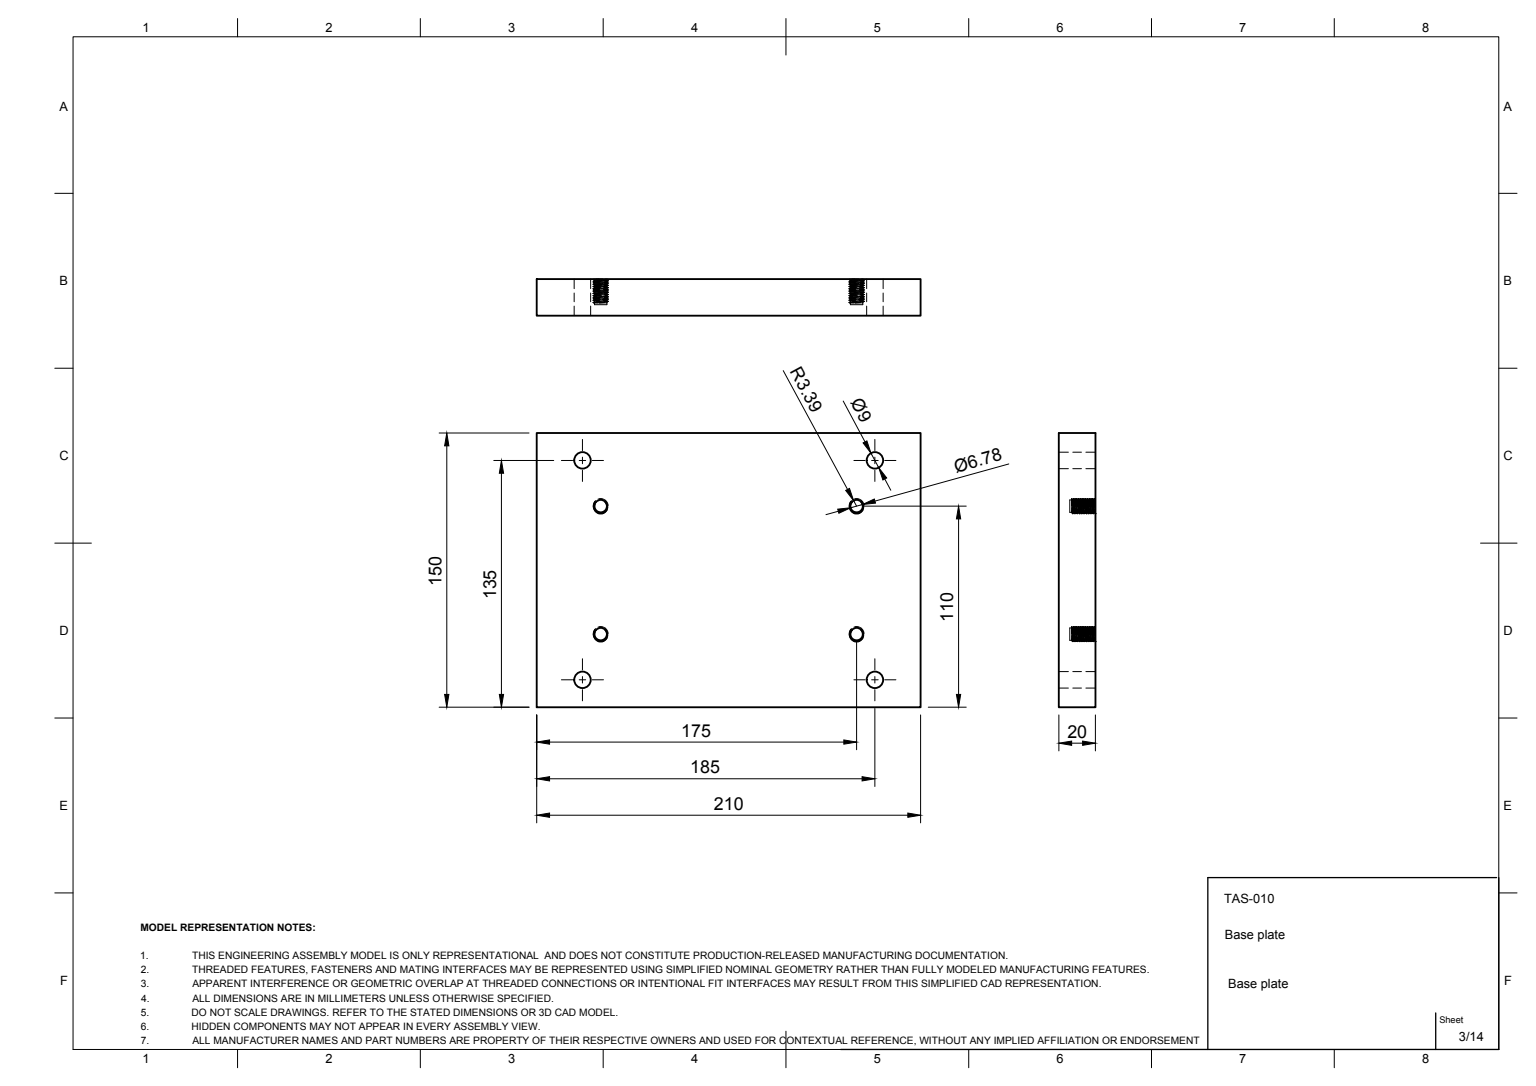
ISO-10303-21;
HEADER;
/* Generated by software containing ST-Developer
 * from STEP Tools, Inc. (www.steptools.com) 
 */

FILE_DESCRIPTION(
/* description */ (
'Independent keyed-quill tailstock, native coupled50mm slider andM16x2
 feed screw, conical dead center, bronze sleeves/thrust washers, cross
-pinned handwheel and bolted guide key. Custom center taper; no standa
rd taper compatibility, machine-bed compatibility or load rating assig
ned.'),
/* implementation_level */ '2;1');

FILE_NAME(
/* name */ 'Base plate.step',
/* time_stamp */ '2026-11-14T07:17:36-08:00',
/* author */ (''),
/* organization */ (''),
/* preprocessor_version */ 'ST-DEVELOPER v20.2',
/* originating_system */ 'Autodesk Translation Framework v15.17.0.0',
/* authorisation */ '');

FILE_SCHEMA (('AUTOMOTIVE_DESIGN { 1 0 10303 214 3 1 1 }'));
ENDSEC;

DATA;
#10=MECHANICAL_DESIGN_GEOMETRIC_PRESENTATION_REPRESENTATION('',(#153),#289387);
#119=SHAPE_REPRESENTATION_RELATIONSHIP('SRR','None',#289454,#136);
#136=ADVANCED_BREP_SHAPE_REPRESENTATION('',(#170),#289370);
#153=STYLED_ITEM('',(#289548),#170);
#170=MANIFOLD_SOLID_BREP('Body1',#16841);
#187=FACE_BOUND('',#1186,.T.);
#188=FACE_BOUND('',#1187,.T.);
#189=FACE_BOUND('',#1188,.T.);
#190=FACE_BOUND('',#1189,.T.);
#191=FACE_BOUND('',#1190,.T.);
#192=FACE_BOUND('',#1191,.T.);
#193=FACE_BOUND('',#1192,.T.);
#194=FACE_BOUND('',#1193,.T.);
#195=FACE_BOUND('',#1195,.T.);
#196=FACE_BOUND('',#1196,.T.);
#197=FACE_BOUND('',#1197,.T.);
#198=FACE_BOUND('',#1198,.T.);
#273=B_SPLINE_SURFACE_WITH_KNOTS('',3,3,((#55782,#55783,#55784,#55785,#55786,
#55787,#55788,#55789,#55790,#55791,#55792,#55793,#55794,#55795,#55796,#55797,
#55798,#55799,#55800,#55801,#55802,#55803,#55804,#55805,#55806,#55807,#55808,
#55809,#55810,#55811,#55812,#55813,#55814,#55815,#55816,#55817,#55818,#55819,
#55820,#55821,#55822,#55823,#55824,#55825,#55826,#55827,#55828,#55829,#55830,
#55831,#55832,#55833,#55834,#55835,#55836,#55837,#55838,#55839,#55840,#55841,
#55842,#55843,#55844,#55845,#55846,#55847,#55848,#55849,#55850,#55851,#55852),
(#55853,#55854,#55855,#55856,#55857,#55858,#55859,#55860,#55861,#55862,
#55863,#55864,#55865,#55866,#55867,#55868,#55869,#55870,#55871,#55872,#55873,
#55874,#55875,#55876,#55877,#55878,#55879,#55880,#55881,#55882,#55883,#55884,
#55885,#55886,#55887,#55888,#55889,#55890,#55891,#55892,#55893,#55894,#55895,
#55896,#55897,#55898,#55899,#55900,#55901,#55902,#55903,#55904,#55905,#55906,
#55907,#55908,#55909,#55910,#55911,#55912,#55913,#55914,#55915,#55916,#55917,
#55918,#55919,#55920,#55921,#55922,#55923),(#55924,#55925,#55926,#55927,
#55928,#55929,#55930,#55931,#55932,#55933,#55934,#55935,#55936,#55937,#55938,
#55939,#55940,#55941,#55942,#55943,#55944,#55945,#55946,#55947,#55948,#55949,
#55950,#55951,#55952,#55953,#55954,#55955,#55956,#55957,#55958,#55959,#55960,
#55961,#55962,#55963,#55964,#55965,#55966,#55967,#55968,#55969,#55970,#55971,
#55972,#55973,#55974,#55975,#55976,#55977,#55978,#55979,#55980,#55981,#55982,
#55983,#55984,#55985,#55986,#55987,#55988,#55989,#55990,#55991,#55992,#55993,
#55994),(#55995,#55996,#55997,#55998,#55999,#56000,#56001,#56002,#56003,
#56004,#56005,#56006,#56007,#56008,#56009,#56010,#56011,#56012,#56013,#56014,
#56015,#56016,#56017,#56018,#56019,#56020,#56021,#56022,#56023,#56024,#56025,
#56026,#56027,#56028,#56029,#56030,#56031,#56032,#56033,#56034,#56035,#56036,
#56037,#56038,#56039,#56040,#56041,#56042,#56043,#56044,#56045,#56046,#56047,
#56048,#56049,#56050,#56051,#56052,#56053,#56054,#56055,#56056,#56057,#56058,
#56059,#56060,#56061,#56062,#56063,#56064,#56065)),.UNSPECIFIED.,.F.,.F.,
 .F.,(4,4),(4,1,1,1,1,1,1,1,1,1,1,1,1,1,1,1,1,1,1,1,1,1,1,1,1,1,1,1,1,1,
1,1,1,1,1,1,1,1,1,1,1,1,1,1,1,1,1,1,1,1,1,1,1,1,1,1,1,1,1,1,1,1,1,1,1,1,
1,1,4),(-0.000703873626500094,0.0807256881124021),(11.8568339491899,12.8481671993964,
13.8387965759765,14.8294259525565,15.8200553291365,16.8106847057165,17.8013140822966,
18.7919434588766,19.7825728354566,20.7732022120367,21.7638315886167,22.7544609651967,
23.7450903417767,24.7357197183568,25.7263490949368,26.7169784715168,27.7076078480968,
28.6982372246769,29.6888666012569,30.6794959778369,31.6701253544169,32.660754730997,
33.651384107577,34.642013484157,35.6326428607371,36.6232722373171,37.6139016138971,
38.6045309904771,39.5951603670572,40.5857897436372,41.5764191202172,42.5670484967972,
43.5576778733773,44.5483072499573,45.5389366265373,46.5295660031174,47.5201953796974,
48.5108247562774,49.5014541328574,50.4920835094375,51.4827128860175,52.4733422625975,
53.4639716391775,54.4546010157576,55.4452303923376,56.4358597689176,57.4264891454977,
58.4171185220777,59.4077478986577,60.3983772752377,61.3890066518178,62.3796360283978,
63.3702654049778,64.3608947815578,65.3515241581379,66.3421535347179,67.3327829112979,
68.3234122878779,69.314041664458,70.304671041038,71.295300417618,72.2859297941981,
73.2765591707781,74.2671885473581,75.2578179239381,76.2484473005182,77.2390766770982,
78.2297060536782,79.2203354302583),.UNSPECIFIED.);
#274=B_SPLINE_SURFACE_WITH_KNOTS('',3,3,((#56163,#56164,#56165,#56166,#56167,
#56168,#56169,#56170,#56171,#56172,#56173,#56174,#56175,#56176,#56177,#56178,
#56179,#56180,#56181,#56182,#56183,#56184,#56185,#56186,#56187,#56188,#56189,
#56190,#56191,#56192,#56193,#56194,#56195,#56196,#56197,#56198,#56199,#56200,
#56201,#56202,#56203,#56204,#56205,#56206,#56207,#56208,#56209,#56210,#56211,
#56212,#56213,#56214,#56215,#56216,#56217,#56218,#56219,#56220,#56221,#56222,
#56223,#56224,#56225,#56226,#56227,#56228,#56229,#56230,#56231,#56232,#56233),
(#56234,#56235,#56236,#56237,#56238,#56239,#56240,#56241,#56242,#56243,
#56244,#56245,#56246,#56247,#56248,#56249,#56250,#56251,#56252,#56253,#56254,
#56255,#56256,#56257,#56258,#56259,#56260,#56261,#56262,#56263,#56264,#56265,
#56266,#56267,#56268,#56269,#56270,#56271,#56272,#56273,#56274,#56275,#56276,
#56277,#56278,#56279,#56280,#56281,#56282,#56283,#56284,#56285,#56286,#56287,
#56288,#56289,#56290,#56291,#56292,#56293,#56294,#56295,#56296,#56297,#56298,
#56299,#56300,#56301,#56302,#56303,#56304),(#56305,#56306,#56307,#56308,
#56309,#56310,#56311,#56312,#56313,#56314,#56315,#56316,#56317,#56318,#56319,
#56320,#56321,#56322,#56323,#56324,#56325,#56326,#56327,#56328,#56329,#56330,
#56331,#56332,#56333,#56334,#56335,#56336,#56337,#56338,#56339,#56340,#56341,
#56342,#56343,#56344,#56345,#56346,#56347,#56348,#56349,#56350,#56351,#56352,
#56353,#56354,#56355,#56356,#56357,#56358,#56359,#56360,#56361,#56362,#56363,
#56364,#56365,#56366,#56367,#56368,#56369,#56370,#56371,#56372,#56373,#56374,
#56375),(#56376,#56377,#56378,#56379,#56380,#56381,#56382,#56383,#56384,
#56385,#56386,#56387,#56388,#56389,#56390,#56391,#56392,#56393,#56394,#56395,
#56396,#56397,#56398,#56399,#56400,#56401,#56402,#56403,#56404,#56405,#56406,
#56407,#56408,#56409,#56410,#56411,#56412,#56413,#56414,#56415,#56416,#56417,
#56418,#56419,#56420,#56421,#56422,#56423,#56424,#56425,#56426,#56427,#56428,
#56429,#56430,#56431,#56432,#56433,#56434,#56435,#56436,#56437,#56438,#56439,
#56440,#56441,#56442,#56443,#56444,#56445,#56446)),.UNSPECIFIED.,.F.,.F.,
 .F.,(4,4),(4,1,1,1,1,1,1,1,1,1,1,1,1,1,1,1,1,1,1,1,1,1,1,1,1,1,1,1,1,1,
1,1,1,1,1,1,1,1,1,1,1,1,1,1,1,1,1,1,1,1,1,1,1,1,1,1,1,1,1,1,1,1,1,1,1,1,
1,1,4),(-0.000445042829947342,0.0809843050226073),(14.3991256467175,15.3897550232976,
16.3803843998776,17.3710137764576,18.3616431530376,19.3522725296177,20.3429019061977,
21.3335312827777,22.3241606593577,23.3147900359378,24.3054194125178,25.2960487890978,
26.2866781656778,27.2773075422579,28.2679369188379,29.2585662954179,30.249195671998,
31.239825048578,32.230454425158,33.221083801738,34.2117131783181,35.2023425548981,
36.1929719314781,37.1836013080582,38.1742306846382,39.1648600612182,40.1554894377982,
41.1461188143783,42.1367481909583,43.1273775675383,44.1180069441183,45.1086363206984,
46.0992656972784,47.0898950738584,48.0805244504384,49.0711538270185,50.0617832035985,
51.0524125801785,52.0430419567586,53.0336713333386,54.0243007099186,55.0149300864986,
56.0055594630787,56.9961888396587,57.9868182162387,58.9774475928187,59.9680769693988,
60.9587063459788,61.9493357225588,62.9399650991389,63.9305944757189,64.9212238522989,
65.9118532288789,66.902482605459,67.893111982039,68.883741358619,69.8743707351991,
70.8650001117791,71.8556294883591,72.8462588649391,73.8368882415191,74.8275176180992,
75.8181469946792,76.8087763712592,77.7994057478393,78.7900351244193,79.7806645009993,
80.7712938775793,81.7626270042512),.UNSPECIFIED.);
#275=B_SPLINE_SURFACE_WITH_KNOTS('',3,3,((#56747,#56748,#56749,#56750,#56751,
#56752,#56753,#56754,#56755,#56756,#56757,#56758,#56759,#56760,#56761,#56762,
#56763,#56764,#56765,#56766,#56767,#56768,#56769,#56770,#56771,#56772,#56773,
#56774,#56775,#56776,#56777,#56778,#56779,#56780,#56781,#56782,#56783,#56784,
#56785,#56786,#56787,#56788,#56789,#56790,#56791,#56792,#56793,#56794,#56795,
#56796,#56797,#56798,#56799,#56800,#56801,#56802,#56803,#56804,#56805,#56806,
#56807,#56808,#56809,#56810,#56811,#56812,#56813,#56814,#56815,#56816,#56817),
(#56818,#56819,#56820,#56821,#56822,#56823,#56824,#56825,#56826,#56827,
#56828,#56829,#56830,#56831,#56832,#56833,#56834,#56835,#56836,#56837,#56838,
#56839,#56840,#56841,#56842,#56843,#56844,#56845,#56846,#56847,#56848,#56849,
#56850,#56851,#56852,#56853,#56854,#56855,#56856,#56857,#56858,#56859,#56860,
#56861,#56862,#56863,#56864,#56865,#56866,#56867,#56868,#56869,#56870,#56871,
#56872,#56873,#56874,#56875,#56876,#56877,#56878,#56879,#56880,#56881,#56882,
#56883,#56884,#56885,#56886,#56887,#56888),(#56889,#56890,#56891,#56892,
#56893,#56894,#56895,#56896,#56897,#56898,#56899,#56900,#56901,#56902,#56903,
#56904,#56905,#56906,#56907,#56908,#56909,#56910,#56911,#56912,#56913,#56914,
#56915,#56916,#56917,#56918,#56919,#56920,#56921,#56922,#56923,#56924,#56925,
#56926,#56927,#56928,#56929,#56930,#56931,#56932,#56933,#56934,#56935,#56936,
#56937,#56938,#56939,#56940,#56941,#56942,#56943,#56944,#56945,#56946,#56947,
#56948,#56949,#56950,#56951,#56952,#56953,#56954,#56955,#56956,#56957,#56958,
#56959),(#56960,#56961,#56962,#56963,#56964,#56965,#56966,#56967,#56968,
#56969,#56970,#56971,#56972,#56973,#56974,#56975,#56976,#56977,#56978,#56979,
#56980,#56981,#56982,#56983,#56984,#56985,#56986,#56987,#56988,#56989,#56990,
#56991,#56992,#56993,#56994,#56995,#56996,#56997,#56998,#56999,#57000,#57001,
#57002,#57003,#57004,#57005,#57006,#57007,#57008,#57009,#57010,#57011,#57012,
#57013,#57014,#57015,#57016,#57017,#57018,#57019,#57020,#57021,#57022,#57023,
#57024,#57025,#57026,#57027,#57028,#57029,#57030)),.UNSPECIFIED.,.F.,.F.,
 .F.,(4,4),(4,1,1,1,1,1,1,1,1,1,1,1,1,1,1,1,1,1,1,1,1,1,1,1,1,1,1,1,1,1,
1,1,1,1,1,1,1,1,1,1,1,1,1,1,1,1,1,1,1,1,1,1,1,1,1,1,1,1,1,1,1,1,1,1,1,1,
1,1,4),(-0.000689732099215623,0.0807182050540442),(11.8568480907172,12.8481671993964,
13.8387965759765,14.8294259525565,15.8200553291365,16.8106847057165,17.8013140822966,
18.7919434588766,19.7825728354566,20.7732022120367,21.7638315886167,22.7544609651967,
23.7450903417767,24.7357197183568,25.7263490949368,26.7169784715168,27.7076078480968,
28.6982372246769,29.6888666012569,30.6794959778369,31.6701253544169,32.660754730997,
33.651384107577,34.642013484157,35.6326428607371,36.6232722373171,37.6139016138971,
38.6045309904771,39.5951603670572,40.5857897436372,41.5764191202172,42.5670484967972,
43.5576778733773,44.5483072499573,45.5389366265373,46.5295660031174,47.5201953796974,
48.5108247562774,49.5014541328574,50.4920835094375,51.4827128860175,52.4733422625975,
53.4639716391775,54.4546010157576,55.4452303923376,56.4358597689176,57.4264891454977,
58.4171185220777,59.4077478986577,60.3983772752377,61.3890066518178,62.3796360283978,
63.3702654049778,64.3608947815578,65.3515241581379,66.3421535347179,67.3327829112979,
68.3234122878779,69.314041664458,70.304671041038,71.295300417618,72.2859297941981,
73.2765591707781,74.2671885473581,75.2578179239381,76.2484473005182,77.2390766770982,
78.2297060536782,79.2203354302583),.UNSPECIFIED.);
#276=B_SPLINE_SURFACE_WITH_KNOTS('',3,3,((#57125,#57126,#57127,#57128,#57129,
#57130,#57131,#57132,#57133,#57134,#57135,#57136,#57137,#57138,#57139,#57140,
#57141,#57142,#57143,#57144,#57145,#57146,#57147,#57148,#57149,#57150,#57151,
#57152,#57153,#57154,#57155,#57156,#57157,#57158,#57159,#57160,#57161,#57162,
#57163,#57164,#57165,#57166,#57167,#57168,#57169,#57170,#57171,#57172,#57173,
#57174,#57175,#57176,#57177,#57178,#57179,#57180,#57181,#57182,#57183,#57184,
#57185,#57186,#57187,#57188,#57189,#57190,#57191,#57192,#57193,#57194,#57195),
(#57196,#57197,#57198,#57199,#57200,#57201,#57202,#57203,#57204,#57205,
#57206,#57207,#57208,#57209,#57210,#57211,#57212,#57213,#57214,#57215,#57216,
#57217,#57218,#57219,#57220,#57221,#57222,#57223,#57224,#57225,#57226,#57227,
#57228,#57229,#57230,#57231,#57232,#57233,#57234,#57235,#57236,#57237,#57238,
#57239,#57240,#57241,#57242,#57243,#57244,#57245,#57246,#57247,#57248,#57249,
#57250,#57251,#57252,#57253,#57254,#57255,#57256,#57257,#57258,#57259,#57260,
#57261,#57262,#57263,#57264,#57265,#57266),(#57267,#57268,#57269,#57270,
#57271,#57272,#57273,#57274,#57275,#57276,#57277,#57278,#57279,#57280,#57281,
#57282,#57283,#57284,#57285,#57286,#57287,#57288,#57289,#57290,#57291,#57292,
#57293,#57294,#57295,#57296,#57297,#57298,#57299,#57300,#57301,#57302,#57303,
#57304,#57305,#57306,#57307,#57308,#57309,#57310,#57311,#57312,#57313,#57314,
#57315,#57316,#57317,#57318,#57319,#57320,#57321,#57322,#57323,#57324,#57325,
#57326,#57327,#57328,#57329,#57330,#57331,#57332,#57333,#57334,#57335,#57336,
#57337),(#57338,#57339,#57340,#57341,#57342,#57343,#57344,#57345,#57346,
#57347,#57348,#57349,#57350,#57351,#57352,#57353,#57354,#57355,#57356,#57357,
#57358,#57359,#57360,#57361,#57362,#57363,#57364,#57365,#57366,#57367,#57368,
#57369,#57370,#57371,#57372,#57373,#57374,#57375,#57376,#57377,#57378,#57379,
#57380,#57381,#57382,#57383,#57384,#57385,#57386,#57387,#57388,#57389,#57390,
#57391,#57392,#57393,#57394,#57395,#57396,#57397,#57398,#57399,#57400,#57401,
#57402,#57403,#57404,#57405,#57406,#57407,#57408)),.UNSPECIFIED.,.F.,.F.,
 .F.,(4,4),(4,1,1,1,1,1,1,1,1,1,1,1,1,1,1,1,1,1,1,1,1,1,1,1,1,1,1,1,1,1,
1,1,1,1,1,1,1,1,1,1,1,1,1,1,1,1,1,1,1,1,1,1,1,1,1,1,1,1,1,1,1,1,1,1,1,1,
1,1,4),(-0.000437656372986427,0.0809703040897196),(14.3991256467175,15.3897550232976,
16.3803843998776,17.3710137764576,18.3616431530376,19.3522725296177,20.3429019061977,
21.3335312827777,22.3241606593577,23.3147900359378,24.3054194125178,25.2960487890978,
26.2866781656779,27.2773075422579,28.2679369188379,29.2585662954179,30.249195671998,
31.239825048578,32.230454425158,33.221083801738,34.2117131783181,35.2023425548981,
36.1929719314781,37.1836013080582,38.1742306846382,39.1648600612182,40.1554894377982,
41.1461188143783,42.1367481909583,43.1273775675383,44.1180069441183,45.1086363206984,
46.0992656972784,47.0898950738584,48.0805244504385,49.0711538270185,50.0617832035985,
51.0524125801785,52.0430419567586,53.0336713333386,54.0243007099186,55.0149300864986,
56.0055594630787,56.9961888396587,57.9868182162387,58.9774475928188,59.9680769693988,
60.9587063459788,61.9493357225588,62.9399650991389,63.9305944757189,64.9212238522989,
65.911853228879,66.902482605459,67.893111982039,68.883741358619,69.8743707351991,
70.8650001117791,71.8556294883591,72.8462588649391,73.8368882415192,74.8275176180992,
75.8181469946792,76.8087763712593,77.7994057478393,78.7900351244193,79.7806645009993,
80.7712938775794,81.7626130033183),.UNSPECIFIED.);
#277=B_SPLINE_SURFACE_WITH_KNOTS('',3,3,((#57712,#57713,#57714,#57715,#57716,
#57717,#57718,#57719,#57720,#57721,#57722,#57723,#57724,#57725,#57726,#57727,
#57728,#57729,#57730,#57731,#57732,#57733,#57734,#57735,#57736,#57737,#57738,
#57739,#57740,#57741,#57742,#57743,#57744,#57745,#57746,#57747,#57748,#57749,
#57750,#57751,#57752,#57753,#57754,#57755,#57756,#57757,#57758,#57759,#57760,
#57761,#57762,#57763,#57764,#57765,#57766,#57767,#57768,#57769,#57770,#57771,
#57772,#57773,#57774,#57775,#57776,#57777,#57778,#57779,#57780,#57781,#57782),
(#57783,#57784,#57785,#57786,#57787,#57788,#57789,#57790,#57791,#57792,
#57793,#57794,#57795,#57796,#57797,#57798,#57799,#57800,#57801,#57802,#57803,
#57804,#57805,#57806,#57807,#57808,#57809,#57810,#57811,#57812,#57813,#57814,
#57815,#57816,#57817,#57818,#57819,#57820,#57821,#57822,#57823,#57824,#57825,
#57826,#57827,#57828,#57829,#57830,#57831,#57832,#57833,#57834,#57835,#57836,
#57837,#57838,#57839,#57840,#57841,#57842,#57843,#57844,#57845,#57846,#57847,
#57848,#57849,#57850,#57851,#57852,#57853),(#57854,#57855,#57856,#57857,
#57858,#57859,#57860,#57861,#57862,#57863,#57864,#57865,#57866,#57867,#57868,
#57869,#57870,#57871,#57872,#57873,#57874,#57875,#57876,#57877,#57878,#57879,
#57880,#57881,#57882,#57883,#57884,#57885,#57886,#57887,#57888,#57889,#57890,
#57891,#57892,#57893,#57894,#57895,#57896,#57897,#57898,#57899,#57900,#57901,
#57902,#57903,#57904,#57905,#57906,#57907,#57908,#57909,#57910,#57911,#57912,
#57913,#57914,#57915,#57916,#57917,#57918,#57919,#57920,#57921,#57922,#57923,
#57924),(#57925,#57926,#57927,#57928,#57929,#57930,#57931,#57932,#57933,
#57934,#57935,#57936,#57937,#57938,#57939,#57940,#57941,#57942,#57943,#57944,
#57945,#57946,#57947,#57948,#57949,#57950,#57951,#57952,#57953,#57954,#57955,
#57956,#57957,#57958,#57959,#57960,#57961,#57962,#57963,#57964,#57965,#57966,
#57967,#57968,#57969,#57970,#57971,#57972,#57973,#57974,#57975,#57976,#57977,
#57978,#57979,#57980,#57981,#57982,#57983,#57984,#57985,#57986,#57987,#57988,
#57989,#57990,#57991,#57992,#57993,#57994,#57995)),.UNSPECIFIED.,.F.,.F.,
 .F.,(4,4),(4,1,1,1,1,1,1,1,1,1,1,1,1,1,1,1,1,1,1,1,1,1,1,1,1,1,1,1,1,1,
1,1,1,1,1,1,1,1,1,1,1,1,1,1,1,1,1,1,1,1,1,1,1,1,1,1,1,1,1,1,1,1,1,1,1,1,
1,1,4),(-0.000703899666689691,0.0807257072263232),(11.8568339231497,12.8481671993964,
13.8387965759764,14.8294259525565,15.8200553291365,16.8106847057165,17.8013140822965,
18.7919434588766,19.7825728354566,20.7732022120366,21.7638315886167,22.7544609651967,
23.7450903417767,24.7357197183567,25.7263490949368,26.7169784715168,27.7076078480968,
28.6982372246768,29.6888666012569,30.6794959778369,31.6701253544169,32.660754730997,
33.651384107577,34.642013484157,35.632642860737,36.6232722373171,37.6139016138971,
38.6045309904771,39.5951603670571,40.5857897436372,41.5764191202172,42.5670484967972,
43.5576778733773,44.5483072499573,45.5389366265373,46.5295660031173,47.5201953796974,
48.5108247562774,49.5014541328574,50.4920835094374,51.4827128860175,52.4733422625975,
53.4639716391775,54.4546010157575,55.4452303923376,56.4358597689176,57.4264891454976,
58.4171185220777,59.4077478986577,60.3983772752377,61.3890066518177,62.3796360283978,
63.3702654049778,64.3608947815578,65.3515241581378,66.3421535347179,67.3327829112979,
68.3234122878779,69.314041664458,70.304671041038,71.295300417618,72.285929794198,
73.2765591707781,74.2671885473581,75.2578179239381,76.2484473005182,77.2390766770982,
78.2297060536782,79.2203354302582),.UNSPECIFIED.);
#278=B_SPLINE_SURFACE_WITH_KNOTS('',3,3,((#58093,#58094,#58095,#58096,#58097,
#58098,#58099,#58100,#58101,#58102,#58103,#58104,#58105,#58106,#58107,#58108,
#58109,#58110,#58111,#58112,#58113,#58114,#58115,#58116,#58117,#58118,#58119,
#58120,#58121,#58122,#58123,#58124,#58125,#58126,#58127,#58128,#58129,#58130,
#58131,#58132,#58133,#58134,#58135,#58136,#58137,#58138,#58139,#58140,#58141,
#58142,#58143,#58144,#58145,#58146,#58147,#58148,#58149,#58150,#58151,#58152,
#58153,#58154,#58155,#58156,#58157,#58158,#58159,#58160,#58161,#58162,#58163),
(#58164,#58165,#58166,#58167,#58168,#58169,#58170,#58171,#58172,#58173,
#58174,#58175,#58176,#58177,#58178,#58179,#58180,#58181,#58182,#58183,#58184,
#58185,#58186,#58187,#58188,#58189,#58190,#58191,#58192,#58193,#58194,#58195,
#58196,#58197,#58198,#58199,#58200,#58201,#58202,#58203,#58204,#58205,#58206,
#58207,#58208,#58209,#58210,#58211,#58212,#58213,#58214,#58215,#58216,#58217,
#58218,#58219,#58220,#58221,#58222,#58223,#58224,#58225,#58226,#58227,#58228,
#58229,#58230,#58231,#58232,#58233,#58234),(#58235,#58236,#58237,#58238,
#58239,#58240,#58241,#58242,#58243,#58244,#58245,#58246,#58247,#58248,#58249,
#58250,#58251,#58252,#58253,#58254,#58255,#58256,#58257,#58258,#58259,#58260,
#58261,#58262,#58263,#58264,#58265,#58266,#58267,#58268,#58269,#58270,#58271,
#58272,#58273,#58274,#58275,#58276,#58277,#58278,#58279,#58280,#58281,#58282,
#58283,#58284,#58285,#58286,#58287,#58288,#58289,#58290,#58291,#58292,#58293,
#58294,#58295,#58296,#58297,#58298,#58299,#58300,#58301,#58302,#58303,#58304,
#58305),(#58306,#58307,#58308,#58309,#58310,#58311,#58312,#58313,#58314,
#58315,#58316,#58317,#58318,#58319,#58320,#58321,#58322,#58323,#58324,#58325,
#58326,#58327,#58328,#58329,#58330,#58331,#58332,#58333,#58334,#58335,#58336,
#58337,#58338,#58339,#58340,#58341,#58342,#58343,#58344,#58345,#58346,#58347,
#58348,#58349,#58350,#58351,#58352,#58353,#58354,#58355,#58356,#58357,#58358,
#58359,#58360,#58361,#58362,#58363,#58364,#58365,#58366,#58367,#58368,#58369,
#58370,#58371,#58372,#58373,#58374,#58375,#58376)),.UNSPECIFIED.,.F.,.F.,
 .F.,(4,4),(4,1,1,1,1,1,1,1,1,1,1,1,1,1,1,1,1,1,1,1,1,1,1,1,1,1,1,1,1,1,
1,1,1,1,1,1,1,1,1,1,1,1,1,1,1,1,1,1,1,1,1,1,1,1,1,1,1,1,1,1,1,1,1,1,1,1,
1,1,4),(-0.000445070994418236,0.080984343609613),(14.3991256467175,15.3897550232975,
16.3803843998776,17.3710137764576,18.3616431530376,19.3522725296176,20.3429019061977,
21.3335312827777,22.3241606593577,23.3147900359377,24.3054194125178,25.2960487890978,
26.2866781656778,27.2773075422579,28.2679369188379,29.2585662954179,30.2491956719979,
31.239825048578,32.230454425158,33.221083801738,34.211713178318,35.2023425548981,
36.1929719314781,37.1836013080581,38.1742306846382,39.1648600612182,40.1554894377982,
41.1461188143782,42.1367481909583,43.1273775675383,44.1180069441183,45.1086363206983,
46.0992656972784,47.0898950738584,48.0805244504384,49.0711538270185,50.0617832035985,
51.0524125801785,52.0430419567585,53.0336713333386,54.0243007099186,55.0149300864986,
56.0055594630786,56.9961888396587,57.9868182162387,58.9774475928187,59.9680769693988,
60.9587063459788,61.9493357225588,62.9399650991388,63.9305944757189,64.9212238522989,
65.9118532288789,66.9024826054589,67.893111982039,68.883741358619,69.874370735199,
70.8650001117791,71.8556294883591,72.8462588649391,73.8368882415191,74.8275176180992,
75.8181469946792,76.8087763712592,77.7994057478392,78.7900351244193,79.7806645009993,
80.7712938775793,81.7626270428382),.UNSPECIFIED.);
#279=B_SPLINE_SURFACE_WITH_KNOTS('',3,3,((#58677,#58678,#58679,#58680,#58681,
#58682,#58683,#58684,#58685,#58686,#58687,#58688,#58689,#58690,#58691,#58692,
#58693,#58694,#58695,#58696,#58697,#58698,#58699,#58700,#58701,#58702,#58703,
#58704,#58705,#58706,#58707,#58708,#58709,#58710,#58711,#58712,#58713,#58714,
#58715,#58716,#58717,#58718,#58719,#58720,#58721,#58722,#58723,#58724,#58725,
#58726,#58727,#58728,#58729,#58730,#58731,#58732,#58733,#58734,#58735,#58736,
#58737,#58738,#58739,#58740,#58741,#58742,#58743,#58744,#58745,#58746,#58747),
(#58748,#58749,#58750,#58751,#58752,#58753,#58754,#58755,#58756,#58757,
#58758,#58759,#58760,#58761,#58762,#58763,#58764,#58765,#58766,#58767,#58768,
#58769,#58770,#58771,#58772,#58773,#58774,#58775,#58776,#58777,#58778,#58779,
#58780,#58781,#58782,#58783,#58784,#58785,#58786,#58787,#58788,#58789,#58790,
#58791,#58792,#58793,#58794,#58795,#58796,#58797,#58798,#58799,#58800,#58801,
#58802,#58803,#58804,#58805,#58806,#58807,#58808,#58809,#58810,#58811,#58812,
#58813,#58814,#58815,#58816,#58817,#58818),(#58819,#58820,#58821,#58822,
#58823,#58824,#58825,#58826,#58827,#58828,#58829,#58830,#58831,#58832,#58833,
#58834,#58835,#58836,#58837,#58838,#58839,#58840,#58841,#58842,#58843,#58844,
#58845,#58846,#58847,#58848,#58849,#58850,#58851,#58852,#58853,#58854,#58855,
#58856,#58857,#58858,#58859,#58860,#58861,#58862,#58863,#58864,#58865,#58866,
#58867,#58868,#58869,#58870,#58871,#58872,#58873,#58874,#58875,#58876,#58877,
#58878,#58879,#58880,#58881,#58882,#58883,#58884,#58885,#58886,#58887,#58888,
#58889),(#58890,#58891,#58892,#58893,#58894,#58895,#58896,#58897,#58898,
#58899,#58900,#58901,#58902,#58903,#58904,#58905,#58906,#58907,#58908,#58909,
#58910,#58911,#58912,#58913,#58914,#58915,#58916,#58917,#58918,#58919,#58920,
#58921,#58922,#58923,#58924,#58925,#58926,#58927,#58928,#58929,#58930,#58931,
#58932,#58933,#58934,#58935,#58936,#58937,#58938,#58939,#58940,#58941,#58942,
#58943,#58944,#58945,#58946,#58947,#58948,#58949,#58950,#58951,#58952,#58953,
#58954,#58955,#58956,#58957,#58958,#58959,#58960)),.UNSPECIFIED.,.F.,.F.,
 .F.,(4,4),(4,1,1,1,1,1,1,1,1,1,1,1,1,1,1,1,1,1,1,1,1,1,1,1,1,1,1,1,1,1,
1,1,1,1,1,1,1,1,1,1,1,1,1,1,1,1,1,1,1,1,1,1,1,1,1,1,1,1,1,1,1,1,1,1,1,1,
1,1,4),(-0.00068967791227708,0.0807181852368366),(11.8568481449041,12.8481671993964,
13.8387965759765,14.8294259525565,15.8200553291365,16.8106847057165,17.8013140822966,
18.7919434588766,19.7825728354566,20.7732022120367,21.7638315886167,22.7544609651967,
23.7450903417767,24.7357197183568,25.7263490949368,26.7169784715168,27.7076078480968,
28.6982372246769,29.6888666012569,30.6794959778369,31.6701253544169,32.660754730997,
33.651384107577,34.642013484157,35.6326428607371,36.6232722373171,37.6139016138971,
38.6045309904771,39.5951603670572,40.5857897436372,41.5764191202172,42.5670484967972,
43.5576778733773,44.5483072499573,45.5389366265373,46.5295660031174,47.5201953796974,
48.5108247562774,49.5014541328574,50.4920835094375,51.4827128860175,52.4733422625975,
53.4639716391775,54.4546010157576,55.4452303923376,56.4358597689176,57.4264891454977,
58.4171185220777,59.4077478986577,60.3983772752377,61.3890066518178,62.3796360283978,
63.3702654049778,64.3608947815578,65.3515241581379,66.3421535347179,67.3327829112979,
68.3234122878779,69.314041664458,70.304671041038,71.295300417618,72.2859297941981,
73.2765591707781,74.2671885473581,75.2578179239381,76.2484473005182,77.2390766770982,
78.2297060536782,79.2203354302583),.UNSPECIFIED.);
#280=B_SPLINE_SURFACE_WITH_KNOTS('',3,3,((#59055,#59056,#59057,#59058,#59059,
#59060,#59061,#59062,#59063,#59064,#59065,#59066,#59067,#59068,#59069,#59070,
#59071,#59072,#59073,#59074,#59075,#59076,#59077,#59078,#59079,#59080,#59081,
#59082,#59083,#59084,#59085,#59086,#59087,#59088,#59089,#59090,#59091,#59092,
#59093,#59094,#59095,#59096,#59097,#59098,#59099,#59100,#59101,#59102,#59103,
#59104,#59105,#59106,#59107,#59108,#59109,#59110,#59111,#59112,#59113,#59114,
#59115,#59116,#59117,#59118,#59119,#59120,#59121,#59122,#59123,#59124,#59125),
(#59126,#59127,#59128,#59129,#59130,#59131,#59132,#59133,#59134,#59135,
#59136,#59137,#59138,#59139,#59140,#59141,#59142,#59143,#59144,#59145,#59146,
#59147,#59148,#59149,#59150,#59151,#59152,#59153,#59154,#59155,#59156,#59157,
#59158,#59159,#59160,#59161,#59162,#59163,#59164,#59165,#59166,#59167,#59168,
#59169,#59170,#59171,#59172,#59173,#59174,#59175,#59176,#59177,#59178,#59179,
#59180,#59181,#59182,#59183,#59184,#59185,#59186,#59187,#59188,#59189,#59190,
#59191,#59192,#59193,#59194,#59195,#59196),(#59197,#59198,#59199,#59200,
#59201,#59202,#59203,#59204,#59205,#59206,#59207,#59208,#59209,#59210,#59211,
#59212,#59213,#59214,#59215,#59216,#59217,#59218,#59219,#59220,#59221,#59222,
#59223,#59224,#59225,#59226,#59227,#59228,#59229,#59230,#59231,#59232,#59233,
#59234,#59235,#59236,#59237,#59238,#59239,#59240,#59241,#59242,#59243,#59244,
#59245,#59246,#59247,#59248,#59249,#59250,#59251,#59252,#59253,#59254,#59255,
#59256,#59257,#59258,#59259,#59260,#59261,#59262,#59263,#59264,#59265,#59266,
#59267),(#59268,#59269,#59270,#59271,#59272,#59273,#59274,#59275,#59276,
#59277,#59278,#59279,#59280,#59281,#59282,#59283,#59284,#59285,#59286,#59287,
#59288,#59289,#59290,#59291,#59292,#59293,#59294,#59295,#59296,#59297,#59298,
#59299,#59300,#59301,#59302,#59303,#59304,#59305,#59306,#59307,#59308,#59309,
#59310,#59311,#59312,#59313,#59314,#59315,#59316,#59317,#59318,#59319,#59320,
#59321,#59322,#59323,#59324,#59325,#59326,#59327,#59328,#59329,#59330,#59331,
#59332,#59333,#59334,#59335,#59336,#59337,#59338)),.UNSPECIFIED.,.F.,.F.,
 .F.,(4,4),(4,1,1,1,1,1,1,1,1,1,1,1,1,1,1,1,1,1,1,1,1,1,1,1,1,1,1,1,1,1,
1,1,1,1,1,1,1,1,1,1,1,1,1,1,1,1,1,1,1,1,1,1,1,1,1,1,1,1,1,1,1,1,1,1,1,1,
1,1,4),(-0.00043763828538554,0.0809702546783821),(14.3991256467175,15.3897550232976,
16.3803843998776,17.3710137764576,18.3616431530376,19.3522725296177,20.3429019061977,
21.3335312827777,22.3241606593577,23.3147900359378,24.3054194125178,25.2960487890978,
26.2866781656779,27.2773075422579,28.2679369188379,29.2585662954179,30.249195671998,
31.239825048578,32.230454425158,33.221083801738,34.2117131783181,35.2023425548981,
36.1929719314781,37.1836013080582,38.1742306846382,39.1648600612182,40.1554894377982,
41.1461188143783,42.1367481909583,43.1273775675383,44.1180069441183,45.1086363206984,
46.0992656972784,47.0898950738584,48.0805244504385,49.0711538270185,50.0617832035985,
51.0524125801785,52.0430419567586,53.0336713333386,54.0243007099186,55.0149300864986,
56.0055594630787,56.9961888396587,57.9868182162387,58.9774475928188,59.9680769693988,
60.9587063459788,61.9493357225588,62.9399650991389,63.9305944757189,64.9212238522989,
65.911853228879,66.902482605459,67.893111982039,68.883741358619,69.8743707351991,
70.8650001117791,71.8556294883591,72.8462588649391,73.8368882415192,74.8275176180992,
75.8181469946792,76.8087763712593,77.7994057478393,78.7900351244193,79.7806645009993,
80.7712938775794,81.7626129539069),.UNSPECIFIED.);
#303=PLANE('',#17160);
#304=PLANE('',#17161);
#305=PLANE('',#17162);
#306=PLANE('',#17163);
#307=PLANE('',#17164);
#308=PLANE('',#17165);
#309=PLANE('',#17166);
#310=PLANE('',#17167);
#311=PLANE('',#17180);
#312=PLANE('',#17181);
#313=PLANE('',#17182);
#314=PLANE('',#17183);
#315=PLANE('',#17184);
#316=PLANE('',#17185);
#423=FACE_OUTER_BOUND('',#1073,.T.);
#424=FACE_OUTER_BOUND('',#1074,.T.);
#425=FACE_OUTER_BOUND('',#1075,.T.);
#426=FACE_OUTER_BOUND('',#1076,.T.);
#427=FACE_OUTER_BOUND('',#1077,.T.);
#428=FACE_OUTER_BOUND('',#1078,.T.);
#429=FACE_OUTER_BOUND('',#1079,.T.);
#430=FACE_OUTER_BOUND('',#1080,.T.);
#431=FACE_OUTER_BOUND('',#1081,.T.);
#432=FACE_OUTER_BOUND('',#1082,.T.);
#433=FACE_OUTER_BOUND('',#1083,.T.);
#434=FACE_OUTER_BOUND('',#1084,.T.);
#435=FACE_OUTER_BOUND('',#1085,.T.);
#436=FACE_OUTER_BOUND('',#1086,.T.);
#437=FACE_OUTER_BOUND('',#1087,.T.);
#438=FACE_OUTER_BOUND('',#1088,.T.);
#439=FACE_OUTER_BOUND('',#1089,.T.);
#440=FACE_OUTER_BOUND('',#1090,.T.);
#441=FACE_OUTER_BOUND('',#1091,.T.);
#442=FACE_OUTER_BOUND('',#1092,.T.);
#443=FACE_OUTER_BOUND('',#1093,.T.);
#444=FACE_OUTER_BOUND('',#1094,.T.);
#445=FACE_OUTER_BOUND('',#1095,.T.);
#446=FACE_OUTER_BOUND('',#1096,.T.);
#447=FACE_OUTER_BOUND('',#1097,.T.);
#448=FACE_OUTER_BOUND('',#1098,.T.);
#449=FACE_OUTER_BOUND('',#1099,.T.);
#450=FACE_OUTER_BOUND('',#1100,.T.);
#451=FACE_OUTER_BOUND('',#1101,.T.);
#452=FACE_OUTER_BOUND('',#1102,.T.);
#453=FACE_OUTER_BOUND('',#1103,.T.);
#454=FACE_OUTER_BOUND('',#1104,.T.);
#455=FACE_OUTER_BOUND('',#1105,.T.);
#456=FACE_OUTER_BOUND('',#1106,.T.);
#457=FACE_OUTER_BOUND('',#1107,.T.);
#458=FACE_OUTER_BOUND('',#1108,.T.);
#459=FACE_OUTER_BOUND('',#1109,.T.);
#460=FACE_OUTER_BOUND('',#1110,.T.);
#461=FACE_OUTER_BOUND('',#1111,.T.);
#462=FACE_OUTER_BOUND('',#1112,.T.);
#463=FACE_OUTER_BOUND('',#1113,.T.);
#464=FACE_OUTER_BOUND('',#1114,.T.);
#465=FACE_OUTER_BOUND('',#1115,.T.);
#466=FACE_OUTER_BOUND('',#1116,.T.);
#467=FACE_OUTER_BOUND('',#1117,.T.);
#468=FACE_OUTER_BOUND('',#1118,.T.);
#469=FACE_OUTER_BOUND('',#1119,.T.);
#470=FACE_OUTER_BOUND('',#1120,.T.);
#471=FACE_OUTER_BOUND('',#1121,.T.);
#472=FACE_OUTER_BOUND('',#1122,.T.);
#473=FACE_OUTER_BOUND('',#1123,.T.);
#474=FACE_OUTER_BOUND('',#1124,.T.);
#475=FACE_OUTER_BOUND('',#1125,.T.);
#476=FACE_OUTER_BOUND('',#1126,.T.);
#477=FACE_OUTER_BOUND('',#1127,.T.);
#478=FACE_OUTER_BOUND('',#1128,.T.);
#479=FACE_OUTER_BOUND('',#1129,.T.);
#480=FACE_OUTER_BOUND('',#1130,.T.);
#481=FACE_OUTER_BOUND('',#1131,.T.);
#482=FACE_OUTER_BOUND('',#1132,.T.);
#483=FACE_OUTER_BOUND('',#1133,.T.);
#484=FACE_OUTER_BOUND('',#1134,.T.);
#485=FACE_OUTER_BOUND('',#1135,.T.);
#486=FACE_OUTER_BOUND('',#1136,.T.);
#487=FACE_OUTER_BOUND('',#1137,.T.);
#488=FACE_OUTER_BOUND('',#1138,.T.);
#489=FACE_OUTER_BOUND('',#1139,.T.);
#490=FACE_OUTER_BOUND('',#1140,.T.);
#491=FACE_OUTER_BOUND('',#1141,.T.);
#492=FACE_OUTER_BOUND('',#1142,.T.);
#493=FACE_OUTER_BOUND('',#1143,.T.);
#494=FACE_OUTER_BOUND('',#1144,.T.);
#495=FACE_OUTER_BOUND('',#1145,.T.);
#496=FACE_OUTER_BOUND('',#1146,.T.);
#497=FACE_OUTER_BOUND('',#1147,.T.);
#498=FACE_OUTER_BOUND('',#1148,.T.);
#499=FACE_OUTER_BOUND('',#1149,.T.);
#500=FACE_OUTER_BOUND('',#1150,.T.);
#501=FACE_OUTER_BOUND('',#1151,.T.);
#502=FACE_OUTER_BOUND('',#1152,.T.);
#503=FACE_OUTER_BOUND('',#1153,.T.);
#504=FACE_OUTER_BOUND('',#1154,.T.);
#505=FACE_OUTER_BOUND('',#1155,.T.);
#506=FACE_OUTER_BOUND('',#1156,.T.);
#507=FACE_OUTER_BOUND('',#1157,.T.);
#508=FACE_OUTER_BOUND('',#1158,.T.);
#509=FACE_OUTER_BOUND('',#1159,.T.);
#510=FACE_OUTER_BOUND('',#1160,.T.);
#511=FACE_OUTER_BOUND('',#1161,.T.);
#512=FACE_OUTER_BOUND('',#1162,.T.);
#513=FACE_OUTER_BOUND('',#1163,.T.);
#514=FACE_OUTER_BOUND('',#1164,.T.);
#515=FACE_OUTER_BOUND('',#1165,.T.);
#516=FACE_OUTER_BOUND('',#1166,.T.);
#517=FACE_OUTER_BOUND('',#1167,.T.);
#518=FACE_OUTER_BOUND('',#1168,.T.);
#519=FACE_OUTER_BOUND('',#1169,.T.);
#520=FACE_OUTER_BOUND('',#1170,.T.);
#521=FACE_OUTER_BOUND('',#1171,.T.);
#522=FACE_OUTER_BOUND('',#1172,.T.);
#523=FACE_OUTER_BOUND('',#1173,.T.);
#524=FACE_OUTER_BOUND('',#1174,.T.);
#525=FACE_OUTER_BOUND('',#1175,.T.);
#526=FACE_OUTER_BOUND('',#1176,.T.);
#527=FACE_OUTER_BOUND('',#1177,.T.);
#528=FACE_OUTER_BOUND('',#1178,.T.);
#529=FACE_OUTER_BOUND('',#1179,.T.);
#530=FACE_OUTER_BOUND('',#1180,.T.);
#531=FACE_OUTER_BOUND('',#1181,.T.);
#532=FACE_OUTER_BOUND('',#1182,.T.);
#533=FACE_OUTER_BOUND('',#1183,.T.);
#534=FACE_OUTER_BOUND('',#1184,.T.);
#535=FACE_OUTER_BOUND('',#1185,.T.);
#536=FACE_OUTER_BOUND('',#1194,.T.);
#1073=EDGE_LOOP('',(#10161,#10162,#10163,#10164,#10165,#10166));
#1074=EDGE_LOOP('',(#10167,#10168,#10169,#10170,#10171,#10172));
#1075=EDGE_LOOP('',(#10173,#10174,#10175,#10176,#10177,#10178));
#1076=EDGE_LOOP('',(#10179,#10180,#10181,#10182,#10183,#10184));
#1077=EDGE_LOOP('',(#10185,#10186,#10187,#10188,#10189,#10190));
#1078=EDGE_LOOP('',(#10191,#10192,#10193,#10194,#10195,#10196));
#1079=EDGE_LOOP('',(#10197,#10198,#10199,#10200,#10201,#10202));
#1080=EDGE_LOOP('',(#10203,#10204,#10205,#10206,#10207,#10208));
#1081=EDGE_LOOP('',(#10209,#10210,#10211,#10212,#10213,#10214));
#1082=EDGE_LOOP('',(#10215,#10216,#10217,#10218,#10219,#10220));
#1083=EDGE_LOOP('',(#10221,#10222,#10223,#10224,#10225,#10226,#10227,#10228));
#1084=EDGE_LOOP('',(#10229,#10230,#10231,#10232,#10233));
#1085=EDGE_LOOP('',(#10234,#10235,#10236,#10237,#10238));
#1086=EDGE_LOOP('',(#10239,#10240,#10241,#10242,#10243));
#1087=EDGE_LOOP('',(#10244,#10245,#10246,#10247,#10248));
#1088=EDGE_LOOP('',(#10249,#10250,#10251,#10252,#10253));
#1089=EDGE_LOOP('',(#10254,#10255,#10256,#10257,#10258));
#1090=EDGE_LOOP('',(#10259,#10260,#10261,#10262,#10263));
#1091=EDGE_LOOP('',(#10264,#10265,#10266,#10267,#10268));
#1092=EDGE_LOOP('',(#10269,#10270,#10271,#10272));
#1093=EDGE_LOOP('',(#10273,#10274,#10275,#10276,#10277,#10278));
#1094=EDGE_LOOP('',(#10279,#10280,#10281,#10282,#10283,#10284));
#1095=EDGE_LOOP('',(#10285,#10286,#10287,#10288,#10289,#10290));
#1096=EDGE_LOOP('',(#10291,#10292,#10293,#10294,#10295,#10296));
#1097=EDGE_LOOP('',(#10297,#10298,#10299,#10300,#10301,#10302));
#1098=EDGE_LOOP('',(#10303,#10304,#10305,#10306,#10307,#10308));
#1099=EDGE_LOOP('',(#10309,#10310,#10311,#10312,#10313,#10314));
#1100=EDGE_LOOP('',(#10315,#10316,#10317,#10318,#10319,#10320));
#1101=EDGE_LOOP('',(#10321,#10322,#10323,#10324,#10325,#10326));
#1102=EDGE_LOOP('',(#10327,#10328,#10329,#10330,#10331,#10332));
#1103=EDGE_LOOP('',(#10333,#10334,#10335,#10336,#10337,#10338,#10339,#10340));
#1104=EDGE_LOOP('',(#10341,#10342,#10343,#10344,#10345));
#1105=EDGE_LOOP('',(#10346,#10347,#10348,#10349,#10350));
#1106=EDGE_LOOP('',(#10351,#10352,#10353,#10354,#10355));
#1107=EDGE_LOOP('',(#10356,#10357,#10358,#10359,#10360));
#1108=EDGE_LOOP('',(#10361,#10362,#10363,#10364,#10365));
#1109=EDGE_LOOP('',(#10366,#10367,#10368,#10369,#10370));
#1110=EDGE_LOOP('',(#10371,#10372,#10373,#10374,#10375));
#1111=EDGE_LOOP('',(#10376,#10377,#10378,#10379,#10380));
#1112=EDGE_LOOP('',(#10381,#10382,#10383,#10384));
#1113=EDGE_LOOP('',(#10385,#10386,#10387,#10388,#10389,#10390));
#1114=EDGE_LOOP('',(#10391,#10392,#10393,#10394,#10395,#10396));
#1115=EDGE_LOOP('',(#10397,#10398,#10399,#10400,#10401,#10402));
#1116=EDGE_LOOP('',(#10403,#10404,#10405,#10406,#10407,#10408));
#1117=EDGE_LOOP('',(#10409,#10410,#10411,#10412,#10413,#10414));
#1118=EDGE_LOOP('',(#10415,#10416,#10417,#10418,#10419,#10420));
#1119=EDGE_LOOP('',(#10421,#10422,#10423,#10424,#10425,#10426));
#1120=EDGE_LOOP('',(#10427,#10428,#10429,#10430,#10431,#10432));
#1121=EDGE_LOOP('',(#10433,#10434,#10435,#10436,#10437,#10438));
#1122=EDGE_LOOP('',(#10439,#10440,#10441,#10442,#10443,#10444));
#1123=EDGE_LOOP('',(#10445,#10446,#10447,#10448,#10449,#10450,#10451,#10452));
#1124=EDGE_LOOP('',(#10453,#10454,#10455,#10456,#10457));
#1125=EDGE_LOOP('',(#10458,#10459,#10460,#10461,#10462));
#1126=EDGE_LOOP('',(#10463,#10464,#10465,#10466,#10467));
#1127=EDGE_LOOP('',(#10468,#10469,#10470,#10471,#10472));
#1128=EDGE_LOOP('',(#10473,#10474,#10475,#10476,#10477));
#1129=EDGE_LOOP('',(#10478,#10479,#10480,#10481,#10482));
#1130=EDGE_LOOP('',(#10483,#10484,#10485,#10486,#10487));
#1131=EDGE_LOOP('',(#10488,#10489,#10490,#10491,#10492));
#1132=EDGE_LOOP('',(#10493,#10494,#10495,#10496));
#1133=EDGE_LOOP('',(#10497,#10498,#10499,#10500,#10501,#10502));
#1134=EDGE_LOOP('',(#10503,#10504,#10505,#10506,#10507,#10508));
#1135=EDGE_LOOP('',(#10509,#10510,#10511,#10512,#10513,#10514));
#1136=EDGE_LOOP('',(#10515,#10516,#10517,#10518,#10519,#10520));
#1137=EDGE_LOOP('',(#10521,#10522,#10523,#10524,#10525,#10526));
#1138=EDGE_LOOP('',(#10527,#10528,#10529,#10530,#10531,#10532));
#1139=EDGE_LOOP('',(#10533,#10534,#10535,#10536,#10537,#10538));
#1140=EDGE_LOOP('',(#10539,#10540,#10541,#10542,#10543,#10544));
#1141=EDGE_LOOP('',(#10545,#10546,#10547,#10548,#10549,#10550));
#1142=EDGE_LOOP('',(#10551,#10552,#10553,#10554,#10555,#10556));
#1143=EDGE_LOOP('',(#10557,#10558,#10559,#10560,#10561,#10562,#10563,#10564));
#1144=EDGE_LOOP('',(#10565,#10566,#10567,#10568,#10569));
#1145=EDGE_LOOP('',(#10570,#10571,#10572,#10573,#10574));
#1146=EDGE_LOOP('',(#10575,#10576,#10577,#10578,#10579));
#1147=EDGE_LOOP('',(#10580,#10581,#10582,#10583,#10584));
#1148=EDGE_LOOP('',(#10585,#10586,#10587,#10588,#10589));
#1149=EDGE_LOOP('',(#10590,#10591,#10592,#10593,#10594));
#1150=EDGE_LOOP('',(#10595,#10596,#10597,#10598,#10599));
#1151=EDGE_LOOP('',(#10600,#10601,#10602,#10603,#10604));
#1152=EDGE_LOOP('',(#10605,#10606,#10607,#10608));
#1153=EDGE_LOOP('',(#10609,#10610,#10611,#10612,#10613,#10614));
#1154=EDGE_LOOP('',(#10615,#10616,#10617,#10618,#10619,#10620));
#1155=EDGE_LOOP('',(#10621,#10622,#10623,#10624,#10625,#10626));
#1156=EDGE_LOOP('',(#10627,#10628,#10629,#10630,#10631,#10632));
#1157=EDGE_LOOP('',(#10633,#10634,#10635,#10636,#10637,#10638));
#1158=EDGE_LOOP('',(#10639,#10640,#10641,#10642,#10643,#10644));
#1159=EDGE_LOOP('',(#10645,#10646,#10647,#10648,#10649,#10650));
#1160=EDGE_LOOP('',(#10651,#10652,#10653,#10654,#10655,#10656));
#1161=EDGE_LOOP('',(#10657,#10658,#10659,#10660,#10661));
#1162=EDGE_LOOP('',(#10662,#10663,#10664,#10665,#10666,#10667,#10668,#10669,
#10670,#10671,#10672,#10673,#10674,#10675,#10676,#10677,#10678,#10679,#10680,
#10681,#10682,#10683,#10684,#10685,#10686,#10687,#10688,#10689,#10690,#10691,
#10692,#10693,#10694,#10695,#10696,#10697,#10698,#10699,#10700,#10701));
#1163=EDGE_LOOP('',(#10702,#10703,#10704,#10705,#10706,#10707,#10708,#10709,
#10710,#10711,#10712,#10713,#10714,#10715,#10716,#10717,#10718,#10719,#10720,
#10721,#10722,#10723,#10724,#10725,#10726,#10727,#10728,#10729,#10730,#10731,
#10732,#10733,#10734,#10735,#10736,#10737,#10738,#10739,#10740,#10741,#10742));
#1164=EDGE_LOOP('',(#10743,#10744,#10745,#10746,#10747));
#1165=EDGE_LOOP('',(#10748,#10749,#10750,#10751,#10752,#10753,#10754,#10755,
#10756,#10757,#10758,#10759,#10760,#10761,#10762,#10763,#10764,#10765,#10766,
#10767,#10768,#10769,#10770,#10771,#10772,#10773,#10774,#10775,#10776,#10777,
#10778,#10779,#10780,#10781,#10782,#10783,#10784,#10785,#10786,#10787));
#1166=EDGE_LOOP('',(#10788,#10789,#10790,#10791,#10792,#10793,#10794,#10795,
#10796,#10797,#10798,#10799,#10800,#10801,#10802,#10803,#10804,#10805,#10806,
#10807,#10808,#10809,#10810,#10811,#10812,#10813,#10814,#10815,#10816,#10817,
#10818,#10819,#10820,#10821,#10822,#10823,#10824,#10825,#10826,#10827,#10828));
#1167=EDGE_LOOP('',(#10829,#10830,#10831,#10832,#10833));
#1168=EDGE_LOOP('',(#10834,#10835,#10836,#10837,#10838,#10839,#10840,#10841,
#10842,#10843,#10844,#10845,#10846,#10847,#10848,#10849,#10850,#10851,#10852,
#10853,#10854,#10855,#10856,#10857,#10858,#10859,#10860,#10861,#10862,#10863,
#10864,#10865,#10866,#10867,#10868,#10869,#10870,#10871,#10872,#10873));
#1169=EDGE_LOOP('',(#10874,#10875,#10876,#10877,#10878,#10879,#10880,#10881,
#10882,#10883,#10884,#10885,#10886,#10887,#10888,#10889,#10890,#10891,#10892,
#10893,#10894,#10895,#10896,#10897,#10898,#10899,#10900,#10901,#10902,#10903,
#10904,#10905,#10906,#10907,#10908,#10909,#10910,#10911,#10912,#10913,#10914));
#1170=EDGE_LOOP('',(#10915,#10916,#10917,#10918,#10919));
#1171=EDGE_LOOP('',(#10920,#10921,#10922,#10923,#10924,#10925,#10926,#10927,
#10928,#10929,#10930,#10931,#10932,#10933,#10934,#10935,#10936,#10937,#10938,
#10939,#10940,#10941,#10942,#10943,#10944,#10945,#10946,#10947,#10948,#10949,
#10950,#10951,#10952,#10953,#10954,#10955,#10956,#10957,#10958,#10959));
#1172=EDGE_LOOP('',(#10960,#10961,#10962,#10963,#10964,#10965,#10966,#10967,
#10968,#10969,#10970,#10971,#10972,#10973,#10974,#10975,#10976,#10977,#10978,
#10979,#10980,#10981,#10982,#10983,#10984,#10985,#10986,#10987,#10988,#10989,
#10990,#10991,#10992,#10993,#10994,#10995,#10996,#10997,#10998,#10999,#11000));
#1173=EDGE_LOOP('',(#11001));
#1174=EDGE_LOOP('',(#11002));
#1175=EDGE_LOOP('',(#11003));
#1176=EDGE_LOOP('',(#11004));
#1177=EDGE_LOOP('',(#11005,#11006,#11007,#11008));
#1178=EDGE_LOOP('',(#11009,#11010,#11011,#11012));
#1179=EDGE_LOOP('',(#11013,#11014,#11015,#11016));
#1180=EDGE_LOOP('',(#11017,#11018,#11019,#11020));
#1181=EDGE_LOOP('',(#11021,#11022,#11023,#11024));
#1182=EDGE_LOOP('',(#11025,#11026,#11027,#11028));
#1183=EDGE_LOOP('',(#11029,#11030,#11031,#11032));
#1184=EDGE_LOOP('',(#11033,#11034,#11035,#11036));
#1185=EDGE_LOOP('',(#11037,#11038,#11039,#11040));
#1186=EDGE_LOOP('',(#11041,#11042,#11043,#11044,#11045));
#1187=EDGE_LOOP('',(#11046,#11047,#11048,#11049,#11050));
#1188=EDGE_LOOP('',(#11051));
#1189=EDGE_LOOP('',(#11052));
#1190=EDGE_LOOP('',(#11053));
#1191=EDGE_LOOP('',(#11054));
#1192=EDGE_LOOP('',(#11055,#11056,#11057,#11058,#11059));
#1193=EDGE_LOOP('',(#11060,#11061,#11062,#11063,#11064));
#1194=EDGE_LOOP('',(#11065,#11066,#11067,#11068));
#1195=EDGE_LOOP('',(#11069));
#1196=EDGE_LOOP('',(#11070));
#1197=EDGE_LOOP('',(#11071));
#1198=EDGE_LOOP('',(#11072));
#1809=CIRCLE('',#17049,4.085);
#1810=CIRCLE('',#17059,4.085);
#1811=CIRCLE('',#17061,3.38975);
#1812=CIRCLE('',#17062,3.38975);
#1813=CIRCLE('',#17063,3.38975);
#1814=CIRCLE('',#17073,3.38975);
#1815=CIRCLE('',#17075,4.085);
#1816=CIRCLE('',#17085,4.085);
#1817=CIRCLE('',#17087,3.38975);
#1818=CIRCLE('',#17088,3.38975);
#1819=CIRCLE('',#17089,3.38975);
#1820=CIRCLE('',#17099,3.38975);
#1821=CIRCLE('',#17101,4.085);
#1822=CIRCLE('',#17111,4.085);
#1823=CIRCLE('',#17113,3.38975);
#1824=CIRCLE('',#17114,3.38975);
#1825=CIRCLE('',#17115,3.38975);
#1826=CIRCLE('',#17125,3.38975);
#1827=CIRCLE('',#17127,4.085);
#1828=CIRCLE('',#17137,4.085);
#1829=CIRCLE('',#17139,3.38975);
#1830=CIRCLE('',#17140,3.38975);
#1831=CIRCLE('',#17141,3.38975);
#1832=CIRCLE('',#17151,3.38975);
#1833=CIRCLE('',#17169,4.5);
#1834=CIRCLE('',#17170,4.5);
#1835=CIRCLE('',#17172,4.5);
#1836=CIRCLE('',#17173,4.5);
#1837=CIRCLE('',#17175,4.5);
#1838=CIRCLE('',#17176,4.5);
#1839=CIRCLE('',#17178,4.5);
#1840=CIRCLE('',#17179,4.5);
#1989=B_SPLINE_CURVE_WITH_KNOTS('',3,(#20219,#20220,#20221,#20222,#20223,
#20224,#20225,#20226,#20227,#20228,#20229,#20230,#20231,#20232,#20233,#20234,
#20235,#20236,#20237,#20238,#20239,#20240,#20241,#20242,#20243,#20244,#20245,
#20246,#20247,#20248,#20249,#20250,#20251,#20252,#20253,#20254,#20255,#20256,
#20257,#20258,#20259,#20260,#20261,#20262,#20263,#20264,#20265,#20266,#20267,
#20268,#20269,#20270,#20271,#20272,#20273,#20274,#20275,#20276,#20277,#20278,
#20279,#20280,#20281,#20282,#20283,#20284,#20285,#20286,#20287,#20288,#20289,
#20290,#20291,#20292,#20293,#20294,#20295,#20296,#20297,#20298,#20299,#20300,
#20301,#20302,#20303,#20304,#20305,#20306,#20307,#20308,#20309,#20310,#20311,
#20312,#20313,#20314,#20315,#20316,#20317,#20318,#20319,#20320,#20321,#20322,
#20323,#20324,#20325,#20326,#20327,#20328,#20329,#20330,#20331,#20332,#20333,
#20334,#20335,#20336,#20337,#20338,#20339,#20340,#20341,#20342,#20343,#20344,
#20345,#20346,#20347,#20348,#20349,#20350,#20351,#20352,#20353,#20354,#20355,
#20356,#20357,#20358,#20359,#20360,#20361,#20362,#20363),.UNSPECIFIED.,
 .F.,.F.,(4,3,3,3,3,3,3,3,3,3,3,3,3,3,3,3,3,3,3,3,3,3,3,3,3,3,3,3,3,3,3,
3,3,3,3,3,3,3,3,3,3,3,3,3,3,3,3,3,4),(74.4826090335725,74.5701170669696,
74.6575762165587,74.7450105784093,74.8324408957047,74.9198879037736,75.0074269134415,
75.0950130962531,75.1827404978775,75.2578179239381,75.3457798849692,75.4336308010057,
75.5213935021216,75.6122752269211,75.6999373474644,75.7875855687495,75.8752403914981,
75.962922316007,76.0506986045304,76.1385311052508,76.2264862371109,76.2484473005182,
76.3362730397008,76.4239894702698,76.5116195619046,76.6025517013038,76.6900866998096,
76.7776100410487,76.8651423567182,76.9527042798826,77.0403648632325,77.1280840300195,
77.2159301399878,77.2390766770982,77.3262112033101,77.4132347402867,77.5001710454324,
77.5913629214631,77.6782061467429,77.7650395395892,77.8518844243916,77.9387621301685,
78.0257467155559,78.1127937623897,78.199978776898,78.2297060536782,78.3409628987117,
78.4504383987289,78.5398161890533),.UNSPECIFIED.);
#1990=B_SPLINE_CURVE_WITH_KNOTS('',3,(#20365,#20366,#20367,#20368),
 .UNSPECIFIED.,.F.,.F.,(4,4),(78.5398163397448,79.2203354302583),
 .UNSPECIFIED.);
#1991=B_SPLINE_CURVE_WITH_KNOTS('',3,(#20372,#20373,#20374,#20375,#20376,
#20377,#20378,#20379,#20380,#20381,#20382,#20383,#20384,#20385,#20386,#20387,
#20388,#20389,#20390,#20391,#20392,#20393,#20394,#20395,#20396,#20397,#20398,
#20399,#20400,#20401,#20402,#20403,#20404,#20405,#20406,#20407,#20408,#20409,
#20410,#20411,#20412,#20413,#20414),.UNSPECIFIED.,.F.,.F.,(4,3,3,3,3,3,
3,3,3,3,3,3,3,3,4),(78.5398163399586,78.6513081866131,78.7649916437635,
78.7900351244193,78.8773287774196,78.9645133671013,79.0516124728846,79.1386521216673,
79.2256605320351,79.3126588903471,79.3996683708265,79.4867645491849,79.5739037704035,
79.6611841726733,79.7442522064414),.UNSPECIFIED.);
#1992=B_SPLINE_CURVE_WITH_KNOTS('',3,(#20415,#20416,#20417,#20418,#20419,
#20420,#20421,#20422,#20423,#20424,#20425,#20426,#20427,#20428,#20429,#20430,
#20431,#20432,#20433,#20434,#20435,#20436,#20437,#20438,#20439,#20440,#20441,
#20442,#20443,#20444,#20445,#20446,#20447,#20448,#20449,#20450,#20451,#20452,
#20453,#20454,#20455,#20456,#20457,#20458,#20459,#20460,#20461,#20462,#20463,
#20464,#20465,#20466,#20467,#20468,#20469,#20470,#20471,#20472,#20473,#20474,
#20475,#20476,#20477,#20478,#20479,#20480,#20481,#20482,#20483,#20484,#20485,
#20486,#20487,#20488,#20489,#20490,#20491,#20492,#20493,#20494,#20495,#20496,
#20497,#20498,#20499,#20500,#20501,#20502,#20503,#20504,#20505,#20506,#20507,
#20508,#20509,#20510,#20511,#20512,#20513,#20514,#20515,#20516,#20517,#20518,
#20519,#20520,#20521,#20522,#20523,#20524,#20525,#20526,#20527,#20528,#20529,
#20530,#20531,#20532,#20533,#20534,#20535,#20536,#20537,#20538,#20539,#20540,
#20541,#20542,#20543,#20544,#20545,#20546,#20547,#20548,#20549,#20550,#20551,
#20552,#20553,#20554,#20555,#20556,#20557,#20558,#20559,#20560,#20561,#20562),
 .UNSPECIFIED.,.F.,.F.,(4,3,3,3,3,3,3,3,3,3,3,3,3,3,3,3,3,3,3,3,3,3,3,3,
3,3,3,3,3,3,3,3,3,3,3,3,3,3,3,3,3,3,3,3,3,3,3,3,3,4),(74.4816274087652,
74.5692304822722,74.6568785799873,74.7446691313286,74.8275176180992,74.9153495028009,
75.0030705517629,75.0907037488907,75.1816341546142,75.2691685016855,75.3566898130181,
75.4442187278137,75.531775885644,75.6194297201104,75.7071409756895,75.7949775432399,
75.8181469946792,75.9059726632625,75.9936877005556,76.0813150947037,76.1722477542731,
76.2597768495321,76.3472931203132,76.4348172103102,76.5223697637486,76.6100193409493,
76.6977265363025,76.785559361159,76.8087763712592,76.8965156836257,76.9841440069646,
77.0716844351596,77.1626495992445,77.2500916523099,77.3375210019096,77.4249583849954,
77.5124245392801,77.5999886071116,77.6876107096917,77.7753597026586,77.7994057478393,
77.8864293135118,77.9733148215533,78.0601212169649,78.1468700360845,78.2335827631578,
78.3203031262511,78.4070268007935,78.4938095091331,78.5398163397448),
 .UNSPECIFIED.);
#1993=B_SPLINE_CURVE_WITH_KNOTS('',3,(#20568,#20569,#20570,#20571,#20572,
#20573,#20574,#20575,#20576,#20577,#20578,#20579,#20580,#20581,#20582,#20583,
#20584,#20585,#20586,#20587,#20588,#20589,#20590,#20591,#20592,#20593,#20594,
#20595,#20596,#20597,#20598,#20599,#20600,#20601,#20602,#20603,#20604,#20605,
#20606,#20607,#20608,#20609,#20610,#20611,#20612,#20613,#20614,#20615,#20616,
#20617,#20618,#20619,#20620,#20621,#20622,#20623,#20624,#20625,#20626,#20627,
#20628,#20629,#20630,#20631,#20632,#20633,#20634,#20635,#20636,#20637,#20638,
#20639,#20640,#20641,#20642,#20643,#20644,#20645,#20646,#20647,#20648,#20649,
#20650,#20651,#20652,#20653,#20654,#20655,#20656,#20657,#20658,#20659,#20660,
#20661,#20662,#20663,#20664,#20665,#20666,#20667,#20668,#20669,#20670,#20671,
#20672,#20673,#20674,#20675,#20676,#20677,#20678,#20679,#20680,#20681,#20682,
#20683,#20684,#20685,#20686,#20687,#20688,#20689,#20690,#20691,#20692,#20693,
#20694,#20695,#20696,#20697,#20698,#20699,#20700,#20701,#20702,#20703,#20704,
#20705,#20706,#20707,#20708,#20709,#20710,#20711,#20712,#20713,#20714,#20715),
 .UNSPECIFIED.,.F.,.F.,(4,3,3,3,3,3,3,3,3,3,3,3,3,3,3,3,3,3,3,3,3,3,3,3,
3,3,3,3,3,3,3,3,3,3,3,3,3,3,3,3,3,3,3,3,3,3,3,3,3,4),(68.1983639736923,
68.2861814027768,68.3234122878779,68.4112289331686,68.4989347821535,68.5865528361021,
68.6774889396466,68.7650083795268,68.8525148961314,68.9400291443268,69.0275717794539,
69.1152113763737,69.2029085438011,69.2907313485085,69.314041664458,69.4018606984001,
69.4895689314358,69.5771893620946,69.6681245719626,69.755646355417,69.8431551993798,
69.9306717562514,70.0182166788918,70.1058585206193,70.19355791062,70.2813828885069,
70.304671041038,70.3924904087626,70.4801989997041,70.5678198116346,70.6587548873826,
70.7462771072879,70.8337864071766,70.9213034388543,71.0088488545995,71.0964912138051,
71.184191136065,71.2720166636101,71.295300417618,71.3826886082915,71.4699662262677,
71.5571567686942,71.6445910516527,71.731686798181,71.8187708746251,71.9058643773058,
71.9935560410698,72.0807764618647,72.1687037471133,72.2566310323619),
 .UNSPECIFIED.);
#1994=B_SPLINE_CURVE_WITH_KNOTS('',3,(#20716,#20717,#20718,#20719,#20720,
#20721,#20722,#20723,#20724,#20725,#20726,#20727,#20728,#20729,#20730,#20731,
#20732,#20733,#20734,#20735,#20736,#20737,#20738,#20739,#20740,#20741,#20742,
#20743,#20744,#20745,#20746,#20747,#20748,#20749,#20750,#20751,#20752,#20753,
#20754,#20755,#20756,#20757,#20758,#20759,#20760,#20761,#20762,#20763,#20764,
#20765,#20766,#20767,#20768,#20769,#20770,#20771,#20772,#20773,#20774,#20775,
#20776,#20777,#20778,#20779,#20780,#20781,#20782,#20783,#20784,#20785,#20786,
#20787,#20788,#20789,#20790,#20791,#20792,#20793,#20794,#20795,#20796,#20797,
#20798,#20799,#20800),.UNSPECIFIED.,.F.,.F.,(4,3,3,3,3,3,3,3,3,3,3,3,3,
3,3,3,3,3,3,3,3,3,3,3,3,3,3,3,4),(72.2566310325652,72.2859297941981,72.3737616647174,
72.4614826996036,72.5491158827769,72.640046293777,72.7275806272787,72.8151019252055,
72.9026308267726,72.9901879715657,73.0778417933396,73.1655530364124,73.2533895918213,
73.2765591707781,73.3643847882656,73.4520997741813,73.5397271167352,73.6306597955631,
73.7181888390195,73.8057050580113,73.8932290962889,73.9807815981339,74.068431124189,
74.1561382685975,74.2439710431921,74.2671885473581,74.3549358239911,74.4425594684545,
74.4826090335725),.UNSPECIFIED.);
#1995=B_SPLINE_CURVE_WITH_KNOTS('',3,(#20802,#20803,#20804,#20805,#20806,
#20807,#20808,#20809,#20810,#20811,#20812,#20813,#20814,#20815,#20816,#20817,
#20818,#20819,#20820,#20821,#20822,#20823,#20824,#20825,#20826,#20827,#20828,
#20829,#20830,#20831,#20832,#20833,#20834,#20835,#20836,#20837,#20838,#20839,
#20840,#20841,#20842,#20843,#20844,#20845,#20846,#20847,#20848,#20849,#20850,
#20851,#20852,#20853,#20854,#20855,#20856,#20857,#20858,#20859,#20860,#20861,
#20862,#20863,#20864,#20865,#20866,#20867,#20868,#20869,#20870,#20871,#20872,
#20873,#20874,#20875,#20876,#20877,#20878,#20879,#20880,#20881,#20882,#20883),
 .UNSPECIFIED.,.F.,.F.,(4,3,3,3,3,3,3,3,3,3,3,3,3,3,3,3,3,3,3,3,3,3,3,3,
3,3,3,4),(72.2566310325652,72.3454126124315,72.4342219267591,72.5230774207564,
72.6120589912192,72.7011092478249,72.7903164501228,72.8462588649391,72.9340782408894,
73.0217868401024,73.1094076603398,73.2003427329872,73.2878649612343,73.3753742694632,
73.4628913094705,73.5504367335256,73.63807910097,73.725779031437,73.8136045670799,
73.8368882415191,73.924681465638,74.0123709321393,74.0999774797657,74.1875218796041,
74.2750311973064,74.362520405566,74.4500269116099,74.4816274087652),
 .UNSPECIFIED.);
#1996=B_SPLINE_CURVE_WITH_KNOTS('',3,(#20884,#20885,#20886,#20887,#20888,
#20889,#20890,#20891,#20892,#20893,#20894,#20895,#20896,#20897,#20898,#20899,
#20900,#20901,#20902,#20903,#20904,#20905,#20906,#20907,#20908,#20909,#20910,
#20911,#20912,#20913,#20914,#20915,#20916,#20917,#20918,#20919,#20920,#20921,
#20922,#20923,#20924,#20925,#20926,#20927,#20928,#20929,#20930,#20931,#20932,
#20933,#20934,#20935,#20936,#20937,#20938,#20939,#20940,#20941,#20942,#20943,
#20944,#20945,#20946,#20947,#20948,#20949,#20950,#20951,#20952,#20953,#20954,
#20955,#20956,#20957,#20958,#20959,#20960,#20961,#20962,#20963,#20964,#20965,
#20966,#20967,#20968,#20969,#20970,#20971,#20972,#20973,#20974,#20975,#20976,
#20977,#20978,#20979,#20980,#20981,#20982,#20983,#20984,#20985,#20986,#20987,
#20988,#20989,#20990,#20991,#20992,#20993,#20994,#20995,#20996,#20997,#20998,
#20999,#21000,#21001,#21002,#21003,#21004,#21005,#21006,#21007,#21008,#21009,
#21010,#21011,#21012,#21013,#21014,#21015,#21016,#21017,#21018,#21019,#21020,
#21021,#21022,#21023,#21024,#21025,#21026,#21027,#21028,#21029,#21030,#21031),
 .UNSPECIFIED.,.F.,.F.,(4,3,3,3,3,3,3,3,3,3,3,3,3,3,3,3,3,3,3,3,3,3,3,3,
3,3,3,3,3,3,3,3,3,3,3,3,3,3,3,3,3,3,3,3,3,3,3,3,3,4),(68.1993401913434,
68.2868763835785,68.3743883543492,68.4618967634435,68.5494222631017,68.6370391881809,
68.7247035247109,68.8125067513156,68.883741358619,68.9715591938061,69.0592662331119,
69.1468854764006,69.2378211337504,69.3253417530268,69.4128494433357,69.5003648582877,
69.5879086519626,69.6755493894878,69.763247688409,69.8510716026728,69.8743707351991,
69.9621887255292,70.0498959227571,70.1375153265216,70.2284509246788,70.3159717097113,
70.4034795674247,70.4909951512383,70.5785391150419,70.6661800236928,70.7538784945183,
70.8417025804987,70.8650001117791,70.9528167537017,71.0405225993166,71.1281406498969,
71.2190767547046,71.3065961912421,71.3941027045195,71.4816169494061,71.569159581247,
71.6567991749293,71.7444963391443,71.8323191406998,71.8556294883591,71.9558798743633,
72.0526975273649,72.1492455770458,72.2453959286712,72.256631032376),
 .UNSPECIFIED.);
#1997=B_SPLINE_CURVE_WITH_KNOTS('',3,(#21037,#21038,#21039,#21040,#21041,
#21042,#21043,#21044,#21045,#21046,#21047,#21048,#21049,#21050,#21051,#21052,
#21053,#21054,#21055,#21056,#21057,#21058,#21059,#21060,#21061,#21062,#21063,
#21064,#21065,#21066,#21067,#21068,#21069,#21070,#21071,#21072,#21073,#21074,
#21075,#21076,#21077,#21078,#21079,#21080,#21081,#21082,#21083,#21084,#21085,
#21086,#21087,#21088,#21089,#21090,#21091,#21092,#21093,#21094,#21095,#21096,
#21097,#21098,#21099,#21100,#21101,#21102,#21103,#21104,#21105,#21106,#21107,
#21108,#21109,#21110,#21111,#21112,#21113,#21114,#21115,#21116,#21117,#21118,
#21119,#21120,#21121,#21122,#21123,#21124,#21125,#21126,#21127,#21128,#21129,
#21130,#21131,#21132,#21133,#21134,#21135,#21136,#21137,#21138,#21139,#21140,
#21141,#21142,#21143,#21144,#21145,#21146,#21147,#21148,#21149,#21150,#21151,
#21152,#21153,#21154,#21155,#21156,#21157,#21158,#21159,#21160,#21161,#21162,
#21163,#21164,#21165,#21166,#21167,#21168,#21169,#21170,#21171,#21172,#21173,
#21174,#21175,#21176,#21177,#21178,#21179,#21180,#21181,#21182,#21183,#21184),
 .UNSPECIFIED.,.F.,.F.,(4,3,3,3,3,3,3,3,3,3,3,3,3,3,3,3,3,3,3,3,3,3,3,3,
3,3,3,3,3,3,3,3,3,3,3,3,3,3,3,3,3,3,3,3,3,3,3,3,3,4),(61.9155759069306,
62.0030907077314,62.0906332894479,62.1782725403716,62.2659688151231,62.3537913799992,
62.3796360283978,62.467453738876,62.5551606542545,62.642779774532,62.7337154783378,
62.8212359776401,62.9087435492969,62.9962588470419,63.0838025250797,63.1714431498601,
63.2591413375884,63.3469651437694,63.3702654049778,63.4580831367133,63.5457900732474,
63.6334092145556,63.7243449104309,63.8118654303222,63.8993730223703,63.986888340288,
64.0744320382573,64.162072682515,64.249770889479,64.337594714396,64.3608947815578,
64.4487125433212,64.5364195101921,64.6240386821059,64.7149743666099,64.8024949175758,
64.8900025408166,64.9775178900099,65.0650616193034,65.1527022947983,65.2404005329847,
65.3282243888632,65.3515241581379,65.4399938083171,65.5283489317369,65.6166094520782,
65.705818520405,65.7939460921638,65.8836959087747,65.9734457253856),
 .UNSPECIFIED.);
#1998=B_SPLINE_CURVE_WITH_KNOTS('',3,(#21185,#21186,#21187,#21188,#21189,
#21190,#21191,#21192,#21193,#21194,#21195,#21196,#21197,#21198,#21199,#21200,
#21201,#21202,#21203,#21204,#21205,#21206,#21207,#21208,#21209,#21210,#21211,
#21212,#21213,#21214,#21215,#21216,#21217,#21218,#21219,#21220,#21221,#21222,
#21223,#21224,#21225,#21226,#21227,#21228,#21229,#21230,#21231,#21232,#21233,
#21234,#21235,#21236,#21237,#21238,#21239,#21240,#21241,#21242,#21243,#21244,
#21245,#21246,#21247,#21248,#21249,#21250,#21251,#21252,#21253,#21254,#21255,
#21256,#21257,#21258,#21259,#21260,#21261,#21262,#21263),.UNSPECIFIED.,
 .F.,.F.,(4,3,3,3,3,3,3,3,3,3,3,3,3,3,3,3,3,3,3,3,3,3,3,3,3,3,4),(65.9734457255974,
66.0719666577025,66.1708766449107,66.2703103694164,66.3421535347179,66.4299713697137,
66.5176784088316,66.6052976519356,66.6962333093559,66.7837539284567,66.8712616185937,
66.9587770333778,67.0463208268888,67.1339615642567,67.2216598630244,67.3094837771413,
67.3327829112979,67.4206084666378,67.5083214326648,67.5959318437032,67.6834846166537,
67.7710004523481,67.8585000197182,67.9460405122724,68.033599715588,68.1212547564394,
68.1983639736923),.UNSPECIFIED.);
#1999=B_SPLINE_CURVE_WITH_KNOTS('',3,(#21265,#21266,#21267,#21268,#21269,
#21270,#21271,#21272,#21273,#21274,#21275,#21276,#21277,#21278,#21279,#21280,
#21281,#21282,#21283,#21284,#21285,#21286,#21287,#21288,#21289,#21290,#21291,
#21292,#21293,#21294,#21295,#21296,#21297,#21298,#21299,#21300,#21301,#21302,
#21303,#21304,#21305,#21306,#21307,#21308,#21309,#21310,#21311,#21312,#21313,
#21314,#21315,#21316,#21317,#21318,#21319,#21320,#21321,#21322,#21323,#21324,
#21325,#21326,#21327,#21328,#21329,#21330,#21331,#21332,#21333,#21334,#21335,
#21336,#21337,#21338,#21339,#21340,#21341,#21342,#21343,#21344,#21345,#21346),
 .UNSPECIFIED.,.F.,.F.,(4,3,3,3,3,3,3,3,3,3,3,3,3,3,3,3,3,3,3,3,3,3,3,3,
3,3,3,4),(65.9734457255662,66.0604573171653,66.1473630253179,66.2341866877522,
66.3209558483152,66.4076973522101,66.4944326209606,66.5811830669334,66.6680217727008,
66.7549076097697,66.8419276275401,66.902482605459,66.9903003674263,67.0780073345023,
67.1656265066219,67.2565621910491,67.3440827422207,67.4315903656668,67.5191057150651,
67.6066494445629,67.6942901202597,67.7819883586472,67.8698122147238,67.893111982039,
67.9809173626158,68.0686254649819,68.1562390275125,68.1993401913434),
 .UNSPECIFIED.);
#2000=B_SPLINE_CURVE_WITH_KNOTS('',3,(#21347,#21348,#21349,#21350,#21351,
#21352,#21353,#21354,#21355,#21356,#21357,#21358,#21359,#21360,#21361,#21362,
#21363,#21364,#21365,#21366,#21367,#21368,#21369,#21370,#21371,#21372,#21373,
#21374,#21375,#21376,#21377,#21378,#21379,#21380,#21381,#21382,#21383,#21384,
#21385,#21386,#21387,#21388,#21389,#21390,#21391,#21392,#21393,#21394,#21395,
#21396,#21397,#21398,#21399,#21400,#21401,#21402,#21403,#21404,#21405,#21406,
#21407,#21408,#21409,#21410,#21411,#21412,#21413,#21414,#21415,#21416,#21417,
#21418,#21419,#21420,#21421,#21422,#21423,#21424,#21425,#21426,#21427,#21428,
#21429,#21430,#21431,#21432,#21433,#21434,#21435,#21436,#21437,#21438,#21439,
#21440,#21441,#21442,#21443,#21444,#21445,#21446,#21447,#21448,#21449,#21450,
#21451,#21452,#21453,#21454,#21455,#21456,#21457,#21458,#21459,#21460,#21461,
#21462,#21463,#21464,#21465,#21466,#21467,#21468,#21469,#21470,#21471,#21472,
#21473,#21474,#21475,#21476,#21477,#21478,#21479,#21480,#21481,#21482,#21483,
#21484,#21485,#21486,#21487,#21488,#21489,#21490,#21491,#21492,#21493,#21494,
#21495,#21496,#21497),.UNSPECIFIED.,.F.,.F.,(4,3,3,3,3,3,3,3,3,3,3,3,3,
3,3,3,3,3,3,3,3,3,3,3,3,3,3,3,3,3,3,3,3,3,3,3,3,3,3,3,3,3,3,3,3,3,3,3,3,
3,4),(61.9154863879853,61.9493357225588,62.0371534448199,62.1248603719797,
62.2124795040232,62.3034152034126,62.3909357143681,62.4784432976163,62.5659586068789,
62.6535022963475,62.741142932374,62.8288411312538,62.9166649483632,62.9399650991389,
63.0277828231756,63.1154897520975,63.2031088858876,63.2940445846165,63.3815650972695,
63.4690726821944,63.5565879931111,63.6441316842093,63.7317723218213,63.8194705222627,
63.9072943408872,63.9305944757189,64.018412204507,64.1061191382139,64.1937382768165,
64.2846739737518,64.3721944912548,64.4597020810347,64.5472173968066,64.6347610927545,
64.7224017351837,64.8100999404289,64.8979237638009,64.9212238522989,65.0090415627175,
65.0967484780368,65.1843675982553,65.2753033020833,65.3628238013271,65.4503313729256,
65.537846670613,65.6253903485929,65.7130309733168,65.800729160989,65.8885529671151,
65.9118532288789,65.9734457253856),.UNSPECIFIED.);
#2001=B_SPLINE_CURVE_WITH_KNOTS('',3,(#21503,#21504,#21505,#21506,#21507,
#21508,#21509,#21510,#21511,#21512,#21513,#21514,#21515,#21516,#21517,#21518,
#21519,#21520,#21521,#21522,#21523,#21524,#21525,#21526,#21527,#21528,#21529,
#21530,#21531,#21532,#21533,#21534,#21535,#21536,#21537,#21538,#21539,#21540,
#21541,#21542,#21543,#21544,#21545,#21546,#21547,#21548,#21549,#21550,#21551,
#21552,#21553,#21554,#21555,#21556,#21557,#21558,#21559,#21560,#21561,#21562,
#21563,#21564,#21565,#21566,#21567,#21568,#21569,#21570,#21571,#21572,#21573,
#21574,#21575,#21576,#21577,#21578,#21579,#21580,#21581,#21582,#21583,#21584,
#21585,#21586,#21587,#21588,#21589,#21590,#21591,#21592,#21593,#21594,#21595,
#21596,#21597,#21598,#21599,#21600,#21601,#21602,#21603,#21604,#21605,#21606,
#21607,#21608,#21609,#21610,#21611,#21612,#21613,#21614,#21615,#21616,#21617,
#21618,#21619,#21620,#21621,#21622,#21623,#21624,#21625,#21626,#21627,#21628,
#21629,#21630,#21631,#21632,#21633,#21634,#21635,#21636,#21637,#21638,#21639,
#21640,#21641,#21642,#21643,#21644,#21645,#21646,#21647,#21648,#21649,#21650),
 .UNSPECIFIED.,.F.,.F.,(4,3,3,3,3,3,3,3,3,3,3,3,3,3,3,3,3,3,3,3,3,3,3,3,
3,3,3,3,3,3,3,3,3,3,3,3,3,3,3,3,3,3,3,3,3,3,3,3,3,4),(55.6330521042359,
55.7206607554735,55.810060632154,55.8975784438563,55.9850858650237,56.0726035486431,
56.1634176037117,56.2510662026952,56.3387753400529,56.4266064512809,56.4358597689176,
56.5236774924357,56.6113844208514,56.6990035541482,56.7899392530668,56.8774597652612,
56.964967349741,57.0524826602265,57.1400263509079,57.2276669881264,57.3153651881873,
57.4031890064531,57.4264891454977,57.5143068691386,57.6020137976755,57.6896329310915,
57.7805686299648,57.8680891422733,57.955596726865,58.0431120374602,58.130655728249,
58.2182963655708,58.305994565733,58.393818384096,58.4171185220777,58.5049362463864,
58.5926431755944,58.6802623096844,58.7711980083061,58.8587185212908,58.9462261065584,
59.0337414178285,59.1212851092902,59.2089257472791,59.2966239481054,59.3844477671235,
59.4077478986577,59.5162980940452,59.6233575451915,59.6902604180837),
 .UNSPECIFIED.);
#2002=B_SPLINE_CURVE_WITH_KNOTS('',3,(#21651,#21652,#21653,#21654,#21655,
#21656,#21657,#21658,#21659,#21660,#21661,#21662,#21663,#21664,#21665,#21666,
#21667,#21668,#21669,#21670,#21671,#21672,#21673,#21674,#21675,#21676,#21677,
#21678,#21679,#21680,#21681,#21682,#21683,#21684,#21685,#21686,#21687,#21688,
#21689,#21690,#21691,#21692,#21693,#21694,#21695,#21696,#21697,#21698,#21699,
#21700,#21701,#21702,#21703,#21704,#21705,#21706,#21707,#21708,#21709,#21710,
#21711,#21712,#21713,#21714,#21715,#21716,#21717,#21718,#21719,#21720,#21721,
#21722,#21723,#21724,#21725,#21726,#21727,#21728,#21729),.UNSPECIFIED.,
 .F.,.F.,(4,3,3,3,3,3,3,3,3,3,3,3,3,3,3,3,3,3,3,3,3,3,3,3,3,3,4),(59.690260418206,
59.778775025335,59.8656202876019,59.9524524305452,60.0392927619904,60.1290638903022,
60.2160327288199,60.3072050020288,60.3983772752377,60.4861949992754,60.5739019281985,
60.6615210619898,60.7524567607183,60.8399772733726,60.9274848582988,61.0150001692168,
61.1025438603164,61.1901844979299,61.2778826983729,61.365706516999,61.3890066518178,
61.4768208703852,61.564528918874,61.6522906658881,61.7398425050512,61.8277092059909,
61.9155759069306),.UNSPECIFIED.);
#2003=B_SPLINE_CURVE_WITH_KNOTS('',3,(#21731,#21732,#21733,#21734,#21735,
#21736,#21737,#21738,#21739,#21740,#21741,#21742,#21743,#21744,#21745,#21746,
#21747,#21748,#21749,#21750,#21751,#21752,#21753,#21754,#21755,#21756,#21757,
#21758,#21759,#21760,#21761,#21762,#21763,#21764,#21765,#21766,#21767,#21768,
#21769,#21770,#21771,#21772,#21773,#21774,#21775,#21776,#21777,#21778,#21779,
#21780,#21781,#21782,#21783,#21784,#21785,#21786,#21787,#21788,#21789,#21790,
#21791,#21792,#21793,#21794,#21795,#21796,#21797,#21798,#21799,#21800,#21801,
#21802,#21803,#21804,#21805,#21806,#21807,#21808,#21809),.UNSPECIFIED.,
 .F.,.F.,(4,3,3,3,3,3,3,3,3,3,3,3,3,3,3,3,3,3,3,3,3,3,3,3,3,3,4),(59.69026041843,
59.7976956857346,59.9067549033635,59.9680769693988,60.0558946930392,60.1436016215755,
60.2312207549911,60.3221564538646,60.4096769661725,60.4971845507636,60.5846998613582,
60.6722435521463,60.7598841894676,60.8475823896291,60.9354062079916,60.9587063459788,
61.0465260468161,61.1342344663959,61.2218546067637,61.3094092403329,61.3969287920588,
61.4844339306926,61.5719453095894,61.6595334389296,61.7471595670043,61.8349150953348,
61.9154863879853),.UNSPECIFIED.);
#2004=B_SPLINE_CURVE_WITH_KNOTS('',3,(#21810,#21811,#21812,#21813,#21814,
#21815,#21816,#21817,#21818,#21819,#21820,#21821,#21822,#21823,#21824,#21825,
#21826,#21827,#21828,#21829,#21830,#21831,#21832,#21833,#21834,#21835,#21836,
#21837,#21838,#21839,#21840,#21841,#21842,#21843,#21844,#21845,#21846,#21847,
#21848,#21849,#21850,#21851,#21852,#21853,#21854,#21855,#21856,#21857,#21858,
#21859,#21860,#21861,#21862,#21863,#21864,#21865,#21866,#21867,#21868,#21869,
#21870,#21871,#21872,#21873,#21874,#21875,#21876,#21877,#21878,#21879,#21880,
#21881,#21882,#21883,#21884,#21885,#21886,#21887,#21888,#21889,#21890,#21891,
#21892,#21893,#21894,#21895,#21896,#21897,#21898,#21899,#21900,#21901,#21902,
#21903,#21904,#21905,#21906,#21907,#21908,#21909,#21910,#21911,#21912,#21913,
#21914,#21915,#21916,#21917,#21918,#21919,#21920,#21921,#21922,#21923,#21924,
#21925,#21926,#21927,#21928,#21929,#21930,#21931,#21932,#21933,#21934,#21935,
#21936,#21937,#21938,#21939,#21940,#21941,#21942,#21943,#21944,#21945,#21946,
#21947,#21948,#21949,#21950,#21951,#21952,#21953,#21954,#21955,#21956,#21957,
#21958,#21959,#21960),.UNSPECIFIED.,.F.,.F.,(4,3,3,3,3,3,3,3,3,3,3,3,3,
3,3,3,3,3,3,3,3,3,3,3,3,3,3,3,3,3,3,3,3,3,3,3,3,3,3,3,3,3,3,3,3,3,3,3,3,
3,4),(55.6321400113866,55.7196839623112,55.8073249236283,55.8950235724135,
55.9828476845365,56.0055594630787,56.0933771867246,56.1810841152679,56.2687032486923,
56.3596389475631,56.4471594598829,56.5346670444873,56.6221823550963,56.7097260459,
56.7973666832387,56.8850648834184,56.9728887018007,56.9961888396587,57.0840065633094,
57.1717134918572,57.2593326252856,57.3502683241548,57.4377888364785,57.5252964210864,
57.6128117316991,57.7003554225064,57.7879960598478,57.8756942600305,57.9635180784152,
57.9868182162387,58.0746359399784,58.1623428686156,58.2499620021338,58.3408977009694,
58.4284182133827,58.51592579808,58.6034411087818,58.6909847996785,58.778625437108,
58.8663236373786,58.9541474558496,58.9774475928187,59.0665491959921,59.1535112710725,
59.2403929922435,59.3272158153754,59.4179769660831,59.5047630081782,59.5915521904114,
59.6783867689599,59.690260418206),.UNSPECIFIED.);
#2005=B_SPLINE_CURVE_WITH_KNOTS('',3,(#21966,#21967,#21968,#21969,#21970,
#21971,#21972,#21973,#21974,#21975,#21976,#21977,#21978,#21979,#21980,#21981,
#21982,#21983,#21984,#21985,#21986,#21987,#21988,#21989,#21990,#21991,#21992,
#21993,#21994,#21995,#21996,#21997,#21998,#21999,#22000,#22001,#22002,#22003,
#22004,#22005,#22006,#22007,#22008,#22009,#22010,#22011,#22012,#22013,#22014,
#22015,#22016,#22017,#22018,#22019,#22020,#22021,#22022,#22023,#22024,#22025,
#22026,#22027,#22028,#22029,#22030,#22031,#22032,#22033,#22034,#22035,#22036,
#22037,#22038,#22039,#22040,#22041,#22042,#22043,#22044,#22045,#22046,#22047,
#22048,#22049,#22050,#22051,#22052,#22053,#22054,#22055,#22056,#22057,#22058,
#22059,#22060,#22061,#22062,#22063,#22064,#22065,#22066,#22067,#22068,#22069,
#22070,#22071,#22072,#22073,#22074,#22075,#22076,#22077,#22078,#22079,#22080,
#22081,#22082,#22083,#22084,#22085,#22086,#22087,#22088,#22089,#22090,#22091,
#22092,#22093,#22094,#22095,#22096,#22097,#22098,#22099,#22100,#22101,#22102,
#22103,#22104,#22105,#22106,#22107,#22108,#22109,#22110,#22111,#22112,#22113),
 .UNSPECIFIED.,.F.,.F.,(4,3,3,3,3,3,3,3,3,3,3,3,3,3,3,3,3,3,3,3,3,3,3,3,
3,3,3,3,3,3,3,3,3,3,3,3,3,3,3,3,3,3,3,3,3,3,3,3,3,4),(49.3487618580268,
49.4365675179812,49.5014541328574,49.5892718565182,49.6769787850765,49.7645979185153,
49.8555336173805,49.943054129715,50.0305617143339,50.1180770249574,50.2056207157755,
50.2932613531282,50.3809595533219,50.4687833717177,50.4920835094375,50.5799012330959,
50.6676081616517,50.7552272950882,50.8461629939543,50.9336835062864,51.0211910909029,
51.1087064015241,51.1962500923399,51.2838907296903,51.3715889298819,51.4594127482754,
51.4827128860175,51.5705306096754,51.6582375382308,51.7458566716667,51.836792370533,
51.9243128828645,52.0118204674805,52.099335778101,52.1868794689162,52.274520106266,
52.3622183064568,52.4500421248497,52.4733422625975,52.5604221705833,52.647391777892,
52.7342748965892,52.8210968701786,52.9078870050405,52.994666687068,53.0814572896196,
53.168330509625,53.2552470964572,53.3422944291726,53.4070751108548),
 .UNSPECIFIED.);
#2006=B_SPLINE_CURVE_WITH_KNOTS('',3,(#22114,#22115,#22116,#22117,#22118,
#22119,#22120,#22121,#22122,#22123,#22124,#22125,#22126,#22127,#22128,#22129,
#22130,#22131,#22132,#22133,#22134,#22135,#22136,#22137,#22138,#22139,#22140,
#22141,#22142,#22143,#22144,#22145,#22146,#22147,#22148,#22149,#22150,#22151,
#22152,#22153,#22154,#22155,#22156,#22157,#22158,#22159,#22160,#22161,#22162,
#22163,#22164,#22165,#22166,#22167,#22168,#22169,#22170,#22171,#22172,#22173,
#22174,#22175,#22176,#22177,#22178,#22179,#22180,#22181,#22182,#22183,#22184,
#22185,#22186,#22187,#22188,#22189,#22190,#22191,#22192,#22193,#22194,#22195,
#22196,#22197,#22198),.UNSPECIFIED.,.F.,.F.,(4,3,3,3,3,3,3,3,3,3,3,3,3,
3,3,3,3,3,3,3,3,3,3,3,3,3,3,3,4),(53.4070751110265,53.4639716391775,53.5517893628235,
53.6394962913669,53.727115424791,53.8180511236619,53.9055716359818,53.9930792205862,
54.0805945311955,54.1681382219994,54.2557788593382,54.3434770595181,54.4313008779004,
54.4546010157576,54.5424187394083,54.6301256679562,54.7177448013845,54.8086805002537,
54.8962010125774,54.9837085971854,55.0712239077979,55.1587675986051,55.2464082359467,
55.3341064361294,55.4219302545142,55.4452303923376,55.5330632331826,55.6207748462577,
55.6330521042359),.UNSPECIFIED.);
#2007=B_SPLINE_CURVE_WITH_KNOTS('',3,(#22200,#22201,#22202,#22203,#22204,
#22205,#22206,#22207,#22208,#22209,#22210,#22211,#22212,#22213,#22214,#22215,
#22216,#22217,#22218,#22219,#22220,#22221,#22222,#22223,#22224,#22225,#22226,
#22227,#22228,#22229,#22230,#22231,#22232,#22233,#22234,#22235,#22236,#22237,
#22238,#22239,#22240,#22241,#22242,#22243,#22244,#22245,#22246,#22247,#22248,
#22249,#22250,#22251,#22252,#22253,#22254,#22255,#22256,#22257,#22258,#22259,
#22260,#22261,#22262,#22263,#22264,#22265,#22266,#22267,#22268,#22269,#22270,
#22271,#22272,#22273,#22274,#22275,#22276,#22277,#22278),.UNSPECIFIED.,
 .F.,.F.,(4,3,3,3,3,3,3,3,3,3,3,3,3,3,3,3,3,3,3,3,3,3,3,3,3,3,4),(53.4070751110265,
53.4952697145472,53.5834738756985,53.6717071431052,53.7600512896597,53.8484511190458,
53.9370104138994,54.0243007099186,54.1121184335766,54.199825362132,54.287444495568,
54.3783801944343,54.465900706766,54.5534082913819,54.6409236020024,54.7284672928175,
54.8161079301673,54.9038061303585,54.9916299487513,55.0149300864986,55.1027351464046,
55.1904358985645,55.2780531741883,55.3665748834878,55.4540907992995,55.543115405343,
55.6321400113866),.UNSPECIFIED.);
#2008=B_SPLINE_CURVE_WITH_KNOTS('',3,(#22279,#22280,#22281,#22282,#22283,
#22284,#22285,#22286,#22287,#22288,#22289,#22290,#22291,#22292,#22293,#22294,
#22295,#22296,#22297,#22298,#22299,#22300,#22301,#22302,#22303,#22304,#22305,
#22306,#22307,#22308,#22309,#22310,#22311,#22312,#22313,#22314,#22315,#22316,
#22317,#22318,#22319,#22320,#22321,#22322,#22323,#22324,#22325,#22326,#22327,
#22328,#22329,#22330,#22331,#22332,#22333,#22334,#22335,#22336,#22337,#22338,
#22339,#22340,#22341,#22342,#22343,#22344,#22345,#22346,#22347,#22348,#22349,
#22350,#22351,#22352,#22353,#22354,#22355,#22356,#22357,#22358,#22359,#22360,
#22361,#22362,#22363,#22364,#22365,#22366,#22367,#22368,#22369,#22370,#22371,
#22372,#22373,#22374,#22375,#22376,#22377,#22378,#22379,#22380,#22381,#22382,
#22383,#22384,#22385,#22386,#22387,#22388,#22389,#22390,#22391,#22392,#22393,
#22394,#22395,#22396,#22397,#22398,#22399,#22400,#22401,#22402,#22403,#22404,
#22405,#22406,#22407,#22408,#22409,#22410,#22411,#22412,#22413,#22414,#22415,
#22416,#22417,#22418,#22419,#22420,#22421,#22422,#22423),.UNSPECIFIED.,
 .F.,.F.,(4,3,3,3,3,3,3,3,3,3,3,3,3,3,3,3,3,3,3,3,3,3,3,3,3,3,3,3,3,3,3,
3,3,3,3,3,3,3,3,3,3,3,3,3,3,3,3,3,4),(49.3498253603234,49.4388200907328,
49.5263372418594,49.6138446717405,49.7013630332064,49.7914680758044,49.8791179240511,
49.9704505638248,50.0617832035985,50.1496009272582,50.2373078558154,50.3249269892531,
50.4158626881187,50.5033832004519,50.5908907850695,50.678406095692,50.7659497865093,
50.853590423861,50.9412886240534,51.029112442448,51.0524125801785,51.1402303038378,
51.2279372323945,51.3155563658318,51.4064920646977,51.4940125770307,51.581520161648,
51.6690354722701,51.7565791630868,51.8442198004381,51.9319180006304,52.0197418190249,
52.0430419567586,52.1308596804195,52.2185666089776,52.3061857424166,52.3971214412818,
52.4846419536162,52.5721495382348,52.6596648488581,52.7472085396768,52.8348491770294,
52.922547377223,53.0103711956187,53.0336713333386,53.1327118219618,53.2314411214165,
53.3295918555088,53.4070751108161),.UNSPECIFIED.);
#2009=B_SPLINE_CURVE_WITH_KNOTS('',3,(#22429,#22430,#22431,#22432,#22433,
#22434,#22435,#22436,#22437,#22438,#22439,#22440,#22441,#22442,#22443,#22444,
#22445,#22446,#22447,#22448,#22449,#22450,#22451,#22452,#22453,#22454,#22455,
#22456,#22457,#22458,#22459,#22460,#22461,#22462,#22463,#22464,#22465,#22466,
#22467,#22468,#22469,#22470,#22471,#22472,#22473,#22474,#22475,#22476,#22477,
#22478,#22479,#22480,#22481,#22482,#22483,#22484,#22485,#22486,#22487,#22488,
#22489,#22490,#22491,#22492,#22493,#22494,#22495,#22496,#22497,#22498,#22499,
#22500,#22501,#22502,#22503,#22504,#22505,#22506,#22507,#22508,#22509,#22510,
#22511,#22512,#22513,#22514,#22515,#22516,#22517,#22518,#22519,#22520,#22521,
#22522,#22523,#22524,#22525,#22526,#22527,#22528,#22529,#22530,#22531,#22532,
#22533,#22534,#22535,#22536,#22537,#22538,#22539,#22540,#22541,#22542,#22543,
#22544,#22545,#22546,#22547,#22548,#22549,#22550,#22551,#22552,#22553,#22554,
#22555,#22556,#22557,#22558,#22559,#22560,#22561,#22562,#22563,#22564,#22565,
#22566,#22567,#22568,#22569,#22570,#22571,#22572,#22573,#22574,#22575,#22576),
 .UNSPECIFIED.,.F.,.F.,(4,3,3,3,3,3,3,3,3,3,3,3,3,3,3,3,3,3,3,3,3,3,3,3,
3,3,3,3,3,3,3,3,3,3,3,3,3,3,3,3,3,3,3,3,3,3,3,3,3,4),(43.0661023012462,
43.1536126300917,43.2411442446049,43.3287694089535,43.4164457561466,43.5042559095106,
43.5576778733773,43.6454955970372,43.7332025255944,43.8208216590323,43.9117573578979,
43.9992778702314,44.0867854548493,44.1743007654716,44.2618444562889,44.3494850936406,
44.4371832938334,44.5250071122282,44.5483072499573,44.6361249736169,44.7238319021739,
44.8114510356116,44.9023867344773,44.9899072468106,45.0774148314283,45.1649301420504,
45.2524738328672,45.3401144702188,45.4278126704111,45.5156364888057,45.5389366265373,
45.6267543501969,45.7144612787542,45.802080412192,45.8930161110577,45.980536623391,
46.0680442080088,46.1555595186313,46.2431032094489,46.3307438468006,46.4184420469933,
46.5062658653882,46.5295660031174,46.6186563250419,46.7076259258587,46.7964937259141,
46.885263700463,46.9739759768097,47.062651294479,47.1238898038469),
 .UNSPECIFIED.);
#2010=B_SPLINE_CURVE_WITH_KNOTS('',3,(#22577,#22578,#22579,#22580,#22581,
#22582,#22583,#22584,#22585,#22586,#22587,#22588,#22589,#22590,#22591,#22592,
#22593,#22594,#22595,#22596,#22597,#22598,#22599,#22600,#22601,#22602,#22603,
#22604,#22605,#22606,#22607,#22608,#22609,#22610,#22611,#22612,#22613,#22614,
#22615,#22616,#22617,#22618,#22619,#22620,#22621,#22622,#22623,#22624,#22625,
#22626,#22627,#22628,#22629,#22630,#22631,#22632,#22633,#22634,#22635,#22636,
#22637,#22638,#22639,#22640,#22641,#22642,#22643,#22644,#22645,#22646,#22647,
#22648,#22649,#22650,#22651,#22652,#22653,#22654,#22655),.UNSPECIFIED.,
 .F.,.F.,(4,3,3,3,3,3,3,3,3,3,3,3,3,3,3,3,3,3,3,3,3,3,3,3,3,3,4),(47.123889804041,
47.2229661979551,47.3199017158507,47.420048547774,47.5201953796974,47.608013103357,
47.695720031914,47.7833391653517,47.8742748642174,47.9617953765507,48.0493029611683,
48.1368182717907,48.2243619626077,48.3120025999592,48.3997008001519,48.4875246185464,
48.5108247562774,48.5986518170988,48.6863658894003,48.773976252068,48.8615284126728,
48.9490430731687,49.0365409030647,49.1240737168936,49.2116250160482,49.2992578782039,
49.3487618580268),.UNSPECIFIED.);
#2011=B_SPLINE_CURVE_WITH_KNOTS('',3,(#22657,#22658,#22659,#22660,#22661,
#22662,#22663,#22664,#22665,#22666,#22667,#22668,#22669,#22670,#22671,#22672,
#22673,#22674,#22675,#22676,#22677,#22678,#22679,#22680,#22681,#22682,#22683,
#22684,#22685,#22686,#22687,#22688,#22689,#22690,#22691,#22692,#22693,#22694,
#22695,#22696,#22697,#22698,#22699,#22700,#22701,#22702,#22703,#22704,#22705,
#22706,#22707,#22708,#22709,#22710,#22711,#22712,#22713,#22714,#22715,#22716,
#22717,#22718,#22719,#22720,#22721,#22722,#22723,#22724,#22725,#22726,#22727,
#22728,#22729,#22730,#22731,#22732,#22733,#22734,#22735,#22736,#22737,#22738),
 .UNSPECIFIED.,.F.,.F.,(4,3,3,3,3,3,3,3,3,3,3,3,3,3,3,3,3,3,3,3,3,3,3,3,
3,3,3,4),(47.1238898040778,47.2112205230625,47.2984421477901,47.3855782233591,
47.4726547355854,47.5596998923632,47.646734849843,47.7337807519318,47.8209134726754,
47.9080890145208,47.9954065966317,48.0805244504384,48.1683421740981,48.2560491026553,
48.3436682360932,48.4346039349589,48.5221244472922,48.60963203191,48.6971473425325,
48.7846910333495,48.8723316707012,48.9600298708938,49.0478536892886,49.0711538270185,
49.1589647615717,49.2466781854582,49.3342970290963,49.3498253603234),
 .UNSPECIFIED.);
#2012=B_SPLINE_CURVE_WITH_KNOTS('',3,(#22739,#22740,#22741,#22742,#22743,
#22744,#22745,#22746,#22747,#22748,#22749,#22750,#22751,#22752,#22753,#22754,
#22755,#22756,#22757,#22758,#22759,#22760,#22761,#22762,#22763,#22764,#22765,
#22766,#22767,#22768,#22769,#22770,#22771,#22772,#22773,#22774,#22775,#22776,
#22777,#22778,#22779,#22780,#22781,#22782,#22783,#22784,#22785,#22786,#22787,
#22788,#22789,#22790,#22791,#22792,#22793,#22794,#22795,#22796,#22797,#22798,
#22799,#22800,#22801,#22802,#22803,#22804,#22805,#22806,#22807,#22808,#22809,
#22810,#22811,#22812,#22813,#22814,#22815,#22816,#22817,#22818,#22819,#22820,
#22821,#22822,#22823,#22824,#22825,#22826,#22827,#22828,#22829,#22830,#22831,
#22832,#22833,#22834,#22835,#22836,#22837,#22838,#22839,#22840,#22841,#22842,
#22843,#22844,#22845,#22846,#22847,#22848,#22849,#22850,#22851,#22852,#22853,
#22854,#22855,#22856,#22857,#22858,#22859,#22860,#22861,#22862,#22863,#22864,
#22865,#22866,#22867,#22868,#22869,#22870,#22871,#22872,#22873,#22874,#22875,
#22876,#22877,#22878,#22879,#22880,#22881,#22882,#22883,#22884,#22885,#22886,
#22887,#22888,#22889),.UNSPECIFIED.,.F.,.F.,(4,3,3,3,3,3,3,3,3,3,3,3,3,
3,3,3,3,3,3,3,3,3,3,3,3,3,3,3,3,3,3,3,3,3,3,3,3,3,3,3,3,3,3,3,3,3,3,3,3,
3,4),(43.0658096208517,43.1273775675383,43.215195291199,43.3029022197572,
43.3905213531959,43.4814570520612,43.5689775643956,43.6564851490144,43.7440004596378,
43.831544150456,43.9191847878087,44.0068829880025,44.0947068063982,44.1180069441183,
44.2058246677777,44.2935315963345,44.381150729772,44.4720864286378,44.5596069409708,
44.6471145255883,44.7346298362104,44.8221735270271,44.9098141643784,44.9975123645708,
45.0853361829653,45.1086363206984,45.1964540443581,45.2841609729151,45.3717801063527,
45.4627158052184,45.5502363175517,45.6377439021694,45.7252592127917,45.8128029036086,
45.9004435409601,45.9881417411528,46.0759655595475,46.0992656972784,46.1870834209382,
46.2747903494953,46.362409482933,46.4533451817987,46.5408656941322,46.62837327875,
46.7158885893725,46.8034322801896,46.8910729175413,46.9787711177341,47.0665949361289,
47.0898950738584,47.1238898038469),.UNSPECIFIED.);
#2013=B_SPLINE_CURVE_WITH_KNOTS('',3,(#22895,#22896,#22897,#22898,#22899,
#22900,#22901,#22902,#22903,#22904,#22905,#22906,#22907,#22908,#22909,#22910,
#22911,#22912,#22913,#22914,#22915,#22916,#22917,#22918,#22919,#22920,#22921,
#22922,#22923,#22924,#22925,#22926,#22927,#22928,#22929,#22930,#22931,#22932,
#22933,#22934,#22935,#22936,#22937,#22938,#22939,#22940,#22941,#22942,#22943,
#22944,#22945,#22946,#22947,#22948,#22949,#22950,#22951,#22952,#22953,#22954,
#22955,#22956,#22957,#22958,#22959,#22960,#22961,#22962,#22963,#22964,#22965,
#22966,#22967,#22968,#22969,#22970,#22971,#22972,#22973,#22974,#22975,#22976,
#22977,#22978,#22979,#22980,#22981,#22982,#22983,#22984,#22985,#22986,#22987,
#22988,#22989,#22990,#22991,#22992,#22993,#22994,#22995,#22996,#22997,#22998,
#22999,#23000,#23001,#23002,#23003,#23004,#23005,#23006,#23007,#23008,#23009,
#23010,#23011,#23012,#23013,#23014,#23015,#23016,#23017,#23018,#23019,#23020,
#23021,#23022,#23023,#23024,#23025,#23026,#23027,#23028,#23029,#23030,#23031,
#23032,#23033,#23034,#23035,#23036,#23037,#23038,#23039,#23040,#23041,#23042),
 .UNSPECIFIED.,.F.,.F.,(4,3,3,3,3,3,3,3,3,3,3,3,3,3,3,3,3,3,3,3,3,3,3,3,
3,3,3,3,3,3,3,3,3,3,3,3,3,3,3,3,3,3,3,3,3,3,3,3,3,4),(36.7834743401322,
36.8711071637446,36.9586711087439,37.0461970549791,37.1337056646341,37.2212175932281,
37.3087534936155,37.3963842592218,37.4840686230105,37.5718836331408,37.6139016138971,
37.7017193375657,37.7894262661317,37.8770453995785,37.9679810984408,38.0555016107834,
38.1430091954105,38.2305245060423,38.3180681968688,38.4057088342298,38.493407034432,
38.5812308528361,38.6045309904771,38.6923487141351,38.7800556426903,38.8676747761262,
38.9586104749926,39.0461309873241,39.13363857194,39.2211538825605,39.3086975733757,
39.3963382107255,39.4840364109164,39.5718602293094,39.5951603670572,39.6829780907158,
39.7706850192718,39.8583041527084,39.9492398515745,40.0367603639067,40.1242679485233,
40.2117832591444,40.2993269499602,40.3869675873106,40.4746657875022,40.5624896058956,
40.5857897436372,40.69875304535,40.809605914276,40.8407044964449),
 .UNSPECIFIED.);
#2014=B_SPLINE_CURVE_WITH_KNOTS('',3,(#23043,#23044,#23045,#23046,#23047,
#23048,#23049,#23050,#23051,#23052,#23053,#23054,#23055,#23056,#23057,#23058,
#23059,#23060,#23061,#23062,#23063,#23064,#23065,#23066,#23067,#23068,#23069,
#23070,#23071,#23072,#23073,#23074,#23075,#23076,#23077,#23078,#23079,#23080,
#23081,#23082,#23083,#23084,#23085,#23086,#23087,#23088,#23089,#23090,#23091,
#23092,#23093,#23094,#23095,#23096,#23097,#23098,#23099,#23100,#23101,#23102,
#23103,#23104,#23105,#23106,#23107,#23108,#23109,#23110,#23111,#23112,#23113,
#23114,#23115,#23116,#23117,#23118,#23119,#23120,#23121,#23122,#23123,#23124),
 .UNSPECIFIED.,.F.,.F.,(4,3,3,3,3,3,3,3,3,3,3,3,3,3,3,3,3,3,3,3,3,3,3,3,
3,3,3,4),(40.8407044966673,40.9273584362594,41.0139637234753,41.1005454082162,
41.1871250286611,41.273724117299,41.360413926364,41.4471549251205,41.5340255171113,
41.5764191202172,41.6642368438767,41.7519437724335,41.8395629058709,41.9304986047367,
42.0180191170698,42.1055267016873,42.1930420123095,42.2805857031267,42.3682263404781,
42.4559245406708,42.5437483590651,42.5670484967972,42.6548657909635,42.7425763493776,
42.8301869080249,42.917739060608,43.005257970339,43.0661023012462),
 .UNSPECIFIED.);
#2015=B_SPLINE_CURVE_WITH_KNOTS('',3,(#23126,#23127,#23128,#23129,#23130,
#23131,#23132,#23133,#23134,#23135,#23136,#23137,#23138,#23139,#23140,#23141,
#23142,#23143,#23144,#23145,#23146,#23147,#23148,#23149,#23150,#23151,#23152,
#23153,#23154,#23155,#23156,#23157,#23158,#23159,#23160,#23161,#23162,#23163,
#23164,#23165,#23166,#23167,#23168,#23169,#23170,#23171,#23172,#23173,#23174,
#23175,#23176,#23177,#23178,#23179,#23180,#23181,#23182,#23183,#23184,#23185,
#23186,#23187,#23188,#23189,#23190,#23191,#23192,#23193,#23194,#23195,#23196,
#23197,#23198,#23199,#23200,#23201,#23202,#23203,#23204),.UNSPECIFIED.,
 .F.,.F.,(4,3,3,3,3,3,3,3,3,3,3,3,3,3,3,3,3,3,3,3,3,3,3,3,3,3,4),(40.8407044968328,
40.9448640922798,41.0502373864949,41.1461188143783,41.2339365380362,41.3216434665914,
41.4092626000271,41.5001982988935,41.5877188112251,41.6752263958409,41.7627417064615,
41.8502853972766,41.9379260346264,42.0256242348173,42.1134480532102,42.1367481909583,
42.224569549295,42.31227922823,42.3999002315181,42.4874540511531,42.574972225742,
42.6624754241101,42.7499842991571,42.8375628974725,42.9251792654583,43.0129084798028,
43.0658096208517),.UNSPECIFIED.);
#2016=B_SPLINE_CURVE_WITH_KNOTS('',3,(#23205,#23206,#23207,#23208,#23209,
#23210,#23211,#23212,#23213,#23214,#23215,#23216,#23217,#23218,#23219,#23220,
#23221,#23222,#23223,#23224,#23225,#23226,#23227,#23228,#23229,#23230,#23231,
#23232,#23233,#23234,#23235,#23236,#23237,#23238,#23239,#23240,#23241,#23242,
#23243,#23244,#23245,#23246,#23247,#23248,#23249,#23250,#23251,#23252,#23253,
#23254,#23255,#23256,#23257,#23258,#23259,#23260,#23261,#23262,#23263,#23264,
#23265,#23266,#23267,#23268,#23269,#23270,#23271,#23272,#23273,#23274,#23275,
#23276,#23277,#23278,#23279,#23280,#23281,#23282,#23283,#23284,#23285,#23286,
#23287,#23288,#23289,#23290,#23291,#23292,#23293,#23294,#23295,#23296,#23297,
#23298,#23299,#23300,#23301,#23302,#23303,#23304,#23305,#23306,#23307,#23308,
#23309,#23310,#23311,#23312,#23313,#23314,#23315,#23316,#23317,#23318,#23319,
#23320,#23321,#23322,#23323,#23324,#23325,#23326,#23327,#23328,#23329,#23330,
#23331,#23332,#23333,#23334,#23335,#23336,#23337,#23338,#23339,#23340,#23341,
#23342,#23343,#23344,#23345,#23346,#23347,#23348,#23349,#23350,#23351,#23352),
 .UNSPECIFIED.,.F.,.F.,(4,3,3,3,3,3,3,3,3,3,3,3,3,3,3,3,3,3,3,3,3,3,3,3,
3,3,3,3,3,3,3,3,3,3,3,3,3,3,3,3,3,3,3,3,3,3,3,3,3,4),(36.7826549237052,
36.8701876778202,36.9578143457823,37.0454928584368,37.1333043041305,37.1836013080582,
37.2714190317939,37.359125960428,37.446745093943,37.5376807927799,37.6252013051928,
37.7127088898905,37.800224200593,37.8877678914908,37.9754085289231,38.0631067291966,
38.1509305476717,38.1742306846382,38.2620484082878,38.349755336835,38.4373744702625,
38.528310169132,38.6158306814555,38.7033382660635,38.7908535766762,38.8783972674837,
38.9660379048259,39.053736105009,39.1415599233944,39.1648600612182,39.2526777848656,
39.3403847134099,39.4280038468351,39.5189395457055,39.6064600580255,39.6939676426297,
39.7814829532385,39.8690266440421,39.9566672813798,40.0443654815587,40.1321892999396,
40.1554894377982,40.242885923383,40.3301773559143,40.4173849585116,40.5045298834924,
40.5916445938404,40.6787389692804,40.7658659689735,40.8407044966673),
 .UNSPECIFIED.);
#2017=B_SPLINE_CURVE_WITH_KNOTS('',3,(#23358,#23359,#23360,#23361,#23362,
#23363,#23364,#23365,#23366,#23367,#23368,#23369,#23370,#23371,#23372,#23373,
#23374,#23375,#23376,#23377,#23378,#23379,#23380,#23381,#23382,#23383,#23384,
#23385,#23386,#23387,#23388,#23389,#23390,#23391,#23392,#23393,#23394,#23395,
#23396,#23397,#23398,#23399,#23400,#23401,#23402,#23403,#23404,#23405,#23406,
#23407,#23408,#23409,#23410,#23411,#23412,#23413,#23414,#23415,#23416,#23417,
#23418,#23419,#23420,#23421,#23422,#23423,#23424,#23425,#23426,#23427,#23428,
#23429,#23430,#23431,#23432,#23433,#23434,#23435,#23436,#23437,#23438,#23439,
#23440,#23441,#23442,#23443,#23444,#23445,#23446,#23447,#23448,#23449,#23450,
#23451,#23452,#23453,#23454,#23455,#23456,#23457,#23458,#23459,#23460,#23461,
#23462,#23463,#23464,#23465,#23466,#23467,#23468,#23469,#23470,#23471,#23472,
#23473,#23474,#23475,#23476,#23477,#23478,#23479,#23480,#23481,#23482,#23483,
#23484,#23485,#23486,#23487,#23488,#23489,#23490,#23491,#23492,#23493,#23494,
#23495,#23496,#23497,#23498,#23499,#23500,#23501,#23502,#23503,#23504,#23505),
 .UNSPECIFIED.,.F.,.F.,(4,3,3,3,3,3,3,3,3,3,3,3,3,3,3,3,3,3,3,3,3,3,3,3,
3,3,3,3,3,3,3,3,3,3,3,3,3,3,3,3,3,3,3,3,3,3,3,3,3,4),(30.499179135538,30.5893375566874,
30.6794959778369,30.7673137002222,30.855020627484,30.9426397596071,31.0335754589583,
31.1210959699375,31.2086035531887,31.2961188624336,31.3836625518638,31.4713031878215,
31.5590013866146,31.6468252036119,31.6701253544169,31.7579430786979,31.8456500078836,
31.9332691419565,32.0242048405866,32.1117253535674,32.1992329388361,32.286748250112,
32.3742919415847,32.4619325795915,32.5496307804401,32.6374545994864,32.660754730997,
32.7485724546252,32.8362793831518,32.9238985165601,33.0148342154372,33.1023547277439,
33.1898623123359,33.2773776229338,33.3649213137274,33.4525619510574,33.5402601512295,
33.6280839696054,33.651384107577,33.738220097311,33.8249459930007,33.9115858335185,
33.9981647381679,34.0847124762968,34.1712506300867,34.2578007697305,34.3444298640546,
34.4311037988402,34.5178962961427,34.557519189277),.UNSPECIFIED.);
#2018=B_SPLINE_CURVE_WITH_KNOTS('',3,(#23506,#23507,#23508,#23509,#23510,
#23511,#23512,#23513,#23514,#23515,#23516,#23517,#23518,#23519,#23520,#23521,
#23522,#23523,#23524,#23525,#23526,#23527,#23528,#23529,#23530,#23531,#23532,
#23533,#23534,#23535,#23536,#23537,#23538,#23539,#23540,#23541,#23542,#23543,
#23544,#23545,#23546,#23547,#23548,#23549,#23550,#23551,#23552,#23553,#23554,
#23555,#23556,#23557,#23558,#23559,#23560,#23561,#23562,#23563,#23564,#23565,
#23566,#23567,#23568,#23569,#23570,#23571,#23572,#23573,#23574,#23575,#23576,
#23577,#23578,#23579,#23580,#23581,#23582,#23583,#23584,#23585,#23586,#23587),
 .UNSPECIFIED.,.F.,.F.,(4,3,3,3,3,3,3,3,3,3,3,3,3,3,3,3,3,3,3,3,3,3,3,3,
3,3,3,4),(34.5575191894877,34.642013484157,34.7298312078922,34.8175381365257,
34.9051572700407,34.9960929688778,35.08361348129,35.1711210659872,35.2586363766893,
35.3461800675866,35.4338207050184,35.5215189052913,35.6093427237659,35.6326428607371,
35.7204605843868,35.8081675129339,35.8957866463615,35.986722345231,36.0742428575545,
36.1617504421624,36.2492657527751,36.3368094435825,36.4244500809247,36.5121482811081,
36.5999720994938,36.6232722373171,36.7110751645277,36.7834743401322),
 .UNSPECIFIED.);
#2019=B_SPLINE_CURVE_WITH_KNOTS('',3,(#23589,#23590,#23591,#23592,#23593,
#23594,#23595,#23596,#23597,#23598,#23599,#23600,#23601,#23602,#23603,#23604,
#23605,#23606,#23607,#23608,#23609,#23610,#23611,#23612,#23613,#23614,#23615,
#23616,#23617,#23618,#23619,#23620,#23621,#23622,#23623,#23624,#23625,#23626,
#23627,#23628,#23629,#23630,#23631,#23632,#23633,#23634,#23635,#23636,#23637,
#23638,#23639,#23640,#23641,#23642,#23643,#23644,#23645,#23646,#23647,#23648,
#23649,#23650,#23651,#23652,#23653,#23654,#23655,#23656,#23657,#23658,#23659,
#23660,#23661,#23662,#23663,#23664,#23665,#23666,#23667,#23668,#23669,#23670),
 .UNSPECIFIED.,.F.,.F.,(4,3,3,3,3,3,3,3,3,3,3,3,3,3,3,3,3,3,3,3,3,3,3,3,
3,3,3,4),(34.5575191894877,34.6452189793789,34.7329127217104,34.8206207339508,
34.9083633387032,34.9962128811143,35.0841246971867,35.1721722031937,35.2023425548981,
35.2901602785259,35.377867207052,35.4654863404597,35.556422039337,35.6439425516432,
35.731450136235,35.8189654468322,35.9065091376253,35.9941497749548,36.0818479751265,
36.1696717935019,36.1929719314781,36.2807796097188,36.3684824147923,36.4561011804982,
36.543654685054,36.6311690814345,36.7186812679009,36.7826549237052),
 .UNSPECIFIED.);
#2020=B_SPLINE_CURVE_WITH_KNOTS('',3,(#23671,#23672,#23673,#23674,#23675,
#23676,#23677,#23678,#23679,#23680,#23681,#23682,#23683,#23684,#23685,#23686,
#23687,#23688,#23689,#23690,#23691,#23692,#23693,#23694,#23695,#23696,#23697,
#23698,#23699,#23700,#23701,#23702,#23703,#23704,#23705,#23706,#23707,#23708,
#23709,#23710,#23711,#23712,#23713,#23714,#23715,#23716,#23717,#23718,#23719,
#23720,#23721,#23722,#23723,#23724,#23725,#23726,#23727,#23728,#23729,#23730,
#23731,#23732,#23733,#23734,#23735,#23736,#23737,#23738,#23739,#23740,#23741,
#23742,#23743,#23744,#23745,#23746,#23747,#23748,#23749,#23750,#23751,#23752,
#23753,#23754,#23755,#23756,#23757,#23758,#23759,#23760,#23761,#23762,#23763,
#23764,#23765,#23766,#23767,#23768,#23769,#23770,#23771,#23772,#23773,#23774,
#23775,#23776,#23777,#23778,#23779,#23780,#23781,#23782,#23783,#23784,#23785,
#23786,#23787,#23788,#23789,#23790,#23791,#23792,#23793,#23794,#23795,#23796,
#23797,#23798,#23799,#23800,#23801,#23802,#23803,#23804,#23805,#23806,#23807,
#23808,#23809,#23810,#23811,#23812,#23813,#23814,#23815,#23816,#23817,#23818),
 .UNSPECIFIED.,.F.,.F.,(4,3,3,3,3,3,3,3,3,3,3,3,3,3,3,3,3,3,3,3,3,3,3,3,
3,3,3,3,3,3,3,3,3,3,3,3,3,3,3,3,3,3,3,3,3,3,3,3,3,4),(30.5002984399058,
30.5878602452616,30.6753851607737,30.7628935103742,30.8504059492333,30.9379431304048,
31.0255755475,31.1132622557034,31.2010787172136,31.239825048578,31.3276427771969,
31.415349710767,31.5029688492647,31.5939045462514,31.6814250637303,31.7689326535164,
31.8564479693238,31.9439916653367,32.0316323078755,32.1193305132559,32.2071543367997,
32.230454425158,32.3182721490473,32.4059790778497,32.4935982115487,32.5845339103224,
32.6720544229544,32.7595620078844,32.8470773188319,32.9346210099875,33.0222616476948,
33.1099598482538,33.1977836670276,33.221083801738,33.3089015241168,33.3966084513723,
33.4842275834887,33.5751632828423,33.6626837938146,33.7501913770588,33.8377066862966,
33.9252503757199,34.0128910116704,34.1005892104557,34.1884130274459,34.2117131783181,
34.313067474497,34.4140179484392,34.5142334839579,34.5575191892806),
 .UNSPECIFIED.);
#2021=B_SPLINE_CURVE_WITH_KNOTS('',3,(#23824,#23825,#23826,#23827,#23828,
#23829,#23830,#23831,#23832,#23833,#23834,#23835,#23836,#23837,#23838,#23839,
#23840,#23841,#23842,#23843,#23844,#23845,#23846,#23847,#23848,#23849,#23850,
#23851,#23852,#23853,#23854,#23855,#23856,#23857,#23858,#23859,#23860,#23861,
#23862,#23863,#23864,#23865,#23866,#23867,#23868,#23869,#23870,#23871,#23872,
#23873,#23874,#23875,#23876,#23877,#23878,#23879,#23880,#23881,#23882,#23883,
#23884,#23885,#23886,#23887,#23888,#23889,#23890,#23891,#23892,#23893,#23894,
#23895,#23896,#23897,#23898,#23899,#23900,#23901,#23902,#23903,#23904,#23905,
#23906,#23907,#23908,#23909,#23910,#23911,#23912,#23913,#23914,#23915,#23916,
#23917,#23918,#23919,#23920,#23921,#23922,#23923,#23924,#23925,#23926,#23927,
#23928,#23929,#23930,#23931,#23932,#23933,#23934,#23935,#23936,#23937,#23938,
#23939,#23940,#23941,#23942,#23943,#23944,#23945,#23946,#23947,#23948,#23949,
#23950,#23951,#23952,#23953,#23954,#23955,#23956,#23957,#23958,#23959,#23960,
#23961,#23962,#23963,#23964,#23965,#23966,#23967,#23968,#23969,#23970,#23971),
 .UNSPECIFIED.,.F.,.F.,(4,3,3,3,3,3,3,3,3,3,3,3,3,3,3,3,3,3,3,3,3,3,3,3,
3,3,3,3,3,3,3,3,3,3,3,3,3,3,3,3,3,3,3,3,3,3,3,3,3,4),(24.2166288571228,
24.3041368674925,24.3916596706009,24.4792726971757,24.566931069276,24.6547311885646,
24.7357197183568,24.8235373294678,24.9112441438101,24.9988631615165,25.0897989031941,
25.1773192967496,25.2648267616694,25.3523419518016,25.4398855214642,25.5275260372822,
25.6152241155778,25.7030478124688,25.7263490949368,25.8141668559407,25.9018738221971,
25.9894929936409,26.0804286783753,26.1679492292338,26.2554568525008,26.3429722018544,
26.4305159314423,26.5181566074283,26.6058548462211,26.6936787028705,26.7169784715168,
26.8047962016822,26.8925031369463,26.9801222772827,27.0710579736345,27.1585784933031,
27.2460860854053,27.3336014036538,27.4211451022311,27.5087857475037,27.5964839557206,
27.6843077822307,27.7076078480968,27.7974230850532,27.8871096166564,27.9766849091007,
28.0661443963394,28.1555357321797,28.2448678041985,28.2743338823081),
 .UNSPECIFIED.);
#2022=B_SPLINE_CURVE_WITH_KNOTS('',3,(#23972,#23973,#23974,#23975,#23976,
#23977,#23978,#23979,#23980,#23981,#23982,#23983,#23984,#23985,#23986,#23987,
#23988,#23989,#23990,#23991,#23992,#23993,#23994,#23995,#23996,#23997,#23998,
#23999,#24000,#24001,#24002,#24003,#24004,#24005,#24006,#24007,#24008,#24009,
#24010,#24011,#24012,#24013,#24014,#24015,#24016,#24017,#24018,#24019,#24020,
#24021,#24022,#24023,#24024,#24025,#24026,#24027,#24028,#24029,#24030,#24031,
#24032,#24033,#24034,#24035,#24036,#24037,#24038,#24039,#24040,#24041,#24042,
#24043,#24044,#24045,#24046,#24047,#24048,#24049,#24050,#24051,#24052,#24053),
 .UNSPECIFIED.,.F.,.F.,(4,3,3,3,3,3,3,3,3,3,3,3,3,3,3,3,3,3,3,3,3,3,3,3,
3,3,3,4),(28.2743338824658,28.3691609854844,28.4643913559285,28.5598306987876,
28.655571310451,28.6982372246769,28.7860549532668,28.8737618868075,28.9613810252757,
29.0523167222734,29.1398372397223,29.227344829478,29.3148601452551,29.4024038412383,
29.4900444837466,29.5777426890967,29.6655665126103,29.6888666012569,29.7766954671533,
29.8670059257014,29.9546146136881,30.0421651506947,30.1296782383663,30.2171745458006,
30.3047008000479,30.392245862666,30.4798596297893,30.499179135538),
 .UNSPECIFIED.);
#2023=B_SPLINE_CURVE_WITH_KNOTS('',3,(#24055,#24056,#24057,#24058,#24059,
#24060,#24061,#24062,#24063,#24064,#24065,#24066,#24067,#24068,#24069,#24070,
#24071,#24072,#24073,#24074,#24075,#24076,#24077,#24078,#24079,#24080,#24081,
#24082,#24083,#24084,#24085,#24086,#24087,#24088,#24089,#24090,#24091,#24092,
#24093,#24094,#24095,#24096,#24097,#24098,#24099,#24100,#24101,#24102,#24103,
#24104,#24105,#24106,#24107,#24108,#24109,#24110,#24111,#24112,#24113,#24114,
#24115,#24116,#24117,#24118,#24119,#24120,#24121,#24122,#24123,#24124,#24125,
#24126,#24127,#24128,#24129,#24130,#24131,#24132,#24133,#24134,#24135,#24136),
 .UNSPECIFIED.,.F.,.F.,(4,3,3,3,3,3,3,3,3,3,3,3,3,3,3,3,3,3,3,3,3,3,3,3,
3,3,3,4),(28.2743338824903,28.3620519963626,28.4496594121888,28.5371792514047,
28.6273526319063,28.7147749201041,28.8021846607065,28.8896026161822,28.9770495498907,
29.0645934767364,29.1521957096281,29.2399222139786,29.2585662954179,29.3463840255884,
29.4340909608579,29.5217101012003,29.61264579755,29.7001663172262,29.7876739093364,
29.8751892275934,29.9627329261795,30.0503735714618,30.1380717796889,30.2258956062094,
30.249195671998,30.3370125939292,30.4247058191897,30.5002984399058),
 .UNSPECIFIED.);
#2024=B_SPLINE_CURVE_WITH_KNOTS('',3,(#24137,#24138,#24139,#24140,#24141,
#24142,#24143,#24144,#24145,#24146,#24147,#24148,#24149,#24150,#24151,#24152,
#24153,#24154,#24155,#24156,#24157,#24158,#24159,#24160,#24161,#24162,#24163,
#24164,#24165,#24166,#24167,#24168,#24169,#24170,#24171,#24172,#24173,#24174,
#24175,#24176,#24177,#24178,#24179,#24180,#24181,#24182,#24183,#24184,#24185,
#24186,#24187,#24188,#24189,#24190,#24191,#24192,#24193,#24194,#24195,#24196,
#24197,#24198,#24199,#24200,#24201,#24202,#24203,#24204,#24205,#24206,#24207,
#24208,#24209,#24210,#24211,#24212,#24213,#24214,#24215,#24216,#24217,#24218,
#24219,#24220,#24221,#24222,#24223,#24224,#24225,#24226,#24227,#24228,#24229,
#24230,#24231,#24232,#24233,#24234,#24235,#24236,#24237,#24238,#24239,#24240,
#24241,#24242,#24243,#24244,#24245,#24246,#24247,#24248,#24249,#24250,#24251,
#24252,#24253,#24254,#24255,#24256,#24257,#24258,#24259,#24260,#24261,#24262,
#24263,#24264,#24265,#24266,#24267,#24268,#24269,#24270,#24271,#24272,#24273,
#24274,#24275,#24276,#24277,#24278,#24279,#24280,#24281,#24282,#24283,#24284,
#24285,#24286,#24287),.UNSPECIFIED.,.F.,.F.,(4,3,3,3,3,3,3,3,3,3,3,3,3,
3,3,3,3,3,3,3,3,3,3,3,3,3,3,3,3,3,3,3,3,3,3,3,3,3,3,3,3,3,3,3,3,3,3,3,3,
3,4),(24.2161577207422,24.3054194125178,24.3932361228833,24.4809420238797,
24.5685601168336,24.6594962008666,24.7470156471117,24.8345221580275,24.9220363884866,
25.0095789938273,25.0972185432613,25.1849156528371,25.272738384953,25.2960487890978,
25.3838667793172,25.4715739764554,25.5591933801517,25.6501289783424,25.7376497633592,
25.8251576210765,25.9126732049139,26.0002171687608,26.0878580774833,26.1755565483974,
26.2633806344902,26.2866781656778,26.374495984922,26.4622030113276,26.5498222447462,
26.6407579069351,26.7282785239503,26.8157862148092,26.9033016331222,26.9908454329701,
27.0784861808025,27.1661844924512,27.2540084228901,27.2773075422579,27.3651251529403,
27.4528319668475,27.540450984113,27.6313867259536,27.7189071190562,27.8064145835193,
27.8939297731919,27.981473342392,28.0691138577458,28.1568119355757,28.2446356320024,
28.2679369188379,28.2743338823081),.UNSPECIFIED.);
#2025=B_SPLINE_CURVE_WITH_KNOTS('',3,(#24293,#24294,#24295,#24296,#24297,
#24298,#24299,#24300,#24301,#24302,#24303,#24304,#24305,#24306,#24307,#24308,
#24309,#24310,#24311,#24312,#24313,#24314,#24315,#24316,#24317,#24318,#24319,
#24320,#24321,#24322,#24323,#24324,#24325,#24326,#24327,#24328,#24329,#24330,
#24331,#24332,#24333,#24334,#24335,#24336,#24337,#24338,#24339,#24340,#24341,
#24342,#24343,#24344,#24345,#24346,#24347,#24348,#24349,#24350,#24351,#24352,
#24353,#24354,#24355,#24356,#24357,#24358,#24359,#24360,#24361,#24362,#24363,
#24364,#24365,#24366,#24367,#24368,#24369,#24370,#24371,#24372,#24373,#24374),
 .UNSPECIFIED.,.F.,.F.,(4,3,3,3,3,3,3,3,3,3,3,3,3,3,3,3,3,3,3,3,3,3,3,3,
3,3,3,4),(15.7079632679489,15.7948129073667,15.8816405851577,15.9684675747776,
16.0553151447895,16.1422596712941,16.2292557094213,16.3163945808846,16.3803843998776,
16.4682246539636,16.5559529120477,16.6435921541955,16.7345198569782,16.8220572814542,
16.9095805630079,16.9971103333933,17.0846672239183,17.1723191161491,17.2600274501478,
17.3478596747392,17.3710137764576,17.4589553852618,17.5467937138014,17.6345494372581,
17.7222397192476,17.8098921203792,17.8975365443745,17.9331346413009),
 .UNSPECIFIED.);
#2026=B_SPLINE_CURVE_WITH_KNOTS('',3,(#24376,#24377,#24378,#24379,#24380),
 .UNSPECIFIED.,.F.,.F.,(4,1,4),(14.3991256467175,15.3897550232976,15.7079551067824),
 .UNSPECIFIED.);
#2027=B_SPLINE_CURVE_WITH_KNOTS('',3,(#24384,#24385,#24386,#24387,#24388,
#24389,#24390,#24391,#24392,#24393,#24394,#24395,#24396,#24397,#24398,#24399,
#24400,#24401,#24402,#24403,#24404,#24405,#24406,#24407,#24408,#24409,#24410,
#24411,#24412,#24413,#24414,#24415,#24416,#24417,#24418,#24419,#24420,#24421,
#24422,#24423,#24424,#24425,#24426,#24427,#24428,#24429,#24430,#24431,#24432,
#24433,#24434,#24435,#24436,#24437,#24438,#24439,#24440,#24441,#24442,#24443,
#24444,#24445,#24446,#24447),.UNSPECIFIED.,.F.,.F.,(4,3,3,3,3,3,3,3,3,3,
3,3,3,3,3,3,3,3,3,3,3,4),(13.8752088702729,13.9625086734267,14.0496981221134,
14.1368008016614,14.2238420656039,14.3108508994986,14.3978484911417,14.4848560152793,
14.5719483730037,14.6590827513909,14.7463566208474,14.8294259525565,14.9162035714637,
15.0028731802399,15.0910094411765,15.1775356372996,15.2640329274542,15.3505229365851,
15.4398830193721,15.5264647163637,15.6172139920484,15.707963267733),
 .UNSPECIFIED.);
#2028=B_SPLINE_CURVE_WITH_KNOTS('',3,(#24448,#24449,#24450,#24451,#24452,
#24453,#24454,#24455,#24456,#24457,#24458,#24459,#24460,#24461,#24462,#24463,
#24464,#24465,#24466,#24467,#24468,#24469,#24470,#24471,#24472,#24473,#24474,
#24475,#24476,#24477,#24478,#24479,#24480,#24481,#24482,#24483,#24484,#24485,
#24486,#24487,#24488,#24489,#24490,#24491,#24492,#24493,#24494,#24495,#24496,
#24497,#24498,#24499,#24500,#24501,#24502,#24503,#24504,#24505,#24506,#24507,
#24508,#24509,#24510,#24511,#24512,#24513,#24514,#24515,#24516,#24517,#24518,
#24519,#24520,#24521,#24522,#24523,#24524,#24525,#24526,#24527,#24528,#24529),
 .UNSPECIFIED.,.F.,.F.,(4,3,3,3,3,3,3,3,3,3,3,3,3,3,3,3,3,3,3,3,3,3,3,3,
3,3,3,4),(15.7079632679489,15.8200553291365,15.9077986255125,15.9954301993008,
16.0829731472548,16.1739370920625,16.2613798278848,16.3488091818115,16.4362458908085,
16.5237106921039,16.6112724073114,16.6988915726886,16.7866367930526,16.8106847057165,
16.8985113458652,16.9862271592627,17.0738551349147,17.1647875033374,17.2523166917918,
17.3398328754298,17.4273566980425,17.5149088038202,17.6025576686082,17.6902639964774,
17.7780957334192,17.8013140822966,17.8891406047116,17.9338701936111),
 .UNSPECIFIED.);
#2029=B_SPLINE_CURVE_WITH_KNOTS('',3,(#24535,#24536,#24537,#24538,#24539,
#24540,#24541,#24542,#24543,#24544,#24545,#24546,#24547,#24548,#24549,#24550,
#24551,#24552,#24553,#24554,#24555,#24556,#24557,#24558,#24559,#24560,#24561,
#24562,#24563,#24564,#24565,#24566,#24567,#24568,#24569,#24570,#24571,#24572,
#24573,#24574,#24575,#24576,#24577,#24578,#24579,#24580,#24581,#24582,#24583,
#24584,#24585,#24586,#24587,#24588,#24589,#24590,#24591,#24592,#24593,#24594,
#24595,#24596,#24597,#24598,#24599,#24600,#24601,#24602,#24603,#24604,#24605,
#24606,#24607,#24608,#24609,#24610,#24611,#24612,#24613,#24614,#24615,#24616,
#24617,#24618,#24619,#24620,#24621,#24622,#24623,#24624,#24625,#24626,#24627,
#24628,#24629,#24630,#24631),.UNSPECIFIED.,.F.,.F.,(4,3,3,3,3,3,3,3,3,3,
3,3,3,3,3,3,3,3,3,3,3,3,3,3,3,3,3,3,3,3,3,3,4),(64.4958550710578,64.5877405518754,
64.6795367572376,64.7712749401722,64.8629839192416,64.9546874336248,65.0464092117959,
65.1382299601248,65.2301041586777,65.3221260934564,65.3815388542818,65.4728325704167,
65.5640050659998,65.655083664424,65.7461008284763,65.837086533478,65.9280653184272,
66.0190617110135,66.1101639042974,66.2013201136695,66.2926413727528,66.3721682308618,
66.4665065443583,66.560706841006,66.6547911225413,66.7487656647496,66.8426763541279,
66.9365429023764,67.0303849773091,67.1242488409515,67.218122240913,67.3120618969904,
67.3627976074418),.UNSPECIFIED.);
#2030=B_SPLINE_CURVE_WITH_KNOTS('',3,(#24639,#24640,#24641,#24642,#24643,
#24644,#24645,#24646,#24647,#24648,#24649,#24650,#24651,#24652,#24653,#24654,
#24655,#24656,#24657,#24658,#24659,#24660,#24661,#24662,#24663,#24664,#24665,
#24666,#24667,#24668,#24669,#24670,#24671,#24672,#24673,#24674,#24675,#24676,
#24677,#24678,#24679,#24680,#24681,#24682,#24683,#24684,#24685,#24686,#24687,
#24688,#24689,#24690,#24691,#24692,#24693,#24694,#24695,#24696,#24697,#24698,
#24699,#24700,#24701,#24702,#24703,#24704,#24705,#24706,#24707,#24708,#24709,
#24710,#24711,#24712,#24713,#24714,#24715,#24716,#24717,#24718,#24719,#24720,
#24721,#24722,#24723,#24724,#24725,#24726,#24727,#24728,#24729,#24730,#24731,
#24732,#24733,#24734,#24735,#24736,#24737,#24738,#24739,#24740,#24741,#24742,
#24743,#24744,#24745,#24746,#24747,#24748,#24749,#24750,#24751,#24752,#24753,
#24754,#24755,#24756,#24757,#24758,#24759,#24760,#24761,#24762,#24763,#24764,
#24765,#24766,#24767,#24768,#24769,#24770,#24771,#24772),.UNSPECIFIED.,
 .F.,.F.,(4,2,2,2,2,2,2,2,2,2,2,2,2,2,2,2,2,2,2,2,2,2,2,2,2,2,2,2,2,2,2,
2,2,2,2,2,2,2,2,2,2,2,2,2,2,2,2,2,2,2,2,2,2,2,2,2,2,2,2,2,2,2,2,2,2,2,4),
(-3.81628572195454,-3.80643866773546,-3.7289890269469,-3.69635642028847,
-3.67358696555601,-3.66320759461619,-3.65514947879411,-3.64613200947775,
-3.63063531030959,-3.55907881352723,-3.50755825416349,-3.49841117462634,
-3.49325168255072,-3.48862143572503,-3.48299898076068,-3.46907587129048,
-3.40635520315938,-3.35744886171428,-3.33831875457717,-3.32860719420934,
-3.32140484128649,-3.31228641200962,-3.29661977844063,-3.21096461869517,
-3.1695503074049,-3.16116346153608,-3.15621127170026,-3.15164116660213,
-3.14477432000345,-3.12611839396488,-3.06726478415051,-3.0201942606498,
-3.0012775305463,-2.99166579553305,-2.98453840907989,-2.97551984633461,
-2.96004985263678,-2.88696905702268,-2.83345567295407,-2.82454988046004,
-2.81951645394583,-2.81494804271254,-2.80940386974122,-2.7983829638169,
-2.73357372147411,-2.67347785362427,-2.65993518965042,-2.65136291329667,
-2.64324935287387,-2.6321021168385,-2.6056649026294,-2.52424439657405,-2.50434946360095,
-2.49082995178553,-2.48488795705161,-2.48038824328513,-2.47493942167255,
-2.46410293089154,-2.41853432457841,-2.37833645217606,-2.33545254736092,
-2.32278435908247,-2.314394627258,-2.30627661646385,-2.29644905848072,-2.27193380836389,
-2.2561223525901),.UNSPECIFIED.);
#2031=B_SPLINE_CURVE_WITH_KNOTS('',3,(#24778,#24779,#24780,#24781,#24782,
#24783,#24784,#24785,#24786,#24787,#24788,#24789,#24790,#24791,#24792,#24793,
#24794,#24795,#24796,#24797,#24798,#24799,#24800,#24801,#24802,#24803,#24804,
#24805,#24806,#24807,#24808,#24809,#24810,#24811,#24812,#24813,#24814,#24815,
#24816,#24817,#24818,#24819,#24820,#24821,#24822,#24823,#24824,#24825,#24826,
#24827,#24828,#24829,#24830,#24831,#24832,#24833,#24834,#24835,#24836,#24837,
#24838,#24839,#24840,#24841,#24842,#24843,#24844,#24845,#24846,#24847,#24848,
#24849,#24850,#24851,#24852,#24853,#24854,#24855,#24856,#24857,#24858,#24859,
#24860,#24861,#24862,#24863,#24864,#24865,#24866,#24867,#24868,#24869,#24870,
#24871,#24872,#24873,#24874,#24875,#24876,#24877,#24878,#24879,#24880,#24881,
#24882,#24883,#24884,#24885,#24886,#24887,#24888,#24889,#24890,#24891,#24892,
#24893,#24894,#24895,#24896,#24897,#24898,#24899,#24900,#24901,#24902,#24903,
#24904,#24905,#24906,#24907,#24908,#24909,#24910,#24911,#24912,#24913,#24914,
#24915,#24916,#24917,#24918,#24919,#24920,#24921,#24922,#24923,#24924,#24925,
#24926,#24927,#24928,#24929,#24930,#24931,#24932,#24933,#24934,#24935,#24936,
#24937,#24938,#24939,#24940,#24941,#24942,#24943,#24944,#24945,#24946,#24947,
#24948,#24949,#24950,#24951,#24952,#24953,#24954,#24955,#24956,#24957),
 .UNSPECIFIED.,.F.,.F.,(4,2,2,2,2,2,2,2,2,2,2,2,2,2,2,2,2,2,2,2,2,2,2,2,
2,2,2,2,2,2,2,2,2,2,2,2,2,2,2,2,2,2,2,2,2,2,2,2,2,2,2,2,2,2,2,2,2,2,2,2,
2,2,2,2,2,2,2,2,2,2,2,2,2,2,2,2,2,2,2,2,2,2,2,2,2,2,2,2,2,4),(-2.01531219133444,
-1.97096131187465,-1.94756113517625,-1.94012698067682,-1.93585896379917,
-1.93117853264063,-1.92401861146501,-1.90127538153087,-1.85608032338612,
-1.7953930822805,-1.77945826407955,-1.77031186389807,-1.76235986603929,
-1.75241944841608,-1.73187216898625,-1.7036030330738,-1.63827855192118,
-1.61166123377425,-1.60392378503505,-1.59912260304415,-1.59439272034915,
-1.58697909918242,-1.56155070245692,-1.50514178477934,-1.45364292800775,
-1.4402684875885,-1.43174241624239,-1.42363150611853,-1.41242250868104,
-1.38366511411774,-1.33624150178711,-1.28002778215006,-1.26961715772864,
-1.26419204985738,-1.25970042936202,-1.25375555082318,-1.24017236639701,
-1.22013779695266,-1.13714097247456,-1.11180009033715,-1.10185986700301,
-1.09371496844786,-1.08536373188661,-1.07288434001335,-1.03233235013473,
-0.990736192507835,-0.940181824435997,-0.931553161911691,-0.926558014688438,
-0.921941243659147,-0.91514398324735,-0.89569732817667,-0.861273493568097,
-0.784285653885893,-0.769118888227675,-0.760212979008701,-0.752212948901535,
-0.741854731159591,-0.718910832501713,-0.685777787176493,-0.621731810715002,
-0.601004644388216,-0.593859184212681,-0.589646692354204,-0.584937044622535,
-0.57754343499821,-0.552081844565888,-0.495521376069438,-0.443741022768495,
-0.430382057575451,-0.421885099929604,-0.413817257681648,-0.402695451495442,
-0.374366526264463,-0.32808343751111,-0.270131437119352,-0.259755235098674,
-0.254347945347254,-0.249852551390498,-0.243889204688283,-0.230266639408721,
-0.210171112010424,-0.130796095410969,-0.10267291099376,-0.0912231649876788,
-0.0831159360069332,-0.0746101682316521,-0.065963232373048,-0.0534862628334782,
-0.00100290464424951),.UNSPECIFIED.);
#2032=B_SPLINE_CURVE_WITH_KNOTS('',3,(#24958,#24959,#24960,#24961,#24962,
#24963,#24964,#24965,#24966,#24967,#24968,#24969,#24970,#24971,#24972,#24973),
 .UNSPECIFIED.,.F.,.F.,(4,3,3,3,3,4),(64.140690693207,64.2575058528083,
64.3766585668236,64.3909094777018,64.4829385165591,64.4958550710578),
 .UNSPECIFIED.);
#2033=B_SPLINE_CURVE_WITH_KNOTS('',3,(#24974,#24975,#24976,#24977,#24978,
#24979,#24980,#24981,#24982,#24983,#24984,#24985,#24986,#24987,#24988,#24989,
#24990,#24991,#24992,#24993,#24994,#24995,#24996,#24997,#24998,#24999,#25000,
#25001,#25002,#25003,#25004,#25005,#25006,#25007,#25008,#25009,#25010,#25011,
#25012,#25013,#25014,#25015,#25016,#25017,#25018,#25019,#25020,#25021,#25022,
#25023,#25024,#25025,#25026,#25027,#25028,#25029,#25030,#25031,#25032,#25033,
#25034,#25035,#25036,#25037,#25038,#25039,#25040,#25041,#25042,#25043,#25044,
#25045,#25046,#25047,#25048,#25049,#25050,#25051,#25052,#25053,#25054,#25055,
#25056,#25057,#25058,#25059,#25060,#25061,#25062,#25063,#25064,#25065,#25066,
#25067,#25068,#25069,#25070,#25071,#25072,#25073,#25074,#25075,#25076,#25077,
#25078,#25079,#25080,#25081,#25082,#25083,#25084,#25085,#25086,#25087,#25088,
#25089,#25090,#25091,#25092,#25093,#25094,#25095,#25096,#25097,#25098,#25099,
#25100,#25101,#25102,#25103,#25104,#25105,#25106,#25107,#25108,#25109,#25110,
#25111,#25112,#25113,#25114,#25115,#25116,#25117,#25118,#25119,#25120,#25121,
#25122,#25123,#25124,#25125,#25126,#25127,#25128,#25129,#25130,#25131,#25132,
#25133,#25134,#25135,#25136,#25137,#25138,#25139,#25140,#25141,#25142,#25143,
#25144,#25145,#25146,#25147,#25148,#25149,#25150,#25151,#25152,#25153,#25154,
#25155,#25156,#25157,#25158,#25159,#25160,#25161,#25162,#25163),
 .UNSPECIFIED.,.F.,.F.,(4,2,2,2,2,2,2,2,2,2,2,2,2,2,2,2,2,2,2,2,2,2,2,2,
2,2,2,2,2,2,2,2,2,2,2,2,2,2,2,2,2,2,2,2,2,2,2,2,2,2,2,2,2,2,2,2,2,2,2,2,
2,2,2,2,2,2,2,2,2,2,2,2,2,2,2,2,2,2,2,2,2,2,2,2,2,2,2,2,2,2,2,2,2,2,4),
(-2.2561223525901,-2.18794493316781,-2.16784145467791,-2.15422362973131,
-2.14827233054965,-2.14377949514829,-2.1383574728123,-2.12763696378004,
-2.07557068505986,-2.02542814297983,-1.99574320518035,-1.98441137185593,
-1.97627866777529,-1.96778863923089,-1.95459516740641,-1.90824864460455,
-1.89817232295126,-1.84077040935874,-1.82031324231676,-1.8132018540541,
-1.80899524807701,-1.80424703975124,-1.79675841565914,-1.77051407282385,
-1.71005738041494,-1.66326870247198,-1.6500470236948,-1.64154701615231,
-1.63341026123651,-1.62208140725898,-1.59245367695536,-1.54248569914341,
-1.49027052229501,-1.47955910320356,-1.47413652359918,-1.46964222528885,
-1.46368601126918,-1.45003657433854,-1.42986341020308,-1.3449342106813,
-1.32115512340047,-1.31144513322938,-1.30335826944968,-1.2949329915766,
-1.28207363598626,-1.23646386735105,-1.22321428986379,-1.16289446283588,
-1.14605691371847,-1.13943804721623,-1.1349042727704,-1.12986844816081,
-1.12103714641948,-1.06611443058207,-0.994986364904734,-0.979376181905608,
-0.970300594820869,-0.96313886242011,-0.953492839907699,-0.93454392951832,
-0.887477121232493,-0.828581870965259,-0.810035182976642,-0.80316990231603,
-0.798593420351695,-0.793649828027475,-0.785249947783325,-0.742837271944505,
-0.671029293352246,-0.647770207755661,-0.637195310418267,-0.629151311747035,
-0.620455931256036,-0.606272863559826,-0.54151183771968,-0.479609055870956,
-0.469567961823065,-0.464219184322762,-0.45971757121563,-0.453661550533784,
-0.439401333543605,-0.41792941366668,-0.369125605709504,-0.317542713439205,
-0.30405674825885,-0.295504788460245,-0.287400283035914,-0.276250164385121,
-0.247956891016996,-0.201846031289555,-0.143710562412784,-0.133296880966846,
-0.127869765806824,-0.123377778264526,-0.121332009443736),.UNSPECIFIED.);
#2034=B_SPLINE_CURVE_WITH_KNOTS('',3,(#25168,#25169,#25170,#25171,#25172,
#25173,#25174,#25175,#25176,#25177,#25178,#25179,#25180,#25181,#25182,#25183,
#25184,#25185,#25186,#25187,#25188,#25189,#25190,#25191,#25192,#25193,#25194,
#25195,#25196,#25197,#25198,#25199,#25200,#25201,#25202,#25203,#25204,#25205,
#25206,#25207,#25208,#25209,#25210,#25211,#25212,#25213,#25214,#25215,#25216,
#25217,#25218,#25219,#25220,#25221,#25222,#25223,#25224,#25225,#25226,#25227,
#25228,#25229,#25230,#25231,#25232,#25233,#25234,#25235,#25236,#25237,#25238,
#25239,#25240,#25241,#25242,#25243,#25244,#25245,#25246,#25247,#25248,#25249,
#25250,#25251,#25252,#25253,#25254,#25255,#25256,#25257,#25258,#25259,#25260,
#25261,#25262,#25263,#25264,#25265,#25266,#25267,#25268,#25269,#25270,#25271,
#25272,#25273,#25274,#25275,#25276,#25277,#25278,#25279,#25280,#25281,#25282,
#25283,#25284,#25285,#25286,#25287,#25288,#25289,#25290,#25291,#25292,#25293,
#25294,#25295,#25296,#25297,#25298,#25299,#25300,#25301,#25302,#25303,#25304,
#25305,#25306,#25307,#25308,#25309,#25310,#25311,#25312,#25313,#25314,#25315,
#25316,#25317,#25318,#25319,#25320,#25321,#25322,#25323,#25324,#25325,#25326,
#25327,#25328,#25329,#25330,#25331,#25332,#25333,#25334,#25335,#25336,#25337,
#25338,#25339,#25340,#25341,#25342,#25343,#25344,#25345,#25346,#25347,#25348,
#25349,#25350,#25351,#25352,#25353,#25354,#25355,#25356,#25357,#25358,#25359),
 .UNSPECIFIED.,.F.,.F.,(4,2,2,2,2,2,2,2,2,2,2,2,2,2,2,2,2,2,2,2,2,2,2,2,
2,2,2,2,2,2,2,2,2,2,2,2,2,2,2,2,2,2,2,2,2,2,2,2,2,2,2,2,2,2,2,2,2,2,2,2,
2,2,2,2,2,2,2,2,2,2,2,2,2,2,2,2,2,2,2,2,2,2,2,2,2,2,2,2,2,2,2,2,2,2,2,4),
(-4.14997297189533,-4.14175280985412,-4.13037581294682,-4.12223295960013,
-4.11375152378661,-4.10061097619511,-4.05524450759479,-3.99356736209229,
-3.96709865418571,-3.95959235541146,-3.95484099186147,-3.95063549212644,
-3.94353654203057,-3.92319554151643,-3.86570010853809,-3.81412382355199,
-3.79835311594367,-3.78933105270749,-3.78136549577479,-3.77124412373233,
-3.74965750732048,-3.67556716598835,-3.63231136666082,-3.62388542106676,
-3.61893613379583,-3.61436226395951,-3.6075125494846,-3.58908242772295,
-3.52272435917552,-3.48920764799781,-3.46609479234241,-3.45571694454457,
-3.44772376651123,-3.43884840681707,-3.42379430597422,-3.34567611473376,
-3.31168948387026,-3.2923933633627,-3.28562337163558,-3.28101831218048,
-3.27602491719038,-3.26739292921559,-3.21666532276177,-3.17490649941335,
-3.13454377999092,-3.12208197223847,-3.11373638625083,-3.10559262176385,
-3.09375529190372,-3.06254761665708,-2.98649192995047,-2.96703260199048,
-2.9537273454854,-2.94783011469683,-2.94338221750868,-2.93793826692684,
-2.92711143942573,-2.88161821217879,-2.84160645049755,-2.79846740250153,
-2.78578352559344,-2.77739365405816,-2.76928310847887,-2.7594740325812,
-2.73505907295769,-2.65099954408003,-2.63089631075354,-2.61727987405498,
-2.61132973271163,-2.60683699047224,-2.60141327344442,-2.59101639031986,
-2.53442580253256,-2.48719093474166,-2.45849676747668,-2.44729230058081,
-2.43917868153043,-2.43064426261403,-2.41724435874358,-2.36459778103599,
-2.31678983370526,-2.29528955557359,-2.28101511737841,-2.27495678142308,
-2.27045484688171,-2.26510755064471,-2.25507378871593,-2.19290431935607,
-2.13594938551761,-2.11923113358561,-2.1090566243364,-2.10108555629539,
-2.09209533465508,-2.07648189546139,-2.02609908967989,-2.01531219133444),
 .UNSPECIFIED.);
#2035=B_SPLINE_CURVE_WITH_KNOTS('',3,(#25361,#25362,#25363,#25364,#25365,
#25366,#25367,#25368,#25369,#25370),.UNSPECIFIED.,.F.,.F.,(4,2,2,2,4),(-0.121332009443736,
-0.117433076213923,-0.103846755183921,-0.0838035258490438,-0.000973468615732111),
 .UNSPECIFIED.);
#2036=B_SPLINE_CURVE_WITH_KNOTS('',3,(#25371,#25372,#25373,#25374,#25375,
#25376,#25377,#25378,#25379,#25380,#25381,#25382,#25383,#25384,#25385,#25386,
#25387,#25388,#25389,#25390,#25391,#25392,#25393,#25394,#25395,#25396,#25397,
#25398,#25399,#25400,#25401,#25402,#25403,#25404,#25405,#25406,#25407,#25408,
#25409,#25410,#25411,#25412,#25413,#25414,#25415,#25416,#25417,#25418,#25419,
#25420,#25421,#25422,#25423,#25424,#25425,#25426,#25427,#25428,#25429,#25430,
#25431,#25432,#25433,#25434,#25435,#25436,#25437,#25438,#25439,#25440,#25441,
#25442,#25443,#25444,#25445,#25446,#25447,#25448,#25449,#25450,#25451,#25452,
#25453,#25454,#25455,#25456,#25457,#25458,#25459,#25460,#25461,#25462,#25463,
#25464,#25465,#25466,#25467,#25468,#25469,#25470,#25471,#25472,#25473,#25474,
#25475,#25476,#25477,#25478,#25479,#25480,#25481,#25482,#25483,#25484,#25485,
#25486,#25487,#25488,#25489,#25490,#25491,#25492,#25493,#25494,#25495,#25496,
#25497,#25498,#25499,#25500,#25501,#25502,#25503,#25504,#25505,#25506,#25507,
#25508,#25509,#25510,#25511,#25512,#25513,#25514,#25515,#25516,#25517,#25518,
#25519,#25520,#25521,#25522,#25523,#25524,#25525,#25526,#25527,#25528,#25529,
#25530,#25531,#25532,#25533,#25534,#25535,#25536,#25537,#25538,#25539,#25540,
#25541,#25542,#25543,#25544,#25545,#25546,#25547,#25548,#25549,#25550),
 .UNSPECIFIED.,.F.,.F.,(4,2,2,2,2,2,2,2,2,2,2,2,2,2,2,2,2,2,2,2,2,2,2,2,
2,2,2,2,2,2,2,2,2,2,2,2,2,2,2,2,2,2,2,2,2,2,2,2,2,2,2,2,2,2,2,2,2,2,2,2,
2,2,2,2,2,2,2,2,2,2,2,2,2,2,2,2,2,2,2,2,2,2,2,2,2,2,2,2,2,4),(-4.27052942922916,
-4.25429608667662,-4.24189246233734,-4.23394077902904,-4.22637806059236,
-4.21788881580779,-4.20471119481784,-4.15669264777507,-4.09273857851959,
-4.07044249891397,-4.06333035151339,-4.05866025259778,-4.05438312449549,
-4.04690037690266,-4.02298512396386,-3.9619226238932,-3.92931818631836,
-3.90663328978521,-3.89632577966203,-3.88834058971791,-3.87942704856534,
-3.86418783388835,-3.78754415413371,-3.75277100860208,-3.73320376740374,
-3.72640049481753,-3.72178935922745,-3.71680797056926,-3.70823233804472,
-3.65874078138611,-3.61839519129027,-3.58981122413048,-3.56910490693356,
-3.55913713158848,-3.55125708078362,-3.54215973658435,-3.52645005771721,
-3.44140062524049,-3.39977130676857,-3.39139790766936,-3.38645964699668,
-3.38187920586303,-3.37499521014691,-3.35631764829852,-3.29020497394183,
-3.25672740134996,-3.23363211907124,-3.22325655728246,-3.21526304321925,
-3.20638518967482,-3.19132148289614,-3.11326159206311,-3.07923831950518,
-3.0599288293698,-3.05315679855113,-3.04855106943138,-3.04355775160095,
-3.03492742643413,-2.98424479437167,-2.94252974762593,-2.90207995312105,
-2.88961004440993,-2.88126237069658,-2.8731190523521,-2.86128689714784,
-2.83012900129916,-2.75400889655473,-2.73454282862846,-2.72123399018241,
-2.71533586833474,-2.7108876553485,-2.70544381965799,-2.69461841189559,
-2.6491539582444,-2.59445299180117,-2.57335947109049,-2.55676425383213,
-2.54757474456073,-2.5396276892574,-2.52974884828246,-2.50954160536983,
-2.41915711567073,-2.39863016650045,-2.38481135655669,-2.37882708512889,
-2.37433114919786,-2.36893101188502,-2.3583292058588,-2.30335561144317,
-2.25592392382822),.UNSPECIFIED.);
#2037=B_SPLINE_CURVE_WITH_KNOTS('',3,(#25556,#25557,#25558,#25559,#25560,
#25561,#25562,#25563,#25564,#25565,#25566,#25567,#25568,#25569,#25570,#25571,
#25572,#25573,#25574,#25575,#25576,#25577,#25578,#25579,#25580,#25581,#25582,
#25583,#25584,#25585,#25586,#25587,#25588,#25589,#25590,#25591,#25592,#25593,
#25594,#25595,#25596,#25597,#25598,#25599,#25600,#25601,#25602,#25603,#25604,
#25605,#25606,#25607,#25608,#25609,#25610,#25611,#25612,#25613,#25614,#25615,
#25616,#25617,#25618,#25619,#25620,#25621,#25622,#25623,#25624,#25625,#25626,
#25627,#25628,#25629,#25630,#25631,#25632,#25633,#25634,#25635,#25636,#25637,
#25638,#25639,#25640,#25641,#25642,#25643,#25644,#25645,#25646,#25647,#25648,
#25649,#25650,#25651,#25652,#25653,#25654,#25655,#25656,#25657,#25658,#25659,
#25660,#25661,#25662,#25663,#25664,#25665,#25666,#25667,#25668,#25669,#25670,
#25671,#25672,#25673,#25674,#25675,#25676,#25677,#25678,#25679,#25680,#25681,
#25682,#25683,#25684,#25685,#25686,#25687,#25688,#25689,#25690,#25691,#25692,
#25693,#25694,#25695,#25696,#25697,#25698,#25699,#25700,#25701,#25702,#25703,
#25704,#25705,#25706,#25707,#25708,#25709,#25710,#25711,#25712,#25713,#25714,
#25715,#25716,#25717,#25718,#25719,#25720,#25721,#25722,#25723,#25724,#25725,
#25726,#25727,#25728,#25729,#25730,#25731,#25732,#25733,#25734,#25735),
 .UNSPECIFIED.,.F.,.F.,(4,2,2,2,2,2,2,2,2,2,2,2,2,2,2,2,2,2,2,2,2,2,2,2,
2,2,2,2,2,2,2,2,2,2,2,2,2,2,2,2,2,2,2,2,2,2,2,2,2,2,2,2,2,2,2,2,2,2,2,2,
2,2,2,2,2,2,2,2,2,2,2,2,2,2,2,2,2,2,2,2,2,2,2,2,2,2,2,2,2,4),(-2.01483558329388,
-1.98146997080009,-1.9013990607951,-1.88509494854619,-1.87587112226953,
-1.86792759796362,-1.85809598862794,-1.83814631598668,-1.81102482899631,
-1.76935892470915,-1.7187272628708,-1.71009908524082,-1.70510649637509,
-1.70050108304905,-1.69372891065386,-1.674416017502,-1.64037990843735,-1.56228782284944,
-1.54722317896616,-1.53834566574842,-1.5303530491234,-1.5199794815247,-1.49689167240493,
-1.46343162693712,-1.39734653935908,-1.3786915508109,-1.37181125363298,
-1.36723185993088,-1.36229324201418,-1.35391632785418,-1.31218521735816,
-1.22725870489533,-1.21151793100958,-1.20241466060299,-1.19453648803323,
-1.18458036031997,-1.16393443449333,-1.13546984099662,-1.09503163767455,
-1.04551525724752,-1.03693915802589,-1.03195810524928,-1.02734787554124,
-1.02054666436825,-1.00099204092101,-0.966251665472124,-0.889497804930624,
-0.874268311749744,-0.865357625128378,-0.857373361616169,-0.84706473601712,
-0.824366315493667,-0.791734014558436,-0.730439506069875,-0.706837621557959,
-0.699385320367477,-0.695114480357264,-0.690439835975098,-0.683302146968559,
-0.660756391237086,-0.616280905357298,-0.554591487400057,-0.538669151672547,
-0.529527229051855,-0.521577711713218,-0.511638641921982,-0.491087788238012,
-0.462808205106245,-0.397376080178613,-0.37088946344326,-0.363163975281902,
-0.358365921414574,-0.353631480009471,-0.346203280632927,-0.320633563231771,
-0.263539306729855,-0.212920748432954,-0.199566083306558,-0.191041640922275,
-0.182924372277182,-0.171693313924057,-0.142789756659854,-0.0949498372545458,
-0.0645510533513762,-0.0348535101730009,-0.026907829164859,-0.0220624118465178,
-0.0178631925402166,-0.0131574371654451,-0.000968299569621017),
 .UNSPECIFIED.);
#2038=B_SPLINE_CURVE_WITH_KNOTS('',3,(#25736,#25737,#25738,#25739,#25740,
#25741),.UNSPECIFIED.,.F.,.F.,(4,2,4),(-4.27074430843839,-4.17177255499699,
-4.14997297189533),.UNSPECIFIED.);
#2039=B_SPLINE_CURVE_WITH_KNOTS('',3,(#25742,#25743,#25744,#25745,#25746,
#25747,#25748,#25749,#25750,#25751,#25752,#25753,#25754,#25755,#25756,#25757,
#25758,#25759,#25760,#25761,#25762,#25763,#25764,#25765,#25766,#25767,#25768,
#25769,#25770,#25771,#25772,#25773,#25774,#25775,#25776,#25777,#25778,#25779,
#25780,#25781,#25782,#25783,#25784,#25785,#25786,#25787,#25788,#25789,#25790,
#25791,#25792,#25793,#25794,#25795,#25796,#25797,#25798,#25799,#25800,#25801,
#25802,#25803,#25804,#25805,#25806,#25807,#25808,#25809,#25810,#25811,#25812,
#25813,#25814,#25815,#25816,#25817,#25818,#25819,#25820,#25821,#25822,#25823,
#25824,#25825,#25826,#25827,#25828,#25829,#25830,#25831,#25832,#25833,#25834,
#25835,#25836,#25837,#25838,#25839,#25840,#25841,#25842,#25843,#25844,#25845,
#25846,#25847,#25848,#25849,#25850,#25851,#25852,#25853,#25854,#25855,#25856,
#25857,#25858,#25859,#25860,#25861,#25862,#25863,#25864,#25865,#25866,#25867,
#25868,#25869,#25870,#25871,#25872,#25873,#25874,#25875,#25876,#25877,#25878,
#25879,#25880,#25881,#25882,#25883,#25884,#25885,#25886,#25887,#25888,#25889,
#25890,#25891,#25892,#25893,#25894,#25895,#25896,#25897,#25898,#25899,#25900,
#25901,#25902,#25903,#25904,#25905,#25906,#25907,#25908,#25909,#25910,#25911,
#25912,#25913,#25914,#25915,#25916,#25917,#25918,#25919,#25920,#25921,#25922,
#25923,#25924,#25925,#25926,#25927,#25928,#25929,#25930,#25931,#25932,#25933,
#25934,#25935),.UNSPECIFIED.,.F.,.F.,(4,2,2,2,2,2,2,2,2,2,2,2,2,2,2,2,2,
2,2,2,2,2,2,2,2,2,2,2,2,2,2,2,2,2,2,2,2,2,2,2,2,2,2,2,2,2,2,2,2,2,2,2,2,
2,2,2,2,2,2,2,2,2,2,2,2,2,2,2,2,2,2,2,2,2,2,2,2,2,2,2,2,2,2,2,2,2,2,2,2,
2,2,2,2,2,2,2,4),(-2.25592392382822,-2.25509772448687,-2.22604616088193,
-2.2147931936834,-2.20667046526772,-2.19814949501622,-2.18481979597181,
-2.13515473211171,-2.06928391620988,-2.05040305233839,-2.04349142525006,
-2.03890564972634,-2.03397616402601,-2.02564434418445,-1.98519838365541,
-1.89804659705601,-1.88275775494733,-1.87375049727423,-1.86578182040898,
-1.85563434551231,-1.83389918493884,-1.80326680949065,-1.78895291866272,
-1.72636402023525,-1.71223008409015,-1.70660547898419,-1.70205886177658,
-1.69705307334562,-1.68836334520215,-1.63267645076848,-1.56213408797115,
-1.54648335400425,-1.53739885166856,-1.52951760645157,-1.51953197034122,
-1.49872281005177,-1.46993969556415,-1.42987384975932,-1.38436881565051,
-1.3735413800765,-1.36809765563457,-1.36365022117063,-1.35775393485197,
-1.34445274399215,-1.3249993145377,-1.24906216761986,-1.21770995572906,
-1.20585609420836,-1.19844969266466,-1.19024380732931,-1.17851142796023,
-1.14552960020076,-1.08405886506413,-1.04375992626897,-1.03531772755092,
-1.03036519774514,-1.02573955510586,-1.0188557138071,-0.998611340913551,
-0.961807728180398,-0.888710974307031,-0.873265031959592,-0.864224769029754,
-0.857058841488895,-0.847365324935507,-0.828162119087105,-0.778739690749397,
-0.715111736795599,-0.701762200208794,-0.695920275116706,-0.691428623404823,
-0.686000538516135,-0.675252405452841,-0.632026708672024,-0.550141623298073,
-0.535601750725324,-0.526833217318771,-0.51881386196569,-0.508222603528512,
-0.483765704786974,-0.447274539175102,-0.392165484605573,-0.368738970813097,
-0.361303430491097,-0.35703583624684,-0.352358179246472,-0.345205180855147,
-0.3225106488646,-0.277490393886692,-0.216546810538548,-0.200615633642746,
-0.19147192401294,-0.183522738882751,-0.173586563679768,-0.153051329620543,
-0.124801908219954,-0.121337432739625),.UNSPECIFIED.);
#2040=B_SPLINE_CURVE_WITH_KNOTS('',3,(#25940,#25941,#25942,#25943,#25944,
#25945,#25946,#25947,#25948,#25949,#25950,#25951,#25952,#25953,#25954,#25955,
#25956,#25957,#25958,#25959,#25960,#25961,#25962,#25963,#25964,#25965,#25966,
#25967,#25968,#25969,#25970,#25971,#25972,#25973,#25974,#25975,#25976,#25977,
#25978,#25979,#25980,#25981,#25982,#25983,#25984,#25985,#25986,#25987,#25988,
#25989,#25990,#25991,#25992,#25993,#25994,#25995,#25996,#25997,#25998,#25999,
#26000,#26001,#26002,#26003,#26004,#26005,#26006,#26007,#26008,#26009,#26010,
#26011,#26012,#26013,#26014,#26015,#26016,#26017,#26018,#26019,#26020,#26021,
#26022,#26023,#26024,#26025,#26026,#26027,#26028,#26029,#26030,#26031,#26032,
#26033,#26034,#26035,#26036,#26037,#26038,#26039,#26040,#26041,#26042,#26043,
#26044,#26045,#26046,#26047,#26048,#26049,#26050,#26051,#26052,#26053,#26054,
#26055,#26056,#26057,#26058,#26059,#26060,#26061,#26062,#26063,#26064,#26065,
#26066,#26067,#26068,#26069,#26070,#26071,#26072,#26073,#26074,#26075,#26076,
#26077,#26078,#26079,#26080,#26081,#26082,#26083,#26084,#26085,#26086,#26087,
#26088,#26089,#26090,#26091,#26092,#26093,#26094,#26095,#26096,#26097,#26098,
#26099,#26100,#26101,#26102,#26103,#26104,#26105,#26106,#26107,#26108,#26109,
#26110,#26111,#26112,#26113,#26114,#26115,#26116,#26117,#26118,#26119,#26120,
#26121,#26122,#26123,#26124,#26125,#26126,#26127,#26128,#26129,#26130,#26131,
#26132,#26133),.UNSPECIFIED.,.F.,.F.,(4,2,2,2,2,2,2,2,2,2,2,2,2,2,2,2,2,
2,2,2,2,2,2,2,2,2,2,2,2,2,2,2,2,2,2,2,2,2,2,2,2,2,2,2,2,2,2,2,2,2,2,2,2,
2,2,2,2,2,2,2,2,2,2,2,2,2,2,2,2,2,2,2,2,2,2,2,2,2,2,2,2,2,2,2,2,2,2,2,2,
2,2,2,2,2,2,2,4),(-4.14962318045641,-4.1028957960099,-4.08275900568692,
-4.06912658694941,-4.06317385603533,-4.0586808858808,-4.0532588951427,-4.04254418367616,
-3.99908569264534,-3.96184529779788,-3.93011045994395,-3.9078403237579,
-3.89760179270109,-3.88962379880533,-3.88067061621028,-3.86523959745287,
-3.79024039014005,-3.75455682673976,-3.73468134476241,-3.72784069100265,
-3.7232225535565,-3.71825409106203,-3.70973957344812,-3.66381801838261,
-3.60658244311081,-3.57472885223454,-3.56312605608663,-3.55494288680084,
-3.54652272604857,-3.53368745502535,-3.49270668607016,-3.42685734092462,
-3.40842353150009,-3.39562367392045,-3.38981395054324,-3.3853295905105,
-3.37979394882608,-3.36849150217141,-3.30279723580273,-3.24230950096875,
-3.22877073103537,-3.22020776403621,-3.21210828654061,-3.20099001525198,
-3.17474106010809,-3.0928213271413,-3.07287792515606,-3.05933836039104,
-3.05340129179138,-3.04890953367263,-3.04347597965416,-3.03270210301197,
-2.98804432518389,-2.94981852831422,-2.91940699686237,-2.89778214898395,
-2.88765353987126,-2.87968669941273,-2.8706678483747,-2.85532494797824,
-2.7812012098716,-2.74502247619566,-2.72498228424258,-2.71812207451106,
-2.71350036536338,-2.70853880595768,-2.70005630817717,-2.65817569796323,
-2.59789249244724,-2.56521190653692,-2.55351264110632,-2.54531207950257,
-2.53789891706674,-2.52791603502456,-2.50204181511961,-2.41971468496225,
-2.39973982716349,-2.38618501249799,-2.38024525794339,-2.37575317598825,
-2.37032132615861,-2.35988651544004,-2.30402094495244,-2.25633609613713,
-2.22748416951023,-2.216258275786,-2.20814066078074,-2.19961225283119,-2.18624359390648,
-2.13506495998405,-2.06320870499089,-2.04961366545058,-2.04373013050453,
-2.03923443671887,-2.0338363107999,-2.02324313951954,-2.01483558329388),
 .UNSPECIFIED.);
#2041=B_SPLINE_CURVE_WITH_KNOTS('',3,(#26135,#26136,#26137,#26138,#26139,
#26140,#26141,#26142,#26143,#26144,#26145,#26146,#26147,#26148,#26149,#26150),
 .UNSPECIFIED.,.F.,.F.,(4,2,2,2,2,2,2,4),(-0.121337432739625,-0.0618078407377174,
-0.0331277321209469,-0.0252541111211411,-0.0204242108037896,-0.0162322866714006,
-0.0115143057840549,-0.000968283308026432),.UNSPECIFIED.);
#2042=B_SPLINE_CURVE_WITH_KNOTS('',3,(#26151,#26152,#26153,#26154,#26155,
#26156,#26157,#26158,#26159,#26160,#26161,#26162,#26163,#26164,#26165,#26166,
#26167,#26168,#26169,#26170,#26171,#26172,#26173,#26174,#26175,#26176,#26177,
#26178,#26179,#26180,#26181,#26182,#26183,#26184,#26185,#26186,#26187,#26188,
#26189,#26190,#26191,#26192,#26193,#26194,#26195,#26196,#26197,#26198,#26199,
#26200,#26201,#26202,#26203,#26204,#26205,#26206,#26207,#26208,#26209,#26210,
#26211,#26212,#26213,#26214,#26215,#26216,#26217,#26218,#26219,#26220,#26221,
#26222,#26223,#26224,#26225,#26226,#26227,#26228,#26229,#26230,#26231,#26232,
#26233,#26234,#26235,#26236,#26237,#26238,#26239,#26240,#26241,#26242,#26243,
#26244,#26245,#26246,#26247,#26248,#26249,#26250,#26251,#26252,#26253,#26254,
#26255,#26256,#26257,#26258,#26259,#26260,#26261,#26262,#26263,#26264,#26265,
#26266,#26267,#26268,#26269,#26270,#26271,#26272,#26273,#26274,#26275,#26276,
#26277,#26278,#26279,#26280,#26281,#26282,#26283,#26284,#26285,#26286,#26287,
#26288,#26289,#26290,#26291,#26292,#26293,#26294,#26295,#26296,#26297,#26298,
#26299,#26300,#26301,#26302,#26303,#26304,#26305,#26306,#26307,#26308,#26309,
#26310,#26311,#26312,#26313,#26314,#26315,#26316,#26317,#26318,#26319,#26320,
#26321,#26322,#26323,#26324,#26325,#26326),.UNSPECIFIED.,.F.,.F.,(4,2,2,
2,2,2,2,2,2,2,2,2,2,2,2,2,2,2,2,2,2,2,2,2,2,2,2,2,2,2,2,2,2,2,2,2,2,2,2,
2,2,2,2,2,2,2,2,2,2,2,2,2,2,2,2,2,2,2,2,2,2,2,2,2,2,2,2,2,2,2,2,2,2,2,2,
2,2,2,2,2,2,2,2,2,2,2,2,4),(-4.27088769108607,-4.20004372531903,-4.14914235892196,
-4.13345932591378,-4.12445452384894,-4.11648529184639,-4.10633337336792,
-4.08457294509138,-3.99632771463989,-3.97593631328513,-3.96218203730146,
-3.95620862655621,-3.95171370854859,-3.94630606005889,-3.93566562522522,
-3.88209760055788,-3.8329164599968,-3.80355051269102,-3.79225658557803,
-3.78412711381278,-3.77561918178471,-3.76235248873147,-3.71447525398381,
-3.65504464061249,-3.62900339592296,-3.62153293064927,-3.6167887482915,
-3.6119989428363,-3.60431519313883,-3.57812380107546,-3.51231833243977,
-3.4839748807748,-3.46339133305325,-3.45344491365451,-3.44549321287851,
-3.436352820761,-3.42044367120488,-3.35783884579242,-3.31405513001084,-3.291699619411,
-3.28458093032357,-3.27990932723283,-3.27563324685243,-3.26815678962916,
-3.24431268032594,-3.18318042327872,-3.15056237791546,-3.12787064523814,
-3.11756164931361,-3.10957592699966,-3.10066242502559,-3.08542491170151,
-3.00875537939623,-2.97399161419925,-2.95442714487183,-2.94762397493205,
-2.9430126787236,-2.93803084840681,-2.92945397631968,-2.87994016749372,
-2.83954993887013,-2.79689367558644,-2.78424620441127,-2.77586347760682,
-2.76774748335614,-2.75791658437811,-2.73336054434251,-2.66292898004654,
-2.62103789304483,-2.61265543376131,-2.60771519135555,-2.60313575224147,
-2.59625740450049,-2.57762166966302,-2.51146558949516,-2.47798053908104,
-2.45488169541337,-2.444505478082,-2.43651181103716,-2.42763414294334,-2.41257164953648,
-2.33450029544884,-2.30048227697617,-2.28117453168675,-2.2744026674282,
-2.26979693117235,-2.2648034725179,-2.2563897994296),.UNSPECIFIED.);
#2043=B_SPLINE_CURVE_WITH_KNOTS('',3,(#26332,#26333,#26334,#26335,#26336,
#26337,#26338,#26339,#26340,#26341,#26342,#26343,#26344,#26345,#26346,#26347,
#26348,#26349,#26350,#26351,#26352,#26353,#26354,#26355,#26356,#26357,#26358,
#26359,#26360,#26361,#26362,#26363,#26364,#26365,#26366,#26367,#26368,#26369,
#26370,#26371,#26372,#26373,#26374,#26375,#26376,#26377,#26378,#26379,#26380,
#26381,#26382,#26383,#26384,#26385,#26386,#26387,#26388,#26389,#26390,#26391,
#26392,#26393,#26394,#26395,#26396,#26397,#26398,#26399,#26400,#26401,#26402,
#26403,#26404,#26405,#26406,#26407,#26408,#26409,#26410,#26411,#26412,#26413,
#26414,#26415,#26416,#26417,#26418,#26419,#26420,#26421,#26422,#26423,#26424,
#26425,#26426,#26427,#26428,#26429,#26430,#26431,#26432,#26433,#26434,#26435,
#26436,#26437,#26438,#26439,#26440,#26441,#26442,#26443,#26444,#26445,#26446,
#26447,#26448,#26449,#26450,#26451,#26452,#26453,#26454,#26455,#26456,#26457,
#26458,#26459,#26460,#26461,#26462,#26463,#26464,#26465,#26466,#26467,#26468,
#26469,#26470,#26471,#26472,#26473,#26474,#26475,#26476,#26477,#26478,#26479,
#26480,#26481,#26482,#26483,#26484,#26485,#26486,#26487,#26488,#26489,#26490,
#26491,#26492,#26493,#26494,#26495,#26496,#26497,#26498,#26499,#26500,#26501,
#26502,#26503,#26504,#26505,#26506,#26507),.UNSPECIFIED.,.F.,.F.,(4,2,2,
2,2,2,2,2,2,2,2,2,2,2,2,2,2,2,2,2,2,2,2,2,2,2,2,2,2,2,2,2,2,2,2,2,2,2,2,
2,2,2,2,2,2,2,2,2,2,2,2,2,2,2,2,2,2,2,2,2,2,2,2,2,2,2,2,2,2,2,2,2,2,2,2,
2,2,2,2,2,2,2,2,2,2,2,2,4),(-2.01518237751153,-2.00712267182729,-1.99118164185661,
-1.98203396219234,-1.97408229311294,-1.96414428584733,-1.94361021744035,
-1.86818283021456,-1.82477456357156,-1.81627202923764,-1.81130564793156,
-1.8066853654038,-1.79983560130326,-1.77989048470612,-1.74400127065025,
-1.66927830353965,-1.65398749885286,-1.64497896036268,-1.63700907656819,
-1.62685996487116,-1.60512088576757,-1.57448259577334,-1.56016142804056,
-1.49755033751929,-1.48342800771361,-1.47780476550589,-1.47325798139218,
-1.46825028170607,-1.45955381381507,-1.40415589212679,-1.33327440080836,
-1.31764360669135,-1.3085625158484,-1.30139983486098,-1.29175690289879,
-1.27283051875749,-1.22620615384422,-1.16811132376968,-1.14856092222509,
-1.14156124308222,-1.13737299838398,-1.13259503869666,-1.12496641779449,
-1.09700639176037,-1.02650397903811,-0.989979396661249,-0.977603521736925,
-0.970106193280953,-0.961980596347843,-0.950708124087972,-0.921502356220064,
-0.872791769537386,-0.818514677423666,-0.80806324464688,-0.80262790350713,
-0.798136169257348,-0.792200997560694,-0.778673625854444,-0.758753957580906,
-0.677230124270598,-0.650589393444395,-0.639425461393946,-0.631318364546774,
-0.622770363894216,-0.609305026236667,-0.551308156133949,-0.490366365208866,
-0.474257389725327,-0.467756145605437,-0.463196460717531,-0.458092893110004,
-0.448941605778493,-0.395505074884607,-0.323317398358109,-0.30778705253575,
-0.29872841746435,-0.291564419957689,-0.281895001676472,-0.262822232408237,
-0.214022824110003,-0.151869558229802,-0.137260569222616,-0.13156168362851,
-0.126997564361412,-0.122030045159923,-0.113518120049323,-0.0671101170439002,
-0.000969905577444465),.UNSPECIFIED.);
#2044=B_SPLINE_CURVE_WITH_KNOTS('',3,(#26508,#26509,#26510,#26511,#26512,
#26513,#26514,#26515,#26516,#26517,#26518,#26519,#26520,#26521,#26522,#26523,
#26524,#26525),.UNSPECIFIED.,.F.,.F.,(4,2,2,2,2,2,2,2,4),(-4.27030726125859,
-4.25516597735123,-4.24333685644313,-4.23537379914972,-4.22781707357167,
-4.21934216175756,-4.20623630186715,-4.15957631638503,-4.14962318045641),
 .UNSPECIFIED.);
#2045=B_SPLINE_CURVE_WITH_KNOTS('',3,(#26526,#26527,#26528,#26529,#26530,
#26531,#26532,#26533,#26534,#26535,#26536,#26537,#26538,#26539,#26540,#26541,
#26542,#26543,#26544,#26545,#26546,#26547,#26548,#26549,#26550,#26551,#26552,
#26553,#26554,#26555,#26556,#26557,#26558,#26559,#26560,#26561,#26562,#26563,
#26564,#26565,#26566,#26567,#26568,#26569,#26570,#26571,#26572,#26573,#26574,
#26575,#26576,#26577,#26578,#26579,#26580,#26581,#26582,#26583,#26584,#26585,
#26586,#26587,#26588,#26589,#26590,#26591,#26592,#26593,#26594,#26595,#26596,
#26597,#26598,#26599,#26600,#26601,#26602,#26603,#26604,#26605,#26606,#26607,
#26608,#26609,#26610,#26611,#26612,#26613,#26614,#26615,#26616,#26617,#26618,
#26619,#26620,#26621,#26622,#26623,#26624,#26625,#26626,#26627,#26628,#26629,
#26630,#26631,#26632,#26633,#26634,#26635,#26636,#26637,#26638,#26639,#26640,
#26641,#26642,#26643,#26644,#26645,#26646,#26647,#26648,#26649,#26650,#26651,
#26652,#26653,#26654,#26655,#26656,#26657,#26658,#26659,#26660,#26661,#26662,
#26663,#26664,#26665,#26666,#26667,#26668,#26669,#26670,#26671,#26672,#26673,
#26674,#26675,#26676,#26677,#26678,#26679,#26680,#26681,#26682,#26683,#26684,
#26685,#26686,#26687,#26688,#26689,#26690,#26691,#26692,#26693,#26694,#26695,
#26696,#26697,#26698,#26699,#26700,#26701,#26702,#26703,#26704,#26705,#26706,
#26707,#26708,#26709,#26710,#26711,#26712,#26713),.UNSPECIFIED.,.F.,.F.,
(4,2,2,2,2,2,2,2,2,2,2,2,2,2,2,2,2,2,2,2,2,2,2,2,2,2,2,2,2,2,2,2,2,2,2,
2,2,2,2,2,2,2,2,2,2,2,2,2,2,2,2,2,2,2,2,2,2,2,2,2,2,2,2,2,2,2,2,2,2,2,2,
2,2,2,2,2,2,2,2,2,2,2,2,2,2,2,2,2,2,2,2,2,2,4),(-2.2563897994296,-2.25617264032142,
-2.20548091493677,-2.16239880479492,-2.13603967360701,-2.11649455008548,
-2.10673645545922,-2.09879612689942,-2.08951252865022,-2.0724450112368,
-2.05054452174938,-1.9913809212883,-1.94809717958013,-1.93959655682586,
-1.93463094162031,-1.93001107380822,-1.92316149683891,-1.90321368826529,
-1.86731364179743,-1.79262592726506,-1.77733406828992,-1.76832595052375,
-1.76035706376507,-1.75021007597095,-1.72847913483958,-1.69785584032169,
-1.6835832988613,-1.62109641911143,-1.60684770186615,-1.60120462159643,
-1.59665354252745,-1.59165708695002,-1.58301162189285,-1.52731288514099,
-1.45668679721837,-1.44104088890487,-1.43195720885795,-1.42407552750146,
-1.41408781097425,-1.39326820372732,-1.36446501805632,-1.32442006286722,
-1.27892357405158,-1.26809647150321,-1.26265268935592,-1.25820507785457,
-1.25230838856538,-1.23900562082609,-1.21954924184611,-1.14358421193059,
-1.11225368255816,-1.1004020157078,-1.09299578363841,-1.08478911903266,
-1.07305370419699,-1.04004773065855,-0.978484287935924,-0.938296895608987,
-0.929857768897369,-0.924905782371132,-0.920279569120465,-0.913393334851917,
-0.89312996778754,-0.856269068150209,-0.783264590511267,-0.767809334516993,
-0.758766858735784,-0.751600905690986,-0.741909614046922,-0.722719555433789,
-0.673279741278467,-0.609661140823291,-0.596298622174021,-0.590454380069076,
-0.585962399243232,-0.580535735965111,-0.569795483902219,-0.526646412262396,
-0.444631843080524,-0.43010976242088,-0.421344692650201,-0.413323926836748,
-0.402724014990961,-0.378213109111515,-0.34159938752182,-0.286177902529273,
-0.263172628756111,-0.255777931681658,-0.251517996100755,-0.246832340785092,
-0.239640249955974,-0.216564334649234,-0.170119922424535,-0.121724239606687),
 .UNSPECIFIED.);
#2046=B_SPLINE_CURVE_WITH_KNOTS('',3,(#26718,#26719,#26720,#26721,#26722,
#26723,#26724,#26725,#26726,#26727,#26728,#26729,#26730,#26731,#26732,#26733,
#26734,#26735,#26736,#26737,#26738,#26739,#26740,#26741,#26742,#26743,#26744,
#26745,#26746,#26747,#26748,#26749,#26750,#26751,#26752,#26753,#26754,#26755,
#26756,#26757,#26758,#26759,#26760,#26761,#26762,#26763,#26764,#26765,#26766,
#26767,#26768,#26769,#26770,#26771,#26772,#26773,#26774,#26775,#26776,#26777,
#26778,#26779,#26780,#26781,#26782,#26783,#26784,#26785,#26786,#26787,#26788,
#26789,#26790,#26791,#26792,#26793,#26794,#26795,#26796,#26797,#26798,#26799,
#26800,#26801,#26802,#26803,#26804,#26805,#26806,#26807,#26808,#26809,#26810,
#26811,#26812,#26813,#26814,#26815,#26816,#26817,#26818,#26819,#26820,#26821,
#26822,#26823,#26824,#26825,#26826,#26827,#26828,#26829,#26830,#26831,#26832,
#26833,#26834,#26835,#26836,#26837,#26838,#26839,#26840,#26841,#26842,#26843,
#26844,#26845,#26846,#26847,#26848,#26849,#26850,#26851,#26852,#26853,#26854,
#26855,#26856,#26857,#26858,#26859,#26860,#26861,#26862,#26863,#26864,#26865,
#26866,#26867,#26868,#26869,#26870,#26871,#26872,#26873,#26874,#26875,#26876,
#26877,#26878,#26879,#26880,#26881,#26882,#26883,#26884,#26885,#26886,#26887,
#26888,#26889,#26890,#26891,#26892,#26893,#26894,#26895,#26896,#26897,#26898,
#26899),.UNSPECIFIED.,.F.,.F.,(4,2,2,2,2,2,2,2,2,2,2,2,2,2,2,2,2,2,2,2,
2,2,2,2,2,2,2,2,2,2,2,2,2,2,2,2,2,2,2,2,2,2,2,2,2,2,2,2,2,2,2,2,2,2,2,2,
2,2,2,2,2,2,2,2,2,2,2,2,2,2,2,2,2,2,2,2,2,2,2,2,2,2,2,2,2,2,2,2,2,2,4),
(-4.150311630865,-4.10299606945067,-4.04866005705388,-4.02763646472151,
-4.01108239179314,-4.00190113589708,-3.9939533593162,-3.98406339802608,
-3.96379447430992,-3.87349631164672,-3.85297464905975,-3.83915834661892,
-3.83317449473006,-3.82867859751466,-3.82327817113619,-3.81267488599199,
-3.75791305318404,-3.70951103085173,-3.68040989731729,-3.66915040706937,
-3.66102658338615,-3.65250766041913,-3.63918796389323,-3.5898475880222,
-3.53168627666754,-3.51420208619552,-3.50188153059365,-3.49615681753122,
-3.49167467013618,-3.48606190448439,-3.47435184063762,-3.40907058508016,
-3.3487781532683,-3.33524332664059,-3.32668061176186,-3.31857983213367,
-3.3074572917442,-3.28117326184155,-3.19928156222836,-3.17933899259548,
-3.16579944878879,-3.15986203239535,-3.1553698585564,-3.14993561436056,
-3.13915984533944,-3.08863721037576,-3.03849098707347,-3.01760520099758,
-3.00113222885726,-2.99196706203714,-2.98401750621197,-2.97410481560841,
-2.95371062609174,-2.87829723089774,-2.83455551857323,-2.82611372437498,
-2.82116050704404,-2.81658746736636,-2.8097455165801,-2.7913770206207,-2.73228693213745,
-2.67531679882263,-2.66188268054417,-2.65334022653678,-2.64522853396833,
-2.63404222977097,-2.60725359781217,-2.52594021823729,-2.50604141679827,
-2.49252268731131,-2.48658854971494,-2.48209635260447,-2.47665900551617,
-2.46619983429442,-2.41081304996555,-2.36281507161715,-2.33385274932512,
-2.32261126610228,-2.31449022374852,-2.30596517243245,-2.29261662411509,
-2.24230405587675,-2.18496900304924,-2.15934795996631,-2.15191388056291,
-2.14717717336084,-2.14295913276517,-2.13579418290333,-2.11299865930798,
-2.06761808012842,-2.01518237751153),.UNSPECIFIED.);
#2047=B_SPLINE_CURVE_WITH_KNOTS('',3,(#26901,#26902,#26903,#26904,#26905,
#26906,#26907,#26908,#26909,#26910,#26911,#26912,#26913,#26914,#26915,#26916),
 .UNSPECIFIED.,.F.,.F.,(4,2,2,2,2,2,2,4),(-0.121724239606687,-0.109689116409445,
-0.0943349200454781,-0.085398485909038,-0.077419071321713,-0.0671558646773077,
-0.0559205022536955,-0.000968878777332341),.UNSPECIFIED.);
#2048=B_SPLINE_CURVE_WITH_KNOTS('',3,(#26917,#26918,#26919,#26920,#26921,
#26922,#26923,#26924,#26925,#26926,#26927,#26928,#26929,#26930,#26931,#26932,
#26933,#26934,#26935,#26936,#26937,#26938,#26939,#26940,#26941,#26942,#26943,
#26944,#26945,#26946,#26947,#26948,#26949,#26950,#26951,#26952,#26953,#26954,
#26955,#26956,#26957,#26958,#26959,#26960,#26961,#26962,#26963,#26964,#26965,
#26966,#26967,#26968,#26969,#26970,#26971,#26972,#26973,#26974,#26975,#26976,
#26977,#26978,#26979,#26980,#26981,#26982,#26983,#26984,#26985,#26986,#26987,
#26988,#26989,#26990,#26991,#26992,#26993,#26994,#26995,#26996,#26997,#26998,
#26999,#27000,#27001,#27002,#27003,#27004,#27005,#27006,#27007,#27008,#27009,
#27010,#27011,#27012,#27013,#27014,#27015,#27016,#27017,#27018,#27019,#27020,
#27021,#27022,#27023,#27024,#27025,#27026,#27027,#27028,#27029,#27030,#27031,
#27032,#27033,#27034,#27035,#27036,#27037,#27038,#27039,#27040,#27041,#27042,
#27043,#27044,#27045,#27046,#27047,#27048,#27049,#27050,#27051,#27052,#27053,
#27054,#27055,#27056,#27057,#27058,#27059,#27060,#27061,#27062,#27063,#27064,
#27065,#27066,#27067,#27068,#27069,#27070,#27071,#27072,#27073,#27074,#27075,
#27076,#27077,#27078,#27079,#27080,#27081,#27082,#27083,#27084,#27085,#27086,
#27087,#27088,#27089,#27090,#27091,#27092,#27093,#27094),.UNSPECIFIED.,
 .F.,.F.,(4,2,2,2,2,2,2,2,2,2,2,2,2,2,2,2,2,2,2,2,2,2,2,2,2,2,2,2,2,2,2,
2,2,2,2,2,2,2,2,2,2,2,2,2,2,2,2,2,2,2,2,2,2,2,2,2,2,2,2,2,2,2,2,2,2,2,2,
2,2,2,2,2,2,2,2,2,2,2,2,2,2,2,2,2,2,2,2,2,4),(-4.27045015464869,-4.20640916810718,
-4.19280331839385,-4.1868548159002,-4.18236190733064,-4.17693615137862,
-4.16620333481853,-4.12235615445556,-4.06637267137441,-4.0450377523509,
-4.02830086392083,-4.01908294880951,-4.01113813674298,-4.00129671497593,
-3.98129639143793,-3.89061914063169,-3.87007413576324,-3.85624671806726,
-3.85026097593406,-3.84576487366844,-3.84036568257061,-3.82976885373702,
-3.77510230313344,-3.7266266749074,-3.69750016649203,-3.68623725311328,
-3.67811277671187,-3.66959477443106,-3.65627992672295,-3.60709454706857,
-3.54879891223297,-3.5229826891724,-3.51553158633684,-3.51079137281393,
-3.50657624053097,-3.49942682828737,-3.47867763530581,-3.41462090646091,
-3.38149031616098,-3.35855667068276,-3.34820724436601,-3.34021640822844,
-3.3313238356518,-3.3161901806783,-3.23866728094364,-3.20435570605279,-3.18494596439479,
-3.17816136321212,-3.17355318203797,-3.16856406508616,-3.15995420526856,
-3.10969996494943,-3.06864322732716,-3.02723231353269,-3.01468240993723,
-3.0063186188984,-2.99818727124355,-2.98829591405804,-2.96334071683561,
-2.87995589929294,-2.85990049593513,-2.84630657219629,-2.84035983369153,
-2.83586679092081,-2.83043907458261,-2.8200257796388,-2.76371298148047,
-2.71629917337403,-2.68754071533038,-2.67632645442353,-2.66821011019436,
-2.65967668629844,-2.64628656644235,-2.59419721711936,-2.54575881315529,
-2.52428005794654,-2.51001496540451,-2.50395752044758,-2.49945507387976,
-2.49410576206915,-2.48406438087974,-2.40806717401893,-2.37295270227563,
-2.34910749997286,-2.3386109027513,-2.33060247116314,-2.32178599736271,
-2.30702015288851,-2.25620565721006),.UNSPECIFIED.);
#2049=B_SPLINE_CURVE_WITH_KNOTS('',3,(#27100,#27101,#27102,#27103,#27104,
#27105,#27106,#27107,#27108,#27109,#27110,#27111,#27112,#27113,#27114,#27115,
#27116,#27117,#27118,#27119,#27120,#27121,#27122,#27123,#27124,#27125,#27126,
#27127,#27128,#27129,#27130,#27131,#27132,#27133,#27134,#27135,#27136,#27137,
#27138,#27139,#27140,#27141,#27142,#27143,#27144,#27145,#27146,#27147,#27148,
#27149,#27150,#27151,#27152,#27153,#27154,#27155,#27156,#27157,#27158,#27159,
#27160,#27161,#27162,#27163,#27164,#27165,#27166,#27167,#27168,#27169,#27170,
#27171,#27172,#27173,#27174,#27175,#27176,#27177,#27178,#27179,#27180,#27181,
#27182,#27183,#27184,#27185,#27186,#27187,#27188,#27189,#27190,#27191,#27192,
#27193,#27194,#27195,#27196,#27197,#27198,#27199,#27200,#27201,#27202,#27203,
#27204,#27205,#27206,#27207,#27208,#27209,#27210,#27211,#27212,#27213,#27214,
#27215,#27216,#27217,#27218,#27219,#27220,#27221,#27222,#27223,#27224,#27225,
#27226,#27227,#27228,#27229,#27230,#27231,#27232,#27233,#27234,#27235,#27236,
#27237,#27238,#27239,#27240,#27241,#27242,#27243,#27244,#27245,#27246,#27247,
#27248,#27249,#27250,#27251,#27252,#27253,#27254,#27255,#27256,#27257,#27258,
#27259,#27260,#27261,#27262,#27263,#27264,#27265,#27266,#27267,#27268,#27269,
#27270,#27271,#27272,#27273,#27274,#27275,#27276,#27277,#27278,#27279),
 .UNSPECIFIED.,.F.,.F.,(4,2,2,2,2,2,2,2,2,2,2,2,2,2,2,2,2,2,2,2,2,2,2,2,
2,2,2,2,2,2,2,2,2,2,2,2,2,2,2,2,2,2,2,2,2,2,2,2,2,2,2,2,2,2,2,2,2,2,2,2,
2,2,2,2,2,2,2,2,2,2,2,2,2,2,2,2,2,2,2,2,2,2,2,2,2,2,2,2,2,4),(-2.01551633957596,
-1.97100294214132,-1.93094368306841,-1.92250712211063,-1.9175550915435,
-1.91292751069057,-1.90603734297219,-1.88574768779601,-1.8488109357755,
-1.77590885108523,-1.76044003913263,-1.75139356733603,-1.74422654750104,
-1.73453655721479,-1.7153596835281,-1.66592165405107,-1.60236003205732,
-1.5889210109553,-1.58306324824702,-1.57856943506887,-1.57315126665527,
-1.562457496166,-1.51975618965176,-1.43698418138697,-1.42256787867547,-1.41382358314604,
-1.40579449200453,-1.39514277907982,-1.37030500794304,-1.33294258801471,
-1.27558170491081,-1.25510795881394,-1.2479925161802,-1.24378379757422,
-1.2390360088733,-1.23154760573345,-1.20529809726063,-1.14480583622687,
-1.09807169318314,-1.08485524782977,-1.07635792298543,-1.06822333168301,
-1.0568969728353,-1.02727497182618,-0.977325459186844,-0.925052903035115,
-0.914344412661386,-0.908923649618214,-0.904430599112063,-0.898476233371473,
-0.884834196318552,-0.864675376124207,-0.779929506593619,-0.75593463786887,
-0.746231063123578,-0.73814638105055,-0.729720122856109,-0.716852606929916,
-0.671103401529981,-0.657071987480944,-0.595146126709241,-0.580266777580344,
-0.574533852783794,-0.569961289634649,-0.565009983052622,-0.556573928640137,
-0.513005122451566,-0.438075136822825,-0.417225725296742,-0.407233269581727,
-0.399279360523891,-0.390173951717792,-0.373990834946602,-0.319159360216256,
-0.254820611503855,-0.242215616854905,-0.23644079240197,-0.231958330174234,
-0.226393722524574,-0.214936164036624,-0.19910293447049,-0.164283060489829,
-0.0964739508057076,-0.0805613449356902,-0.0706123990424877,-0.0626618732903943,
-0.05517979311657,-0.0461811186475704,-0.029023611973482,-0.000968453055024552),
 .UNSPECIFIED.);
#2050=B_SPLINE_CURVE_WITH_KNOTS('',3,(#27280,#27281,#27282,#27283,#27284,
#27285,#27286,#27287,#27288,#27289,#27290,#27291,#27292,#27293,#27294,#27295),
 .UNSPECIFIED.,.F.,.F.,(4,2,2,2,2,2,2,4),(-4.27056840112397,-4.19726488735619,
-4.17775155830065,-4.17095443887722,-4.16634410714741,-4.16135979777357,
-4.15277192253053,-4.150311630865),.UNSPECIFIED.);
#2051=B_SPLINE_CURVE_WITH_KNOTS('',3,(#27296,#27297,#27298,#27299,#27300,
#27301,#27302,#27303,#27304,#27305,#27306,#27307,#27308,#27309,#27310,#27311,
#27312,#27313,#27314,#27315,#27316,#27317,#27318,#27319,#27320,#27321,#27322,
#27323,#27324,#27325,#27326,#27327,#27328,#27329,#27330,#27331,#27332,#27333,
#27334,#27335,#27336,#27337,#27338,#27339,#27340,#27341,#27342,#27343,#27344,
#27345,#27346,#27347,#27348,#27349,#27350,#27351,#27352,#27353,#27354,#27355,
#27356,#27357,#27358,#27359,#27360,#27361,#27362,#27363,#27364,#27365,#27366,
#27367,#27368,#27369,#27370,#27371,#27372,#27373,#27374,#27375,#27376,#27377,
#27378,#27379,#27380,#27381,#27382,#27383,#27384,#27385,#27386,#27387,#27388,
#27389,#27390,#27391,#27392,#27393,#27394,#27395,#27396,#27397,#27398,#27399,
#27400,#27401,#27402,#27403,#27404,#27405,#27406,#27407,#27408,#27409,#27410,
#27411,#27412,#27413,#27414,#27415,#27416,#27417,#27418,#27419,#27420,#27421,
#27422,#27423,#27424,#27425,#27426,#27427,#27428,#27429,#27430,#27431,#27432,
#27433,#27434,#27435,#27436,#27437,#27438,#27439,#27440,#27441,#27442,#27443,
#27444,#27445,#27446,#27447,#27448,#27449,#27450,#27451,#27452,#27453,#27454,
#27455,#27456,#27457,#27458,#27459,#27460,#27461,#27462,#27463,#27464,#27465,
#27466,#27467,#27468,#27469,#27470,#27471,#27472,#27473,#27474,#27475,#27476,
#27477,#27478,#27479,#27480,#27481,#27482,#27483,#27484,#27485,#27486,#27487),
 .UNSPECIFIED.,.F.,.F.,(4,2,2,2,2,2,2,2,2,2,2,2,2,2,2,2,2,2,2,2,2,2,2,2,
2,2,2,2,2,2,2,2,2,2,2,2,2,2,2,2,2,2,2,2,2,2,2,2,2,2,2,2,2,2,2,2,2,2,2,2,
2,2,2,2,2,2,2,2,2,2,2,2,2,2,2,2,2,2,2,2,2,2,2,2,2,2,2,2,2,2,2,2,2,2,2,4),
(-2.25620565721006,-2.22674092288587,-2.17861356694801,-2.17006384376556,
-2.1650876096842,-2.16052647962773,-2.15375021966668,-2.13584867970713,
-2.10485121727545,-2.02455130533443,-2.00841585248802,-1.99922720731249,
-1.99127998732835,-1.98139975680707,-1.96118516900079,-1.886341567801,-1.84187966313487,
-1.83337239223273,-1.82840520954572,-1.82378584202544,-1.81693979999276,
-1.79702333186233,-1.76121833635185,-1.68635600701543,-1.6709014944024,
-1.66194303702644,-1.65396529365384,-1.64373395712913,-1.62150869152567,
-1.5898710638916,-1.55255422062084,-1.50907080851806,-1.49835548384483,
-1.49293315610587,-1.4884399269554,-1.48248678176424,-1.468853485301,-1.44871347772828,
-1.36424333154351,-1.34002873882752,-1.33029090831023,-1.32219763087632,
-1.31378292792677,-1.30097492012888,-1.25610984146421,-1.21740752431863,
-1.17258687220201,-1.16180380234664,-1.15636845560637,-1.15187691404446,
-1.14594225158098,-1.13241706141475,-1.11250160188752,-1.03102495646972,
-1.00434833218206,-0.993179787569088,-0.985072168699662,-0.976526147784555,
-0.963069388925572,-0.905323299020189,-0.844829562827071,-0.828205390863629,
-0.82162099049646,-0.817048046047516,-0.811981325450983,-0.80300411144634,
-0.791565098502637,-0.764730777377551,-0.675964674855657,-0.660849409084116,
-0.651962019042687,-0.643972513331658,-0.633620067058567,-0.610657365934555,
-0.577463843072448,-0.512945867461247,-0.492732449152739,-0.485649855044167,
-0.481447554902438,-0.476692727640427,-0.469168693905066,-0.442487052039814,
-0.379663346979327,-0.335488782814744,-0.322421084625329,-0.313955024257332,
-0.305804270204379,-0.294378107978197,-0.263960037262439,-0.187834051313414,
-0.157993534932162,-0.150022430082447,-0.145171331567268,-0.140480200037555,
-0.133261617963766,-0.121363534210794),.UNSPECIFIED.);
#2052=B_SPLINE_CURVE_WITH_KNOTS('',3,(#27492,#27493,#27494,#27495,#27496,
#27497,#27498,#27499,#27500,#27501,#27502,#27503,#27504,#27505,#27506,#27507,
#27508,#27509,#27510,#27511,#27512,#27513,#27514,#27515,#27516,#27517,#27518,
#27519,#27520,#27521,#27522,#27523,#27524,#27525,#27526,#27527,#27528,#27529,
#27530,#27531,#27532,#27533,#27534,#27535,#27536,#27537,#27538,#27539,#27540,
#27541,#27542,#27543,#27544,#27545,#27546,#27547,#27548,#27549,#27550,#27551,
#27552,#27553,#27554,#27555,#27556,#27557,#27558,#27559,#27560,#27561,#27562,
#27563,#27564,#27565,#27566,#27567,#27568,#27569,#27570,#27571,#27572,#27573,
#27574,#27575,#27576,#27577,#27578,#27579,#27580,#27581,#27582,#27583,#27584,
#27585,#27586,#27587,#27588,#27589,#27590,#27591,#27592,#27593,#27594,#27595,
#27596,#27597,#27598,#27599,#27600,#27601,#27602,#27603,#27604,#27605,#27606,
#27607,#27608,#27609,#27610,#27611,#27612,#27613,#27614,#27615,#27616,#27617,
#27618,#27619,#27620,#27621,#27622,#27623,#27624,#27625,#27626,#27627,#27628,
#27629,#27630,#27631,#27632,#27633,#27634,#27635,#27636,#27637,#27638,#27639,
#27640,#27641,#27642,#27643,#27644,#27645,#27646,#27647,#27648,#27649,#27650,
#27651,#27652,#27653,#27654,#27655,#27656,#27657,#27658,#27659,#27660,#27661,
#27662,#27663,#27664,#27665,#27666,#27667,#27668,#27669,#27670,#27671,#27672,
#27673,#27674,#27675,#27676,#27677,#27678,#27679,#27680,#27681,#27682,#27683,
#27684,#27685),.UNSPECIFIED.,.F.,.F.,(4,2,2,2,2,2,2,2,2,2,2,2,2,2,2,2,2,
2,2,2,2,2,2,2,2,2,2,2,2,2,2,2,2,2,2,2,2,2,2,2,2,2,2,2,2,2,2,2,2,2,2,2,2,
2,2,2,2,2,2,2,2,2,2,2,2,2,2,2,2,2,2,2,2,2,2,2,2,2,2,2,2,2,2,2,2,2,2,2,2,
2,2,2,2,2,2,2,4),(-4.15043685499169,-4.1419927963705,-4.12026298144975,
-4.11011617157691,-4.10214740112473,-4.09313939879801,-4.07784758435589,
-4.00322628867515,-3.967329236326,-3.94738238206905,-3.94053314281837,-3.93591337263554,
-3.93094781458924,-3.92244702024144,-3.87896328723779,-3.80354361600812,
-3.78302437652005,-3.77308986646971,-3.76513953175498,-3.75599179194078,
-3.74004631031488,-3.68203228549128,-3.63484953189147,-3.61158047460792,
-3.60436854905171,-3.59967841803399,-3.5954216481394,-3.58804559255959,
-3.56523623776591,-3.5031541827577,-3.47036983655162,-3.4476000414642,-3.43727858967008,
-3.4292919530732,-3.4203863402354,-3.4051851838402,-3.31684715138366,-3.28986934246889,
-3.27839204643009,-3.26939110276455,-3.26431904240687,-3.25974754922955,
-3.25421199364198,-3.2406204803456,-3.17748921793959,-3.11828981083343,
-3.10478579052343,-3.09622964950842,-3.0881261934985,-3.07698561908038,
-3.05053063620219,-2.96883599039273,-2.94890917238161,-2.93537738443129,
-2.92944143940272,-2.92494955409566,-2.91951464673511,-2.90873472537767,
-2.86397913383808,-2.82548925544464,-2.78030972617508,-2.76747877868622,
-2.75905919739266,-2.7509685826569,-2.74124295120193,-2.71710846127403,
-2.63257753541481,-2.61243936553908,-2.59880592406649,-2.59285268922707,
-2.58835931440768,-2.58293680561772,-2.5722209886904,-2.52875550863412,
-2.49150493957345,-2.45977309719104,-2.43750376856466,-2.42726478468193,
-2.41928611753453,-2.4103318480017,-2.39489808849618,-2.319904261361,-2.28421062147483,
-2.26433104739607,-2.25748949931945,-2.25287089246033,-2.24790207488413,
-2.23938723230488,-2.19354971461565,-2.13624343551609,-2.10493442165203,
-2.09308368434727,-2.08567658415935,-2.07746779196152,-2.06572701939312,
-2.03268716434458,-2.01551633957596),.UNSPECIFIED.);
#2053=B_SPLINE_CURVE_WITH_KNOTS('',3,(#27687,#27688,#27689,#27690,#27691,
#27692,#27693,#27694),.UNSPECIFIED.,.F.,.F.,(4,2,2,4),(-0.121363534210794,
-0.109923186150701,-0.0624718254002537,-0.000969694913198329),
 .UNSPECIFIED.);
#2054=B_SPLINE_CURVE_WITH_KNOTS('',3,(#27695,#27696,#27697,#27698,#27699,
#27700,#27701,#27702,#27703,#27704,#27705,#27706,#27707,#27708,#27709,#27710,
#27711,#27712,#27713,#27714,#27715,#27716,#27717,#27718,#27719,#27720,#27721,
#27722,#27723,#27724,#27725,#27726,#27727,#27728,#27729,#27730,#27731,#27732,
#27733,#27734,#27735,#27736,#27737,#27738,#27739,#27740,#27741,#27742,#27743,
#27744,#27745,#27746,#27747,#27748,#27749,#27750,#27751,#27752,#27753,#27754,
#27755,#27756,#27757,#27758,#27759,#27760,#27761,#27762,#27763,#27764,#27765,
#27766,#27767,#27768,#27769,#27770,#27771,#27772,#27773,#27774,#27775,#27776,
#27777,#27778,#27779,#27780,#27781,#27782,#27783,#27784,#27785,#27786,#27787,
#27788,#27789,#27790,#27791,#27792,#27793,#27794,#27795,#27796,#27797,#27798,
#27799,#27800,#27801,#27802,#27803,#27804,#27805,#27806,#27807,#27808,#27809,
#27810,#27811,#27812,#27813,#27814,#27815,#27816,#27817,#27818,#27819,#27820,
#27821,#27822,#27823,#27824,#27825,#27826,#27827,#27828,#27829,#27830,#27831,
#27832,#27833,#27834,#27835,#27836,#27837,#27838,#27839,#27840,#27841,#27842,
#27843,#27844,#27845,#27846,#27847,#27848,#27849,#27850,#27851,#27852,#27853,
#27854,#27855,#27856,#27857,#27858,#27859,#27860,#27861,#27862,#27863,#27864,
#27865,#27866,#27867,#27868,#27869,#27870,#27871,#27872,#27873,#27874,#27875,
#27876,#27877,#27878,#27879,#27880,#27881,#27882,#27883,#27884,#27885,#27886,
#27887,#27888,#27889,#27890,#27891,#27892,#27893),.UNSPECIFIED.,.F.,.F.,
(4,3,3,3,3,3,3,3,3,3,3,3,3,3,3,3,3,3,3,3,3,3,3,3,3,3,3,3,3,3,3,3,3,3,3,
3,3,3,3,3,3,3,3,3,3,3,3,3,3,3,3,3,3,3,3,3,3,3,3,3,3,3,3,3,3,3,4),(-16.4167960594917,
-16.3231866235492,-16.2295268848231,-16.1346626699374,-16.040780714902,
-15.9454253700912,-15.8500700252804,-15.7580593298271,-15.6661696621755,
-15.574374570756,-15.4826447796787,-15.3909489505858,-15.2992633144944,
-15.207564116827,-15.1157697393145,-15.023926043559,-14.9319324069698,-14.8594406487004,
-14.7674299217847,-14.6755402223328,-14.5837450988209,-14.492015275348,
-14.4003194136853,-14.3086337448901,-14.2169345144247,-14.1251401041729,
-14.0332963756617,-13.9413027066307,-13.8688112721204,-13.7768007118962,
-13.6849111794219,-13.5931162229543,-13.5013865659418,-13.4096908703253,
-13.318005366967,-13.2263063011332,-13.1345120532514,-13.0426684861021,
-12.9506749751077,-12.8781818955404,-12.786171091896,-12.6942813167991,
-12.6024861188083,-12.5107562228943,-12.4190602900613,-12.3273745514424,
-12.2356752525775,-12.1438807765432,-12.0520369835985,-11.9600432530071,
-11.8875525189603,-11.7955415539488,-11.7036516144507,-11.6118562492808,
-11.5201261827394,-11.4284300772306,-11.3367441641075,-11.2450446891281,
-11.1532500355945,-11.0614060641193,-10.969412155172,-10.8969231423803,
-10.8060912020345,-10.7154002356709,-10.6247905981352,-10.5342411095498,
-10.4882942057671),.UNSPECIFIED.);
#2055=B_SPLINE_CURVE_WITH_KNOTS('',3,(#27899,#27900,#27901,#27902,#27903,
#27904,#27905,#27906,#27907,#27908,#27909,#27910,#27911,#27912,#27913,#27914,
#27915,#27916,#27917,#27918,#27919,#27920,#27921,#27922,#27923,#27924,#27925,
#27926,#27927,#27928,#27929,#27930,#27931,#27932,#27933,#27934,#27935,#27936,
#27937,#27938,#27939,#27940,#27941,#27942,#27943,#27944,#27945,#27946,#27947,
#27948,#27949,#27950,#27951,#27952,#27953,#27954,#27955,#27956,#27957,#27958,
#27959,#27960,#27961,#27962,#27963,#27964,#27965,#27966,#27967,#27968,#27969,
#27970,#27971,#27972,#27973,#27974,#27975,#27976,#27977,#27978,#27979,#27980,
#27981,#27982,#27983,#27984,#27985,#27986,#27987,#27988,#27989,#27990,#27991,
#27992,#27993,#27994,#27995,#27996,#27997,#27998,#27999,#28000,#28001,#28002,
#28003,#28004,#28005,#28006,#28007,#28008,#28009,#28010,#28011,#28012,#28013,
#28014,#28015,#28016,#28017,#28018,#28019,#28020,#28021,#28022,#28023,#28024),
 .UNSPECIFIED.,.F.,.F.,(4,2,2,2,2,2,2,2,2,2,2,2,2,2,2,2,2,2,2,2,2,2,2,2,
2,2,2,2,2,2,2,2,2,2,2,2,2,2,2,2,2,2,2,2,2,2,2,2,2,2,2,2,2,2,2,2,2,2,2,2,
2,2,4),(0.000239007866642453,0.00318305016454312,0.00679207464510367,0.0172466284369836,
0.0769673619474505,0.122954072103129,0.140861551821579,0.150881365847671,
0.1596828971895,0.170863291190468,0.194007000851062,0.273005688525858,0.305932246158347,
0.325093786965003,0.331890676084245,0.336513067537287,0.341376727708402,
0.34972879403149,0.393628126390447,0.468758665022071,0.487766655437066,
0.497199828562151,0.5048357524462,0.513704255035803,0.529324403857262,0.619191266485426,
0.658198851426284,0.668293771046563,0.673423197069837,0.677846792969457,
0.683626747950734,0.696674199810325,0.760803263280959,0.8107866841944,0.830135837775079,
0.839912206488528,0.847146427656818,0.856286215974925,0.871959717286507,
0.937838545693914,0.977402766009273,0.998499383907113,1.005550638497,1.0102651641193,
1.01526232509509,1.02379215622777,1.06623872462077,1.12578115720227,1.14775073965833,
1.16486976607114,1.17419354231179,1.1821771218247,1.19200168904993,1.21173750065209,
1.30303662410998,1.32365591982206,1.33752876585011,1.34353448614347,1.34803425906185,
1.35341223548036,1.36396453008937,1.41961717955807,1.42898336541552),
 .UNSPECIFIED.);
#2056=B_SPLINE_CURVE_WITH_KNOTS('',3,(#28027,#28028,#28029,#28030,#28031,
#28032,#28033,#28034,#28035,#28036,#28037,#28038,#28039,#28040,#28041,#28042,
#28043,#28044,#28045,#28046,#28047,#28048,#28049,#28050,#28051,#28052,#28053,
#28054,#28055,#28056,#28057,#28058,#28059,#28060,#28061,#28062,#28063,#28064,
#28065,#28066,#28067,#28068,#28069,#28070,#28071,#28072,#28073,#28074,#28075,
#28076,#28077,#28078,#28079,#28080,#28081,#28082,#28083,#28084,#28085,#28086,
#28087,#28088,#28089,#28090,#28091,#28092,#28093,#28094,#28095,#28096,#28097,
#28098,#28099,#28100,#28101,#28102,#28103,#28104,#28105,#28106,#28107,#28108,
#28109,#28110,#28111,#28112,#28113,#28114,#28115,#28116,#28117,#28118,#28119,
#28120,#28121,#28122,#28123,#28124,#28125,#28126,#28127,#28128,#28129,#28130,
#28131,#28132,#28133,#28134,#28135,#28136,#28137,#28138,#28139,#28140,#28141,
#28142,#28143,#28144,#28145,#28146,#28147,#28148,#28149,#28150,#28151,#28152,
#28153,#28154,#28155,#28156,#28157,#28158,#28159,#28160,#28161,#28162,#28163,
#28164,#28165,#28166,#28167,#28168,#28169,#28170,#28171,#28172,#28173,#28174,
#28175,#28176,#28177,#28178,#28179,#28180,#28181,#28182,#28183,#28184,#28185,
#28186,#28187,#28188,#28189,#28190,#28191,#28192,#28193,#28194,#28195,#28196,
#28197,#28198,#28199,#28200,#28201,#28202,#28203,#28204),.UNSPECIFIED.,
 .F.,.F.,(4,2,2,2,2,2,2,2,2,2,2,2,2,2,2,2,2,2,2,2,2,2,2,2,2,2,2,2,2,2,2,
2,2,2,2,2,2,2,2,2,2,2,2,2,2,2,2,2,2,2,2,2,2,2,2,2,2,2,2,2,2,2,2,2,2,2,2,
2,2,2,2,2,2,2,2,2,2,2,2,2,2,2,2,2,2,2,2,2,4),(-4.02407322506492,-4.01684615812316,
-3.95297570902188,-3.90421498575493,-3.88504620935784,-3.87530282427345,
-3.86807088789497,-3.8589047995826,-3.8431108092334,-3.78310802528751,-3.73942647125242,
-3.71713566051703,-3.70995356631042,-3.70521239123192,-3.70087298610828,
-3.69319560061104,-3.6674783872908,-3.60819888538897,-3.57598547663887,
-3.55347551207692,-3.54316464254709,-3.53514145305865,-3.52614721469809,
-3.51066566198414,-3.43551533470643,-3.39979648673552,-3.37988975750343,
-3.3730303874555,-3.36840094064498,-3.3634498747333,-3.35496208612577,-3.31077821760017,
-3.25221004912553,-3.22001510984916,-3.20840641653873,-3.2002529590541,
-3.19189373426824,-3.1792165221942,-3.14073896558892,-3.07209761455203,
-3.04442119374092,-3.03684141370282,-3.03209247807399,-3.02790838978219,
-3.02091953792342,-3.00145052028715,-2.94323825833587,-2.89127770623233,
-2.87544548946516,-2.86640260894449,-2.85842629218569,-2.84830073736399,
-2.82673707096946,-2.7385292621348,-2.7181541427148,-2.70440489058742,-2.6984244324262,
-2.69392191030839,-2.68850207349082,-2.67813783289135,-2.62020502255187,
-2.57387140102453,-2.5454981561429,-2.53433364362457,-2.52622347853048,
-2.51766973302586,-2.50418970510008,-2.44896022657446,-2.39571829556286,
-2.37097857255921,-2.36362402375918,-2.35890401615598,-2.35467501666104,
-2.34744182311128,-2.32595316564627,-2.26934029012784,-2.21377276203436,
-2.20039586146863,-2.19186910195483,-2.18375812457399,-2.17255001510732,
-2.14562312531643,-2.06445987829934,-2.04457410756517,-2.03106334885449,
-2.02513323148761,-2.02064327949749,-2.01520731591665,-2.01509656764977),
 .UNSPECIFIED.);
#2057=B_SPLINE_CURVE_WITH_KNOTS('',3,(#28210,#28211,#28212,#28213,#28214,
#28215,#28216,#28217,#28218,#28219,#28220,#28221,#28222,#28223,#28224,#28225,
#28226,#28227,#28228,#28229,#28230,#28231,#28232,#28233,#28234,#28235,#28236,
#28237,#28238,#28239,#28240,#28241,#28242,#28243,#28244,#28245,#28246,#28247,
#28248,#28249,#28250,#28251,#28252,#28253,#28254,#28255,#28256,#28257,#28258,
#28259,#28260,#28261,#28262,#28263,#28264,#28265,#28266,#28267,#28268,#28269,
#28270,#28271,#28272,#28273,#28274,#28275,#28276,#28277,#28278,#28279,#28280,
#28281,#28282,#28283,#28284,#28285,#28286,#28287,#28288,#28289,#28290,#28291,
#28292,#28293,#28294,#28295,#28296,#28297,#28298,#28299,#28300,#28301,#28302,
#28303,#28304,#28305,#28306,#28307,#28308,#28309,#28310,#28311,#28312,#28313,
#28314,#28315,#28316,#28317,#28318,#28319,#28320,#28321,#28322,#28323,#28324,
#28325,#28326,#28327,#28328,#28329,#28330,#28331,#28332,#28333,#28334,#28335,
#28336,#28337,#28338,#28339,#28340,#28341,#28342,#28343,#28344,#28345,#28346,
#28347,#28348,#28349,#28350,#28351,#28352,#28353,#28354),.UNSPECIFIED.,
 .F.,.F.,(4,3,3,3,3,3,3,3,3,3,3,3,3,3,3,3,3,3,3,3,3,3,3,3,3,3,3,3,3,3,3,
3,3,3,3,3,3,3,3,3,3,3,3,3,3,3,3,3,4),(74.4826134213612,74.5701017723267,
74.6575413414613,74.7449561905202,74.8323670824359,74.9197947723584,75.0073147299331,
75.0948819850037,75.182590823232,75.2578179239381,75.345788390083,75.4336477306673,
75.5214187672958,75.6122973339486,75.6999675202677,75.787623694431,75.8752863492957,
75.9629759772044,76.0507597426102,76.138599596557,76.2265618479682,76.2484473005182,
76.3363312061505,76.4241058872677,76.5117942396746,76.6027045443526,76.690297437038,
76.7778784327587,76.865468097327,76.9530869976608,77.0408037132434,77.1285785844341,
77.2164793426409,77.2390766770982,77.3260776811172,77.4129675814226,77.4997702486672,
77.5910122242935,77.677722446241,77.7644232260262,77.8511359862967,77.9378821551616,
78.0247366814142,78.1116543275945,78.1987119327436,78.2297060536782,78.3416490186313,
78.4517318766385,78.5398162005936),.UNSPECIFIED.);
#2058=B_SPLINE_CURVE_WITH_KNOTS('',3,(#28356,#28357,#28358,#28359),
 .UNSPECIFIED.,.F.,.F.,(4,4),(78.5398163397448,79.2203354302583),
 .UNSPECIFIED.);
#2059=B_SPLINE_CURVE_WITH_KNOTS('',3,(#28363,#28364,#28365,#28366,#28367,
#28368,#28369,#28370,#28371,#28372,#28373,#28374,#28375,#28376,#28377,#28378,
#28379,#28380,#28381,#28382,#28383,#28384,#28385,#28386,#28387,#28388,#28389,
#28390,#28391,#28392,#28393,#28394,#28395,#28396,#28397,#28398,#28399,#28400,
#28401,#28402,#28403,#28404,#28405),.UNSPECIFIED.,.F.,.F.,(4,3,3,3,3,3,
3,3,3,3,3,3,3,3,4),(78.5398163398758,78.6511929986185,78.7647319104916,
78.7900351244193,78.8773823755869,78.9646206369788,79.0517734317144,79.1388666078676,
79.2259284415399,79.3129800697699,79.4000426173296,79.4871912470598,79.5743826688074,
79.6617143219692,79.7442523237011),.UNSPECIFIED.);
#2060=B_SPLINE_CURVE_WITH_KNOTS('',3,(#28406,#28407,#28408,#28409,#28410,
#28411,#28412,#28413,#28414,#28415,#28416,#28417,#28418,#28419,#28420,#28421,
#28422,#28423,#28424,#28425,#28426,#28427,#28428,#28429,#28430,#28431,#28432,
#28433,#28434,#28435,#28436,#28437,#28438,#28439,#28440,#28441,#28442,#28443,
#28444,#28445,#28446,#28447,#28448,#28449,#28450,#28451,#28452,#28453,#28454,
#28455,#28456,#28457,#28458,#28459,#28460,#28461,#28462,#28463,#28464,#28465,
#28466,#28467,#28468,#28469,#28470,#28471,#28472,#28473,#28474,#28475,#28476,
#28477,#28478,#28479,#28480,#28481,#28482,#28483,#28484,#28485,#28486,#28487,
#28488,#28489,#28490,#28491,#28492,#28493,#28494,#28495,#28496,#28497,#28498,
#28499,#28500,#28501,#28502,#28503,#28504,#28505,#28506,#28507,#28508,#28509,
#28510,#28511,#28512,#28513,#28514,#28515,#28516,#28517,#28518,#28519,#28520,
#28521,#28522,#28523,#28524,#28525,#28526,#28527,#28528,#28529,#28530,#28531,
#28532,#28533,#28534,#28535,#28536,#28537,#28538,#28539,#28540,#28541,#28542,
#28543,#28544,#28545,#28546,#28547,#28548,#28549,#28550,#28551,#28552,#28553),
 .UNSPECIFIED.,.F.,.F.,(4,3,3,3,3,3,3,3,3,3,3,3,3,3,3,3,3,3,3,3,3,3,3,3,
3,3,3,3,3,3,3,3,3,3,3,3,3,3,3,3,3,3,3,3,3,3,3,3,3,4),(74.4816293874842,
74.5692291182483,74.6568738997928,74.7446611966697,74.8275176180992,74.9153514936717,
75.0030745173814,75.0907096711157,75.1816393365611,75.2691755835765,75.356698770865,
75.4442295357681,75.531788515978,75.6194441230468,75.7071571243338,75.7949953852759,
75.8181469946792,75.9059803180108,75.9937030526064,76.0813381770006,76.172267951283,
76.259804809245,76.3473288411951,76.4348606823757,76.522420968548,76.6100782122204,
76.6977930443859,76.7856334044264,76.8087763712593,76.8964962279262,76.9841050707776,
77.0716260157815,77.1625984822888,77.2500211632198,77.3374312133021,77.4248493891094,
77.5122964480626,77.5998416802232,77.6874450752849,77.7751756908071,77.7994057478393,
77.8864521187219,77.9733602235073,78.0601890785893,78.1469602031835,78.2336950644677,
78.3204372261484,78.4071825266451,78.493986476461,78.5398163397448),
 .UNSPECIFIED.);
#2061=B_SPLINE_CURVE_WITH_KNOTS('',3,(#28559,#28560,#28561,#28562,#28563,
#28564,#28565,#28566,#28567,#28568,#28569,#28570,#28571,#28572,#28573,#28574,
#28575,#28576,#28577,#28578,#28579,#28580,#28581,#28582,#28583,#28584,#28585,
#28586,#28587,#28588,#28589,#28590,#28591,#28592,#28593,#28594,#28595,#28596,
#28597,#28598,#28599,#28600,#28601,#28602,#28603,#28604,#28605,#28606,#28607,
#28608,#28609,#28610,#28611,#28612,#28613,#28614,#28615,#28616,#28617,#28618,
#28619,#28620,#28621,#28622,#28623,#28624,#28625,#28626,#28627,#28628,#28629,
#28630,#28631,#28632,#28633,#28634,#28635,#28636,#28637,#28638,#28639,#28640,
#28641,#28642,#28643,#28644,#28645,#28646,#28647,#28648,#28649,#28650,#28651,
#28652,#28653,#28654,#28655,#28656,#28657,#28658,#28659,#28660,#28661,#28662,
#28663,#28664,#28665,#28666,#28667,#28668,#28669,#28670,#28671,#28672,#28673,
#28674,#28675,#28676,#28677,#28678,#28679,#28680,#28681,#28682,#28683,#28684,
#28685,#28686,#28687,#28688,#28689,#28690,#28691,#28692,#28693,#28694,#28695,
#28696,#28697,#28698,#28699,#28700,#28701,#28702,#28703,#28704,#28705,#28706),
 .UNSPECIFIED.,.F.,.F.,(4,3,3,3,3,3,3,3,3,3,3,3,3,3,3,3,3,3,3,3,3,3,3,3,
3,3,3,3,3,3,3,3,3,3,3,3,3,3,3,3,3,3,3,3,3,3,3,3,3,4),(68.1983677761468,
68.2861854312294,68.3234122878779,68.4112283839335,68.4989336833237,68.5865511879601,
68.6774874975223,68.7650063922156,68.8525123660811,68.9400260745581,69.0275681735632,
69.115207242346,69.2029038856652,69.2907261761316,69.314041664458,69.4018609765982,
69.4895694847055,69.5771901870388,69.6681252937887,69.7556473388717,69.8431564403359,
69.9306732503291,70.0182184214548,70.1058605036167,70.1935601296495,70.2813853353724,
70.304671041038,70.392491752492,70.4802016945542,70.5678238633181,70.6587584326056,
70.7462820149109,70.8337926768927,70.9213110688809,71.0088578416761,71.0965015462834,
71.1842028087346,71.2720296586304,71.295300417618,71.3826851492496,71.4699593048868,
71.557146385153,71.6445819660545,71.7316742688595,71.8187549134235,71.9058449991257,
71.9935415074355,72.0807585750809,72.1686948037228,72.2566310323648),
 .UNSPECIFIED.);
#2062=B_SPLINE_CURVE_WITH_KNOTS('',3,(#28707,#28708,#28709,#28710,#28711,
#28712,#28713,#28714,#28715,#28716,#28717,#28718,#28719,#28720,#28721,#28722,
#28723,#28724,#28725,#28726,#28727,#28728,#28729,#28730,#28731,#28732,#28733,
#28734,#28735,#28736,#28737,#28738,#28739,#28740,#28741,#28742,#28743,#28744,
#28745,#28746,#28747,#28748,#28749,#28750,#28751,#28752,#28753,#28754,#28755,
#28756,#28757,#28758,#28759,#28760,#28761,#28762,#28763,#28764,#28765,#28766,
#28767,#28768,#28769,#28770,#28771,#28772,#28773,#28774,#28775,#28776,#28777,
#28778,#28779,#28780,#28781,#28782,#28783,#28784,#28785,#28786,#28787,#28788,
#28789,#28790,#28791),.UNSPECIFIED.,.F.,.F.,(4,3,3,3,3,3,3,3,3,3,3,3,3,
3,3,3,3,3,3,3,3,3,3,3,3,3,3,3,4),(72.2566310325652,72.2859297941981,72.3737636727309,
72.461486699375,72.5491218560152,72.6400515203606,72.7275877701938,72.8151109602629,
72.9026417279069,72.9902007108153,73.0778563205066,73.1655693243747,73.2534075878187,
73.2765591707781,73.3643925061663,73.4521152528864,73.5397503894581,73.6306801591956,
73.7182170293888,73.8057410735688,73.8932729269646,73.9808332253236,74.0684904810804,
74.1562053252846,74.244045697205,74.2671885473581,74.3549162028477,74.4425201963733,
74.4826134213612),.UNSPECIFIED.);
#2063=B_SPLINE_CURVE_WITH_KNOTS('',3,(#28793,#28794,#28795,#28796,#28797,
#28798,#28799,#28800,#28801,#28802,#28803,#28804,#28805,#28806,#28807,#28808,
#28809,#28810,#28811,#28812,#28813,#28814,#28815,#28816,#28817,#28818,#28819,
#28820,#28821,#28822,#28823,#28824,#28825,#28826,#28827,#28828,#28829,#28830,
#28831,#28832,#28833,#28834,#28835,#28836,#28837,#28838,#28839,#28840,#28841,
#28842,#28843,#28844,#28845,#28846,#28847,#28848,#28849,#28850,#28851,#28852,
#28853,#28854,#28855,#28856,#28857,#28858,#28859,#28860,#28861,#28862,#28863,
#28864,#28865,#28866,#28867,#28868,#28869,#28870,#28871,#28872,#28873,#28874),
 .UNSPECIFIED.,.F.,.F.,(4,3,3,3,3,3,3,3,3,3,3,3,3,3,3,3,3,3,3,3,3,3,3,3,
3,3,3,4),(72.2566310325652,72.3454121702325,72.4342210251386,72.5230760434829,
72.6120571169164,72.701106864289,72.7903135426155,72.8462588649391,72.9340795741427,
73.0217895139422,73.1094116804342,73.2003462505698,73.2878698305936,73.3753804902946,
73.462898880005,73.550445650528,73.6380893528825,73.7257906130895,73.8136174607711,
73.8368882415192,73.924678010106,74.0123640175841,74.0999671063111,74.1875080509712,
74.2750139307472,74.3624997101212,74.4500028156712,74.4816293874842),
 .UNSPECIFIED.);
#2064=B_SPLINE_CURVE_WITH_KNOTS('',3,(#28875,#28876,#28877,#28878,#28879,
#28880,#28881,#28882,#28883,#28884,#28885,#28886,#28887,#28888,#28889,#28890,
#28891,#28892,#28893,#28894,#28895,#28896,#28897,#28898,#28899,#28900,#28901,
#28902,#28903,#28904,#28905,#28906,#28907,#28908,#28909,#28910,#28911,#28912,
#28913,#28914,#28915,#28916,#28917,#28918,#28919,#28920,#28921,#28922,#28923,
#28924,#28925,#28926,#28927,#28928,#28929,#28930,#28931,#28932,#28933,#28934,
#28935,#28936,#28937,#28938,#28939,#28940,#28941,#28942,#28943,#28944,#28945,
#28946,#28947,#28948,#28949,#28950,#28951,#28952,#28953,#28954,#28955,#28956,
#28957,#28958,#28959,#28960,#28961,#28962,#28963,#28964,#28965,#28966,#28967,
#28968,#28969,#28970,#28971,#28972,#28973,#28974,#28975,#28976,#28977,#28978,
#28979,#28980,#28981,#28982,#28983,#28984,#28985,#28986,#28987,#28988,#28989,
#28990,#28991,#28992,#28993,#28994,#28995,#28996,#28997,#28998,#28999,#29000,
#29001,#29002,#29003,#29004,#29005,#29006,#29007,#29008,#29009,#29010,#29011,
#29012,#29013,#29014,#29015,#29016,#29017,#29018,#29019,#29020,#29021,#29022),
 .UNSPECIFIED.,.F.,.F.,(4,3,3,3,3,3,3,3,3,3,3,3,3,3,3,3,3,3,3,3,3,3,3,3,
3,3,3,3,3,3,3,3,3,3,3,3,3,3,3,3,3,3,3,3,3,3,3,3,3,4),(68.1993438421936,
68.2868799544457,68.3743918464848,68.4619001781807,68.5494256018561,68.6370424526399,
68.7247067162602,68.8125098704793,68.883741358619,68.9715592198387,69.0592662846378,
69.146885552858,69.2378212006506,69.3253418433216,69.4128495564218,69.5003649935408,
69.5879088087369,69.6755495667265,69.7632478855214,69.8510718186493,69.8743707351991,
69.9621889539972,70.0498963808031,70.1375160149733,70.228451527074,70.3159725431061,
70.403480631639,70.4909964458431,70.5785406393583,70.666181775562,70.75388047295,
70.8417047823176,70.8650001117791,70.9528162087551,71.0405215090665,71.1281390146236,
71.2190753238406,71.306594219448,71.3941001942232,71.4816139036052,71.5691560035092,
71.6567950731775,71.7444917173757,71.8323140087043,71.8556294883591,71.9558798743625,
72.0526994036399,72.149249270526,72.2454013365002,72.2566310323726),
 .UNSPECIFIED.);
#2065=B_SPLINE_CURVE_WITH_KNOTS('',3,(#29028,#29029,#29030,#29031,#29032,
#29033,#29034,#29035,#29036,#29037,#29038,#29039,#29040,#29041,#29042,#29043,
#29044,#29045,#29046,#29047,#29048,#29049,#29050,#29051,#29052,#29053,#29054,
#29055,#29056,#29057,#29058,#29059,#29060,#29061,#29062,#29063,#29064,#29065,
#29066,#29067,#29068,#29069,#29070,#29071,#29072,#29073,#29074,#29075,#29076,
#29077,#29078,#29079,#29080,#29081,#29082,#29083,#29084,#29085,#29086,#29087,
#29088,#29089,#29090,#29091,#29092,#29093,#29094,#29095,#29096,#29097,#29098,
#29099,#29100,#29101,#29102,#29103,#29104,#29105,#29106,#29107,#29108,#29109,
#29110,#29111,#29112,#29113,#29114,#29115,#29116,#29117,#29118,#29119,#29120,
#29121,#29122,#29123,#29124,#29125,#29126,#29127,#29128,#29129,#29130,#29131,
#29132,#29133,#29134,#29135,#29136,#29137,#29138,#29139,#29140,#29141,#29142,
#29143,#29144,#29145,#29146,#29147,#29148,#29149,#29150,#29151,#29152,#29153,
#29154,#29155,#29156,#29157,#29158,#29159,#29160,#29161,#29162,#29163,#29164,
#29165,#29166,#29167,#29168,#29169,#29170,#29171,#29172,#29173,#29174,#29175),
 .UNSPECIFIED.,.F.,.F.,(4,3,3,3,3,3,3,3,3,3,3,3,3,3,3,3,3,3,3,3,3,3,3,3,
3,3,3,3,3,3,3,3,3,3,3,3,3,3,3,3,3,3,3,3,3,3,3,3,3,4),(61.9155795617456,
62.0030943691385,62.0906369582788,62.1782762169576,62.2659725002026,62.3537950725185,
62.3796360283978,62.4674537280612,62.5551606326324,62.6427797421225,62.7337154499794,
62.8212359386107,62.9087434996574,62.9962587868648,63.0838024544475,63.1714430689489,
63.2591412464879,63.3469650426888,63.3702654049778,63.4580831375179,63.5457900747693,
63.6334092167075,63.7243449123138,63.8118654326169,63.8993730249961,63.986888343164,
64.0744320413037,64.1620726856125,64.2497708925579,64.3375947173568,64.3608947815578,
64.4487125810028,64.5364195857099,64.6240387955683,64.7149744658895,64.8024950548288,
64.8900027159882,64.9775181030047,65.0650618699846,65.1527025827746,65.2404008580718,
65.3282247505097,65.3515241581379,65.4399937122585,65.5283487397423,65.6166091643991,
65.7058183046457,65.793945781903,65.8836957536443,65.9734457253856),
 .UNSPECIFIED.);
#2066=B_SPLINE_CURVE_WITH_KNOTS('',3,(#29176,#29177,#29178,#29179,#29180,
#29181,#29182,#29183,#29184,#29185,#29186,#29187,#29188,#29189,#29190,#29191,
#29192,#29193,#29194,#29195,#29196,#29197,#29198,#29199,#29200,#29201,#29202,
#29203,#29204,#29205,#29206,#29207,#29208,#29209,#29210,#29211,#29212,#29213,
#29214,#29215,#29216,#29217,#29218,#29219,#29220,#29221,#29222,#29223,#29224,
#29225,#29226,#29227,#29228,#29229,#29230,#29231,#29232,#29233,#29234,#29235,
#29236,#29237,#29238,#29239,#29240,#29241,#29242,#29243,#29244,#29245,#29246,
#29247,#29248,#29249,#29250,#29251,#29252,#29253,#29254),.UNSPECIFIED.,
 .F.,.F.,(4,3,3,3,3,3,3,3,3,3,3,3,3,3,3,3,3,3,3,3,3,3,3,3,3,3,4),(65.9734457256018,
66.071966587094,66.170876506416,66.2703101698331,66.3421535347179,66.4299713959743,
66.5176784608089,66.6052977290641,66.6962333768433,66.7837540195464,66.8712617326777,
66.9587771698269,67.0463209850518,67.1339617430687,67.2216600618898,67.3094839950423,
67.3327829112979,67.4206086965015,67.508321893594,67.5959325367783,67.6834855424027,
67.7710016110476,67.8585014113932,67.9460421365112,68.0336015719711,68.1212568443822,
68.1983677761468),.UNSPECIFIED.);
#2067=B_SPLINE_CURVE_WITH_KNOTS('',3,(#29256,#29257,#29258,#29259,#29260,
#29261,#29262,#29263,#29264,#29265,#29266,#29267,#29268,#29269,#29270,#29271,
#29272,#29273,#29274,#29275,#29276,#29277,#29278,#29279,#29280,#29281,#29282,
#29283,#29284,#29285,#29286,#29287,#29288,#29289,#29290,#29291,#29292,#29293,
#29294,#29295,#29296,#29297,#29298,#29299,#29300,#29301,#29302,#29303,#29304,
#29305,#29306,#29307,#29308,#29309,#29310,#29311,#29312,#29313,#29314,#29315,
#29316,#29317,#29318,#29319,#29320,#29321,#29322,#29323,#29324,#29325,#29326,
#29327,#29328,#29329,#29330,#29331,#29332,#29333,#29334,#29335,#29336,#29337),
 .UNSPECIFIED.,.F.,.F.,(4,3,3,3,3,3,3,3,3,3,3,3,3,3,3,3,3,3,3,3,3,3,3,3,
3,3,3,4),(65.9734457255634,66.0604573157416,66.1473630223652,66.2341866831643,
66.3209558419399,66.4076973439539,66.4944326107321,66.5811830546428,66.6680217582215,
66.7549075930277,66.8419276084371,66.902482605459,66.9903004048339,67.0780074094708,
67.1656266192589,67.2565622896064,67.3440828784753,67.4315905395642,67.5191059265102,
67.6066496934205,67.6942904061413,67.7819886813696,67.8698125737395,67.893111982039,
67.9809172828592,68.0686253054638,68.1562387884845,68.1993438421936),
 .UNSPECIFIED.);
#2068=B_SPLINE_CURVE_WITH_KNOTS('',3,(#29338,#29339,#29340,#29341,#29342,
#29343,#29344,#29345,#29346,#29347,#29348,#29349,#29350,#29351,#29352,#29353,
#29354,#29355,#29356,#29357,#29358,#29359,#29360,#29361,#29362,#29363,#29364,
#29365,#29366,#29367,#29368,#29369,#29370,#29371,#29372,#29373,#29374,#29375,
#29376,#29377,#29378,#29379,#29380,#29381,#29382,#29383,#29384,#29385,#29386,
#29387,#29388,#29389,#29390,#29391,#29392,#29393,#29394,#29395,#29396,#29397,
#29398,#29399,#29400,#29401,#29402,#29403,#29404,#29405,#29406,#29407,#29408,
#29409,#29410,#29411,#29412,#29413,#29414,#29415,#29416,#29417,#29418,#29419,
#29420,#29421,#29422,#29423,#29424,#29425,#29426,#29427,#29428,#29429,#29430,
#29431,#29432,#29433,#29434,#29435,#29436,#29437,#29438,#29439,#29440,#29441,
#29442,#29443,#29444,#29445,#29446,#29447,#29448,#29449,#29450,#29451,#29452,
#29453,#29454,#29455,#29456,#29457,#29458,#29459,#29460,#29461,#29462,#29463,
#29464,#29465,#29466,#29467,#29468,#29469,#29470,#29471,#29472,#29473,#29474,
#29475,#29476,#29477,#29478,#29479,#29480,#29481,#29482,#29483,#29484,#29485,
#29486,#29487,#29488),.UNSPECIFIED.,.F.,.F.,(4,3,3,3,3,3,3,3,3,3,3,3,3,
3,3,3,3,3,3,3,3,3,3,3,3,3,3,3,3,3,3,3,3,3,3,3,3,3,3,3,3,3,3,3,3,3,3,3,3,
3,4),(61.9154900696683,61.9493357225588,62.0371534434491,62.1248603692403,
62.2124794999189,62.3034151998214,62.3909357094296,62.4784432913393,62.5659585992737,
62.6535022874257,62.7411429221594,62.8288411197586,62.9166649356151,62.9399650991389,
63.0277828228104,63.115489751354,63.2031088847533,63.294044583624,63.3815650958578,
63.4690726803538,63.5565879908324,63.644131681484,63.7317723186389,63.8194705186166,
63.9072943367714,63.9305944757189,64.0184122103381,64.1061191498958,64.1937382943618,
64.2846739891039,64.3721945124643,64.4597021080895,64.5472174296879,64.6347611314377,
64.722401779603,64.8100999905526,64.8979238195393,64.9212238522989,65.0090415519821,
65.0967484565731,65.184367566083,65.2753032739325,65.3628237625834,65.4503313236495,
65.5378466108761,65.6253902784785,65.7130308929987,65.8007290705565,65.8885528667756,
65.911853228879,65.9734457253856),.UNSPECIFIED.);
#2069=B_SPLINE_CURVE_WITH_KNOTS('',3,(#29494,#29495,#29496,#29497,#29498,
#29499,#29500,#29501,#29502,#29503,#29504,#29505,#29506,#29507,#29508,#29509,
#29510,#29511,#29512,#29513,#29514,#29515,#29516,#29517,#29518,#29519,#29520,
#29521,#29522,#29523,#29524,#29525,#29526,#29527,#29528,#29529,#29530,#29531,
#29532,#29533,#29534,#29535,#29536,#29537,#29538,#29539,#29540,#29541,#29542,
#29543,#29544,#29545,#29546,#29547,#29548,#29549,#29550,#29551,#29552,#29553,
#29554,#29555,#29556,#29557,#29558,#29559,#29560,#29561,#29562,#29563,#29564,
#29565,#29566,#29567,#29568,#29569,#29570,#29571,#29572,#29573,#29574,#29575,
#29576,#29577,#29578,#29579,#29580,#29581,#29582,#29583,#29584,#29585,#29586,
#29587,#29588,#29589,#29590,#29591,#29592,#29593,#29594,#29595,#29596,#29597,
#29598,#29599,#29600,#29601,#29602,#29603,#29604,#29605,#29606,#29607,#29608,
#29609,#29610,#29611,#29612,#29613,#29614,#29615,#29616,#29617,#29618,#29619,
#29620,#29621,#29622,#29623,#29624,#29625,#29626,#29627,#29628,#29629,#29630,
#29631,#29632,#29633,#29634,#29635,#29636,#29637,#29638,#29639,#29640,#29641),
 .UNSPECIFIED.,.F.,.F.,(4,3,3,3,3,3,3,3,3,3,3,3,3,3,3,3,3,3,3,3,3,3,3,3,
3,3,3,3,3,3,3,3,3,3,3,3,3,3,3,3,3,3,3,3,3,3,3,3,3,4),(55.6330557694626,
55.7206644177684,55.8100638366621,55.8975816477305,55.9850890690198,56.0726067535167,
56.1634200073669,56.2510686078768,56.3387777472702,56.4266088599168,56.4358597689176,
56.5236774922701,56.6113844205208,56.699003553653,56.7899392526336,56.8774597646661,
56.9649673489852,57.0524826593115,57.1400263498352,57.227666986899,57.315365186807,
57.4031890049234,57.4264891454977,57.5143068690178,57.6020137974319,57.6896329307235,
57.7805686296428,57.8680891418233,57.955596726286,58.0431120367513,58.1306557274094,
58.2182963646001,58.3059945646306,58.3938183828625,58.4171185220777,58.5049362472607,
58.5926431773456,58.6802623123135,58.7711980106065,58.8587185244669,58.9462261106077,
59.0337414227479,59.1212851150754,59.2089257539194,59.2966239555957,59.3844477754498,
59.4077478986577,59.5162980886054,59.6233575348318,59.6902604180773),
 .UNSPECIFIED.);
#2070=B_SPLINE_CURVE_WITH_KNOTS('',3,(#29642,#29643,#29644,#29645,#29646,
#29647,#29648,#29649,#29650,#29651,#29652,#29653,#29654,#29655,#29656,#29657,
#29658,#29659,#29660,#29661,#29662,#29663,#29664,#29665,#29666,#29667,#29668,
#29669,#29670,#29671,#29672,#29673,#29674,#29675,#29676,#29677,#29678,#29679,
#29680,#29681,#29682,#29683,#29684,#29685,#29686,#29687,#29688,#29689,#29690,
#29691,#29692,#29693,#29694,#29695,#29696,#29697,#29698,#29699,#29700,#29701,
#29702,#29703,#29704,#29705,#29706,#29707,#29708,#29709,#29710,#29711,#29712,
#29713,#29714,#29715,#29716,#29717,#29718,#29719,#29720),.UNSPECIFIED.,
 .F.,.F.,(4,3,3,3,3,3,3,3,3,3,3,3,3,3,3,3,3,3,3,3,3,3,3,3,3,3,4),(59.690260418206,
59.778775025335,59.8656202866809,59.9524524287172,60.0392927592702,60.1290638882621,
60.21603272593,60.3072050005838,60.3983772752377,60.4861949989082,60.5739019274507,
60.661521060849,60.7524567597201,60.8399772719529,60.9274848564478,61.0150001669254,
61.1025438575758,61.1901844947297,61.2778826947062,61.3657065128596,61.3890066518178,
61.4768208758585,61.5645289299151,61.6522915878727,61.7398434324448,61.8277114970952,
61.9155795617456),.UNSPECIFIED.);
#2071=B_SPLINE_CURVE_WITH_KNOTS('',3,(#29722,#29723,#29724,#29725,#29726,
#29727,#29728,#29729,#29730,#29731,#29732,#29733,#29734,#29735,#29736,#29737,
#29738,#29739,#29740,#29741,#29742,#29743,#29744,#29745,#29746,#29747,#29748,
#29749,#29750,#29751,#29752,#29753,#29754,#29755,#29756,#29757,#29758,#29759,
#29760,#29761,#29762,#29763,#29764,#29765,#29766,#29767,#29768,#29769,#29770,
#29771,#29772,#29773,#29774,#29775,#29776,#29777,#29778,#29779,#29780,#29781,
#29782,#29783,#29784,#29785,#29786,#29787,#29788,#29789,#29790,#29791,#29792,
#29793,#29794,#29795,#29796,#29797,#29798,#29799,#29800),.UNSPECIFIED.,
 .F.,.F.,(4,3,3,3,3,3,3,3,3,3,3,3,3,3,3,3,3,3,3,3,3,3,3,3,3,3,4),(59.6902604184428,
59.7976956859157,59.9067549038095,59.9680769693988,60.0558946929192,60.1436016213334,
60.2312207546254,60.3221564535446,60.4096769657254,60.4971845501883,60.5846998606539,
60.6722435513123,60.7598841885032,60.8475823885341,60.9354062067663,60.9587063459788,
61.0465260474664,61.1342344677518,61.2218546088791,61.3094092434363,61.3969287962241,
61.4844339359927,61.5719453160961,61.6595334475953,61.7471595778553,61.8349151106683,
61.9154900696683),.UNSPECIFIED.);
#2072=B_SPLINE_CURVE_WITH_KNOTS('',3,(#29801,#29802,#29803,#29804,#29805,
#29806,#29807,#29808,#29809,#29810,#29811,#29812,#29813,#29814,#29815,#29816,
#29817,#29818,#29819,#29820,#29821,#29822,#29823,#29824,#29825,#29826,#29827,
#29828,#29829,#29830,#29831,#29832,#29833,#29834,#29835,#29836,#29837,#29838,
#29839,#29840,#29841,#29842,#29843,#29844,#29845,#29846,#29847,#29848,#29849,
#29850,#29851,#29852,#29853,#29854,#29855,#29856,#29857,#29858,#29859,#29860,
#29861,#29862,#29863,#29864,#29865,#29866,#29867,#29868,#29869,#29870,#29871,
#29872,#29873,#29874,#29875,#29876,#29877,#29878,#29879,#29880,#29881,#29882,
#29883,#29884,#29885,#29886,#29887,#29888,#29889,#29890,#29891,#29892,#29893,
#29894,#29895,#29896,#29897,#29898,#29899,#29900,#29901,#29902,#29903,#29904,
#29905,#29906,#29907,#29908,#29909,#29910,#29911,#29912,#29913,#29914,#29915,
#29916,#29917,#29918,#29919,#29920,#29921,#29922,#29923,#29924,#29925,#29926,
#29927,#29928,#29929,#29930,#29931,#29932,#29933,#29934,#29935,#29936,#29937,
#29938,#29939,#29940,#29941,#29942,#29943,#29944,#29945,#29946,#29947,#29948,
#29949,#29950,#29951),.UNSPECIFIED.,.F.,.F.,(4,3,3,3,3,3,3,3,3,3,3,3,3,
3,3,3,3,3,3,3,3,3,3,3,3,3,3,3,3,3,3,3,3,3,3,3,3,3,3,3,3,3,3,3,3,3,3,3,3,
3,4),(55.6321436659148,55.7196876184786,55.8073285818317,55.8950272334287,
55.9828513473999,56.0055594630787,56.0933771867062,56.1810841152312,56.268703248637,
56.3596389475147,56.4471594598168,56.5346670444033,56.622182354995,56.7097260457814,
56.7973666831032,56.8850648832665,56.9728887016325,56.9961888396587,57.0840065632835,
57.1717134918052,57.259332625207,57.350268324086,57.4377888363829,57.525296420964,
57.6128117315495,57.7003554223297,57.7879960596445,57.8756942598004,57.9635180781585,
57.9868182162387,58.0746359401024,58.1623428688641,58.2499620025063,58.3408977012954,
58.4284182138326,58.5159257986535,58.6034411094777,58.6909848004959,58.7786254380462,
58.8663236384361,58.954147457025,58.9774475928188,59.0665491959922,59.1535112708394,
59.2403929917781,59.3272158146787,59.4179769655605,59.5047630074283,59.5915521894354,
59.6783867677613,59.690260418206),.UNSPECIFIED.);
#2073=B_SPLINE_CURVE_WITH_KNOTS('',3,(#29957,#29958,#29959,#29960,#29961,
#29962,#29963,#29964,#29965,#29966,#29967,#29968,#29969,#29970,#29971,#29972,
#29973,#29974,#29975,#29976,#29977,#29978,#29979,#29980,#29981,#29982,#29983,
#29984,#29985,#29986,#29987,#29988,#29989,#29990,#29991,#29992,#29993,#29994,
#29995,#29996,#29997,#29998,#29999,#30000,#30001,#30002,#30003,#30004,#30005,
#30006,#30007,#30008,#30009,#30010,#30011,#30012,#30013,#30014,#30015,#30016,
#30017,#30018,#30019,#30020,#30021,#30022,#30023,#30024,#30025,#30026,#30027,
#30028,#30029,#30030,#30031,#30032,#30033,#30034,#30035,#30036,#30037,#30038,
#30039,#30040,#30041,#30042,#30043,#30044,#30045,#30046,#30047,#30048,#30049,
#30050,#30051,#30052,#30053,#30054,#30055,#30056,#30057,#30058,#30059,#30060,
#30061,#30062,#30063,#30064,#30065,#30066,#30067,#30068,#30069,#30070,#30071,
#30072,#30073,#30074,#30075,#30076,#30077,#30078,#30079,#30080,#30081,#30082,
#30083,#30084,#30085,#30086,#30087,#30088,#30089,#30090,#30091,#30092,#30093,
#30094,#30095,#30096,#30097,#30098,#30099,#30100,#30101,#30102,#30103,#30104),
 .UNSPECIFIED.,.F.,.F.,(4,3,3,3,3,3,3,3,3,3,3,3,3,3,3,3,3,3,3,3,3,3,3,3,
3,3,3,3,3,3,3,3,3,3,3,3,3,3,3,3,3,3,3,3,3,3,3,3,3,4),(49.3487655263348,
49.4365711876644,49.5014541328574,49.5892718565205,49.676978785081,49.764597918522,
49.8555336173865,49.9430541297232,50.0305617143443,50.11807702497,50.2056207157903,
50.2932613531451,50.3809595533411,50.4687833717389,50.4920835094375,50.5799012330941,
50.6676081616481,50.7552272950827,50.8461629939495,50.9336835062799,51.0211910908946,
51.108706401514,51.1962500923282,51.2838907296769,51.3715889298668,51.4594127482588,
51.4827128860175,51.5705306096707,51.6582375382213,51.7458566716524,51.8367923705205,
51.9243128828472,52.0118204674583,52.0993357780739,52.1868794688843,52.2745201062292,
52.3622183064152,52.4500421248034,52.4733422625975,52.5604221705999,52.6473917779251,
52.7342748966387,52.8210968702446,52.9078870051228,52.9946666871667,53.0814572897348,
53.1683305097564,53.2552470966048,53.3422944293362,53.4070751108575),
 .UNSPECIFIED.);
#2074=B_SPLINE_CURVE_WITH_KNOTS('',3,(#30105,#30106,#30107,#30108,#30109,
#30110,#30111,#30112,#30113,#30114,#30115,#30116,#30117,#30118,#30119,#30120,
#30121,#30122,#30123,#30124,#30125,#30126,#30127,#30128,#30129,#30130,#30131,
#30132,#30133,#30134,#30135,#30136,#30137,#30138,#30139,#30140,#30141,#30142,
#30143,#30144,#30145,#30146,#30147,#30148,#30149,#30150,#30151,#30152,#30153,
#30154,#30155,#30156,#30157,#30158,#30159,#30160,#30161,#30162,#30163,#30164,
#30165,#30166,#30167,#30168,#30169,#30170,#30171,#30172,#30173,#30174,#30175,
#30176,#30177,#30178,#30179,#30180,#30181,#30182,#30183,#30184,#30185,#30186,
#30187,#30188,#30189),.UNSPECIFIED.,.F.,.F.,(4,3,3,3,3,3,3,3,3,3,3,3,3,
3,3,3,3,3,3,3,3,3,3,3,3,3,3,3,4),(53.4070751110265,53.4639716391775,53.551789362805,
53.63949629133,53.7271154247358,53.8180511236135,53.9055716359155,53.9930792205021,
54.0805945310936,54.1681382218801,54.2557788592019,54.3434770593653,54.4313008777312,
54.4546010157576,54.5424187393823,54.6301256679039,54.7177448013059,54.8086805001848,
54.8962010124817,54.9837085970627,55.0712239076482,55.1587675984283,55.2464082357429,
55.3341064358986,55.4219302542566,55.4452303923376,55.5330632323005,55.6207748440915,
55.6330557694626),.UNSPECIFIED.);
#2075=B_SPLINE_CURVE_WITH_KNOTS('',3,(#30191,#30192,#30193,#30194,#30195,
#30196,#30197,#30198,#30199,#30200,#30201,#30202,#30203,#30204,#30205,#30206,
#30207,#30208,#30209,#30210,#30211,#30212,#30213,#30214,#30215,#30216,#30217,
#30218,#30219,#30220,#30221,#30222,#30223,#30224,#30225,#30226,#30227,#30228,
#30229,#30230,#30231,#30232,#30233,#30234,#30235,#30236,#30237,#30238,#30239,
#30240,#30241,#30242,#30243,#30244,#30245,#30246,#30247,#30248,#30249,#30250,
#30251,#30252,#30253,#30254,#30255,#30256,#30257,#30258,#30259,#30260,#30261,
#30262,#30263,#30264,#30265,#30266,#30267,#30268,#30269),.UNSPECIFIED.,
 .F.,.F.,(4,3,3,3,3,3,3,3,3,3,3,3,3,3,3,3,3,3,3,3,3,3,3,3,3,3,4),(53.4070751110265,
53.4952697145479,53.5834738756999,53.6717071431074,53.7600512896627,53.8484511190497,
53.9370104139044,54.0243007099186,54.1121184335719,54.1998253621223,54.2874444955536,
54.3783801944217,54.4659007067484,54.5534082913594,54.6409236019752,54.7284672927857,
54.8161079301308,54.9038061303171,54.9916299487052,55.0149300864986,55.1027351460835,
55.1904358979974,55.2780531734501,55.3665757965662,55.4540917123707,55.5431176891427,
55.6321436659148),.UNSPECIFIED.);
#2076=B_SPLINE_CURVE_WITH_KNOTS('',3,(#30270,#30271,#30272,#30273,#30274,
#30275,#30276,#30277,#30278,#30279,#30280,#30281,#30282,#30283,#30284,#30285,
#30286,#30287,#30288,#30289,#30290,#30291,#30292,#30293,#30294,#30295,#30296,
#30297,#30298,#30299,#30300,#30301,#30302,#30303,#30304,#30305,#30306,#30307,
#30308,#30309,#30310,#30311,#30312,#30313,#30314,#30315,#30316,#30317,#30318,
#30319,#30320,#30321,#30322,#30323,#30324,#30325,#30326,#30327,#30328,#30329,
#30330,#30331,#30332,#30333,#30334,#30335,#30336,#30337,#30338,#30339,#30340,
#30341,#30342,#30343,#30344,#30345,#30346,#30347,#30348,#30349,#30350,#30351,
#30352,#30353,#30354,#30355,#30356,#30357,#30358,#30359,#30360,#30361,#30362,
#30363,#30364,#30365,#30366,#30367,#30368,#30369,#30370,#30371,#30372,#30373,
#30374,#30375,#30376,#30377,#30378,#30379,#30380,#30381,#30382,#30383,#30384,
#30385,#30386,#30387,#30388,#30389,#30390,#30391,#30392,#30393,#30394,#30395,
#30396,#30397,#30398,#30399,#30400,#30401,#30402,#30403,#30404,#30405,#30406,
#30407,#30408,#30409,#30410,#30411,#30412,#30413,#30414),.UNSPECIFIED.,
 .F.,.F.,(4,3,3,3,3,3,3,3,3,3,3,3,3,3,3,3,3,3,3,3,3,3,3,3,3,3,3,3,3,3,3,
3,3,3,3,3,3,3,3,3,3,3,3,3,3,3,3,3,4),(49.3498290191458,49.4388232922024,
49.5263404425959,49.6138478724993,49.7013662347429,49.7914704769568,49.8791203266202,
49.9704517651093,50.0617832035985,50.1496009272579,50.2373078558148,50.3249269892522,
50.4158626881179,50.5033832004509,50.5908907850685,50.6784060956906,50.7659497865075,
50.8535904238588,50.9412886240512,51.0291124424458,51.0524125801785,51.1402303038372,
51.2279372323932,51.3155563658296,51.4064920646957,51.494012577028,51.5815201616446,
51.6690354722663,51.7565791630819,51.8442198004324,51.9319180006241,52.0197418190178,
52.0430419567586,52.1308596804216,52.218566608982,52.3061857424226,52.3971214412871,
52.4846419536238,52.572149538245,52.6596648488705,52.7472085396912,52.834849177046,
52.9225473772421,53.0103711956399,53.0336713333386,53.132711821951,53.2314411213962,
53.3295918554785,53.4070751108119),.UNSPECIFIED.);
#2077=B_SPLINE_CURVE_WITH_KNOTS('',3,(#30420,#30421,#30422,#30423,#30424,
#30425,#30426,#30427,#30428,#30429,#30430,#30431,#30432,#30433,#30434,#30435,
#30436,#30437,#30438,#30439,#30440,#30441,#30442,#30443,#30444,#30445,#30446,
#30447,#30448,#30449,#30450,#30451,#30452,#30453,#30454,#30455,#30456,#30457,
#30458,#30459,#30460,#30461,#30462,#30463,#30464,#30465,#30466,#30467,#30468,
#30469,#30470,#30471,#30472,#30473,#30474,#30475,#30476,#30477,#30478,#30479,
#30480,#30481,#30482,#30483,#30484,#30485,#30486,#30487,#30488,#30489,#30490,
#30491,#30492,#30493,#30494,#30495,#30496,#30497,#30498,#30499,#30500,#30501,
#30502,#30503,#30504,#30505,#30506,#30507,#30508,#30509,#30510,#30511,#30512,
#30513,#30514,#30515,#30516,#30517,#30518,#30519,#30520,#30521,#30522,#30523,
#30524,#30525,#30526,#30527,#30528,#30529,#30530,#30531,#30532,#30533,#30534,
#30535,#30536,#30537,#30538,#30539,#30540,#30541,#30542,#30543,#30544,#30545,
#30546,#30547,#30548,#30549,#30550,#30551,#30552,#30553,#30554,#30555,#30556,
#30557,#30558,#30559,#30560,#30561,#30562,#30563,#30564,#30565,#30566,#30567),
 .UNSPECIFIED.,.F.,.F.,(4,3,3,3,3,3,3,3,3,3,3,3,3,3,3,3,3,3,3,3,3,3,3,3,
3,3,3,3,3,3,3,3,3,3,3,3,3,3,3,3,3,3,3,3,3,3,3,3,3,4),(43.066105953779,43.1536162830819,
43.2411478989153,43.3287730650111,43.4164494147267,43.5042595695875,43.5576778733773,
43.6454955970374,43.733202525595,43.8208216590329,43.9117573578984,43.9992778702323,
44.0867854548505,44.1743007654736,44.2618444562913,44.3494850936434,44.4371832938366,
44.5250071122318,44.5483072499573,44.6361249736168,44.7238319021737,44.8114510356111,
44.9023867344769,44.9899072468099,45.0774148314276,45.1649301420498,45.2524738328665,
45.3401144702178,45.42781267041,45.5156364888046,45.5389366265373,45.6267543501968,
45.7144612787537,45.802080412191,45.8930161110568,45.9805366233901,46.0680442080077,
46.1555595186299,46.2431032094466,46.3307438467981,46.418442046991,46.5062658653857,
46.5295660031174,46.6186563250424,46.7076259258596,46.796493725915,46.8852637004644,
46.9739759768119,47.0626512944817,47.1238898038469),.UNSPECIFIED.);
#2078=B_SPLINE_CURVE_WITH_KNOTS('',3,(#30568,#30569,#30570,#30571,#30572,
#30573,#30574,#30575,#30576,#30577,#30578,#30579,#30580,#30581,#30582,#30583,
#30584,#30585,#30586,#30587,#30588,#30589,#30590,#30591,#30592,#30593,#30594,
#30595,#30596,#30597,#30598,#30599,#30600,#30601,#30602,#30603,#30604,#30605,
#30606,#30607,#30608,#30609,#30610,#30611,#30612,#30613,#30614,#30615,#30616,
#30617,#30618,#30619,#30620,#30621,#30622,#30623,#30624,#30625,#30626,#30627,
#30628,#30629,#30630,#30631,#30632,#30633,#30634,#30635,#30636,#30637,#30638,
#30639,#30640,#30641,#30642,#30643,#30644,#30645,#30646),.UNSPECIFIED.,
 .F.,.F.,(4,3,3,3,3,3,3,3,3,3,3,3,3,3,3,3,3,3,3,3,3,3,3,3,3,3,4),(47.1238898040446,
47.2229661979578,47.3199017158542,47.4200485477758,47.5201953796974,47.6080131033568,
47.6957200319136,47.783339165351,47.8742748642168,47.96179537655,48.0493029611675,
48.1368182717895,48.2243619626063,48.3120025999577,48.3997008001501,48.4875246185446,
48.5108247562774,48.5986518168607,48.6863658889768,48.773976251605,48.8615284122451,
48.9490430728508,49.0365409029311,49.1240737177044,49.2116250178335,49.2992578827453,
49.3487655263348),.UNSPECIFIED.);
#2079=B_SPLINE_CURVE_WITH_KNOTS('',3,(#30648,#30649,#30650,#30651,#30652,
#30653,#30654,#30655,#30656,#30657,#30658,#30659,#30660,#30661,#30662,#30663,
#30664,#30665,#30666,#30667,#30668,#30669,#30670,#30671,#30672,#30673,#30674,
#30675,#30676,#30677,#30678,#30679,#30680,#30681,#30682,#30683,#30684,#30685,
#30686,#30687,#30688,#30689,#30690,#30691,#30692,#30693,#30694,#30695,#30696,
#30697,#30698,#30699,#30700,#30701,#30702,#30703,#30704,#30705,#30706,#30707,
#30708,#30709,#30710,#30711,#30712,#30713,#30714,#30715,#30716,#30717,#30718,
#30719,#30720,#30721,#30722,#30723,#30724,#30725,#30726,#30727,#30728,#30729),
 .UNSPECIFIED.,.F.,.F.,(4,3,3,3,3,3,3,3,3,3,3,3,3,3,3,3,3,3,3,3,3,3,3,3,
3,3,3,4),(47.1238898040745,47.2112205230592,47.2984421477868,47.3855782233556,
47.4726547355819,47.5596998923597,47.6467348498394,47.7337807519277,47.8209134726712,
47.9080890145165,47.9954065966275,48.0805244504385,48.1683421740981,48.2560491026549,
48.3436682360924,48.4346039349582,48.5221244472913,48.609632031909,48.6971473425312,
48.7846910333482,48.8723316706997,48.9600298708923,49.047853689287,49.0711538270185,
49.1589647608137,49.2466781839727,49.3342970267764,49.3498290191458),
 .UNSPECIFIED.);
#2080=B_SPLINE_CURVE_WITH_KNOTS('',3,(#30730,#30731,#30732,#30733,#30734,
#30735,#30736,#30737,#30738,#30739,#30740,#30741,#30742,#30743,#30744,#30745,
#30746,#30747,#30748,#30749,#30750,#30751,#30752,#30753,#30754,#30755,#30756,
#30757,#30758,#30759,#30760,#30761,#30762,#30763,#30764,#30765,#30766,#30767,
#30768,#30769,#30770,#30771,#30772,#30773,#30774,#30775,#30776,#30777,#30778,
#30779,#30780,#30781,#30782,#30783,#30784,#30785,#30786,#30787,#30788,#30789,
#30790,#30791,#30792,#30793,#30794,#30795,#30796,#30797,#30798,#30799,#30800,
#30801,#30802,#30803,#30804,#30805,#30806,#30807,#30808,#30809,#30810,#30811,
#30812,#30813,#30814,#30815,#30816,#30817,#30818,#30819,#30820,#30821,#30822,
#30823,#30824,#30825,#30826,#30827,#30828,#30829,#30830,#30831,#30832,#30833,
#30834,#30835,#30836,#30837,#30838,#30839,#30840,#30841,#30842,#30843,#30844,
#30845,#30846,#30847,#30848,#30849,#30850,#30851,#30852,#30853,#30854,#30855,
#30856,#30857,#30858,#30859,#30860,#30861,#30862,#30863,#30864,#30865,#30866,
#30867,#30868,#30869,#30870,#30871,#30872,#30873,#30874,#30875,#30876,#30877,
#30878,#30879,#30880),.UNSPECIFIED.,.F.,.F.,(4,3,3,3,3,3,3,3,3,3,3,3,3,
3,3,3,3,3,3,3,3,3,3,3,3,3,3,3,3,3,3,3,3,3,3,3,3,3,3,3,3,3,3,3,3,3,3,3,3,
3,4),(43.0658132987337,43.1273775675383,43.2151952912011,43.3029022197614,
43.3905213532023,43.4814570520668,43.5689775644035,43.6564851490246,43.7440004596503,
43.8315441504707,43.9191847878257,44.0068829880218,44.0947068064199,44.1180069441183,
44.205824667777,44.293531596333,44.3811507297697,44.4720864286357,44.559606940968,
44.6471145255847,44.734629836206,44.8221735270219,44.9098141643725,44.9975123645641,
45.0853361829578,45.1086363206984,45.1964540443579,45.2841609729148,45.3717801063522,
45.462715805218,45.5502363175511,45.6377439021686,45.7252592127907,45.8128029036075,
45.9004435409588,45.9881417411512,46.0759655595456,46.0992656972784,46.1870834209385,
46.274790349496,46.3624094829342,46.4533451817997,46.5408656941335,46.6283732787517,
46.7158885893745,46.803432280192,46.8910729175441,46.9787711177372,47.0665949361323,
47.0898950738584,47.1238898038469),.UNSPECIFIED.);
#2081=B_SPLINE_CURVE_WITH_KNOTS('',3,(#30886,#30887,#30888,#30889,#30890,
#30891,#30892,#30893,#30894,#30895,#30896,#30897,#30898,#30899,#30900,#30901,
#30902,#30903,#30904,#30905,#30906,#30907,#30908,#30909,#30910,#30911,#30912,
#30913,#30914,#30915,#30916,#30917,#30918,#30919,#30920,#30921,#30922,#30923,
#30924,#30925,#30926,#30927,#30928,#30929,#30930,#30931,#30932,#30933,#30934,
#30935,#30936,#30937,#30938,#30939,#30940,#30941,#30942,#30943,#30944,#30945,
#30946,#30947,#30948,#30949,#30950,#30951,#30952,#30953,#30954,#30955,#30956,
#30957,#30958,#30959,#30960,#30961,#30962,#30963,#30964,#30965,#30966,#30967,
#30968,#30969,#30970,#30971,#30972,#30973,#30974,#30975,#30976,#30977,#30978,
#30979,#30980,#30981,#30982,#30983,#30984,#30985,#30986,#30987,#30988,#30989,
#30990,#30991,#30992,#30993,#30994,#30995,#30996,#30997,#30998,#30999,#31000,
#31001,#31002,#31003,#31004,#31005,#31006,#31007,#31008,#31009,#31010,#31011,
#31012,#31013,#31014,#31015,#31016,#31017,#31018,#31019,#31020,#31021,#31022,
#31023,#31024,#31025,#31026,#31027,#31028,#31029,#31030,#31031,#31032,#31033),
 .UNSPECIFIED.,.F.,.F.,(4,3,3,3,3,3,3,3,3,3,3,3,3,3,3,3,3,3,3,3,3,3,3,3,
3,3,3,3,3,3,3,3,3,3,3,3,3,3,3,3,3,3,3,3,3,3,3,3,3,4),(36.7834780077634,
36.8711108279984,36.9586747705779,37.0462007156381,37.1337093249822,37.221221254129,
37.308757155933,37.3963879233731,37.4840722897725,37.5718873015088,37.6139016138971,
37.7017193375818,37.7894262661642,37.8770453996276,37.9679810984838,38.0555016108434,
38.1430091954876,38.2305245061365,38.3180681969803,38.4057088343586,38.4934070345781,
38.5812308529995,38.6045309904771,38.6923487141303,38.7800556426808,38.867674776112,
38.9586104749801,39.0461309873068,39.1336385719179,39.2211538825335,39.3086975733438,
39.3963382106888,39.484036410875,39.5718602292632,39.5951603670572,39.6829780907142,
39.7706850192686,39.8583041527034,39.9492398515702,40.0367603639006,40.1242679485154,
40.2117832591348,40.2993269499485,40.386967587297,40.4746657874866,40.5624896058781,
40.5857897436372,40.6987530453557,40.8096059142877,40.8407044965426),
 .UNSPECIFIED.);
#2082=B_SPLINE_CURVE_WITH_KNOTS('',3,(#31034,#31035,#31036,#31037,#31038,
#31039,#31040,#31041,#31042,#31043,#31044,#31045,#31046,#31047,#31048,#31049,
#31050,#31051,#31052,#31053,#31054,#31055,#31056,#31057,#31058,#31059,#31060,
#31061,#31062,#31063,#31064,#31065,#31066,#31067,#31068,#31069,#31070,#31071,
#31072,#31073,#31074,#31075,#31076,#31077,#31078,#31079,#31080,#31081,#31082,
#31083,#31084,#31085,#31086,#31087,#31088,#31089,#31090,#31091,#31092,#31093,
#31094,#31095,#31096,#31097,#31098,#31099,#31100,#31101,#31102,#31103,#31104,
#31105,#31106,#31107,#31108,#31109,#31110,#31111,#31112,#31113,#31114,#31115),
 .UNSPECIFIED.,.F.,.F.,(4,3,3,3,3,3,3,3,3,3,3,3,3,3,3,3,3,3,3,3,3,3,3,3,
3,3,3,4),(40.8407044966673,40.9273584362615,41.0139637234795,41.1005454082225,
41.1871250286696,41.2737241173095,41.3604139263767,41.4471549251354,41.5340255171284,
41.5764191202172,41.6642368438759,41.751943772432,41.8395629058689,41.9304986047349,
42.0180191170672,42.1055267016839,42.1930420123052,42.2805857031212,42.3682263404716,
42.4559245406634,42.543748359057,42.5670484967972,42.6548657905452,42.7425763486162,
42.8301869071651,42.9177390596797,43.0052579701394,43.066105953779),
 .UNSPECIFIED.);
#2083=B_SPLINE_CURVE_WITH_KNOTS('',3,(#31117,#31118,#31119,#31120,#31121,
#31122,#31123,#31124,#31125,#31126,#31127,#31128,#31129,#31130,#31131,#31132,
#31133,#31134,#31135,#31136,#31137,#31138,#31139,#31140,#31141,#31142,#31143,
#31144,#31145,#31146,#31147,#31148,#31149,#31150,#31151,#31152,#31153,#31154,
#31155,#31156,#31157,#31158,#31159,#31160,#31161,#31162,#31163,#31164,#31165,
#31166,#31167,#31168,#31169,#31170,#31171,#31172,#31173,#31174,#31175,#31176,
#31177,#31178,#31179,#31180,#31181,#31182,#31183,#31184,#31185,#31186,#31187,
#31188,#31189,#31190,#31191,#31192,#31193,#31194,#31195),.UNSPECIFIED.,
 .F.,.F.,(4,3,3,3,3,3,3,3,3,3,3,3,3,3,3,3,3,3,3,3,3,3,3,3,3,3,4),(40.8407044968387,
40.9448640923073,41.0502373865448,41.1461188143783,41.2339365380315,41.321643466582,
41.4092626000131,41.5001982988812,41.5877188112079,41.675226395819,41.7627417064346,
41.8502853972449,41.9379260345899,42.0256242347759,42.1134480531641,42.1367481909583,
42.224569549071,42.3122792278348,42.3999002310044,42.487454050736,42.5749722254964,
42.6624754241107,42.7499842994785,42.8375628990187,42.9251792682597,43.0129084859427,
43.0658132987337),.UNSPECIFIED.);
#2084=B_SPLINE_CURVE_WITH_KNOTS('',3,(#31196,#31197,#31198,#31199,#31200,
#31201,#31202,#31203,#31204,#31205,#31206,#31207,#31208,#31209,#31210,#31211,
#31212,#31213,#31214,#31215,#31216,#31217,#31218,#31219,#31220,#31221,#31222,
#31223,#31224,#31225,#31226,#31227,#31228,#31229,#31230,#31231,#31232,#31233,
#31234,#31235,#31236,#31237,#31238,#31239,#31240,#31241,#31242,#31243,#31244,
#31245,#31246,#31247,#31248,#31249,#31250,#31251,#31252,#31253,#31254,#31255,
#31256,#31257,#31258,#31259,#31260,#31261,#31262,#31263,#31264,#31265,#31266,
#31267,#31268,#31269,#31270,#31271,#31272,#31273,#31274,#31275,#31276,#31277,
#31278,#31279,#31280,#31281,#31282,#31283,#31284,#31285,#31286,#31287,#31288,
#31289,#31290,#31291,#31292,#31293,#31294,#31295,#31296,#31297,#31298,#31299,
#31300,#31301,#31302,#31303,#31304,#31305,#31306,#31307,#31308,#31309,#31310,
#31311,#31312,#31313,#31314,#31315,#31316,#31317,#31318,#31319,#31320,#31321,
#31322,#31323,#31324,#31325,#31326,#31327,#31328,#31329,#31330,#31331,#31332,
#31333,#31334,#31335,#31336,#31337,#31338,#31339,#31340,#31341,#31342,#31343),
 .UNSPECIFIED.,.F.,.F.,(4,3,3,3,3,3,3,3,3,3,3,3,3,3,3,3,3,3,3,3,3,3,3,3,
3,3,3,3,3,3,3,3,3,3,3,3,3,3,3,3,3,3,3,3,3,3,3,3,3,4),(36.7826585774627,
36.8701913327661,36.9578180023401,37.0454965173817,37.1333079644416,37.1836013080582,
37.2714190319113,37.3591259606641,37.4467450942998,37.5376807930921,37.6252013056277,
37.7127088904491,37.8002242012759,37.8877678922981,37.9754085298552,38.0631067302538,
38.1509305488533,38.1742306846382,38.2620484082614,38.3497553367818,38.4373744701828,
38.5283101690622,38.6158306813589,38.7033382659399,38.7908535765259,38.8783972673068,
38.9660379046225,39.0537361047798,39.1415599231395,39.1648600612182,39.2526777848493,
39.3403847133773,39.4280038467855,39.5189395456621,39.6064600579645,39.6939676425513,
39.7814829531424,39.8690266439274,39.9566672812469,40.0443654814074,40.1321892997699,
40.1554894377982,40.2428859234006,40.3301773559497,40.417384958565,40.5045298835637,
40.5916445939301,40.6787389693881,40.7658659690996,40.8407044966673),
 .UNSPECIFIED.);
#2085=B_SPLINE_CURVE_WITH_KNOTS('',3,(#31349,#31350,#31351,#31352,#31353,
#31354,#31355,#31356,#31357,#31358,#31359,#31360,#31361,#31362,#31363,#31364,
#31365,#31366,#31367,#31368,#31369,#31370,#31371,#31372,#31373,#31374,#31375,
#31376,#31377,#31378,#31379,#31380,#31381,#31382,#31383,#31384,#31385,#31386,
#31387,#31388,#31389,#31390,#31391,#31392,#31393,#31394,#31395,#31396,#31397,
#31398,#31399,#31400,#31401,#31402,#31403,#31404,#31405,#31406,#31407,#31408,
#31409,#31410,#31411,#31412,#31413,#31414,#31415,#31416,#31417,#31418,#31419,
#31420,#31421,#31422,#31423,#31424,#31425,#31426,#31427,#31428,#31429,#31430,
#31431,#31432,#31433,#31434,#31435,#31436,#31437,#31438,#31439,#31440,#31441,
#31442,#31443,#31444,#31445,#31446,#31447,#31448,#31449,#31450,#31451,#31452,
#31453,#31454,#31455,#31456,#31457,#31458,#31459,#31460,#31461,#31462,#31463,
#31464,#31465,#31466,#31467,#31468,#31469,#31470,#31471,#31472,#31473,#31474,
#31475,#31476,#31477,#31478,#31479,#31480,#31481,#31482,#31483,#31484,#31485,
#31486,#31487,#31488,#31489,#31490,#31491,#31492,#31493,#31494,#31495,#31496),
 .UNSPECIFIED.,.F.,.F.,(4,3,3,3,3,3,3,3,3,3,3,3,3,3,3,3,3,3,3,3,3,3,3,3,
3,3,3,3,3,3,3,3,3,3,3,3,3,3,3,3,3,3,3,3,3,3,3,3,3,4),(30.4991828016751,
30.589339389756,30.6794959778369,30.7673136989645,30.8550206249472,30.9426397557717,
31.0335754556023,31.1210959652419,31.2086035471408,31.2961188550221,31.3836625430786,
31.4713031776546,31.5590013750598,31.6468251906704,31.6701253544169,31.7579430795308,
31.8456500095597,31.9332691444848,32.0242048427988,32.1117253566494,32.1992329427927,
32.2867482549473,32.3742919473016,32.4619325861903,32.5496307879217,32.637454607846,
32.660754730997,32.7485724544946,32.8362793828906,32.9238985161683,33.0148342150944,
33.1023547272717,33.1898623117352,33.2773776222052,33.3649213128719,33.4525619500772,
33.5402601501255,33.6280839683802,33.651384107577,33.738220097186,33.8249459927482,
33.9115858331361,33.9981647376526,34.0847124756467,34.1712506293001,34.2578007688055,
34.3444298629893,34.4311037976332,34.517896294793,34.5575191892807),
 .UNSPECIFIED.);
#2086=B_SPLINE_CURVE_WITH_KNOTS('',3,(#31497,#31498,#31499,#31500,#31501,
#31502,#31503,#31504,#31505,#31506,#31507,#31508,#31509,#31510,#31511,#31512,
#31513,#31514,#31515,#31516,#31517,#31518,#31519,#31520,#31521,#31522,#31523,
#31524,#31525,#31526,#31527,#31528,#31529,#31530,#31531,#31532,#31533,#31534,
#31535,#31536,#31537,#31538,#31539,#31540,#31541,#31542,#31543,#31544,#31545,
#31546,#31547,#31548,#31549,#31550,#31551,#31552,#31553,#31554,#31555,#31556,
#31557,#31558,#31559,#31560,#31561,#31562,#31563,#31564,#31565,#31566,#31567,
#31568,#31569,#31570,#31571,#31572,#31573,#31574,#31575,#31576,#31577,#31578),
 .UNSPECIFIED.,.F.,.F.,(4,3,3,3,3,3,3,3,3,3,3,3,3,3,3,3,3,3,3,3,3,3,3,3,
3,3,3,4),(34.5575191894877,34.642013484157,34.7298312080103,34.8175381367635,
34.9051572703995,34.9960929691917,35.0836134817277,35.1711210665493,35.2586363773767,
35.3461800683992,35.4338207059567,35.5215189063556,35.6093427249555,35.6326428607371,
35.7204605843602,35.8081675128806,35.8957866462814,35.9867223451609,36.0742428574575,
36.1617504420386,36.2492657526244,36.336809443405,36.4244500807206,36.5121482808776,
36.5999720992373,36.6232722373171,36.7110751632177,36.7834780077634),
 .UNSPECIFIED.);
#2087=B_SPLINE_CURVE_WITH_KNOTS('',3,(#31580,#31581,#31582,#31583,#31584,
#31585,#31586,#31587,#31588,#31589,#31590,#31591,#31592,#31593,#31594,#31595,
#31596,#31597,#31598,#31599,#31600,#31601,#31602,#31603,#31604,#31605,#31606,
#31607,#31608,#31609,#31610,#31611,#31612,#31613,#31614,#31615,#31616,#31617,
#31618,#31619,#31620,#31621,#31622,#31623,#31624,#31625,#31626,#31627,#31628,
#31629,#31630,#31631,#31632,#31633,#31634,#31635,#31636,#31637,#31638,#31639,
#31640,#31641,#31642,#31643,#31644,#31645,#31646,#31647,#31648,#31649,#31650,
#31651,#31652,#31653,#31654,#31655,#31656,#31657,#31658,#31659,#31660,#31661),
 .UNSPECIFIED.,.F.,.F.,(4,3,3,3,3,3,3,3,3,3,3,3,3,3,3,3,3,3,3,3,3,3,3,3,
3,3,3,4),(34.5575191894877,34.6452189800033,34.7329127229612,34.820620735829,
34.9083633412095,34.9962128842465,35.0841247009442,35.1721722075712,35.2023425548981,
35.2901602783961,35.3778672067924,35.4654863400703,35.5564220389963,35.643942551174,
35.7314501356379,35.8189654461081,35.9065091367756,35.9941497739812,36.08184797403,
36.1696717922849,36.1929719314781,36.2807796092137,36.3684824138544,36.4561011792004,
36.543654683778,36.6311690802082,36.7186812678126,36.7826585774627),
 .UNSPECIFIED.);
#2088=B_SPLINE_CURVE_WITH_KNOTS('',3,(#31662,#31663,#31664,#31665,#31666,
#31667,#31668,#31669,#31670,#31671,#31672,#31673,#31674,#31675,#31676,#31677,
#31678,#31679,#31680,#31681,#31682,#31683,#31684,#31685,#31686,#31687,#31688,
#31689,#31690,#31691,#31692,#31693,#31694,#31695,#31696,#31697,#31698,#31699,
#31700,#31701,#31702,#31703,#31704,#31705,#31706,#31707,#31708,#31709,#31710,
#31711,#31712,#31713,#31714,#31715,#31716,#31717,#31718,#31719,#31720,#31721,
#31722,#31723,#31724,#31725,#31726,#31727,#31728,#31729,#31730,#31731,#31732,
#31733,#31734,#31735,#31736,#31737,#31738,#31739,#31740,#31741,#31742,#31743,
#31744,#31745,#31746,#31747,#31748,#31749,#31750,#31751,#31752,#31753,#31754,
#31755,#31756,#31757,#31758,#31759,#31760,#31761,#31762,#31763,#31764,#31765,
#31766,#31767,#31768,#31769,#31770,#31771,#31772,#31773,#31774,#31775,#31776,
#31777,#31778,#31779,#31780,#31781,#31782,#31783,#31784,#31785,#31786,#31787,
#31788,#31789,#31790,#31791,#31792,#31793,#31794,#31795,#31796,#31797,#31798,
#31799,#31800,#31801,#31802,#31803,#31804,#31805,#31806,#31807,#31808,#31809),
 .UNSPECIFIED.,.F.,.F.,(4,3,3,3,3,3,3,3,3,3,3,3,3,3,3,3,3,3,3,3,3,3,3,3,
3,3,3,3,3,3,3,3,3,3,3,3,3,3,3,3,3,3,3,3,3,3,3,3,3,4),(30.5003021062259,
30.5878638989066,30.6753888028352,30.7628971416267,30.8504095704628,30.9379467424075,
31.0255791506396,31.1132658507174,31.20108230312,31.239825048578,31.3276427827913,
31.4153497220206,31.5029688662351,31.5939045611004,31.6814250844032,31.7689326800424,
31.8564480017262,31.9439917036335,32.0316323520613,32.1193305633352,32.2071543927338,
32.230454425158,32.31827214858,32.4059790769219,32.4935982101664,32.5845339091129,
32.6720544213114,32.7595620058162,32.8470773163472,32.9346210070955,33.0222616444118,
33.1099598445888,33.1977836629968,33.221083801738,33.308901522868,33.3966084488531,
33.4842275796802,33.5751632795099,33.6626837891521,33.7501913710535,33.8377066789376,
33.9252503669967,34.0128910015754,34.100589198983,34.1884130145959,34.2117131783181,
34.3130674767471,34.4140179529364,34.514233490631,34.5575191892756),
 .UNSPECIFIED.);
#2089=B_SPLINE_CURVE_WITH_KNOTS('',3,(#31815,#31816,#31817,#31818,#31819,
#31820,#31821,#31822,#31823,#31824,#31825,#31826,#31827,#31828,#31829,#31830,
#31831,#31832,#31833,#31834,#31835,#31836,#31837,#31838,#31839,#31840,#31841,
#31842,#31843,#31844,#31845,#31846,#31847,#31848,#31849,#31850,#31851,#31852,
#31853,#31854,#31855,#31856,#31857,#31858,#31859,#31860,#31861,#31862,#31863,
#31864,#31865,#31866,#31867,#31868,#31869,#31870,#31871,#31872,#31873,#31874,
#31875,#31876,#31877,#31878,#31879,#31880,#31881,#31882,#31883,#31884,#31885,
#31886,#31887,#31888,#31889,#31890,#31891,#31892,#31893,#31894,#31895,#31896,
#31897,#31898,#31899,#31900,#31901,#31902,#31903,#31904,#31905,#31906,#31907,
#31908,#31909,#31910,#31911,#31912,#31913,#31914,#31915,#31916,#31917,#31918,
#31919,#31920,#31921,#31922,#31923,#31924,#31925,#31926,#31927,#31928,#31929,
#31930,#31931,#31932,#31933,#31934,#31935,#31936,#31937,#31938,#31939,#31940,
#31941,#31942,#31943,#31944,#31945,#31946,#31947,#31948,#31949,#31950,#31951,
#31952,#31953,#31954,#31955,#31956,#31957,#31958,#31959,#31960,#31961,#31962),
 .UNSPECIFIED.,.F.,.F.,(4,3,3,3,3,3,3,3,3,3,3,3,3,3,3,3,3,3,3,3,3,3,3,3,
3,3,3,3,3,3,3,3,3,3,3,3,3,3,3,3,3,3,3,3,3,3,3,3,3,4),(24.2166325011217,
24.3041405351431,24.3916633633866,24.4792764164281,24.5669348162689,24.6547349628873,
24.7357197183568,24.8235372555985,24.9112439949562,24.9988629366597,25.0897987064443,
25.1773190219343,25.2648264081598,25.3523415190524,25.4398850090128,25.527525444838,
25.615223442877,25.7030470597342,25.7263490949368,25.814166892366,25.9018738954422,
25.9894931040527,26.0804287749857,26.1679493636392,26.2554570248679,26.3429724123092,
26.4305161800693,26.5181568941627,26.6058551710695,26.6936790655524,26.7169784715168,
26.804796201569,26.8925031368074,26.9801222772054,27.0710579735669,27.1585784935172,
27.2460860859821,27.3336014046745,27.4211451037779,27.508785749695,27.5964839586264,
27.6843077859491,27.7076078480968,27.7974230785268,27.8871096033914,27.9766848889006,
28.0661443689486,28.1555356974574,28.2448677619689,28.2743338823081),
 .UNSPECIFIED.);
#2090=B_SPLINE_CURVE_WITH_KNOTS('',3,(#31963,#31964,#31965,#31966,#31967,
#31968,#31969,#31970,#31971,#31972,#31973,#31974,#31975,#31976,#31977,#31978,
#31979,#31980,#31981,#31982,#31983,#31984,#31985,#31986,#31987,#31988,#31989,
#31990,#31991,#31992,#31993,#31994,#31995,#31996,#31997,#31998,#31999,#32000,
#32001,#32002,#32003,#32004,#32005,#32006,#32007,#32008,#32009,#32010,#32011,
#32012,#32013,#32014,#32015,#32016,#32017,#32018,#32019,#32020,#32021,#32022,
#32023,#32024,#32025,#32026,#32027,#32028,#32029,#32030,#32031,#32032,#32033,
#32034,#32035,#32036,#32037,#32038,#32039,#32040,#32041,#32042,#32043,#32044),
 .UNSPECIFIED.,.F.,.F.,(4,3,3,3,3,3,3,3,3,3,3,3,3,3,3,3,3,3,3,3,3,3,3,3,
3,3,3,4),(28.2743338824685,28.3691609663371,28.4643913168018,28.5598306393145,
28.6555712304409,28.6982372246769,28.7860549589011,28.8737618981413,28.9613810423672,
29.0523167372284,29.1398372605426,29.2273448561933,29.3148601778887,29.4024038798072,
29.4900445282464,29.5777427395317,29.6655665689418,29.6888666012569,29.7766954664404,
29.8670063833447,29.9546150704636,30.0421656067926,30.1296786939772,30.2171750011152,
30.3047012558658,30.3922463191219,30.4798600883877,30.4991828016751),
 .UNSPECIFIED.);
#2091=B_SPLINE_CURVE_WITH_KNOTS('',3,(#32046,#32047,#32048,#32049,#32050,
#32051,#32052,#32053,#32054,#32055,#32056,#32057,#32058,#32059,#32060,#32061,
#32062,#32063,#32064,#32065,#32066,#32067,#32068,#32069,#32070,#32071,#32072,
#32073,#32074,#32075,#32076,#32077,#32078,#32079,#32080,#32081,#32082,#32083,
#32084,#32085,#32086,#32087,#32088,#32089,#32090,#32091,#32092,#32093,#32094,
#32095,#32096,#32097,#32098,#32099,#32100,#32101,#32102,#32103,#32104,#32105,
#32106,#32107,#32108,#32109,#32110,#32111,#32112,#32113,#32114,#32115,#32116,
#32117,#32118,#32119,#32120,#32121,#32122,#32123,#32124,#32125,#32126,#32127),
 .UNSPECIFIED.,.F.,.F.,(4,3,3,3,3,3,3,3,3,3,3,3,3,3,3,3,3,3,3,3,3,3,3,3,
3,3,3,4),(28.2743338824878,28.3620520321736,28.4496594841827,28.5371793599059,
28.6273527268449,28.7147750521331,28.8021848299805,28.8896028228172,28.9770497939646,
29.0645937581805,29.1521960284464,29.2399225699005,29.2585662954179,29.3463840254717,
29.4340909607114,29.5217101011108,29.6126457974717,29.7001663174231,29.7876739098888,
29.8751892285822,29.9627329276854,30.0503735736029,30.1380717825348,30.2258956098576,
30.249195671998,30.3370125832184,30.4247057976887,30.5003021062259),
 .UNSPECIFIED.);
#2092=B_SPLINE_CURVE_WITH_KNOTS('',3,(#32128,#32129,#32130,#32131,#32132,
#32133,#32134,#32135,#32136,#32137,#32138,#32139,#32140,#32141,#32142,#32143,
#32144,#32145,#32146,#32147,#32148,#32149,#32150,#32151,#32152,#32153,#32154,
#32155,#32156,#32157,#32158,#32159,#32160,#32161,#32162,#32163,#32164,#32165,
#32166,#32167,#32168,#32169,#32170,#32171,#32172,#32173,#32174,#32175,#32176,
#32177,#32178,#32179,#32180,#32181,#32182,#32183,#32184,#32185,#32186,#32187,
#32188,#32189,#32190,#32191,#32192,#32193,#32194,#32195,#32196,#32197,#32198,
#32199,#32200,#32201,#32202,#32203,#32204,#32205,#32206,#32207,#32208,#32209,
#32210,#32211,#32212,#32213,#32214,#32215,#32216,#32217,#32218,#32219,#32220,
#32221,#32222,#32223,#32224,#32225,#32226,#32227,#32228,#32229,#32230,#32231,
#32232,#32233,#32234,#32235,#32236,#32237,#32238,#32239,#32240,#32241,#32242,
#32243,#32244,#32245,#32246,#32247,#32248,#32249,#32250,#32251,#32252,#32253,
#32254,#32255,#32256,#32257,#32258,#32259,#32260,#32261,#32262,#32263,#32264,
#32265,#32266,#32267,#32268,#32269,#32270,#32271,#32272,#32273,#32274,#32275,
#32276,#32277,#32278),.UNSPECIFIED.,.F.,.F.,(4,3,3,3,3,3,3,3,3,3,3,3,3,
3,3,3,3,3,3,3,3,3,3,3,3,3,3,3,3,3,3,3,3,3,3,3,3,3,3,3,3,3,3,3,3,3,3,3,3,
3,4),(24.2161615786844,24.3054194125178,24.393235614427,24.4809409996466,
24.5685585701688,24.6594948475349,24.7470137580256,24.8345197291811,24.922033416444,
25.0095754757204,25.0972144775499,25.1849110379788,25.2727332228469,25.2960487890978,
25.3838670018774,25.4715744238134,25.5591940542576,25.6501295681851,25.7376505833635,
25.8251586721042,25.9126744875772,26.0002186834226,26.0878598235176,26.1755585257106,
26.2633828411844,26.2866781656779,26.3744960037511,26.4622030498209,26.5498223037114,
26.6407579585298,26.7282785979179,26.8157863118169,26.9033017538155,26.9908455779736,
27.0784863509278,27.1661846882012,27.2540086448129,27.2773075422579,27.3651250796296,
27.4528318191191,27.5404507609564,27.6313865306916,27.7189068463188,27.8064142326825,
27.8939293437142,27.9814728338144,28.0691132697803,28.1568112679608,28.2446348849586,
28.2679369188379,28.2743338823081),.UNSPECIFIED.);
#2093=B_SPLINE_CURVE_WITH_KNOTS('',3,(#32284,#32285,#32286,#32287,#32288,
#32289,#32290,#32291,#32292,#32293,#32294,#32295,#32296,#32297,#32298,#32299,
#32300,#32301,#32302,#32303,#32304,#32305,#32306,#32307,#32308,#32309,#32310,
#32311,#32312,#32313,#32314,#32315,#32316,#32317,#32318,#32319,#32320,#32321,
#32322,#32323,#32324,#32325,#32326,#32327,#32328,#32329,#32330,#32331,#32332,
#32333,#32334,#32335,#32336,#32337,#32338,#32339,#32340,#32341,#32342,#32343,
#32344,#32345,#32346,#32347,#32348,#32349,#32350,#32351,#32352,#32353,#32354,
#32355,#32356,#32357,#32358,#32359,#32360,#32361,#32362,#32363,#32364,#32365),
 .UNSPECIFIED.,.F.,.F.,(4,3,3,3,3,3,3,3,3,3,3,3,3,3,3,3,3,3,3,3,3,3,3,3,
3,3,3,4),(15.7079632679489,15.7946703424306,15.8813545315613,15.9680372193346,
16.0547397844141,16.1415388412398,16.228388975724,16.3153822983035,16.3803843998776,
16.4682786364247,16.5560616599551,16.6437563744183,16.7346635496732,16.8222578350669,
16.9098383863582,16.9974257698594,17.0850405516535,17.1727504498517,17.260516922345,
17.3484070344364,17.3710137764576,17.4589624375309,17.5468079926991,17.6345711086995,
17.7222690062869,17.8099291514913,17.897581481792,17.933138501431),
 .UNSPECIFIED.);
#2094=B_SPLINE_CURVE_WITH_KNOTS('',3,(#32367,#32368,#32369,#32370,#32371),
 .UNSPECIFIED.,.F.,.F.,(4,1,4),(14.3991256467175,15.3897550232976,15.7079550219993),
 .UNSPECIFIED.);
#2095=B_SPLINE_CURVE_WITH_KNOTS('',3,(#32375,#32376,#32377,#32378,#32379,
#32380,#32381,#32382,#32383,#32384,#32385,#32386,#32387,#32388,#32389,#32390,
#32391,#32392,#32393,#32394,#32395,#32396,#32397,#32398,#32399,#32400,#32401,
#32402,#32403,#32404,#32405,#32406,#32407,#32408,#32409,#32410,#32411,#32412,
#32413,#32414,#32415,#32416,#32417,#32418,#32419,#32420,#32421,#32422,#32423,
#32424,#32425,#32426,#32427,#32428,#32429,#32430,#32431,#32432,#32433,#32434,
#32435,#32436,#32437,#32438),.UNSPECIFIED.,.F.,.F.,(4,3,3,3,3,3,3,3,3,3,
3,3,3,3,3,3,3,3,3,3,3,4),(13.8752087529905,13.9625599527458,14.049801399386,
14.1369566191565,14.2240510610285,14.3111134548194,14.3981649381222,14.4852266357263,
14.5723733096138,14.6595621693105,14.7468902564328,14.8294259525565,14.9162044260086,
15.0028750623154,15.091011087993,15.1775387385182,15.2640376415103,15.3505294215583,
15.4398878831029,15.5264717366794,15.617217502208,15.7079632677367),
 .UNSPECIFIED.);
#2096=B_SPLINE_CURVE_WITH_KNOTS('',3,(#32439,#32440,#32441,#32442,#32443,
#32444,#32445,#32446,#32447,#32448,#32449,#32450,#32451,#32452,#32453,#32454,
#32455,#32456,#32457,#32458,#32459,#32460,#32461,#32462,#32463,#32464,#32465,
#32466,#32467,#32468,#32469,#32470,#32471,#32472,#32473,#32474,#32475,#32476,
#32477,#32478,#32479,#32480,#32481,#32482,#32483,#32484,#32485,#32486,#32487,
#32488,#32489,#32490,#32491,#32492,#32493,#32494,#32495,#32496,#32497,#32498,
#32499,#32500,#32501,#32502,#32503,#32504,#32505,#32506,#32507,#32508,#32509,
#32510,#32511,#32512,#32513,#32514,#32515,#32516,#32517,#32518,#32519,#32520),
 .UNSPECIFIED.,.F.,.F.,(4,3,3,3,3,3,3,3,3,3,3,3,3,3,3,3,3,3,3,3,3,3,3,3,
3,3,3,4),(15.7079632679489,15.8200553291365,15.9077801590785,15.9953930214419,
16.0829170361697,16.173887994863,16.2613113585393,16.3487212103233,16.4361383070159,
16.5235834056171,16.6111253805921,16.6987247599939,16.7864502769504,16.8106847057165,
16.8985189148338,16.9862423685142,17.0738780459568,17.1648075504993,17.2523445445389,
17.3398685584644,17.4274002275394,17.5149601874335,17.602616878146,17.6903310246347,
17.7781705099498,17.8013140822966,17.8891423087798,17.9338728552279),
 .UNSPECIFIED.);
#2097=B_SPLINE_CURVE_WITH_KNOTS('',3,(#32526,#32527,#32528,#32529,#32530,
#32531,#32532,#32533,#32534,#32535,#32536,#32537,#32538,#32539,#32540,#32541,
#32542,#32543,#32544,#32545,#32546,#32547,#32548,#32549,#32550,#32551,#32552,
#32553,#32554,#32555,#32556,#32557,#32558,#32559,#32560,#32561,#32562,#32563,
#32564,#32565,#32566,#32567,#32568,#32569,#32570,#32571,#32572,#32573,#32574,
#32575,#32576,#32577,#32578,#32579,#32580,#32581,#32582,#32583,#32584,#32585,
#32586,#32587,#32588,#32589,#32590,#32591,#32592,#32593,#32594,#32595,#32596,
#32597,#32598,#32599,#32600,#32601,#32602,#32603,#32604,#32605,#32606,#32607,
#32608,#32609,#32610,#32611,#32612,#32613,#32614,#32615,#32616,#32617,#32618,
#32619,#32620,#32621,#32622),.UNSPECIFIED.,.F.,.F.,(4,3,3,3,3,3,3,3,3,3,
3,3,3,3,3,3,3,3,3,3,3,3,3,3,3,3,3,3,3,3,3,3,4),(64.4958654271813,64.5878114726323,
64.6796682202886,64.7714666576999,64.8632356888753,64.9549989780416,65.0467801784818,
65.1386594553566,65.2305917565556,65.3226705696143,65.3815388542818,65.4726940042981,
65.5637278110629,65.6546677268432,65.7455466697704,65.8363944318674,65.9272356637036,
66.0180950050278,66.1090616969139,66.200083004819,66.2912717783792,66.3721682308618,
66.4666155697857,66.5609252154487,66.6551188983848,66.7492022645659,66.8432212250325,
66.9371952485092,67.0311437590025,67.1251117412093,67.2190879270455,67.3131274215545,
67.3627976074418),.UNSPECIFIED.);
#2098=B_SPLINE_CURVE_WITH_KNOTS('',3,(#32630,#32631,#32632,#32633,#32634,
#32635,#32636,#32637,#32638,#32639,#32640,#32641,#32642,#32643,#32644,#32645,
#32646,#32647,#32648,#32649,#32650,#32651,#32652,#32653,#32654,#32655,#32656,
#32657,#32658,#32659,#32660,#32661,#32662,#32663,#32664,#32665,#32666,#32667,
#32668,#32669,#32670,#32671,#32672,#32673,#32674,#32675,#32676,#32677,#32678,
#32679,#32680,#32681,#32682,#32683,#32684,#32685,#32686,#32687,#32688,#32689,
#32690,#32691,#32692,#32693,#32694,#32695,#32696,#32697,#32698,#32699,#32700,
#32701,#32702,#32703,#32704,#32705,#32706,#32707,#32708,#32709,#32710,#32711,
#32712,#32713,#32714,#32715,#32716,#32717,#32718,#32719,#32720,#32721,#32722,
#32723,#32724,#32725,#32726,#32727,#32728,#32729,#32730,#32731,#32732,#32733,
#32734,#32735,#32736,#32737,#32738,#32739,#32740,#32741,#32742,#32743,#32744,
#32745,#32746,#32747,#32748,#32749,#32750,#32751,#32752,#32753,#32754,#32755,
#32756,#32757,#32758,#32759,#32760,#32761,#32762,#32763,#32764,#32765,#32766,
#32767),.UNSPECIFIED.,.F.,.F.,(4,2,2,2,2,2,2,2,2,2,2,2,2,2,2,2,2,2,2,2,
2,2,2,2,2,2,2,2,2,2,2,2,2,2,2,2,2,2,2,2,2,2,2,2,2,2,2,2,2,2,2,2,2,2,2,2,
2,2,2,2,2,2,2,2,2,2,2,2,4),(-3.81646514822443,-3.80352815874458,-3.74055056205899,
-3.6908910055397,-3.67160982941172,-3.66182442746867,-3.65456573177332,
-3.64537017487538,-3.62953057477486,-3.57391740471288,-3.52733622427903,
-3.50426956775655,-3.49698761023047,-3.49221053925842,-3.48787708604674,
-3.48025265988004,-3.45518881362056,-3.39537599510592,-3.36309191692142,
-3.34055429809831,-3.33024160712699,-3.32222124734079,-3.31323481495827,
-3.29778023865283,-3.22209772637379,-3.18651335334593,-3.16664977008392,
-3.15980085945556,-3.15517806771929,-3.15023395777695,-3.1417623667696,
-3.09904416338619,-3.03933890749073,-3.00684096618422,-2.99520428269995,
-2.98705224957573,-2.97968775404413,-2.9678900560391,-2.93669357636674,
-2.86010100596757,-2.84058945054392,-2.82727147287481,-2.82139621045025,
-2.81696558366223,-2.81154234728002,-2.80082238375559,-2.74751669952281,
-2.69817545346558,-2.66873737097169,-2.65742225990942,-2.64927841175236,
-2.64075547667854,-2.62746323568623,-2.57899698750133,-2.52042991410282,
-2.49457147695174,-2.48710482355436,-2.48235212473586,-2.47755031232083,
-2.46982254882778,-2.44342430688665,-2.37789105680805,-2.33561274883014,
-2.32299363831771,-2.31461541659801,-2.30649326662958,-2.29664195739933,
-2.27196551483348,-2.25634167253437),.UNSPECIFIED.);
#2099=B_SPLINE_CURVE_WITH_KNOTS('',3,(#32773,#32774,#32775,#32776,#32777,
#32778,#32779,#32780,#32781,#32782,#32783,#32784,#32785,#32786,#32787,#32788,
#32789,#32790,#32791,#32792,#32793,#32794,#32795,#32796,#32797,#32798,#32799,
#32800,#32801,#32802,#32803,#32804,#32805,#32806,#32807,#32808,#32809,#32810,
#32811,#32812,#32813,#32814,#32815,#32816,#32817,#32818,#32819,#32820,#32821,
#32822,#32823,#32824,#32825,#32826,#32827,#32828,#32829,#32830,#32831,#32832,
#32833,#32834,#32835,#32836,#32837,#32838,#32839,#32840,#32841,#32842,#32843,
#32844,#32845,#32846,#32847,#32848,#32849,#32850,#32851,#32852,#32853,#32854,
#32855,#32856,#32857,#32858,#32859,#32860,#32861,#32862,#32863,#32864,#32865,
#32866,#32867,#32868,#32869,#32870,#32871,#32872,#32873,#32874,#32875,#32876,
#32877,#32878,#32879,#32880,#32881,#32882,#32883,#32884,#32885,#32886,#32887,
#32888,#32889,#32890,#32891,#32892,#32893,#32894,#32895,#32896,#32897,#32898,
#32899,#32900,#32901,#32902,#32903,#32904,#32905,#32906,#32907,#32908,#32909,
#32910,#32911,#32912,#32913,#32914,#32915,#32916,#32917,#32918,#32919,#32920,
#32921,#32922,#32923,#32924,#32925,#32926,#32927,#32928,#32929,#32930,#32931,
#32932,#32933,#32934,#32935,#32936,#32937,#32938,#32939,#32940,#32941,#32942,
#32943,#32944,#32945,#32946,#32947,#32948,#32949,#32950,#32951,#32952),
 .UNSPECIFIED.,.F.,.F.,(4,2,2,2,2,2,2,2,2,2,2,2,2,2,2,2,2,2,2,2,2,2,2,2,
2,2,2,2,2,2,2,2,2,2,2,2,2,2,2,2,2,2,2,2,2,2,2,2,2,2,2,2,2,2,2,2,2,2,2,2,
2,2,2,2,2,2,2,2,2,2,2,2,2,2,2,2,2,2,2,2,2,2,2,2,2,2,2,2,2,4),(-2.0152369081143,
-1.97116093935254,-1.94753091842145,-1.94007625758421,-1.93580516021273,
-1.93112989406986,-1.92399263265513,-1.90146055648256,-1.85703316133956,
-1.79531564131364,-1.77939599561947,-1.77025411929421,-1.76230369882244,
-1.75236221422394,-1.73180134000087,-1.70350427661139,-1.63795986816285,
-1.61155643991754,-1.60384784489885,-1.59905375859423,-1.59432123444,-1.58688781614374,
-1.56121123397106,-1.50359636533397,-1.45351941985236,-1.4401843381907,
-1.43166916120953,-1.42355885213667,-1.41233493704493,-1.38344051228533,
-1.33561744850789,-1.2800359484559,-1.2695959769893,-1.26416635707667,-1.25967788516117,
-1.25374660794778,-1.2402335856419,-1.22034290657674,-1.13923059349499,
-1.11220447488099,-1.10097379473918,-1.09285550331387,-1.08432887637475,
-1.07096819851719,-1.01584699984061,-0.959944641081289,-0.937610543838119,
-0.930280989868928,-0.926030573676456,-0.92131532273394,-0.914023034669241,
-0.890052052828789,-0.840042899972904,-0.786122648137173,-0.770164885024668,
-0.761006059984599,-0.753042549073807,-0.74308594691075,-0.722494924734582,
-0.694157093842313,-0.628436109119681,-0.602158900285102,-0.594468386963779,
-0.589677894380495,-0.584971859334526,-0.577579010137999,-0.55206638376495,
-0.495245912786879,-0.443731306813558,-0.430386365139749,-0.421899033029062,
-0.413841244311261,-0.402735400359603,-0.374467917606038,-0.32834286763478,
-0.270175548509306,-0.259654219484075,-0.254286783417145,-0.249794225459742,
-0.243797336648389,-0.229943113817842,-0.209358714925704,-0.130315938037314,
-0.102350790602122,-0.0909273173276217,-0.082827828262194,-0.0743211133442966,
-0.0656697704768997,-0.0531761502260062,-0.00100806979219698),
 .UNSPECIFIED.);
#2100=B_SPLINE_CURVE_WITH_KNOTS('',3,(#32953,#32954,#32955,#32956,#32957,
#32958,#32959,#32960,#32961,#32962,#32963,#32964,#32965,#32966,#32967,#32968),
 .UNSPECIFIED.,.F.,.F.,(4,3,3,3,3,4),(64.1406906932474,64.2573851651463,
64.3763858948088,64.3909094777018,64.482998908666,64.4958654271813),
 .UNSPECIFIED.);
#2101=B_SPLINE_CURVE_WITH_KNOTS('',3,(#32969,#32970,#32971,#32972,#32973,
#32974,#32975,#32976,#32977,#32978,#32979,#32980,#32981,#32982,#32983,#32984,
#32985,#32986,#32987,#32988,#32989,#32990,#32991,#32992,#32993,#32994,#32995,
#32996,#32997,#32998,#32999,#33000,#33001,#33002,#33003,#33004,#33005,#33006,
#33007,#33008,#33009,#33010,#33011,#33012,#33013,#33014,#33015,#33016,#33017,
#33018,#33019,#33020,#33021,#33022,#33023,#33024,#33025,#33026,#33027,#33028,
#33029,#33030,#33031,#33032,#33033,#33034,#33035,#33036,#33037,#33038,#33039,
#33040,#33041,#33042,#33043,#33044,#33045,#33046,#33047,#33048,#33049,#33050,
#33051,#33052,#33053,#33054,#33055,#33056,#33057,#33058,#33059,#33060,#33061,
#33062,#33063,#33064,#33065,#33066,#33067,#33068,#33069,#33070,#33071,#33072,
#33073,#33074,#33075,#33076,#33077,#33078,#33079,#33080,#33081,#33082,#33083,
#33084,#33085,#33086,#33087,#33088,#33089,#33090,#33091,#33092,#33093,#33094,
#33095,#33096,#33097,#33098,#33099,#33100,#33101,#33102,#33103,#33104,#33105,
#33106,#33107,#33108,#33109,#33110,#33111,#33112,#33113,#33114,#33115,#33116,
#33117,#33118,#33119,#33120,#33121,#33122,#33123,#33124,#33125,#33126,#33127,
#33128,#33129,#33130,#33131,#33132,#33133,#33134,#33135,#33136,#33137,#33138,
#33139,#33140,#33141,#33142,#33143,#33144,#33145,#33146,#33147,#33148,#33149,
#33150,#33151,#33152,#33153,#33154,#33155,#33156,#33157,#33158,#33159,#33160),
 .UNSPECIFIED.,.F.,.F.,(4,2,2,2,2,2,2,2,2,2,2,2,2,2,2,2,2,2,2,2,2,2,2,2,
2,2,2,2,2,2,2,2,2,2,2,2,2,2,2,2,2,2,2,2,2,2,2,2,2,2,2,2,2,2,2,2,2,2,2,2,
2,2,2,2,2,2,2,2,2,2,2,2,2,2,2,2,2,2,2,2,2,2,2,2,2,2,2,2,2,2,2,2,2,2,2,4),
(-2.25634167253437,-2.1881420344393,-2.168049575673,-2.15443780714628,-2.14848912535191,
-2.14399843087398,-2.13857965438789,-2.1278681277045,-2.07562952988243,
-2.02559161652123,-1.99594302048512,-1.98461882665343,-1.97649022553089,
-1.96800342456545,-1.95481309853747,-1.90846483912855,-1.89825580196821,
-1.8406412797465,-1.82044982449514,-1.81337296613433,-1.8091737887011,-1.80441908458761,
-1.79689650610624,-1.77023834151946,-1.70756403287971,-1.66318085017836,
-1.65010005426361,-1.64162975442101,-1.63347794624088,-1.62205532028647,
-1.59167987103848,-1.51168740437092,-1.4851849960617,-1.47745602659865,
-1.47265573711118,-1.46792043575924,-1.46049050806918,-1.43491065187996,
-1.37778351626714,-1.32717028643306,-1.31381420923002,-1.30528918918205,
-1.29717168323605,-1.28594095701279,-1.25704474645925,-1.2092365884578,
-1.15360020172603,-1.14315697578276,-1.13772406855693,-1.13323346151996,
-1.12729891705099,-1.11376971895252,-1.09384515720563,-1.01225908311068,
-0.985657119725443,-0.97450007176338,-0.966395847790362,-0.957849093610993,
-0.944382161237028,-0.886282830960741,-0.825168733458591,-0.809251393647724,
-0.802779764037206,-0.798225573719969,-0.793110374492047,-0.78390122175292,
-0.77207225341405,-0.743743823259087,-0.658682421702079,-0.642964108802933,
-0.633866118567348,-0.62598815048635,-0.616026594938854,-0.595347393056453,
-0.5668176888279,-0.526448952506956,-0.476958390382105,-0.468383587220673,
-0.463403023196974,-0.458793320209024,-0.451992976380947,-0.432442005601048,
-0.397712976123245,-0.320904985965978,-0.305683162035318,-0.296774785984468,
-0.288791398065986,-0.278482337522529,-0.255776856562214,-0.223129826757771,
-0.16177743509034,-0.138221073863547,-0.130773566383219,-0.126504039896551,
-0.121829508555764,-0.121375378727905),.UNSPECIFIED.);
#2102=B_SPLINE_CURVE_WITH_KNOTS('',3,(#33165,#33166,#33167,#33168,#33169,
#33170,#33171,#33172,#33173,#33174,#33175,#33176,#33177,#33178,#33179,#33180,
#33181,#33182,#33183,#33184,#33185,#33186,#33187,#33188,#33189,#33190,#33191,
#33192,#33193,#33194,#33195,#33196,#33197,#33198,#33199,#33200,#33201,#33202,
#33203,#33204,#33205,#33206,#33207,#33208,#33209,#33210,#33211,#33212,#33213,
#33214,#33215,#33216,#33217,#33218,#33219,#33220,#33221,#33222,#33223,#33224,
#33225,#33226,#33227,#33228,#33229,#33230,#33231,#33232,#33233,#33234,#33235,
#33236,#33237,#33238,#33239,#33240,#33241,#33242,#33243,#33244,#33245,#33246,
#33247,#33248,#33249,#33250,#33251,#33252,#33253,#33254,#33255,#33256,#33257,
#33258,#33259,#33260,#33261,#33262,#33263,#33264,#33265,#33266,#33267,#33268,
#33269,#33270,#33271,#33272,#33273,#33274,#33275,#33276,#33277,#33278,#33279,
#33280,#33281,#33282,#33283,#33284,#33285,#33286,#33287,#33288,#33289,#33290,
#33291,#33292,#33293,#33294,#33295,#33296,#33297,#33298,#33299,#33300,#33301,
#33302,#33303,#33304,#33305,#33306,#33307,#33308,#33309,#33310,#33311,#33312,
#33313,#33314,#33315,#33316,#33317,#33318,#33319,#33320,#33321,#33322,#33323,
#33324,#33325,#33326,#33327,#33328,#33329,#33330,#33331,#33332,#33333,#33334,
#33335,#33336,#33337,#33338,#33339,#33340,#33341,#33342,#33343,#33344,#33345,
#33346,#33347,#33348,#33349,#33350,#33351,#33352),.UNSPECIFIED.,.F.,.F.,
(4,2,2,2,2,2,2,2,2,2,2,2,2,2,2,2,2,2,2,2,2,2,2,2,2,2,2,2,2,2,2,2,2,2,2,
2,2,2,2,2,2,2,2,2,2,2,2,2,2,2,2,2,2,2,2,2,2,2,2,2,2,2,2,2,2,2,2,2,2,2,2,
2,2,2,2,2,2,2,2,2,2,2,2,2,2,2,2,2,2,2,2,2,2,4),(-4.14975517296478,-4.13455580645905,
-4.12556746444321,-4.11760059569648,-4.10743503864127,-4.08557563722847,
-3.99748878645955,-3.97711222049083,-3.96336669675091,-3.95739663488861,
-3.95290411702709,-3.94749941603641,-3.93686532659078,-3.88059503089609,
-3.83328555535685,-3.80456852375864,-3.79336379782498,-3.7852526376491,
-3.77672322487416,-3.76333652335401,-3.71114023639411,-3.6554136412058,
-3.63013529370559,-3.62273467647168,-3.61800690547128,-3.61378676931684,
-3.6066006522728,-3.58551993804436,-3.52860828680488,-3.47287461898424,
-3.45949144678285,-3.45096297484923,-3.44285184213696,-3.43164571717561,
-3.4047296050034,-3.3256044775181,-3.30454586333963,-3.29047843660382,-3.28445526310384,
-3.27995829565801,-3.27459140202592,-3.26445852073142,-3.18899221391022,
-3.15366979070076,-3.12973423087392,-3.11922683391053,-3.11122072388365,
-3.10241733510474,-3.08769953292715,-3.00713677151403,-2.9592361420963,
-2.95069446403207,-2.94572163867358,-2.94116251510814,-2.93547991723627,
-2.92097098527908,-2.85870140447019,-2.79996955020488,-2.7864838334342,
-2.77793401815398,-2.76983299011081,-2.75869010586304,-2.73218762975779,
-2.65056516586576,-2.63064755019404,-2.61712164255023,-2.61118836144776,
-2.60669880272143,-2.60126746436783,-2.59049618255,-2.54583656858252,-2.50760199607605,
-2.47720377496632,-2.45558779147849,-2.4454639032615,-2.43750120172481,
-2.42848761357944,-2.41315551316623,-2.33897810795571,-2.28628831249504,
-2.27767187816894,-2.27268312163263,-2.26813184656009,-2.26140143449232,
-2.24380539206789,-2.18408900143524,-2.1358713255419,-2.11914928345012,
-2.10897547445082,-2.10100681350048,-2.09202135067769,-2.0764219268981,
-2.02612709481119,-2.0152369081143),.UNSPECIFIED.);
#2103=B_SPLINE_CURVE_WITH_KNOTS('',3,(#33354,#33355,#33356,#33357,#33358,
#33359,#33360,#33361),.UNSPECIFIED.,.F.,.F.,(4,2,2,4),(-0.121375378727905,
-0.114690093556633,-0.0921226174557673,-0.000975323762489068),
 .UNSPECIFIED.);
#2104=B_SPLINE_CURVE_WITH_KNOTS('',3,(#33362,#33363,#33364,#33365,#33366,
#33367,#33368,#33369,#33370,#33371,#33372,#33373,#33374,#33375,#33376,#33377,
#33378,#33379,#33380,#33381,#33382,#33383,#33384,#33385,#33386,#33387,#33388,
#33389,#33390,#33391,#33392,#33393,#33394,#33395,#33396,#33397,#33398,#33399,
#33400,#33401,#33402,#33403,#33404,#33405,#33406,#33407,#33408,#33409,#33410,
#33411,#33412,#33413,#33414,#33415,#33416,#33417,#33418,#33419,#33420,#33421,
#33422,#33423,#33424,#33425,#33426,#33427,#33428,#33429,#33430,#33431,#33432,
#33433,#33434,#33435,#33436,#33437,#33438,#33439,#33440,#33441,#33442,#33443,
#33444,#33445,#33446,#33447,#33448,#33449,#33450,#33451,#33452,#33453,#33454,
#33455,#33456,#33457,#33458,#33459,#33460,#33461,#33462,#33463,#33464,#33465,
#33466,#33467,#33468,#33469,#33470,#33471,#33472,#33473,#33474,#33475,#33476,
#33477,#33478,#33479,#33480,#33481,#33482,#33483,#33484,#33485,#33486,#33487,
#33488,#33489,#33490,#33491,#33492,#33493,#33494,#33495,#33496,#33497,#33498,
#33499,#33500,#33501,#33502,#33503,#33504,#33505,#33506,#33507,#33508,#33509,
#33510,#33511,#33512,#33513,#33514,#33515,#33516,#33517,#33518,#33519,#33520,
#33521,#33522,#33523,#33524,#33525,#33526,#33527,#33528,#33529,#33530,#33531,
#33532,#33533,#33534,#33535,#33536,#33537,#33538,#33539),.UNSPECIFIED.,
 .F.,.F.,(4,2,2,2,2,2,2,2,2,2,2,2,2,2,2,2,2,2,2,2,2,2,2,2,2,2,2,2,2,2,2,
2,2,2,2,2,2,2,2,2,2,2,2,2,2,2,2,2,2,2,2,2,2,2,2,2,2,2,2,2,2,2,2,2,2,2,2,
2,2,2,2,2,2,2,2,2,2,2,2,2,2,2,2,2,2,2,2,2,4),(-4.27125438342981,-4.25501503648509,
-4.24260511705344,-4.23465441741718,-4.22709219941081,-4.21860334803321,
-4.20542534814838,-4.15740314793215,-4.09923643068426,-4.07206829635785,
-4.06450393322421,-4.05974027376557,-4.05497257873807,-4.04738941569824,
-4.02234537977007,-3.96228631289094,-3.91372246976973,-3.90067833068308,
-3.89221664485113,-3.88415466816843,-3.8727770921359,-3.84489478392995,
-3.7649527655659,-3.74516285058777,-3.73169712707356,-3.72577274294145,
-3.72128221104,-3.71584007187348,-3.70502115078077,-3.65964884495702,-3.61991933351525,
-3.57638523703159,-3.56367201746124,-3.55527675665466,-3.54717128623843,
-3.53738109235133,-3.51308591487986,-3.42884257392313,-3.40872384254713,
-3.39509979276722,-3.38914856092271,-3.38465589053771,-3.37923346272373,
-3.36851601051705,-3.32501628043338,-3.28770273394464,-3.25601417416582,
-3.23376567816179,-3.22353092260851,-3.21555361718432,-3.20659896962883,
-3.19115987088382,-3.11619463079249,-3.08046995413687,-3.06057975224822,
-3.05373739595098,-3.04911907461424,-3.04415168149525,-3.03564167781744,
-2.9908661521944,-2.91482699786847,-2.89552106398494,-2.88580792449511,
-2.87863983810974,-2.8696129527188,-2.85423082916165,-2.78046699105375,
-2.7274082730617,-2.71878458698864,-2.71379288662701,-2.7092400356556,-2.70250860873931,
-2.6849169020748,-2.61766719826348,-2.56722834046539,-2.55407975898685,
-2.54559653088004,-2.53754623185693,-2.52623989463462,-2.49882076215399,
-2.41830902274939,-2.39847263128795,-2.38498422640902,-2.37905578439826,
-2.37456471207313,-2.36912503088202,-2.35865213340398,-2.30357121827838,
-2.25622471834554),.UNSPECIFIED.);
#2105=B_SPLINE_CURVE_WITH_KNOTS('',3,(#33545,#33546,#33547,#33548,#33549,
#33550,#33551,#33552,#33553,#33554,#33555,#33556,#33557,#33558,#33559,#33560,
#33561,#33562,#33563,#33564,#33565,#33566,#33567,#33568,#33569,#33570,#33571,
#33572,#33573,#33574,#33575,#33576,#33577,#33578,#33579,#33580,#33581,#33582,
#33583,#33584,#33585,#33586,#33587,#33588,#33589,#33590,#33591,#33592,#33593,
#33594,#33595,#33596,#33597,#33598,#33599,#33600,#33601,#33602,#33603,#33604,
#33605,#33606,#33607,#33608,#33609,#33610,#33611,#33612,#33613,#33614,#33615,
#33616,#33617,#33618,#33619,#33620,#33621,#33622,#33623,#33624,#33625,#33626,
#33627,#33628,#33629,#33630,#33631,#33632,#33633,#33634,#33635,#33636,#33637,
#33638,#33639,#33640,#33641,#33642,#33643,#33644,#33645,#33646,#33647,#33648,
#33649,#33650,#33651,#33652,#33653,#33654,#33655,#33656,#33657,#33658,#33659,
#33660,#33661,#33662,#33663,#33664,#33665,#33666,#33667,#33668,#33669,#33670,
#33671,#33672,#33673,#33674,#33675,#33676,#33677,#33678,#33679,#33680,#33681,
#33682,#33683,#33684,#33685,#33686,#33687,#33688,#33689,#33690,#33691,#33692,
#33693,#33694,#33695,#33696,#33697,#33698,#33699,#33700,#33701,#33702,#33703,
#33704,#33705,#33706,#33707,#33708,#33709,#33710,#33711,#33712,#33713,#33714,
#33715,#33716,#33717,#33718,#33719,#33720,#33721,#33722),.UNSPECIFIED.,
 .F.,.F.,(4,2,2,2,2,2,2,2,2,2,2,2,2,2,2,2,2,2,2,2,2,2,2,2,2,2,2,2,2,2,2,
2,2,2,2,2,2,2,2,2,2,2,2,2,2,2,2,2,2,2,2,2,2,2,2,2,2,2,2,2,2,2,2,2,2,2,2,
2,2,2,2,2,2,2,2,2,2,2,2,2,2,2,2,2,2,2,2,2,4),(-2.01521772153702,-1.98189085311168,
-1.90192497698326,-1.88553068491922,-1.87628868202977,-1.86834789004264,
-1.85854333615922,-1.838736961262,-1.81188688524793,-1.76967090638649,-1.71907053077995,
-1.71044459355391,-1.70545297332107,-1.7008483173261,-1.69407731971124,
-1.67476911418862,-1.64074638077149,-1.56260627468835,-1.54754614456766,
-1.53867045799165,-1.53067908408467,-1.52030667513674,-1.4972202789615,
-1.46376290481328,-1.39771405901254,-1.37901132537832,-1.37212511413708,
-1.36754516291517,-1.36260988022624,-1.35424621040038,-1.31287723514507,
-1.22731770615837,-1.21170187761505,-1.20262624485003,-1.19546625661394,
-1.18582495524724,-1.16689470595396,-1.1201291530442,-1.06178273901728,
-1.04255668617962,-1.03560095446714,-1.0310083758883,-1.02609650594405,
-1.01784021525856,-0.979217569618965,-0.891117769050643,-0.875281537132275,
-0.866159406749446,-0.858285873741104,-0.848363292283576,-0.827896276301347,
-0.752617947548739,-0.709000681849122,-0.700500487252411,-0.69553636561546,
-0.69091907495662,-0.684075273781897,-0.664160007638736,-0.628350626862018,
-0.553520026184348,-0.538248685217414,-0.529247523979435,-0.521281811057072,
-0.511134897410401,-0.489388178113713,-0.458728402328911,-0.444277199347154,
-0.381359106747041,-0.367591630640181,-0.36202819565,-0.357496954051565,
-0.352461575228102,-0.343626805114538,-0.332424032639677,-0.306467348974908,
-0.220414383883096,-0.204698632238166,-0.194807308056524,-0.186863593828534,
-0.177692822509181,-0.16117448170027,-0.14021024908188,-0.0645403267953068,
-0.0348516411336477,-0.0269078611245573,-0.0220637278553226,-0.0178656397223858,
-0.0131614481692901,-0.000969409447366421),.UNSPECIFIED.);
#2106=B_SPLINE_CURVE_WITH_KNOTS('',3,(#33723,#33724,#33725,#33726,#33727,
#33728,#33729,#33730),.UNSPECIFIED.,.F.,.F.,(4,2,2,4),(-4.27041062777532,
-4.20060841514599,-4.15017306640079,-4.14975517296478),.UNSPECIFIED.);
#2107=B_SPLINE_CURVE_WITH_KNOTS('',3,(#33731,#33732,#33733,#33734,#33735,
#33736,#33737,#33738,#33739,#33740,#33741,#33742,#33743,#33744,#33745,#33746,
#33747,#33748,#33749,#33750,#33751,#33752,#33753,#33754,#33755,#33756,#33757,
#33758,#33759,#33760,#33761,#33762,#33763,#33764,#33765,#33766,#33767,#33768,
#33769,#33770,#33771,#33772,#33773,#33774,#33775,#33776,#33777,#33778,#33779,
#33780,#33781,#33782,#33783,#33784,#33785,#33786,#33787,#33788,#33789,#33790,
#33791,#33792,#33793,#33794,#33795,#33796,#33797,#33798,#33799,#33800,#33801,
#33802,#33803,#33804,#33805,#33806,#33807,#33808,#33809,#33810,#33811,#33812,
#33813,#33814,#33815,#33816,#33817,#33818,#33819,#33820,#33821,#33822,#33823,
#33824,#33825,#33826,#33827,#33828,#33829,#33830,#33831,#33832,#33833,#33834,
#33835,#33836,#33837,#33838,#33839,#33840,#33841,#33842,#33843,#33844,#33845,
#33846,#33847,#33848,#33849,#33850,#33851,#33852,#33853,#33854,#33855,#33856,
#33857,#33858,#33859,#33860,#33861,#33862,#33863,#33864,#33865,#33866,#33867,
#33868,#33869,#33870,#33871,#33872,#33873,#33874,#33875,#33876,#33877,#33878,
#33879,#33880,#33881,#33882,#33883,#33884,#33885,#33886,#33887,#33888,#33889,
#33890,#33891,#33892,#33893,#33894,#33895,#33896,#33897,#33898,#33899,#33900,
#33901,#33902,#33903,#33904,#33905,#33906,#33907,#33908,#33909,#33910,#33911,
#33912,#33913,#33914,#33915,#33916,#33917,#33918,#33919,#33920,#33921,#33922),
 .UNSPECIFIED.,.F.,.F.,(4,2,2,2,2,2,2,2,2,2,2,2,2,2,2,2,2,2,2,2,2,2,2,2,
2,2,2,2,2,2,2,2,2,2,2,2,2,2,2,2,2,2,2,2,2,2,2,2,2,2,2,2,2,2,2,2,2,2,2,2,
2,2,2,2,2,2,2,2,2,2,2,2,2,2,2,2,2,2,2,2,2,2,2,2,2,2,2,2,2,2,2,2,2,2,2,4),
(-2.25622471834554,-2.25536552022434,-2.2263312213498,-2.21508125273909,
-2.20695984282477,-2.19843959820622,-2.18510984640676,-2.13543462955219,
-2.06954903287775,-2.0506677105141,-2.04375646235058,-2.03917118349923,
-2.03424269187976,-2.02591367806257,-1.98553135179024,-1.89823898096635,
-1.88279518260011,-1.87384010957296,-1.8658638278209,-1.85563232409652,
-1.83339864969124,-1.8017424399485,-1.76444015904065,-1.72095929769792,
-1.71024466643675,-1.70482314777365,-1.70033095952526,-1.69437991573311,
-1.68075482211882,-1.66063109265217,-1.57638798090588,-1.55206705678386,
-1.5422734746708,-1.53416791689761,-1.52577529122092,-1.51307147037056,
-1.46963808682529,-1.42987874954713,-1.38450816488483,-1.37369021161422,
-1.36824872106627,-1.36380174637027,-1.3579045354989,-1.34459559291259,
-1.32512609984941,-1.24902049537014,-1.21780106291181,-1.20596326157002,
-1.19782065680891,-1.18947759237621,-1.17702226000682,-1.13671198085963,
-1.09495253559571,-1.04786311567467,-1.03708992884157,-1.03165735441404,
-1.0271669086193,-1.02123237517546,-1.00770260449622,-0.987776380251331,
-0.90615254887284,-0.879595278557972,-0.868444245878143,-0.86034116349014,
-0.851792687214371,-0.838316633907228,-0.779904302837737,-0.718216134589707,
-0.703027116179809,-0.696639467277713,-0.692098004501017,-0.686943111476073,
-0.677542229674619,-0.626720905989134,-0.551878241313314,-0.536607702827611,
-0.527606601711726,-0.519640694239043,-0.509493193811317,-0.487743790768027,
-0.45707882617708,-0.442614713573513,-0.379658936821854,-0.365930164001574,
-0.360373089550245,-0.355798193213172,-0.350742414127901,-0.341811809955642,
-0.287605582224593,-0.215870373411604,-0.200310179304,-0.191247303456596,
-0.184087022954339,-0.174431897017359,-0.155423316492378,-0.121316291652191),
 .UNSPECIFIED.);
#2108=B_SPLINE_CURVE_WITH_KNOTS('',3,(#33927,#33928,#33929,#33930,#33931,
#33932,#33933,#33934,#33935,#33936,#33937,#33938,#33939,#33940,#33941,#33942,
#33943,#33944,#33945,#33946,#33947,#33948,#33949,#33950,#33951,#33952,#33953,
#33954,#33955,#33956,#33957,#33958,#33959,#33960,#33961,#33962,#33963,#33964,
#33965,#33966,#33967,#33968,#33969,#33970,#33971,#33972,#33973,#33974,#33975,
#33976,#33977,#33978,#33979,#33980,#33981,#33982,#33983,#33984,#33985,#33986,
#33987,#33988,#33989,#33990,#33991,#33992,#33993,#33994,#33995,#33996,#33997,
#33998,#33999,#34000,#34001,#34002,#34003,#34004,#34005,#34006,#34007,#34008,
#34009,#34010,#34011,#34012,#34013,#34014,#34015,#34016,#34017,#34018,#34019,
#34020,#34021,#34022,#34023,#34024,#34025,#34026,#34027,#34028,#34029,#34030,
#34031,#34032,#34033,#34034,#34035,#34036,#34037,#34038,#34039,#34040,#34041,
#34042,#34043,#34044,#34045,#34046,#34047,#34048,#34049,#34050,#34051,#34052,
#34053,#34054,#34055,#34056,#34057,#34058,#34059,#34060,#34061,#34062,#34063,
#34064,#34065,#34066,#34067,#34068,#34069,#34070,#34071,#34072,#34073,#34074,
#34075,#34076,#34077,#34078,#34079,#34080,#34081,#34082,#34083,#34084,#34085,
#34086,#34087,#34088,#34089,#34090,#34091,#34092,#34093,#34094,#34095,#34096,
#34097,#34098,#34099,#34100,#34101,#34102,#34103,#34104,#34105,#34106,#34107,
#34108,#34109,#34110,#34111,#34112,#34113,#34114,#34115,#34116),
 .UNSPECIFIED.,.F.,.F.,(4,2,2,2,2,2,2,2,2,2,2,2,2,2,2,2,2,2,2,2,2,2,2,2,
2,2,2,2,2,2,2,2,2,2,2,2,2,2,2,2,2,2,2,2,2,2,2,2,2,2,2,2,2,2,2,2,2,2,2,2,
2,2,2,2,2,2,2,2,2,2,2,2,2,2,2,2,2,2,2,2,2,2,2,2,2,2,2,2,2,2,2,2,2,2,4),
(-4.15039881543784,-4.11479463190062,-4.07497675799088,-4.06667127640619,
-4.06174828731719,-4.05716099185009,-4.0502361285809,-4.03124919218212,
-3.94184048425317,-3.92126782833572,-3.90498135058491,-3.89585576632678,
-3.88790537197335,-3.87794541119152,-3.85727461500573,-3.76753823808888,
-3.74705294636872,-3.73325477609339,-3.72727507837133,-3.72278084264605,
-3.71738084643567,-3.70709482045411,-3.63244252110455,-3.59675740841868,
-3.57265758734148,-3.56212247252427,-3.55411104617841,-3.54531736437953,
-3.53065379020532,-3.44965729922197,-3.40203535889951,-3.393497559649,-3.38852479200425,
-3.38396413034893,-3.37827791318012,-3.36375025005964,-3.30147516923983,
-3.25260141180522,-3.23351915224546,-3.22384857891598,-3.21668531871961,
-3.20762973691661,-3.19211032229828,-3.11987835296335,-3.06558246290022,
-3.05694859346522,-3.05195516559223,-3.04740408765511,-3.04068009896399,
-3.0231356547161,-2.96336771938735,-2.95040476509661,-2.91993745716488,
-2.89828531993084,-2.88815294038015,-2.88018689362551,-2.87117299847572,
-2.85584900336914,-2.78152778202518,-2.74544933135652,-2.72544237557882,
-2.71858671558012,-2.71396639039326,-2.70900463200773,-2.70051891299499,
-2.65843322432584,-2.59829384919797,-2.56565012929148,-2.55395607632598,
-2.54575744642759,-2.53834497438165,-2.52836151328386,-2.50246524163413,
-2.42014337336625,-2.40016819903877,-2.3866134437444,-2.38067423788575,
-2.37618287581889,-2.37075248957991,-2.36032231954279,-2.30435307992658,
-2.25671992832685,-2.22788576231526,-2.21666318913448,-2.20854714480596,
-2.20001973962504,-2.18665147938341,-2.13546424758547,-2.06359329968271,
-2.05000033540087,-2.04411768037304,-2.03962273002691,-2.0342258026487,
-2.02363614110582,-2.01521772153702),.UNSPECIFIED.);
#2109=B_SPLINE_CURVE_WITH_KNOTS('',3,(#34118,#34119,#34120,#34121,#34122,
#34123,#34124,#34125,#34126,#34127,#34128,#34129,#34130,#34131,#34132,#34133,
#34134,#34135),.UNSPECIFIED.,.F.,.F.,(4,2,2,2,2,2,2,2,4),(-0.121316291652191,
-0.107361750950517,-0.061796577017454,-0.0331257074193108,-0.0252540591814017,
-0.0204254665052418,-0.0162346899153542,-0.0115182785010899,-0.000969384353663965),
 .UNSPECIFIED.);
#2110=B_SPLINE_CURVE_WITH_KNOTS('',3,(#34136,#34137,#34138,#34139,#34140,
#34141,#34142,#34143,#34144,#34145,#34146,#34147,#34148,#34149,#34150,#34151,
#34152,#34153,#34154,#34155,#34156,#34157,#34158,#34159,#34160,#34161,#34162,
#34163,#34164,#34165,#34166,#34167,#34168,#34169,#34170,#34171,#34172,#34173,
#34174,#34175,#34176,#34177,#34178,#34179,#34180,#34181,#34182,#34183,#34184,
#34185,#34186,#34187,#34188,#34189,#34190,#34191,#34192,#34193,#34194,#34195,
#34196,#34197,#34198,#34199,#34200,#34201,#34202,#34203,#34204,#34205,#34206,
#34207,#34208,#34209,#34210,#34211,#34212,#34213,#34214,#34215,#34216,#34217,
#34218,#34219,#34220,#34221,#34222,#34223,#34224,#34225,#34226,#34227,#34228,
#34229,#34230,#34231,#34232,#34233,#34234,#34235,#34236,#34237,#34238,#34239,
#34240,#34241,#34242,#34243,#34244,#34245,#34246,#34247,#34248,#34249,#34250,
#34251,#34252,#34253,#34254,#34255,#34256,#34257,#34258,#34259,#34260,#34261,
#34262,#34263,#34264,#34265,#34266,#34267,#34268,#34269,#34270,#34271,#34272,
#34273,#34274,#34275,#34276,#34277,#34278,#34279,#34280,#34281,#34282,#34283,
#34284,#34285,#34286,#34287,#34288,#34289,#34290,#34291,#34292,#34293,#34294,
#34295,#34296,#34297,#34298,#34299,#34300,#34301,#34302,#34303,#34304,#34305,
#34306,#34307,#34308,#34309),.UNSPECIFIED.,.F.,.F.,(4,2,2,2,2,2,2,2,2,2,
2,2,2,2,2,2,2,2,2,2,2,2,2,2,2,2,2,2,2,2,2,2,2,2,2,2,2,2,2,2,2,2,2,2,2,2,
2,2,2,2,2,2,2,2,2,2,2,2,2,2,2,2,2,2,2,2,2,2,2,2,2,2,2,2,2,2,2,2,2,2,2,2,
2,2,2,2,4),(-4.27162971850408,-4.21647145483053,-4.16935911810154,-4.14070617443029,
-4.12950679259992,-4.12139380677792,-4.11285740367882,-4.09944885629476,
-4.04646006949341,-3.99134782946366,-3.96619574600893,-3.95880428730962,
-3.95407704652289,-3.94985293354377,-3.94265223304114,-3.92146440205188,
-3.86460330963846,-3.8133320373352,-3.79760013347601,-3.7885857185974,-3.78061867797267,
-3.77048429354131,-3.75391110738484,-3.67617235962659,-3.63512231336485,
-3.62460829613906,-3.619225870845,-3.61472848607077,-3.60882420596542,-3.59510384854512,
-3.53175324938251,-3.47242878199998,-3.45892037960446,-3.45036351153777,
-3.44226087351411,-3.43112399531668,-3.40470154143459,-3.32293733235216,
-3.30300268693756,-3.2894668338292,-3.28353027001578,-3.2790384958121,-3.2736046531874,
-3.26316023679669,-3.20744021218963,-3.15963795216371,-3.13074302890395,
-3.11951128464398,-3.11139276834333,-3.10286645866028,-3.08950780457596,
-3.03879173020421,-2.98880058588685,-2.96737538921008,-2.95313516320461,
-2.94708214192599,-2.94262071031482,-2.93728822221085,-2.92732429090972,
-2.85089527879434,-2.80115910526737,-2.78657615176535,-2.77779812319084,
-2.76978053137152,-2.7593874387562,-2.73644951866057,-2.66407402854572,
-2.6214472071367,-2.61304066857376,-2.60809559919181,-2.60351970426755,
-2.59665861654961,-2.57814627226511,-2.51184798938324,-2.47833472858878,
-2.45522256679618,-2.44484479204605,-2.43685173195352,-2.42797665594156,
-2.41292369964032,-2.33475596651531,-2.30077297787767,-2.28147708800115,
-2.27470707716446,-2.27010206256504,-2.26510897589423,-2.25669555075149),
 .UNSPECIFIED.);
#2111=B_SPLINE_CURVE_WITH_KNOTS('',3,(#34315,#34316,#34317,#34318,#34319,
#34320,#34321,#34322,#34323,#34324,#34325,#34326,#34327,#34328,#34329,#34330,
#34331,#34332,#34333,#34334,#34335,#34336,#34337,#34338,#34339,#34340,#34341,
#34342,#34343,#34344,#34345,#34346,#34347,#34348,#34349,#34350,#34351,#34352,
#34353,#34354,#34355,#34356,#34357,#34358,#34359,#34360,#34361,#34362,#34363,
#34364,#34365,#34366,#34367,#34368,#34369,#34370,#34371,#34372,#34373,#34374,
#34375,#34376,#34377,#34378,#34379,#34380,#34381,#34382,#34383,#34384,#34385,
#34386,#34387,#34388,#34389,#34390,#34391,#34392,#34393,#34394,#34395,#34396,
#34397,#34398,#34399,#34400,#34401,#34402,#34403,#34404,#34405,#34406,#34407,
#34408,#34409,#34410,#34411,#34412,#34413,#34414,#34415,#34416,#34417,#34418,
#34419,#34420,#34421,#34422,#34423,#34424,#34425,#34426,#34427,#34428,#34429,
#34430,#34431,#34432,#34433,#34434,#34435,#34436,#34437,#34438,#34439,#34440,
#34441,#34442,#34443,#34444,#34445,#34446,#34447,#34448,#34449,#34450,#34451,
#34452,#34453,#34454,#34455,#34456,#34457,#34458,#34459,#34460,#34461,#34462,
#34463,#34464,#34465,#34466,#34467,#34468,#34469,#34470,#34471,#34472,#34473,
#34474,#34475,#34476,#34477,#34478,#34479,#34480,#34481,#34482,#34483,#34484,
#34485,#34486,#34487,#34488,#34489,#34490,#34491,#34492,#34493,#34494,#34495,
#34496,#34497,#34498),.UNSPECIFIED.,.F.,.F.,(4,2,2,2,2,2,2,2,2,2,2,2,2,
2,2,2,2,2,2,2,2,2,2,2,2,2,2,2,2,2,2,2,2,2,2,2,2,2,2,2,2,2,2,2,2,2,2,2,2,
2,2,2,2,2,2,2,2,2,2,2,2,2,2,2,2,2,2,2,2,2,2,2,2,2,2,2,2,2,2,2,2,2,2,2,2,
2,2,2,2,2,2,4),(-2.01520948096664,-2.00714966847584,-1.99120964466136,-1.98206359854776,
-1.9741140621053,-1.96417976659391,-1.9436580874181,-1.86826470998595,-1.82479760849636,
-1.81629583250565,-1.811330398371,-1.80671156184379,-1.79986500223167,-1.77993818866968,
-1.74410159940624,-1.66927627089529,-1.65399714801093,-1.64499254446706,
-1.63702447368903,-1.62687550007638,-1.60512834508337,-1.57447188850431,
-1.56005588883022,-1.49722787237706,-1.48333823662209,-1.47775362881404,
-1.47321658496489,-1.46819038909922,-1.45940341807256,-1.44828100046701,
-1.42262517206948,-1.33898213335442,-1.319984716643,-1.31021051423517,-1.30227130083805,
-1.2930051921322,-1.27601870830014,-1.25425667506102,-1.19588572288241,
-1.151537258383,-1.14303198573574,-1.13806614390089,-1.13344830994648,-1.12660520695635,
-1.10670328369768,-1.07093864220888,-0.996000658509977,-0.980556083160654,
-0.971601336953702,-0.963625801812645,-0.953395889306798,-0.931168427582342,
-0.899523888576052,-0.862214307362673,-0.818732447730419,-0.808018510606879,
-0.802597406683794,-0.798105599198714,-0.79215510823377,-0.778531478421417,
-0.758410106682633,-0.674183301024425,-0.649857248695053,-0.640063376602571,
-0.631958227018882,-0.623566683980017,-0.610865829747433,-0.567461727852808,
-0.527686177663002,-0.482310317332872,-0.47149264194447,-0.466051484430089,
-0.461604893462648,-0.455708335641188,-0.442401438811369,-0.422935488793669,
-0.346857777686487,-0.315621487148793,-0.303782398475346,-0.295640057984666,
-0.287298202427402,-0.274846507863389,-0.234570170721794,-0.192797259552049,
-0.145692833123208,-0.134920400312372,-0.129488251705744,-0.124998184520262,
-0.119064185883121,-0.105535772772246,-0.0856116831592208,-0.000971006619263802),
 .UNSPECIFIED.);
#2112=B_SPLINE_CURVE_WITH_KNOTS('',3,(#34499,#34500,#34501,#34502,#34503,
#34504,#34505,#34506,#34507,#34508,#34509,#34510,#34511,#34512,#34513,#34514,
#34515,#34516),.UNSPECIFIED.,.F.,.F.,(4,2,2,2,2,2,2,2,4),(-4.27109517320269,
-4.25595028618041,-4.24411643550503,-4.23615525313697,-4.22859989927471,
-4.22012636940361,-4.20702173602339,-4.16036421318888,-4.15039881543784),
 .UNSPECIFIED.);
#2113=B_SPLINE_CURVE_WITH_KNOTS('',3,(#34517,#34518,#34519,#34520,#34521,
#34522,#34523,#34524,#34525,#34526,#34527,#34528,#34529,#34530,#34531,#34532,
#34533,#34534,#34535,#34536,#34537,#34538,#34539,#34540,#34541,#34542,#34543,
#34544,#34545,#34546,#34547,#34548,#34549,#34550,#34551,#34552,#34553,#34554,
#34555,#34556,#34557,#34558,#34559,#34560,#34561,#34562,#34563,#34564,#34565,
#34566,#34567,#34568,#34569,#34570,#34571,#34572,#34573,#34574,#34575,#34576,
#34577,#34578,#34579,#34580,#34581,#34582,#34583,#34584,#34585,#34586,#34587,
#34588,#34589,#34590,#34591,#34592,#34593,#34594,#34595,#34596,#34597,#34598,
#34599,#34600,#34601,#34602,#34603,#34604,#34605,#34606,#34607,#34608,#34609,
#34610,#34611,#34612,#34613,#34614,#34615,#34616,#34617,#34618,#34619,#34620,
#34621,#34622,#34623,#34624,#34625,#34626,#34627,#34628,#34629,#34630,#34631,
#34632,#34633,#34634,#34635,#34636,#34637,#34638,#34639,#34640,#34641,#34642,
#34643,#34644,#34645,#34646,#34647,#34648,#34649,#34650,#34651,#34652,#34653,
#34654,#34655,#34656,#34657,#34658,#34659,#34660,#34661,#34662,#34663,#34664,
#34665,#34666,#34667,#34668,#34669,#34670,#34671,#34672,#34673,#34674,#34675,
#34676,#34677,#34678,#34679,#34680,#34681,#34682,#34683,#34684,#34685,#34686,
#34687,#34688,#34689,#34690,#34691,#34692,#34693,#34694,#34695,#34696,#34697,
#34698,#34699,#34700,#34701,#34702,#34703,#34704),.UNSPECIFIED.,.F.,.F.,
(4,2,2,2,2,2,2,2,2,2,2,2,2,2,2,2,2,2,2,2,2,2,2,2,2,2,2,2,2,2,2,2,2,2,2,
2,2,2,2,2,2,2,2,2,2,2,2,2,2,2,2,2,2,2,2,2,2,2,2,2,2,2,2,2,2,2,2,2,2,2,2,
2,2,2,2,2,2,2,2,2,2,2,2,2,2,2,2,2,2,2,2,2,2,4),(-2.25669555075149,-2.25647827895454,
-2.20578058586402,-2.16268910067092,-2.13632276437092,-2.11677383023448,
-2.10701565089744,-2.09907620001544,-2.08979480068367,-2.07273525067124,
-2.05084829556189,-1.99176820740479,-1.94834782052542,-1.93984615853667,
-1.9348806641097,-1.9302616643194,-1.92341471009007,-1.90348559916168,-1.86764277222077,
-1.79282472224593,-1.7775441896738,-1.76853912840511,-1.76057087696362,
-1.75042198070147,-1.72867628794975,-1.69802317465763,-1.68362096182469,
-1.62082906624937,-1.60689818337004,-1.60130672704128,-1.59676803218511,
-1.59174535291663,-1.58297530352149,-1.52841708151284,-1.45670808658164,
-1.4411391115441,-1.43207254033551,-1.42491009139806,-1.41525301632689,
-1.39624432081175,-1.34825113184082,-1.28766038015784,-1.27113260619435,
-1.26456398245095,-1.2599939956188,-1.25492155714437,-1.24591584879435,
-1.19490619992112,-1.11940826874441,-1.10402666402093,-1.09508498211598,
-1.0871072916481,-1.07685537733022,-1.05449601422997,-1.02257682305855,
-0.985463330744092,-0.942240468954855,-0.931538012105892,-0.926119254621201,
-0.921627344919087,-0.915674046792797,-0.902033083617493,-0.881875275748018,
-0.797135529117148,-0.773130621423109,-0.763426894080399,-0.755343659332821,
-0.746920618150429,-0.734061707832606,-0.688413450433646,-0.674871928842943,
-0.613983211505506,-0.597814347758796,-0.591304877975362,-0.586745006251162,
-0.581647886094767,-0.572522621328682,-0.519828088916931,-0.446696116133087,
-0.431254578705578,-0.422216765547528,-0.415052805950926,-0.405362078722874,
-0.386165424468412,-0.336727645992747,-0.273083181667143,-0.259746139481906,
-0.253907238003859,-0.249416934433612,-0.24398947565407,-0.233240119710802,
-0.189992222714209,-0.121892388973597,-0.121708560596655),.UNSPECIFIED.);
#2114=B_SPLINE_CURVE_WITH_KNOTS('',3,(#34709,#34710,#34711,#34712,#34713,
#34714,#34715,#34716,#34717,#34718,#34719,#34720,#34721,#34722,#34723,#34724,
#34725,#34726,#34727,#34728,#34729,#34730,#34731,#34732,#34733,#34734,#34735,
#34736,#34737,#34738,#34739,#34740,#34741,#34742,#34743,#34744,#34745,#34746,
#34747,#34748,#34749,#34750,#34751,#34752,#34753,#34754,#34755,#34756,#34757,
#34758,#34759,#34760,#34761,#34762,#34763,#34764,#34765,#34766,#34767,#34768,
#34769,#34770,#34771,#34772,#34773,#34774,#34775,#34776,#34777,#34778,#34779,
#34780,#34781,#34782,#34783,#34784,#34785,#34786,#34787,#34788,#34789,#34790,
#34791,#34792,#34793,#34794,#34795,#34796,#34797,#34798,#34799,#34800,#34801,
#34802,#34803,#34804,#34805,#34806,#34807,#34808,#34809,#34810,#34811,#34812,
#34813,#34814,#34815,#34816,#34817,#34818,#34819,#34820,#34821,#34822,#34823,
#34824,#34825,#34826,#34827,#34828,#34829,#34830,#34831,#34832,#34833,#34834,
#34835,#34836,#34837,#34838,#34839,#34840,#34841,#34842,#34843,#34844,#34845,
#34846,#34847,#34848,#34849,#34850,#34851,#34852,#34853,#34854,#34855,#34856,
#34857,#34858,#34859,#34860,#34861,#34862,#34863,#34864,#34865,#34866,#34867,
#34868,#34869,#34870,#34871,#34872,#34873,#34874,#34875,#34876,#34877,#34878,
#34879,#34880,#34881,#34882,#34883,#34884,#34885,#34886,#34887,#34888,#34889,
#34890,#34891,#34892),.UNSPECIFIED.,.F.,.F.,(4,2,2,2,2,2,2,2,2,2,2,2,2,
2,2,2,2,2,2,2,2,2,2,2,2,2,2,2,2,2,2,2,2,2,2,2,2,2,2,2,2,2,2,2,2,2,2,2,2,
2,2,2,2,2,2,2,2,2,2,2,2,2,2,2,2,2,2,2,2,2,2,2,2,2,2,2,2,2,2,2,2,2,2,2,2,
2,2,2,2,2,2,4),(-4.15027967554863,-4.14937388203919,-4.09344939889395,-4.04579468576531,
-4.01695395733201,-4.00573109430837,-3.99761549210625,-3.98908913029071,
-3.97572374309468,-3.92130918179524,-3.86728344800363,-3.84237233664458,
-3.83500391597726,-3.83028216152486,-3.82605527591796,-3.81883620293387,
-3.79747995843651,-3.73401372265628,-3.68454609972552,-3.67145226361893,
-3.6629814182495,-3.65492686095805,-3.64358731177808,-3.61594467822811,
-3.5357293408631,-3.51591949993915,-3.50244476091155,-3.49651942694312,
-3.49202946323963,-3.48658959364629,-3.47577970153583,-3.43052383209003,
-3.39103653714101,-3.34719942263865,-3.33446540892421,-3.32606687266516,
-3.31796581536067,-3.30819023665638,-3.28398326157704,-3.19964409645301,
-3.17952059517719,-3.16589485981238,-3.15994389013728,-3.15545184075872,
-3.15003067911981,-3.13931715331926,-3.09587695755976,-3.05868726476909,
-3.02690120917323,-3.0046068268778,-2.99436531761095,-2.98638832381839,
-2.97743978961056,-2.96202630565742,-2.88686132114048,-2.83575042883008,
-2.82667852656827,-2.82159194461223,-2.8170269386768,-2.81048989921304,
-2.79415938011912,-2.73335926399411,-2.67542744237923,-2.6619629098778,
-2.65341568467747,-2.64530963875434,-2.63414777431965,-2.6075155577395,
-2.52600660098006,-2.50609318920533,-2.49256800147907,-2.48663365013921,
-2.48214249519008,-2.47670810662228,-2.46625930554312,-2.41066259864094,
-2.36279188127302,-2.33387455273174,-2.3226406742808,-2.31452250201875,
-2.30599822709262,-2.29264633273593,-2.24214136140902,-2.18496208613476,
-2.15937392327269,-2.1519438744113,-2.14720881417966,-2.14299161146603,
-2.13582721378967,-2.11302658787055,-2.06762420495383,-2.01520948096664),
 .UNSPECIFIED.);
#2115=B_SPLINE_CURVE_WITH_KNOTS('',3,(#34894,#34895,#34896,#34897,#34898,
#34899,#34900,#34901,#34902,#34903,#34904,#34905,#34906,#34907,#34908,#34909),
 .UNSPECIFIED.,.F.,.F.,(4,2,2,2,2,2,2,4),(-0.121708560596655,-0.0989053417075304,
-0.0886612869199451,-0.0806657415004705,-0.0718170542222974,-0.0626305895064228,
-0.0422719233860505,-0.000969933537610637),.UNSPECIFIED.);
#2116=B_SPLINE_CURVE_WITH_KNOTS('',3,(#34910,#34911,#34912,#34913,#34914,
#34915,#34916,#34917,#34918,#34919,#34920,#34921,#34922,#34923,#34924,#34925,
#34926,#34927,#34928,#34929,#34930,#34931,#34932,#34933,#34934,#34935,#34936,
#34937,#34938,#34939,#34940,#34941,#34942,#34943,#34944,#34945,#34946,#34947,
#34948,#34949,#34950,#34951,#34952,#34953,#34954,#34955,#34956,#34957,#34958,
#34959,#34960,#34961,#34962,#34963,#34964,#34965,#34966,#34967,#34968,#34969,
#34970,#34971,#34972,#34973,#34974,#34975,#34976,#34977,#34978,#34979,#34980,
#34981,#34982,#34983,#34984,#34985,#34986,#34987,#34988,#34989,#34990,#34991,
#34992,#34993,#34994,#34995,#34996,#34997,#34998,#34999,#35000,#35001,#35002,
#35003,#35004,#35005,#35006,#35007,#35008,#35009,#35010,#35011,#35012,#35013,
#35014,#35015,#35016,#35017,#35018,#35019,#35020,#35021,#35022,#35023,#35024,
#35025,#35026,#35027,#35028,#35029,#35030,#35031,#35032,#35033,#35034,#35035,
#35036,#35037,#35038,#35039,#35040,#35041,#35042,#35043,#35044,#35045,#35046,
#35047,#35048,#35049,#35050,#35051,#35052,#35053,#35054,#35055,#35056,#35057,
#35058,#35059,#35060,#35061,#35062,#35063,#35064,#35065,#35066,#35067,#35068,
#35069,#35070,#35071,#35072,#35073,#35074,#35075,#35076,#35077,#35078,#35079,
#35080,#35081,#35082,#35083,#35084,#35085),.UNSPECIFIED.,.F.,.F.,(4,2,2,
2,2,2,2,2,2,2,2,2,2,2,2,2,2,2,2,2,2,2,2,2,2,2,2,2,2,2,2,2,2,2,2,2,2,2,2,
2,2,2,2,2,2,2,2,2,2,2,2,2,2,2,2,2,2,2,2,2,2,2,2,2,2,2,2,2,2,2,2,2,2,2,2,
2,2,2,2,2,2,2,2,2,2,2,2,4),(-4.27062365544879,-4.2045854016667,-4.19594776882903,
-4.18871320832504,-4.1840190730819,-4.17917307545253,-4.17122421916764,
-4.14176590148942,-4.07982410625505,-4.05144086621091,-4.03083792688231,
-4.02088977072974,-4.01294005531295,-4.00380572398322,-3.98791739849639,
-3.92090316498426,-3.86210949373818,-3.85345171741014,-3.84845329333739,
-3.84390473758457,-3.83719463006745,-3.81975505817798,-3.75990468608033,
-3.7123058962321,-3.69332118613209,-3.68366884260179,-3.67650714934979,
-3.66743785317878,-3.65185473269206,-3.58041310104364,-3.5256247144009,
-3.51689024162895,-3.51187532397132,-3.50733377283615,-3.50172882381573,
-3.48771414779401,-3.42496923263108,-3.36597081471164,-3.35247377611142,
-3.34392014424755,-3.3358178393593,-3.32467700619564,-3.29820919005584,
-3.21651417438742,-3.19658699185784,-3.18305534790896,-3.17712006671082,
-3.17262902203515,-3.167195766215,-3.15642123192552,-3.11175150030842,-3.0735105775042,
-3.02801563126963,-3.0151644298852,-3.00674187060416,-2.99865586845352,
-2.9889449512708,-2.96489947351059,-2.88023905105316,-2.86009124081783,
-2.84645350092496,-2.84050018196501,-2.83600758449604,-2.83058726262261,
-2.82020597141197,-2.76330846481984,-2.71624935782424,-2.68761628669727,
-2.67642022183258,-2.66830834663445,-2.65977196016267,-2.6463609650568,
-2.59320424871988,-2.54532411989866,-2.52417145256917,-2.51005861896083,
-2.50402675351805,-2.49952764668416,-2.49416346978328,-2.48404860475659,
-2.40844300856654,-2.37315847519949,-2.34923736215947,-2.33873005593193,
-2.33072176651715,-2.32191375841392,-2.30718277846463,-2.25630106598102),
 .UNSPECIFIED.);
#2117=B_SPLINE_CURVE_WITH_KNOTS('',3,(#35091,#35092,#35093,#35094,#35095,
#35096,#35097,#35098,#35099,#35100,#35101,#35102,#35103,#35104,#35105,#35106,
#35107,#35108,#35109,#35110,#35111,#35112,#35113,#35114,#35115,#35116,#35117,
#35118,#35119,#35120,#35121,#35122,#35123,#35124,#35125,#35126,#35127,#35128,
#35129,#35130,#35131,#35132,#35133,#35134,#35135,#35136,#35137,#35138,#35139,
#35140,#35141,#35142,#35143,#35144,#35145,#35146,#35147,#35148,#35149,#35150,
#35151,#35152,#35153,#35154,#35155,#35156,#35157,#35158,#35159,#35160,#35161,
#35162,#35163,#35164,#35165,#35166,#35167,#35168,#35169,#35170,#35171,#35172,
#35173,#35174,#35175,#35176,#35177,#35178,#35179,#35180,#35181,#35182,#35183,
#35184,#35185,#35186,#35187,#35188,#35189,#35190,#35191,#35192,#35193,#35194,
#35195,#35196,#35197,#35198,#35199,#35200,#35201,#35202,#35203,#35204,#35205,
#35206,#35207,#35208,#35209,#35210,#35211,#35212,#35213,#35214,#35215,#35216,
#35217,#35218,#35219,#35220,#35221,#35222,#35223,#35224,#35225,#35226,#35227,
#35228,#35229,#35230,#35231,#35232,#35233,#35234,#35235,#35236,#35237,#35238,
#35239,#35240,#35241,#35242,#35243,#35244,#35245,#35246,#35247,#35248,#35249,
#35250,#35251,#35252,#35253,#35254,#35255,#35256,#35257,#35258,#35259,#35260,
#35261,#35262,#35263,#35264,#35265,#35266,#35267,#35268,#35269,#35270,#35271,
#35272),.UNSPECIFIED.,.F.,.F.,(4,2,2,2,2,2,2,2,2,2,2,2,2,2,2,2,2,2,2,2,
2,2,2,2,2,2,2,2,2,2,2,2,2,2,2,2,2,2,2,2,2,2,2,2,2,2,2,2,2,2,2,2,2,2,2,2,
2,2,2,2,2,2,2,2,2,2,2,2,2,2,2,2,2,2,2,2,2,2,2,2,2,2,2,2,2,2,2,2,2,2,4),
(-2.01540403041363,-1.97105087182943,-1.93084919110475,-1.9224104388942,
-1.91745914148358,-1.91283411580665,-1.90595068542143,-1.88570462132828,
-1.84889588021947,-1.77578571549031,-1.76033977362606,-1.75130039884835,
-1.74413574399215,-1.73444478558129,-1.71525041721242,-1.66580267212204,
-1.60216460957617,-1.58881549615542,-1.58297417643701,-1.57848325181503,
-1.57305659400479,-1.56231314834687,-1.51912740404222,-1.43715435929942,
-1.42262529873154,-1.41385990755967,-1.40584139840264,-1.39524837742795,
-1.37077410014621,-1.33424309267047,-1.27904087477932,-1.25572791374213,
-1.24830390298614,-1.24403896045695,-1.23936025072194,-1.23219942426583,
-1.20942266243595,-1.16409962945601,-1.1035462346794,-1.08761075996848,
-1.07846702204661,-1.07051931868482,-1.06058708637759,-1.04006878571749,
-0.964690282576342,-0.92123806632143,-0.912738303588415,-0.907774032884151,
-0.903156268135697,-0.896311282261529,-0.876388936118637,-0.840560173777627,
-0.765753188958409,-0.750477526058375,-0.741474998318385,-0.733508786457134,
-0.723362210779881,-0.701620321460426,-0.670971413661392,-0.656560136610894,
-0.593750419093718,-0.579860058722233,-0.574276101613057,-0.569739966332332,
-0.564715296331333,-0.555932041671417,-0.544814981055154,-0.519175287262509,
-0.435630593574715,-0.416578711984817,-0.406795181440412,-0.398857230770941,
-0.389602566155293,-0.372666787672479,-0.350990251114021,-0.29308907677258,
-0.248139866157751,-0.239633955500326,-0.23466870949306,-0.230052247722714,
-0.223212344624252,-0.203328493638811,-0.165047205734008,-0.0968343148362305,
-0.0807251579815768,-0.0707223802273352,-0.0627697178572486,-0.0552960657740107,
-0.0463378343276242,-0.0291380055809453,-0.000969506735735101),
 .UNSPECIFIED.);
#2118=B_SPLINE_CURVE_WITH_KNOTS('',3,(#35273,#35274,#35275,#35276,#35277,
#35278,#35279,#35280,#35281,#35282,#35283,#35284,#35285,#35286,#35287,#35288),
 .UNSPECIFIED.,.F.,.F.,(4,2,2,2,2,2,2,4),(-4.27050797530105,-4.20918175648102,
-4.18921511742037,-4.17566477666909,-4.16972660284406,-4.16523563613543,
-4.15980525540617,-4.15027967554863),.UNSPECIFIED.);
#2119=B_SPLINE_CURVE_WITH_KNOTS('',3,(#35289,#35290,#35291,#35292,#35293,
#35294,#35295,#35296,#35297,#35298,#35299,#35300,#35301,#35302,#35303,#35304,
#35305,#35306,#35307,#35308,#35309,#35310,#35311,#35312,#35313,#35314,#35315,
#35316,#35317,#35318,#35319,#35320,#35321,#35322,#35323,#35324,#35325,#35326,
#35327,#35328,#35329,#35330,#35331,#35332,#35333,#35334,#35335,#35336,#35337,
#35338,#35339,#35340,#35341,#35342,#35343,#35344,#35345,#35346,#35347,#35348,
#35349,#35350,#35351,#35352,#35353,#35354,#35355,#35356,#35357,#35358,#35359,
#35360,#35361,#35362,#35363,#35364,#35365,#35366,#35367,#35368,#35369,#35370,
#35371,#35372,#35373,#35374,#35375,#35376,#35377,#35378,#35379,#35380,#35381,
#35382,#35383,#35384,#35385,#35386,#35387,#35388,#35389,#35390,#35391,#35392,
#35393,#35394,#35395,#35396,#35397,#35398,#35399,#35400,#35401,#35402,#35403,
#35404,#35405,#35406,#35407,#35408,#35409,#35410,#35411,#35412,#35413,#35414,
#35415,#35416,#35417,#35418,#35419,#35420,#35421,#35422,#35423,#35424,#35425,
#35426,#35427,#35428,#35429,#35430,#35431,#35432,#35433,#35434,#35435,#35436,
#35437,#35438,#35439,#35440,#35441,#35442,#35443,#35444,#35445,#35446,#35447,
#35448,#35449,#35450,#35451,#35452,#35453,#35454,#35455,#35456,#35457,#35458,
#35459,#35460,#35461,#35462,#35463,#35464,#35465,#35466,#35467,#35468,#35469,
#35470,#35471,#35472,#35473,#35474,#35475,#35476,#35477,#35478,#35479,#35480),
 .UNSPECIFIED.,.F.,.F.,(4,2,2,2,2,2,2,2,2,2,2,2,2,2,2,2,2,2,2,2,2,2,2,2,
2,2,2,2,2,2,2,2,2,2,2,2,2,2,2,2,2,2,2,2,2,2,2,2,2,2,2,2,2,2,2,2,2,2,2,2,
2,2,2,2,2,2,2,2,2,2,2,2,2,2,2,2,2,2,2,2,2,2,2,2,2,2,2,2,2,2,2,2,2,2,2,4),
(-2.25630106598102,-2.22665188879084,-2.17869341128798,-2.17014812749761,
-2.16517353502421,-2.16061327301725,-2.15383763824685,-2.13593453700016,
-2.10493148874884,-2.02461880953053,-2.008489005903,-1.99930281207444,-1.99135738846346,
-1.98147908044215,-1.96126788018294,-1.88643911726412,-1.84194590014947,
-1.83343942038279,-1.82847310019824,-1.82385501306422,-1.81701180837149,
-1.79711164667502,-1.7613539425913,-1.68639388790096,-1.67095006657059,
-1.66199507027169,-1.65401890969819,-1.64378763498014,-1.62155477871562,
-1.58990006365558,-1.55259707823166,-1.50911627441789,-1.49840176846068,
-1.49298032102185,-1.48848819578634,-1.48253724097305,-1.46891237560183,
-1.44878900710068,-1.3645481816212,-1.34022673719909,-1.33043315772026,
-1.32232767956074,-1.31393521513241,-1.30123179687271,-1.25780207293039,
-1.21804096198826,-1.17266992891469,-1.16185205132341,-1.1564106215643,
-1.15196371009145,-1.14606660037006,-1.13275795317811,-1.11328895698438,
-1.03718695050705,-1.00596565688298,-0.994127752130195,-0.98598521223695,
-0.97764232529372,-0.965187474978963,-0.924881387000842,-0.883120502128747,
-0.836029481961262,-0.82525642770728,-0.819823926033665,-0.815333544401949,
-0.809399101155309,-0.795869557094396,-0.775943688955905,-0.694322035280049,
-0.667764199661518,-0.656613205219409,-0.648510217404342,-0.639961900885749,
-0.626486229351708,-0.568080916515301,-0.506404869931409,-0.491201225169912,
-0.484812416709915,-0.4802708344267,-0.475116628138645,-0.465718842718387,
-0.418204251226746,-0.339084702663833,-0.324158143105303,-0.315311005813255,
-0.307314811154912,-0.296892298533253,-0.273490499830659,-0.239348203981405,
-0.169039366723416,-0.154450184279452,-0.148755300277396,-0.144193160304904,
-0.139226329550409,-0.1307130459406,-0.12134621462309),.UNSPECIFIED.);
#2120=B_SPLINE_CURVE_WITH_KNOTS('',3,(#35485,#35486,#35487,#35488,#35489,
#35490,#35491,#35492,#35493,#35494,#35495,#35496,#35497,#35498,#35499,#35500,
#35501,#35502,#35503,#35504,#35505,#35506,#35507,#35508,#35509,#35510,#35511,
#35512,#35513,#35514,#35515,#35516,#35517,#35518,#35519,#35520,#35521,#35522,
#35523,#35524,#35525,#35526,#35527,#35528,#35529,#35530,#35531,#35532,#35533,
#35534,#35535,#35536,#35537,#35538,#35539,#35540,#35541,#35542,#35543,#35544,
#35545,#35546,#35547,#35548,#35549,#35550,#35551,#35552,#35553,#35554,#35555,
#35556,#35557,#35558,#35559,#35560,#35561,#35562,#35563,#35564,#35565,#35566,
#35567,#35568,#35569,#35570,#35571,#35572,#35573,#35574,#35575,#35576,#35577,
#35578,#35579,#35580,#35581,#35582,#35583,#35584,#35585,#35586,#35587,#35588,
#35589,#35590,#35591,#35592,#35593,#35594,#35595,#35596,#35597,#35598,#35599,
#35600,#35601,#35602,#35603,#35604,#35605,#35606,#35607,#35608,#35609,#35610,
#35611,#35612,#35613,#35614,#35615,#35616,#35617,#35618,#35619,#35620,#35621,
#35622,#35623,#35624,#35625,#35626,#35627,#35628,#35629,#35630,#35631,#35632,
#35633,#35634,#35635,#35636,#35637,#35638,#35639,#35640,#35641,#35642,#35643,
#35644,#35645,#35646,#35647,#35648,#35649,#35650,#35651,#35652,#35653,#35654,
#35655,#35656,#35657,#35658,#35659,#35660,#35661,#35662,#35663,#35664,#35665,
#35666,#35667,#35668,#35669,#35670,#35671,#35672,#35673,#35674,#35675,#35676,
#35677,#35678),.UNSPECIFIED.,.F.,.F.,(4,2,2,2,2,2,2,2,2,2,2,2,2,2,2,2,2,
2,2,2,2,2,2,2,2,2,2,2,2,2,2,2,2,2,2,2,2,2,2,2,2,2,2,2,2,2,2,2,2,2,2,2,2,
2,2,2,2,2,2,2,2,2,2,2,2,2,2,2,2,2,2,2,2,2,2,2,2,2,2,2,2,2,2,2,2,2,2,2,2,
2,2,2,2,2,2,2,4),(-4.15012784700328,-4.13768479087268,-4.11856038692716,
-4.10888262908483,-4.10171943274022,-4.09267098242306,-4.07718174678539,
-4.00462979355366,-3.95114543254014,-3.94221997146866,-3.93716484225613,
-3.9325888492165,-3.92702866492889,-3.91328394762036,-3.85029839280303,
-3.83580949968707,-3.80513830683069,-3.78338664403422,-3.77323799165445,
-3.76527125700535,-3.75626931161481,-3.74099745979581,-3.66620715221463,
-3.63040419672153,-3.61048991443097,-3.60364585284258,-3.59902809761266,
-3.59406323625909,-3.58556118908269,-3.54203078285546,-3.46664636078207,
-3.44613911912456,-3.43620860411234,-3.42826082946351,-3.41911543440626,
-3.40317277771717,-3.34494399390341,-3.29792230798571,-3.27469641717895,
-3.26749016680202,-3.2628021815342,-3.2585461780006,-3.25116953473084,-3.22834090593342,
-3.16627705022579,-3.11718274732264,-3.10411091757459,-3.09564516189169,
-3.0875890428566,-3.0762363730723,-3.04850387674872,-2.96840978302202,-2.9486111058567,
-2.93514217874399,-2.92921822140438,-2.92472879498221,-2.91928895502453,
-2.90847736434631,-2.8631834416426,-2.82360754468627,-2.7798968508195,-2.76717310780248,
-2.75877726160425,-2.75067583975485,-2.74089619370489,-2.71665888095593,
-2.63237133622941,-2.61225307828568,-2.59863028859254,-2.59268021320517,
-2.5881886725426,-2.58276792116707,-2.5720546432161,-2.52859810689668,-2.49136551580897,
-2.45962357568752,-2.4373511814138,-2.42711407875539,-2.41913830473275,
-2.41018885156645,-2.39476780294479,-2.31969439184951,-2.28405057724413,
-2.26418949417452,-2.25735177354734,-2.252735174401,-2.24776806466829,-2.23925557601856,
-2.19343191938615,-2.1361209766679,-2.10481334371136,-2.09296558141158,
-2.08556108274967,-2.07735584576061,-2.06562164239614,-2.03261516951048,
-2.01540403041363),.UNSPECIFIED.);
#2121=B_SPLINE_CURVE_WITH_KNOTS('',3,(#35680,#35681,#35682,#35683,#35684,
#35685,#35686,#35687),.UNSPECIFIED.,.F.,.F.,(4,2,2,4),(-0.12134621462309,
-0.0841733796356287,-0.0489133595461245,-0.000970789400192507),
 .UNSPECIFIED.);
#2122=B_SPLINE_CURVE_WITH_KNOTS('',3,(#35688,#35689,#35690,#35691,#35692,
#35693,#35694,#35695,#35696,#35697,#35698,#35699,#35700,#35701,#35702,#35703,
#35704,#35705,#35706,#35707,#35708,#35709,#35710,#35711,#35712,#35713,#35714,
#35715,#35716,#35717,#35718,#35719,#35720,#35721,#35722,#35723,#35724,#35725,
#35726,#35727,#35728,#35729,#35730,#35731,#35732,#35733,#35734,#35735,#35736,
#35737,#35738,#35739,#35740,#35741,#35742,#35743,#35744,#35745,#35746,#35747,
#35748,#35749,#35750,#35751,#35752,#35753,#35754,#35755,#35756,#35757,#35758,
#35759,#35760,#35761,#35762,#35763,#35764,#35765,#35766,#35767,#35768,#35769,
#35770,#35771,#35772,#35773,#35774,#35775,#35776,#35777,#35778,#35779,#35780,
#35781,#35782,#35783,#35784,#35785,#35786,#35787,#35788,#35789,#35790,#35791,
#35792,#35793,#35794,#35795,#35796,#35797,#35798,#35799,#35800,#35801,#35802,
#35803,#35804,#35805,#35806,#35807,#35808,#35809,#35810,#35811,#35812,#35813,
#35814,#35815,#35816,#35817,#35818,#35819,#35820,#35821,#35822,#35823,#35824,
#35825,#35826,#35827,#35828,#35829,#35830,#35831,#35832,#35833,#35834,#35835,
#35836,#35837,#35838,#35839,#35840,#35841,#35842,#35843,#35844,#35845,#35846,
#35847,#35848,#35849,#35850,#35851,#35852,#35853,#35854,#35855,#35856,#35857,
#35858,#35859,#35860,#35861,#35862,#35863,#35864,#35865,#35866,#35867,#35868,
#35869,#35870,#35871,#35872,#35873,#35874,#35875,#35876,#35877,#35878,#35879,
#35880,#35881,#35882,#35883,#35884,#35885,#35886),.UNSPECIFIED.,.F.,.F.,
(4,3,3,3,3,3,3,3,3,3,3,3,3,3,3,3,3,3,3,3,3,3,3,3,3,3,3,3,3,3,3,3,3,3,3,
3,3,3,3,3,3,3,3,3,3,3,3,3,3,3,3,3,3,3,3,3,3,3,3,3,3,3,3,3,3,3,4),(-16.4167960594917,
-16.3231866314087,-16.2295269003941,-16.1346626816157,-16.0407807338294,
-15.9454253795549,-15.8500700252804,-15.7580593289838,-15.666169660585,
-15.5743745685141,-15.4826447769296,-15.3909489474181,-15.2992633109964,
-15.207564113087,-15.1157697354696,-15.0239260396849,-14.9319324031901,
-14.8594406487004,-14.7674298823043,-14.6755401432034,-14.5837449799275,
-14.4920151166801,-14.4003192152502,-14.308633506742,-14.2169342366647,
-14.1251397872016,-14.0332960196421,-13.941302312234,-13.8688112721204,
-13.7768007953962,-13.6849113464236,-13.5931164733523,-13.5013868992429,
-13.4096912862,-13.3180058649905,-13.2263068807854,-13.1345127132284,-13.0426692258026,
-12.9506757927242,-12.8781818955404,-12.7861710643817,-12.6942812623679,
-12.6024860380833,-12.510756116906,-12.4190601594478,-12.3273743968664,
-12.2356750747262,-12.1438805766162,-12.0520367622262,-11.9600430114395,
-11.8875525189603,-11.7955413127616,-11.7036511308559,-11.6118555223852,
-11.5201252122009,-11.4284288629229,-11.3367427061933,-11.245042988059,
-11.1532480935682,-11.0614038819903,-10.9694097368279,-10.8969231423803,
-10.8060917931932,-10.7154014179413,-10.624792371434,-10.5342434733015,
-10.4883010731468),.UNSPECIFIED.);
#2123=B_SPLINE_CURVE_WITH_KNOTS('',3,(#35892,#35893,#35894,#35895,#35896,
#35897,#35898,#35899,#35900,#35901,#35902,#35903,#35904,#35905,#35906,#35907,
#35908,#35909,#35910,#35911,#35912,#35913,#35914,#35915,#35916,#35917,#35918,
#35919,#35920,#35921,#35922,#35923,#35924,#35925,#35926,#35927,#35928,#35929,
#35930,#35931,#35932,#35933,#35934,#35935,#35936,#35937,#35938,#35939,#35940,
#35941,#35942,#35943,#35944,#35945,#35946,#35947,#35948,#35949,#35950,#35951,
#35952,#35953,#35954,#35955,#35956,#35957,#35958,#35959,#35960,#35961,#35962,
#35963,#35964,#35965,#35966,#35967,#35968,#35969,#35970,#35971,#35972,#35973,
#35974,#35975,#35976,#35977,#35978,#35979,#35980,#35981,#35982,#35983,#35984,
#35985,#35986,#35987,#35988,#35989,#35990,#35991,#35992,#35993,#35994,#35995,
#35996,#35997,#35998,#35999,#36000,#36001,#36002,#36003,#36004,#36005,#36006,
#36007,#36008,#36009,#36010,#36011,#36012,#36013,#36014,#36015,#36016,#36017,
#36018,#36019),.UNSPECIFIED.,.F.,.F.,(4,2,2,2,2,2,2,2,2,2,2,2,2,2,2,2,2,
2,2,2,2,2,2,2,2,2,2,2,2,2,2,2,2,2,2,2,2,2,2,2,2,2,2,2,2,2,2,2,2,2,2,2,2,
2,2,2,2,2,2,2,2,2,2,4),(0.000234205929175261,0.00314848603653745,0.0067045111635944,
0.0168739000398768,0.0615307527646696,0.107334776582209,0.134796991517308,
0.146454022578125,0.155357023913133,0.1652275816112,0.182046717494131,0.274726979642122,
0.320861047165836,0.329525968901998,0.334551414402502,0.339045553572495,
0.345512518537176,0.362198977451867,0.422255985535926,0.46061653869019,
0.485633015473455,0.496017784180939,0.503706305636458,0.511933002375833,
0.525114218951138,0.577956322639473,0.637361486507521,0.654976985957441,
0.667261308249631,0.672788245216847,0.677173157397879,0.682612824762992,
0.693104287233814,0.735392797844991,0.810846433052819,0.83035092034576,
0.840176814946397,0.847438120612499,0.856601019533708,0.872291963298752,
0.937037200195196,0.977056452679149,0.998292865919186,1.00537849982969,
1.01011462818581,1.01511874622903,1.02366974728301,1.06906727212008,1.126308523086,
1.14786674619417,1.16474307983491,1.17401558827739,1.18199803909754,1.19187567048779,
1.21191633823506,1.30302015212422,1.32363980923898,1.33751136488475,1.3435116830711,
1.34800515020899,1.35337159037266,1.36388540057331,1.42020101528312,1.42896226070502),
 .UNSPECIFIED.);
#2124=B_SPLINE_CURVE_WITH_KNOTS('',3,(#36022,#36023,#36024,#36025,#36026,
#36027,#36028,#36029,#36030,#36031,#36032,#36033,#36034,#36035,#36036,#36037,
#36038,#36039,#36040,#36041,#36042,#36043,#36044,#36045,#36046,#36047,#36048,
#36049,#36050,#36051,#36052,#36053,#36054,#36055,#36056,#36057,#36058,#36059,
#36060,#36061,#36062,#36063,#36064,#36065,#36066,#36067,#36068,#36069,#36070,
#36071,#36072,#36073,#36074,#36075,#36076,#36077,#36078,#36079,#36080,#36081,
#36082,#36083,#36084,#36085,#36086,#36087,#36088,#36089,#36090,#36091,#36092,
#36093,#36094,#36095,#36096,#36097,#36098,#36099,#36100,#36101,#36102,#36103,
#36104,#36105,#36106,#36107,#36108,#36109,#36110,#36111,#36112,#36113,#36114,
#36115,#36116,#36117,#36118,#36119,#36120,#36121,#36122,#36123,#36124,#36125,
#36126,#36127,#36128,#36129,#36130,#36131,#36132,#36133,#36134,#36135,#36136,
#36137,#36138,#36139,#36140,#36141,#36142,#36143,#36144,#36145,#36146,#36147,
#36148,#36149,#36150,#36151,#36152,#36153,#36154,#36155,#36156,#36157,#36158,
#36159,#36160,#36161,#36162,#36163,#36164,#36165,#36166,#36167,#36168,#36169,
#36170,#36171,#36172,#36173,#36174,#36175,#36176,#36177,#36178,#36179,#36180,
#36181,#36182,#36183,#36184,#36185,#36186,#36187,#36188,#36189,#36190,#36191,
#36192,#36193,#36194,#36195,#36196,#36197,#36198,#36199),.UNSPECIFIED.,
 .F.,.F.,(4,2,2,2,2,2,2,2,2,2,2,2,2,2,2,2,2,2,2,2,2,2,2,2,2,2,2,2,2,2,2,
2,2,2,2,2,2,2,2,2,2,2,2,2,2,2,2,2,2,2,2,2,2,2,2,2,2,2,2,2,2,2,2,2,2,2,2,
2,2,2,2,2,2,2,2,2,2,2,2,2,2,2,2,2,2,2,2,2,4),(-4.02494338810148,-4.02193033969876,
-3.93992493724719,-3.90898528817333,-3.88701568625783,-3.87674877851422,
-3.86867619689505,-3.85953432808841,-3.84394574206266,-3.77645666986379,
-3.73831257456779,-3.7176502615311,-3.710629551744,-3.70590583610625,-3.70087859080669,
-3.69222160968196,-3.643742635999,-3.60482700916446,-3.56046904788309,-3.54766406691828,
-3.53922113783566,-3.53107721596669,-3.52124854456094,-3.49689370347662,
-3.41231019774439,-3.39212798293188,-3.37846348207257,-3.37249735705626,
-3.36800653077206,-3.36261445928767,-3.35229640830421,-3.27786616873493,
-3.24206093108382,-3.2179332598802,-3.20742999625514,-3.1994619848219,-3.19073705975483,
-3.17624657194768,-3.09373918090561,-3.0467226990626,-3.03822771032295,
-3.03328531554629,-3.02873160499058,-3.02305902147951,-3.0086003235589,
-2.94621901314478,-2.90693705366131,-2.88931455408222,-2.87482004812651,
-2.86604936768864,-2.85800870802107,-2.84754196753151,-2.8242333757087,
-2.73879282065517,-2.7186051338215,-2.70494404426304,-2.69897577112925,
-2.6944722943758,-2.6890391924984,-2.67861256474836,-2.62251078304219,-2.57499960297815,
-2.54621023157496,-2.53499083918056,-2.52687249649355,-2.51936057425587,
-2.50690999221778,-2.4695974098945,-2.39985326444936,-2.37200580601915,
-2.36438676671624,-2.35961144442308,-2.35542554360662,-2.34842693245584,
-2.32886154200221,-2.27072975957472,-2.21429030497882,-2.20088224133076,
-2.1923506436553,-2.18424566655486,-2.17306335946067,-2.1462659572014,-2.06490482925812,
-2.04500240947859,-2.03148397396127,-2.02555345366618,-2.0210642215966,
-2.01563046295169,-2.01551729291411),.UNSPECIFIED.);
#2125=B_SPLINE_CURVE_WITH_KNOTS('',3,(#36205,#36206,#36207,#36208,#36209,
#36210,#36211,#36212,#36213,#36214,#36215,#36216,#36217,#36218,#36219,#36220,
#36221,#36222,#36223,#36224,#36225,#36226,#36227,#36228,#36229,#36230,#36231,
#36232,#36233,#36234,#36235,#36236,#36237,#36238,#36239,#36240,#36241,#36242,
#36243,#36244,#36245,#36246,#36247,#36248,#36249,#36250,#36251,#36252,#36253,
#36254,#36255,#36256,#36257,#36258,#36259,#36260,#36261,#36262,#36263,#36264,
#36265,#36266,#36267,#36268,#36269,#36270,#36271,#36272,#36273,#36274,#36275,
#36276,#36277,#36278,#36279,#36280,#36281,#36282,#36283,#36284,#36285,#36286,
#36287,#36288,#36289,#36290,#36291,#36292,#36293,#36294,#36295,#36296,#36297,
#36298,#36299,#36300,#36301,#36302,#36303,#36304,#36305,#36306,#36307,#36308,
#36309,#36310,#36311,#36312,#36313,#36314,#36315,#36316,#36317,#36318,#36319,
#36320,#36321,#36322,#36323,#36324,#36325,#36326,#36327,#36328,#36329,#36330,
#36331,#36332,#36333,#36334,#36335,#36336,#36337,#36338,#36339,#36340,#36341,
#36342,#36343,#36344,#36345,#36346,#36347,#36348,#36349),.UNSPECIFIED.,
 .F.,.F.,(4,3,3,3,3,3,3,3,3,3,3,3,3,3,3,3,3,3,3,3,3,3,3,3,3,3,3,3,3,3,3,
3,3,3,3,3,3,3,3,3,3,3,3,3,3,3,3,3,4),(74.4826090388022,74.5701171009061,
74.6575762790477,74.7450106693487,74.8324410149635,74.9198880511916,75.0074270886218,
75.0950132990107,75.182740727668,75.2578179239381,75.345779870584,75.4336307723664,
75.521393459374,75.612275189517,75.6999372963985,75.7875855042096,75.8752403136858,
75.9629222251375,76.0506985009842,76.1385309892356,76.2264861090207,76.2484473005182,
76.3362729479242,76.4239892867612,76.5116192868255,76.6025514606096,76.6900863685774,
76.7776096198249,76.8651418461542,76.9527036807354,77.0403641770883,77.1280832577018,
77.215929283375,77.2390766770982,77.3262114351889,77.413235203979,77.500171740674,
77.5913635297995,77.6782069848409,77.7650406065135,77.8518857190326,77.9387636512412,
78.0257484601057,78.1127957290388,78.199980961869,78.2297060536782,78.3409616690792,
78.450436080729,78.5398161890327),.UNSPECIFIED.);
#2126=B_SPLINE_CURVE_WITH_KNOTS('',3,(#36351,#36352,#36353,#36354),
 .UNSPECIFIED.,.F.,.F.,(4,4),(78.5398163397448,79.2203354302582),
 .UNSPECIFIED.);
#2127=B_SPLINE_CURVE_WITH_KNOTS('',3,(#36358,#36359,#36360,#36361,#36362,
#36363,#36364,#36365,#36366,#36367,#36368,#36369,#36370,#36371,#36372,#36373,
#36374,#36375,#36376,#36377,#36378,#36379,#36380,#36381,#36382,#36383,#36384,
#36385,#36386,#36387,#36388,#36389,#36390,#36391,#36392,#36393,#36394,#36395,
#36396,#36397,#36398,#36399,#36400),.UNSPECIFIED.,.F.,.F.,(4,3,3,3,3,3,
3,3,3,3,3,3,3,3,4),(78.5398163399585,78.6513084307211,78.7649921971891,
78.7900351244193,78.8773286503125,78.9645131129572,79.0516120919081,79.1386516146217,
79.2256598993982,79.3126581327151,79.3996674889143,79.4867635448239,79.573902644392,
79.6611829276023,79.7442522065205),.UNSPECIFIED.);
#2128=B_SPLINE_CURVE_WITH_KNOTS('',3,(#36401,#36402,#36403,#36404,#36405,
#36406,#36407,#36408,#36409,#36410,#36411,#36412,#36413,#36414,#36415,#36416,
#36417,#36418,#36419,#36420,#36421,#36422,#36423,#36424,#36425,#36426,#36427,
#36428,#36429,#36430,#36431,#36432,#36433,#36434,#36435,#36436,#36437,#36438,
#36439,#36440,#36441,#36442,#36443,#36444,#36445,#36446,#36447,#36448,#36449,
#36450,#36451,#36452,#36453,#36454,#36455,#36456,#36457,#36458,#36459,#36460,
#36461,#36462,#36463,#36464,#36465,#36466,#36467,#36468,#36469,#36470,#36471,
#36472,#36473,#36474,#36475,#36476,#36477,#36478,#36479,#36480,#36481,#36482,
#36483,#36484,#36485,#36486,#36487,#36488,#36489,#36490,#36491,#36492,#36493,
#36494,#36495,#36496,#36497,#36498,#36499,#36500,#36501,#36502,#36503,#36504,
#36505,#36506,#36507,#36508,#36509,#36510,#36511,#36512,#36513,#36514,#36515,
#36516,#36517,#36518,#36519,#36520,#36521,#36522,#36523,#36524,#36525,#36526,
#36527,#36528,#36529,#36530,#36531,#36532,#36533,#36534,#36535,#36536,#36537,
#36538,#36539,#36540,#36541,#36542,#36543,#36544,#36545,#36546,#36547,#36548),
 .UNSPECIFIED.,.F.,.F.,(4,3,3,3,3,3,3,3,3,3,3,3,3,3,3,3,3,3,3,3,3,3,3,3,
3,3,3,3,3,3,3,3,3,3,3,3,3,3,3,3,3,3,3,3,3,3,3,3,3,4),(74.4816274181351,
74.5692304984992,74.656878603019,74.7446691610334,74.8275176180992,74.9153494983652,
75.003070542925,75.0907037356887,75.1816341430626,75.2691684858901,75.3566897930302,
75.4442187036887,75.5317758574419,75.6194296879387,75.7071409396066,75.7949775033597,
75.8181469946792,75.9059726472772,75.9936876684966,76.0813150465029,76.1722477120974,
76.2597767911498,76.3472930457285,76.4348171195448,76.5223696568421,76.6100192180418,
76.697726397457,76.7855592065891,76.8087763712592,76.8965157262234,76.9841440922057,
77.0716845630408,77.1626497111406,77.25009180658,77.3375211983859,77.4249586234669,
77.5124248194916,77.5999889284807,77.6876110719292,77.7753601050296,77.7994057478392,
77.8864292608986,77.9733147168126,78.0601210604153,78.1468698280841,78.2335825041045,
78.3203028169223,78.4070264415887,78.4938091009427,78.5398163397448),
 .UNSPECIFIED.);
#2129=B_SPLINE_CURVE_WITH_KNOTS('',3,(#36554,#36555,#36556,#36557,#36558,
#36559,#36560,#36561,#36562,#36563,#36564,#36565,#36566,#36567,#36568,#36569,
#36570,#36571,#36572,#36573,#36574,#36575,#36576,#36577,#36578,#36579,#36580,
#36581,#36582,#36583,#36584,#36585,#36586,#36587,#36588,#36589,#36590,#36591,
#36592,#36593,#36594,#36595,#36596,#36597,#36598,#36599,#36600,#36601,#36602,
#36603,#36604,#36605,#36606,#36607,#36608,#36609,#36610,#36611,#36612,#36613,
#36614,#36615,#36616,#36617,#36618,#36619,#36620,#36621,#36622,#36623,#36624,
#36625,#36626,#36627,#36628,#36629,#36630,#36631,#36632,#36633,#36634,#36635,
#36636,#36637,#36638,#36639,#36640,#36641,#36642,#36643,#36644,#36645,#36646,
#36647,#36648,#36649,#36650,#36651,#36652,#36653,#36654,#36655,#36656,#36657,
#36658,#36659,#36660,#36661,#36662,#36663,#36664,#36665,#36666,#36667,#36668,
#36669,#36670,#36671,#36672,#36673,#36674,#36675,#36676,#36677,#36678,#36679,
#36680,#36681,#36682,#36683,#36684,#36685,#36686,#36687,#36688,#36689,#36690,
#36691,#36692,#36693,#36694,#36695,#36696,#36697,#36698,#36699,#36700,#36701),
 .UNSPECIFIED.,.F.,.F.,(4,3,3,3,3,3,3,3,3,3,3,3,3,3,3,3,3,3,3,3,3,3,3,3,
3,3,3,3,3,3,3,3,3,3,3,3,3,3,3,3,3,3,3,3,3,3,3,3,3,4),(68.1983639794465,
68.2861814082633,68.3234122878779,68.4112289338761,68.498934783569,68.5865528382251,
68.6774889415042,68.7650083820866,68.8525148993902,68.9400291482807,69.0275717840982,
69.1152113816981,69.2029085498004,69.2907313551699,69.314041664458,69.4018606979925,
69.4895689306246,69.5771893608844,69.6681245709036,69.7556463539722,69.8431551975548,
69.9306717540522,70.0182166763247,70.1058585176953,70.1935579073452,70.2813828848927,
70.304671041038,70.3924904070348,70.4801989962389,70.5678198064247,70.6587548828238,
70.7462771009769,70.8337863991138,70.9213034290419,71.0088488430415,71.0964912005166,
71.1841911210527,71.2720166468968,71.295300417618,71.3826886130108,71.4699662357104,
71.5571567828598,71.6445910640475,71.7316868152726,71.8187708963969,71.9058644037372,
71.9935560608934,72.0807764862596,72.1687037593107,72.2566310323619),
 .UNSPECIFIED.);
#2130=B_SPLINE_CURVE_WITH_KNOTS('',3,(#36702,#36703,#36704,#36705,#36706,
#36707,#36708,#36709,#36710,#36711,#36712,#36713,#36714,#36715,#36716,#36717,
#36718,#36719,#36720,#36721,#36722,#36723,#36724,#36725,#36726,#36727,#36728,
#36729,#36730,#36731,#36732,#36733,#36734,#36735,#36736,#36737,#36738,#36739,
#36740,#36741,#36742,#36743,#36744,#36745,#36746,#36747,#36748,#36749,#36750,
#36751,#36752,#36753,#36754,#36755,#36756,#36757,#36758,#36759,#36760,#36761,
#36762,#36763,#36764,#36765,#36766,#36767,#36768,#36769,#36770,#36771,#36772,
#36773,#36774,#36775,#36776,#36777,#36778,#36779,#36780,#36781,#36782,#36783,
#36784,#36785,#36786),.UNSPECIFIED.,.F.,.F.,(4,3,3,3,3,3,3,3,3,3,3,3,3,
3,3,3,3,3,3,3,3,3,3,3,3,3,3,3,4),(72.2566310325652,72.285929794198,72.3737616617343,
72.46148269366,72.5491158738982,72.6400462860082,72.7275806166556,72.8151019117628,
72.9026308105475,72.9901879525983,73.0778417717025,73.1655530121446,73.2533895649997,
73.2765591707781,73.3643847775249,73.4520997526408,73.5397270843495,73.6306597672255,
73.7181887997928,73.8057050078983,73.8932290353041,73.9807815263042,74.0684310416082,
74.1561381753079,74.2439709393373,74.2671885473581,74.3549358526297,74.4425595257674,
74.4826090388022),.UNSPECIFIED.);
#2131=B_SPLINE_CURVE_WITH_KNOTS('',3,(#36788,#36789,#36790,#36791,#36792,
#36793,#36794,#36795,#36796,#36797,#36798,#36799,#36800,#36801,#36802,#36803,
#36804,#36805,#36806,#36807,#36808,#36809,#36810,#36811,#36812,#36813,#36814,
#36815,#36816,#36817,#36818,#36819,#36820,#36821,#36822,#36823,#36824,#36825,
#36826,#36827,#36828,#36829,#36830,#36831,#36832,#36833,#36834,#36835,#36836,
#36837,#36838,#36839,#36840,#36841,#36842,#36843,#36844,#36845,#36846,#36847,
#36848,#36849,#36850,#36851,#36852,#36853,#36854,#36855,#36856,#36857,#36858,
#36859,#36860,#36861,#36862,#36863,#36864,#36865,#36866,#36867,#36868,#36869),
 .UNSPECIFIED.,.F.,.F.,(4,3,3,3,3,3,3,3,3,3,3,3,3,3,3,3,3,3,3,3,3,3,3,3,
3,3,3,4),(72.2566310325652,72.3454126132022,72.434221928334,72.523077423167,
72.6120589945079,72.701109252016,72.7903164552464,72.8462588649391,72.934078238315,
73.0217868349393,73.1094076525767,73.2003427261945,73.2878649518309,73.3753742574496,
73.4628912948501,73.5504367163045,73.6380790811704,73.7257790090688,73.8136045421773,
73.8368882415191,73.9246814727248,74.0123709463197,74.0999775010394,74.1875219079629,
74.2750312327159,74.362520448007,74.4500269610276,74.4816274181351),
 .UNSPECIFIED.);
#2132=B_SPLINE_CURVE_WITH_KNOTS('',3,(#36870,#36871,#36872,#36873,#36874,
#36875,#36876,#36877,#36878,#36879,#36880,#36881,#36882,#36883,#36884,#36885,
#36886,#36887,#36888,#36889,#36890,#36891,#36892,#36893,#36894,#36895,#36896,
#36897,#36898,#36899,#36900,#36901,#36902,#36903,#36904,#36905,#36906,#36907,
#36908,#36909,#36910,#36911,#36912,#36913,#36914,#36915,#36916,#36917,#36918,
#36919,#36920,#36921,#36922,#36923,#36924,#36925,#36926,#36927,#36928,#36929,
#36930,#36931,#36932,#36933,#36934,#36935,#36936,#36937,#36938,#36939,#36940,
#36941,#36942,#36943,#36944,#36945,#36946,#36947,#36948,#36949,#36950,#36951,
#36952,#36953,#36954,#36955,#36956,#36957,#36958,#36959,#36960,#36961,#36962,
#36963,#36964,#36965,#36966,#36967,#36968,#36969,#36970,#36971,#36972,#36973,
#36974,#36975,#36976,#36977,#36978,#36979,#36980,#36981,#36982,#36983,#36984,
#36985,#36986,#36987,#36988,#36989,#36990,#36991,#36992,#36993,#36994,#36995,
#36996,#36997,#36998,#36999,#37000,#37001,#37002,#37003,#37004,#37005,#37006,
#37007,#37008,#37009,#37010,#37011,#37012,#37013,#37014,#37015,#37016,#37017),
 .UNSPECIFIED.,.F.,.F.,(4,3,3,3,3,3,3,3,3,3,3,3,3,3,3,3,3,3,3,3,3,3,3,3,
3,3,3,3,3,3,3,3,3,3,3,3,3,3,3,3,3,3,3,3,3,3,3,3,3,4),(68.1993401972453,
68.2868763896218,68.3743883605345,68.4618967697717,68.549422269573,68.6370391947937,
68.7247035314655,68.8125067582073,68.883741358619,68.9715591937461,69.0592662329932,
69.1468854762243,69.2378211335961,69.3253417528177,69.4128494430728,69.5003648579722,
69.5879086515959,69.675549389072,69.7632476879449,69.851071602163,69.874370735199,
69.9621887251155,70.0498959219278,70.1375153252757,70.2284509235886,70.3159717082027,
70.4034795654982,70.4909951488949,70.5785391122832,70.6661800205218,70.7538784909369,
70.8417025765127,70.8650001117791,70.9528167547558,71.0405226014255,71.1281406530599,
71.2190767574723,71.3065961950559,71.3941027093744,71.4816169552964,71.569159588166,
71.6567991828616,71.7444963480818,71.8323191506235,71.8556294883591,71.9558798743633,
72.0526975236685,72.1492455697667,72.2453959180088,72.2566310323761),
 .UNSPECIFIED.);
#2133=B_SPLINE_CURVE_WITH_KNOTS('',3,(#37023,#37024,#37025,#37026,#37027,
#37028,#37029,#37030,#37031,#37032,#37033,#37034,#37035,#37036,#37037,#37038,
#37039,#37040,#37041,#37042,#37043,#37044,#37045,#37046,#37047,#37048,#37049,
#37050,#37051,#37052,#37053,#37054,#37055,#37056,#37057,#37058,#37059,#37060,
#37061,#37062,#37063,#37064,#37065,#37066,#37067,#37068,#37069,#37070,#37071,
#37072,#37073,#37074,#37075,#37076,#37077,#37078,#37079,#37080,#37081,#37082,
#37083,#37084,#37085,#37086,#37087,#37088,#37089,#37090,#37091,#37092,#37093,
#37094,#37095,#37096,#37097,#37098,#37099,#37100,#37101,#37102,#37103,#37104,
#37105,#37106,#37107,#37108,#37109,#37110,#37111,#37112,#37113,#37114,#37115,
#37116,#37117,#37118,#37119,#37120,#37121,#37122,#37123,#37124,#37125,#37126,
#37127,#37128,#37129,#37130,#37131,#37132,#37133,#37134,#37135,#37136,#37137,
#37138,#37139,#37140,#37141,#37142,#37143,#37144,#37145,#37146,#37147,#37148,
#37149,#37150,#37151,#37152,#37153,#37154,#37155,#37156,#37157,#37158,#37159,
#37160,#37161,#37162,#37163,#37164,#37165,#37166,#37167,#37168,#37169,#37170),
 .UNSPECIFIED.,.F.,.F.,(4,3,3,3,3,3,3,3,3,3,3,3,3,3,3,3,3,3,3,3,3,3,3,3,
3,3,3,3,3,3,3,3,3,3,3,3,3,3,3,3,3,3,3,3,3,3,3,3,3,4),(61.9155759128088,
62.0030907136044,62.0906332953162,62.178272546237,62.2659688209867,62.3537913858594,
62.3796360283978,62.4674537388885,62.5551606542796,62.6427797745698,62.7337154783708,
62.8212359776857,62.9087435493546,62.9962588471121,63.083802525162,63.1714431499544,
63.2591413376945,63.346965143887,63.3702654049778,63.458083136711,63.5457900732432,
63.6334092145493,63.7243449104253,63.8118654303149,63.8993730223614,63.9868883402774,
64.0744320382452,64.1620726825017,64.2497708894643,64.3375947143806,64.3608947815578,
64.4487125432784,64.5364195101062,64.6240386819771,64.7149743664972,64.80249491742,
64.8900025406175,64.9775178897679,65.0650616190193,65.1527022944715,65.2404005326154,
65.3282243884524,65.3515241581378,65.4399938084303,65.528348931963,65.6166094524169,
65.7058185206591,65.7939460925293,65.8836959089575,65.9734457253856),
 .UNSPECIFIED.);
#2134=B_SPLINE_CURVE_WITH_KNOTS('',3,(#37171,#37172,#37173,#37174,#37175,
#37176,#37177,#37178,#37179,#37180,#37181,#37182,#37183,#37184,#37185,#37186,
#37187,#37188,#37189,#37190,#37191,#37192,#37193,#37194,#37195,#37196,#37197,
#37198,#37199,#37200,#37201,#37202,#37203,#37204,#37205,#37206,#37207,#37208,
#37209,#37210,#37211,#37212,#37213,#37214,#37215,#37216,#37217,#37218,#37219,
#37220,#37221,#37222,#37223,#37224,#37225,#37226,#37227,#37228,#37229,#37230,
#37231,#37232,#37233,#37234,#37235,#37236,#37237,#37238,#37239,#37240,#37241,
#37242,#37243,#37244,#37245,#37246,#37247,#37248,#37249),.UNSPECIFIED.,
 .F.,.F.,(4,3,3,3,3,3,3,3,3,3,3,3,3,3,3,3,3,3,3,3,3,3,3,3,3,3,4),(65.9734457255974,
66.0719666577997,66.1708766451026,66.270310369695,66.3421535347179,66.4299713696735,
66.5176784087517,66.6052976518168,66.6962333092519,66.7837539283157,66.8712616184165,
66.9587770331652,67.0463208266417,67.1339615639766,67.2216598627118,67.3094837767978,
67.3327829112979,67.4206084663604,67.5083214321086,67.5959318428673,67.6834846155375,
67.7710004509517,67.8585000180416,67.9460405103184,68.0335997133571,68.1212547539381,
68.1983639794465),.UNSPECIFIED.);
#2135=B_SPLINE_CURVE_WITH_KNOTS('',3,(#37251,#37252,#37253,#37254,#37255,
#37256,#37257,#37258,#37259,#37260,#37261,#37262,#37263,#37264,#37265,#37266,
#37267,#37268,#37269,#37270,#37271,#37272,#37273,#37274,#37275,#37276,#37277,
#37278,#37279,#37280,#37281,#37282,#37283,#37284,#37285,#37286,#37287,#37288,
#37289,#37290,#37291,#37292,#37293,#37294,#37295,#37296,#37297,#37298,#37299,
#37300,#37301,#37302,#37303,#37304,#37305,#37306,#37307,#37308,#37309,#37310,
#37311,#37312,#37313,#37314,#37315,#37316,#37317,#37318,#37319,#37320,#37321,
#37322,#37323,#37324,#37325,#37326,#37327,#37328,#37329,#37330,#37331,#37332),
 .UNSPECIFIED.,.F.,.F.,(4,3,3,3,3,3,3,3,3,3,3,3,3,3,3,3,3,3,3,3,3,3,3,3,
3,3,3,4),(65.9734457255662,66.0604573171659,66.1473630253195,66.2341866877546,
66.3209558483189,66.4076973522153,66.4944326209674,66.581183066942,66.6680217727115,
66.7549076097825,66.8419276275553,66.9024826054589,66.9903003673624,67.0780073343742,
67.1656265064294,67.2565621908806,67.3440827419878,67.4315903653695,67.5191057147038,
67.6066494441382,67.6942901197717,67.781988358096,67.8698122141105,67.893111982039,
67.9809173627593,68.0686254652694,68.1562390279435,68.1993401972453),
 .UNSPECIFIED.);
#2136=B_SPLINE_CURVE_WITH_KNOTS('',3,(#37333,#37334,#37335,#37336,#37337,
#37338,#37339,#37340,#37341,#37342,#37343,#37344,#37345,#37346,#37347,#37348,
#37349,#37350,#37351,#37352,#37353,#37354,#37355,#37356,#37357,#37358,#37359,
#37360,#37361,#37362,#37363,#37364,#37365,#37366,#37367,#37368,#37369,#37370,
#37371,#37372,#37373,#37374,#37375,#37376,#37377,#37378,#37379,#37380,#37381,
#37382,#37383,#37384,#37385,#37386,#37387,#37388,#37389,#37390,#37391,#37392,
#37393,#37394,#37395,#37396,#37397,#37398,#37399,#37400,#37401,#37402,#37403,
#37404,#37405,#37406,#37407,#37408,#37409,#37410,#37411,#37412,#37413,#37414,
#37415,#37416,#37417,#37418,#37419,#37420,#37421,#37422,#37423,#37424,#37425,
#37426,#37427,#37428,#37429,#37430,#37431,#37432,#37433,#37434,#37435,#37436,
#37437,#37438,#37439,#37440,#37441,#37442,#37443,#37444,#37445,#37446,#37447,
#37448,#37449,#37450,#37451,#37452,#37453,#37454,#37455,#37456,#37457,#37458,
#37459,#37460,#37461,#37462,#37463,#37464,#37465,#37466,#37467,#37468,#37469,
#37470,#37471,#37472,#37473,#37474,#37475,#37476,#37477,#37478,#37479,#37480,
#37481,#37482,#37483),.UNSPECIFIED.,.F.,.F.,(4,3,3,3,3,3,3,3,3,3,3,3,3,
3,3,3,3,3,3,3,3,3,3,3,3,3,3,3,3,3,3,3,3,3,3,3,3,3,3,3,3,3,3,3,3,3,3,3,3,
3,4),(61.9154863939113,61.9493357225588,62.0371534448221,62.1248603719843,
62.21247950403,62.3034152034186,62.3909357143763,62.4784432976267,62.5659586068916,
62.6535022963624,62.7411429323911,62.828841131273,62.9166649483845,62.9399650991388,
63.0277828231757,63.115489752098,63.2031088858884,63.2940445846172,63.3815650972706,
63.4690726821958,63.5565879931129,63.6441316842115,63.731772321824,63.8194705222658,
63.9072943408907,63.9305944757189,64.0184122044976,64.1061191381951,64.1937382767883,
64.2846739737272,64.3721944912207,64.4597020809913,64.5472173967536,64.6347610926922,
64.7224017351121,64.8100999403481,64.8979237637111,64.9212238522989,65.0090415627361,
65.096748478074,65.184367598311,65.275303302132,65.3628238013942,65.4503313730109,
65.5378466707163,65.6253903487142,65.7130309734558,65.8007291611456,65.8885529672889,
65.9118532288789,65.9734457253856),.UNSPECIFIED.);
#2137=B_SPLINE_CURVE_WITH_KNOTS('',3,(#37489,#37490,#37491,#37492,#37493,
#37494,#37495,#37496,#37497,#37498,#37499,#37500,#37501,#37502,#37503,#37504,
#37505,#37506,#37507,#37508,#37509,#37510,#37511,#37512,#37513,#37514,#37515,
#37516,#37517,#37518,#37519,#37520,#37521,#37522,#37523,#37524,#37525,#37526,
#37527,#37528,#37529,#37530,#37531,#37532,#37533,#37534,#37535,#37536,#37537,
#37538,#37539,#37540,#37541,#37542,#37543,#37544,#37545,#37546,#37547,#37548,
#37549,#37550,#37551,#37552,#37553,#37554,#37555,#37556,#37557,#37558,#37559,
#37560,#37561,#37562,#37563,#37564,#37565,#37566,#37567,#37568,#37569,#37570,
#37571,#37572,#37573,#37574,#37575,#37576,#37577,#37578,#37579,#37580,#37581,
#37582,#37583,#37584,#37585,#37586,#37587,#37588,#37589,#37590,#37591,#37592,
#37593,#37594,#37595,#37596,#37597,#37598,#37599,#37600,#37601,#37602,#37603,
#37604,#37605,#37606,#37607,#37608,#37609,#37610,#37611,#37612,#37613,#37614,
#37615,#37616,#37617,#37618,#37619,#37620,#37621,#37622,#37623,#37624,#37625,
#37626,#37627,#37628,#37629,#37630,#37631,#37632,#37633,#37634,#37635,#37636),
 .UNSPECIFIED.,.F.,.F.,(4,3,3,3,3,3,3,3,3,3,3,3,3,3,3,3,3,3,3,3,3,3,3,3,
3,3,3,3,3,3,3,3,3,3,3,3,3,3,3,3,3,3,3,3,3,3,3,3,3,4),(55.6330521101367,
55.7206607613694,55.8100606373129,55.8975784490138,55.9850858701811,56.0726035538017,
56.1634176075807,56.2510662065663,56.3387753439269,56.426606455157,56.4358597689176,
56.5236774924359,56.6113844208518,56.6990035541487,56.7899392530673,56.8774597652619,
56.9649673497418,57.0524826602275,57.1400263509091,57.2276669881277,57.3153651881888,
57.4031890064548,57.4264891454976,57.5143068691385,57.6020137976754,57.6896329310915,
57.7805686299647,57.8680891422732,57.9555967268649,58.0431120374601,58.1306557282489,
58.2182963655708,58.3059945657329,58.393818384096,58.4171185220777,58.5049362463856,
58.5926431755931,58.6802623096824,58.7711980083043,58.8587185212883,58.9462261065552,
59.0337414178245,59.1212851092855,59.2089257472737,59.2966239480993,59.3844477671167,
59.4077478986577,59.5162980940516,59.6233575452028,59.6902604180839),
 .UNSPECIFIED.);
#2138=B_SPLINE_CURVE_WITH_KNOTS('',3,(#37637,#37638,#37639,#37640,#37641,
#37642,#37643,#37644,#37645,#37646,#37647,#37648,#37649,#37650,#37651,#37652,
#37653,#37654,#37655,#37656,#37657,#37658,#37659,#37660,#37661,#37662,#37663,
#37664,#37665,#37666,#37667,#37668,#37669,#37670,#37671,#37672,#37673,#37674,
#37675,#37676,#37677,#37678,#37679,#37680,#37681,#37682,#37683,#37684,#37685,
#37686,#37687,#37688,#37689,#37690,#37691,#37692,#37693,#37694,#37695,#37696,
#37697,#37698,#37699,#37700,#37701,#37702,#37703,#37704,#37705,#37706,#37707,
#37708,#37709,#37710,#37711,#37712,#37713,#37714,#37715),.UNSPECIFIED.,
 .F.,.F.,(4,3,3,3,3,3,3,3,3,3,3,3,3,3,3,3,3,3,3,3,3,3,3,3,3,3,4),(59.6902604182061,
59.7787750253351,59.8656202876032,59.9524524305475,60.0392927619938,60.1290638903048,
60.2160327288235,60.3072050020306,60.3983772752377,60.4861949992756,60.5739019281986,
60.6615210619902,60.7524567607187,60.8399772733732,60.9274848582996,61.015000169218,
61.1025438603181,61.190184497932,61.2778826983752,61.3657065170016,61.3890066518177,
61.476820870378,61.5645289188598,61.6522906673471,61.739842506503,61.8277092096559,
61.9155759128088),.UNSPECIFIED.);
#2139=B_SPLINE_CURVE_WITH_KNOTS('',3,(#37717,#37718,#37719,#37720,#37721,
#37722,#37723,#37724,#37725,#37726,#37727,#37728,#37729,#37730,#37731,#37732,
#37733,#37734,#37735,#37736,#37737,#37738,#37739,#37740,#37741,#37742,#37743,
#37744,#37745,#37746,#37747,#37748,#37749,#37750,#37751,#37752,#37753,#37754,
#37755,#37756,#37757,#37758,#37759,#37760,#37761,#37762,#37763,#37764,#37765,
#37766,#37767,#37768,#37769,#37770,#37771,#37772,#37773,#37774,#37775,#37776,
#37777,#37778,#37779,#37780,#37781,#37782,#37783,#37784,#37785,#37786,#37787,
#37788,#37789,#37790,#37791,#37792,#37793,#37794,#37795),.UNSPECIFIED.,
 .F.,.F.,(4,3,3,3,3,3,3,3,3,3,3,3,3,3,3,3,3,3,3,3,3,3,3,3,3,3,4),(59.69026041843,
59.7976956857359,59.9067549033646,59.9680769693988,60.0558946930393,60.1436016215757,
60.2312207549914,60.3221564538648,60.4096769661728,60.4971845507641,60.5846998613588,
60.6722435521473,60.7598841894687,60.8475823896304,60.935406207993,60.9587063459788,
61.0465260468144,61.1342344663927,61.221854606759,61.309409240327,61.3969287920519,
61.4844339306849,61.5719453095809,61.6595334389219,61.7471595669974,61.8349150953326,
61.9154863939113),.UNSPECIFIED.);
#2140=B_SPLINE_CURVE_WITH_KNOTS('',3,(#37796,#37797,#37798,#37799,#37800,
#37801,#37802,#37803,#37804,#37805,#37806,#37807,#37808,#37809,#37810,#37811,
#37812,#37813,#37814,#37815,#37816,#37817,#37818,#37819,#37820,#37821,#37822,
#37823,#37824,#37825,#37826,#37827,#37828,#37829,#37830,#37831,#37832,#37833,
#37834,#37835,#37836,#37837,#37838,#37839,#37840,#37841,#37842,#37843,#37844,
#37845,#37846,#37847,#37848,#37849,#37850,#37851,#37852,#37853,#37854,#37855,
#37856,#37857,#37858,#37859,#37860,#37861,#37862,#37863,#37864,#37865,#37866,
#37867,#37868,#37869,#37870,#37871,#37872,#37873,#37874,#37875,#37876,#37877,
#37878,#37879,#37880,#37881,#37882,#37883,#37884,#37885,#37886,#37887,#37888,
#37889,#37890,#37891,#37892,#37893,#37894,#37895,#37896,#37897,#37898,#37899,
#37900,#37901,#37902,#37903,#37904,#37905,#37906,#37907,#37908,#37909,#37910,
#37911,#37912,#37913,#37914,#37915,#37916,#37917,#37918,#37919,#37920,#37921,
#37922,#37923,#37924,#37925,#37926,#37927,#37928,#37929,#37930,#37931,#37932,
#37933,#37934,#37935,#37936,#37937,#37938,#37939,#37940,#37941,#37942,#37943,
#37944,#37945,#37946),.UNSPECIFIED.,.F.,.F.,(4,3,3,3,3,3,3,3,3,3,3,3,3,
3,3,3,3,3,3,3,3,3,3,3,3,3,3,3,3,3,3,3,3,3,3,3,3,3,3,3,3,3,3,3,3,3,3,3,3,
3,4),(55.6321400172702,55.719683968197,55.8073249295175,55.8950235783074,
55.9828476904339,56.0055594630786,56.0933771867245,56.1810841152678,56.2687032486918,
56.3596389475627,56.4471594598825,56.5346670444869,56.6221823550959,56.7097260458995,
56.7973666832383,56.8850648834183,56.9728887018007,56.9961888396587,57.0840065633094,
57.1717134918572,57.2593326252853,57.3502683241545,57.4377888364782,57.5252964210861,
57.6128117316991,57.7003554225062,57.7879960598478,57.8756942600309,57.9635180784157,
57.9868182162387,58.0746359399782,58.1623428686151,58.2499620021326,58.3408977009683,
58.4284182133814,58.5159257980787,58.6034411087804,58.6909847996761,58.7786254371054,
58.8663236373754,58.954147455846,58.9774475928187,59.0665491959921,59.1535112710729,
59.2403929922443,59.3272158153765,59.4179769660839,59.5047630081795,59.5915521904117,
59.6783867689608,59.6902604182061),.UNSPECIFIED.);
#2141=B_SPLINE_CURVE_WITH_KNOTS('',3,(#37952,#37953,#37954,#37955,#37956,
#37957,#37958,#37959,#37960,#37961,#37962,#37963,#37964,#37965,#37966,#37967,
#37968,#37969,#37970,#37971,#37972,#37973,#37974,#37975,#37976,#37977,#37978,
#37979,#37980,#37981,#37982,#37983,#37984,#37985,#37986,#37987,#37988,#37989,
#37990,#37991,#37992,#37993,#37994,#37995,#37996,#37997,#37998,#37999,#38000,
#38001,#38002,#38003,#38004,#38005,#38006,#38007,#38008,#38009,#38010,#38011,
#38012,#38013,#38014,#38015,#38016,#38017,#38018,#38019,#38020,#38021,#38022,
#38023,#38024,#38025,#38026,#38027,#38028,#38029,#38030,#38031,#38032,#38033,
#38034,#38035,#38036,#38037,#38038,#38039,#38040,#38041,#38042,#38043,#38044,
#38045,#38046,#38047,#38048,#38049,#38050,#38051,#38052,#38053,#38054,#38055,
#38056,#38057,#38058,#38059,#38060,#38061,#38062,#38063,#38064,#38065,#38066,
#38067,#38068,#38069,#38070,#38071,#38072,#38073,#38074,#38075,#38076,#38077,
#38078,#38079,#38080,#38081,#38082,#38083,#38084,#38085,#38086,#38087,#38088,
#38089,#38090,#38091,#38092,#38093,#38094,#38095,#38096,#38097,#38098,#38099),
 .UNSPECIFIED.,.F.,.F.,(4,3,3,3,3,3,3,3,3,3,3,3,3,3,3,3,3,3,3,3,3,3,3,3,
3,3,3,3,3,3,3,3,3,3,3,3,3,3,3,3,3,3,3,3,3,3,3,3,3,4),(49.3487618639327,
49.4365675238893,49.5014541328574,49.5892718565182,49.6769787850764,49.7645979185152,
49.8555336173805,49.943054129715,50.0305617143338,50.1180770249573,50.2056207157754,
50.293261353128,50.3809595533218,50.4687833717175,50.4920835094374,50.5799012330958,
50.6676081616516,50.755227295088,50.8461629939542,50.9336835062863,51.0211910909028,
51.108706401524,51.1962500923399,51.2838907296903,51.3715889298818,51.4594127482754,
51.4827128860175,51.5705306096755,51.6582375382309,51.7458566716667,51.8367923705331,
51.9243128828646,52.0118204674806,52.0993357781011,52.1868794689165,52.2745201062663,
52.3622183064571,52.4500421248501,52.4733422625975,52.5604221705832,52.6473917778918,
52.7342748965889,52.8210968701783,52.90788700504,52.9946666870674,53.0814572896191,
53.1683305096244,53.2552470964566,53.3422944291719,53.4070751108547),
 .UNSPECIFIED.);
#2142=B_SPLINE_CURVE_WITH_KNOTS('',3,(#38100,#38101,#38102,#38103,#38104,
#38105,#38106,#38107,#38108,#38109,#38110,#38111,#38112,#38113,#38114,#38115,
#38116,#38117,#38118,#38119,#38120,#38121,#38122,#38123,#38124,#38125,#38126,
#38127,#38128,#38129,#38130,#38131,#38132,#38133,#38134,#38135,#38136,#38137,
#38138,#38139,#38140,#38141,#38142,#38143,#38144,#38145,#38146,#38147,#38148,
#38149,#38150,#38151,#38152,#38153,#38154,#38155,#38156,#38157,#38158,#38159,
#38160,#38161,#38162,#38163,#38164,#38165,#38166,#38167,#38168,#38169,#38170,
#38171,#38172,#38173,#38174,#38175,#38176,#38177,#38178,#38179,#38180,#38181,
#38182,#38183,#38184),.UNSPECIFIED.,.F.,.F.,(4,3,3,3,3,3,3,3,3,3,3,3,3,
3,3,3,3,3,3,3,3,3,3,3,3,3,3,3,4),(53.4070751110265,53.4639716391775,53.5517893628234,
53.6394962913667,53.7271154247907,53.8180511236615,53.9055716359814,53.9930792205857,
54.0805945311949,54.1681382219988,54.2557788593375,54.3434770595174,54.4313008778997,
54.4546010157575,54.5424187394083,54.6301256679563,54.7177448013847,54.8086805002538,
54.8962010125776,54.9837085971856,55.0712239077982,55.1587675986054,55.2464082359471,
55.3341064361299,55.4219302545147,55.4452303923376,55.5330632331811,55.6207748462539,
55.6330521101367),.UNSPECIFIED.);
#2143=B_SPLINE_CURVE_WITH_KNOTS('',3,(#38186,#38187,#38188,#38189,#38190,
#38191,#38192,#38193,#38194,#38195,#38196,#38197,#38198,#38199,#38200,#38201,
#38202,#38203,#38204,#38205,#38206,#38207,#38208,#38209,#38210,#38211,#38212,
#38213,#38214,#38215,#38216,#38217,#38218,#38219,#38220,#38221,#38222,#38223,
#38224,#38225,#38226,#38227,#38228,#38229,#38230,#38231,#38232,#38233,#38234,
#38235,#38236,#38237,#38238,#38239,#38240,#38241,#38242,#38243,#38244,#38245,
#38246,#38247,#38248,#38249,#38250,#38251,#38252,#38253,#38254,#38255,#38256,
#38257,#38258,#38259,#38260,#38261,#38262,#38263,#38264),.UNSPECIFIED.,
 .F.,.F.,(4,3,3,3,3,3,3,3,3,3,3,3,3,3,3,3,3,3,3,3,3,3,3,3,3,3,4),(53.4070751110265,
53.495269714547,53.5834738756981,53.6717071431048,53.760051289659,53.8484511190451,
53.9370104138986,54.0243007099186,54.1121184335766,54.1998253621318,54.287444495568,
54.3783801944343,54.4659007067658,54.5534082913818,54.6409236020025,54.7284672928177,
54.8161079301674,54.9038061303583,54.991629948751,55.0149300864986,55.1027351464041,
55.1904358985635,55.2780531741872,55.3665748849579,55.4540908007695,55.5431154090198,
55.6321400172702),.UNSPECIFIED.);
#2144=B_SPLINE_CURVE_WITH_KNOTS('',3,(#38265,#38266,#38267,#38268,#38269,
#38270,#38271,#38272,#38273,#38274,#38275,#38276,#38277,#38278,#38279,#38280,
#38281,#38282,#38283,#38284,#38285,#38286,#38287,#38288,#38289,#38290,#38291,
#38292,#38293,#38294,#38295,#38296,#38297,#38298,#38299,#38300,#38301,#38302,
#38303,#38304,#38305,#38306,#38307,#38308,#38309,#38310,#38311,#38312,#38313,
#38314,#38315,#38316,#38317,#38318,#38319,#38320,#38321,#38322,#38323,#38324,
#38325,#38326,#38327,#38328,#38329,#38330,#38331,#38332,#38333,#38334,#38335,
#38336,#38337,#38338,#38339,#38340,#38341,#38342,#38343,#38344,#38345,#38346,
#38347,#38348,#38349,#38350,#38351,#38352,#38353,#38354,#38355,#38356,#38357,
#38358,#38359,#38360,#38361,#38362,#38363,#38364,#38365,#38366,#38367,#38368,
#38369,#38370,#38371,#38372,#38373,#38374,#38375,#38376,#38377,#38378,#38379,
#38380,#38381,#38382,#38383,#38384,#38385,#38386,#38387,#38388,#38389,#38390,
#38391,#38392,#38393,#38394,#38395,#38396,#38397,#38398,#38399,#38400,#38401,
#38402,#38403,#38404,#38405,#38406,#38407,#38408,#38409),.UNSPECIFIED.,
 .F.,.F.,(4,3,3,3,3,3,3,3,3,3,3,3,3,3,3,3,3,3,3,3,3,3,3,3,3,3,3,3,3,3,3,
3,3,3,3,3,3,3,3,3,3,3,3,3,3,3,3,3,4),(49.349825366214,49.438820095887,49.5263372470124,
49.6138446768933,49.7013630383602,49.7914680796698,49.8791179279186,49.9704505657586,
50.0617832035985,50.1496009272581,50.2373078558151,50.3249269892527,50.4158626881185,
50.5033832004516,50.5908907850692,50.6784060956915,50.7659497865088,50.8535904238602,
50.9412886240528,51.0291124424473,51.0524125801785,51.140230303838,51.227937232395,
51.3155563658324,51.4064920646981,51.4940125770313,51.5815201616488,51.669035472271,
51.7565791630885,51.8442198004398,51.931918000632,52.0197418190264,52.0430419567585,
52.1308596804193,52.2185666089775,52.3061857424157,52.3971214412811,52.4846419536155,
52.5721495382344,52.6596648488578,52.7472085396758,52.8348491770283,52.9225473772215,
53.010371195617,53.0336713333386,53.132711821959,53.2314411214127,53.3295918555023,
53.4070751108162),.UNSPECIFIED.);
#2145=B_SPLINE_CURVE_WITH_KNOTS('',3,(#38415,#38416,#38417,#38418,#38419,
#38420,#38421,#38422,#38423,#38424,#38425,#38426,#38427,#38428,#38429,#38430,
#38431,#38432,#38433,#38434,#38435,#38436,#38437,#38438,#38439,#38440,#38441,
#38442,#38443,#38444,#38445,#38446,#38447,#38448,#38449,#38450,#38451,#38452,
#38453,#38454,#38455,#38456,#38457,#38458,#38459,#38460,#38461,#38462,#38463,
#38464,#38465,#38466,#38467,#38468,#38469,#38470,#38471,#38472,#38473,#38474,
#38475,#38476,#38477,#38478,#38479,#38480,#38481,#38482,#38483,#38484,#38485,
#38486,#38487,#38488,#38489,#38490,#38491,#38492,#38493,#38494,#38495,#38496,
#38497,#38498,#38499,#38500,#38501,#38502,#38503,#38504,#38505,#38506,#38507,
#38508,#38509,#38510,#38511,#38512,#38513,#38514,#38515,#38516,#38517,#38518,
#38519,#38520,#38521,#38522,#38523,#38524,#38525,#38526,#38527,#38528,#38529,
#38530,#38531,#38532,#38533,#38534,#38535,#38536,#38537,#38538,#38539,#38540,
#38541,#38542,#38543,#38544,#38545,#38546,#38547,#38548,#38549,#38550,#38551,
#38552,#38553,#38554,#38555,#38556,#38557,#38558,#38559,#38560,#38561,#38562),
 .UNSPECIFIED.,.F.,.F.,(4,3,3,3,3,3,3,3,3,3,3,3,3,3,3,3,3,3,3,3,3,3,3,3,
3,3,3,3,3,3,3,3,3,3,3,3,3,3,3,3,3,3,3,3,3,3,3,3,3,4),(43.0661023071267,
43.1536126359731,43.2411442504889,43.3287694148403,43.4164457620375,43.5042559154041,
43.5576778733773,43.6454955970373,43.7332025255947,43.8208216590325,43.9117573578981,
43.9992778702315,44.0867854548494,44.1743007654717,44.2618444562881,44.3494850936399,
44.4371832938329,44.5250071122277,44.5483072499573,44.6361249736169,44.7238319021739,
44.8114510356114,44.9023867344772,44.9899072468106,45.0774148314281,45.1649301420503,
45.2524738328671,45.3401144702187,45.4278126704115,45.515636488806,45.5389366265373,
45.6267543501971,45.7144612787543,45.8020804121921,45.8930161110578,45.9805366233911,
46.0680442080088,46.155559518631,46.2431032094478,46.3307438467994,46.4184420469919,
46.5062658653866,46.5295660031173,46.6186563250416,46.7076259258581,46.7964937259127,
46.8852637004615,46.9739759768084,47.0626512944777,47.1238898038469),
 .UNSPECIFIED.);
#2146=B_SPLINE_CURVE_WITH_KNOTS('',3,(#38563,#38564,#38565,#38566,#38567,
#38568,#38569,#38570,#38571,#38572,#38573,#38574,#38575,#38576,#38577,#38578,
#38579,#38580,#38581,#38582,#38583,#38584,#38585,#38586,#38587,#38588,#38589,
#38590,#38591,#38592,#38593,#38594,#38595,#38596,#38597,#38598,#38599,#38600,
#38601,#38602,#38603,#38604,#38605,#38606,#38607,#38608,#38609,#38610,#38611,
#38612,#38613,#38614,#38615,#38616,#38617,#38618,#38619,#38620,#38621,#38622,
#38623,#38624,#38625,#38626,#38627,#38628,#38629,#38630,#38631,#38632,#38633,
#38634,#38635,#38636,#38637,#38638,#38639,#38640,#38641),.UNSPECIFIED.,
 .F.,.F.,(4,3,3,3,3,3,3,3,3,3,3,3,3,3,3,3,3,3,3,3,3,3,3,3,3,3,4),(47.123889804041,
47.2229661979551,47.3199017158515,47.4200485477744,47.5201953796974,47.6080131033571,
47.695720031914,47.7833391653516,47.8742748642173,47.9617953765506,48.0493029611683,
48.1368182717905,48.2243619626075,48.312002599959,48.3997008001517,48.4875246185463,
48.5108247562774,48.5986518170984,48.6863658893996,48.7739762520672,48.8615284126721,
48.9490430731682,49.0365409030645,49.1240737168949,49.2116250160511,49.2992578782112,
49.3487618639327),.UNSPECIFIED.);
#2147=B_SPLINE_CURVE_WITH_KNOTS('',3,(#38643,#38644,#38645,#38646,#38647,
#38648,#38649,#38650,#38651,#38652,#38653,#38654,#38655,#38656,#38657,#38658,
#38659,#38660,#38661,#38662,#38663,#38664,#38665,#38666,#38667,#38668,#38669,
#38670,#38671,#38672,#38673,#38674,#38675,#38676,#38677,#38678,#38679,#38680,
#38681,#38682,#38683,#38684,#38685,#38686,#38687,#38688,#38689,#38690,#38691,
#38692,#38693,#38694,#38695,#38696,#38697,#38698,#38699,#38700,#38701,#38702,
#38703,#38704,#38705,#38706,#38707,#38708,#38709,#38710,#38711,#38712,#38713,
#38714,#38715,#38716,#38717,#38718,#38719,#38720,#38721,#38722,#38723,#38724),
 .UNSPECIFIED.,.F.,.F.,(4,3,3,3,3,3,3,3,3,3,3,3,3,3,3,3,3,3,3,3,3,3,3,3,
3,3,3,4),(47.1238898040779,47.2112205230627,47.2984421477902,47.3855782233591,
47.4726547355854,47.5596998923632,47.6467348498431,47.7337807519317,47.8209134726753,
47.9080890145206,47.9954065966316,48.0805244504384,48.1683421740981,48.2560491026551,
48.3436682360925,48.4346039349582,48.5221244472915,48.6096320319093,48.6971473425316,
48.7846910333487,48.8723316707002,48.960029870893,49.0478536892879,49.0711538270185,
49.1589647615704,49.2466781854555,49.3342970290918,49.349825366214),
 .UNSPECIFIED.);
#2148=B_SPLINE_CURVE_WITH_KNOTS('',3,(#38725,#38726,#38727,#38728,#38729,
#38730,#38731,#38732,#38733,#38734,#38735,#38736,#38737,#38738,#38739,#38740,
#38741,#38742,#38743,#38744,#38745,#38746,#38747,#38748,#38749,#38750,#38751,
#38752,#38753,#38754,#38755,#38756,#38757,#38758,#38759,#38760,#38761,#38762,
#38763,#38764,#38765,#38766,#38767,#38768,#38769,#38770,#38771,#38772,#38773,
#38774,#38775,#38776,#38777,#38778,#38779,#38780,#38781,#38782,#38783,#38784,
#38785,#38786,#38787,#38788,#38789,#38790,#38791,#38792,#38793,#38794,#38795,
#38796,#38797,#38798,#38799,#38800,#38801,#38802,#38803,#38804,#38805,#38806,
#38807,#38808,#38809,#38810,#38811,#38812,#38813,#38814,#38815,#38816,#38817,
#38818,#38819,#38820,#38821,#38822,#38823,#38824,#38825,#38826,#38827,#38828,
#38829,#38830,#38831,#38832,#38833,#38834,#38835,#38836,#38837,#38838,#38839,
#38840,#38841,#38842,#38843,#38844,#38845,#38846,#38847,#38848,#38849,#38850,
#38851,#38852,#38853,#38854,#38855,#38856,#38857,#38858,#38859,#38860,#38861,
#38862,#38863,#38864,#38865,#38866,#38867,#38868,#38869,#38870,#38871,#38872,
#38873,#38874,#38875),.UNSPECIFIED.,.F.,.F.,(4,3,3,3,3,3,3,3,3,3,3,3,3,
3,3,3,3,3,3,3,3,3,3,3,3,3,3,3,3,3,3,3,3,3,3,3,3,3,3,3,3,3,3,3,3,3,3,3,3,
3,4),(43.065809626773,43.1273775675383,43.215195291199,43.3029022197571,
43.3905213531958,43.4814570520611,43.5689775643955,43.6564851490144,43.7440004596378,
43.8315441504559,43.9191847878086,44.0068829880024,44.0947068063982,44.1180069441183,
44.2058246677778,44.2935315963346,44.381150729772,44.4720864286378,44.5596069409709,
44.6471145255884,44.7346298362105,44.8221735270273,44.9098141643786,44.9975123645711,
45.0853361829655,45.1086363206983,45.1964540443579,45.2841609729149,45.3717801063525,
45.4627158052182,45.5502363175514,45.637743902169,45.7252592127913,45.8128029036082,
45.9004435409597,45.9881417411522,46.0759655595468,46.0992656972784,46.1870834209383,
46.2747903494955,46.3624094829334,46.453345181799,46.5408656941325,46.6283732787504,
46.715888589373,46.8034322801902,46.8910729175419,46.9787711177347,47.0665949361295,
47.0898950738584,47.1238898038469),.UNSPECIFIED.);
#2149=B_SPLINE_CURVE_WITH_KNOTS('',3,(#38881,#38882,#38883,#38884,#38885,
#38886,#38887,#38888,#38889,#38890,#38891,#38892,#38893,#38894,#38895,#38896,
#38897,#38898,#38899,#38900,#38901,#38902,#38903,#38904,#38905,#38906,#38907,
#38908,#38909,#38910,#38911,#38912,#38913,#38914,#38915,#38916,#38917,#38918,
#38919,#38920,#38921,#38922,#38923,#38924,#38925,#38926,#38927,#38928,#38929,
#38930,#38931,#38932,#38933,#38934,#38935,#38936,#38937,#38938,#38939,#38940,
#38941,#38942,#38943,#38944,#38945,#38946,#38947,#38948,#38949,#38950,#38951,
#38952,#38953,#38954,#38955,#38956,#38957,#38958,#38959,#38960,#38961,#38962,
#38963,#38964,#38965,#38966,#38967,#38968,#38969,#38970,#38971,#38972,#38973,
#38974,#38975,#38976,#38977,#38978,#38979,#38980,#38981,#38982,#38983,#38984,
#38985,#38986,#38987,#38988,#38989,#38990,#38991,#38992,#38993,#38994,#38995,
#38996,#38997,#38998,#38999,#39000,#39001,#39002,#39003,#39004,#39005,#39006,
#39007,#39008,#39009,#39010,#39011,#39012,#39013,#39014,#39015,#39016,#39017,
#39018,#39019,#39020,#39021,#39022,#39023,#39024,#39025,#39026,#39027,#39028),
 .UNSPECIFIED.,.F.,.F.,(4,3,3,3,3,3,3,3,3,3,3,3,3,3,3,3,3,3,3,3,3,3,3,3,
3,3,3,3,3,3,3,3,3,3,3,3,3,3,3,3,3,3,3,3,3,3,3,3,3,4),(36.7834743460371,
36.8711071696441,36.9586711146396,37.0461970608729,37.1337056705273,37.2212175991222,
37.3087534995119,37.3963842651212,37.4840686289141,37.571883639047,37.6139016138971,
37.7017193375656,37.7894262661317,37.8770453995784,37.9679810984408,38.0555016107834,
38.1430091954105,38.2305245060422,38.3180681968687,38.4057088342297,38.4934070344319,
38.581230852836,38.6045309904771,38.6923487141351,38.7800556426905,38.8676747761264,
38.9586104749927,39.0461309873243,39.1336385719403,39.2211538825609,39.3086975733762,
39.396338210726,39.484036410917,39.57186022931,39.5951603670571,39.6829780907157,
39.7706850192716,39.8583041527081,39.9492398515742,40.0367603639064,40.1242679485229,
40.211783259144,40.2993269499597,40.38696758731,40.4746657875014,40.5624896058948,
40.5857897436372,40.6987530453519,40.8096059142798,40.8407044964449),
 .UNSPECIFIED.);
#2150=B_SPLINE_CURVE_WITH_KNOTS('',3,(#39029,#39030,#39031,#39032,#39033,
#39034,#39035,#39036,#39037,#39038,#39039,#39040,#39041,#39042,#39043,#39044,
#39045,#39046,#39047,#39048,#39049,#39050,#39051,#39052,#39053,#39054,#39055,
#39056,#39057,#39058,#39059,#39060,#39061,#39062,#39063,#39064,#39065,#39066,
#39067,#39068,#39069,#39070,#39071,#39072,#39073,#39074,#39075,#39076,#39077,
#39078,#39079,#39080,#39081,#39082,#39083,#39084,#39085,#39086,#39087,#39088,
#39089,#39090,#39091,#39092,#39093,#39094,#39095,#39096,#39097,#39098,#39099,
#39100,#39101,#39102,#39103,#39104,#39105,#39106,#39107,#39108,#39109,#39110),
 .UNSPECIFIED.,.F.,.F.,(4,3,3,3,3,3,3,3,3,3,3,3,3,3,3,3,3,3,3,3,3,3,3,3,
3,3,3,4),(40.8407044966673,40.9273584362595,41.0139637234755,41.1005454082163,
41.1871250286611,41.2737241172989,41.3604139263639,41.4471549251205,41.5340255171112,
41.5764191202172,41.6642368438766,41.7519437724335,41.8395629058709,41.9304986047367,
42.0180191170698,42.1055267016874,42.1930420123095,42.2805857031267,42.368226340478,
42.4559245406704,42.5437483590649,42.5670484967972,42.654865790963,42.7425763493764,
42.8301869080235,42.9177390606068,43.0052579703391,43.0661023071267),
 .UNSPECIFIED.);
#2151=B_SPLINE_CURVE_WITH_KNOTS('',3,(#39112,#39113,#39114,#39115,#39116,
#39117,#39118,#39119,#39120,#39121,#39122,#39123,#39124,#39125,#39126,#39127,
#39128,#39129,#39130,#39131,#39132,#39133,#39134,#39135,#39136,#39137,#39138,
#39139,#39140,#39141,#39142,#39143,#39144,#39145,#39146,#39147,#39148,#39149,
#39150,#39151,#39152,#39153,#39154,#39155,#39156,#39157,#39158,#39159,#39160,
#39161,#39162,#39163,#39164,#39165,#39166,#39167,#39168,#39169,#39170,#39171,
#39172,#39173,#39174,#39175,#39176,#39177,#39178,#39179,#39180,#39181,#39182,
#39183,#39184,#39185,#39186,#39187,#39188,#39189,#39190),.UNSPECIFIED.,
 .F.,.F.,(4,3,3,3,3,3,3,3,3,3,3,3,3,3,3,3,3,3,3,3,3,3,3,3,3,3,4),(40.8407044968327,
40.9448640922813,41.0502373864982,41.1461188143782,41.233936538036,41.3216434665913,
41.409262600027,41.5001982988934,41.5877188112249,41.6752263958407,41.7627417064611,
41.8502853972763,41.9379260346261,42.0256242348169,42.1134480532097,42.1367481909583,
42.2245695492947,42.3122792282294,42.3999002315174,42.4874540511525,42.5749722257416,
42.6624754241103,42.7499842991578,42.8375628974753,42.925179265463,43.012908479813,
43.065809626773),.UNSPECIFIED.);
#2152=B_SPLINE_CURVE_WITH_KNOTS('',3,(#39191,#39192,#39193,#39194,#39195,
#39196,#39197,#39198,#39199,#39200,#39201,#39202,#39203,#39204,#39205,#39206,
#39207,#39208,#39209,#39210,#39211,#39212,#39213,#39214,#39215,#39216,#39217,
#39218,#39219,#39220,#39221,#39222,#39223,#39224,#39225,#39226,#39227,#39228,
#39229,#39230,#39231,#39232,#39233,#39234,#39235,#39236,#39237,#39238,#39239,
#39240,#39241,#39242,#39243,#39244,#39245,#39246,#39247,#39248,#39249,#39250,
#39251,#39252,#39253,#39254,#39255,#39256,#39257,#39258,#39259,#39260,#39261,
#39262,#39263,#39264,#39265,#39266,#39267,#39268,#39269,#39270,#39271,#39272,
#39273,#39274,#39275,#39276,#39277,#39278,#39279,#39280,#39281,#39282,#39283,
#39284,#39285,#39286,#39287,#39288,#39289,#39290,#39291,#39292,#39293,#39294,
#39295,#39296,#39297,#39298,#39299,#39300,#39301,#39302,#39303,#39304,#39305,
#39306,#39307,#39308,#39309,#39310,#39311,#39312,#39313,#39314,#39315,#39316,
#39317,#39318,#39319,#39320,#39321,#39322,#39323,#39324,#39325,#39326,#39327,
#39328,#39329,#39330,#39331,#39332,#39333,#39334,#39335,#39336,#39337,#39338),
 .UNSPECIFIED.,.F.,.F.,(4,3,3,3,3,3,3,3,3,3,3,3,3,3,3,3,3,3,3,3,3,3,3,3,
3,3,3,3,3,3,3,3,3,3,3,3,3,3,3,3,3,3,3,3,3,3,3,3,3,4),(36.7826549295876,
36.8701876837048,36.95781435167,37.0454928643294,37.1333043100256,37.1836013080581,
37.2714190317937,37.3591259604276,37.4467450939429,37.5376807927798,37.6252013051925,
37.71270888989,37.8002242005926,37.8877678914898,37.9754085289219,38.0631067291953,
38.1509305476702,38.1742306846382,38.2620484082879,38.349755336835,38.4373744702629,
38.5283101691323,38.6158306814557,38.7033382660637,38.7908535766762,38.8783972674836,
38.9660379048257,39.0537361050092,39.1415599233948,39.1648600612182,39.2526777848656,
39.3403847134098,39.4280038468348,39.5189395457052,39.6064600580253,39.6939676426298,
39.7814829532385,39.8690266440419,39.9566672813797,40.0443654815585,40.1321892999391,
40.1554894377982,40.242885923383,40.3301773559143,40.4173849585111,40.5045298834919,
40.5916445938398,40.6787389692797,40.7658659689728,40.8407044966673),
 .UNSPECIFIED.);
#2153=B_SPLINE_CURVE_WITH_KNOTS('',3,(#39344,#39345,#39346,#39347,#39348,
#39349,#39350,#39351,#39352,#39353,#39354,#39355,#39356,#39357,#39358,#39359,
#39360,#39361,#39362,#39363,#39364,#39365,#39366,#39367,#39368,#39369,#39370,
#39371,#39372,#39373,#39374,#39375,#39376,#39377,#39378,#39379,#39380,#39381,
#39382,#39383,#39384,#39385,#39386,#39387,#39388,#39389,#39390,#39391,#39392,
#39393,#39394,#39395,#39396,#39397,#39398,#39399,#39400,#39401,#39402,#39403,
#39404,#39405,#39406,#39407,#39408,#39409,#39410,#39411,#39412,#39413,#39414,
#39415,#39416,#39417,#39418,#39419,#39420,#39421,#39422,#39423,#39424,#39425,
#39426,#39427,#39428,#39429,#39430,#39431,#39432,#39433,#39434,#39435,#39436,
#39437,#39438,#39439,#39440,#39441,#39442,#39443,#39444,#39445,#39446,#39447,
#39448,#39449,#39450,#39451,#39452,#39453,#39454,#39455,#39456,#39457,#39458,
#39459,#39460,#39461,#39462,#39463,#39464,#39465,#39466,#39467,#39468,#39469,
#39470,#39471,#39472,#39473,#39474,#39475,#39476,#39477,#39478,#39479,#39480,
#39481,#39482,#39483,#39484,#39485,#39486,#39487,#39488,#39489,#39490,#39491),
 .UNSPECIFIED.,.F.,.F.,(4,3,3,3,3,3,3,3,3,3,3,3,3,3,3,3,3,3,3,3,3,3,3,3,
3,3,3,3,3,3,3,3,3,3,3,3,3,3,3,3,3,3,3,3,3,3,3,3,3,4),(30.4991791414397,
30.5893375596383,30.6794959778369,30.7673137002237,30.8550206274869,30.9426397596114,
31.0335754589621,31.1210959699427,31.2086035531954,31.2961188624419,31.3836625518737,
31.4713031878329,31.5590013866275,31.6468252036264,31.6701253544169,31.7579430786971,
31.845650007882,31.933269141954,32.0242048405844,32.1117253535643,32.1992329388321,
32.2867482501072,32.3742919415789,32.4619325795848,32.5496307804325,32.637454599478,
32.660754730997,32.7485724546253,32.8362793831521,32.9238985165603,33.0148342154374,
33.1023547277442,33.1898623123364,33.2773776229343,33.364921313728,33.4525619510581,
33.5402601512304,33.6280839696064,33.651384107577,33.7382200973112,33.824945993001,
33.9115858335191,33.9981647381688,34.084712476298,34.1712506300881,34.2578007697322,
34.3444298640565,34.4311037988424,34.5178962961451,34.557519189277),
 .UNSPECIFIED.);
#2154=B_SPLINE_CURVE_WITH_KNOTS('',3,(#39492,#39493,#39494,#39495,#39496,
#39497,#39498,#39499,#39500,#39501,#39502,#39503,#39504,#39505,#39506,#39507,
#39508,#39509,#39510,#39511,#39512,#39513,#39514,#39515,#39516,#39517,#39518,
#39519,#39520,#39521,#39522,#39523,#39524,#39525,#39526,#39527,#39528,#39529,
#39530,#39531,#39532,#39533,#39534,#39535,#39536,#39537,#39538,#39539,#39540,
#39541,#39542,#39543,#39544,#39545,#39546,#39547,#39548,#39549,#39550,#39551,
#39552,#39553,#39554,#39555,#39556,#39557,#39558,#39559,#39560,#39561,#39562,
#39563,#39564,#39565,#39566,#39567,#39568,#39569,#39570,#39571,#39572,#39573),
 .UNSPECIFIED.,.F.,.F.,(4,3,3,3,3,3,3,3,3,3,3,3,3,3,3,3,3,3,3,3,3,3,3,3,
3,3,3,4),(34.5575191894877,34.642013484157,34.7298312078921,34.8175381365255,
34.9051572700406,34.9960929688777,35.0836134812899,35.171121065987,35.2586363766889,
35.3461800675859,35.4338207050176,35.5215189052904,35.6093427237649,35.632642860737,
35.7204605843868,35.8081675129339,35.8957866463617,35.9867223452311,36.0742428575547,
36.1617504421628,36.2492657527756,36.3368094435831,36.4244500809253,36.5121482811088,
36.5999720994945,36.6232722373171,36.7110751645256,36.7834743460371),
 .UNSPECIFIED.);
#2155=B_SPLINE_CURVE_WITH_KNOTS('',3,(#39575,#39576,#39577,#39578,#39579,
#39580,#39581,#39582,#39583,#39584,#39585,#39586,#39587,#39588,#39589,#39590,
#39591,#39592,#39593,#39594,#39595,#39596,#39597,#39598,#39599,#39600,#39601,
#39602,#39603,#39604,#39605,#39606,#39607,#39608,#39609,#39610,#39611,#39612,
#39613,#39614,#39615,#39616,#39617,#39618,#39619,#39620,#39621,#39622,#39623,
#39624,#39625,#39626,#39627,#39628,#39629,#39630,#39631,#39632,#39633,#39634,
#39635,#39636,#39637,#39638,#39639,#39640,#39641,#39642,#39643,#39644,#39645,
#39646,#39647,#39648,#39649,#39650,#39651,#39652,#39653,#39654,#39655,#39656),
 .UNSPECIFIED.,.F.,.F.,(4,3,3,3,3,3,3,3,3,3,3,3,3,3,3,3,3,3,3,3,3,3,3,3,
3,3,3,4),(34.5575191894877,34.6452189793779,34.7329127217085,34.8206207339479,
34.908363338699,34.9962128811091,35.0841246971806,35.1721722031867,35.2023425548981,
35.290160278526,35.3778672070522,35.46548634046,35.5564220393372,35.6439425516434,
35.7314501362353,35.8189654468328,35.9065091376259,35.9941497749554,36.0818479751271,
36.1696717935025,36.1929719314781,36.2807796097185,36.368482414792,36.4561011804981,
36.5436546850546,36.6311690814359,36.7186812679047,36.7826549295876),
 .UNSPECIFIED.);
#2156=B_SPLINE_CURVE_WITH_KNOTS('',3,(#39657,#39658,#39659,#39660,#39661,
#39662,#39663,#39664,#39665,#39666,#39667,#39668,#39669,#39670,#39671,#39672,
#39673,#39674,#39675,#39676,#39677,#39678,#39679,#39680,#39681,#39682,#39683,
#39684,#39685,#39686,#39687,#39688,#39689,#39690,#39691,#39692,#39693,#39694,
#39695,#39696,#39697,#39698,#39699,#39700,#39701,#39702,#39703,#39704,#39705,
#39706,#39707,#39708,#39709,#39710,#39711,#39712,#39713,#39714,#39715,#39716,
#39717,#39718,#39719,#39720,#39721,#39722,#39723,#39724,#39725,#39726,#39727,
#39728,#39729,#39730,#39731,#39732,#39733,#39734,#39735,#39736,#39737,#39738,
#39739,#39740,#39741,#39742,#39743,#39744,#39745,#39746,#39747,#39748,#39749,
#39750,#39751,#39752,#39753,#39754,#39755,#39756,#39757,#39758,#39759,#39760,
#39761,#39762,#39763,#39764,#39765,#39766,#39767,#39768,#39769,#39770,#39771,
#39772,#39773,#39774,#39775,#39776,#39777,#39778,#39779,#39780,#39781,#39782,
#39783,#39784,#39785,#39786,#39787,#39788,#39789,#39790,#39791,#39792,#39793,
#39794,#39795,#39796,#39797,#39798,#39799,#39800,#39801,#39802,#39803,#39804),
 .UNSPECIFIED.,.F.,.F.,(4,3,3,3,3,3,3,3,3,3,3,3,3,3,3,3,3,3,3,3,3,3,3,3,
3,3,3,3,3,3,3,3,3,3,3,3,3,3,3,3,3,3,3,3,3,3,3,3,3,4),(30.5002984457891,
30.5878602511594,30.6753851666878,30.7628935163061,30.8504059551847,30.9379431363765,
31.0255755534935,31.11326226172,31.2010787232516,31.239825048578,31.3276427771878,
31.4153497107485,31.5029688492368,31.5939045462269,31.6814250636965,31.7689326534729,
31.8564479692708,31.9439916652747,32.031632307804,32.119330513175,32.2071543367094,
32.230454425158,32.3182721490478,32.405979077851,32.4935982115503,32.5845339103238,
32.6720544229564,32.7595620078866,32.8470773188349,32.9346210099905,33.0222616476981,
33.1099598482573,33.1977836670317,33.221083801738,33.308901524119,33.3966084513758,
33.4842275834946,33.5751632828475,33.6626837938218,33.7501913770681,33.8377066863083,
33.9252503757335,34.0128910116863,34.1005892104745,34.1884130274668,34.211713178318,
34.3130674744917,34.4140179484278,34.5142334839426,34.5575191892806),
 .UNSPECIFIED.);
#2157=B_SPLINE_CURVE_WITH_KNOTS('',3,(#39810,#39811,#39812,#39813,#39814,
#39815,#39816,#39817,#39818,#39819,#39820,#39821,#39822,#39823,#39824,#39825,
#39826,#39827,#39828,#39829,#39830,#39831,#39832,#39833,#39834,#39835,#39836,
#39837,#39838,#39839,#39840,#39841,#39842,#39843,#39844,#39845,#39846,#39847,
#39848,#39849,#39850,#39851,#39852,#39853,#39854,#39855,#39856,#39857,#39858,
#39859,#39860,#39861,#39862,#39863,#39864,#39865,#39866,#39867,#39868,#39869,
#39870,#39871,#39872,#39873,#39874,#39875,#39876,#39877,#39878,#39879,#39880,
#39881,#39882,#39883,#39884,#39885,#39886,#39887,#39888,#39889,#39890,#39891,
#39892,#39893,#39894,#39895,#39896,#39897,#39898,#39899,#39900,#39901,#39902,
#39903,#39904,#39905,#39906,#39907,#39908,#39909,#39910,#39911,#39912,#39913,
#39914,#39915,#39916,#39917,#39918,#39919,#39920,#39921,#39922,#39923,#39924,
#39925,#39926,#39927,#39928,#39929,#39930,#39931,#39932,#39933,#39934,#39935,
#39936,#39937,#39938,#39939,#39940,#39941,#39942,#39943,#39944,#39945,#39946,
#39947,#39948,#39949,#39950,#39951,#39952,#39953,#39954,#39955,#39956,#39957),
 .UNSPECIFIED.,.F.,.F.,(4,3,3,3,3,3,3,3,3,3,3,3,3,3,3,3,3,3,3,3,3,3,3,3,
3,3,3,3,3,3,3,3,3,3,3,3,3,3,3,3,3,3,3,3,3,3,3,3,3,4),(24.2166288630184,
24.3041368733513,24.3916596764232,24.4792727029618,24.5669310750263,24.6547311942768,
24.7357197183567,24.8235373295578,24.9112441439916,24.9988631617908,25.089798903434,
25.1773192970847,25.2648267621001,25.352341952329,25.4398855220887,25.5275260380041,
25.6152241163975,25.7030478133862,25.7263490949368,25.8141668558993,25.9018738221139,
25.9894929935152,26.0804286782654,26.1679492290807,26.2554568523045,26.3429722016151,
26.4305159311601,26.5181566071029,26.6058548458523,26.6936787024586,26.7169784715168,
26.8047962016812,26.8925031369437,26.9801222772785,27.0710579736308,27.158578493298,
27.2460860853985,27.3336014036452,27.4211451022205,27.5087857474913,27.5964839557064,
27.6843077822142,27.7076078480968,27.7974230850615,27.8871096166733,27.9766849091273,
28.0661443963749,28.1555357322244,28.2448678042523,28.2743338823081),
 .UNSPECIFIED.);
#2158=B_SPLINE_CURVE_WITH_KNOTS('',3,(#39958,#39959,#39960,#39961,#39962,
#39963,#39964,#39965,#39966,#39967,#39968,#39969,#39970,#39971,#39972,#39973,
#39974,#39975,#39976,#39977,#39978,#39979,#39980,#39981,#39982,#39983,#39984,
#39985,#39986,#39987,#39988,#39989,#39990,#39991,#39992,#39993,#39994,#39995,
#39996,#39997,#39998,#39999,#40000,#40001,#40002,#40003,#40004,#40005,#40006,
#40007,#40008,#40009,#40010,#40011,#40012,#40013,#40014,#40015,#40016,#40017,
#40018,#40019,#40020,#40021,#40022,#40023,#40024,#40025,#40026,#40027,#40028,
#40029,#40030,#40031,#40032,#40033,#40034,#40035,#40036,#40037,#40038,#40039),
 .UNSPECIFIED.,.F.,.F.,(4,3,3,3,3,3,3,3,3,3,3,3,3,3,3,3,3,3,3,3,3,3,3,3,
3,3,3,4),(28.2743338824658,28.3691609855058,28.4643913559718,28.5598306988534,
28.6555713105395,28.6982372246768,28.7860549532608,28.8737618867956,28.961381025258,
29.0523167222579,29.1398372397006,29.2273448294501,29.314860145221,29.402403841198,
29.4900444837001,29.5777426890439,29.6655665125512,29.6888666012569,29.7766954671531,
29.8670059264389,29.9546146144252,30.0421651514316,30.1296782391034,30.2171745465378,
30.3047008007868,30.3922458634067,30.4798596305342,30.4991791414397),
 .UNSPECIFIED.);
#2159=B_SPLINE_CURVE_WITH_KNOTS('',3,(#40041,#40042,#40043,#40044,#40045,
#40046,#40047,#40048,#40049,#40050,#40051,#40052,#40053,#40054,#40055,#40056,
#40057,#40058,#40059,#40060,#40061,#40062,#40063,#40064,#40065,#40066,#40067,
#40068,#40069,#40070,#40071,#40072,#40073,#40074,#40075,#40076,#40077,#40078,
#40079,#40080,#40081,#40082,#40083,#40084,#40085,#40086,#40087,#40088,#40089,
#40090,#40091,#40092,#40093,#40094,#40095,#40096,#40097,#40098,#40099,#40100,
#40101,#40102,#40103,#40104,#40105,#40106,#40107,#40108,#40109,#40110,#40111,
#40112,#40113,#40114,#40115,#40116,#40117,#40118,#40119,#40120,#40121,#40122),
 .UNSPECIFIED.,.F.,.F.,(4,3,3,3,3,3,3,3,3,3,3,3,3,3,3,3,3,3,3,3,3,3,3,3,
3,3,3,4),(28.2743338824903,28.3620519963015,28.449659412066,28.5371792512195,
28.6273526317443,28.7147749198788,28.8021846604177,28.8896026158296,28.9770495494742,
29.0645934762563,29.1521957090843,29.2399222133715,29.2585662954179,29.3463840255869,
29.4340909608545,29.5217101011948,29.6126457975452,29.7001663172191,29.7876739093267,
29.8751892275808,29.9627329261642,30.0503735714435,30.1380717796675,30.225895606185,
30.2491956719979,30.3370125939443,30.4247058192211,30.5002984457891),
 .UNSPECIFIED.);
#2160=B_SPLINE_CURVE_WITH_KNOTS('',3,(#40123,#40124,#40125,#40126,#40127,
#40128,#40129,#40130,#40131,#40132,#40133,#40134,#40135,#40136,#40137,#40138,
#40139,#40140,#40141,#40142,#40143,#40144,#40145,#40146,#40147,#40148,#40149,
#40150,#40151,#40152,#40153,#40154,#40155,#40156,#40157,#40158,#40159,#40160,
#40161,#40162,#40163,#40164,#40165,#40166,#40167,#40168,#40169,#40170,#40171,
#40172,#40173,#40174,#40175,#40176,#40177,#40178,#40179,#40180,#40181,#40182,
#40183,#40184,#40185,#40186,#40187,#40188,#40189,#40190,#40191,#40192,#40193,
#40194,#40195,#40196,#40197,#40198,#40199,#40200,#40201,#40202,#40203,#40204,
#40205,#40206,#40207,#40208,#40209,#40210,#40211,#40212,#40213,#40214,#40215,
#40216,#40217,#40218,#40219,#40220,#40221,#40222,#40223,#40224,#40225,#40226,
#40227,#40228,#40229,#40230,#40231,#40232,#40233,#40234,#40235,#40236,#40237,
#40238,#40239,#40240,#40241,#40242,#40243,#40244,#40245,#40246,#40247,#40248,
#40249,#40250,#40251,#40252,#40253,#40254,#40255,#40256,#40257,#40258,#40259,
#40260,#40261,#40262,#40263,#40264,#40265,#40266,#40267,#40268,#40269,#40270,
#40271,#40272,#40273),.UNSPECIFIED.,.F.,.F.,(4,3,3,3,3,3,3,3,3,3,3,3,3,
3,3,3,3,3,3,3,3,3,3,3,3,3,3,3,3,3,3,3,3,3,3,3,3,3,3,3,3,3,3,3,3,3,3,3,3,
3,4),(24.2161577263113,24.3054194125178,24.3932361238663,24.4809420258599,
24.5685601198239,24.6594962034832,24.7470156507643,24.8345221627239,24.9220363942335,
25.0095790006303,25.0972185511234,25.1849156617613,25.2727383949358,25.2960487890978,
25.383866778914,25.471573975645,25.5591933789306,25.650128977274,25.737649761874,
25.8251576191729,25.9126732025909,26.0002171660178,26.0878580743214,26.1755565448169,
26.2633806304946,26.2866781656778,26.3744959848762,26.4622030112343,26.5498222446037,
26.6407579068105,26.7282785237727,26.8157862145775,26.9033016328351,26.9908454326265,
27.0784861804008,27.1661844919903,27.2540084223693,27.2773075422579,27.3651251530745,
27.452831967118,27.5404509845215,27.6313867263111,27.7189071195555,27.8064145841616,
27.8939297739781,27.981473343323,28.0691138588222,28.1568119367978,28.2446356333698,
28.2679369188379,28.2743338823081),.UNSPECIFIED.);
#2161=B_SPLINE_CURVE_WITH_KNOTS('',3,(#40279,#40280,#40281,#40282,#40283,
#40284,#40285,#40286,#40287,#40288,#40289,#40290,#40291,#40292,#40293,#40294,
#40295,#40296,#40297,#40298,#40299,#40300,#40301,#40302,#40303,#40304,#40305,
#40306,#40307,#40308,#40309,#40310,#40311,#40312,#40313,#40314,#40315,#40316,
#40317,#40318,#40319,#40320,#40321,#40322,#40323,#40324,#40325,#40326,#40327,
#40328,#40329,#40330,#40331,#40332,#40333,#40334,#40335,#40336,#40337,#40338,
#40339,#40340,#40341,#40342,#40343,#40344,#40345,#40346,#40347,#40348,#40349,
#40350,#40351,#40352,#40353,#40354,#40355,#40356,#40357,#40358,#40359,#40360),
 .UNSPECIFIED.,.F.,.F.,(4,3,3,3,3,3,3,3,3,3,3,3,3,3,3,3,3,3,3,3,3,3,3,3,
3,3,3,4),(15.7079632679489,15.7948132816696,15.88164133663,15.9684687059855,
16.0553166580006,16.142261568354,16.2292579918144,16.3163972482091,16.3803843998776,
16.468224529064,16.5559526601206,16.6435917732961,16.7345195236913,16.8220568152346,
16.9095799626407,16.9971095978197,17.084666352235,17.1723181077271,17.2600263044656,
17.3478583920922,17.3710137764576,17.4589553673584,17.5467936775551,17.6345493822514,
17.7222396449223,17.8098920264127,17.8975364303658,17.9331346486732),
 .UNSPECIFIED.);
#2162=B_SPLINE_CURVE_WITH_KNOTS('',3,(#40362,#40363,#40364,#40365,#40366),
 .UNSPECIFIED.,.F.,.F.,(4,1,4),(14.3991256467175,15.3897550232975,15.707955107058),
 .UNSPECIFIED.);
#2163=B_SPLINE_CURVE_WITH_KNOTS('',3,(#40370,#40371,#40372,#40373,#40374,
#40375,#40376,#40377,#40378,#40379,#40380,#40381,#40382,#40383,#40384,#40385,
#40386,#40387,#40388,#40389,#40390,#40391,#40392,#40393,#40394,#40395,#40396,
#40397,#40398,#40399,#40400,#40401,#40402,#40403,#40404,#40405,#40406,#40407,
#40408,#40409,#40410,#40411,#40412,#40413,#40414,#40415,#40416,#40417,#40418,
#40419,#40420,#40421,#40422,#40423,#40424,#40425,#40426,#40427,#40428,#40429,
#40430,#40431,#40432,#40433),.UNSPECIFIED.,.F.,.F.,(4,3,3,3,3,3,3,3,3,3,
3,3,3,3,3,3,3,3,3,3,3,4),(13.8752088702144,13.9625085938209,14.0496979618328,
14.1368005596739,14.223841740639,14.3108504907928,14.3978479980121,14.4848554371231,
14.571947709351,14.659082001847,14.7463557856079,14.8294259525565,14.9162035685692,
15.002873174162,15.0910094358584,15.1775356280929,15.2640329140993,15.3505229188245,
15.4398830060516,15.5264646980202,15.6172139828766,15.707963267733),
 .UNSPECIFIED.);
#2164=B_SPLINE_CURVE_WITH_KNOTS('',3,(#40434,#40435,#40436,#40437,#40438,
#40439,#40440,#40441,#40442,#40443,#40444,#40445,#40446,#40447,#40448,#40449,
#40450,#40451,#40452,#40453,#40454,#40455,#40456,#40457,#40458,#40459,#40460,
#40461,#40462,#40463,#40464,#40465,#40466,#40467,#40468,#40469,#40470,#40471,
#40472,#40473,#40474,#40475,#40476,#40477,#40478,#40479,#40480,#40481,#40482,
#40483,#40484,#40485,#40486,#40487,#40488,#40489,#40490,#40491,#40492,#40493,
#40494,#40495,#40496,#40497,#40498,#40499,#40500,#40501,#40502,#40503,#40504,
#40505,#40506,#40507,#40508,#40509,#40510,#40511,#40512,#40513,#40514,#40515),
 .UNSPECIFIED.,.F.,.F.,(4,3,3,3,3,3,3,3,3,3,3,3,3,3,3,3,3,3,3,3,3,3,3,3,
3,3,3,4),(15.7079632679489,15.8200553291365,15.9077986523985,15.9954302534377,
16.0829732289737,16.1739371635665,16.2613799276287,16.3488093099911,16.4362460475909,
16.5237108776269,16.6112726216378,16.6988918158899,16.7866370650151,16.8106847057165,
16.8985113353392,16.9862271381107,17.0738551030503,17.1647874754561,17.2523166530516,
17.3398328257959,17.4273566374916,17.5149087323411,17.6025575862392,17.6902639032282,
17.7780956293868,17.8013140822965,17.8891406021589,17.9338702011125),
 .UNSPECIFIED.);
#2165=B_SPLINE_CURVE_WITH_KNOTS('',3,(#40521,#40522,#40523,#40524,#40525,
#40526,#40527,#40528,#40529,#40530,#40531,#40532,#40533,#40534,#40535,#40536,
#40537,#40538,#40539,#40540,#40541,#40542,#40543,#40544,#40545,#40546,#40547,
#40548,#40549,#40550,#40551,#40552,#40553,#40554,#40555,#40556,#40557,#40558,
#40559,#40560,#40561,#40562,#40563,#40564,#40565,#40566,#40567,#40568,#40569,
#40570,#40571,#40572,#40573,#40574,#40575,#40576,#40577,#40578,#40579,#40580,
#40581,#40582,#40583,#40584,#40585,#40586,#40587,#40588,#40589,#40590,#40591,
#40592,#40593,#40594,#40595,#40596,#40597,#40598,#40599,#40600,#40601,#40602,
#40603,#40604,#40605,#40606,#40607,#40608,#40609,#40610,#40611,#40612,#40613,
#40614,#40615,#40616,#40617),.UNSPECIFIED.,.F.,.F.,(4,3,3,3,3,3,3,3,3,3,
3,3,3,3,3,3,3,3,3,3,3,3,3,3,3,3,3,3,3,3,3,3,4),(64.4958550652426,64.5877404030811,
64.6795364658092,64.7712745072369,64.862983345553,64.954686720116,65.0464083595795,
65.1382289717397,65.2301030353743,65.3221248384973,65.3815388542818,65.4728329308018,
65.5640057866637,65.6550847449215,65.7461022669468,65.8370883287862,65.928067469142,
66.0190642154069,66.1101667576848,66.2013233141153,66.292644913399,66.3721682308618,
66.4665062483791,66.5607062484631,66.6547902335657,66.7487644812764,66.842674877868,
66.936541135683,67.0303829231798,67.1242465059106,67.218119628696,67.3120590157693,
67.3627976074418),.UNSPECIFIED.);
#2166=B_SPLINE_CURVE_WITH_KNOTS('',3,(#40625,#40626,#40627,#40628,#40629,
#40630,#40631,#40632,#40633,#40634,#40635,#40636,#40637,#40638,#40639,#40640,
#40641,#40642,#40643,#40644,#40645,#40646,#40647,#40648,#40649,#40650,#40651,
#40652,#40653,#40654,#40655,#40656,#40657,#40658,#40659,#40660,#40661,#40662,
#40663,#40664,#40665,#40666,#40667,#40668,#40669,#40670,#40671,#40672,#40673,
#40674,#40675,#40676,#40677,#40678,#40679,#40680,#40681,#40682,#40683,#40684,
#40685,#40686,#40687,#40688,#40689,#40690,#40691,#40692,#40693,#40694,#40695,
#40696,#40697,#40698,#40699,#40700,#40701,#40702,#40703,#40704,#40705,#40706,
#40707,#40708,#40709,#40710,#40711,#40712,#40713,#40714,#40715,#40716,#40717,
#40718,#40719,#40720,#40721,#40722,#40723,#40724,#40725,#40726,#40727,#40728,
#40729,#40730,#40731,#40732,#40733,#40734,#40735,#40736,#40737,#40738,#40739,
#40740,#40741,#40742,#40743,#40744,#40745,#40746,#40747,#40748,#40749,#40750,
#40751,#40752,#40753,#40754,#40755,#40756,#40757,#40758,#40759,#40760,#40761,
#40762),.UNSPECIFIED.,.F.,.F.,(4,2,2,2,2,2,2,2,2,2,2,2,2,2,2,2,2,2,2,2,
2,2,2,2,2,2,2,2,2,2,2,2,2,2,2,2,2,2,2,2,2,2,2,2,2,2,2,2,2,2,2,2,2,2,2,2,
2,2,2,2,2,2,2,2,2,2,2,2,4),(-3.81690193809338,-3.80414545028679,-3.74006670025191,
-3.69143912438751,-3.67227555739686,-3.66253149013823,-3.65529778374144,
-3.64612779634758,-3.6303228501089,-3.57080907174332,-3.52674181012936,
-3.50434173804963,-3.49714682080329,-3.49240217095334,-3.48806388982645,
-3.48039696001934,-3.45481822290918,-3.39538903941858,-3.36314194761511,
-3.3406137393263,-3.33029784217486,-3.32227202401578,-3.31327616013516,
-3.2977952451329,-3.22257762170979,-3.18687473232911,-3.1669709983955,-3.16011060326152,
-3.15547992791916,-3.15052693251671,-3.1420346445659,-3.09741113398896,
-3.02265432295446,-3.00243450222272,-2.99258160859251,-2.98467194293698,
-2.97554600821613,-2.95958025925697,-2.90534583632465,-2.85485954733824,
-2.83850678214073,-2.82678223374312,-2.82118593506205,-2.81671656323342,
-2.81101396826663,-2.79881933994248,-2.73399278679964,-2.6738834699548,
-2.66033836246495,-2.65176457330894,-2.64364960445811,-2.63250047144603,
-2.60605909251575,-2.52462372080695,-2.5047252556928,-2.49120335488778,
-2.48526031934081,-2.48075981992556,-2.47531004946878,-2.46447168822773,
-2.41889546612772,-2.3786913472785,-2.33579892213381,-2.32312843674949,
-2.31473721833348,-2.30661779422243,-2.2967885560053,-2.27226928694569,
-2.25645475069973),.UNSPECIFIED.);
#2167=B_SPLINE_CURVE_WITH_KNOTS('',3,(#40768,#40769,#40770,#40771,#40772,
#40773,#40774,#40775,#40776,#40777,#40778,#40779,#40780,#40781,#40782,#40783,
#40784,#40785,#40786,#40787,#40788,#40789,#40790,#40791,#40792,#40793,#40794,
#40795,#40796,#40797,#40798,#40799,#40800,#40801,#40802,#40803,#40804,#40805,
#40806,#40807,#40808,#40809,#40810,#40811,#40812,#40813,#40814,#40815,#40816,
#40817,#40818,#40819,#40820,#40821,#40822,#40823,#40824,#40825,#40826,#40827,
#40828,#40829,#40830,#40831,#40832,#40833,#40834,#40835,#40836,#40837,#40838,
#40839,#40840,#40841,#40842,#40843,#40844,#40845,#40846,#40847,#40848,#40849,
#40850,#40851,#40852,#40853,#40854,#40855,#40856,#40857,#40858,#40859,#40860,
#40861,#40862,#40863,#40864,#40865,#40866,#40867,#40868,#40869,#40870,#40871,
#40872,#40873,#40874,#40875,#40876,#40877,#40878,#40879,#40880,#40881,#40882,
#40883,#40884,#40885,#40886,#40887,#40888,#40889,#40890,#40891,#40892,#40893,
#40894,#40895,#40896,#40897,#40898,#40899,#40900,#40901,#40902,#40903,#40904,
#40905,#40906,#40907,#40908,#40909,#40910,#40911,#40912,#40913,#40914,#40915,
#40916,#40917,#40918,#40919,#40920,#40921,#40922,#40923,#40924,#40925,#40926,
#40927,#40928,#40929,#40930,#40931,#40932,#40933,#40934,#40935,#40936,#40937,
#40938,#40939,#40940,#40941,#40942,#40943,#40944,#40945,#40946,#40947),
 .UNSPECIFIED.,.F.,.F.,(4,2,2,2,2,2,2,2,2,2,2,2,2,2,2,2,2,2,2,2,2,2,2,2,
2,2,2,2,2,2,2,2,2,2,2,2,2,2,2,2,2,2,2,2,2,2,2,2,2,2,2,2,2,2,2,2,2,2,2,2,
2,2,2,2,2,2,2,2,2,2,2,2,2,2,2,2,2,2,2,2,2,2,2,2,2,2,2,2,2,4),(-2.01531234407017,
-1.97096071078704,-1.94756117148109,-1.94012707427523,-1.93585906585756,
-1.93117861938418,-1.92401863266923,-1.90127479300297,-1.85607749715525,
-1.79539326600502,-1.77945841106368,-1.77031199891029,-1.76235999565864,
-1.75241957764504,-1.73187232048903,-1.70360323259721,-1.63827914899585,
-1.61166142695045,-1.60392394047654,-1.59912274772414,-1.59439286442838,
-1.58697925931703,-1.56155110645004,-1.50514337105469,-1.45364312936907,
-1.44026864850318,-1.43174256154302,-1.42363164322879,-1.41242264472587,
-1.38366530533075,-1.3362418665076,-1.280027888161,-1.26961727198234,-1.26419216174676,
-1.25970053465287,-1.25375564008212,-1.24017238688386,-1.22013767941578,
-1.13713900350793,-1.11179980248811,-1.10185975090524,-1.0937148900344,
-1.08536358891572,-1.07288389784815,-1.03232843341363,-0.99073421416931,
-0.940181800771379,-0.931553232076937,-0.926558103314133,-0.921941325626722,
-0.915144016305742,-0.895696934292268,-0.86127186389371,-0.784286112040376,
-0.769119060862726,-0.760213094409259,-0.752213079457205,-0.741854976089624,
-0.718911761965742,-0.685780168885447,-0.621742558040532,-0.601006840376462,
-0.593860350086747,-0.589647664390503,-0.584938237636751,-0.577545741920772,
-0.552096825450915,-0.495596634234857,-0.443744339147798,-0.430383760090047,
-0.421886454731182,-0.413818752528643,-0.402697901897264,-0.374376201577517,
-0.328113283163754,-0.270139775620982,-0.259758510931615,-0.254350155192959,
-0.249854865442335,-0.24389290665396,-0.230278661201946,-0.210200479535493,
-0.130807265518076,-0.102676346592433,-0.0912254172311799,-0.0831179788853059,
-0.0746125335939819,-0.0659661057019032,-0.0534904667728278,-0.00100289086636027),
 .UNSPECIFIED.);
#2168=B_SPLINE_CURVE_WITH_KNOTS('',3,(#40948,#40949,#40950,#40951,#40952,
#40953,#40954,#40955,#40956,#40957,#40958,#40959,#40960,#40961,#40962,#40963),
 .UNSPECIFIED.,.F.,.F.,(4,3,3,3,3,4),(64.1406906932069,64.2575061085724,
64.376659147886,64.3909094777018,64.4829383736409,64.4958550652426),
 .UNSPECIFIED.);
#2169=B_SPLINE_CURVE_WITH_KNOTS('',3,(#40964,#40965,#40966,#40967,#40968,
#40969,#40970,#40971,#40972,#40973,#40974,#40975,#40976,#40977,#40978,#40979,
#40980,#40981,#40982,#40983,#40984,#40985,#40986,#40987,#40988,#40989,#40990,
#40991,#40992,#40993,#40994,#40995,#40996,#40997,#40998,#40999,#41000,#41001,
#41002,#41003,#41004,#41005,#41006,#41007,#41008,#41009,#41010,#41011,#41012,
#41013,#41014,#41015,#41016,#41017,#41018,#41019,#41020,#41021,#41022,#41023,
#41024,#41025,#41026,#41027,#41028,#41029,#41030,#41031,#41032,#41033,#41034,
#41035,#41036,#41037,#41038,#41039,#41040,#41041,#41042,#41043,#41044,#41045,
#41046,#41047,#41048,#41049,#41050,#41051,#41052,#41053,#41054,#41055,#41056,
#41057,#41058,#41059,#41060,#41061,#41062,#41063,#41064,#41065,#41066,#41067,
#41068,#41069,#41070,#41071,#41072,#41073,#41074,#41075,#41076,#41077,#41078,
#41079,#41080,#41081,#41082,#41083,#41084,#41085,#41086,#41087,#41088,#41089,
#41090,#41091,#41092,#41093,#41094,#41095,#41096,#41097,#41098,#41099,#41100,
#41101,#41102,#41103,#41104,#41105,#41106,#41107,#41108,#41109,#41110,#41111,
#41112,#41113,#41114,#41115,#41116,#41117,#41118,#41119,#41120,#41121,#41122,
#41123,#41124,#41125,#41126,#41127,#41128,#41129,#41130,#41131,#41132,#41133,
#41134,#41135,#41136,#41137,#41138,#41139,#41140,#41141,#41142,#41143,#41144,
#41145,#41146,#41147,#41148,#41149,#41150,#41151,#41152,#41153,#41154,#41155),
 .UNSPECIFIED.,.F.,.F.,(4,2,2,2,2,2,2,2,2,2,2,2,2,2,2,2,2,2,2,2,2,2,2,2,
2,2,2,2,2,2,2,2,2,2,2,2,2,2,2,2,2,2,2,2,2,2,2,2,2,2,2,2,2,2,2,2,2,2,2,2,
2,2,2,2,2,2,2,2,2,2,2,2,2,2,2,2,2,2,2,2,2,2,2,2,2,2,2,2,2,2,2,2,2,2,2,4),
(-2.25645475069973,-2.188265448513,-2.16815843609405,-2.15453821968529,
-2.14858587548042,-2.14409225088409,-2.13866927501132,-2.12794687637382,
-2.07587180914517,-2.02572030966631,-1.99603011594337,-1.98469628771983,
-1.97656215447964,-1.96807063594224,-1.95487485215768,-1.90852023295647,
-1.89844238129165,-1.84103080710226,-1.82056959567721,-1.81345690373307,
-1.80924954920082,-1.80450052140059,-1.79701064568396,-1.77076241439251,
-1.71029880931953,-1.66349789525828,-1.65027370516261,-1.64177216833422,
-1.63363400967182,-1.62230330094654,-1.59267139016292,-1.54269769962391,
-1.4904687176247,-1.47975562867317,-1.47433213963494,-1.46983704915597,
-1.46387973493251,-1.45022757179672,-1.43005017310064,-1.34509617745399,
-1.3213205756484,-1.31161009754599,-1.303522105511,-1.29509490721011,-1.28223109408553,
-1.23658046206208,-1.22311545002981,-1.16236323575234,-1.14601326662377,
-1.13947205713935,-1.13490538025649,-1.12981840470572,-1.12074815780125,
-1.06918814745251,-0.994513787886353,-0.97921918350772,-0.970210408231548,
-0.962241540986392,-0.95209543013702,-0.930370163976092,-0.899759061955401,
-0.885554438346332,-0.823229219635458,-0.808794455182487,-0.803121969379304,
-0.798563805297194,-0.79358192782134,-0.78500582672239,-0.73552007182797,
-0.657057653698884,-0.642038768689281,-0.633170033097429,-0.625174299932297,
-0.614780909739931,-0.591576030415419,-0.557865252858062,-0.490267689536701,
-0.47307611811594,-0.466400594942164,-0.461857112838476,-0.45684337744927,
-0.448116895776467,-0.392670159420877,-0.321954874120637,-0.306301508353274,
-0.297216285368031,-0.289334882880902,-0.279349669776681,-0.258543889233515,
-0.229767793039436,-0.189691094015558,-0.14418007717786,-0.133351997982961,
-0.127908072083656,-0.123460552149581,-0.121335708249485),.UNSPECIFIED.);
#2170=B_SPLINE_CURVE_WITH_KNOTS('',3,(#41160,#41161,#41162,#41163,#41164,
#41165,#41166,#41167,#41168,#41169,#41170,#41171,#41172,#41173,#41174,#41175,
#41176,#41177,#41178,#41179,#41180,#41181,#41182,#41183,#41184,#41185,#41186,
#41187,#41188,#41189,#41190,#41191,#41192,#41193,#41194,#41195,#41196,#41197,
#41198,#41199,#41200,#41201,#41202,#41203,#41204,#41205,#41206,#41207,#41208,
#41209,#41210,#41211,#41212,#41213,#41214,#41215,#41216,#41217,#41218,#41219,
#41220,#41221,#41222,#41223,#41224,#41225,#41226,#41227,#41228,#41229,#41230,
#41231,#41232,#41233,#41234,#41235,#41236,#41237,#41238,#41239,#41240,#41241,
#41242,#41243,#41244,#41245,#41246,#41247,#41248,#41249,#41250,#41251,#41252,
#41253,#41254,#41255,#41256,#41257,#41258,#41259,#41260,#41261,#41262,#41263,
#41264,#41265,#41266,#41267,#41268,#41269,#41270,#41271,#41272,#41273,#41274,
#41275,#41276,#41277,#41278,#41279,#41280,#41281,#41282,#41283,#41284,#41285,
#41286,#41287,#41288,#41289,#41290,#41291,#41292,#41293,#41294,#41295,#41296,
#41297,#41298,#41299,#41300,#41301,#41302,#41303,#41304,#41305,#41306,#41307,
#41308,#41309,#41310,#41311,#41312,#41313,#41314,#41315,#41316,#41317,#41318,
#41319,#41320,#41321,#41322,#41323,#41324,#41325,#41326,#41327,#41328,#41329,
#41330,#41331,#41332,#41333,#41334,#41335,#41336,#41337,#41338,#41339,#41340,
#41341,#41342,#41343,#41344,#41345,#41346,#41347,#41348,#41349),
 .UNSPECIFIED.,.F.,.F.,(4,2,2,2,2,2,2,2,2,2,2,2,2,2,2,2,2,2,2,2,2,2,2,2,
2,2,2,2,2,2,2,2,2,2,2,2,2,2,2,2,2,2,2,2,2,2,2,2,2,2,2,2,2,2,2,2,2,2,2,2,
2,2,2,2,2,2,2,2,2,2,2,2,2,2,2,2,2,2,2,2,2,2,2,2,2,2,2,2,2,2,2,2,2,2,4),
(-4.15000030030656,-4.13522595040735,-4.12612224403312,-4.1181680101193,
-4.1081727281752,-4.08730727980301,-4.01243572831013,-3.96889446418885,
-3.96046012439918,-3.95550915659461,-3.95093640263236,-3.94409228744308,
-3.92570181317871,-3.86664531623664,-3.81430169542254,-3.79843147169064,
-3.78938914649105,-3.78142655973881,-3.7713372622721,-3.7499361892784,-3.67564526612205,
-3.63231580287583,-3.62388759687953,-3.61893782158866,-3.61436420297819,
-3.60751588561074,-3.58909591392204,-3.52272747619935,-3.48920904052984,
-3.4660953789852,-3.45571739364971,-3.4477241928364,-3.43884889150076,-3.42379510032387,
-3.3456744712235,-3.31168912620144,-3.29239344926946,-3.2856235084116,-3.28101845485011,
-3.27602503329004,-3.2673929348142,-3.21666315206821,-3.1749022291993,-3.13454329118665,
-3.12208179672211,-3.11373626683079,-3.10559244226796,-3.09375481510775,
-3.06254465986431,-2.98649171791725,-2.96703262970778,-2.95372748759616,
-2.94783027314582,-2.94338237337333,-2.93793840032815,-2.92711147250309,
-2.88161688398382,-2.84160215013881,-2.79846697280289,-2.78578337991619,
-2.77739355973636,-2.76928296414223,-2.75947370479395,-2.73505758917039,
-2.65099955049287,-2.6308964216389,-2.61728003269597,-2.61132989618514,
-2.6068371504258,-2.60141341958735,-2.59101648509901,-2.5344267690082,-2.48719136814472,
-2.45849700874451,-2.44729250972131,-2.43917887915967,-2.43064445830223,
-2.41724457248662,-2.36459922493143,-2.3167899239068,-2.29528969457129,
-2.28101527636916,-2.27495694014567,-2.2704550016318,-2.26510769534646,
-2.25507390069574,-2.19290508873731,-2.13594954400614,-2.11923130021793,
-2.10905678828977,-2.10108571336672,-2.09209547865436,-2.07648200164671,
-2.02609895850442,-2.01531234407017),.UNSPECIFIED.);
#2171=B_SPLINE_CURVE_WITH_KNOTS('',3,(#41351,#41352,#41353,#41354,#41355,
#41356,#41357,#41358,#41359,#41360),.UNSPECIFIED.,.F.,.F.,(4,2,2,2,4),(-0.121335708249485,
-0.117564260348161,-0.104263477214096,-0.0848110634910586,-0.000973465629640573),
 .UNSPECIFIED.);
#2172=B_SPLINE_CURVE_WITH_KNOTS('',3,(#41361,#41362,#41363,#41364,#41365,
#41366,#41367,#41368,#41369,#41370,#41371,#41372,#41373,#41374,#41375,#41376,
#41377,#41378,#41379,#41380,#41381,#41382,#41383,#41384,#41385,#41386,#41387,
#41388,#41389,#41390,#41391,#41392,#41393,#41394,#41395,#41396,#41397,#41398,
#41399,#41400,#41401,#41402,#41403,#41404,#41405,#41406,#41407,#41408,#41409,
#41410,#41411,#41412,#41413,#41414,#41415,#41416,#41417,#41418,#41419,#41420,
#41421,#41422,#41423,#41424,#41425,#41426,#41427,#41428,#41429,#41430,#41431,
#41432,#41433,#41434,#41435,#41436,#41437,#41438,#41439,#41440,#41441,#41442,
#41443,#41444,#41445,#41446,#41447,#41448,#41449,#41450,#41451,#41452,#41453,
#41454,#41455,#41456,#41457,#41458,#41459,#41460,#41461,#41462,#41463,#41464,
#41465,#41466,#41467,#41468,#41469,#41470,#41471,#41472,#41473,#41474,#41475,
#41476,#41477,#41478,#41479,#41480,#41481,#41482,#41483,#41484,#41485,#41486,
#41487,#41488,#41489,#41490,#41491,#41492,#41493,#41494,#41495,#41496,#41497,
#41498,#41499,#41500,#41501,#41502,#41503,#41504,#41505,#41506,#41507,#41508,
#41509,#41510,#41511,#41512,#41513,#41514,#41515,#41516,#41517,#41518,#41519,
#41520,#41521,#41522,#41523,#41524,#41525,#41526,#41527,#41528,#41529,#41530,
#41531,#41532,#41533,#41534,#41535,#41536,#41537,#41538,#41539,#41540,#41541,
#41542,#41543,#41544,#41545,#41546),.UNSPECIFIED.,.F.,.F.,(4,2,2,2,2,2,
2,2,2,2,2,2,2,2,2,2,2,2,2,2,2,2,2,2,2,2,2,2,2,2,2,2,2,2,2,2,2,2,2,2,2,2,
2,2,2,2,2,2,2,2,2,2,2,2,2,2,2,2,2,2,2,2,2,2,2,2,2,2,2,2,2,2,2,2,2,2,2,2,
2,2,2,2,2,2,2,2,2,2,2,2,2,2,4),(-4.27050795113119,-4.25427509224251,-4.24187184123641,
-4.23392038678693,-4.22635788692161,-4.21786888783709,-4.2046916503057,
-4.15667450537091,-4.11270201949893,-4.08562384944383,-4.07412039256904,
-4.06510399142198,-4.06002892635896,-4.0554590881063,-4.04889385528842,
-4.03238977752879,-3.97175555728779,-3.9594578584735,-3.91284132260937,
-3.89991610359644,-3.89147808861424,-3.8834006826038,-3.87372829332611,
-3.85018088847584,-3.77871234957384,-3.74995726080526,-3.73801905846285,
-3.72874440550528,-3.72361487282174,-3.71906372566782,-3.71261803819451,
-3.69689454521145,-3.63559155388604,-3.62185217026508,-3.57615591480885,
-3.56329060002804,-3.55486447135609,-3.54677901353323,-3.53707346595768,
-3.51306677924514,-3.42837831455247,-3.40822977720239,-3.39459162077917,
-3.38863782059636,-3.38414465071832,-3.37872316129739,-3.36801149609525,
-3.32462882414156,-3.28740567162125,-3.25561117235718,-3.23331213371091,
-3.22306855011089,-3.21508981602223,-3.20613910625361,-3.19072098630399,
-3.11559915966695,-3.07998223187042,-3.0601288465694,-3.05329070598799,
-3.04867293115153,-3.04370336182409,-3.03518412404142,-2.9885336060331,
-2.95121881375009,-2.91919561683897,-2.89678677364846,-2.88652468954481,
-2.87854389247775,-2.86960359737184,-2.8542365922706,-2.77865856591189,
-2.72776651118525,-2.71876113431754,-2.71368788927925,-2.70911634267098,
-2.70254397524677,-2.68599921173671,-2.61765484911533,-2.56695345195617,
-2.55379060483459,-2.54530373379731,-2.53725374869916,-2.52595409457097,
-2.49858219706786,-2.41803478742769,-2.39819670598228,-2.38470740196583,
-2.37877838414161,-2.37428671496978,-2.36884589115274,-2.35836939704919,
-2.30339600301409,-2.25596412166985),.UNSPECIFIED.);
#2173=B_SPLINE_CURVE_WITH_KNOTS('',3,(#41552,#41553,#41554,#41555,#41556,
#41557,#41558,#41559,#41560,#41561,#41562,#41563,#41564,#41565,#41566,#41567,
#41568,#41569,#41570,#41571,#41572,#41573,#41574,#41575,#41576,#41577,#41578,
#41579,#41580,#41581,#41582,#41583,#41584,#41585,#41586,#41587,#41588,#41589,
#41590,#41591,#41592,#41593,#41594,#41595,#41596,#41597,#41598,#41599,#41600,
#41601,#41602,#41603,#41604,#41605,#41606,#41607,#41608,#41609,#41610,#41611,
#41612,#41613,#41614,#41615,#41616,#41617,#41618,#41619,#41620,#41621,#41622,
#41623,#41624,#41625,#41626,#41627,#41628,#41629,#41630,#41631,#41632,#41633,
#41634,#41635,#41636,#41637,#41638,#41639,#41640,#41641,#41642,#41643,#41644,
#41645,#41646,#41647,#41648,#41649,#41650,#41651,#41652,#41653,#41654,#41655,
#41656,#41657,#41658,#41659,#41660,#41661,#41662,#41663,#41664,#41665,#41666,
#41667,#41668,#41669,#41670,#41671,#41672,#41673,#41674,#41675,#41676,#41677,
#41678,#41679,#41680,#41681,#41682,#41683,#41684,#41685,#41686,#41687,#41688,
#41689,#41690,#41691,#41692,#41693,#41694,#41695,#41696,#41697,#41698,#41699,
#41700,#41701,#41702,#41703,#41704,#41705,#41706,#41707,#41708,#41709,#41710,
#41711,#41712,#41713,#41714,#41715,#41716,#41717,#41718,#41719,#41720,#41721,
#41722,#41723,#41724,#41725,#41726,#41727,#41728,#41729),.UNSPECIFIED.,
 .F.,.F.,(4,2,2,2,2,2,2,2,2,2,2,2,2,2,2,2,2,2,2,2,2,2,2,2,2,2,2,2,2,2,2,
2,2,2,2,2,2,2,2,2,2,2,2,2,2,2,2,2,2,2,2,2,2,2,2,2,2,2,2,2,2,2,2,2,2,2,2,
2,2,2,2,2,2,2,2,2,2,2,2,2,2,2,2,2,2,2,2,2,4),(-2.01478766729567,-1.98142389693945,
-1.90135735049127,-1.88505447692978,-1.87583124846293,-1.8678881810667,
-1.85805706238154,-1.83810810408146,-1.81098734267399,-1.76932464463373,
-1.71869675514139,-1.71006912025876,-1.7050768304324,-1.70047168013875,
-1.69369987558578,-1.6743878931761,-1.64035314228899,-1.56226691515312,
-1.54720299431889,-1.53832596575697,-1.53033382050518,-1.51996091430828,
-1.49687480223465,-1.46341745743288,-1.39734061014468,-1.37868245833986,
-1.3718019831211,-1.36722274917873,-1.36228461190409,-1.35390908580366,
-1.31220651445861,-1.22724137417402,-1.21151030866746,-1.2024094486579,
-1.19453151211719,-1.18457323705081,-1.16391317723629,-1.13542029563517,
-1.09502048355667,-1.04552330017201,-1.03694835231939,-1.03196772929687,
-1.02735769767903,-1.02055649438021,-1.0009998139111,-0.966252100677531,
-0.889520172021265,-0.874289459176133,-0.865378858957684,-0.857395149079794,
-0.847087909724196,-0.824395548004203,-0.791775153128422,-0.730540570037904,
-0.706878780679631,-0.699421142699084,-0.695149448922323,-0.69047613921818,
-0.683344178148795,-0.660850803202293,-0.616563122089116,-0.554623296238921,
-0.53870543267637,-0.529564798957579,-0.521615667916473,-0.51167611442652,
-0.491120496375201,-0.462830958785143,-0.397318212727982,-0.370912933643943,
-0.363200716833005,-0.358405702039758,-0.353669053240905,-0.346229507236389,
-0.320527900062388,-0.262788045056662,-0.212936707808891,-0.199603655886079,
-0.191083975175575,-0.182964918134244,-0.171721015387564,-0.142716955262853,
-0.0645510868593842,-0.0348535160217683,-0.0269078290753282,-0.0220624077458015,
-0.0178631849065608,-0.0131574246501657,-0.000968296068967554),
 .UNSPECIFIED.);
#2174=B_SPLINE_CURVE_WITH_KNOTS('',3,(#41730,#41731,#41732,#41733,#41734,
#41735,#41736,#41737),.UNSPECIFIED.,.F.,.F.,(4,2,2,4),(-4.27065792886625,
-4.20615549532007,-4.15140004945084,-4.15000030030656),.UNSPECIFIED.);
#2175=B_SPLINE_CURVE_WITH_KNOTS('',3,(#41738,#41739,#41740,#41741,#41742,
#41743,#41744,#41745,#41746,#41747,#41748,#41749,#41750,#41751,#41752,#41753,
#41754,#41755,#41756,#41757,#41758,#41759,#41760,#41761,#41762,#41763,#41764,
#41765,#41766,#41767,#41768,#41769,#41770,#41771,#41772,#41773,#41774,#41775,
#41776,#41777,#41778,#41779,#41780,#41781,#41782,#41783,#41784,#41785,#41786,
#41787,#41788,#41789,#41790,#41791,#41792,#41793,#41794,#41795,#41796,#41797,
#41798,#41799,#41800,#41801,#41802,#41803,#41804,#41805,#41806,#41807,#41808,
#41809,#41810,#41811,#41812,#41813,#41814,#41815,#41816,#41817,#41818,#41819,
#41820,#41821,#41822,#41823,#41824,#41825,#41826,#41827,#41828,#41829,#41830,
#41831,#41832,#41833,#41834,#41835,#41836,#41837,#41838,#41839,#41840,#41841,
#41842,#41843,#41844,#41845,#41846,#41847,#41848,#41849,#41850,#41851,#41852,
#41853,#41854,#41855,#41856,#41857,#41858,#41859,#41860,#41861,#41862,#41863,
#41864,#41865,#41866,#41867,#41868,#41869,#41870,#41871,#41872,#41873,#41874,
#41875,#41876,#41877,#41878,#41879,#41880,#41881,#41882,#41883,#41884,#41885,
#41886,#41887,#41888,#41889,#41890,#41891,#41892,#41893,#41894,#41895,#41896,
#41897,#41898,#41899,#41900,#41901,#41902,#41903,#41904,#41905,#41906,#41907,
#41908,#41909,#41910,#41911,#41912,#41913,#41914,#41915,#41916,#41917,#41918,
#41919,#41920,#41921,#41922,#41923,#41924,#41925,#41926,#41927,#41928,#41929,
#41930,#41931),.UNSPECIFIED.,.F.,.F.,(4,2,2,2,2,2,2,2,2,2,2,2,2,2,2,2,2,
2,2,2,2,2,2,2,2,2,2,2,2,2,2,2,2,2,2,2,2,2,2,2,2,2,2,2,2,2,2,2,2,2,2,2,2,
2,2,2,2,2,2,2,2,2,2,2,2,2,2,2,2,2,2,2,2,2,2,2,2,2,2,2,2,2,2,2,2,2,2,2,2,
2,2,2,2,2,2,2,4),(-2.25596412166985,-2.2551379854961,-2.22608637296791,
-2.21483339454486,-2.20671065979714,-2.19818968427851,-2.18485997948021,
-2.13519491500529,-2.06932410101386,-2.05044322982937,-2.0435315989119,
-2.03894582033343,-2.03401633038426,-2.02568450100034,-1.98523838899684,
-1.8980868588721,-1.88279795745333,-1.87379068302208,-1.86582200203709,
-1.85567453631106,-1.83393945445079,-1.80330724510446,-1.78899408232026,
-1.72640696377141,-1.71227107524586,-1.7066461540982,-1.70209946070938,
-1.69709383233158,-1.68840486469955,-1.63237114707048,-1.56221973169301,
-1.54654398055015,-1.53745411601684,-1.52957353028796,-1.5195957794005,
-1.49883118563971,-1.47013551359376,-1.42996647931124,-1.38441460968031,
-1.37358379276728,-1.368139405013,-1.36369202641143,-1.35779658776674,-1.34450037687088,
-1.32505718286995,-1.2492349082855,-1.21777785050964,-1.20591201062179,
-1.19850358834704,-1.19029985459145,-1.17857926328215,-1.14570108425752,
-1.08463669812455,-1.04382719482968,-1.03537074901929,-1.03041516031307,
-1.02579118732442,-1.01891630498404,-0.998748193815775,-0.962177584793591,
-0.888682651366288,-0.873274256426061,-0.864242062250927,-0.857075087309936,
-0.847370404398088,-0.828107243776125,-0.779058623815314,-0.715933260550799,
-0.70238689527521,-0.696859539065917,-0.692290403115334,-0.687214992189357,
-0.678195560823048,-0.66668565535097,-0.639582154705785,-0.551522355782278,
-0.536256091590146,-0.527338087300591,-0.519355704225066,-0.509061387720614,
-0.486447549114657,-0.453993099161195,-0.393692380463093,-0.369003787485475,
-0.361452964589601,-0.357163310527772,-0.352506372867473,-0.345457394138663,
-0.323745255209453,-0.28220043928023,-0.216426521639242,-0.200578912559654,
-0.191453180469336,-0.183578121966971,-0.173655586895282,-0.153195701320748,
-0.121341169407626),.UNSPECIFIED.);
#2176=B_SPLINE_CURVE_WITH_KNOTS('',3,(#41936,#41937,#41938,#41939,#41940,
#41941,#41942,#41943,#41944,#41945,#41946,#41947,#41948,#41949,#41950,#41951,
#41952,#41953,#41954,#41955,#41956,#41957,#41958,#41959,#41960,#41961,#41962,
#41963,#41964,#41965,#41966,#41967,#41968,#41969,#41970,#41971,#41972,#41973,
#41974,#41975,#41976,#41977,#41978,#41979,#41980,#41981,#41982,#41983,#41984,
#41985,#41986,#41987,#41988,#41989,#41990,#41991,#41992,#41993,#41994,#41995,
#41996,#41997,#41998,#41999,#42000,#42001,#42002,#42003,#42004,#42005,#42006,
#42007,#42008,#42009,#42010,#42011,#42012,#42013,#42014,#42015,#42016,#42017,
#42018,#42019,#42020,#42021,#42022,#42023,#42024,#42025,#42026,#42027,#42028,
#42029,#42030,#42031,#42032,#42033,#42034,#42035,#42036,#42037,#42038,#42039,
#42040,#42041,#42042,#42043,#42044,#42045,#42046,#42047,#42048,#42049,#42050,
#42051,#42052,#42053,#42054,#42055,#42056,#42057,#42058,#42059,#42060,#42061,
#42062,#42063,#42064,#42065,#42066,#42067,#42068,#42069,#42070,#42071,#42072,
#42073,#42074,#42075,#42076,#42077,#42078,#42079,#42080,#42081,#42082,#42083,
#42084,#42085,#42086,#42087,#42088,#42089,#42090,#42091,#42092,#42093,#42094,
#42095,#42096,#42097,#42098,#42099,#42100,#42101,#42102,#42103,#42104,#42105,
#42106,#42107,#42108,#42109,#42110,#42111,#42112,#42113,#42114,#42115,#42116,
#42117,#42118,#42119,#42120,#42121,#42122,#42123,#42124,#42125,#42126,#42127,
#42128,#42129),.UNSPECIFIED.,.F.,.F.,(4,2,2,2,2,2,2,2,2,2,2,2,2,2,2,2,2,
2,2,2,2,2,2,2,2,2,2,2,2,2,2,2,2,2,2,2,2,2,2,2,2,2,2,2,2,2,2,2,2,2,2,2,2,
2,2,2,2,2,2,2,2,2,2,2,2,2,2,2,2,2,2,2,2,2,2,2,2,2,2,2,2,2,2,2,2,2,2,2,2,
2,2,2,2,2,2,2,4),(-4.14944962827019,-4.10272140609561,-4.08258792449977,
-4.06895732269192,-4.0630051093006,-4.0585124126523,-4.05309060779653,-4.04237586294686,
-3.99890483705526,-3.96163290205661,-3.92992911186437,-3.90767433471585,
-3.89743876646285,-3.88946148643534,-3.88050745468491,-3.86507065031023,
-3.79013679466601,-3.75442114178497,-3.7345353890308,-3.72769376701249,
-3.72307564625416,-3.71810795052731,-3.70959615865846,-3.66414295848549,
-3.60656472702333,-3.57461604067516,-3.56300244048753,-3.55481768050234,
-3.54640097371988,-3.53358120895505,-3.49276629443858,-3.42675806024391,
-3.40830696029781,-3.39549868426518,-3.38968768882651,-3.38520352012154,
-3.37966957362805,-3.3683749946506,-3.30267708708476,-3.24218935864597,
-3.2286512886369,-3.22008880150768,-3.21198980315496,-3.2008722298171,-3.17462532518238,
-3.09270988792749,-3.07276761846719,-3.05922882914262,-3.05329210381133,
-3.0488006065242,-3.04336736872438,-3.03259412001313,-2.98793890818088,
-2.94971515760834,-2.91930559132735,-2.89768210045214,-2.88755409757852,
-2.87958772172778,-2.8705693834402,-2.85522732124278,-2.78110857098009,
-2.74493162950937,-2.72489250355291,-2.71803268118483,-2.71341123853565,
-2.70844997079813,-2.69996798124049,-2.65809049066428,-2.59781035034129,
-2.56513156021299,-2.55343296377898,-2.545232876767,-2.53782014683422,-2.52783785220864,
-2.50196522337615,-2.41964289722171,-2.39966921094172,-2.3861151904895,
-2.38017578238232,-2.37568396150665,-2.37025242555052,-2.359818212147,-2.3039562408426,
-2.25627402553365,-2.22742373468864,-2.21619848866257,-2.2080813446159,
-2.19955343348292,-2.18618555700907,-2.13500995014627,-2.06315795336684,
-2.04956370438327,-2.04368051160335,-2.03918507904081,-2.03378726581433,
-2.02319470450396,-2.01478766729567),.UNSPECIFIED.);
#2177=B_SPLINE_CURVE_WITH_KNOTS('',3,(#42131,#42132,#42133,#42134,#42135,
#42136,#42137,#42138,#42139,#42140,#42141,#42142,#42143,#42144,#42145,#42146,
#42147,#42148),.UNSPECIFIED.,.F.,.F.,(4,2,2,2,2,2,2,2,4),(-0.121341169407626,
-0.0779221281061221,-0.0618078642818699,-0.0331277363369873,-0.0252541112093821,
-0.0204242081549965,-0.0162322816208417,-0.0115142974486633,-0.000968280968871609),
 .UNSPECIFIED.);
#2178=B_SPLINE_CURVE_WITH_KNOTS('',3,(#42149,#42150,#42151,#42152,#42153,
#42154,#42155,#42156,#42157,#42158,#42159,#42160,#42161,#42162,#42163,#42164,
#42165,#42166,#42167,#42168,#42169,#42170,#42171,#42172,#42173,#42174,#42175,
#42176,#42177,#42178,#42179,#42180,#42181,#42182,#42183,#42184,#42185,#42186,
#42187,#42188,#42189,#42190,#42191,#42192,#42193,#42194,#42195,#42196,#42197,
#42198,#42199,#42200,#42201,#42202,#42203,#42204,#42205,#42206,#42207,#42208,
#42209,#42210,#42211,#42212,#42213,#42214,#42215,#42216,#42217,#42218,#42219,
#42220,#42221,#42222,#42223,#42224,#42225,#42226,#42227,#42228,#42229,#42230,
#42231,#42232,#42233,#42234,#42235,#42236,#42237,#42238,#42239,#42240,#42241,
#42242,#42243,#42244,#42245,#42246,#42247,#42248,#42249,#42250,#42251,#42252,
#42253,#42254,#42255,#42256,#42257,#42258,#42259,#42260,#42261,#42262,#42263,
#42264,#42265,#42266,#42267,#42268,#42269,#42270,#42271,#42272,#42273,#42274,
#42275,#42276,#42277,#42278,#42279,#42280,#42281,#42282,#42283,#42284,#42285,
#42286,#42287,#42288,#42289,#42290,#42291,#42292,#42293,#42294,#42295,#42296,
#42297,#42298,#42299,#42300,#42301,#42302,#42303,#42304,#42305,#42306,#42307,
#42308,#42309,#42310,#42311,#42312,#42313,#42314,#42315,#42316,#42317,#42318,
#42319,#42320,#42321,#42322,#42323,#42324),.UNSPECIFIED.,.F.,.F.,(4,2,2,
2,2,2,2,2,2,2,2,2,2,2,2,2,2,2,2,2,2,2,2,2,2,2,2,2,2,2,2,2,2,2,2,2,2,2,2,
2,2,2,2,2,2,2,2,2,2,2,2,2,2,2,2,2,2,2,2,2,2,2,2,2,2,2,2,2,2,2,2,2,2,2,2,
2,2,2,2,2,2,2,2,2,2,2,2,4),(-4.27077141273018,-4.20105219826454,-4.14924389285938,
-4.13344224297557,-4.12441342514241,-4.11644815710638,-4.10633566142047,
-4.08480338250272,-3.99625327394331,-3.97584256128733,-3.96207920923777,
-3.95610438645374,-3.95160946410396,-3.94620310348259,-3.93556874363832,
-3.88185273707762,-3.83276997960473,-3.80343763128845,-3.79214828949464,
-3.78401976837386,-3.77551076219949,-3.76223801797066,-3.7142017728616,
-3.65491380183328,-3.628900991073,-3.62143313151392,-3.61668958897118,-3.61189936620572,
-3.60421327101246,-3.5779971029985,-3.51221809101799,-3.4838788400994,-3.46329761859604,
-3.45335178833144,-3.4454003311876,-3.43625997065038,-3.42035022059746,
-3.35781378604334,-3.31398312054217,-3.29161478810358,-3.28449488725363,
-3.27982313319493,-3.27554746804555,-3.26807276610443,-3.24424598363636,
-3.18310022914985,-3.15048040740447,-3.12778803788044,-3.1174791186472,
-3.10949359475921,-3.10058045609086,-3.08534392797141,-3.00867199750743,
-2.97391170144308,-2.95434863372959,-2.94754575748717,-2.94293460850252,
-2.93795287863359,-2.92937606689271,-2.8798590595513,-2.83945987944723,
-2.79681775425765,-2.78417163056702,-2.7757893350776,-2.76767342070266,
-2.75784220126321,-2.73328315891535,-2.66285743987781,-2.62096900211229,
-2.61258682758397,-2.60764673373456,-2.6030674157682,-2.59618922529461,
-2.57755375690348,-2.51139982883573,-2.47791577687259,-2.4548176091818,
-2.44444168628536,-2.43644824230045,-2.42757081793226,-2.41250872731763,
-2.33443976584731,-2.30042262870487,-2.28111540045391,-2.27434372236135,
-2.26973811384994,-2.26474479455262,-2.25633136259072),.UNSPECIFIED.);
#2179=B_SPLINE_CURVE_WITH_KNOTS('',3,(#42330,#42331,#42332,#42333,#42334,
#42335,#42336,#42337,#42338,#42339,#42340,#42341,#42342,#42343,#42344,#42345,
#42346,#42347,#42348,#42349,#42350,#42351,#42352,#42353,#42354,#42355,#42356,
#42357,#42358,#42359,#42360,#42361,#42362,#42363,#42364,#42365,#42366,#42367,
#42368,#42369,#42370,#42371,#42372,#42373,#42374,#42375,#42376,#42377,#42378,
#42379,#42380,#42381,#42382,#42383,#42384,#42385,#42386,#42387,#42388,#42389,
#42390,#42391,#42392,#42393,#42394,#42395,#42396,#42397,#42398,#42399,#42400,
#42401,#42402,#42403,#42404,#42405,#42406,#42407,#42408,#42409,#42410,#42411,
#42412,#42413,#42414,#42415,#42416,#42417,#42418,#42419,#42420,#42421,#42422,
#42423,#42424,#42425,#42426,#42427,#42428,#42429,#42430,#42431,#42432,#42433,
#42434,#42435,#42436,#42437,#42438,#42439,#42440,#42441,#42442,#42443,#42444,
#42445,#42446,#42447,#42448,#42449,#42450,#42451,#42452,#42453,#42454,#42455,
#42456,#42457,#42458,#42459,#42460,#42461,#42462,#42463,#42464,#42465,#42466,
#42467,#42468,#42469,#42470,#42471,#42472,#42473,#42474,#42475,#42476,#42477,
#42478,#42479,#42480,#42481,#42482,#42483,#42484,#42485,#42486,#42487,#42488,
#42489,#42490,#42491,#42492,#42493,#42494,#42495,#42496,#42497,#42498,#42499,
#42500,#42501,#42502,#42503,#42504,#42505,#42506,#42507,#42508,#42509),
 .UNSPECIFIED.,.F.,.F.,(4,2,2,2,2,2,2,2,2,2,2,2,2,2,2,2,2,2,2,2,2,2,2,2,
2,2,2,2,2,2,2,2,2,2,2,2,2,2,2,2,2,2,2,2,2,2,2,2,2,2,2,2,2,2,2,2,2,2,2,2,
2,2,2,2,2,2,2,2,2,2,2,2,2,2,2,2,2,2,2,2,2,2,2,2,2,2,2,2,2,4),(-2.01490391173078,
-2.00684535224932,-1.99090656987869,-1.98176017668548,-1.97380962364891,
-1.96387300794123,-1.94334180002067,-1.86792495598627,-1.82452300238471,
-1.81602166620701,-1.81105598315887,-1.80643634844941,-1.79958754143215,
-1.77964518344978,-1.74376087128699,-1.66904877564289,-1.65376009335782,
-1.64475281449409,-1.63678405031052,-1.62663637114586,-1.60490038662731,
-1.57426647920632,-1.5599476420277,-1.49734608835629,-1.48322500072579,
-1.4776024289568,-1.47305625539427,-1.46804932085783,-1.45935436473628,
-1.44838425205299,-1.42328463243156,-1.34383558802149,-1.32129581333781,
-1.31112254981907,-1.30313330385377,-1.29424076639659,-1.27910275296648,
-1.23217962721677,-1.1635671918925,-1.147320065754,-1.14079681607781,-1.13623381255421,
-1.13114051978483,-1.12203734467052,-1.07003987364534,-0.996017413151274,
-0.980660974733026,-0.971639983970414,-0.963674770547508,-0.953553013990797,
-0.931962159377523,-0.901620565065788,-0.863360154938796,-0.81870850428584,
-0.807936563039386,-0.802503883960917,-0.798012824260372,-0.792076555194154,
-0.778538659530865,-0.758595594619598,-0.676735387771622,-0.650406572167471,
-0.63928109732649,-0.631181493311016,-0.622623022395973,-0.609101340019434,
-0.549122463871583,-0.484447291352478,-0.472190648028661,-0.466478497620411,
-0.461997831358171,-0.456376405049407,-0.444614461941354,-0.428205263096451,
-0.377392401210721,-0.323901138220019,-0.308041959160418,-0.298913584026355,
-0.291038545814011,-0.281119056319411,-0.260677242259078,-0.185436394360557,
-0.141752422474655,-0.133250781584499,-0.128285605539653,-0.123667022012404,
-0.116820600046438,-0.0968914194916686,-0.0610422761434274,-0.000969899208267077),
 .UNSPECIFIED.);
#2180=B_SPLINE_CURVE_WITH_KNOTS('',3,(#42510,#42511,#42512,#42513,#42514,
#42515,#42516,#42517,#42518,#42519,#42520,#42521,#42522,#42523,#42524,#42525,
#42526,#42527),.UNSPECIFIED.,.F.,.F.,(4,2,2,2,2,2,2,2,4),(-4.27012660728948,
-4.25498622149472,-4.2431578084548,-4.2351952117576,-4.22763892455177,-4.21916450486579,
-4.20605940887692,-4.15940214927043,-4.14944962827019),.UNSPECIFIED.);
#2181=B_SPLINE_CURVE_WITH_KNOTS('',3,(#42528,#42529,#42530,#42531,#42532,
#42533,#42534,#42535,#42536,#42537,#42538,#42539,#42540,#42541,#42542,#42543,
#42544,#42545,#42546,#42547,#42548,#42549,#42550,#42551,#42552,#42553,#42554,
#42555,#42556,#42557,#42558,#42559,#42560,#42561,#42562,#42563,#42564,#42565,
#42566,#42567,#42568,#42569,#42570,#42571,#42572,#42573,#42574,#42575,#42576,
#42577,#42578,#42579,#42580,#42581,#42582,#42583,#42584,#42585,#42586,#42587,
#42588,#42589,#42590,#42591,#42592,#42593,#42594,#42595,#42596,#42597,#42598,
#42599,#42600,#42601,#42602,#42603,#42604,#42605,#42606,#42607,#42608,#42609,
#42610,#42611,#42612,#42613,#42614,#42615,#42616,#42617,#42618,#42619,#42620,
#42621,#42622,#42623,#42624,#42625,#42626,#42627,#42628,#42629,#42630,#42631,
#42632,#42633,#42634,#42635,#42636,#42637,#42638,#42639,#42640,#42641,#42642,
#42643,#42644,#42645,#42646,#42647,#42648,#42649,#42650,#42651,#42652,#42653,
#42654,#42655,#42656,#42657,#42658,#42659,#42660,#42661,#42662,#42663,#42664,
#42665,#42666,#42667,#42668,#42669,#42670,#42671,#42672,#42673,#42674,#42675,
#42676,#42677,#42678,#42679,#42680,#42681,#42682,#42683,#42684,#42685,#42686,
#42687,#42688,#42689,#42690,#42691,#42692,#42693,#42694,#42695,#42696,#42697,
#42698,#42699,#42700,#42701,#42702,#42703,#42704,#42705,#42706,#42707,#42708,
#42709,#42710,#42711,#42712,#42713,#42714,#42715),.UNSPECIFIED.,.F.,.F.,
(4,2,2,2,2,2,2,2,2,2,2,2,2,2,2,2,2,2,2,2,2,2,2,2,2,2,2,2,2,2,2,2,2,2,2,
2,2,2,2,2,2,2,2,2,2,2,2,2,2,2,2,2,2,2,2,2,2,2,2,2,2,2,2,2,2,2,2,2,2,2,2,
2,2,2,2,2,2,2,2,2,2,2,2,2,2,2,2,2,2,2,2,2,2,4),(-2.25633136259072,-2.25611420428663,
-2.205423913953,-2.16234303250262,-2.13598465614483,-2.11644008911717,-2.10668226851988,
-2.09874216096065,-2.08945881864354,-2.07239176352989,-2.05049186031272,
-1.99132974510706,-1.94804750420133,-1.93954712231086,-1.93458164623434,
-1.92996190624213,-1.92311251593076,-1.90316522735521,-1.86726606648813,
-1.79258072422572,-1.77728927043214,-1.76828139901652,-1.76031273457428,
-1.75016603562434,-1.72843573570909,-1.69781336398404,-1.68354151740539,
-1.62105706991491,-1.60680803792044,-1.60116500163194,-1.59661402246382,
-1.59161776383681,-1.58297281037486,-1.5273236251959,-1.45664432114345,
-1.44100257420494,-1.43191994530131,-1.4247585915353,-1.41512072864443,
-1.39621673224777,-1.34996760181333,-1.29253993250546,-1.27215969970025,
-1.26505610757361,-1.26084977607255,-1.25609962115271,-1.24859881512431,
-1.22219843646328,-1.16090447572383,-1.11506542301896,-1.10189672705302,
-1.09340962723013,-1.08527027217187,-1.07391304283904,-1.04404545349864,
-0.993345872906739,-0.942091550420042,-0.931425399759648,-0.926013246505853,
-0.921519720914318,-0.915554771644664,-0.901847634071452,-0.881551810127337,
-0.794815563417974,-0.771899977648793,-0.761665833410531,-0.753669663013639,
-0.74481159518382,-0.729838700391571,-0.711437220831915,-0.669050121975928,
-0.604364299781365,-0.594522156343336,-0.58921608361287,-0.585161181357674,
-0.579324383659973,-0.56636677947008,-0.547612743951881,-0.478859343724038,
-0.440657941406307,-0.42811978653128,-0.419759862084431,-0.411533850779681,
-0.399691311011088,-0.365718575283084,-0.30013634393097,-0.264835119969563,
-0.256584954392791,-0.251673787837895,-0.247024098672018,-0.24001355455095,
-0.218655483690113,-0.178302679697445,-0.121704891590291),.UNSPECIFIED.);
#2182=B_SPLINE_CURVE_WITH_KNOTS('',3,(#42720,#42721,#42722,#42723,#42724,
#42725,#42726,#42727,#42728,#42729,#42730,#42731,#42732,#42733,#42734,#42735,
#42736,#42737,#42738,#42739,#42740,#42741,#42742,#42743,#42744,#42745,#42746,
#42747,#42748,#42749,#42750,#42751,#42752,#42753,#42754,#42755,#42756,#42757,
#42758,#42759,#42760,#42761,#42762,#42763,#42764,#42765,#42766,#42767,#42768,
#42769,#42770,#42771,#42772,#42773,#42774,#42775,#42776,#42777,#42778,#42779,
#42780,#42781,#42782,#42783,#42784,#42785,#42786,#42787,#42788,#42789,#42790,
#42791,#42792,#42793,#42794,#42795,#42796,#42797,#42798,#42799,#42800,#42801,
#42802,#42803,#42804,#42805,#42806,#42807,#42808,#42809,#42810,#42811,#42812,
#42813,#42814,#42815,#42816,#42817,#42818,#42819,#42820,#42821,#42822,#42823,
#42824,#42825,#42826,#42827,#42828,#42829,#42830,#42831,#42832,#42833,#42834,
#42835,#42836,#42837,#42838,#42839,#42840,#42841,#42842,#42843,#42844,#42845,
#42846,#42847,#42848,#42849,#42850,#42851,#42852,#42853,#42854,#42855,#42856,
#42857,#42858,#42859,#42860,#42861,#42862,#42863,#42864,#42865,#42866,#42867,
#42868,#42869,#42870,#42871,#42872,#42873,#42874,#42875,#42876,#42877,#42878,
#42879,#42880,#42881,#42882,#42883,#42884,#42885,#42886,#42887,#42888,#42889,
#42890,#42891,#42892,#42893,#42894,#42895,#42896,#42897,#42898,#42899,#42900,
#42901,#42902,#42903),.UNSPECIFIED.,.F.,.F.,(4,2,2,2,2,2,2,2,2,2,2,2,2,
2,2,2,2,2,2,2,2,2,2,2,2,2,2,2,2,2,2,2,2,2,2,2,2,2,2,2,2,2,2,2,2,2,2,2,2,
2,2,2,2,2,2,2,2,2,2,2,2,2,2,2,2,2,2,2,2,2,2,2,2,2,2,2,2,2,2,2,2,2,2,2,2,
2,2,2,2,2,2,4),(-4.14974432138309,-4.14846791814416,-4.1036272995958,-4.06490612048757,
-4.02002009343704,-4.00721019973488,-3.99879533019438,-3.99070270227857,
-3.98096668996061,-3.95676135527686,-3.87233139240616,-3.85220164525164,
-3.8385725713699,-3.83262037532498,-3.82812741643513,-3.82270495771739,
-3.81231492892195,-3.75560081303903,-3.70844624827614,-3.67978042381591,
-3.66857943454785,-3.66046607618611,-3.65192989614318,-3.63852280614711,
-3.58554570844267,-3.53810888423012,-3.51659395565881,-3.5023126293188,
-3.49625301678665,-3.49179090280551,-3.48646252704252,-3.47651771098314,
-3.40002224132401,-3.35174657283295,-3.33641956993802,-3.32748836299764,
-3.31950735118771,-3.3092333136485,-3.28674614761279,-3.19948611351233,
-3.17916142907747,-3.16543945796852,-3.15947192283691,-3.15497800549799,
-3.14956737735978,-3.13890959644952,-3.08732629807925,-3.03780055198441,
-3.01704952850813,-3.00065677860689,-2.9915085673212,-2.98355858826363,
-2.97362552027617,-2.95311262981357,-2.87784506758503,-2.83415859324948,
-2.82571944116168,-2.82076723188937,-2.81619466980269,-2.80935277403457,
-2.79098031407557,-2.73190392937765,-2.6749448647585,-2.66151274274947,
-2.65297151067771,-2.64486094521406,-2.63367614088364,-2.60689082964362,
-2.5255895245627,-2.50569357709456,-2.49217677593529,-2.48624347676095,
-2.4817519106473,-2.47631532209191,-2.46585759553819,-2.41047929418916,
-2.36248768990101,-2.33352931465428,-2.32228939467599,-2.31416948994504,
-2.30564563992768,-2.29229898705041,-2.24199412460632,-2.18466667900874,
-2.15904915059887,-2.15161610823454,-2.14688006467059,-2.1426626170076,
-2.13549867704365,-2.11270638785466,-2.06733228386177,-2.01490391173078),
 .UNSPECIFIED.);
#2183=B_SPLINE_CURVE_WITH_KNOTS('',3,(#42905,#42906,#42907,#42908,#42909,
#42910,#42911,#42912,#42913,#42914,#42915,#42916,#42917,#42918,#42919,#42920,
#42921,#42922),.UNSPECIFIED.,.F.,.F.,(4,2,2,2,2,2,2,2,4),(-0.121704891590291,
-0.11342614004661,-0.0976371836018917,-0.0877231932451925,-0.0797752166259034,
-0.0706147557324629,-0.0609728232183739,-0.0409692035001258,-0.000968868351203119),
 .UNSPECIFIED.);
#2184=B_SPLINE_CURVE_WITH_KNOTS('',3,(#42923,#42924,#42925,#42926,#42927,
#42928,#42929,#42930,#42931,#42932,#42933,#42934,#42935,#42936,#42937,#42938,
#42939,#42940,#42941,#42942,#42943,#42944,#42945,#42946,#42947,#42948,#42949,
#42950,#42951,#42952,#42953,#42954,#42955,#42956,#42957,#42958,#42959,#42960,
#42961,#42962,#42963,#42964,#42965,#42966,#42967,#42968,#42969,#42970,#42971,
#42972,#42973,#42974,#42975,#42976,#42977,#42978,#42979,#42980,#42981,#42982,
#42983,#42984,#42985,#42986,#42987,#42988,#42989,#42990,#42991,#42992,#42993,
#42994,#42995,#42996,#42997,#42998,#42999,#43000,#43001,#43002,#43003,#43004,
#43005,#43006,#43007,#43008,#43009,#43010,#43011,#43012,#43013,#43014,#43015,
#43016,#43017,#43018,#43019,#43020,#43021,#43022,#43023,#43024,#43025,#43026,
#43027,#43028,#43029,#43030,#43031,#43032,#43033,#43034,#43035,#43036,#43037,
#43038,#43039,#43040,#43041,#43042,#43043,#43044,#43045,#43046,#43047,#43048,
#43049,#43050,#43051,#43052,#43053,#43054,#43055,#43056,#43057,#43058,#43059,
#43060,#43061,#43062,#43063,#43064,#43065,#43066,#43067,#43068,#43069,#43070,
#43071,#43072,#43073,#43074,#43075,#43076,#43077,#43078,#43079,#43080,#43081,
#43082,#43083,#43084,#43085,#43086,#43087,#43088,#43089,#43090,#43091,#43092,
#43093,#43094,#43095,#43096,#43097,#43098,#43099,#43100),.UNSPECIFIED.,
 .F.,.F.,(4,2,2,2,2,2,2,2,2,2,2,2,2,2,2,2,2,2,2,2,2,2,2,2,2,2,2,2,2,2,2,
2,2,2,2,2,2,2,2,2,2,2,2,2,2,2,2,2,2,2,2,2,2,2,2,2,2,2,2,2,2,2,2,2,2,2,2,
2,2,2,2,2,2,2,2,2,2,2,2,2,2,2,2,2,2,2,2,2,4),(-4.27047542831303,-4.2028023511958,
-4.19484108710681,-4.1880475844779,-4.18343780883772,-4.17845196673257,
-4.16985735720432,-4.11993171814948,-4.06570981841995,-4.04470792430685,
-4.02816651065322,-4.01898762311436,-4.01103937520636,-4.00114554164588,
-3.9808561284274,-3.89058365570733,-3.87006317533269,-3.85624731979524,
-3.85026343488629,-3.84576741756672,-3.84036672789001,-3.82976259748566,
-3.77483604142693,-3.72654571371871,-3.69748263550418,-3.68622794122822,
-3.67810474517564,-3.66958397342759,-3.65625605077966,-3.60666091536594,
-3.54871575368378,-3.52297016480168,-3.51552516790668,-3.51078619120127,
-3.50656998205983,-3.49941491668109,-3.47861923074858,-3.41460643206202,
-3.38148303174929,-3.35855263437229,-3.34820363271455,-3.34021273237256,
-3.33131969027148,-3.31618422149891,-3.23867249433833,-3.20435376611551,
-3.18494143175752,-3.1781564394202,-3.17354813118027,-3.16855903212778,
-3.1599495016037,-3.10970432333238,-3.06868702967458,-3.02723215719761,
-3.01467854240712,-3.00631391868362,-2.99818297232946,-2.98829361080563,
-2.96335366835513,-2.87994817748842,-2.8598910227536,-2.84629619300653,
-2.84034924079151,-2.83585611403274,-2.8304283907749,-2.82001532402029,
-2.76369406971441,-2.71628420232577,-2.68752692754953,-2.67631270100351,
-2.66819625783259,-2.65966261957234,-2.64627192651873,-2.59416504461488,
-2.54574443551906,-2.52426462729073,-2.50999897537829,-2.50394137708579,
-2.49943884997888,-2.49408948254307,-2.48404809314821,-2.40804882580328,
-2.37293413781144,-2.34908870617247,-2.3385919604751,-2.33058339815916,
-2.32176676297337,-2.30700060463983,-2.25618542829049),.UNSPECIFIED.);
#2185=B_SPLINE_CURVE_WITH_KNOTS('',3,(#43106,#43107,#43108,#43109,#43110,
#43111,#43112,#43113,#43114,#43115,#43116,#43117,#43118,#43119,#43120,#43121,
#43122,#43123,#43124,#43125,#43126,#43127,#43128,#43129,#43130,#43131,#43132,
#43133,#43134,#43135,#43136,#43137,#43138,#43139,#43140,#43141,#43142,#43143,
#43144,#43145,#43146,#43147,#43148,#43149,#43150,#43151,#43152,#43153,#43154,
#43155,#43156,#43157,#43158,#43159,#43160,#43161,#43162,#43163,#43164,#43165,
#43166,#43167,#43168,#43169,#43170,#43171,#43172,#43173,#43174,#43175,#43176,
#43177,#43178,#43179,#43180,#43181,#43182,#43183,#43184,#43185,#43186,#43187,
#43188,#43189,#43190,#43191,#43192,#43193,#43194,#43195,#43196,#43197,#43198,
#43199,#43200,#43201,#43202,#43203,#43204,#43205,#43206,#43207,#43208,#43209,
#43210,#43211,#43212,#43213,#43214,#43215,#43216,#43217,#43218,#43219,#43220,
#43221,#43222,#43223,#43224,#43225,#43226,#43227,#43228,#43229,#43230,#43231,
#43232,#43233,#43234,#43235,#43236,#43237,#43238,#43239,#43240,#43241,#43242,
#43243,#43244,#43245,#43246,#43247,#43248,#43249,#43250,#43251,#43252,#43253,
#43254,#43255,#43256,#43257,#43258,#43259,#43260,#43261,#43262,#43263,#43264,
#43265,#43266,#43267,#43268,#43269,#43270,#43271,#43272,#43273,#43274,#43275,
#43276,#43277,#43278,#43279,#43280,#43281,#43282,#43283,#43284,#43285),
 .UNSPECIFIED.,.F.,.F.,(4,2,2,2,2,2,2,2,2,2,2,2,2,2,2,2,2,2,2,2,2,2,2,2,
2,2,2,2,2,2,2,2,2,2,2,2,2,2,2,2,2,2,2,2,2,2,2,2,2,2,2,2,2,2,2,2,2,2,2,2,
2,2,2,2,2,2,2,2,2,2,2,2,2,2,2,2,2,2,2,2,2,2,2,2,2,2,2,2,2,4),(-2.01554578796151,
-1.97103123005403,-1.93097181759248,-1.92253513746472,-1.91758303054684,
-1.9129553724187,-1.90606508035253,-1.88577498368381,-1.84883727333426,
-1.77593475546572,-1.76046564052153,-1.75141901115537,-1.74425187666022,
-1.73456174434985,-1.71538463815053,-1.66594597785084,-1.60238378534787,
-1.58894412989728,-1.58308620274509,-1.57859231117078,-1.57317410730551,
-1.56248042901183,-1.51978089673919,-1.43700366905451,-1.42258772503365,
-1.41384341047713,-1.40581415108061,-1.39516198893724,-1.37032201041875,
-1.33295478886762,-1.27558186874864,-1.25512205871348,-1.24800824509256,
-1.24379977332218,-1.23905147948378,-1.23156093796387,-1.20528740017942,
-1.14467072668409,-1.09807316746509,-1.0848632965148,-1.07636721830375,
-1.06823170834232,-1.05690056197673,-1.02724233745582,-0.977184103456037,
-0.925077313692892,-0.914361436720255,-0.908939171293729,-0.904446196472628,
-0.898493654406605,-0.884862827502424,-0.864727554532776,-0.780313496705148,
-0.756139403078319,-0.746367819413911,-0.738266688958129,-0.729864493060608,
-0.717117419951956,-0.673105607219358,-0.633796923416527,-0.588642416944584,
-0.577838773629542,-0.572399576055189,-0.567908660094148,-0.561979783383725,
-0.548487716707292,-0.528640596521868,-0.448026995938828,-0.420686381152166,
-0.409393112258311,-0.401345376190143,-0.392858894504195,-0.379692361252308,
-0.328859248556321,-0.259893106967106,-0.243977875884682,-0.237505865760107,
-0.232951017645036,-0.22783466941652,-0.218621332049285,-0.206785395676726,
-0.165911353814076,-0.0971919190351272,-0.0808855130853292,-0.0708260347570257,
-0.0628665444576238,-0.0553961706292034,-0.0464698457397591,-0.0292329749492484,
-0.000968449818818451),.UNSPECIFIED.);
#2186=B_SPLINE_CURVE_WITH_KNOTS('',3,(#43286,#43287,#43288,#43289,#43290,
#43291,#43292,#43293,#43294,#43295,#43296,#43297,#43298,#43299,#43300,#43301),
 .UNSPECIFIED.,.F.,.F.,(4,2,2,2,2,2,2,4),(-4.26995744812625,-4.20854418514327,
-4.18863575523228,-4.17511314825444,-4.16917905860353,-4.16468764681411,
-4.15925216914881,-4.14974432138309),.UNSPECIFIED.);
#2187=B_SPLINE_CURVE_WITH_KNOTS('',3,(#43302,#43303,#43304,#43305,#43306,
#43307,#43308,#43309,#43310,#43311,#43312,#43313,#43314,#43315,#43316,#43317,
#43318,#43319,#43320,#43321,#43322,#43323,#43324,#43325,#43326,#43327,#43328,
#43329,#43330,#43331,#43332,#43333,#43334,#43335,#43336,#43337,#43338,#43339,
#43340,#43341,#43342,#43343,#43344,#43345,#43346,#43347,#43348,#43349,#43350,
#43351,#43352,#43353,#43354,#43355,#43356,#43357,#43358,#43359,#43360,#43361,
#43362,#43363,#43364,#43365,#43366,#43367,#43368,#43369,#43370,#43371,#43372,
#43373,#43374,#43375,#43376,#43377,#43378,#43379,#43380,#43381,#43382,#43383,
#43384,#43385,#43386,#43387,#43388,#43389,#43390,#43391,#43392,#43393,#43394,
#43395,#43396,#43397,#43398,#43399,#43400,#43401,#43402,#43403,#43404,#43405,
#43406,#43407,#43408,#43409,#43410,#43411,#43412,#43413,#43414,#43415,#43416,
#43417,#43418,#43419,#43420,#43421,#43422,#43423,#43424,#43425,#43426,#43427,
#43428,#43429,#43430,#43431,#43432,#43433,#43434,#43435,#43436,#43437,#43438,
#43439,#43440,#43441,#43442,#43443,#43444,#43445,#43446,#43447,#43448,#43449,
#43450,#43451,#43452,#43453,#43454,#43455,#43456,#43457,#43458,#43459,#43460,
#43461,#43462,#43463,#43464,#43465,#43466,#43467,#43468,#43469,#43470,#43471,
#43472,#43473,#43474,#43475,#43476,#43477,#43478,#43479,#43480,#43481,#43482,
#43483,#43484,#43485,#43486,#43487,#43488,#43489,#43490,#43491,#43492,#43493,
#43494,#43495),.UNSPECIFIED.,.F.,.F.,(4,2,2,2,2,2,2,2,2,2,2,2,2,2,2,2,2,
2,2,2,2,2,2,2,2,2,2,2,2,2,2,2,2,2,2,2,2,2,2,2,2,2,2,2,2,2,2,2,2,2,2,2,2,
2,2,2,2,2,2,2,2,2,2,2,2,2,2,2,2,2,2,2,2,2,2,2,2,2,2,2,2,2,2,2,2,2,2,2,2,
2,2,2,2,2,2,2,4),(-2.25618542829049,-2.22672059863037,-2.17859210143867,
-2.17004222970896,-2.1650659111468,-2.16050470499341,-2.1537283333742,-2.13582650511268,
-2.10482854960935,-2.02452735676493,-2.00839162929354,-1.99920282934488,
-1.99125547618372,-1.98137508075322,-1.96116015673039,-1.88631530576674,
-1.84185274236897,-1.83334533127237,-1.82837806589094,-1.82375862046547,
-1.81691246100755,-1.79699563439922,-1.76118995674109,-1.68632661276455,
-1.67087182616814,-1.66191321567541,-1.65393533907042,-1.64370383577268,
-1.62147822395032,-1.58984011650555,-1.55252263692881,-1.50903851142576,
-1.49832301054929,-1.49290059266807,-1.48840728803549,-1.48245404131109,
-1.46882050516715,-1.44868013474766,-1.36420813090703,-1.33999353643743,
-1.33025560499249,-1.32216220690252,-1.31374734055386,-1.30093900636659,
-1.25607154766657,-1.21736994013372,-1.17254908536673,-1.16176587002138,
-1.15633043915348,-1.15183882155036,-1.14590404961739,-1.13237857279693,
-1.11246265301048,-1.0309829314971,-1.00430736412699,-0.993138841805342,
-0.985031121717851,-0.976484888847862,-0.963027568594057,-0.905270167198867,
-0.844756859122124,-0.828154058201975,-0.82157301903771,-0.817000569930036,
-0.811932286096004,-0.802947933605645,-0.79149704777724,-0.764618230914736,
-0.675965070528053,-0.660824581060035,-0.651931904544749,-0.643943374134029,
-0.63360032557256,-0.610695460654489,-0.577625649227347,-0.513832000422512,
-0.492876160719128,-0.485703479298056,-0.481484818892183,-0.476751726807192,
-0.469330506797591,-0.443841535130703,-0.387137730974593,-0.33602256950956,
-0.322670478763516,-0.314146339563308,-0.306028421477061,-0.294794925446189,
-0.265875084129225,-0.21798950604371,-0.162533150278821,-0.152084654529271,
-0.146650504880891,-0.142159549066541,-0.136225133701574,-0.122698376414465,
-0.121351841344903),.UNSPECIFIED.);
#2188=B_SPLINE_CURVE_WITH_KNOTS('',3,(#43500,#43501,#43502,#43503,#43504,
#43505,#43506,#43507,#43508,#43509,#43510,#43511,#43512,#43513,#43514,#43515,
#43516,#43517,#43518,#43519,#43520,#43521,#43522,#43523,#43524,#43525,#43526,
#43527,#43528,#43529,#43530,#43531,#43532,#43533,#43534,#43535,#43536,#43537,
#43538,#43539,#43540,#43541,#43542,#43543,#43544,#43545,#43546,#43547,#43548,
#43549,#43550,#43551,#43552,#43553,#43554,#43555,#43556,#43557,#43558,#43559,
#43560,#43561,#43562,#43563,#43564,#43565,#43566,#43567,#43568,#43569,#43570,
#43571,#43572,#43573,#43574,#43575,#43576,#43577,#43578,#43579,#43580,#43581,
#43582,#43583,#43584,#43585,#43586,#43587,#43588,#43589,#43590,#43591,#43592,
#43593,#43594,#43595,#43596,#43597,#43598,#43599,#43600,#43601,#43602,#43603,
#43604,#43605,#43606,#43607,#43608,#43609,#43610,#43611,#43612,#43613,#43614,
#43615,#43616,#43617,#43618,#43619,#43620,#43621,#43622,#43623,#43624,#43625,
#43626,#43627,#43628,#43629,#43630,#43631,#43632,#43633,#43634,#43635,#43636,
#43637,#43638,#43639,#43640,#43641,#43642,#43643,#43644,#43645,#43646,#43647,
#43648,#43649,#43650,#43651,#43652,#43653,#43654,#43655,#43656,#43657,#43658,
#43659,#43660,#43661,#43662,#43663,#43664,#43665,#43666,#43667,#43668,#43669,
#43670,#43671,#43672,#43673,#43674,#43675,#43676,#43677,#43678,#43679,#43680,
#43681,#43682,#43683,#43684,#43685,#43686,#43687,#43688,#43689,#43690,#43691),
 .UNSPECIFIED.,.F.,.F.,(4,2,2,2,2,2,2,2,2,2,2,2,2,2,2,2,2,2,2,2,2,2,2,2,
2,2,2,2,2,2,2,2,2,2,2,2,2,2,2,2,2,2,2,2,2,2,2,2,2,2,2,2,2,2,2,2,2,2,2,2,
2,2,2,2,2,2,2,2,2,2,2,2,2,2,2,2,2,2,2,2,2,2,2,2,2,2,2,2,2,2,2,2,2,2,2,4),
(-4.15046929847984,-4.13270632885826,-4.11676300793453,-4.10770559221249,
-4.09974473951702,-4.08967792181627,-4.06840763326063,-3.99397118374691,
-3.95398662443728,-3.94359230127021,-3.93823371708984,-3.93373316049068,
-3.92779520758228,-3.91442227744894,-3.85092751156094,-3.83634860473377,
-3.79028711258421,-3.77739761162911,-3.76896663538752,-3.76088437034561,
-3.75119214915331,-3.72727135145519,-3.6561071401658,-3.61720744870898,
-3.60693711676568,-3.6016032777906,-3.59709899907138,-3.59112497792671,
-3.57754808483821,-3.51424339085961,-3.46489198826929,-3.44574486133427,
-3.43606094823155,-3.42889512652169,-3.41984579887042,-3.40436097570136,
-3.33172920355803,-3.27846586088945,-3.26945068362377,-3.26437556346478,
-3.25980512841828,-3.25427457441599,-3.24071306075823,-3.17755239429721,
-3.11833702358862,-3.10483235243416,-3.09627598443772,-3.08817244092739,
-3.07703195171029,-3.05057882524173,-2.96888036571166,-2.94895304253389,
-2.93542094903084,-2.92948489351571,-2.92499293441597,-2.91955794913335,
-2.9087779040026,-2.86402239904391,-2.82553399446278,-2.78035124686849,
-2.76751992338799,-2.75910017209899,-2.75100944876956,-2.74128375303232,
-2.71714947473425,-2.63261651967047,-2.61247798609605,-2.5988443072636,
-2.59289097345053,-2.5883975256516,-2.5829749302194,-2.57225894499987,-2.52879278673367,
-2.49154160446548,-2.45980931837968,-2.43753966588343,-2.42730052285845,
-2.41932172725802,-2.41036730867661,-2.39493327852405,-2.31993857812761,
-2.28424424806978,-2.26436431862397,-2.25752265618995,-2.25290397393512,
-2.24793507666022,-2.23942009929252,-2.19358185224284,-2.13627473018799,
-2.10496524348096,-2.09311431952685,-2.08570710035488,-2.07749817419153,
-2.06575720536979,-2.03271675136986,-2.01554578796151),.UNSPECIFIED.);
#2189=B_SPLINE_CURVE_WITH_KNOTS('',3,(#43693,#43694,#43695,#43696,#43697,
#43698,#43699,#43700),.UNSPECIFIED.,.F.,.F.,(4,2,2,4),(-0.121351841344903,
-0.102778514164449,-0.0579874682746311,-0.00096969038325926),
 .UNSPECIFIED.);
#2190=B_SPLINE_CURVE_WITH_KNOTS('',3,(#43701,#43702,#43703,#43704,#43705,
#43706,#43707,#43708,#43709,#43710,#43711,#43712,#43713,#43714,#43715,#43716,
#43717,#43718,#43719,#43720,#43721,#43722,#43723,#43724,#43725,#43726,#43727,
#43728,#43729,#43730,#43731,#43732,#43733,#43734,#43735,#43736,#43737,#43738,
#43739,#43740,#43741,#43742,#43743,#43744,#43745,#43746,#43747,#43748,#43749,
#43750,#43751,#43752,#43753,#43754,#43755,#43756,#43757,#43758,#43759,#43760,
#43761,#43762,#43763,#43764,#43765,#43766,#43767,#43768,#43769,#43770,#43771,
#43772,#43773,#43774,#43775,#43776,#43777,#43778,#43779,#43780,#43781,#43782,
#43783,#43784,#43785,#43786,#43787,#43788,#43789,#43790,#43791,#43792,#43793,
#43794,#43795,#43796,#43797,#43798,#43799,#43800,#43801,#43802,#43803,#43804,
#43805,#43806,#43807,#43808,#43809,#43810,#43811,#43812,#43813,#43814,#43815,
#43816,#43817,#43818,#43819,#43820,#43821,#43822,#43823,#43824,#43825,#43826,
#43827,#43828,#43829,#43830,#43831,#43832,#43833,#43834,#43835,#43836,#43837,
#43838,#43839,#43840,#43841,#43842,#43843,#43844,#43845,#43846,#43847,#43848,
#43849,#43850,#43851,#43852,#43853,#43854,#43855,#43856,#43857,#43858,#43859,
#43860,#43861,#43862,#43863,#43864,#43865,#43866,#43867,#43868,#43869,#43870,
#43871,#43872,#43873,#43874,#43875,#43876,#43877,#43878,#43879,#43880,#43881,
#43882,#43883,#43884,#43885,#43886,#43887,#43888,#43889,#43890,#43891,#43892,
#43893,#43894,#43895,#43896,#43897,#43898,#43899),.UNSPECIFIED.,.F.,.F.,
(4,3,3,3,3,3,3,3,3,3,3,3,3,3,3,3,3,3,3,3,3,3,3,3,3,3,3,3,3,3,3,3,3,3,3,
3,3,3,3,3,3,3,3,3,3,3,3,3,3,3,3,3,3,3,3,3,3,3,3,3,3,3,3,3,3,3,4),(-16.4167960594917,
-16.3231866235391,-16.229526884803,-16.1346626699223,-16.0407807148777,
-15.945425370079,-15.8500700252804,-15.7580593298291,-15.6661696621795,
-15.5743745707618,-15.4826447796861,-15.3909489505947,-15.2992633145047,
-15.2075641168384,-15.1157697393271,-15.0239260435727,-14.9319324069844,
-14.8594406487004,-14.7674299218298,-14.6755402224228,-14.5837450989567,
-14.4920152755291,-14.400319413912,-14.3086337451621,-14.2169345147419,
-14.1251401045348,-14.0332963760681,-13.941302707081,-13.8688112721204,
-13.7768007117943,-13.6849111792182,-13.5931162226491,-13.5013865655354,
-13.4096908698183,-13.3180053663597,-13.2263063004262,-13.1345120524464,
-13.0426684851999,-12.9506749741105,-12.8781818955404,-12.7861710919384,
-12.6942813168831,-12.602486118933,-12.5107562230586,-12.4190602902644,
-12.3273745516834,-12.2356752528554,-12.1438807768566,-12.0520369839466,
-11.9600432533881,-11.8875525189603,-11.7955415542391,-11.7036516150329,
-11.6118562501565,-11.5201261839085,-11.4284300786933,-11.3367441658633,
-11.2450446911762,-11.1532500379329,-11.0614060667469,-10.9694121580842,
-10.8969231423803,-10.8060912012837,-10.715400234171,-10.6247905958859,
-10.5342411065541,-10.4882942077004),.UNSPECIFIED.);
#2191=B_SPLINE_CURVE_WITH_KNOTS('',3,(#43905,#43906,#43907,#43908,#43909,
#43910,#43911,#43912,#43913,#43914,#43915,#43916,#43917,#43918,#43919,#43920,
#43921,#43922,#43923,#43924,#43925,#43926,#43927,#43928,#43929,#43930,#43931,
#43932,#43933,#43934,#43935,#43936,#43937,#43938,#43939,#43940,#43941,#43942,
#43943,#43944,#43945,#43946,#43947,#43948,#43949,#43950,#43951,#43952,#43953,
#43954,#43955,#43956,#43957,#43958,#43959,#43960,#43961,#43962,#43963,#43964,
#43965,#43966,#43967,#43968,#43969,#43970,#43971,#43972,#43973,#43974,#43975,
#43976,#43977,#43978,#43979,#43980,#43981,#43982,#43983,#43984,#43985,#43986,
#43987,#43988,#43989,#43990,#43991,#43992,#43993,#43994,#43995,#43996,#43997,
#43998,#43999,#44000,#44001,#44002,#44003,#44004,#44005,#44006,#44007,#44008,
#44009,#44010,#44011,#44012,#44013,#44014,#44015,#44016,#44017,#44018,#44019,
#44020,#44021,#44022,#44023,#44024,#44025,#44026,#44027,#44028,#44029,#44030,
#44031,#44032),.UNSPECIFIED.,.F.,.F.,(4,2,2,2,2,2,2,2,2,2,2,2,2,2,2,2,2,
2,2,2,2,2,2,2,2,2,2,2,2,2,2,2,2,2,2,2,2,2,2,2,2,2,2,2,2,2,2,2,2,2,2,2,2,
2,2,2,2,2,2,2,2,2,2,4),(0.000239016707890752,0.00315166214361164,0.00671773766773776,
0.0169827679766186,0.0635487110239646,0.112156318829945,0.129455895946306,
0.143873315375382,0.153203387882427,0.162137432678307,0.17287716353032,
0.194033657182551,0.272985524325323,0.305915699365059,0.325078614379287,
0.331875706730879,0.336498161130002,0.341361930413961,0.349714073947605,
0.393602958573611,0.468743405451748,0.487751158624623,0.497184420264035,
0.504820517838277,0.51368934223756,0.52931039522351,0.619175633277945,0.658185238232473,
0.66828046524847,0.673409994408688,0.677833605850783,0.683613544369486,
0.696660790620161,0.760790654083829,0.81077497077889,0.830124034941486,
0.839900410017414,0.84713465343804,0.856274490851527,0.871948121460915,
0.937828225154308,0.977392726828777,0.998489503837954,1.00554079075414,
1.01025533116603,1.01525251794431,1.02378236126374,1.06622533685266,1.12577146809519,
1.14774179735986,1.16486129990916,1.17418522605343,1.18216887676668,1.19199345952817,
1.21172904406483,1.3030291436912,1.32364860922065,1.3375215734021,1.34352735342838,
1.34802717493649,1.35340521592046,1.36395766346144,1.41960965183253,1.42897696838616),
 .UNSPECIFIED.);
#2192=B_SPLINE_CURVE_WITH_KNOTS('',3,(#44035,#44036,#44037,#44038,#44039,
#44040,#44041,#44042,#44043,#44044,#44045,#44046,#44047,#44048,#44049,#44050,
#44051,#44052,#44053,#44054,#44055,#44056,#44057,#44058,#44059,#44060,#44061,
#44062,#44063,#44064,#44065,#44066,#44067,#44068,#44069,#44070,#44071,#44072,
#44073,#44074,#44075,#44076,#44077,#44078,#44079,#44080,#44081,#44082,#44083,
#44084,#44085,#44086,#44087,#44088,#44089,#44090,#44091,#44092,#44093,#44094,
#44095,#44096,#44097,#44098,#44099,#44100,#44101,#44102,#44103,#44104,#44105,
#44106,#44107,#44108,#44109,#44110,#44111,#44112,#44113,#44114,#44115,#44116,
#44117,#44118,#44119,#44120,#44121,#44122,#44123,#44124,#44125,#44126,#44127,
#44128,#44129,#44130,#44131,#44132,#44133,#44134,#44135,#44136,#44137,#44138,
#44139,#44140,#44141,#44142,#44143,#44144,#44145,#44146,#44147,#44148,#44149,
#44150,#44151,#44152,#44153,#44154,#44155,#44156,#44157,#44158,#44159,#44160,
#44161,#44162,#44163,#44164,#44165,#44166,#44167,#44168,#44169,#44170,#44171,
#44172,#44173,#44174,#44175,#44176,#44177,#44178,#44179,#44180,#44181,#44182,
#44183,#44184,#44185,#44186,#44187,#44188,#44189,#44190,#44191,#44192,#44193,
#44194,#44195,#44196,#44197,#44198,#44199,#44200,#44201,#44202,#44203,#44204,
#44205,#44206,#44207,#44208,#44209,#44210),.UNSPECIFIED.,.F.,.F.,(4,2,2,
2,2,2,2,2,2,2,2,2,2,2,2,2,2,2,2,2,2,2,2,2,2,2,2,2,2,2,2,2,2,2,2,2,2,2,2,
2,2,2,2,2,2,2,2,2,2,2,2,2,2,2,2,2,2,2,2,2,2,2,2,2,2,2,2,2,2,2,2,2,2,2,2,
2,2,2,2,2,2,2,2,2,2,2,2,4),(-4.02414899437559,-4.01725069329091,-3.95119121645565,
-3.91323211790503,-3.88805516392213,-3.8772911778161,-3.86918427641931,
-3.86035722164114,-3.84579108688948,-3.76660016120897,-3.72368939308642,
-3.71292566437222,-3.70743568028743,-3.70287775078405,-3.696902579107,-3.68292552867492,
-3.61991469360162,-3.57106522667542,-3.55179493283753,-3.54205679910813,
-3.5348516529627,-3.52575184739845,-3.51017381466984,-3.4378738824274,-3.40050153883197,
-3.38005104542205,-3.3731274348465,-3.36848553490925,-3.36355630707564,
-3.35517047884301,-3.31607714363579,-3.25353266158283,-3.22030437544304,
-3.20857732616469,-3.2004021206995,-3.19207149277192,-3.17953784307398,
-3.14109450170882,-3.07216486309444,-3.04444276755788,-3.03685934018612,
-3.03210961014489,-3.02792601811024,-3.02094000648734,-3.00149302970198,
-2.94326284724269,-2.89129340084666,-2.87545999123913,-2.86641684277024,
-2.85844052559617,-2.84831529139372,-2.82675364675384,-2.73854237802906,
-2.71816695693039,-2.70441754302905,-2.69843704402835,-2.69393450153278,
-2.6885146518464,-2.67815042909065,-2.62021754296784,-2.57388348214683,
-2.54551001820523,-2.53434543589075,-2.52623522438772,-2.51768143347307,
-2.50420134075086,-2.44897165951614,-2.39572951484344,-2.37098968375173,
-2.36363509616993,-2.35891506173386,-2.35468603588276,-2.34745279183694,
-2.32596393102289,-2.26935087648644,-2.21378315056379,-2.2004061807555,
-2.19187937311335,-2.18376834674631,-2.17256016371868,-2.14563307218365,
-2.0644695723789,-2.04458371551823,-2.03107289414446,-2.02514274496808,
-2.02065276747142,-2.01521677086951,-2.01510602195132),.UNSPECIFIED.);
#2193=B_SPLINE_CURVE_WITH_KNOTS('',3,(#44216,#44217,#44218,#44219,#44220,
#44221,#44222,#44223,#44224,#44225,#44226,#44227,#44228,#44229,#44230,#44231,
#44232,#44233,#44234,#44235,#44236,#44237,#44238,#44239,#44240,#44241,#44242,
#44243,#44244,#44245,#44246,#44247,#44248,#44249,#44250,#44251,#44252,#44253,
#44254,#44255,#44256,#44257,#44258,#44259,#44260,#44261,#44262,#44263,#44264,
#44265,#44266,#44267,#44268,#44269,#44270,#44271,#44272,#44273,#44274,#44275,
#44276,#44277,#44278,#44279,#44280,#44281,#44282,#44283,#44284,#44285,#44286,
#44287,#44288,#44289,#44290,#44291,#44292,#44293,#44294,#44295,#44296,#44297,
#44298,#44299,#44300,#44301,#44302,#44303,#44304,#44305,#44306,#44307,#44308,
#44309,#44310,#44311,#44312,#44313,#44314,#44315,#44316,#44317,#44318,#44319,
#44320,#44321,#44322,#44323,#44324,#44325,#44326,#44327,#44328,#44329,#44330,
#44331,#44332,#44333,#44334,#44335,#44336,#44337,#44338,#44339,#44340,#44341,
#44342,#44343,#44344,#44345,#44346,#44347,#44348,#44349,#44350,#44351,#44352,
#44353,#44354,#44355,#44356,#44357,#44358,#44359,#44360),.UNSPECIFIED.,
 .F.,.F.,(4,3,3,3,3,3,3,3,3,3,3,3,3,3,3,3,3,3,3,3,3,3,3,3,3,3,3,3,3,3,3,
3,3,3,3,3,3,3,3,3,3,3,3,3,3,3,3,3,4),(74.4826134639429,74.5701017210815,
74.6575411968586,74.7449559528723,74.8323667521485,74.9197943499317,75.0073142166116,
75.0948813813697,75.1825901309915,75.2578179239381,75.3457884273519,75.4336478048373,
75.5214188779625,75.612297430782,75.6999676523823,75.78762386132,75.8752865504186,
75.9629762119858,76.0507600100425,76.1385998960894,76.2265621785653,76.2484473005182,
76.3363314594677,76.4241063946703,76.5117950016086,76.6027052110448,76.6902983576817,
76.7778796066848,76.8654695235803,76.9530886749992,77.0408056385432,77.1285807561576,
77.2164817566519,77.2390766770982,77.3260771415733,77.412966501338,77.4997686274976,
77.5910108057702,77.6777204878012,77.7644207287209,77.8511329515665,77.9378785848385,
78.0247325806727,78.1116496986136,78.1987067829138,78.2297060536782,78.3416517190473,
78.4517369676243,78.5398162006367),.UNSPECIFIED.);
#2194=B_SPLINE_CURVE_WITH_KNOTS('',3,(#44362,#44363,#44364,#44365),
 .UNSPECIFIED.,.F.,.F.,(4,4),(78.5398163397448,79.2203354302583),
 .UNSPECIFIED.);
#2195=B_SPLINE_CURVE_WITH_KNOTS('',3,(#44369,#44370,#44371,#44372,#44373,
#44374,#44375,#44376,#44377,#44378,#44379,#44380,#44381,#44382,#44383,#44384,
#44385,#44386,#44387,#44388,#44389,#44390,#44391,#44392,#44393,#44394,#44395,
#44396,#44397,#44398,#44399,#44400,#44401,#44402,#44403,#44404,#44405,#44406,
#44407,#44408,#44409,#44410,#44411),.UNSPECIFIED.,.F.,.F.,(4,3,3,3,3,3,
3,3,3,3,3,3,3,3,4),(78.5398163398759,78.6511924917076,78.7647307704921,
78.7900351244193,78.8773825896874,78.9646210658141,79.0517740756938,79.1388674668699,
79.2259295154673,79.3129813583285,79.4000441200288,79.4871929619449,79.5743845951527,
79.6617164564392,79.7442523245248),.UNSPECIFIED.);
#2196=B_SPLINE_CURVE_WITH_KNOTS('',3,(#44412,#44413,#44414,#44415,#44416,
#44417,#44418,#44419,#44420,#44421,#44422,#44423,#44424,#44425,#44426,#44427,
#44428,#44429,#44430,#44431,#44432,#44433,#44434,#44435,#44436,#44437,#44438,
#44439,#44440,#44441,#44442,#44443,#44444,#44445,#44446,#44447,#44448,#44449,
#44450,#44451,#44452,#44453,#44454,#44455,#44456,#44457,#44458,#44459,#44460,
#44461,#44462,#44463,#44464,#44465,#44466,#44467,#44468,#44469,#44470,#44471,
#44472,#44473,#44474,#44475,#44476,#44477,#44478,#44479,#44480,#44481,#44482,
#44483,#44484,#44485,#44486,#44487,#44488,#44489,#44490,#44491,#44492,#44493,
#44494,#44495,#44496,#44497,#44498,#44499,#44500,#44501,#44502,#44503,#44504,
#44505,#44506,#44507,#44508,#44509,#44510,#44511,#44512,#44513,#44514,#44515,
#44516,#44517,#44518,#44519,#44520,#44521,#44522,#44523,#44524,#44525,#44526,
#44527,#44528,#44529,#44530,#44531,#44532,#44533,#44534,#44535,#44536,#44537,
#44538,#44539,#44540,#44541,#44542,#44543,#44544,#44545,#44546,#44547,#44548,
#44549,#44550,#44551,#44552,#44553,#44554,#44555,#44556,#44557,#44558,#44559),
 .UNSPECIFIED.,.F.,.F.,(4,3,3,3,3,3,3,3,3,3,3,3,3,3,3,3,3,3,3,3,3,3,3,3,
3,3,3,3,3,3,3,3,3,3,3,3,3,3,3,3,3,3,3,3,3,3,3,3,3,4),(74.4816294174661,
74.5692291326888,74.6568738988186,74.7446611805597,74.8275176180992,74.9153515022495,
75.0030745344625,75.0907096966175,75.1816393588752,75.2691756140558,75.3566988094021,
75.4442295822475,75.5317885702762,75.6194441849438,75.7071571937103,75.7949954619019,
75.8181469946792,75.9059803529528,75.9937031226878,76.0813382823747,76.1722680434853,
76.2598049368958,76.3473290042904,76.4348608808726,76.5224212023653,76.6100784810607,
76.6977933481166,76.7856337425876,76.8087763712593,76.8964961427356,76.9841049002744,
77.0716257599405,77.1625982584278,77.2500208544713,77.3374308199701,77.4248489115836,
77.512295886818,77.5998410363746,77.6874443493797,77.7751748842725,77.7994057478393,
77.8864522154222,77.9733604160186,78.0601893663266,78.1469605854896,78.2336955406122,
78.3204377947017,78.4071831868706,78.4939872267225,78.5398163397448),
 .UNSPECIFIED.);
#2197=B_SPLINE_CURVE_WITH_KNOTS('',3,(#44565,#44566,#44567,#44568,#44569,
#44570,#44571,#44572,#44573,#44574,#44575,#44576,#44577,#44578,#44579,#44580,
#44581,#44582,#44583,#44584,#44585,#44586,#44587,#44588,#44589,#44590,#44591,
#44592,#44593,#44594,#44595,#44596,#44597,#44598,#44599,#44600,#44601,#44602,
#44603,#44604,#44605,#44606,#44607,#44608,#44609,#44610,#44611,#44612,#44613,
#44614,#44615,#44616,#44617,#44618,#44619,#44620,#44621,#44622,#44623,#44624,
#44625,#44626,#44627,#44628,#44629,#44630,#44631,#44632,#44633,#44634,#44635,
#44636,#44637,#44638,#44639,#44640,#44641,#44642,#44643,#44644,#44645,#44646,
#44647,#44648,#44649,#44650,#44651,#44652,#44653,#44654,#44655,#44656,#44657,
#44658,#44659,#44660,#44661,#44662,#44663,#44664,#44665,#44666,#44667,#44668,
#44669,#44670,#44671,#44672,#44673,#44674,#44675,#44676,#44677,#44678,#44679,
#44680,#44681,#44682,#44683,#44684,#44685,#44686,#44687,#44688,#44689,#44690,
#44691,#44692,#44693,#44694,#44695,#44696,#44697,#44698,#44699,#44700,#44701,
#44702,#44703,#44704,#44705,#44706,#44707,#44708,#44709,#44710,#44711,#44712),
 .UNSPECIFIED.,.F.,.F.,(4,3,3,3,3,3,3,3,3,3,3,3,3,3,3,3,3,3,3,3,3,3,3,3,
3,3,3,3,3,3,3,3,3,3,3,3,3,3,3,3,3,3,3,3,3,3,3,3,3,4),(68.1983678147316,
68.2861854710949,68.3234122878779,68.4112283810042,68.4989336774631,68.5865511791694,
68.6774874898305,68.7650063816156,68.8525123525859,68.9400260581836,69.0275681543285,
69.1152072202934,69.2029038608162,69.2907261485386,69.314041664458,69.4018609779144,
69.4895694873212,69.5771901909359,69.6681252971987,69.755647343511,69.8431564461835,
69.9306732573624,70.0182184296503,70.1058605129341,70.1935601400665,70.2813853468485,
70.304671041038,70.3924917596528,70.4802017089149,70.5678238849091,70.6587584514977,
70.7462820410624,70.8337927103019,70.9213111095382,71.0088578895641,71.09650160134,
71.1842028709319,71.2720297278734,71.295300417618,71.3826851317177,71.469959269805,
71.5571463325211,71.6445819200016,71.7316742053465,71.8187548325092,71.9058449008842,
71.9935414337543,72.0807584843929,72.1686947583788,72.2566310323648),
 .UNSPECIFIED.);
#2198=B_SPLINE_CURVE_WITH_KNOTS('',3,(#44713,#44714,#44715,#44716,#44717,
#44718,#44719,#44720,#44721,#44722,#44723,#44724,#44725,#44726,#44727,#44728,
#44729,#44730,#44731,#44732,#44733,#44734,#44735,#44736,#44737,#44738,#44739,
#44740,#44741,#44742,#44743,#44744,#44745,#44746,#44747,#44748,#44749,#44750,
#44751,#44752,#44753,#44754,#44755,#44756,#44757,#44758,#44759,#44760,#44761,
#44762,#44763,#44764,#44765,#44766,#44767,#44768,#44769,#44770,#44771,#44772,
#44773,#44774,#44775,#44776,#44777,#44778,#44779,#44780,#44781,#44782,#44783,
#44784,#44785,#44786,#44787,#44788,#44789,#44790,#44791,#44792,#44793,#44794,
#44795,#44796,#44797),.UNSPECIFIED.,.F.,.F.,(4,3,3,3,3,3,3,3,3,3,3,3,3,
3,3,3,3,3,3,3,3,3,3,3,3,3,3,3,4),(72.2566310325652,72.2859297941981,72.3737636821433,
72.4614867181185,72.5491218839988,72.6400515448462,72.7275878036391,72.8151110025499,
72.9026417789087,72.9902007703964,73.0778563884256,73.1655694005009,73.2534076718996,
73.2765591707781,73.3643925445142,73.4521153297987,73.5397505051032,73.6306802603851,
73.7182171694824,73.8057412525619,73.8932731448105,73.9808334819333,74.068490776127,
74.1562056586224,74.2440460683294,74.2671885473581,74.3549161093617,74.4425200092409,
74.4826134639429),.UNSPECIFIED.);
#2199=B_SPLINE_CURVE_WITH_KNOTS('',3,(#44799,#44800,#44801,#44802,#44803,
#44804,#44805,#44806,#44807,#44808,#44809,#44810,#44811,#44812,#44813,#44814,
#44815,#44816,#44817,#44818,#44819,#44820,#44821,#44822,#44823,#44824,#44825,
#44826,#44827,#44828,#44829,#44830,#44831,#44832,#44833,#44834,#44835,#44836,
#44837,#44838,#44839,#44840,#44841,#44842,#44843,#44844,#44845,#44846,#44847,
#44848,#44849,#44850,#44851,#44852,#44853,#44854,#44855,#44856,#44857,#44858,
#44859,#44860,#44861,#44862,#44863,#44864,#44865,#44866,#44867,#44868,#44869,
#44870,#44871,#44872,#44873,#44874,#44875,#44876,#44877,#44878,#44879,#44880),
 .UNSPECIFIED.,.F.,.F.,(4,3,3,3,3,3,3,3,3,3,3,3,3,3,3,3,3,3,3,3,3,3,3,3,
3,3,3,4),(72.2566310325652,72.3454121678946,72.4342210203789,72.5230760362226,
72.6120571070531,72.7011068517644,72.7903135273602,72.8462588649391,72.934079580666,
73.0217895270243,73.1094117001026,73.2003462677797,73.2878698544167,73.3753805207293,
73.4628989170425,73.5504456941521,73.638089403037,73.7257906697492,73.8136175238493,
73.8368882415192,73.924677994041,74.0123639854369,74.0999670580816,74.1875079866763,
74.2750138504675,74.3624996138977,74.4500027036407,74.4816294174661),
 .UNSPECIFIED.);
#2200=B_SPLINE_CURVE_WITH_KNOTS('',3,(#44881,#44882,#44883,#44884,#44885,
#44886,#44887,#44888,#44889,#44890,#44891,#44892,#44893,#44894,#44895,#44896,
#44897,#44898,#44899,#44900,#44901,#44902,#44903,#44904,#44905,#44906,#44907,
#44908,#44909,#44910,#44911,#44912,#44913,#44914,#44915,#44916,#44917,#44918,
#44919,#44920,#44921,#44922,#44923,#44924,#44925,#44926,#44927,#44928,#44929,
#44930,#44931,#44932,#44933,#44934,#44935,#44936,#44937,#44938,#44939,#44940,
#44941,#44942,#44943,#44944,#44945,#44946,#44947,#44948,#44949,#44950,#44951,
#44952,#44953,#44954,#44955,#44956,#44957,#44958,#44959,#44960,#44961,#44962,
#44963,#44964,#44965,#44966,#44967,#44968,#44969,#44970,#44971,#44972,#44973,
#44974,#44975,#44976,#44977,#44978,#44979,#44980,#44981,#44982,#44983,#44984,
#44985,#44986,#44987,#44988,#44989,#44990,#44991,#44992,#44993,#44994,#44995,
#44996,#44997,#44998,#44999,#45000,#45001,#45002,#45003,#45004,#45005,#45006,
#45007,#45008,#45009,#45010,#45011,#45012,#45013,#45014,#45015,#45016,#45017,
#45018,#45019,#45020,#45021,#45022,#45023,#45024,#45025,#45026,#45027,#45028),
 .UNSPECIFIED.,.F.,.F.,(4,3,3,3,3,3,3,3,3,3,3,3,3,3,3,3,3,3,3,3,3,3,3,3,
3,3,3,3,3,3,3,3,3,3,3,3,3,3,3,3,3,3,3,3,3,3,3,3,3,4),(68.1993438798599,
68.2868799916938,68.3743918833257,68.4619002146255,68.5494256379166,68.637042488327,
68.7247067515849,68.8125099054391,68.883741358619,68.971559219945,69.0592662848475,
69.1468855531686,69.2378212009224,69.3253418436864,69.4128495568768,69.500364994083,
69.5879088093621,69.6755495674304,69.7632478863016,69.8510718195009,69.8743707351991,
69.9621889551786,70.0498963831715,70.137516018533,70.2284515301888,70.3159725474149,
70.4034806371411,70.4909964525364,70.5785406472388,70.6661817846189,70.7538804831779,
70.8417047937,70.8650001117791,70.9528162060867,71.0405215037276,71.1281390066153,
71.2190753168333,71.3065942097912,71.394100181929,71.4816138886882,71.5691559859863,
71.6567950530876,71.7444916947385,71.8323139835676,71.8556294883591,71.9558798743625,
72.0526994126788,72.1492492883176,72.2454013625398,72.2566310323726),
 .UNSPECIFIED.);
#2201=B_SPLINE_CURVE_WITH_KNOTS('',3,(#45034,#45035,#45036,#45037,#45038,
#45039,#45040,#45041,#45042,#45043,#45044,#45045,#45046,#45047,#45048,#45049,
#45050,#45051,#45052,#45053,#45054,#45055,#45056,#45057,#45058,#45059,#45060,
#45061,#45062,#45063,#45064,#45065,#45066,#45067,#45068,#45069,#45070,#45071,
#45072,#45073,#45074,#45075,#45076,#45077,#45078,#45079,#45080,#45081,#45082,
#45083,#45084,#45085,#45086,#45087,#45088,#45089,#45090,#45091,#45092,#45093,
#45094,#45095,#45096,#45097,#45098,#45099,#45100,#45101,#45102,#45103,#45104,
#45105,#45106,#45107,#45108,#45109,#45110,#45111,#45112,#45113,#45114,#45115,
#45116,#45117,#45118,#45119,#45120,#45121,#45122,#45123,#45124,#45125,#45126,
#45127,#45128,#45129,#45130,#45131,#45132,#45133,#45134,#45135,#45136,#45137,
#45138,#45139,#45140,#45141,#45142,#45143,#45144,#45145,#45146,#45147,#45148,
#45149,#45150,#45151,#45152,#45153,#45154,#45155,#45156,#45157,#45158,#45159,
#45160,#45161,#45162,#45163,#45164,#45165,#45166,#45167,#45168,#45169,#45170,
#45171,#45172,#45173,#45174,#45175,#45176,#45177,#45178,#45179,#45180,#45181),
 .UNSPECIFIED.,.F.,.F.,(4,3,3,3,3,3,3,3,3,3,3,3,3,3,3,3,3,3,3,3,3,3,3,3,
3,3,3,3,3,3,3,3,3,3,3,3,3,3,3,3,3,3,3,3,3,3,3,3,3,4),(61.9155795994057,
62.0030944068429,62.0906369960354,62.1782762547704,62.2659725380791,62.3537951104487,
62.3796360283978,62.4674537279978,62.5551606325058,62.6427797419325,62.7337154498132,
62.8212359383819,62.9087434993666,62.9962587865121,63.0838024540337,63.1714430684749,
63.2591412459543,63.3469650420966,63.3702654049778,63.4580831375175,63.545790074768,
63.633409216705,63.7243449123116,63.8118654326121,63.8993730249881,63.9868883431528,
64.0744320412883,64.1620726855925,64.2497708925329,64.3375947173261,64.3608947815578,
64.4487125812256,64.5364195861566,64.6240387962398,64.7149744664771,64.8024950556412,
64.8900027170247,64.977518104265,65.0650618714678,65.1527025844783,65.240400859995,
65.3282247526493,65.3515241581379,65.4399937117072,65.5283487386399,65.6166091627478,
65.7058183034073,65.7939457801226,65.8836957527541,65.9734457253856),
 .UNSPECIFIED.);
#2202=B_SPLINE_CURVE_WITH_KNOTS('',3,(#45182,#45183,#45184,#45185,#45186,
#45187,#45188,#45189,#45190,#45191,#45192,#45193,#45194,#45195,#45196,#45197,
#45198,#45199,#45200,#45201,#45202,#45203,#45204,#45205,#45206,#45207,#45208,
#45209,#45210,#45211,#45212,#45213,#45214,#45215,#45216,#45217,#45218,#45219,
#45220,#45221,#45222,#45223,#45224,#45225,#45226,#45227,#45228,#45229,#45230,
#45231,#45232,#45233,#45234,#45235,#45236,#45237,#45238,#45239,#45240,#45241,
#45242,#45243,#45244,#45245,#45246,#45247,#45248,#45249,#45250,#45251,#45252,
#45253,#45254,#45255,#45256,#45257,#45258,#45259,#45260),.UNSPECIFIED.,
 .F.,.F.,(4,3,3,3,3,3,3,3,3,3,3,3,3,3,3,3,3,3,3,3,3,3,3,3,3,3,4),(65.9734457256019,
66.0719665867376,66.1708765057206,66.2703101688383,66.3421535347179,66.4299713960909,
66.5176784610392,66.6052977294049,66.6962333771415,66.7837540199466,66.8712617331766,
66.958777170421,67.0463209857378,67.133961743841,67.2216600627455,67.3094839959762,
67.3327829112979,67.4206086977955,67.5083218961891,67.5959325406812,67.6834855476166,
67.7710016175743,67.8585014192332,67.9460421456659,68.0336015824382,68.1212568561678,
68.1983678147316),.UNSPECIFIED.);
#2203=B_SPLINE_CURVE_WITH_KNOTS('',3,(#45262,#45263,#45264,#45265,#45266,
#45267,#45268,#45269,#45270,#45271,#45272,#45273,#45274,#45275,#45276,#45277,
#45278,#45279,#45280,#45281,#45282,#45283,#45284,#45285,#45286,#45287,#45288,
#45289,#45290,#45291,#45292,#45293,#45294,#45295,#45296,#45297,#45298,#45299,
#45300,#45301,#45302,#45303,#45304,#45305,#45306,#45307,#45308,#45309,#45310,
#45311,#45312,#45313,#45314,#45315,#45316,#45317,#45318,#45319,#45320,#45321,
#45322,#45323,#45324,#45325,#45326,#45327,#45328,#45329,#45330,#45331,#45332,
#45333,#45334,#45335,#45336,#45337,#45338,#45339,#45340,#45341,#45342,#45343),
 .UNSPECIFIED.,.F.,.F.,(4,3,3,3,3,3,3,3,3,3,3,3,3,3,3,3,3,3,3,3,3,3,3,3,
3,3,3,4),(65.9734457255633,66.0604573157294,66.14736302234,66.2341866831258,
66.3209558418872,66.4076973438865,66.4944326106493,66.5811830545443,66.6680217581067,
66.7549075928963,66.8419276082886,66.902482605459,66.990300405037,67.0780074098778,
67.16562661987,67.2565622901411,67.3440828792145,67.4315905405076,67.5191059276573,
67.6066496947706,67.6942904076922,67.7819886831202,67.869812575687,67.893111982039,
67.9809172824462,68.0686253046379,68.1562387872474,68.1993438798599),
 .UNSPECIFIED.);
#2204=B_SPLINE_CURVE_WITH_KNOTS('',3,(#45344,#45345,#45346,#45347,#45348,
#45349,#45350,#45351,#45352,#45353,#45354,#45355,#45356,#45357,#45358,#45359,
#45360,#45361,#45362,#45363,#45364,#45365,#45366,#45367,#45368,#45369,#45370,
#45371,#45372,#45373,#45374,#45375,#45376,#45377,#45378,#45379,#45380,#45381,
#45382,#45383,#45384,#45385,#45386,#45387,#45388,#45389,#45390,#45391,#45392,
#45393,#45394,#45395,#45396,#45397,#45398,#45399,#45400,#45401,#45402,#45403,
#45404,#45405,#45406,#45407,#45408,#45409,#45410,#45411,#45412,#45413,#45414,
#45415,#45416,#45417,#45418,#45419,#45420,#45421,#45422,#45423,#45424,#45425,
#45426,#45427,#45428,#45429,#45430,#45431,#45432,#45433,#45434,#45435,#45436,
#45437,#45438,#45439,#45440,#45441,#45442,#45443,#45444,#45445,#45446,#45447,
#45448,#45449,#45450,#45451,#45452,#45453,#45454,#45455,#45456,#45457,#45458,
#45459,#45460,#45461,#45462,#45463,#45464,#45465,#45466,#45467,#45468,#45469,
#45470,#45471,#45472,#45473,#45474,#45475,#45476,#45477,#45478,#45479,#45480,
#45481,#45482,#45483,#45484,#45485,#45486,#45487,#45488,#45489,#45490,#45491,
#45492,#45493,#45494),.UNSPECIFIED.,.F.,.F.,(4,3,3,3,3,3,3,3,3,3,3,3,3,
3,3,3,3,3,3,3,3,3,3,3,3,3,3,3,3,3,3,3,3,3,3,3,3,3,3,3,3,3,3,3,3,3,3,3,3,
3,4),(61.9154901076124,61.9493357225588,62.0371534434414,62.124860369225,
62.2124794998959,62.3034151998013,62.3909357094019,62.4784432913042,62.5659585992311,
62.6535022873757,62.7411429221022,62.8288411196942,62.9166649355437,62.9399650991389,
63.0277828228076,63.1154897513483,63.2031088847447,63.2940445836165,63.3815650958472,
63.4690726803401,63.5565879908155,63.6441316814639,63.7317723186155,63.8194705185899,
63.9072943367414,63.9305944757189,64.0184122103713,64.1061191499622,64.1937382944615,
64.2846739891911,64.3721945125848,64.4597021082432,64.5472174298747,64.6347611316574,
64.7224017798552,64.8100999908372,64.8979238198559,64.9212238522989,65.0090415519244,
65.0967484564579,65.1843675659104,65.2753032737815,65.3628237623755,65.4503313233851,
65.5378466105556,65.6253902781022,65.7130308925677,65.8007290700712,65.8885528662372,
65.911853228879,65.9734457253856),.UNSPECIFIED.);
#2205=B_SPLINE_CURVE_WITH_KNOTS('',3,(#45500,#45501,#45502,#45503,#45504,
#45505,#45506,#45507,#45508,#45509,#45510,#45511,#45512,#45513,#45514,#45515,
#45516,#45517,#45518,#45519,#45520,#45521,#45522,#45523,#45524,#45525,#45526,
#45527,#45528,#45529,#45530,#45531,#45532,#45533,#45534,#45535,#45536,#45537,
#45538,#45539,#45540,#45541,#45542,#45543,#45544,#45545,#45546,#45547,#45548,
#45549,#45550,#45551,#45552,#45553,#45554,#45555,#45556,#45557,#45558,#45559,
#45560,#45561,#45562,#45563,#45564,#45565,#45566,#45567,#45568,#45569,#45570,
#45571,#45572,#45573,#45574,#45575,#45576,#45577,#45578,#45579,#45580,#45581,
#45582,#45583,#45584,#45585,#45586,#45587,#45588,#45589,#45590,#45591,#45592,
#45593,#45594,#45595,#45596,#45597,#45598,#45599,#45600,#45601,#45602,#45603,
#45604,#45605,#45606,#45607,#45608,#45609,#45610,#45611,#45612,#45613,#45614,
#45615,#45616,#45617,#45618,#45619,#45620,#45621,#45622,#45623,#45624,#45625,
#45626,#45627,#45628,#45629,#45630,#45631,#45632,#45633,#45634,#45635,#45636,
#45637,#45638,#45639,#45640,#45641,#45642,#45643,#45644,#45645,#45646,#45647),
 .UNSPECIFIED.,.F.,.F.,(4,3,3,3,3,3,3,3,3,3,3,3,3,3,3,3,3,3,3,3,3,3,3,3,
3,3,3,3,3,3,3,3,3,3,3,3,3,3,3,3,3,3,3,3,3,3,3,3,3,4),(55.633055807239,55.7206644555141,
55.8100638696896,55.897581680751,55.9850891020412,56.0726067865466,56.1634200321393,
56.2510686326646,56.3387777720785,56.4266088847394,56.4358597689176,56.5236774922691,
56.6113844205186,56.6990035536499,56.7899392526309,56.8774597646623,56.9649673489804,
57.0524826593056,57.1400263498282,57.2276669868911,57.3153651867981,57.4031890049135,
57.4264891454977,57.5143068690169,57.6020137974301,57.6896329307208,57.7805686296404,
57.86808914182,57.9555967262817,58.043112036746,58.1306557274031,58.2182963645929,
58.3059945646225,58.3938183828535,58.4171185220777,58.5049362472664,58.5926431773569,
58.6802623123306,58.7711980106215,58.8587185244875,58.9462261106341,59.0337414227797,
59.1212851151128,59.2089257539622,59.296623955644,59.3844477755035,59.4077478986577,
59.5162980885706,59.6233575347649,59.6902604180773),.UNSPECIFIED.);
#2206=B_SPLINE_CURVE_WITH_KNOTS('',3,(#45648,#45649,#45650,#45651,#45652,
#45653,#45654,#45655,#45656,#45657,#45658,#45659,#45660,#45661,#45662,#45663,
#45664,#45665,#45666,#45667,#45668,#45669,#45670,#45671,#45672,#45673,#45674,
#45675,#45676,#45677,#45678,#45679,#45680,#45681,#45682,#45683,#45684,#45685,
#45686,#45687,#45688,#45689,#45690,#45691,#45692,#45693,#45694,#45695,#45696,
#45697,#45698,#45699,#45700,#45701,#45702,#45703,#45704,#45705,#45706,#45707,
#45708,#45709,#45710,#45711,#45712,#45713,#45714,#45715,#45716,#45717,#45718,
#45719,#45720,#45721,#45722,#45723,#45724,#45725,#45726),.UNSPECIFIED.,
 .F.,.F.,(4,3,3,3,3,3,3,3,3,3,3,3,3,3,3,3,3,3,3,3,3,3,3,3,3,3,4),(59.690260418206,
59.778775025335,59.8656202866756,59.9524524287065,60.0392927592542,60.1290638882501,
60.2160327259131,60.3072050005754,60.3983772752377,60.4861949989052,60.5739019274446,
60.6615210608397,60.7524567597119,60.8399772719413,60.9274848564327,61.0150001669067,
61.1025438575537,61.1901844947038,61.2778826946767,61.3657065128266,61.3890066518178,
61.4768208758908,61.5645289299805,61.6522915973368,61.7398434419403,61.827711520673,
61.9155795994057),.UNSPECIFIED.);
#2207=B_SPLINE_CURVE_WITH_KNOTS('',3,(#45728,#45729,#45730,#45731,#45732,
#45733,#45734,#45735,#45736,#45737,#45738,#45739,#45740,#45741,#45742,#45743,
#45744,#45745,#45746,#45747,#45748,#45749,#45750,#45751,#45752,#45753,#45754,
#45755,#45756,#45757,#45758,#45759,#45760,#45761,#45762,#45763,#45764,#45765,
#45766,#45767,#45768,#45769,#45770,#45771,#45772,#45773,#45774,#45775,#45776,
#45777,#45778,#45779,#45780,#45781,#45782,#45783,#45784,#45785,#45786,#45787,
#45788,#45789,#45790,#45791,#45792,#45793,#45794,#45795,#45796,#45797,#45798,
#45799,#45800,#45801,#45802,#45803,#45804,#45805,#45806),.UNSPECIFIED.,
 .F.,.F.,(4,3,3,3,3,3,3,3,3,3,3,3,3,3,3,3,3,3,3,3,3,3,3,3,3,3,4),(59.6902604184428,
59.7976956859163,59.9067549038113,59.9680769693988,60.0558946929184,60.1436016213319,
60.231220754623,60.3221564535424,60.4096769657224,60.4971845501845,60.5846998606492,
60.6722435513067,60.7598841884968,60.8475823885268,60.9354062067581,60.9587063459788,
61.0465260474693,61.1342344677582,61.2218546088897,61.3094092434533,61.3969287962482,
61.4844339360247,61.5719453161366,61.6595334476544,61.7471595779332,61.8349151107887,
61.9154901076124),.UNSPECIFIED.);
#2208=B_SPLINE_CURVE_WITH_KNOTS('',3,(#45807,#45808,#45809,#45810,#45811,
#45812,#45813,#45814,#45815,#45816,#45817,#45818,#45819,#45820,#45821,#45822,
#45823,#45824,#45825,#45826,#45827,#45828,#45829,#45830,#45831,#45832,#45833,
#45834,#45835,#45836,#45837,#45838,#45839,#45840,#45841,#45842,#45843,#45844,
#45845,#45846,#45847,#45848,#45849,#45850,#45851,#45852,#45853,#45854,#45855,
#45856,#45857,#45858,#45859,#45860,#45861,#45862,#45863,#45864,#45865,#45866,
#45867,#45868,#45869,#45870,#45871,#45872,#45873,#45874,#45875,#45876,#45877,
#45878,#45879,#45880,#45881,#45882,#45883,#45884,#45885,#45886,#45887,#45888,
#45889,#45890,#45891,#45892,#45893,#45894,#45895,#45896,#45897,#45898,#45899,
#45900,#45901,#45902,#45903,#45904,#45905,#45906,#45907,#45908,#45909,#45910,
#45911,#45912,#45913,#45914,#45915,#45916,#45917,#45918,#45919,#45920,#45921,
#45922,#45923,#45924,#45925,#45926,#45927,#45928,#45929,#45930,#45931,#45932,
#45933,#45934,#45935,#45936,#45937,#45938,#45939,#45940,#45941,#45942,#45943,
#45944,#45945,#45946,#45947,#45948,#45949,#45950,#45951,#45952,#45953,#45954,
#45955,#45956,#45957),.UNSPECIFIED.,.F.,.F.,(4,3,3,3,3,3,3,3,3,3,3,3,3,
3,3,3,3,3,3,3,3,3,3,3,3,3,3,3,3,3,3,3,3,3,3,3,3,3,3,3,3,3,3,3,3,3,3,3,3,
3,4),(55.6321437035808,55.719687656161,55.807328619535,55.8950272711616,
55.9828513851517,56.0055594630787,56.0933771867062,56.181084115231,56.2687032486367,
56.3596389475144,56.4471594598163,56.5346670444028,56.6221823549943,56.7097260457809,
56.7973666831025,56.8850648832657,56.9728887016316,56.9961888396587,57.0840065632834,
57.1717134918049,57.2593326252068,57.3502683240858,57.4377888363825,57.5252964209634,
57.6128117315488,57.7003554223288,57.7879960596434,57.875694259799,57.9635180781567,
57.9868182162387,58.0746359401032,58.1623428688656,58.2499620025095,58.3408977012982,
58.4284182138362,58.5159257986579,58.6034411094834,58.6909848005021,58.778625438053,
58.8663236384434,58.954147457033,58.9774475928188,59.0665491959922,59.153511270838,
59.2403929917755,59.3272158146748,59.4179769655576,59.5047630074242,59.5915521894301,
59.6783867677546,59.690260418206),.UNSPECIFIED.);
#2209=B_SPLINE_CURVE_WITH_KNOTS('',3,(#45963,#45964,#45965,#45966,#45967,
#45968,#45969,#45970,#45971,#45972,#45973,#45974,#45975,#45976,#45977,#45978,
#45979,#45980,#45981,#45982,#45983,#45984,#45985,#45986,#45987,#45988,#45989,
#45990,#45991,#45992,#45993,#45994,#45995,#45996,#45997,#45998,#45999,#46000,
#46001,#46002,#46003,#46004,#46005,#46006,#46007,#46008,#46009,#46010,#46011,
#46012,#46013,#46014,#46015,#46016,#46017,#46018,#46019,#46020,#46021,#46022,
#46023,#46024,#46025,#46026,#46027,#46028,#46029,#46030,#46031,#46032,#46033,
#46034,#46035,#46036,#46037,#46038,#46039,#46040,#46041,#46042,#46043,#46044,
#46045,#46046,#46047,#46048,#46049,#46050,#46051,#46052,#46053,#46054,#46055,
#46056,#46057,#46058,#46059,#46060,#46061,#46062,#46063,#46064,#46065,#46066,
#46067,#46068,#46069,#46070,#46071,#46072,#46073,#46074,#46075,#46076,#46077,
#46078,#46079,#46080,#46081,#46082,#46083,#46084,#46085,#46086,#46087,#46088,
#46089,#46090,#46091,#46092,#46093,#46094,#46095,#46096,#46097,#46098,#46099,
#46100,#46101,#46102,#46103,#46104,#46105,#46106,#46107,#46108,#46109,#46110),
 .UNSPECIFIED.,.F.,.F.,(4,3,3,3,3,3,3,3,3,3,3,3,3,3,3,3,3,3,3,3,3,3,3,3,
3,3,3,3,3,3,3,3,3,3,3,3,3,3,3,3,3,3,3,3,3,3,3,3,3,4),(49.3487655641429,
49.4365712254866,49.5014541328574,49.5892718565205,49.676978785081,49.764597918522,
49.8555336173865,49.9430541297232,50.0305617143443,50.11807702497,50.2056207157904,
50.2932613531452,50.3809595533411,50.468783371739,50.4920835094375,50.5799012330941,
50.6676081616481,50.7552272950827,50.8461629939495,50.9336835062799,51.0211910908947,
51.1087064015141,51.1962500923283,51.2838907296771,51.371588929867,51.4594127482591,
51.4827128860175,51.5705306096707,51.6582375382212,51.7458566716522,51.8367923705204,
51.9243128828471,52.0118204674581,52.0993357780737,52.186879468884,52.2745201062289,
52.3622183064147,52.4500421248028,52.4733422625975,52.5604221705999,52.6473917779252,
52.7342748966389,52.8210968702449,52.9078870051233,52.9946666871673,53.0814572897356,
53.1683305097573,53.2552470966057,53.3422944293372,53.4070751108575),
 .UNSPECIFIED.);
#2210=B_SPLINE_CURVE_WITH_KNOTS('',3,(#46111,#46112,#46113,#46114,#46115,
#46116,#46117,#46118,#46119,#46120,#46121,#46122,#46123,#46124,#46125,#46126,
#46127,#46128,#46129,#46130,#46131,#46132,#46133,#46134,#46135,#46136,#46137,
#46138,#46139,#46140,#46141,#46142,#46143,#46144,#46145,#46146,#46147,#46148,
#46149,#46150,#46151,#46152,#46153,#46154,#46155,#46156,#46157,#46158,#46159,
#46160,#46161,#46162,#46163,#46164,#46165,#46166,#46167,#46168,#46169,#46170,
#46171,#46172,#46173,#46174,#46175,#46176,#46177,#46178,#46179,#46180,#46181,
#46182,#46183,#46184,#46185,#46186,#46187,#46188,#46189,#46190,#46191,#46192,
#46193,#46194,#46195),.UNSPECIFIED.,.F.,.F.,(4,3,3,3,3,3,3,3,3,3,3,3,3,
3,3,3,3,3,3,3,3,3,3,3,3,3,3,3,4),(53.4070751110265,53.4639716391775,53.5517893628049,
53.6394962913298,53.7271154247354,53.8180511236132,53.9055716359151,53.9930792205016,
54.080594531093,54.1681382218795,54.2557788592012,54.3434770593642,54.43130087773,
54.4546010157576,54.5424187393821,54.6301256679035,54.7177448013052,54.8086805001843,
54.8962010124809,54.9837085970618,55.0712239076471,55.158767598427,55.2464082357414,
55.3341064358969,55.4219302542547,55.4452303923376,55.533063232291,55.6207748440684,
55.633055807239),.UNSPECIFIED.);
#2211=B_SPLINE_CURVE_WITH_KNOTS('',3,(#46197,#46198,#46199,#46200,#46201,
#46202,#46203,#46204,#46205,#46206,#46207,#46208,#46209,#46210,#46211,#46212,
#46213,#46214,#46215,#46216,#46217,#46218,#46219,#46220,#46221,#46222,#46223,
#46224,#46225,#46226,#46227,#46228,#46229,#46230,#46231,#46232,#46233,#46234,
#46235,#46236,#46237,#46238,#46239,#46240,#46241,#46242,#46243,#46244,#46245,
#46246,#46247,#46248,#46249,#46250,#46251,#46252,#46253,#46254,#46255,#46256,
#46257,#46258,#46259,#46260,#46261,#46262,#46263,#46264,#46265,#46266,#46267,
#46268,#46269,#46270,#46271,#46272,#46273,#46274,#46275),.UNSPECIFIED.,
 .F.,.F.,(4,3,3,3,3,3,3,3,3,3,3,3,3,3,3,3,3,3,3,3,3,3,3,3,3,3,4),(53.4070751110265,
53.4952697145479,53.5834738757,53.6717071431077,53.760051289663,53.8484511190502,
53.937010413905,54.0243007099186,54.1121184335718,54.1998253621224,54.2874444955536,
54.3783801944217,54.4659007067484,54.5534082913595,54.6409236019751,54.7284672927852,
54.8161079301302,54.9038061303163,54.9916299487045,55.0149300864986,55.1027351460802,
55.1904358979913,55.2780531734419,55.3665758059767,55.4540917217808,55.5431177126808,
55.6321437035808),.UNSPECIFIED.);
#2212=B_SPLINE_CURVE_WITH_KNOTS('',3,(#46276,#46277,#46278,#46279,#46280,
#46281,#46282,#46283,#46284,#46285,#46286,#46287,#46288,#46289,#46290,#46291,
#46292,#46293,#46294,#46295,#46296,#46297,#46298,#46299,#46300,#46301,#46302,
#46303,#46304,#46305,#46306,#46307,#46308,#46309,#46310,#46311,#46312,#46313,
#46314,#46315,#46316,#46317,#46318,#46319,#46320,#46321,#46322,#46323,#46324,
#46325,#46326,#46327,#46328,#46329,#46330,#46331,#46332,#46333,#46334,#46335,
#46336,#46337,#46338,#46339,#46340,#46341,#46342,#46343,#46344,#46345,#46346,
#46347,#46348,#46349,#46350,#46351,#46352,#46353,#46354,#46355,#46356,#46357,
#46358,#46359,#46360,#46361,#46362,#46363,#46364,#46365,#46366,#46367,#46368,
#46369,#46370,#46371,#46372,#46373,#46374,#46375,#46376,#46377,#46378,#46379,
#46380,#46381,#46382,#46383,#46384,#46385,#46386,#46387,#46388,#46389,#46390,
#46391,#46392,#46393,#46394,#46395,#46396,#46397,#46398,#46399,#46400,#46401,
#46402,#46403,#46404,#46405,#46406,#46407,#46408,#46409,#46410,#46411,#46412,
#46413,#46414,#46415,#46416,#46417,#46418,#46419,#46420),.UNSPECIFIED.,
 .F.,.F.,(4,3,3,3,3,3,3,3,3,3,3,3,3,3,3,3,3,3,3,3,3,3,3,3,3,3,3,3,3,3,3,
3,3,3,3,3,3,3,3,3,3,3,3,3,3,3,3,3,4),(49.3498290568562,49.4388233251989,
49.5263404755851,49.6138479054887,49.7013662677403,49.7914705017049,49.8791203513828,
49.9704517774906,50.0617832035985,50.149600927258,50.2373078558148,50.324926989252,
50.4158626881178,50.5033832004509,50.5908907850683,50.6784060956903,50.7659497865072,
50.8535904238585,50.9412886240507,51.0291124424452,51.0524125801785,51.1402303038371,
51.227937232393,51.3155563658297,51.4064920646958,51.4940125770281,51.5815201616448,
51.6690354722663,51.7565791630822,51.8442198004329,51.9319180006247,52.0197418190183,
52.0430419567586,52.1308596804217,52.2185666089819,52.3061857424226,52.3971214412871,
52.4846419536239,52.5721495382451,52.6596648488706,52.7472085396905,52.8348491770453,
52.9225473772411,53.0103711956392,53.0336713333386,53.1327118219515,53.2314411213958,
53.3295918554781,53.4070751108119),.UNSPECIFIED.);
#2213=B_SPLINE_CURVE_WITH_KNOTS('',3,(#46426,#46427,#46428,#46429,#46430,
#46431,#46432,#46433,#46434,#46435,#46436,#46437,#46438,#46439,#46440,#46441,
#46442,#46443,#46444,#46445,#46446,#46447,#46448,#46449,#46450,#46451,#46452,
#46453,#46454,#46455,#46456,#46457,#46458,#46459,#46460,#46461,#46462,#46463,
#46464,#46465,#46466,#46467,#46468,#46469,#46470,#46471,#46472,#46473,#46474,
#46475,#46476,#46477,#46478,#46479,#46480,#46481,#46482,#46483,#46484,#46485,
#46486,#46487,#46488,#46489,#46490,#46491,#46492,#46493,#46494,#46495,#46496,
#46497,#46498,#46499,#46500,#46501,#46502,#46503,#46504,#46505,#46506,#46507,
#46508,#46509,#46510,#46511,#46512,#46513,#46514,#46515,#46516,#46517,#46518,
#46519,#46520,#46521,#46522,#46523,#46524,#46525,#46526,#46527,#46528,#46529,
#46530,#46531,#46532,#46533,#46534,#46535,#46536,#46537,#46538,#46539,#46540,
#46541,#46542,#46543,#46544,#46545,#46546,#46547,#46548,#46549,#46550,#46551,
#46552,#46553,#46554,#46555,#46556,#46557,#46558,#46559,#46560,#46561,#46562,
#46563,#46564,#46565,#46566,#46567,#46568,#46569,#46570,#46571,#46572,#46573),
 .UNSPECIFIED.,.F.,.F.,(4,3,3,3,3,3,3,3,3,3,3,3,3,3,3,3,3,3,3,3,3,3,3,3,
3,3,3,3,3,3,3,3,3,3,3,3,3,3,3,3,3,3,3,3,3,3,3,3,3,4),(43.0661059914245,
43.1536163207319,43.2411479365787,43.3287731026926,43.4164494524346,43.5042596073108,
43.5576778733773,43.6454955970374,43.7332025255949,43.8208216590328,43.9117573578984,
43.9992778702322,44.0867854548504,44.1743007654729,44.2618444562906,44.3494850936427,
44.4371832938357,44.5250071122309,44.5483072499573,44.6361249736169,44.7238319021739,
44.8114510356115,44.9023867344772,44.9899072468104,45.077414831428,45.1649301420504,
45.2524738328672,45.3401144702188,45.4278126704114,45.5156364888059,45.5389366265373,
45.6267543501969,45.7144612787539,45.8020804121914,45.8930161110571,45.9805366233903,
46.0680442080077,46.1555595186297,46.2431032094465,46.3307438467979,46.4184420469911,
46.5062658653855,46.5295660031174,46.6186563250424,46.7076259258596,46.7964937259149,
46.8852637004643,46.9739759768119,47.0626512944818,47.1238898038469),
 .UNSPECIFIED.);
#2214=B_SPLINE_CURVE_WITH_KNOTS('',3,(#46574,#46575,#46576,#46577,#46578,
#46579,#46580,#46581,#46582,#46583,#46584,#46585,#46586,#46587,#46588,#46589,
#46590,#46591,#46592,#46593,#46594,#46595,#46596,#46597,#46598,#46599,#46600,
#46601,#46602,#46603,#46604,#46605,#46606,#46607,#46608,#46609,#46610,#46611,
#46612,#46613,#46614,#46615,#46616,#46617,#46618,#46619,#46620,#46621,#46622,
#46623,#46624,#46625,#46626,#46627,#46628,#46629,#46630,#46631,#46632,#46633,
#46634,#46635,#46636,#46637,#46638,#46639,#46640,#46641,#46642,#46643,#46644,
#46645,#46646,#46647,#46648,#46649,#46650,#46651,#46652),.UNSPECIFIED.,
 .F.,.F.,(4,3,3,3,3,3,3,3,3,3,3,3,3,3,3,3,3,3,3,3,3,3,3,3,3,3,4),(47.1238898040446,
47.2229661979578,47.3199017158545,47.420048547776,47.5201953796974,47.6080131033568,
47.6957200319137,47.7833391653511,47.8742748642169,47.96179537655,48.0493029611674,
48.1368182717896,48.2243619626063,48.3120025999576,48.39970080015,48.4875246185445,
48.5108247562774,48.5986518168583,48.6863658889724,48.7739762516002,48.8615284122406,
48.9490430728474,49.0365409029296,49.1240737177127,49.2116250178518,49.2992578827919,
49.3487655641429),.UNSPECIFIED.);
#2215=B_SPLINE_CURVE_WITH_KNOTS('',3,(#46654,#46655,#46656,#46657,#46658,
#46659,#46660,#46661,#46662,#46663,#46664,#46665,#46666,#46667,#46668,#46669,
#46670,#46671,#46672,#46673,#46674,#46675,#46676,#46677,#46678,#46679,#46680,
#46681,#46682,#46683,#46684,#46685,#46686,#46687,#46688,#46689,#46690,#46691,
#46692,#46693,#46694,#46695,#46696,#46697,#46698,#46699,#46700,#46701,#46702,
#46703,#46704,#46705,#46706,#46707,#46708,#46709,#46710,#46711,#46712,#46713,
#46714,#46715,#46716,#46717,#46718,#46719,#46720,#46721,#46722,#46723,#46724,
#46725,#46726,#46727,#46728,#46729,#46730,#46731,#46732,#46733,#46734,#46735),
 .UNSPECIFIED.,.F.,.F.,(4,3,3,3,3,3,3,3,3,3,3,3,3,3,3,3,3,3,3,3,3,3,3,3,
3,3,3,4),(47.1238898040744,47.2112205230592,47.2984421477866,47.3855782233556,
47.4726547355818,47.5596998923596,47.6467348498393,47.7337807519279,47.8209134726714,
47.9080890145168,47.9954065966277,48.0805244504385,48.1683421740981,48.256049102655,
48.3436682360926,48.4346039349583,48.5221244472915,48.6096320319092,48.6971473425314,
48.7846910333482,48.8723316706997,48.9600298708923,49.047853689287,49.0711538270185,
49.1589647608053,49.2466781839562,49.3342970267507,49.3498290568562),
 .UNSPECIFIED.);
#2216=B_SPLINE_CURVE_WITH_KNOTS('',3,(#46736,#46737,#46738,#46739,#46740,
#46741,#46742,#46743,#46744,#46745,#46746,#46747,#46748,#46749,#46750,#46751,
#46752,#46753,#46754,#46755,#46756,#46757,#46758,#46759,#46760,#46761,#46762,
#46763,#46764,#46765,#46766,#46767,#46768,#46769,#46770,#46771,#46772,#46773,
#46774,#46775,#46776,#46777,#46778,#46779,#46780,#46781,#46782,#46783,#46784,
#46785,#46786,#46787,#46788,#46789,#46790,#46791,#46792,#46793,#46794,#46795,
#46796,#46797,#46798,#46799,#46800,#46801,#46802,#46803,#46804,#46805,#46806,
#46807,#46808,#46809,#46810,#46811,#46812,#46813,#46814,#46815,#46816,#46817,
#46818,#46819,#46820,#46821,#46822,#46823,#46824,#46825,#46826,#46827,#46828,
#46829,#46830,#46831,#46832,#46833,#46834,#46835,#46836,#46837,#46838,#46839,
#46840,#46841,#46842,#46843,#46844,#46845,#46846,#46847,#46848,#46849,#46850,
#46851,#46852,#46853,#46854,#46855,#46856,#46857,#46858,#46859,#46860,#46861,
#46862,#46863,#46864,#46865,#46866,#46867,#46868,#46869,#46870,#46871,#46872,
#46873,#46874,#46875,#46876,#46877,#46878,#46879,#46880,#46881,#46882,#46883,
#46884,#46885,#46886),.UNSPECIFIED.,.F.,.F.,(4,3,3,3,3,3,3,3,3,3,3,3,3,
3,3,3,3,3,3,3,3,3,3,3,3,3,3,3,3,3,3,3,3,3,3,3,3,3,3,3,3,3,3,3,3,3,3,3,3,
3,4),(43.0658133366405,43.1273775675383,43.2151952912012,43.3029022197615,
43.3905213532024,43.4814570520669,43.5689775644036,43.6564851490247,43.7440004596504,
43.8315441504708,43.9191847878258,44.0068829880219,44.09470680642,44.1180069441183,
44.205824667777,44.293531596333,44.3811507297696,44.4720864286357,44.559606940968,
44.6471145255847,44.734629836206,44.8221735270219,44.9098141643725,44.9975123645641,
45.0853361829577,45.1086363206984,45.1964540443579,45.2841609729147,45.3717801063521,
45.4627158052179,45.550236317551,45.6377439021685,45.7252592127906,45.8128029036074,
45.9004435409588,45.9881417411512,46.0759655595457,46.0992656972784,46.1870834209386,
46.2747903494961,46.3624094829342,46.4533451817998,46.5408656941336,46.6283732787517,
46.7158885893746,46.8034322801918,46.8910729175439,46.978771117737,47.0665949361321,
47.0898950738584,47.1238898038469),.UNSPECIFIED.);
#2217=B_SPLINE_CURVE_WITH_KNOTS('',3,(#46892,#46893,#46894,#46895,#46896,
#46897,#46898,#46899,#46900,#46901,#46902,#46903,#46904,#46905,#46906,#46907,
#46908,#46909,#46910,#46911,#46912,#46913,#46914,#46915,#46916,#46917,#46918,
#46919,#46920,#46921,#46922,#46923,#46924,#46925,#46926,#46927,#46928,#46929,
#46930,#46931,#46932,#46933,#46934,#46935,#46936,#46937,#46938,#46939,#46940,
#46941,#46942,#46943,#46944,#46945,#46946,#46947,#46948,#46949,#46950,#46951,
#46952,#46953,#46954,#46955,#46956,#46957,#46958,#46959,#46960,#46961,#46962,
#46963,#46964,#46965,#46966,#46967,#46968,#46969,#46970,#46971,#46972,#46973,
#46974,#46975,#46976,#46977,#46978,#46979,#46980,#46981,#46982,#46983,#46984,
#46985,#46986,#46987,#46988,#46989,#46990,#46991,#46992,#46993,#46994,#46995,
#46996,#46997,#46998,#46999,#47000,#47001,#47002,#47003,#47004,#47005,#47006,
#47007,#47008,#47009,#47010,#47011,#47012,#47013,#47014,#47015,#47016,#47017,
#47018,#47019,#47020,#47021,#47022,#47023,#47024,#47025,#47026,#47027,#47028,
#47029,#47030,#47031,#47032,#47033,#47034,#47035,#47036,#47037,#47038,#47039),
 .UNSPECIFIED.,.F.,.F.,(4,3,3,3,3,3,3,3,3,3,3,3,3,3,3,3,3,3,3,3,3,3,3,3,
3,3,3,3,3,3,3,3,3,3,3,3,3,3,3,3,3,3,3,3,3,3,3,3,3,4),(36.7834780455645,
36.8711108657648,36.9586748083193,37.0462007533675,37.1337093627084,37.2212212918609,
37.3087571936796,37.3963879611388,37.4840723275651,37.571887339318,37.6139016138971,
37.7017193375819,37.7894262661645,37.877045399628,37.9679810984841,38.0555016108438,
38.1430091954881,38.2305245061372,38.318068196981,38.4057088343595,38.4934070345791,
38.5812308530006,38.6045309904771,38.6923487141302,38.7800556426807,38.8676747761118,
38.95861047498,39.0461309873066,39.1336385719176,39.2211538825333,39.3086975733436,
39.3963382106886,39.4840364108747,39.5718602292628,39.5951603670572,39.6829780907142,
39.7706850192685,39.8583041527033,39.9492398515701,40.0367603639005,40.1242679485152,
40.2117832591345,40.2993269499484,40.3869675872969,40.4746657874865,40.5624896058781,
40.5857897436372,40.6987530453545,40.809605914287,40.8407044965425),
 .UNSPECIFIED.);
#2218=B_SPLINE_CURVE_WITH_KNOTS('',3,(#47040,#47041,#47042,#47043,#47044,
#47045,#47046,#47047,#47048,#47049,#47050,#47051,#47052,#47053,#47054,#47055,
#47056,#47057,#47058,#47059,#47060,#47061,#47062,#47063,#47064,#47065,#47066,
#47067,#47068,#47069,#47070,#47071,#47072,#47073,#47074,#47075,#47076,#47077,
#47078,#47079,#47080,#47081,#47082,#47083,#47084,#47085,#47086,#47087,#47088,
#47089,#47090,#47091,#47092,#47093,#47094,#47095,#47096,#47097,#47098,#47099,
#47100,#47101,#47102,#47103,#47104,#47105,#47106,#47107,#47108,#47109,#47110,
#47111,#47112,#47113,#47114,#47115,#47116,#47117,#47118,#47119,#47120,#47121),
 .UNSPECIFIED.,.F.,.F.,(4,3,3,3,3,3,3,3,3,3,3,3,3,3,3,3,3,3,3,3,3,3,3,3,
3,3,3,4),(40.8407044966673,40.9273584362615,41.0139637234795,41.1005454082225,
41.1871250286695,41.2737241173095,41.3604139263767,41.4471549251353,41.5340255171282,
41.5764191202172,41.6642368438759,41.7519437724319,41.8395629058685,41.9304986047346,
42.0180191170668,42.1055267016834,42.1930420123047,42.2805857031209,42.3682263404714,
42.4559245406633,42.543748359057,42.5670484967972,42.6548657905408,42.7425763486081,
42.830186907156,42.9177390596702,43.0052579701374,43.0661059914245),
 .UNSPECIFIED.);
#2219=B_SPLINE_CURVE_WITH_KNOTS('',3,(#47123,#47124,#47125,#47126,#47127,
#47128,#47129,#47130,#47131,#47132,#47133,#47134,#47135,#47136,#47137,#47138,
#47139,#47140,#47141,#47142,#47143,#47144,#47145,#47146,#47147,#47148,#47149,
#47150,#47151,#47152,#47153,#47154,#47155,#47156,#47157,#47158,#47159,#47160,
#47161,#47162,#47163,#47164,#47165,#47166,#47167,#47168,#47169,#47170,#47171,
#47172,#47173,#47174,#47175,#47176,#47177,#47178,#47179,#47180,#47181,#47182,
#47183,#47184,#47185,#47186,#47187,#47188,#47189,#47190,#47191,#47192,#47193,
#47194,#47195,#47196,#47197,#47198,#47199,#47200,#47201),.UNSPECIFIED.,
 .F.,.F.,(4,3,3,3,3,3,3,3,3,3,3,3,3,3,3,3,3,3,3,3,3,3,3,3,3,3,4),(40.8407044968387,
40.9448640923073,41.0502373865446,41.1461188143783,41.2339365380315,41.3216434665819,
41.4092626000131,41.5001982988812,41.5877188112079,41.6752263958189,41.7627417064345,
41.8502853972449,41.9379260345899,42.0256242347759,42.1134480531641,42.1367481909583,
42.2245695490687,42.3122792278308,42.3999002309991,42.4874540507318,42.5749722254939,
42.6624754241108,42.7499842994818,42.8375628990347,42.9251792682886,43.012908486006,
43.0658133366405),.UNSPECIFIED.);
#2220=B_SPLINE_CURVE_WITH_KNOTS('',3,(#47202,#47203,#47204,#47205,#47206,
#47207,#47208,#47209,#47210,#47211,#47212,#47213,#47214,#47215,#47216,#47217,
#47218,#47219,#47220,#47221,#47222,#47223,#47224,#47225,#47226,#47227,#47228,
#47229,#47230,#47231,#47232,#47233,#47234,#47235,#47236,#47237,#47238,#47239,
#47240,#47241,#47242,#47243,#47244,#47245,#47246,#47247,#47248,#47249,#47250,
#47251,#47252,#47253,#47254,#47255,#47256,#47257,#47258,#47259,#47260,#47261,
#47262,#47263,#47264,#47265,#47266,#47267,#47268,#47269,#47270,#47271,#47272,
#47273,#47274,#47275,#47276,#47277,#47278,#47279,#47280,#47281,#47282,#47283,
#47284,#47285,#47286,#47287,#47288,#47289,#47290,#47291,#47292,#47293,#47294,
#47295,#47296,#47297,#47298,#47299,#47300,#47301,#47302,#47303,#47304,#47305,
#47306,#47307,#47308,#47309,#47310,#47311,#47312,#47313,#47314,#47315,#47316,
#47317,#47318,#47319,#47320,#47321,#47322,#47323,#47324,#47325,#47326,#47327,
#47328,#47329,#47330,#47331,#47332,#47333,#47334,#47335,#47336,#47337,#47338,
#47339,#47340,#47341,#47342,#47343,#47344,#47345,#47346,#47347,#47348,#47349),
 .UNSPECIFIED.,.F.,.F.,(4,3,3,3,3,3,3,3,3,3,3,3,3,3,3,3,3,3,3,3,3,3,3,3,
3,3,3,3,3,3,3,3,3,3,3,3,3,3,3,3,3,3,3,3,3,3,3,3,3,4),(36.7826586151206,
36.870191370437,36.9578180400284,37.0454965550951,37.1333080021703,37.1836013080582,
37.271419031912,37.3591259606657,37.4467450943021,37.5376807930941,37.6252013056306,
37.7127088904528,37.8002242012807,37.887767892304,37.9754085298621,38.0631067302617,
38.1509305488621,38.1742306846382,38.2620484082612,38.3497553367814,38.4373744701818,
38.5283101690614,38.6158306813579,38.7033382659388,38.7908535765245,38.8783972673053,
38.9660379046209,39.0537361047776,39.1415599231371,39.1648600612182,39.2526777848493,
39.3403847133773,39.4280038467852,39.5189395456618,39.6064600579642,39.6939676425507,
39.7814829531414,39.8690266439265,39.9566672812459,40.0443654814061,40.1321892997682,
40.1554894377982,40.2428859234006,40.3301773559497,40.417384958565,40.5045298835639,
40.5916445939303,40.6787389693886,40.7658659691,40.8407044966673),
 .UNSPECIFIED.);
#2221=B_SPLINE_CURVE_WITH_KNOTS('',3,(#47355,#47356,#47357,#47358,#47359,
#47360,#47361,#47362,#47363,#47364,#47365,#47366,#47367,#47368,#47369,#47370,
#47371,#47372,#47373,#47374,#47375,#47376,#47377,#47378,#47379,#47380,#47381,
#47382,#47383,#47384,#47385,#47386,#47387,#47388,#47389,#47390,#47391,#47392,
#47393,#47394,#47395,#47396,#47397,#47398,#47399,#47400,#47401,#47402,#47403,
#47404,#47405,#47406,#47407,#47408,#47409,#47410,#47411,#47412,#47413,#47414,
#47415,#47416,#47417,#47418,#47419,#47420,#47421,#47422,#47423,#47424,#47425,
#47426,#47427,#47428,#47429,#47430,#47431,#47432,#47433,#47434,#47435,#47436,
#47437,#47438,#47439,#47440,#47441,#47442,#47443,#47444,#47445,#47446,#47447,
#47448,#47449,#47450,#47451,#47452,#47453,#47454,#47455,#47456,#47457,#47458,
#47459,#47460,#47461,#47462,#47463,#47464,#47465,#47466,#47467,#47468,#47469,
#47470,#47471,#47472,#47473,#47474,#47475,#47476,#47477,#47478,#47479,#47480,
#47481,#47482,#47483,#47484,#47485,#47486,#47487,#47488,#47489,#47490,#47491,
#47492,#47493,#47494,#47495,#47496,#47497,#47498,#47499,#47500,#47501,#47502),
 .UNSPECIFIED.,.F.,.F.,(4,3,3,3,3,3,3,3,3,3,3,3,3,3,3,3,3,3,3,3,3,3,3,3,
3,3,3,3,3,3,3,3,3,3,3,3,3,3,3,3,3,3,3,3,3,3,3,3,3,4),(30.4991828394597,
30.5893394086483,30.6794959778369,30.7673136989568,30.8550206249318,30.9426397557483,
31.0335754555819,31.1210959652133,31.208603547104,31.2961188549769,31.383662543025,
31.4713031775926,31.5590013749893,31.6468251905915,31.6701253544169,31.7579430795362,
31.8456500095705,31.9332691445012,32.0242048428132,32.1117253566694,32.1992329428183,
32.2867482549787,32.3742919473387,32.4619325862332,32.5496307879704,32.6374546079003,
32.660754730997,32.7485724544937,32.8362793828887,32.9238985161654,33.0148342150918,
33.1023547272682,33.1898623117308,33.2773776221998,33.3649213128656,33.4525619500699,
33.5402601501174,33.6280839683712,33.651384107577,33.7382200971852,33.8249459927466,
33.9115858331337,33.9981647376494,34.0847124756428,34.1712506292952,34.2578007687998,
34.3444298629828,34.431103797626,34.517896294785,34.5575191892807),
 .UNSPECIFIED.);
#2222=B_SPLINE_CURVE_WITH_KNOTS('',3,(#47503,#47504,#47505,#47506,#47507,
#47508,#47509,#47510,#47511,#47512,#47513,#47514,#47515,#47516,#47517,#47518,
#47519,#47520,#47521,#47522,#47523,#47524,#47525,#47526,#47527,#47528,#47529,
#47530,#47531,#47532,#47533,#47534,#47535,#47536,#47537,#47538,#47539,#47540,
#47541,#47542,#47543,#47544,#47545,#47546,#47547,#47548,#47549,#47550,#47551,
#47552,#47553,#47554,#47555,#47556,#47557,#47558,#47559,#47560,#47561,#47562,
#47563,#47564,#47565,#47566,#47567,#47568,#47569,#47570,#47571,#47572,#47573,
#47574,#47575,#47576,#47577,#47578,#47579,#47580,#47581,#47582,#47583,#47584),
 .UNSPECIFIED.,.F.,.F.,(4,3,3,3,3,3,3,3,3,3,3,3,3,3,3,3,3,3,3,3,3,3,3,3,
3,3,3,4),(34.5575191894877,34.642013484157,34.7298312080111,34.8175381367651,
34.905157270402,34.9960929691939,35.0836134817308,35.1711210665532,35.2586363773814,
35.3461800684051,35.4338207059635,35.5215189063633,35.6093427249641,35.6326428607371,
35.72046058436,35.8081675128802,35.8957866462808,35.9867223451604,36.0742428574568,
36.1617504420376,36.2492657526232,36.3368094434037,36.4244500807191,36.5121482808759,
36.5999720992353,36.6232722373171,36.7110751632043,36.7834780455645),
 .UNSPECIFIED.);
#2223=B_SPLINE_CURVE_WITH_KNOTS('',3,(#47586,#47587,#47588,#47589,#47590,
#47591,#47592,#47593,#47594,#47595,#47596,#47597,#47598,#47599,#47600,#47601,
#47602,#47603,#47604,#47605,#47606,#47607,#47608,#47609,#47610,#47611,#47612,
#47613,#47614,#47615,#47616,#47617,#47618,#47619,#47620,#47621,#47622,#47623,
#47624,#47625,#47626,#47627,#47628,#47629,#47630,#47631,#47632,#47633,#47634,
#47635,#47636,#47637,#47638,#47639,#47640,#47641,#47642,#47643,#47644,#47645,
#47646,#47647,#47648,#47649,#47650,#47651,#47652,#47653,#47654,#47655,#47656,
#47657,#47658,#47659,#47660,#47661,#47662,#47663,#47664,#47665,#47666,#47667),
 .UNSPECIFIED.,.F.,.F.,(4,3,3,3,3,3,3,3,3,3,3,3,3,3,3,3,3,3,3,3,3,3,3,3,
3,3,3,4),(34.5575191894877,34.6452189800071,34.7329127229688,34.8206207358406,
34.9083633412251,34.9962128842659,35.0841247009675,35.1721722075983,35.2023425548981,
35.2901602783952,35.3778672067906,35.4654863400676,35.5564220389939,35.6439425511707,
35.7314501356336,35.818965446103,35.9065091367695,35.9941497739741,36.081847974022,
36.1696717922762,36.1929719314781,36.2807796092091,36.3684824138462,36.4561011791891,
36.5436546837677,36.6311690801989,36.7186812678158,36.7826586151206),
 .UNSPECIFIED.);
#2224=B_SPLINE_CURVE_WITH_KNOTS('',3,(#47668,#47669,#47670,#47671,#47672,
#47673,#47674,#47675,#47676,#47677,#47678,#47679,#47680,#47681,#47682,#47683,
#47684,#47685,#47686,#47687,#47688,#47689,#47690,#47691,#47692,#47693,#47694,
#47695,#47696,#47697,#47698,#47699,#47700,#47701,#47702,#47703,#47704,#47705,
#47706,#47707,#47708,#47709,#47710,#47711,#47712,#47713,#47714,#47715,#47716,
#47717,#47718,#47719,#47720,#47721,#47722,#47723,#47724,#47725,#47726,#47727,
#47728,#47729,#47730,#47731,#47732,#47733,#47734,#47735,#47736,#47737,#47738,
#47739,#47740,#47741,#47742,#47743,#47744,#47745,#47746,#47747,#47748,#47749,
#47750,#47751,#47752,#47753,#47754,#47755,#47756,#47757,#47758,#47759,#47760,
#47761,#47762,#47763,#47764,#47765,#47766,#47767,#47768,#47769,#47770,#47771,
#47772,#47773,#47774,#47775,#47776,#47777,#47778,#47779,#47780,#47781,#47782,
#47783,#47784,#47785,#47786,#47787,#47788,#47789,#47790,#47791,#47792,#47793,
#47794,#47795,#47796,#47797,#47798,#47799,#47800,#47801,#47802,#47803,#47804,
#47805,#47806,#47807,#47808,#47809,#47810,#47811,#47812,#47813,#47814,#47815),
 .UNSPECIFIED.,.F.,.F.,(4,3,3,3,3,3,3,3,3,3,3,3,3,3,3,3,3,3,3,3,3,3,3,3,
3,3,3,3,3,3,3,3,3,3,3,3,3,3,3,3,3,3,3,3,3,3,3,3,3,4),(30.5003021439847,
30.5878639365854,30.6753888404462,30.7628971791787,30.8504096079639,30.9379467798666,
31.0255791880603,31.1132658881075,31.2010823404694,31.239825048578,31.3276427828231,
31.4153497220844,31.5029688663314,31.5939045611847,31.6814250845207,31.7689326801932,
31.8564480019105,31.9439917038511,32.0316323523121,32.1193305636194,32.2071543930516,
32.230454425158,32.3182721485766,32.405979076915,32.4935982101567,32.5845339091044,
32.6720544212997,32.7595620058012,32.8470773163295,32.9346210070747,33.022261644388,
33.1099598445619,33.1977836629669,33.221083801738,33.3089015228609,33.3966084488389,
33.4842275796583,33.5751632794908,33.6626837891255,33.7501913710195,33.8377066788955,
33.9252503669469,34.0128910015178,34.1005891989182,34.1884130145237,34.2117131783181,
34.3130674767607,34.4140179529609,34.5142334906665,34.5575191892756),
 .UNSPECIFIED.);
#2225=B_SPLINE_CURVE_WITH_KNOTS('',3,(#47821,#47822,#47823,#47824,#47825,
#47826,#47827,#47828,#47829,#47830,#47831,#47832,#47833,#47834,#47835,#47836,
#47837,#47838,#47839,#47840,#47841,#47842,#47843,#47844,#47845,#47846,#47847,
#47848,#47849,#47850,#47851,#47852,#47853,#47854,#47855,#47856,#47857,#47858,
#47859,#47860,#47861,#47862,#47863,#47864,#47865,#47866,#47867,#47868,#47869,
#47870,#47871,#47872,#47873,#47874,#47875,#47876,#47877,#47878,#47879,#47880,
#47881,#47882,#47883,#47884,#47885,#47886,#47887,#47888,#47889,#47890,#47891,
#47892,#47893,#47894,#47895,#47896,#47897,#47898,#47899,#47900,#47901,#47902,
#47903,#47904,#47905,#47906,#47907,#47908,#47909,#47910,#47911,#47912,#47913,
#47914,#47915,#47916,#47917,#47918,#47919,#47920,#47921,#47922,#47923,#47924,
#47925,#47926,#47927,#47928,#47929,#47930,#47931,#47932,#47933,#47934,#47935,
#47936,#47937,#47938,#47939,#47940,#47941,#47942,#47943,#47944,#47945,#47946,
#47947,#47948,#47949,#47950,#47951,#47952,#47953,#47954,#47955,#47956,#47957,
#47958,#47959,#47960,#47961,#47962,#47963,#47964,#47965,#47966,#47967,#47968),
 .UNSPECIFIED.,.F.,.F.,(4,3,3,3,3,3,3,3,3,3,3,3,3,3,3,3,3,3,3,3,3,3,3,3,
3,3,3,3,3,3,3,3,3,3,3,3,3,3,3,3,3,3,3,3,3,3,3,3,3,4),(24.2166325387365,
24.3041405728609,24.3916634012199,24.4792764543864,24.5669348543629,24.6547350011096,
24.7357197183568,24.8235372551853,24.9112439941232,24.9988629354017,25.0897987053436,
25.1773190203967,25.2648264061816,25.3523415166308,25.4398850061448,25.5275254415223,
25.6152234391129,25.7030470555221,25.7263490949368,25.8141668925815,25.9018738958755,
25.9894931047059,26.0804287755572,26.1679493644343,26.2554570258878,26.3429724135546,
26.4305161815409,26.5181568958598,26.6058551729917,26.6936790676986,26.7169784715168,
26.8047962015636,26.8925031367968,26.9801222771902,27.0710579735536,27.1585784935006,
27.2460860859628,27.333601404653,27.4211451037538,27.5087857496696,27.5964839586007,
27.6843077859232,27.7076078480968,27.7974230784913,27.8871096033198,27.9766848887918,
28.0661443688007,28.1555356972699,28.2448677617403,28.2743338823081),
 .UNSPECIFIED.);
#2226=B_SPLINE_CURVE_WITH_KNOTS('',3,(#47969,#47970,#47971,#47972,#47973,
#47974,#47975,#47976,#47977,#47978,#47979,#47980,#47981,#47982,#47983,#47984,
#47985,#47986,#47987,#47988,#47989,#47990,#47991,#47992,#47993,#47994,#47995,
#47996,#47997,#47998,#47999,#48000,#48001,#48002,#48003,#48004,#48005,#48006,
#48007,#48008,#48009,#48010,#48011,#48012,#48013,#48014,#48015,#48016,#48017,
#48018,#48019,#48020,#48021,#48022,#48023,#48024,#48025,#48026,#48027,#48028,
#48029,#48030,#48031,#48032,#48033,#48034,#48035,#48036,#48037,#48038,#48039,
#48040,#48041,#48042,#48043,#48044,#48045,#48046,#48047,#48048,#48049,#48050),
 .UNSPECIFIED.,.F.,.F.,(4,3,3,3,3,3,3,3,3,3,3,3,3,3,3,3,3,3,3,3,3,3,3,3,
3,3,3,4),(28.2743338824685,28.3691609662208,28.464391316564,28.5598306389529,
28.6555712299543,28.6982372246769,28.786054958936,28.8737618982115,28.9613810424729,
29.0523167373209,29.1398372606714,29.2273448563586,29.3148601780908,29.4024038800461,
29.4900445285221,29.5777427398441,29.6655665692908,29.6888666012569,29.7766954664342,
29.8670063880624,29.9546150751734,30.0421656114966,30.1296786986772,30.2171750058131,
30.3047012605698,30.3922463238332,30.479860093122,30.4991828394597),
 .UNSPECIFIED.);
#2227=B_SPLINE_CURVE_WITH_KNOTS('',3,(#48052,#48053,#48054,#48055,#48056,
#48057,#48058,#48059,#48060,#48061,#48062,#48063,#48064,#48065,#48066,#48067,
#48068,#48069,#48070,#48071,#48072,#48073,#48074,#48075,#48076,#48077,#48078,
#48079,#48080,#48081,#48082,#48083,#48084,#48085,#48086,#48087,#48088,#48089,
#48090,#48091,#48092,#48093,#48094,#48095,#48096,#48097,#48098,#48099,#48100,
#48101,#48102,#48103,#48104,#48105,#48106,#48107,#48108,#48109,#48110,#48111,
#48112,#48113,#48114,#48115,#48116,#48117,#48118,#48119,#48120,#48121,#48122,
#48123,#48124,#48125,#48126,#48127,#48128,#48129,#48130,#48131,#48132,#48133),
 .UNSPECIFIED.,.F.,.F.,(4,3,3,3,3,3,3,3,3,3,3,3,3,3,3,3,3,3,3,3,3,3,3,3,
3,3,3,4),(28.2743338824878,28.3620520323679,28.4496594845734,28.5371793604949,
28.6273527273603,28.7147750528498,28.8021848308995,28.8896028239389,28.9770497952893,
29.0645937597082,29.1521960301773,29.2399225718329,29.2585662954179,29.3463840254668,
29.434090960702,29.5217101010972,29.6126457974598,29.7001663174082,29.7876739098713,
29.8751892285622,29.9627329276637,30.0503735735801,30.1380717825111,30.2258956098337,
30.249195671998,30.3370125831573,30.4247057975662,30.5003021439847),
 .UNSPECIFIED.);
#2228=B_SPLINE_CURVE_WITH_KNOTS('',3,(#48134,#48135,#48136,#48137,#48138,
#48139,#48140,#48141,#48142,#48143,#48144,#48145,#48146,#48147,#48148,#48149,
#48150,#48151,#48152,#48153,#48154,#48155,#48156,#48157,#48158,#48159,#48160,
#48161,#48162,#48163,#48164,#48165,#48166,#48167,#48168,#48169,#48170,#48171,
#48172,#48173,#48174,#48175,#48176,#48177,#48178,#48179,#48180,#48181,#48182,
#48183,#48184,#48185,#48186,#48187,#48188,#48189,#48190,#48191,#48192,#48193,
#48194,#48195,#48196,#48197,#48198,#48199,#48200,#48201,#48202,#48203,#48204,
#48205,#48206,#48207,#48208,#48209,#48210,#48211,#48212,#48213,#48214,#48215,
#48216,#48217,#48218,#48219,#48220,#48221,#48222,#48223,#48224,#48225,#48226,
#48227,#48228,#48229,#48230,#48231,#48232,#48233,#48234,#48235,#48236,#48237,
#48238,#48239,#48240,#48241,#48242,#48243,#48244,#48245,#48246,#48247,#48248,
#48249,#48250,#48251,#48252,#48253,#48254,#48255,#48256,#48257,#48258,#48259,
#48260,#48261,#48262,#48263,#48264,#48265,#48266,#48267,#48268,#48269,#48270,
#48271,#48272,#48273,#48274,#48275,#48276,#48277,#48278,#48279,#48280,#48281,
#48282,#48283,#48284),.UNSPECIFIED.,.F.,.F.,(4,3,3,3,3,3,3,3,3,3,3,3,3,
3,3,3,3,3,3,3,3,3,3,3,3,3,3,3,3,3,3,3,3,3,3,3,3,3,3,3,3,3,3,3,3,3,3,3,3,
3,4),(24.21616161747,24.3054194125178,24.393235611936,24.4809409946289,
24.5685585625919,24.6594948409052,24.7470137487717,24.8345197172836,24.9220334018862,
25.0095754584884,25.0972144576362,25.1849110153759,25.2727331975642,25.2960487890978,
25.3838670030276,25.4715744261254,25.5591940577416,25.6501295712336,25.7376505876018,
25.8251586775367,25.9126744942071,26.000218691252,26.0878598325432,26.1755585359319,
26.2633828525917,26.2866781656779,26.3744960038223,26.4622030499671,26.5498223039364,
26.6407579587266,26.7282785982027,26.8157863121929,26.9033017542858,26.9908455785413,
27.0784863515969,27.1661846889744,27.254008645693,27.2773075422579,27.3651250792531,
27.4528318183603,27.5404507598101,27.6313865296886,27.7189068449178,27.8064142308805,
27.8939293415086,27.9814728312022,28.0691132667604,28.1568112645317,28.2446348811215,
28.2679369188379,28.2743338823081),.UNSPECIFIED.);
#2229=B_SPLINE_CURVE_WITH_KNOTS('',3,(#48290,#48291,#48292,#48293,#48294,
#48295,#48296,#48297,#48298,#48299,#48300,#48301,#48302,#48303,#48304,#48305,
#48306,#48307,#48308,#48309,#48310,#48311,#48312,#48313,#48314,#48315,#48316,
#48317,#48318,#48319,#48320,#48321,#48322,#48323,#48324,#48325,#48326,#48327,
#48328,#48329,#48330,#48331,#48332,#48333,#48334,#48335,#48336,#48337,#48338,
#48339,#48340,#48341,#48342,#48343,#48344,#48345,#48346,#48347,#48348,#48349,
#48350,#48351,#48352,#48353,#48354,#48355,#48356,#48357,#48358,#48359,#48360,
#48361,#48362,#48363,#48364,#48365,#48366,#48367,#48368,#48369,#48370,#48371),
 .UNSPECIFIED.,.F.,.F.,(4,3,3,3,3,3,3,3,3,3,3,3,3,3,3,3,3,3,3,3,3,3,3,3,
3,3,3,4),(15.7079632679489,15.7946698168415,15.8813534775319,15.9680356344082,
16.0547376665272,16.1415361894612,16.2283857888847,16.3153785783739,16.3803843998776,
16.4682788564933,16.5560621028591,16.6437570426224,16.7346641343518,16.8222586496917,
16.9098394322283,16.9974270480132,17.0850420628687,17.1727521940932,17.2605188998545,
17.3484092437941,17.3710137764576,17.4589624658426,17.5468080500348,17.6345711957375,
17.7222691239434,17.8099293002927,17.8975816624113,17.9331385422654),
 .UNSPECIFIED.);
#2230=B_SPLINE_CURVE_WITH_KNOTS('',3,(#48373,#48374,#48375,#48376,#48377),
 .UNSPECIFIED.,.F.,.F.,(4,1,4),(14.3991256467175,15.3897550232976,15.7079550217499),
 .UNSPECIFIED.);
#2231=B_SPLINE_CURVE_WITH_KNOTS('',3,(#48381,#48382,#48383,#48384,#48385,
#48386,#48387,#48388,#48389,#48390,#48391,#48392,#48393,#48394,#48395,#48396,
#48397,#48398,#48399,#48400,#48401,#48402,#48403,#48404,#48405,#48406,#48407,
#48408,#48409,#48410,#48411,#48412,#48413,#48414,#48415,#48416,#48417,#48418,
#48419,#48420,#48421,#48422,#48423,#48424,#48425,#48426,#48427,#48428,#48429,
#48430,#48431,#48432,#48433,#48434,#48435,#48436,#48437,#48438,#48439,#48440,
#48441,#48442,#48443,#48444),.UNSPECIFIED.,.F.,.F.,(4,3,3,3,3,3,3,3,3,3,
3,3,3,3,3,3,3,3,3,3,3,4),(13.8752087520864,13.9625601789458,14.0498018549144,
14.1369573059842,14.2240519813441,14.3111146099278,14.3981663291118,14.4852282634698,
14.5723751741815,14.6595642711191,14.7468925938367,14.8294259525565,14.9162044274587,
15.0028750659864,15.0910110912051,15.1775387458644,15.2640376537039,15.3505294393131,
15.439887896419,15.5264717573148,15.6172175125258,15.7079632677367),
 .UNSPECIFIED.);
#2232=B_SPLINE_CURVE_WITH_KNOTS('',3,(#48445,#48446,#48447,#48448,#48449,
#48450,#48451,#48452,#48453,#48454,#48455,#48456,#48457,#48458,#48459,#48460,
#48461,#48462,#48463,#48464,#48465,#48466,#48467,#48468,#48469,#48470,#48471,
#48472,#48473,#48474,#48475,#48476,#48477,#48478,#48479,#48480,#48481,#48482,
#48483,#48484,#48485,#48486,#48487,#48488,#48489,#48490,#48491,#48492,#48493,
#48494,#48495,#48496,#48497,#48498,#48499,#48500,#48501,#48502,#48503,#48504,
#48505,#48506,#48507,#48508,#48509,#48510,#48511,#48512,#48513,#48514,#48515,
#48516,#48517,#48518,#48519,#48520,#48521,#48522,#48523,#48524,#48525,#48526),
 .UNSPECIFIED.,.F.,.F.,(4,3,3,3,3,3,3,3,3,3,3,3,3,3,3,3,3,3,3,3,3,3,3,3,
3,3,3,4),(15.7079632679489,15.8200553291365,15.9077800709228,15.9953928439823,
16.082916768368,16.1738877605365,16.2613110318231,16.3487207906136,16.436137793803,
16.523582798485,16.6111246793828,16.6987239645013,16.7864493875845,16.8106847057165,
16.8985189524792,16.9862424441556,17.0738781598958,17.1648076501959,17.2523446830397,
17.3398687358889,17.4274004439648,17.5149604428944,17.6026171724979,17.6903313578386,
17.7781708816529,17.8013140822966,17.8891423167076,17.9338728886362),
 .UNSPECIFIED.);
#2233=B_SPLINE_CURVE_WITH_KNOTS('',3,(#48532,#48533,#48534,#48535,#48536,
#48537,#48538,#48539,#48540,#48541,#48542,#48543,#48544,#48545,#48546,#48547,
#48548,#48549,#48550,#48551,#48552,#48553,#48554,#48555,#48556,#48557,#48558,
#48559,#48560,#48561,#48562,#48563,#48564,#48565,#48566,#48567,#48568,#48569,
#48570,#48571,#48572,#48573,#48574,#48575,#48576,#48577,#48578,#48579,#48580,
#48581,#48582,#48583,#48584,#48585,#48586,#48587,#48588,#48589,#48590,#48591,
#48592,#48593,#48594,#48595,#48596,#48597,#48598,#48599,#48600,#48601,#48602,
#48603,#48604,#48605,#48606,#48607,#48608,#48609,#48610,#48611,#48612,#48613,
#48614,#48615,#48616,#48617,#48618,#48619,#48620,#48621,#48622,#48623,#48624,
#48625,#48626,#48627,#48628),.UNSPECIFIED.,.F.,.F.,(4,3,3,3,3,3,3,3,3,3,
3,3,3,3,3,3,3,3,3,3,3,3,3,3,3,3,3,3,3,3,3,3,4),(64.4958654892591,64.5878117777329,
64.6796687687264,64.7714674489333,64.8632367224699,64.9550002532635,65.0467816942969,
65.1386612087587,65.230593746165,65.32267279102,65.3815388542818,65.4726934888845,
65.5637267792503,65.65466617812,65.7455446050282,65.8363918516251,65.9272325688873,
66.0180913969724,66.1090575805604,66.2000783819247,66.2912666572051,66.3721682308618,
66.4666159606274,66.5609259986622,66.655120074501,66.7492038319741,66.8432231820123,
66.9371975924462,67.0311464863855,67.1251148440193,67.2190914006473,67.3131312555883,
67.3627976074418),.UNSPECIFIED.);
#2234=B_SPLINE_CURVE_WITH_KNOTS('',3,(#48636,#48637,#48638,#48639,#48640,
#48641,#48642,#48643,#48644,#48645,#48646,#48647,#48648,#48649,#48650,#48651,
#48652,#48653,#48654,#48655,#48656,#48657,#48658,#48659,#48660,#48661,#48662,
#48663,#48664,#48665,#48666,#48667,#48668,#48669,#48670,#48671,#48672,#48673,
#48674,#48675,#48676,#48677,#48678,#48679,#48680,#48681,#48682,#48683,#48684,
#48685,#48686,#48687,#48688,#48689,#48690,#48691,#48692,#48693,#48694,#48695,
#48696,#48697,#48698,#48699,#48700,#48701,#48702,#48703,#48704,#48705,#48706,
#48707,#48708,#48709,#48710,#48711,#48712,#48713,#48714,#48715,#48716,#48717,
#48718,#48719,#48720,#48721,#48722,#48723,#48724,#48725,#48726,#48727,#48728,
#48729,#48730,#48731,#48732,#48733,#48734,#48735,#48736,#48737,#48738,#48739,
#48740,#48741,#48742,#48743,#48744,#48745,#48746,#48747,#48748,#48749,#48750,
#48751,#48752,#48753,#48754,#48755,#48756,#48757,#48758,#48759,#48760,#48761,
#48762,#48763,#48764,#48765,#48766,#48767,#48768,#48769,#48770,#48771,#48772,
#48773),.UNSPECIFIED.,.F.,.F.,(4,2,2,2,2,2,2,2,2,2,2,2,2,2,2,2,2,2,2,2,
2,2,2,2,2,2,2,2,2,2,2,2,2,2,2,2,2,2,2,2,2,2,2,2,2,2,2,2,2,2,2,2,2,2,2,2,
2,2,2,2,2,2,2,2,2,2,2,2,4),(-3.8159802817818,-3.80236928524017,-3.75530370914742,
-3.70539731607039,-3.67564854302536,-3.6642164672265,-3.65598257013116,
-3.64735517776101,-3.63386237542377,-3.5789052995534,-3.53734500310367,
-3.51562868770045,-3.50122878070881,-3.49507048308581,-3.49052592416303,
-3.48509252990008,-3.47446797917823,-3.41948587521002,-3.37154346450627,
-3.34261109281059,-3.33134419424982,-3.32318920456458,-3.31461302861812,
-3.30114856638697,-3.24798780205897,-3.19268324308138,-3.17557277292305,
-3.16343646290805,-3.15773838047819,-3.15369957451371,-3.14830620227463,
-3.13797979421403,-3.08043879953883,-3.03375250468406,-3.00528314402067,
-2.99414913468061,-2.98608602511283,-2.97760658199937,-2.96430289364066,
-2.9143495461893,-2.84003610723327,-2.82685565896935,-2.82100429808657,
-2.81657562389555,-2.81113520453627,-2.80065823852271,-2.74667311239221,
-2.69768131291251,-2.66836269863596,-2.65706395587901,-2.64892354714072,
-2.64039685966665,-2.62708318745669,-2.57794967788699,-2.51997090039894,
-2.49423218958418,-2.48677658100827,-2.48202656404952,-2.47722287235016,
-2.46948479101221,-2.44309613626079,-2.37758240781103,-2.33531134436267,
-2.32269382308117,-2.31431656263378,-2.30619527608143,-2.29634492992303,
-2.27167043501862,-2.25604913488483),.UNSPECIFIED.);
#2235=B_SPLINE_CURVE_WITH_KNOTS('',3,(#48779,#48780,#48781,#48782,#48783,
#48784,#48785,#48786,#48787,#48788,#48789,#48790,#48791,#48792,#48793,#48794,
#48795,#48796,#48797,#48798,#48799,#48800,#48801,#48802,#48803,#48804,#48805,
#48806,#48807,#48808,#48809,#48810,#48811,#48812,#48813,#48814,#48815,#48816,
#48817,#48818,#48819,#48820,#48821,#48822,#48823,#48824,#48825,#48826,#48827,
#48828,#48829,#48830,#48831,#48832,#48833,#48834,#48835,#48836,#48837,#48838,
#48839,#48840,#48841,#48842,#48843,#48844,#48845,#48846,#48847,#48848,#48849,
#48850,#48851,#48852,#48853,#48854,#48855,#48856,#48857,#48858,#48859,#48860,
#48861,#48862,#48863,#48864,#48865,#48866,#48867,#48868,#48869,#48870,#48871,
#48872,#48873,#48874,#48875,#48876,#48877,#48878,#48879,#48880,#48881,#48882,
#48883,#48884,#48885,#48886,#48887,#48888,#48889,#48890,#48891,#48892,#48893,
#48894,#48895,#48896,#48897,#48898,#48899,#48900,#48901,#48902,#48903,#48904,
#48905,#48906,#48907,#48908,#48909,#48910,#48911,#48912,#48913,#48914,#48915,
#48916,#48917,#48918,#48919,#48920,#48921,#48922,#48923,#48924,#48925,#48926,
#48927,#48928,#48929,#48930,#48931,#48932,#48933,#48934,#48935,#48936,#48937,
#48938,#48939,#48940,#48941,#48942,#48943,#48944,#48945,#48946,#48947,#48948,
#48949,#48950,#48951,#48952,#48953,#48954,#48955,#48956),.UNSPECIFIED.,
 .F.,.F.,(4,2,2,2,2,2,2,2,2,2,2,2,2,2,2,2,2,2,2,2,2,2,2,2,2,2,2,2,2,2,2,
2,2,2,2,2,2,2,2,2,2,2,2,2,2,2,2,2,2,2,2,2,2,2,2,2,2,2,2,2,2,2,2,2,2,2,2,
2,2,2,2,2,2,2,2,2,2,2,2,2,2,2,2,2,2,2,2,2,4),(-2.01524637946625,-1.97117235359194,
-1.94754198410681,-1.94008740470034,-1.93581638535977,-1.9311412347247,
-1.9240042022512,-1.90147334034537,-1.85704954887112,-1.79532974948722,
-1.7794104985436,-1.77026883070907,-1.76231858115783,-1.75237729671238,
-1.7318167846165,-1.70352017593473,-1.6379760780529,-1.61157416540518,-1.60386591515836,
-1.599071971706,-1.59433952209767,-1.58690611473692,-1.56122832853527,-1.50360611181347,
-1.45354024952445,-1.44020574428231,-1.43169081758819,-1.42358066511926,
-1.41235683362176,-1.38346177215334,-1.33563610667739,-1.28006147076001,
-1.26962145811798,-1.26419190422336,-1.25970354180774,-1.25377248259357,
-1.24026025600279,-1.2203710498627,-1.13927393268819,-1.11223801117913,
-1.10100549967706,-1.09296737951648,-1.08446141052123,-1.07120127978754,
-1.0184293339982,-0.942861807503496,-0.932758346196491,-0.927394150303743,
-0.922883724142963,-0.916822306019369,-0.902590749912535,-0.881187682739607,
-0.831583136723827,-0.780875674958192,-0.767517114608159,-0.758981876333513,
-0.750847493623583,-0.739580408237012,-0.710495026366432,-0.66218164615411,
-0.607297393457773,-0.596820714586557,-0.591380744981763,-0.58695263940325,
-0.58110226227966,-0.567925162310321,-0.493673847496277,-0.443617250335225,
-0.430310419772939,-0.421831183565596,-0.41376984617743,-0.40264082068429,
-0.374198582348755,-0.327584026627377,-0.270017981651149,-0.259699110258334,
-0.25430785025771,-0.250269655836963,-0.244571093057724,-0.232428975475039,
-0.215304479889232,-0.159910383024156,-0.106818477230286,-0.0933557651507457,
-0.0847809752165488,-0.0766275291918341,-0.0685599868093,-0.0576300795599785,
-0.00100809160743357),.UNSPECIFIED.);
#2236=B_SPLINE_CURVE_WITH_KNOTS('',3,(#48957,#48958,#48959,#48960,#48961,
#48962,#48963,#48964,#48965,#48966,#48967,#48968,#48969,#48970,#48971,#48972),
 .UNSPECIFIED.,.F.,.F.,(4,3,3,3,3,4),(64.1406906932476,64.2573846340332,
64.3763846980835,64.3909094777018,64.4829991505123,64.4958654892591),
 .UNSPECIFIED.);
#2237=B_SPLINE_CURVE_WITH_KNOTS('',3,(#48973,#48974,#48975,#48976,#48977,
#48978,#48979,#48980,#48981,#48982,#48983,#48984,#48985,#48986,#48987,#48988,
#48989,#48990,#48991,#48992,#48993,#48994,#48995,#48996,#48997,#48998,#48999,
#49000,#49001,#49002,#49003,#49004,#49005,#49006,#49007,#49008,#49009,#49010,
#49011,#49012,#49013,#49014,#49015,#49016,#49017,#49018,#49019,#49020,#49021,
#49022,#49023,#49024,#49025,#49026,#49027,#49028,#49029,#49030,#49031,#49032,
#49033,#49034,#49035,#49036,#49037,#49038,#49039,#49040,#49041,#49042,#49043,
#49044,#49045,#49046,#49047,#49048,#49049,#49050,#49051,#49052,#49053,#49054,
#49055,#49056,#49057,#49058,#49059,#49060,#49061,#49062,#49063,#49064,#49065,
#49066,#49067,#49068,#49069,#49070,#49071,#49072,#49073,#49074,#49075,#49076,
#49077,#49078,#49079,#49080,#49081,#49082,#49083,#49084,#49085,#49086,#49087,
#49088,#49089,#49090,#49091,#49092,#49093,#49094,#49095,#49096,#49097,#49098,
#49099,#49100,#49101,#49102,#49103,#49104,#49105,#49106,#49107,#49108,#49109,
#49110,#49111,#49112,#49113,#49114,#49115,#49116,#49117,#49118,#49119,#49120,
#49121,#49122,#49123,#49124,#49125,#49126,#49127,#49128,#49129,#49130,#49131,
#49132,#49133,#49134,#49135,#49136,#49137,#49138,#49139,#49140,#49141,#49142,
#49143,#49144,#49145,#49146,#49147,#49148,#49149,#49150,#49151,#49152,#49153,
#49154,#49155,#49156,#49157,#49158,#49159,#49160,#49161,#49162),
 .UNSPECIFIED.,.F.,.F.,(4,2,2,2,2,2,2,2,2,2,2,2,2,2,2,2,2,2,2,2,2,2,2,2,
2,2,2,2,2,2,2,2,2,2,2,2,2,2,2,2,2,2,2,2,2,2,2,2,2,2,2,2,2,2,2,2,2,2,2,2,
2,2,2,2,2,2,2,2,2,2,2,2,2,2,2,2,2,2,2,2,2,2,2,2,2,2,2,2,2,2,2,2,2,2,4),
(-2.25604913488483,-2.18785682196863,-2.1677665984532,-2.15415633770891,
-2.14820831459379,-2.14371811797818,-2.13829994497247,-2.12758962218332,
-2.07535601862155,-2.02532397048771,-1.99567874743702,-1.9843558171834,
-1.9762281176329,-1.96774225382847,-1.95455337705862,-1.90821016361135,
-1.89800167760216,-1.84039253906393,-1.82020439264348,-1.81312844983984,
-1.8089297603779,-1.80417554470848,-1.79665363768787,-1.76999657250674,
-1.70731917786023,-1.66295132923247,-1.64987267443735,-1.6414034449495,
-1.63325244010934,-1.62183055829978,-1.59145440354981,-1.51186515502239,
-1.4850327587046,-1.47727675810207,-1.47247099490959,-1.46774153435521,
-1.46033774641746,-1.43504432541337,-1.37927263921278,-1.32705473382731,
-1.31366328842835,-1.30513166470767,-1.29701900053342,-1.28581315536973,
-1.2570980580444,-1.20980433332651,-1.15335997391034,-1.14295942718709,
-1.1375357734097,-1.13304479263005,-1.12709928463253,-1.11350267226373,
-1.09343690594463,-1.00996122365891,-0.985048121694844,-0.97516537845347,
-0.96703905858256,-0.958678447450702,-0.946129553874666,-0.904674580323758,
-0.863705539291906,-0.813492846415116,-0.80488680199612,-0.79990010068119,
-0.795294144258878,-0.788513475771654,-0.769122775692711,-0.734859512674769,
-0.657191088238776,-0.642073170891989,-0.633186072483549,-0.625198026828659,
-0.614849270916213,-0.591903637284072,-0.558745703553591,-0.494445285291431,
-0.474004190800517,-0.466894047003265,-0.462687188973309,-0.457940424847267,
-0.450451651684341,-0.42417839347516,-0.363549730670916,-0.316901444116721,
-0.303730372528516,-0.295244402092222,-0.287108117489695,-0.275758635725873,
-0.245937237329409,-0.195376087353446,-0.143900431522099,-0.133244640209012,
-0.127835451999951,-0.123343133097485,-0.121334274483195),.UNSPECIFIED.);
#2238=B_SPLINE_CURVE_WITH_KNOTS('',3,(#49167,#49168,#49169,#49170,#49171,
#49172,#49173,#49174,#49175,#49176,#49177,#49178,#49179,#49180,#49181,#49182,
#49183,#49184,#49185,#49186,#49187,#49188,#49189,#49190,#49191,#49192,#49193,
#49194,#49195,#49196,#49197,#49198,#49199,#49200,#49201,#49202,#49203,#49204,
#49205,#49206,#49207,#49208,#49209,#49210,#49211,#49212,#49213,#49214,#49215,
#49216,#49217,#49218,#49219,#49220,#49221,#49222,#49223,#49224,#49225,#49226,
#49227,#49228,#49229,#49230,#49231,#49232,#49233,#49234,#49235,#49236,#49237,
#49238,#49239,#49240,#49241,#49242,#49243,#49244,#49245,#49246,#49247,#49248,
#49249,#49250,#49251,#49252,#49253,#49254,#49255,#49256,#49257,#49258,#49259,
#49260,#49261,#49262,#49263,#49264,#49265,#49266,#49267,#49268,#49269,#49270,
#49271,#49272,#49273,#49274,#49275,#49276,#49277,#49278,#49279,#49280,#49281,
#49282,#49283,#49284,#49285,#49286,#49287,#49288,#49289,#49290,#49291,#49292,
#49293,#49294,#49295,#49296,#49297,#49298,#49299,#49300,#49301,#49302,#49303,
#49304,#49305,#49306,#49307,#49308,#49309,#49310,#49311,#49312,#49313,#49314,
#49315,#49316,#49317,#49318,#49319,#49320,#49321,#49322,#49323,#49324,#49325,
#49326,#49327,#49328,#49329,#49330,#49331,#49332,#49333,#49334,#49335,#49336,
#49337,#49338,#49339,#49340,#49341,#49342,#49343,#49344,#49345,#49346,#49347,
#49348,#49349,#49350,#49351,#49352,#49353,#49354,#49355,#49356,#49357,#49358,
#49359,#49360),.UNSPECIFIED.,.F.,.F.,(4,2,2,2,2,2,2,2,2,2,2,2,2,2,2,2,2,
2,2,2,2,2,2,2,2,2,2,2,2,2,2,2,2,2,2,2,2,2,2,2,2,2,2,2,2,2,2,2,2,2,2,2,2,
2,2,2,2,2,2,2,2,2,2,2,2,2,2,2,2,2,2,2,2,2,2,2,2,2,2,2,2,2,2,2,2,2,2,2,2,
2,2,2,2,2,2,2,4),(-4.14968971221015,-4.14613951770191,-4.13262163571353,
-4.12406566573447,-4.11596862875263,-4.10484711285268,-4.07852895524875,
-3.99670216147919,-3.97676939988255,-3.96323638410418,-3.95730208629117,
-3.95281245028536,-3.94738170196693,-3.93661443909146,-3.89098960514216,
-3.85089696882983,-3.82210862915545,-3.80129997335259,-3.7913166767727,
-3.78343838033831,-3.7743585808226,-3.75871950313345,-3.68813361491474,
-3.63256265076525,-3.62386903190368,-3.61886365513924,-3.61431976026846,
-3.60870090187122,-3.59459458900767,-3.53195385063498,-3.51759732217433,
-3.48696491482241,-3.46523327149188,-3.45508900339031,-3.4471237372455,
-3.43812138120597,-3.42284367255486,-3.34813929946971,-3.31229871400597,
-3.29237302873156,-3.28552826973011,-3.28091088650699,-3.27594737989848,
-3.26744946343817,-3.22429086396982,-3.16499709098304,-3.13258183956557,
-3.12091628752857,-3.11272446056812,-3.10530952507597,-3.09530962117868,
-3.06916829712429,-2.98922582993614,-2.96803754036205,-2.95390921989029,
-2.94787581874199,-2.94337753239159,-2.9380166087374,-2.92791376940292,
-2.86711668424234,-2.8224084221447,-2.79463084720547,-2.78355320158664,
-2.77546252641307,-2.76689014345078,-2.75329564111982,-2.69304424079818,
-2.64395541033935,-2.62020570696751,-2.61294807566401,-2.6082498829655,
-2.60400461130362,-2.59668223221427,-2.57437218158575,-2.51182753723812,
-2.47896322475052,-2.45615794159679,-2.44583366787227,-2.43785007869641,
-2.4289533173454,-2.41378162372494,-2.33662853949002,-2.28623673404108,
-2.27765066894587,-2.27266847580768,-2.26811427010957,-2.26136667566018,
-2.24365075162703,-2.18403519633135,-2.13587825420236,-2.11915654499046,
-2.10898295059721,-2.10101446510982,-2.09202920817599,-2.07643016420023,
-2.02613671851317,-2.01524637946625),.UNSPECIFIED.);
#2239=B_SPLINE_CURVE_WITH_KNOTS('',3,(#49362,#49363,#49364,#49365,#49366,
#49367,#49368,#49369,#49370,#49371),.UNSPECIFIED.,.F.,.F.,(4,2,2,2,4),(-0.121334274483195,
-0.117378401436383,-0.103666538849867,-0.0833593375923389,-0.000975325102178241),
 .UNSPECIFIED.);
#2240=B_SPLINE_CURVE_WITH_KNOTS('',3,(#49372,#49373,#49374,#49375,#49376,
#49377,#49378,#49379,#49380,#49381,#49382,#49383,#49384,#49385,#49386,#49387,
#49388,#49389,#49390,#49391,#49392,#49393,#49394,#49395,#49396,#49397,#49398,
#49399,#49400,#49401,#49402,#49403,#49404,#49405,#49406,#49407,#49408,#49409,
#49410,#49411,#49412,#49413,#49414,#49415,#49416,#49417,#49418,#49419,#49420,
#49421,#49422,#49423,#49424,#49425,#49426,#49427,#49428,#49429,#49430,#49431,
#49432,#49433,#49434,#49435,#49436,#49437,#49438,#49439,#49440,#49441,#49442,
#49443,#49444,#49445,#49446,#49447,#49448,#49449,#49450,#49451,#49452,#49453,
#49454,#49455,#49456,#49457,#49458,#49459,#49460,#49461,#49462,#49463,#49464,
#49465,#49466,#49467,#49468,#49469,#49470,#49471,#49472,#49473,#49474,#49475,
#49476,#49477,#49478,#49479,#49480,#49481,#49482,#49483,#49484,#49485,#49486,
#49487,#49488,#49489,#49490,#49491,#49492,#49493,#49494,#49495,#49496,#49497,
#49498,#49499,#49500,#49501,#49502,#49503,#49504,#49505,#49506,#49507,#49508,
#49509,#49510,#49511,#49512,#49513,#49514,#49515,#49516,#49517,#49518,#49519,
#49520,#49521,#49522,#49523,#49524,#49525,#49526,#49527,#49528,#49529,#49530,
#49531,#49532,#49533,#49534,#49535,#49536,#49537,#49538,#49539,#49540,#49541,
#49542,#49543,#49544,#49545,#49546,#49547,#49548,#49549),.UNSPECIFIED.,
 .F.,.F.,(4,2,2,2,2,2,2,2,2,2,2,2,2,2,2,2,2,2,2,2,2,2,2,2,2,2,2,2,2,2,2,
2,2,2,2,2,2,2,2,2,2,2,2,2,2,2,2,2,2,2,2,2,2,2,2,2,2,2,2,2,2,2,2,2,2,2,2,
2,2,2,2,2,2,2,2,2,2,2,2,2,2,2,2,2,2,2,2,2,4),(-4.27069253146465,-4.25382227564401,
-4.2410426801416,-4.23324808460416,-4.22556529108036,-4.21681634818942,
-4.20237008358997,-4.1342605407797,-4.0923109481809,-4.07047931789365,-4.06341753057571,
-4.05875809547891,-4.05447147190329,-4.04693624734976,-4.0224311118733,
-3.96189731402034,-3.91320956523195,-3.90015976209251,-3.89169779047831,
-3.88363791998101,-3.87226738797422,-3.84442414769242,-3.76445167164648,
-3.74466127208302,-3.73119589173919,-3.72527210468108,-3.72078221765012,
-3.71534109709162,-3.70452486961746,-3.6591753402215,-3.61948628985693,
-3.57591319779884,-3.56319850511883,-3.55480381666027,-3.5467000203529,
-3.53691322525324,-3.51263421085097,-3.42838703269747,-3.40827009117478,
-3.39464748699942,-3.38869703966519,-3.38420502666613,-3.37878347287155,
-3.36806797283986,-3.32458313858687,-3.2872941225708,-3.2555937538825,-3.23334059738502,
-3.22310601583075,-3.21512974845548,-3.20617720020493,-3.19074416813872,
-3.11575537148139,-3.08005534121769,-3.06017455323844,-3.05333398191888,
-3.04871648592878,-3.04374955702078,-3.0352395509004,-2.99017113554231,
-2.91447268163651,-2.89515239069106,-2.8854374846631,-2.87827014713962,
-2.86924687178384,-2.85387762247084,-2.78001722702751,-2.72705236436821,
-2.71843083651246,-2.71344005991677,-2.70888778972161,-2.70215684585707,
-2.68456422902658,-2.61732795283435,-2.5668973474104,-2.55375073916023,
-2.54526876573048,-2.53721964486301,-2.52591494163477,-2.49849966893336,
-2.41799983763994,-2.39816635687508,-2.38467993045638,-2.37875235869401,
-2.37426194619358,-2.36882306565325,-2.35835171448144,-2.30327850121938,
-2.25593923477587),.UNSPECIFIED.);
#2241=B_SPLINE_CURVE_WITH_KNOTS('',3,(#49555,#49556,#49557,#49558,#49559,
#49560,#49561,#49562,#49563,#49564,#49565,#49566,#49567,#49568,#49569,#49570,
#49571,#49572,#49573,#49574,#49575,#49576,#49577,#49578,#49579,#49580,#49581,
#49582,#49583,#49584,#49585,#49586,#49587,#49588,#49589,#49590,#49591,#49592,
#49593,#49594,#49595,#49596,#49597,#49598,#49599,#49600,#49601,#49602,#49603,
#49604,#49605,#49606,#49607,#49608,#49609,#49610,#49611,#49612,#49613,#49614,
#49615,#49616,#49617,#49618,#49619,#49620,#49621,#49622,#49623,#49624,#49625,
#49626,#49627,#49628,#49629,#49630,#49631,#49632,#49633,#49634,#49635,#49636,
#49637,#49638,#49639,#49640,#49641,#49642,#49643,#49644,#49645,#49646,#49647,
#49648,#49649,#49650,#49651,#49652,#49653,#49654,#49655,#49656,#49657,#49658,
#49659,#49660,#49661,#49662,#49663,#49664,#49665,#49666,#49667,#49668,#49669,
#49670,#49671,#49672,#49673,#49674,#49675,#49676,#49677,#49678,#49679,#49680,
#49681,#49682,#49683,#49684,#49685,#49686,#49687,#49688,#49689,#49690,#49691,
#49692,#49693,#49694,#49695,#49696,#49697,#49698,#49699,#49700,#49701,#49702,
#49703,#49704,#49705,#49706,#49707,#49708,#49709,#49710,#49711,#49712,#49713,
#49714,#49715,#49716,#49717,#49718,#49719,#49720,#49721,#49722,#49723,#49724,
#49725,#49726,#49727,#49728,#49729,#49730,#49731,#49732),.UNSPECIFIED.,
 .F.,.F.,(4,2,2,2,2,2,2,2,2,2,2,2,2,2,2,2,2,2,2,2,2,2,2,2,2,2,2,2,2,2,2,
2,2,2,2,2,2,2,2,2,2,2,2,2,2,2,2,2,2,2,2,2,2,2,2,2,2,2,2,2,2,2,2,2,2,2,2,
2,2,2,2,2,2,2,2,2,2,2,2,2,2,2,2,2,2,2,2,2,4),(-2.01502246037067,-1.98169731450777,
-1.90173558673302,-1.88534179650667,-1.87610017858487,-1.86815977443268,
-1.8583557727864,-1.83855078644552,-1.81170282860945,-1.76948827394314,
-1.71888939864403,-1.71026383110115,-1.70527244185678,-1.70066801345141,
-1.69389737184125,-1.67459033691109,-1.64056994241434,-1.56243214447281,
-1.54737291312349,-1.53849769038798,-1.53050669467853,-1.52013472071676,
-1.49704903882493,-1.46359242696767,-1.39754179029721,-1.37884478289928,
-1.37195955880564,-1.36737994953238,-1.36244468686577,-1.35408040494002,
-1.31268467923658,-1.22717780313807,-1.21155281906764,-1.20247550035619,
-1.19531609855523,-1.18567806575067,-1.16676364345449,-1.12027345163667,
-1.06242059062369,-1.04258023954654,-1.03554531205344,-1.0313521582367,
-1.02658668181786,-1.01900971328711,-0.991672189360913,-0.925070766363241,
-0.88479634268939,-0.872029014353895,-0.863624830605795,-0.85543617843434,
-0.843789291295884,-0.811533743398526,-0.752825065341529,-0.708952106137622,
-0.700450621704578,-0.695486224320385,-0.690869081385854,-0.684026076462995,
-0.66411747655555,-0.628328069107437,-0.553461921603732,-0.538014259570234,
-0.529060042405756,-0.521086336756685,-0.510860659524785,-0.488650609722859,
-0.457039276156101,-0.419706029191237,-0.376226435046764,-0.365509402071225,
-0.360088356969347,-0.355597561360689,-0.349649667012437,-0.336037089967,
-0.315937113439235,-0.231966595891586,-0.207458658425235,-0.197637940992484,
-0.189527377553755,-0.181147286875157,-0.168497956766223,-0.125752974196045,
-0.0645402929535018,-0.034851635230439,-0.026907861210298,-0.0220637319845611,
-0.0178656474137155,-0.0131614607899771,-0.000969412843418152),
 .UNSPECIFIED.);
#2242=B_SPLINE_CURVE_WITH_KNOTS('',3,(#49733,#49734,#49735,#49736,#49737,
#49738),.UNSPECIFIED.,.F.,.F.,(4,2,4),(-4.27034593055923,-4.20600833774116,
-4.14968971221015),.UNSPECIFIED.);
#2243=B_SPLINE_CURVE_WITH_KNOTS('',3,(#49739,#49740,#49741,#49742,#49743,
#49744,#49745,#49746,#49747,#49748,#49749,#49750,#49751,#49752,#49753,#49754,
#49755,#49756,#49757,#49758,#49759,#49760,#49761,#49762,#49763,#49764,#49765,
#49766,#49767,#49768,#49769,#49770,#49771,#49772,#49773,#49774,#49775,#49776,
#49777,#49778,#49779,#49780,#49781,#49782,#49783,#49784,#49785,#49786,#49787,
#49788,#49789,#49790,#49791,#49792,#49793,#49794,#49795,#49796,#49797,#49798,
#49799,#49800,#49801,#49802,#49803,#49804,#49805,#49806,#49807,#49808,#49809,
#49810,#49811,#49812,#49813,#49814,#49815,#49816,#49817,#49818,#49819,#49820,
#49821,#49822,#49823,#49824,#49825,#49826,#49827,#49828,#49829,#49830,#49831,
#49832,#49833,#49834,#49835,#49836,#49837,#49838,#49839,#49840,#49841,#49842,
#49843,#49844,#49845,#49846,#49847,#49848,#49849,#49850,#49851,#49852,#49853,
#49854,#49855,#49856,#49857,#49858,#49859,#49860,#49861,#49862,#49863,#49864,
#49865,#49866,#49867,#49868,#49869,#49870,#49871,#49872,#49873,#49874,#49875,
#49876,#49877,#49878,#49879,#49880,#49881,#49882,#49883,#49884,#49885,#49886,
#49887,#49888,#49889,#49890,#49891,#49892,#49893,#49894,#49895,#49896,#49897,
#49898,#49899,#49900,#49901,#49902,#49903,#49904,#49905,#49906,#49907,#49908,
#49909,#49910,#49911,#49912,#49913,#49914,#49915,#49916,#49917,#49918,#49919,
#49920,#49921,#49922,#49923,#49924,#49925,#49926,#49927,#49928,#49929,#49930),
 .UNSPECIFIED.,.F.,.F.,(4,2,2,2,2,2,2,2,2,2,2,2,2,2,2,2,2,2,2,2,2,2,2,2,
2,2,2,2,2,2,2,2,2,2,2,2,2,2,2,2,2,2,2,2,2,2,2,2,2,2,2,2,2,2,2,2,2,2,2,2,
2,2,2,2,2,2,2,2,2,2,2,2,2,2,2,2,2,2,2,2,2,2,2,2,2,2,2,2,2,2,2,2,2,2,2,4),
(-2.25593923477587,-2.2550800414557,-2.22605005401396,-2.21480174339244,
-2.20668152750578,-2.19816253331147,-2.18483473372666,-2.13516675811743,
-2.06929076115446,-2.05041220285426,-2.04350196827854,-2.03891736272286,
-2.03398959635608,-2.02566181201838,-1.98528561620682,-1.89800555339563,
-1.88256410357354,-1.87361036234211,-1.86563524958772,-1.85540522181267,
-1.83317465503591,-1.80152277322564,-1.76422626907087,-1.72075189506879,
-1.71003883794084,-1.70461811566501,-1.70012658756494,-1.69417641947781,
-1.68055333710693,-1.66043258711796,-1.57620231475946,-1.55188450553228,
-1.54209229075394,-1.53398790637176,-1.52559653843235,-1.51289470815902,
-1.46946940876894,-1.42971453814165,-1.38434994422378,-1.37353353023355,
-1.36809282923244,-1.36360363996874,-1.35768114283175,-1.34422045505091,
-1.32443675254983,-1.2445998529737,-1.21661712545391,-1.20522620707125,
-1.19716382796879,-1.18870956817852,-1.1756931807367,-1.12753268451687,
-1.06887401673824,-1.0423783162708,-1.03465305628698,-1.02985577760556,
-1.0251228962551,-1.01769861701944,-0.992161626551961,-0.935222833816181,
-0.884409072451034,-0.871050988798573,-0.862527190624263,-0.854412603354564,
-0.843188781145115,-0.814328499114182,-0.766611290749401,-0.71088080989809,
-0.700446240037341,-0.695015849579098,-0.690525947368874,-0.684590488731045,
-0.671051976519683,-0.651106350960472,-0.569203907306135,-0.542906860628762,
-0.531786573129396,-0.523689487113011,-0.515132634773628,-0.501611462487577,
-0.441578622240588,-0.376801212678062,-0.364645841538989,-0.358952947263029,
-0.354473714820259,-0.348837072030278,-0.336988373591138,-0.32041252621164,
-0.26853063150797,-0.211863930273245,-0.19824643768441,-0.189669715927705,
-0.181581929282899,-0.170519406312706,-0.142846285350935,-0.121312221259422),
 .UNSPECIFIED.);
#2244=B_SPLINE_CURVE_WITH_KNOTS('',3,(#49935,#49936,#49937,#49938,#49939,
#49940,#49941,#49942,#49943,#49944,#49945,#49946,#49947,#49948,#49949,#49950,
#49951,#49952,#49953,#49954,#49955,#49956,#49957,#49958,#49959,#49960,#49961,
#49962,#49963,#49964,#49965,#49966,#49967,#49968,#49969,#49970,#49971,#49972,
#49973,#49974,#49975,#49976,#49977,#49978,#49979,#49980,#49981,#49982,#49983,
#49984,#49985,#49986,#49987,#49988,#49989,#49990,#49991,#49992,#49993,#49994,
#49995,#49996,#49997,#49998,#49999,#50000,#50001,#50002,#50003,#50004,#50005,
#50006,#50007,#50008,#50009,#50010,#50011,#50012,#50013,#50014,#50015,#50016,
#50017,#50018,#50019,#50020,#50021,#50022,#50023,#50024,#50025,#50026,#50027,
#50028,#50029,#50030,#50031,#50032,#50033,#50034,#50035,#50036,#50037,#50038,
#50039,#50040,#50041,#50042,#50043,#50044,#50045,#50046,#50047,#50048,#50049,
#50050,#50051,#50052,#50053,#50054,#50055,#50056,#50057,#50058,#50059,#50060,
#50061,#50062,#50063,#50064,#50065,#50066,#50067,#50068,#50069,#50070,#50071,
#50072,#50073,#50074,#50075,#50076,#50077,#50078,#50079,#50080,#50081,#50082,
#50083,#50084,#50085,#50086,#50087,#50088,#50089,#50090,#50091,#50092,#50093,
#50094,#50095,#50096,#50097,#50098,#50099,#50100,#50101,#50102,#50103,#50104,
#50105,#50106,#50107,#50108,#50109,#50110,#50111,#50112,#50113,#50114,#50115,
#50116,#50117,#50118,#50119,#50120,#50121,#50122,#50123,#50124,#50125,#50126,
#50127,#50128,#50129,#50130),.UNSPECIFIED.,.F.,.F.,(4,2,2,2,2,2,2,2,2,2,
2,2,2,2,2,2,2,2,2,2,2,2,2,2,2,2,2,2,2,2,2,2,2,2,2,2,2,2,2,2,2,2,2,2,2,2,
2,2,2,2,2,2,2,2,2,2,2,2,2,2,2,2,2,2,2,2,2,2,2,2,2,2,2,2,2,2,2,2,2,2,2,2,
2,2,2,2,2,2,2,2,2,2,2,2,2,2,2,4),(-4.14991050821145,-4.10258403056536,-4.08280372408018,
-4.06934364215264,-4.06342116292215,-4.05893181733817,-4.05349079841364,
-4.04267327848696,-3.99729287255898,-3.95753145847438,-3.91406325561467,
-3.90135730538617,-3.89296497549934,-3.88486097738506,-3.87507089466387,
-3.85076662092273,-3.7665644894935,-3.74645229828964,-3.73283238898894,
-3.72688277390483,-3.72239124293459,-3.71697008987701,-3.70625487088741,
-3.6553904889722,-3.60542183439986,-3.5845761651439,-3.56812811842537,-3.55897012962597,
-3.55102326351955,-3.54110940847704,-3.52069606524622,-3.44531330018553,
-3.41554115104302,-3.40334758723133,-3.39392310798449,-3.38876305627559,
-3.38422271837605,-3.3778441766149,-3.36276784594267,-3.3009533336059,-3.25231306484021,
-3.23325322223389,-3.22358713789573,-3.2164245835296,-3.20736645766327,
-3.19183390654462,-3.11977135048715,-3.06533941999265,-3.05670486852015,
-3.05171144694938,-3.04716069726048,-3.04043765779841,-3.02289843783961,
-2.96312970168028,-2.95016545104569,-2.91969943144597,-2.89804824697386,
-2.88791634043941,-2.87995067691451,-2.87093722765783,-2.85561402224077,
-2.78129575563538,-2.74521932994297,-2.72521343008392,-2.71835811146044,
-2.713738011316,-2.70877648959731,-2.70029116682257,-2.65820686740767,-2.59807079980261,
-2.56542875111248,-2.55373527283697,-2.54553704070586,-2.53812492514167,
-2.52814193969286,-2.50224684150195,-2.41992891809295,-2.39995469690588,
-2.38640058933983,-2.38046166899047,-2.37597052381414,-2.37054040170487,
-2.36011074480476,-2.30414385396667,-2.25651314094471,-2.22768040864393,
-2.21645838219754,-2.20834273065099,-2.19981573612492,-2.18644811597091,
-2.13526330321036,-2.06339574347577,-2.0498034354368,-2.04392106431644,
-2.03942633111184,-2.034029665389,-2.02344052083963,-2.01502246037067),
 .UNSPECIFIED.);
#2245=B_SPLINE_CURVE_WITH_KNOTS('',3,(#50132,#50133,#50134,#50135,#50136,
#50137,#50138,#50139,#50140,#50141,#50142,#50143,#50144,#50145,#50146,#50147,
#50148,#50149),.UNSPECIFIED.,.F.,.F.,(4,2,2,2,2,2,2,2,4),(-0.121312221259422,
-0.0984195014592903,-0.0617965384739233,-0.0331257004132508,-0.0252540589033955,
-0.0204254706852453,-0.016234698007148,-0.0115182919411119,-0.000969387966873082),
 .UNSPECIFIED.);
#2246=B_SPLINE_CURVE_WITH_KNOTS('',3,(#50150,#50151,#50152,#50153,#50154,
#50155,#50156,#50157,#50158,#50159,#50160,#50161,#50162,#50163,#50164,#50165,
#50166,#50167,#50168,#50169,#50170,#50171,#50172,#50173,#50174,#50175,#50176,
#50177,#50178,#50179,#50180,#50181,#50182,#50183,#50184,#50185,#50186,#50187,
#50188,#50189,#50190,#50191,#50192,#50193,#50194,#50195,#50196,#50197,#50198,
#50199,#50200,#50201,#50202,#50203,#50204,#50205,#50206,#50207,#50208,#50209,
#50210,#50211,#50212,#50213,#50214,#50215,#50216,#50217,#50218,#50219,#50220,
#50221,#50222,#50223,#50224,#50225,#50226,#50227,#50228,#50229,#50230,#50231,
#50232,#50233,#50234,#50235,#50236,#50237,#50238,#50239,#50240,#50241,#50242,
#50243,#50244,#50245,#50246,#50247,#50248,#50249,#50250,#50251,#50252,#50253,
#50254,#50255,#50256,#50257,#50258,#50259,#50260,#50261,#50262,#50263,#50264,
#50265,#50266,#50267,#50268,#50269,#50270,#50271,#50272,#50273,#50274,#50275,
#50276,#50277,#50278,#50279,#50280,#50281,#50282,#50283,#50284,#50285,#50286,
#50287,#50288,#50289,#50290,#50291,#50292,#50293,#50294,#50295,#50296,#50297,
#50298,#50299,#50300,#50301,#50302,#50303,#50304,#50305,#50306,#50307,#50308,
#50309,#50310,#50311,#50312,#50313,#50314,#50315,#50316,#50317,#50318,#50319,
#50320,#50321,#50322,#50323),.UNSPECIFIED.,.F.,.F.,(4,2,2,2,2,2,2,2,2,2,
2,2,2,2,2,2,2,2,2,2,2,2,2,2,2,2,2,2,2,2,2,2,2,2,2,2,2,2,2,2,2,2,2,2,2,2,
2,2,2,2,2,2,2,2,2,2,2,2,2,2,2,2,2,2,2,2,2,2,2,2,2,2,2,2,2,2,2,2,2,2,2,2,
2,2,2,2,4),(-4.27179890156562,-4.23186784878015,-4.15611311581933,-4.13679228513219,
-4.12707638101779,-4.1199080341674,-4.11088313381104,-4.09551022507233,
-4.02165293833365,-3.98530180834149,-3.96520398302602,-3.95833718332906,
-3.95371451219657,-3.94875599018934,-3.94028658401118,-3.89907062209992,
-3.83824534133803,-3.80542158098759,-3.79370621401721,-3.7855031905106,
-3.77809361624191,-3.76622196597541,-3.73471554955944,-3.65895662485527,
-3.63952164967748,-3.6262280356811,-3.62033293713632,-3.61588548764024,
-3.61044090738187,-3.59960963313656,-3.55406154891125,-3.51395291467636,
-3.48515232452518,-3.46433494081551,-3.4543475771836,-3.4464661252529,-3.43738275109183,
-3.42173768346061,-3.35111860148115,-3.29562793963435,-3.28687623499795,
-3.28185720778926,-3.27731648857647,-3.27065589280916,-3.25355938436952,
-3.18579393001903,-3.13522756519233,-3.12207225016118,-3.1135876300787,
-3.10553806195894,-3.0942362276997,-3.06684610115723,-2.98629851768257,
-2.96645922108836,-2.9529693977907,-2.94704070025515,-2.94254959277758,
-2.9371100642068,-2.92663796449747,-2.87196021014954,-2.80132245417822,
-2.78673624097538,-2.77795728893227,-2.76993950532062,-2.75954708739381,
-2.73661473129622,-2.66422909172293,-2.62159778033585,-2.61319078998254,
-2.60824548722877,-2.60366940403785,-2.5968080752331,-2.57829534358584,
-2.51199366845522,-2.47847884305241,-2.45536562328426,-2.44498738862789,
-2.43699398049138,-2.42811852458821,-2.41306494152108,-2.33489345590886,
-2.30090909812101,-2.28161240347054,-2.27484210241728,-2.27023688857187,
-2.26524358446378,-2.25682980023252),.UNSPECIFIED.);
#2247=B_SPLINE_CURVE_WITH_KNOTS('',3,(#50329,#50330,#50331,#50332,#50333,
#50334,#50335,#50336,#50337,#50338,#50339,#50340,#50341,#50342,#50343,#50344,
#50345,#50346,#50347,#50348,#50349,#50350,#50351,#50352,#50353,#50354,#50355,
#50356,#50357,#50358,#50359,#50360,#50361,#50362,#50363,#50364,#50365,#50366,
#50367,#50368,#50369,#50370,#50371,#50372,#50373,#50374,#50375,#50376,#50377,
#50378,#50379,#50380,#50381,#50382,#50383,#50384,#50385,#50386,#50387,#50388,
#50389,#50390,#50391,#50392,#50393,#50394,#50395,#50396,#50397,#50398,#50399,
#50400,#50401,#50402,#50403,#50404,#50405,#50406,#50407,#50408,#50409,#50410,
#50411,#50412,#50413,#50414,#50415,#50416,#50417,#50418,#50419,#50420,#50421,
#50422,#50423,#50424,#50425,#50426,#50427,#50428,#50429,#50430,#50431,#50432,
#50433,#50434,#50435,#50436,#50437,#50438,#50439,#50440,#50441,#50442,#50443,
#50444,#50445,#50446,#50447,#50448,#50449,#50450,#50451,#50452,#50453,#50454,
#50455,#50456,#50457,#50458,#50459,#50460,#50461,#50462,#50463,#50464,#50465,
#50466,#50467,#50468,#50469,#50470,#50471,#50472,#50473,#50474,#50475,#50476,
#50477,#50478,#50479,#50480,#50481,#50482,#50483,#50484,#50485,#50486,#50487,
#50488,#50489,#50490,#50491,#50492,#50493,#50494,#50495,#50496,#50497,#50498,
#50499,#50500,#50501,#50502,#50503,#50504,#50505,#50506,#50507,#50508,#50509,
#50510,#50511,#50512),.UNSPECIFIED.,.F.,.F.,(4,2,2,2,2,2,2,2,2,2,2,2,2,
2,2,2,2,2,2,2,2,2,2,2,2,2,2,2,2,2,2,2,2,2,2,2,2,2,2,2,2,2,2,2,2,2,2,2,2,
2,2,2,2,2,2,2,2,2,2,2,2,2,2,2,2,2,2,2,2,2,2,2,2,2,2,2,2,2,2,2,2,2,2,2,2,
2,2,2,2,2,2,4),(-2.01495508295737,-2.00689615841809,-1.99095787635076,-1.98181283293574,
-1.97386417025694,-1.96393096995103,-1.94341156801903,-1.86802652050232,
-1.82456397519696,-1.81606312892168,-1.81109823935513,-1.8064799111471,
-1.79963410833907,-1.77970952549718,-1.74387700955012,-1.66905952164474,
-1.65378210197524,-1.64477849293584,-1.63681129693617,-1.62666343070455,
-1.60491862225422,-1.57426545218282,-1.55985073881598,-1.49702891170059,
-1.4831414982134,-1.4775576181753,-1.47302109882991,-1.46799539337194,-1.45920909748763,
-1.44808742164175,-1.42243265291249,-1.33878525297366,-1.31979995593782,
-1.31002880612164,-1.30209056293848,-1.29282388104751,-1.27583124811816,
-1.25405780599962,-1.19561454389183,-1.15137606520766,-1.14287218231421,
-1.13790698348621,-1.13328960556872,-1.12644697680209,-1.10654491983909,
-1.07077727665911,-0.995859699638924,-0.980415474630749,-0.971461436046849,
-0.963486827109749,-0.953258514592142,-0.931036323348952,-0.899401132689867,
-0.862088773811877,-0.818608594539454,-0.807895692988189,-0.802475156607295,
-0.797983845401291,-0.792034046590277,-0.778412144371624,-0.758293468483079,
-0.674082771065319,-0.649753962210217,-0.639960324206288,-0.631855859419937,
-0.623465525661463,-0.610767508812456,-0.567387632567234,-0.527601526817668,
-0.482223677970243,-0.47140670302522,-0.465966047675366,-0.46151995392572,
-0.455624168672415,-0.442319466311555,-0.422857163337568,-0.346804907095297,
-0.315556429021794,-0.303716815498926,-0.296314528806867,-0.288109423296191,
-0.276370796192306,-0.243314325268445,-0.181541391456794,-0.141617731666903,
-0.133188731148189,-0.128240014992132,-0.123614708489622,-0.116727004986083,
-0.0964384694353698,-0.0594955002376233,-0.000970997524927105),
 .UNSPECIFIED.);
#2248=B_SPLINE_CURVE_WITH_KNOTS('',3,(#50513,#50514,#50515,#50516,#50517,
#50518,#50519,#50520,#50521,#50522,#50523,#50524,#50525,#50526,#50527,#50528,
#50529,#50530),.UNSPECIFIED.,.F.,.F.,(4,2,2,2,2,2,2,2,4),(-4.27059030084637,
-4.25544757169058,-4.24361540156102,-4.23565536546824,-4.22810109817617,
-4.21962878643441,-4.20652603409915,-4.15987520303184,-4.14991050821145),
 .UNSPECIFIED.);
#2249=B_SPLINE_CURVE_WITH_KNOTS('',3,(#50531,#50532,#50533,#50534,#50535,
#50536,#50537,#50538,#50539,#50540,#50541,#50542,#50543,#50544,#50545,#50546,
#50547,#50548,#50549,#50550,#50551,#50552,#50553,#50554,#50555,#50556,#50557,
#50558,#50559,#50560,#50561,#50562,#50563,#50564,#50565,#50566,#50567,#50568,
#50569,#50570,#50571,#50572,#50573,#50574,#50575,#50576,#50577,#50578,#50579,
#50580,#50581,#50582,#50583,#50584,#50585,#50586,#50587,#50588,#50589,#50590,
#50591,#50592,#50593,#50594,#50595,#50596,#50597,#50598,#50599,#50600,#50601,
#50602,#50603,#50604,#50605,#50606,#50607,#50608,#50609,#50610,#50611,#50612,
#50613,#50614,#50615,#50616,#50617,#50618,#50619,#50620,#50621,#50622,#50623,
#50624,#50625,#50626,#50627,#50628,#50629,#50630,#50631,#50632,#50633,#50634,
#50635,#50636,#50637,#50638,#50639,#50640,#50641,#50642,#50643,#50644,#50645,
#50646,#50647,#50648,#50649,#50650,#50651,#50652,#50653,#50654,#50655,#50656,
#50657,#50658,#50659,#50660,#50661,#50662,#50663,#50664,#50665,#50666,#50667,
#50668,#50669,#50670,#50671,#50672,#50673,#50674,#50675,#50676,#50677,#50678,
#50679,#50680,#50681,#50682,#50683,#50684,#50685,#50686,#50687,#50688,#50689,
#50690,#50691,#50692,#50693,#50694,#50695,#50696,#50697,#50698,#50699,#50700,
#50701,#50702,#50703,#50704,#50705,#50706,#50707,#50708,#50709,#50710,#50711,
#50712,#50713,#50714,#50715,#50716,#50717,#50718),.UNSPECIFIED.,.F.,.F.,
(4,2,2,2,2,2,2,2,2,2,2,2,2,2,2,2,2,2,2,2,2,2,2,2,2,2,2,2,2,2,2,2,2,2,2,
2,2,2,2,2,2,2,2,2,2,2,2,2,2,2,2,2,2,2,2,2,2,2,2,2,2,2,2,2,2,2,2,2,2,2,2,
2,2,2,2,2,2,2,2,2,2,2,2,2,2,2,2,2,2,2,2,2,2,4),(-2.25682980023252,-2.25661250994356,
-2.20591257576506,-2.16281917118168,-2.13645165548217,-2.1169018521095,
-2.10714324506673,-2.09920344941743,-2.08992165103755,-2.07286138092067,
-2.05097351320595,-1.99189112121632,-1.94846836710502,-1.93996632939605,
-1.93500061792971,-1.93038141875548,-1.92353417342988,-1.90360425218822,
-1.86776004680764,-1.79293828114798,-1.7776571174334,-1.76865167205481,
-1.76068307377045,-1.75053372660918,-1.7287870318966,-1.69813247594623,
-1.6837292262318,-1.62093360426141,-1.60700311727575,-1.60141158179645,
-1.59687272734449,-1.5918497418494,-1.58307889778798,-1.52849127241406,
-1.4568114331574,-1.44123923617918,-1.43217172506076,-1.42500902950786,
-1.41535226570942,-1.39634664209088,-1.34840773421741,-1.28791964058421,
-1.27126858243578,-1.26468001100106,-1.26010659180953,-1.25504232594926,
-1.24607590567697,-1.23465494675142,-1.2078893145758,-1.11890400261765,
-1.10382968798458,-1.09495104026401,-1.08696025643398,-1.07659325769416,
-1.05354021592884,-1.0201545541671,-0.954535073066022,-0.935406972779673,
-0.928463685195102,-0.92387308407564,-0.918956447793143,-0.910679620498813,
-0.871583711698889,-0.78201784921328,-0.767075074254779,-0.758224156700196,
-0.750228098639219,-0.739810878433548,-0.716444905435652,-0.682381818962293,
-0.612588687674437,-0.597492388887194,-0.591112830477054,-0.586572586060987,
-0.581413763313979,-0.571993817454269,-0.517287834361057,-0.447099468186158,
-0.431428251344811,-0.422341143590254,-0.414463128361396,-0.404488982464491,
-0.383733974638334,-0.355054707383274,-0.314847093571687,-0.269304023175076,
-0.258475328608771,-0.253032386465008,-0.248586505264217,-0.242693697072303,
-0.229406404558046,-0.209979860025607,-0.134328372818447,-0.121726265633444),
 .UNSPECIFIED.);
#2250=B_SPLINE_CURVE_WITH_KNOTS('',3,(#50723,#50724,#50725,#50726,#50727,
#50728,#50729,#50730,#50731,#50732,#50733,#50734,#50735,#50736,#50737,#50738,
#50739,#50740,#50741,#50742,#50743,#50744,#50745,#50746,#50747,#50748,#50749,
#50750,#50751,#50752,#50753,#50754,#50755,#50756,#50757,#50758,#50759,#50760,
#50761,#50762,#50763,#50764,#50765,#50766,#50767,#50768,#50769,#50770,#50771,
#50772,#50773,#50774,#50775,#50776,#50777,#50778,#50779,#50780,#50781,#50782,
#50783,#50784,#50785,#50786,#50787,#50788,#50789,#50790,#50791,#50792,#50793,
#50794,#50795,#50796,#50797,#50798,#50799,#50800,#50801,#50802,#50803,#50804,
#50805,#50806,#50807,#50808,#50809,#50810,#50811,#50812,#50813,#50814,#50815,
#50816,#50817,#50818,#50819,#50820,#50821,#50822,#50823,#50824,#50825,#50826,
#50827,#50828,#50829,#50830,#50831,#50832,#50833,#50834,#50835,#50836,#50837,
#50838,#50839,#50840,#50841,#50842,#50843,#50844,#50845,#50846,#50847,#50848,
#50849,#50850,#50851,#50852,#50853,#50854,#50855,#50856,#50857,#50858,#50859,
#50860,#50861,#50862,#50863,#50864,#50865,#50866,#50867,#50868,#50869,#50870,
#50871,#50872,#50873,#50874,#50875,#50876,#50877,#50878,#50879,#50880,#50881,
#50882,#50883,#50884,#50885,#50886,#50887,#50888,#50889,#50890,#50891,#50892,
#50893,#50894,#50895,#50896,#50897,#50898,#50899,#50900,#50901,#50902,#50903,
#50904),.UNSPECIFIED.,.F.,.F.,(4,2,2,2,2,2,2,2,2,2,2,2,2,2,2,2,2,2,2,2,
2,2,2,2,2,2,2,2,2,2,2,2,2,2,2,2,2,2,2,2,2,2,2,2,2,2,2,2,2,2,2,2,2,2,2,2,
2,2,2,2,2,2,2,2,2,2,2,2,2,2,2,2,2,2,2,2,2,2,2,2,2,2,2,2,2,2,2,2,2,2,4),
(-4.14982650109305,-4.1082873562313,-4.03324515804132,-4.01292358148232,
-4.00302634855727,-3.99508089494166,-3.98591142787804,-3.96985567421038,
-3.91185516252669,-3.8648129285416,-3.84158169981968,-3.83437491440773,
-3.82968682075502,-3.82543092738862,-3.81805484803389,-3.7952317618859,
-3.73316273078659,-3.6840670492864,-3.67099515387706,-3.66252939411821,
-3.65447329869181,-3.64312071007598,-3.61538867767319,-3.53529391966009,
-3.51549518972057,-3.50202624071291,-3.49610228589735,-3.4916128655996,
-3.48617303864717,-3.47536149953984,-3.43006828533371,-3.39049394461776,
-3.34678119115582,-3.33405730208145,-3.32566143067199,-3.31756003629561,
-3.30778048711826,-3.28354377230916,-3.19925548416821,-3.1791371768581,
-3.16551436513755,-3.159564287869,-3.15507274944567,-3.14965200580156,-3.13893875631023,
-3.09548280903759,-3.05825154495698,-3.0265084516441,-3.00423550502694,
-2.99399831377212,-2.98602253535218,-2.9770731443316,-2.96165237912129,
-2.88657642140549,-2.83541038289319,-2.82633734706489,-2.82125087459975,
-2.81668653397386,-2.81015123254805,-2.7938288120438,-2.73302986116154,
-2.67510130030553,-2.6616381434093,-2.65309183599168,-2.64498669158846,
-2.63382611939545,-2.60719732470529,-2.52569662487933,-2.50578533783049,
-2.49226160437534,-2.48632789952198,-2.48183723769271,-2.4764034512305,
-2.46595582275543,-2.41036452589907,-2.36249942517703,-2.33358539067036,
-2.32235276123421,-2.31423548341687,-2.30571214072808,-2.29236169239625,
-2.24186162469394,-2.18468907522819,-2.15910380673045,-2.15167458095321,
-2.1469400423572,-2.1427233022465,-2.13555968771329,-2.11276153245501,-2.06736403238497,
-2.01495508295737),.UNSPECIFIED.);
#2251=B_SPLINE_CURVE_WITH_KNOTS('',3,(#50906,#50907,#50908,#50909,#50910,
#50911,#50912,#50913,#50914,#50915,#50916,#50917,#50918,#50919,#50920,#50921),
 .UNSPECIFIED.,.F.,.F.,(4,2,2,2,2,2,2,4),(-0.121726265633444,-0.102713804360095,
-0.0908325869755382,-0.0834232988331032,-0.0752256878954314,-0.0670488432893421,
-0.0557586804094333,-0.000969944449356401),.UNSPECIFIED.);
#2252=B_SPLINE_CURVE_WITH_KNOTS('',3,(#50922,#50923,#50924,#50925,#50926,
#50927,#50928,#50929,#50930,#50931,#50932,#50933,#50934,#50935,#50936,#50937,
#50938,#50939,#50940,#50941,#50942,#50943,#50944,#50945,#50946,#50947,#50948,
#50949,#50950,#50951,#50952,#50953,#50954,#50955,#50956,#50957,#50958,#50959,
#50960,#50961,#50962,#50963,#50964,#50965,#50966,#50967,#50968,#50969,#50970,
#50971,#50972,#50973,#50974,#50975,#50976,#50977,#50978,#50979,#50980,#50981,
#50982,#50983,#50984,#50985,#50986,#50987,#50988,#50989,#50990,#50991,#50992,
#50993,#50994,#50995,#50996,#50997,#50998,#50999,#51000,#51001,#51002,#51003,
#51004,#51005,#51006,#51007,#51008,#51009,#51010,#51011,#51012,#51013,#51014,
#51015,#51016,#51017,#51018,#51019,#51020,#51021,#51022,#51023,#51024,#51025,
#51026,#51027,#51028,#51029,#51030,#51031,#51032,#51033,#51034,#51035,#51036,
#51037,#51038,#51039,#51040,#51041,#51042,#51043,#51044,#51045,#51046,#51047,
#51048,#51049,#51050,#51051,#51052,#51053,#51054,#51055,#51056,#51057,#51058,
#51059,#51060,#51061,#51062,#51063,#51064,#51065,#51066,#51067,#51068,#51069,
#51070,#51071,#51072,#51073,#51074,#51075,#51076,#51077,#51078,#51079,#51080,
#51081,#51082,#51083,#51084,#51085,#51086,#51087,#51088,#51089,#51090,#51091,
#51092,#51093,#51094,#51095,#51096,#51097,#51098,#51099,#51100,#51101),
 .UNSPECIFIED.,.F.,.F.,(4,2,2,2,2,2,2,2,2,2,2,2,2,2,2,2,2,2,2,2,2,2,2,2,
2,2,2,2,2,2,2,2,2,2,2,2,2,2,2,2,2,2,2,2,2,2,2,2,2,2,2,2,2,2,2,2,2,2,2,2,
2,2,2,2,2,2,2,2,2,2,2,2,2,2,2,2,2,2,2,2,2,2,2,2,2,2,2,2,2,4),(-4.27066642005769,
-4.20450669432558,-4.19591865740787,-4.18871611366403,-4.18402833466105,
-4.17917337930773,-4.17118368822046,-4.14103271644137,-4.07807885739943,
-4.03719297500419,-4.02468825619013,-4.01633511798358,-4.00819979996669,
-3.99828582349113,-3.97314189738097,-3.88998252595607,-3.86994487373079,
-3.85636020284215,-3.85041604760643,-3.84592441665616,-3.84049796566513,
-3.82975788290823,-3.76345750597047,-3.72287200729123,-3.70492262509248,
-3.69023113630502,-3.68143124171302,-3.67342075096437,-3.66307499420352,
-3.63946209474127,-3.56748834589091,-3.53859744257702,-3.52662489882081,
-3.51733016194855,-3.51219688443914,-3.50764792098268,-3.50121313539205,
-3.48556689753791,-3.42418867343737,-3.36593649721675,-3.35246218155466,
-3.34391317329678,-3.33580849643624,-3.32465347500487,-3.29807095676384,
-3.21650779525402,-3.19659069829215,-3.18306388503558,-3.17712939848285,
-3.17263838888996,-3.1672044812344,-3.1564267122281,-3.11170137393137,-3.07330764627421,
-3.02799881035847,-3.01516017231304,-3.00674010509332,-2.99865238218313,
-2.9889344048032,-2.9648433797927,-2.88024096795973,-2.86009721401144,-2.8464613928347,
-2.84050837578946,-2.83601577966916,-2.8305951826985,-2.82021266003633,
-2.76333596297476,-2.7162634462516,-2.68762556427817,-2.67642881459227,
-2.66831679128014,-2.65978055953677,-2.64637047528827,-2.59326002313963,
-2.54532916737113,-2.52417745267427,-2.5100650394432,-2.50403322216664,
-2.4995340983232,-2.49416983757404,-2.48405465993704,-2.40844992956381,
-2.37316459242375,-2.3492430700218,-2.33873566156012,-2.33072732260278,
-2.32191928835796,-2.30718833518643,-2.25630608464035),.UNSPECIFIED.);
#2253=B_SPLINE_CURVE_WITH_KNOTS('',3,(#51107,#51108,#51109,#51110,#51111,
#51112,#51113,#51114,#51115,#51116,#51117,#51118,#51119,#51120,#51121,#51122,
#51123,#51124,#51125,#51126,#51127,#51128,#51129,#51130,#51131,#51132,#51133,
#51134,#51135,#51136,#51137,#51138,#51139,#51140,#51141,#51142,#51143,#51144,
#51145,#51146,#51147,#51148,#51149,#51150,#51151,#51152,#51153,#51154,#51155,
#51156,#51157,#51158,#51159,#51160,#51161,#51162,#51163,#51164,#51165,#51166,
#51167,#51168,#51169,#51170,#51171,#51172,#51173,#51174,#51175,#51176,#51177,
#51178,#51179,#51180,#51181,#51182,#51183,#51184,#51185,#51186,#51187,#51188,
#51189,#51190,#51191,#51192,#51193,#51194,#51195,#51196,#51197,#51198,#51199,
#51200,#51201,#51202,#51203,#51204,#51205,#51206,#51207,#51208,#51209,#51210,
#51211,#51212,#51213,#51214,#51215,#51216,#51217,#51218,#51219,#51220,#51221,
#51222,#51223,#51224,#51225,#51226,#51227,#51228,#51229,#51230,#51231,#51232,
#51233,#51234,#51235,#51236,#51237,#51238,#51239,#51240,#51241,#51242,#51243,
#51244,#51245,#51246,#51247,#51248,#51249,#51250,#51251,#51252,#51253,#51254,
#51255,#51256,#51257,#51258,#51259,#51260,#51261,#51262,#51263,#51264,#51265,
#51266,#51267,#51268,#51269,#51270,#51271,#51272,#51273,#51274,#51275,#51276,
#51277,#51278,#51279,#51280,#51281,#51282,#51283,#51284,#51285,#51286,#51287,
#51288),.UNSPECIFIED.,.F.,.F.,(4,2,2,2,2,2,2,2,2,2,2,2,2,2,2,2,2,2,2,2,
2,2,2,2,2,2,2,2,2,2,2,2,2,2,2,2,2,2,2,2,2,2,2,2,2,2,2,2,2,2,2,2,2,2,2,2,
2,2,2,2,2,2,2,2,2,2,2,2,2,2,2,2,2,2,2,2,2,2,2,2,2,2,2,2,2,2,2,2,2,2,4),
(-2.01540403112139,-1.97105136948028,-1.93084922841608,-1.92241046674066,
-1.91745917003503,-1.9128341508167,-1.90595073915008,-1.88570480379444,
-1.84889644755654,-1.77578561155131,-1.76033973643343,-1.75130038095629,
-1.74413573114024,-1.73444476642549,-1.71525033646811,-1.66580262697228,
-1.60216445243628,-1.58881545732867,-1.58297416056085,-1.57848324138124,
-1.5730565755451,-1.56231307435975,-1.51912676950302,-1.43715461635382,
-1.42262543062796,-1.41386001862441,-1.40584152515428,-1.39524857680718,
-1.37077473063976,-1.33424469865971,-1.27904499091919,-1.25572860599391,
-1.24830426835741,-1.2440392661089,-1.23936062382481,-1.23220011854312,
-1.20942644959956,-1.1641148584887,-1.10354597476904,-1.08761064848205,
-1.07846694715354,-1.07051924808615,-1.06058698533554,-1.04006848479775,
-0.964689634107515,-0.921238054893156,-0.91273830108402,-0.907774035032211,
-0.903156274572745,-0.896311295802245,-0.876388979019519,-0.84056029548628,
-0.765753154174027,-0.750477512485586,-0.741474994270852,-0.733508789374499,
-0.72336222092219,-0.701620342579102,-0.670971450466201,-0.656560122439426,
-0.593750375264972,-0.57986004552223,-0.574276096265196,-0.569739965685457,
-0.564715299207513,-0.555932048192157,-0.54481499123808,-0.519175302046611,
-0.435630653447615,-0.416578735157652,-0.406795202486274,-0.398857258392173,
-0.389602611106648,-0.37266689432786,-0.350990459195165,-0.293089836872497,
-0.248139868711028,-0.239633959232288,-0.234668716220123,-0.230052259616926,
-0.223212368372139,-0.203328586427172,-0.165047175600778,-0.0968343570779647,
-0.0807251782686702,-0.0707223989749149,-0.0627697428924434,-0.0552960986842517,
-0.0463378825376443,-0.0291380428848708,-0.000969509926115122),
 .UNSPECIFIED.);
#2254=B_SPLINE_CURVE_WITH_KNOTS('',3,(#51289,#51290,#51291,#51292,#51293,
#51294,#51295,#51296,#51297,#51298,#51299,#51300,#51301,#51302,#51303,#51304),
 .UNSPECIFIED.,.F.,.F.,(4,2,2,2,2,2,2,4),(-4.2700769044163,-4.19726735642565,
-4.17736906543256,-4.17052691070852,-4.16590950518612,-4.16094397358122,
-4.152438800623,-4.14982650109305),.UNSPECIFIED.);
#2255=B_SPLINE_CURVE_WITH_KNOTS('',3,(#51305,#51306,#51307,#51308,#51309,
#51310,#51311,#51312,#51313,#51314,#51315,#51316,#51317,#51318,#51319,#51320,
#51321,#51322,#51323,#51324,#51325,#51326,#51327,#51328,#51329,#51330,#51331,
#51332,#51333,#51334,#51335,#51336,#51337,#51338,#51339,#51340,#51341,#51342,
#51343,#51344,#51345,#51346,#51347,#51348,#51349,#51350,#51351,#51352,#51353,
#51354,#51355,#51356,#51357,#51358,#51359,#51360,#51361,#51362,#51363,#51364,
#51365,#51366,#51367,#51368,#51369,#51370,#51371,#51372,#51373,#51374,#51375,
#51376,#51377,#51378,#51379,#51380,#51381,#51382,#51383,#51384,#51385,#51386,
#51387,#51388,#51389,#51390,#51391,#51392,#51393,#51394,#51395,#51396,#51397,
#51398,#51399,#51400,#51401,#51402,#51403,#51404,#51405,#51406,#51407,#51408,
#51409,#51410,#51411,#51412,#51413,#51414,#51415,#51416,#51417,#51418,#51419,
#51420,#51421,#51422,#51423,#51424,#51425,#51426,#51427,#51428,#51429,#51430,
#51431,#51432,#51433,#51434,#51435,#51436,#51437,#51438,#51439,#51440,#51441,
#51442,#51443,#51444,#51445,#51446,#51447,#51448,#51449,#51450,#51451,#51452,
#51453,#51454,#51455,#51456,#51457,#51458,#51459,#51460,#51461,#51462,#51463,
#51464,#51465,#51466,#51467,#51468,#51469,#51470,#51471,#51472,#51473,#51474,
#51475,#51476,#51477,#51478,#51479,#51480,#51481,#51482,#51483,#51484,#51485,
#51486,#51487,#51488,#51489,#51490,#51491,#51492,#51493,#51494,#51495,#51496,
#51497,#51498),.UNSPECIFIED.,.F.,.F.,(4,2,2,2,2,2,2,2,2,2,2,2,2,2,2,2,2,
2,2,2,2,2,2,2,2,2,2,2,2,2,2,2,2,2,2,2,2,2,2,2,2,2,2,2,2,2,2,2,2,2,2,2,2,
2,2,2,2,2,2,2,2,2,2,2,2,2,2,2,2,2,2,2,2,2,2,2,2,2,2,2,2,2,2,2,2,2,2,2,2,
2,2,2,2,2,2,2,4),(-2.25630608464035,-2.22665608863465,-2.17869788383292,
-2.17015256186819,-2.16517794394682,-2.16061765643055,-2.15384198147782,
-2.13593876315631,-2.10493550210421,-2.02462227724864,-2.00849239269026,
-1.99930614997329,-1.99136068286754,-1.9814823195733,-1.96127100384044,
-1.88644182286149,-1.84194822390737,-1.83344169373867,-1.82847534548915,
-1.82385723388452,-1.81701399612784,-1.79711376566932,-1.76135599915273,
-1.68639514367998,-1.67095126243185,-1.66199622203288,-1.65402001705065,
-1.64378867863304,-1.62155565749395,-1.58990068614956,-1.55259751550503,
-1.5091164493172,-1.49840187926288,-1.49298040097717,-1.48848825145647,
-1.48253726694896,-1.4689123452172,-1.44878890771564,-1.36454833446142,
-1.34022610404596,-1.33043236932,-1.32232682201949,-1.3139343467314,-1.30123103488885,
-1.25780347391481,-1.21804023857895,-1.17266803485197,-1.16185003086918,
-1.15640855809648,-1.15196162368115,-1.14606450014982,-1.13275588923714,
-1.11328701361728,-1.03718725397823,-1.00596326367933,-0.994124996952157,
-0.985982358008743,-0.977639492242221,-0.965184913902923,-0.924882635268002,
-0.883119213883946,-0.836025355105792,-0.825252215367661,-0.819819678630679,
-0.815329273066339,-0.809394805584559,-0.795865237590222,-0.775939367664903,
-0.69431878705586,-0.667759389674627,-0.656608154368171,-0.648505092507639,
-0.639956788739636,-0.626481334627401,-0.568085212898543,-0.506426166795781,
-0.491199464899958,-0.484808698147212,-0.480266811200401,-0.475113532638111,
-0.465720282655782,-0.453578513085589,-0.424013595510056,-0.349463049411302,
-0.328263161010679,-0.318210567271455,-0.310253382564873,-0.301192145033339,
-0.285220312656599,-0.2320659815783,-0.171333807383222,-0.154989143431792,
-0.148450884418965,-0.143886597679154,-0.138802702872771,-0.129739418416578,
-0.121361672833077),.UNSPECIFIED.);
#2256=B_SPLINE_CURVE_WITH_KNOTS('',3,(#51503,#51504,#51505,#51506,#51507,
#51508,#51509,#51510,#51511,#51512,#51513,#51514,#51515,#51516,#51517,#51518,
#51519,#51520,#51521,#51522,#51523,#51524,#51525,#51526,#51527,#51528,#51529,
#51530,#51531,#51532,#51533,#51534,#51535,#51536,#51537,#51538,#51539,#51540,
#51541,#51542,#51543,#51544,#51545,#51546,#51547,#51548,#51549,#51550,#51551,
#51552,#51553,#51554,#51555,#51556,#51557,#51558,#51559,#51560,#51561,#51562,
#51563,#51564,#51565,#51566,#51567,#51568,#51569,#51570,#51571,#51572,#51573,
#51574,#51575,#51576,#51577,#51578,#51579,#51580,#51581,#51582,#51583,#51584,
#51585,#51586,#51587,#51588,#51589,#51590,#51591,#51592,#51593,#51594,#51595,
#51596,#51597,#51598,#51599,#51600,#51601,#51602,#51603,#51604,#51605,#51606,
#51607,#51608,#51609,#51610,#51611,#51612,#51613,#51614,#51615,#51616,#51617,
#51618,#51619,#51620,#51621,#51622,#51623,#51624,#51625,#51626,#51627,#51628,
#51629,#51630,#51631,#51632,#51633,#51634,#51635,#51636,#51637,#51638,#51639,
#51640,#51641,#51642,#51643,#51644,#51645,#51646,#51647,#51648,#51649,#51650,
#51651,#51652,#51653,#51654,#51655,#51656,#51657,#51658,#51659,#51660,#51661,
#51662,#51663,#51664,#51665,#51666,#51667,#51668,#51669,#51670,#51671,#51672,
#51673,#51674,#51675,#51676,#51677,#51678,#51679,#51680,#51681,#51682,#51683,
#51684,#51685,#51686,#51687,#51688,#51689,#51690,#51691,#51692,#51693,#51694,
#51695,#51696),.UNSPECIFIED.,.F.,.F.,(4,2,2,2,2,2,2,2,2,2,2,2,2,2,2,2,2,
2,2,2,2,2,2,2,2,2,2,2,2,2,2,2,2,2,2,2,2,2,2,2,2,2,2,2,2,2,2,2,2,2,2,2,2,
2,2,2,2,2,2,2,2,2,2,2,2,2,2,2,2,2,2,2,2,2,2,2,2,2,2,2,2,2,2,2,2,2,2,2,2,
2,2,2,2,2,2,2,4),(-4.15012799910223,-4.13770291279851,-4.11856720368116,
-4.10888734005964,-4.10172395829129,-4.09267707088321,-4.07719508535689,
-4.00456088298881,-3.95114469027171,-3.94221968518544,-3.93716465558241,
-3.93258862930004,-3.92702828456003,-3.91328258296434,-3.85029795249565,
-3.83580935355281,-3.80513828910692,-3.78338669329017,-3.77323805832315,
-3.76527133227511,-3.75626939157692,-3.74099753609209,-3.66620732335969,
-3.63040431130387,-3.61049001390752,-3.60364595454235,-3.5990282030219,
-3.59406334872494,-3.58556132032129,-3.54203293479802,-3.46664739859655,
-3.44613955153438,-3.43620893417147,-3.42826115932338,-3.41911585377816,
-3.40317359139517,-3.34475719783788,-3.29787751298955,-3.27468857687821,
-3.26748603690984,-3.26279880766999,-3.25854208311828,-3.25116161400311,
-3.22829489262859,-3.16626651847937,-3.11718164650289,-3.10411035642869,
-3.09564471523164,-3.08758854087377,-3.07623551312685,-3.04850065947577,
-2.96840940456376,-2.94861095795744,-2.93514214427853,-2.92921820920294,
-2.92472878803074,-2.91928894084348,-2.90847729856123,-2.86318255149109,
-2.8236048949081,-2.77989650195236,-2.76717293403115,-2.75877712798345,
-2.75067569051386,-2.74089595926649,-2.71665806699367,-2.6323712564819,
-2.61225305439068,-2.5986302936305,-2.59268022619285,-2.58818868980108,
-2.58276794214718,-2.57205466861945,-2.52859814615984,-2.49136559965593,
-2.45962361679968,-2.43735120527208,-2.42711410508525,-2.41913833749668,
-2.41018889650569,-2.39476788277872,-2.31969419661528,-2.28405052658235,
-2.26418949498752,-2.25735178411163,-2.25273518973789,-2.24776808371841,
-2.23925559963183,-2.19343197119745,-2.13612099482066,-2.10481335580357,
-2.09296559891226,-2.0855611059612,-2.07735587741152,-2.06562169077769,
-2.03261531170587,-2.01540403112139),.UNSPECIFIED.);
#2257=B_SPLINE_CURVE_WITH_KNOTS('',3,(#51698,#51699,#51700,#51701,#51702,
#51703,#51704,#51705),.UNSPECIFIED.,.F.,.F.,(4,2,2,4),(-0.121361672833077,
-0.0788430327264066,-0.0196534734691905,-0.000970778274795699),
 .UNSPECIFIED.);
#2258=B_SPLINE_CURVE_WITH_KNOTS('',3,(#51706,#51707,#51708,#51709,#51710,
#51711,#51712,#51713,#51714,#51715,#51716,#51717,#51718,#51719,#51720,#51721,
#51722,#51723,#51724,#51725,#51726,#51727,#51728,#51729,#51730,#51731,#51732,
#51733,#51734,#51735,#51736,#51737,#51738,#51739,#51740,#51741,#51742,#51743,
#51744,#51745,#51746,#51747,#51748,#51749,#51750,#51751,#51752,#51753,#51754,
#51755,#51756,#51757,#51758,#51759,#51760,#51761,#51762,#51763,#51764,#51765,
#51766,#51767,#51768,#51769,#51770,#51771,#51772,#51773,#51774,#51775,#51776,
#51777,#51778,#51779,#51780,#51781,#51782,#51783,#51784,#51785,#51786,#51787,
#51788,#51789,#51790,#51791,#51792,#51793,#51794,#51795,#51796,#51797,#51798,
#51799,#51800,#51801,#51802,#51803,#51804,#51805,#51806,#51807,#51808,#51809,
#51810,#51811,#51812,#51813,#51814,#51815,#51816,#51817,#51818,#51819,#51820,
#51821,#51822,#51823,#51824,#51825,#51826,#51827,#51828,#51829,#51830,#51831,
#51832,#51833,#51834,#51835,#51836,#51837,#51838,#51839,#51840,#51841,#51842,
#51843,#51844,#51845,#51846,#51847,#51848,#51849,#51850,#51851,#51852,#51853,
#51854,#51855,#51856,#51857,#51858,#51859,#51860,#51861,#51862,#51863,#51864,
#51865,#51866,#51867,#51868,#51869,#51870,#51871,#51872,#51873,#51874,#51875,
#51876,#51877,#51878,#51879,#51880,#51881,#51882,#51883,#51884,#51885,#51886,
#51887,#51888,#51889,#51890,#51891,#51892,#51893,#51894,#51895,#51896,#51897,
#51898,#51899,#51900,#51901,#51902,#51903,#51904),.UNSPECIFIED.,.F.,.F.,
(4,3,3,3,3,3,3,3,3,3,3,3,3,3,3,3,3,3,3,3,3,3,3,3,3,3,3,3,3,3,3,3,3,3,3,
3,3,3,3,3,3,3,3,3,3,3,3,3,3,3,3,3,3,3,3,3,3,3,3,3,3,3,3,3,3,3,4),(-16.4167960594917,
-16.3231866314518,-16.2295269004793,-16.1346626816796,-16.0407807339324,
-15.9454253796064,-15.8500700252804,-15.7580593289842,-15.6661696605864,
-15.5743745685169,-15.4826447769347,-15.3909489474259,-15.2992633110076,
-15.2075641131019,-15.1157697354889,-15.0239260397092,-14.93193240322,-14.8594406487004,
-14.7674298820707,-14.675540142735,-14.5837449792239,-14.4920151157411,
-14.4003192140759,-14.3086335053328,-14.2169342350209,-14.1251397853258,
-14.0332960175352,-13.9413023098999,-13.8688112721204,-13.7768007958635,
-13.684911347358,-13.5931164747535,-13.5013869011079,-13.4096912885271,
-13.3180058677772,-13.2263068840292,-13.1345127169216,-13.0426692299422,
-12.9506757972999,-12.8781818955404,-12.7861710642596,-12.6942812621272,
-12.6024860377262,-12.5107561164391,-12.4190601588747,-12.3273743961905,
-12.2356750739514,-12.1438805757485,-12.0520367612691,-11.9600430103993,
-11.8875525189603,-11.7955413114026,-11.7036511281309,-11.6118555182898,
-11.5201252067329,-11.4284288560818,-11.3367426979798,-11.2450429784762,
-11.1532480826281,-11.0614038696983,-10.9694097232057,-10.8969231423803,
-10.8060917963888,-10.7154014243328,-10.6247923810207,-10.5342434860829,
-10.4883011219526),.UNSPECIFIED.);
#2259=B_SPLINE_CURVE_WITH_KNOTS('',3,(#51910,#51911,#51912,#51913,#51914,
#51915,#51916,#51917,#51918,#51919,#51920,#51921,#51922,#51923,#51924,#51925,
#51926,#51927,#51928,#51929,#51930,#51931,#51932,#51933,#51934,#51935,#51936,
#51937,#51938,#51939,#51940,#51941,#51942,#51943,#51944,#51945,#51946,#51947,
#51948,#51949,#51950,#51951,#51952,#51953,#51954,#51955,#51956,#51957,#51958,
#51959,#51960,#51961,#51962,#51963,#51964,#51965,#51966,#51967,#51968,#51969,
#51970,#51971,#51972,#51973,#51974,#51975,#51976,#51977,#51978,#51979,#51980,
#51981,#51982,#51983,#51984,#51985,#51986,#51987,#51988,#51989,#51990,#51991,
#51992,#51993,#51994,#51995,#51996,#51997,#51998,#51999,#52000,#52001,#52002,
#52003,#52004,#52005,#52006,#52007,#52008,#52009,#52010,#52011,#52012,#52013,
#52014,#52015,#52016,#52017,#52018,#52019,#52020,#52021,#52022,#52023,#52024,
#52025,#52026,#52027,#52028,#52029,#52030,#52031,#52032,#52033,#52034,#52035,
#52036,#52037),.UNSPECIFIED.,.F.,.F.,(4,2,2,2,2,2,2,2,2,2,2,2,2,2,2,2,2,
2,2,2,2,2,2,2,2,2,2,2,2,2,2,2,2,2,2,2,2,2,2,2,2,2,2,2,2,2,2,2,2,2,2,2,2,
2,2,2,2,2,2,2,2,2,2,4),(0.00023418752938069,0.00315081488393006,0.00670998306291529,
0.0168928125761018,0.0617594987574512,0.107919044930031,0.13495437600853,
0.146551589240641,0.155447730774231,0.165349469766094,0.182321728836201,
0.274969220724888,0.320871474826383,0.329529544441537,0.334553533174522,
0.339048055301246,0.345518406077316,0.362224844207103,0.422266001158218,
0.460621487816279,0.485635852341467,0.496020108702134,0.503708340411375,
0.511934797877298,0.525115762712998,0.577959271430399,0.637362858857812,
0.654978060519609,0.667262186287639,0.672789027783616,0.677173957550166,
0.682613655152971,0.693105144563507,0.735404306501783,0.810846805884277,
0.830352008521856,0.840178129618988,0.847439558359909,0.856602561112202,
0.872293580606378,0.937032602343338,0.977054528538225,0.998291751472804,
1.0053775651737,1.01011380108815,1.01511794681386,1.02366902545801,1.06908163979997,
1.12631128277454,1.14786738106989,1.1647424587352,1.17401470273502,1.1819971517978,
1.19187506987937,1.21191738201843,1.30301994754333,1.32363958307489,1.33751112151411,
1.34351141290234,1.34800485063959,1.35337123845478,1.36388487750363,1.4202032623988,
1.42896198809384),.UNSPECIFIED.);
#2260=B_SPLINE_CURVE_WITH_KNOTS('',3,(#52040,#52041,#52042,#52043,#52044,
#52045,#52046,#52047,#52048,#52049,#52050,#52051,#52052,#52053,#52054,#52055,
#52056,#52057,#52058,#52059,#52060,#52061,#52062,#52063,#52064,#52065,#52066,
#52067,#52068,#52069,#52070,#52071,#52072,#52073,#52074,#52075,#52076,#52077,
#52078,#52079,#52080,#52081,#52082,#52083,#52084,#52085,#52086,#52087,#52088,
#52089,#52090,#52091,#52092,#52093,#52094,#52095,#52096,#52097,#52098,#52099,
#52100,#52101,#52102,#52103,#52104,#52105,#52106,#52107,#52108,#52109,#52110,
#52111,#52112,#52113,#52114,#52115,#52116,#52117,#52118,#52119,#52120,#52121,
#52122,#52123,#52124,#52125,#52126,#52127,#52128,#52129,#52130,#52131,#52132,
#52133,#52134,#52135,#52136,#52137,#52138,#52139,#52140,#52141,#52142,#52143,
#52144,#52145,#52146,#52147,#52148,#52149,#52150,#52151,#52152,#52153,#52154,
#52155,#52156,#52157,#52158,#52159,#52160,#52161,#52162,#52163,#52164,#52165,
#52166,#52167,#52168,#52169,#52170,#52171,#52172,#52173,#52174,#52175,#52176,
#52177,#52178,#52179,#52180,#52181,#52182,#52183,#52184,#52185,#52186,#52187,
#52188,#52189,#52190,#52191,#52192,#52193,#52194,#52195,#52196,#52197,#52198,
#52199,#52200,#52201,#52202,#52203,#52204,#52205,#52206,#52207,#52208,#52209,
#52210,#52211,#52212,#52213,#52214,#52215,#52216,#52217,#52218,#52219),
 .UNSPECIFIED.,.F.,.F.,(4,2,2,2,2,2,2,2,2,2,2,2,2,2,2,2,2,2,2,2,2,2,2,2,
2,2,2,2,2,2,2,2,2,2,2,2,2,2,2,2,2,2,2,2,2,2,2,2,2,2,2,2,2,2,2,2,2,2,2,2,
2,2,2,2,2,2,2,2,2,2,2,2,2,2,2,2,2,2,2,2,2,2,2,2,2,2,2,2,2,4),(-4.02402267163659,
-4.01660595258704,-3.95364176009931,-3.90430146731395,-3.88483392599072,
-3.87501536411647,-3.86775531655484,-3.85858850312061,-3.84287671102708,
-3.77920201461287,-3.73848912010533,-3.7170474773943,-3.70993954359626,
-3.705199173783,-3.7002031284654,-3.69168818039025,-3.65041139171089,-3.59001474375477,
-3.56790954289913,-3.55071788283664,-3.54138346606413,-3.5334060536903,
-3.52360876674235,-3.50832050943198,-3.41269493655136,-3.39182620271596,
-3.37783653980434,-3.3718171792667,-3.36736237564828,-3.36202916308435,
-3.35198712933449,-3.29045477172602,-3.24614198279102,-3.2185400092547,
-3.20752498482568,-3.19948208104683,-3.19096441943396,-3.17747171542151,
-3.11821642741899,-3.06778904700215,-3.05145196237189,-3.03973923673363,
-3.03415037267497,-3.02968538196736,-3.02398781229025,-3.0118123363106,
-2.94698203397978,-2.93186411164734,-2.88560078676851,-2.87268493316162,
-2.86423951203056,-2.85614471713959,-2.84643799289944,-2.82247190522749,
-2.73812598012657,-2.71801934401764,-2.70439812184665,-2.6984375285932,
-2.69393573458594,-2.68849957327305,-2.67805405001853,-2.62240817981378,
-2.5746329162323,-2.54575474923565,-2.53452556263767,-2.52640726863891,
-2.51890030133127,-2.50646958836968,-2.46934448982591,-2.39943761366767,
-2.37156973861686,-2.36395056390614,-2.35917606270683,-2.35499160524717,
-2.34799665369331,-2.3284502377363,-2.27032315783059,-2.21389269381728,
-2.20048802607827,-2.19195869010734,-2.18385593227559,-2.17267680296184,
-2.14588753507544,-2.06454709742011,-2.04464994359441,-2.03113510631806,
-2.02520618075471,-2.02071816153257,-2.01528587790108,-2.01517272200403),
 .UNSPECIFIED.);
#2261=B_SPLINE_CURVE_WITH_KNOTS('',3,(#52222,#52223,#52224,#52225,#52226,
#52227,#52228,#52229,#52230,#52231,#52232,#52233,#52234,#52235,#52236,#52237,
#52238,#52239,#52240,#52241,#52242,#52243,#52244,#52245,#52246,#52247,#52248,
#52249,#52250,#52251,#52252,#52253,#52254,#52255,#52256,#52257,#52258,#52259,
#52260,#52261,#52262,#52263,#52264,#52265,#52266,#52267,#52268,#52269,#52270,
#52271,#52272,#52273,#52274,#52275,#52276,#52277,#52278,#52279,#52280,#52281,
#52282,#52283,#52284,#52285,#52286,#52287,#52288,#52289,#52290,#52291,#52292,
#52293,#52294,#52295,#52296,#52297,#52298,#52299,#52300,#52301,#52302,#52303,
#52304,#52305,#52306,#52307,#52308,#52309,#52310,#52311,#52312,#52313,#52314,
#52315,#52316,#52317,#52318,#52319,#52320,#52321,#52322,#52323,#52324,#52325,
#52326,#52327,#52328,#52329,#52330,#52331,#52332,#52333,#52334,#52335,#52336,
#52337,#52338,#52339,#52340,#52341,#52342,#52343,#52344,#52345,#52346,#52347,
#52348,#52349,#52350,#52351,#52352,#52353,#52354,#52355,#52356,#52357,#52358,
#52359,#52360,#52361,#52362,#52363,#52364,#52365,#52366,#52367,#52368,#52369,
#52370,#52371,#52372,#52373,#52374,#52375,#52376,#52377,#52378,#52379,#52380,
#52381,#52382,#52383,#52384,#52385,#52386,#52387,#52388,#52389,#52390,#52391,
#52392,#52393,#52394,#52395,#52396,#52397),.UNSPECIFIED.,.F.,.F.,(4,2,2,
2,2,2,2,2,2,2,2,2,2,2,2,2,2,2,2,2,2,2,2,2,2,2,2,2,2,2,2,2,2,2,2,2,2,2,2,
2,2,2,2,2,2,2,2,2,2,2,2,2,2,2,2,2,2,2,2,2,2,2,2,2,2,2,2,2,2,2,2,2,2,2,2,
2,2,2,2,2,2,2,2,2,2,2,2,4),(-2.01517272200403,-2.00451421475811,-1.96106213155183,
-1.87951619754589,-1.86492309862471,-1.85614311422181,-1.84812622090925,
-1.83755726436441,-1.81324564606162,-1.77708203346033,-1.70369549294232,
-1.69307996863779,-1.68767734350376,-1.68318290544184,-1.67720460568732,
-1.66341335324765,-1.64293966426981,-1.55346008976567,-1.53259330238081,
-1.52259968181013,-1.5146479566336,-1.50554850677165,-1.48938602999012,
-1.4347071153928,-1.37072646907013,-1.35774588054285,-1.35196797134065,
-1.34748247238081,-1.34200777300546,-1.3310132088857,-1.31603793420628,
-1.27348537786853,-1.20912347912388,-1.19324792318433,-1.18411814316633,
-1.17617086320738,-1.16622377577733,-1.1456150627671,-1.11722019791397,
-1.05093302106982,-1.02531256885602,-1.01768284795244,-1.01290659752773,
-1.0081551939923,-1.00064276234197,-0.974082766992665,-0.911915808755105,
-0.86703122091171,-0.853922549591104,-0.845449779320622,-0.837306845451479,
-0.825915741171162,-0.79576116729459,-0.695354578463866,-0.683865194435322,
-0.678295195949978,-0.673813967315783,-0.668047991095213,-0.655488413935762,
-0.63752948906932,-0.575701553691541,-0.530441315366723,-0.51730861014069,
-0.508830588232313,-0.500689966397516,-0.489314451871821,-0.4592873642273,
-0.408092241917568,-0.357558247253426,-0.346880926698242,-0.341467588406309,
-0.336975847578333,-0.331017140459763,-0.317340732788108,-0.297107608098964,
-0.211268921629903,-0.187660629047367,-0.17731726515844,-0.169308914596127,
-0.160511666378622,-0.145825197766476,-0.127884076061152,-0.0873207091797893,
-0.0200345644038687,-0.0101360220370331,-0.00509855288362194,-0.00252798223428485,
-0.000974350499079791),.UNSPECIFIED.);
#2262=B_SPLINE_CURVE_WITH_KNOTS('',3,(#52398,#52399,#52400,#52401,#52402,
#52403,#52404,#52405,#52406,#52407,#52408,#52409),.UNSPECIFIED.,.F.,.F.,
(4,2,2,2,2,4),(-4.27068267614152,-4.26906071683224,-4.26567284309363,-4.25534850711771,
-4.18701167929227,-4.15012799910223),.UNSPECIFIED.);
#2263=B_SPLINE_CURVE_WITH_KNOTS('',3,(#52411,#52412,#52413,#52414,#52415,
#52416,#52417,#52418,#52419,#52420,#52421,#52422,#52423),.UNSPECIFIED.,
 .F.,.F.,(4,3,3,3,4),(-10.4883011219526,-10.3977630967638,-10.3072244319694,
-10.2166042167435,-10.133610752539),.UNSPECIFIED.);
#2264=B_SPLINE_CURVE_WITH_KNOTS('',3,(#52424,#52425,#52426,#52427,#52428,
#52429,#52430,#52431,#52432,#52433,#52434,#52435,#52436,#52437,#52438,#52439,
#52440,#52441,#52442,#52443,#52444,#52445,#52446,#52447,#52448,#52449,#52450,
#52451,#52452,#52453,#52454,#52455,#52456,#52457,#52458,#52459,#52460,#52461,
#52462,#52463,#52464,#52465,#52466,#52467,#52468,#52469,#52470,#52471,#52472,
#52473,#52474,#52475,#52476,#52477,#52478,#52479,#52480,#52481,#52482,#52483,
#52484,#52485,#52486,#52487,#52488,#52489,#52490,#52491,#52492,#52493,#52494,
#52495,#52496,#52497,#52498,#52499,#52500,#52501,#52502,#52503,#52504,#52505,
#52506,#52507,#52508,#52509,#52510,#52511,#52512,#52513,#52514,#52515,#52516,
#52517,#52518,#52519,#52520,#52521,#52522,#52523,#52524,#52525,#52526,#52527,
#52528,#52529,#52530,#52531,#52532,#52533,#52534,#52535,#52536,#52537,#52538,
#52539,#52540,#52541,#52542,#52543,#52544,#52545,#52546,#52547,#52548,#52549,
#52550,#52551,#52552,#52553,#52554,#52555,#52556,#52557,#52558,#52559,#52560,
#52561,#52562,#52563,#52564,#52565,#52566,#52567,#52568,#52569,#52570,#52571,
#52572,#52573,#52574,#52575,#52576,#52577,#52578,#52579,#52580,#52581,#52582,
#52583,#52584,#52585,#52586,#52587,#52588,#52589,#52590,#52591,#52592,#52593,
#52594,#52595,#52596,#52597,#52598,#52599,#52600,#52601),.UNSPECIFIED.,
 .F.,.F.,(4,2,2,2,2,2,2,2,2,2,2,2,2,2,2,2,2,2,2,2,2,2,2,2,2,2,2,2,2,2,2,
2,2,2,2,2,2,2,2,2,2,2,2,2,2,2,2,2,2,2,2,2,2,2,2,2,2,2,2,2,2,2,2,2,2,2,2,
2,2,2,2,2,2,2,2,2,2,2,2,2,2,2,2,2,2,2,2,2,4),(1.42896198809384,1.4676069046044,
1.49633027241518,1.50749827636214,1.5155673490849,1.5240365280871,1.53728877174833,
1.5856502766483,1.64518673674128,1.6712521509008,1.6786940485876,1.68341067942742,
1.68819090857537,1.69583141257155,1.72154466244348,1.78102387516357,1.82893164231001,
1.84221479084182,1.85073553946781,1.85887953677657,1.87019885072875,1.89969164795299,
1.94930827429658,2.00173039829016,2.0124269241899,2.01785490779613,2.02235727248275,
2.02833362993651,2.04209051972532,2.06248418843395,2.15077369753267,2.1724548842877,
2.18259358848788,2.19056211931748,2.19957632750544,2.21530288889363,2.26651687946367,
2.32322707232744,2.34464354272712,2.35186934148753,2.35609705492575,2.36081358114991,
2.36816706397028,2.39294998783131,2.44641636492676,2.50135512008876,2.51480899963436,
2.52334897391691,2.53144756370541,2.54259774884853,2.57093333455923,2.61716552701576,
2.67527627765604,2.68567969679657,2.69110154802672,2.69559135910075,2.70153415836735,
2.71511130517783,2.73513362263386,2.8180962147721,2.843405383942,2.85333937569815,
2.86148077414723,2.86982992057021,2.88230887593711,2.9228780881293,2.96449929249285,
3.01508129559219,3.02370613434759,3.02869859883741,3.03330426787174,3.04007886361942,
3.05941690492843,3.09352562777417,3.17153224569895,3.18654898104897,3.19541532466561,
3.20340816947816,3.21379660117432,3.23698277850097,3.27065804936337,3.32737136699031,
3.35346761275655,3.36114044099337,3.36592658200327,3.37066988522707,3.37814303984516,
3.38715189303689,3.44292570109838),.UNSPECIFIED.);
#2265=B_SPLINE_CURVE_WITH_KNOTS('',3,(#52604,#52605,#52606,#52607,#52608,
#52609,#52610,#52611,#52612,#52613,#52614,#52615,#52616,#52617,#52618,#52619,
#52620,#52621,#52622,#52623,#52624,#52625,#52626,#52627,#52628,#52629,#52630,
#52631,#52632,#52633,#52634,#52635,#52636,#52637,#52638,#52639,#52640,#52641,
#52642,#52643,#52644,#52645,#52646,#52647,#52648,#52649,#52650,#52651,#52652,
#52653,#52654,#52655,#52656,#52657,#52658,#52659,#52660,#52661,#52662,#52663,
#52664,#52665,#52666,#52667,#52668,#52669,#52670,#52671,#52672,#52673,#52674,
#52675,#52676,#52677,#52678,#52679,#52680,#52681,#52682,#52683,#52684,#52685,
#52686,#52687,#52688,#52689,#52690,#52691,#52692,#52693,#52694,#52695,#52696,
#52697,#52698,#52699,#52700,#52701,#52702,#52703,#52704,#52705,#52706,#52707,
#52708,#52709,#52710,#52711,#52712,#52713,#52714,#52715,#52716,#52717,#52718,
#52719,#52720,#52721,#52722,#52723,#52724,#52725,#52726,#52727,#52728,#52729,
#52730,#52731,#52732,#52733,#52734,#52735,#52736,#52737,#52738,#52739,#52740,
#52741,#52742,#52743,#52744,#52745,#52746,#52747,#52748),.UNSPECIFIED.,
 .F.,.F.,(4,3,3,3,3,3,3,3,3,3,3,3,3,3,3,3,3,3,3,3,3,3,3,3,3,3,3,3,3,3,3,
3,3,3,3,3,3,3,3,3,3,3,3,3,3,3,3,3,4),(17.9338728886362,18.0215470171645,
18.109145290346,18.1966963826855,18.2842238107557,18.3717482174281,18.4592902384062,
18.5469240273282,18.6346056657183,18.7224257637154,18.7919434588766,18.8797490912985,
18.9674437658401,19.0550504983712,19.1459907905069,19.233498614164,19.3209934256709,
19.4084958923916,19.4960266821179,19.5836543980516,19.6713396497812,19.7591505784758,
19.7825728354566,19.8703935858385,19.9581035608051,20.045725756466,20.1366603134123,
20.2241839074821,20.3116945756246,20.3992129681634,20.4867597358884,20.5744034271253,
20.6621046713552,20.7499314960658,20.7732022120367,20.8610213198291,20.9487296628209,
21.0363502391096,21.127285407798,21.2148074249428,21.3023165347146,21.3898333892518,
21.4773786411749,21.5650208574271,21.6527206487517,21.740546064198,21.7638315886167,
21.8810147460357,21.9911485751285),.UNSPECIFIED.);
#2266=B_SPLINE_CURVE_WITH_KNOTS('',3,(#52749,#52750,#52751,#52752,#52753,
#52754,#52755,#52756,#52757,#52758,#52759,#52760,#52761,#52762,#52763,#52764,
#52765,#52766,#52767,#52768,#52769,#52770,#52771,#52772,#52773,#52774,#52775,
#52776,#52777,#52778,#52779,#52780,#52781,#52782,#52783,#52784,#52785,#52786,
#52787,#52788,#52789,#52790,#52791,#52792,#52793,#52794,#52795,#52796,#52797,
#52798,#52799,#52800,#52801,#52802,#52803,#52804,#52805,#52806,#52807,#52808,
#52809,#52810,#52811,#52812,#52813,#52814,#52815,#52816,#52817,#52818,#52819,
#52820,#52821,#52822,#52823,#52824,#52825,#52826,#52827,#52828,#52829,#52830),
 .UNSPECIFIED.,.F.,.F.,(4,3,3,3,3,3,3,3,3,3,3,3,3,3,3,3,3,3,3,3,3,3,3,3,
3,3,3,4),(21.9911485753198,22.0776479350916,22.1640847934423,22.2504889236019,
22.3368820188365,22.4232857594527,22.5097743554891,22.5963065092834,22.6829750966663,
22.7544609651967,22.842279179636,22.9299866032483,23.0176062353834,23.1085417486826,
23.1960627655776,23.2835708560414,23.3710866732419,23.4586308708177,23.5462720126386,
23.6339707165569,23.7217950337417,23.7450903417767,23.8329109711975,23.9206243020769,
24.0082360027158,24.0957890755062,24.1833037493284,24.2166325387365),
 .UNSPECIFIED.);
#2267=B_SPLINE_CURVE_WITH_KNOTS('',3,(#52832,#52833,#52834,#52835,#52836,
#52837,#52838,#52839,#52840,#52841,#52842,#52843,#52844,#52845,#52846,#52847,
#52848,#52849,#52850,#52851,#52852,#52853,#52854,#52855,#52856,#52857,#52858,
#52859,#52860,#52861,#52862,#52863,#52864,#52865,#52866,#52867,#52868,#52869,
#52870,#52871,#52872,#52873,#52874,#52875,#52876,#52877,#52878,#52879,#52880,
#52881,#52882,#52883,#52884,#52885,#52886,#52887,#52888,#52889,#52890,#52891,
#52892,#52893,#52894,#52895,#52896,#52897,#52898,#52899,#52900,#52901,#52902,
#52903,#52904,#52905,#52906,#52907,#52908,#52909,#52910,#52911,#52912,#52913),
 .UNSPECIFIED.,.F.,.F.,(4,3,3,3,3,3,3,3,3,3,3,3,3,3,3,3,3,3,3,3,3,3,3,3,
3,3,3,4),(21.9911485753334,22.0925692444526,22.1945700829516,22.2972271432548,
22.3241606593577,22.4119814069087,22.4996913790177,22.5873135717981,22.6782481298156,
22.7657717209657,22.8532823861793,22.9408007757831,23.0283475405699,23.1159912288789,
23.2036924701836,23.2915192919947,23.3147900359378,23.4026144680511,23.4903268534229,
23.5810561989288,23.6686091896034,23.75612672866,23.8436294826255,23.9311381021069,
24.0187103272813,24.1063207651217,24.1940286371691,24.21616161747),
 .UNSPECIFIED.);
#2268=B_SPLINE_CURVE_WITH_KNOTS('',3,(#52914,#52915,#52916,#52917,#52918,
#52919,#52920,#52921,#52922,#52923,#52924,#52925,#52926,#52927,#52928,#52929,
#52930,#52931,#52932,#52933,#52934,#52935,#52936,#52937,#52938,#52939,#52940,
#52941,#52942,#52943,#52944,#52945,#52946,#52947,#52948,#52949,#52950,#52951,
#52952,#52953,#52954,#52955,#52956,#52957,#52958,#52959,#52960,#52961,#52962,
#52963,#52964,#52965,#52966,#52967,#52968,#52969,#52970,#52971,#52972,#52973,
#52974,#52975,#52976,#52977,#52978,#52979,#52980,#52981,#52982,#52983,#52984,
#52985,#52986,#52987,#52988,#52989,#52990,#52991,#52992,#52993,#52994,#52995,
#52996,#52997,#52998,#52999,#53000,#53001,#53002,#53003,#53004,#53005,#53006,
#53007,#53008,#53009,#53010,#53011,#53012,#53013,#53014,#53015,#53016,#53017,
#53018,#53019,#53020,#53021,#53022,#53023,#53024,#53025,#53026,#53027,#53028,
#53029,#53030,#53031,#53032,#53033,#53034,#53035,#53036,#53037,#53038,#53039,
#53040,#53041,#53042,#53043,#53044,#53045,#53046,#53047,#53048,#53049,#53050,
#53051,#53052,#53053,#53054,#53055,#53056,#53057,#53058,#53059,#53060,#53061),
 .UNSPECIFIED.,.F.,.F.,(4,3,3,3,3,3,3,3,3,3,3,3,3,3,3,3,3,3,3,3,3,3,3,3,
3,3,3,3,3,3,3,3,3,3,3,3,3,3,3,3,3,3,3,3,3,3,3,3,3,4),(17.9331385422654,
18.0208128771327,18.1085789253771,18.1963916734127,18.2843454815269,18.3616431530376,
18.449367930366,18.5369807394303,18.6245047002394,18.7154756789117,18.8028989874472,
18.8903087837302,18.9777258246176,19.0651708671648,19.152712785992,19.2403121091229,
19.3280375700532,19.3522725296177,19.4401067612013,19.5278302375573,19.6154659378553,
19.7063954338981,19.7939324510954,19.8814564882501,19.9689881806001,20.0565481637901,
20.1442048777122,20.2319190473871,20.3197585556779,20.3429019061977,20.4307340335604,
20.5184556443017,20.6060897189339,20.6970199144144,20.784555920573,20.8720791767411,
20.9596103201831,21.047169988739,21.1348267395123,21.2225411511409,21.3103812019963,
21.3335312827777,21.421325086341,21.5090102364101,21.5966075330255,21.6841377047948,
21.7716264493274,21.8590906176265,21.9465691639125,21.9911485751285),
 .UNSPECIFIED.);
#2269=B_SPLINE_CURVE_WITH_KNOTS('',3,(#53064,#53065,#53066,#53067,#53068,
#53069,#53070,#53071,#53072,#53073,#53074,#53075,#53076,#53077,#53078,#53079,
#53080,#53081,#53082,#53083,#53084,#53085,#53086,#53087,#53088,#53089,#53090,
#53091,#53092,#53093,#53094,#53095,#53096,#53097,#53098,#53099,#53100,#53101,
#53102,#53103,#53104,#53105,#53106,#53107,#53108,#53109,#53110,#53111,#53112,
#53113,#53114,#53115,#53116,#53117,#53118,#53119,#53120,#53121,#53122,#53123,
#53124,#53125,#53126,#53127,#53128,#53129,#53130,#53131,#53132,#53133,#53134,
#53135,#53136,#53137,#53138,#53139,#53140,#53141,#53142,#53143,#53144,#53145,
#53146,#53147,#53148,#53149,#53150,#53151,#53152,#53153,#53154,#53155,#53156,
#53157,#53158,#53159,#53160,#53161,#53162,#53163,#53164,#53165,#53166,#53167,
#53168,#53169,#53170,#53171,#53172,#53173,#53174,#53175,#53176,#53177,#53178,
#53179,#53180,#53181,#53182,#53183,#53184,#53185,#53186,#53187,#53188,#53189,
#53190,#53191,#53192,#53193,#53194,#53195,#53196,#53197,#53198,#53199,#53200,
#53201,#53202,#53203,#53204,#53205,#53206,#53207,#53208,#53209,#53210,#53211,
#53212,#53213,#53214,#53215,#53216,#53217,#53218,#53219,#53220,#53221,#53222,
#53223,#53224,#53225,#53226,#53227,#53228,#53229,#53230,#53231,#53232,#53233,
#53234,#53235,#53236,#53237,#53238,#53239,#53240,#53241),.UNSPECIFIED.,
 .F.,.F.,(4,2,2,2,2,2,2,2,2,2,2,2,2,2,2,2,2,2,2,2,2,2,2,2,2,2,2,2,2,2,2,
2,2,2,2,2,2,2,2,2,2,2,2,2,2,2,2,2,2,2,2,2,2,2,2,2,2,2,2,2,2,2,2,2,2,2,2,
2,2,2,2,2,2,2,2,2,2,2,2,2,2,2,2,2,2,2,2,2,4),(-2.01510602195132,-2.0044317114712,
-1.96086731396523,-1.87949599766812,-1.86487540474218,-1.85608815869749,
-1.84807038027914,-1.83750866339353,-1.81325484667234,-1.77722657183864,
-1.70350257554885,-1.69306672196303,-1.68763383237778,-1.68314108510995,
-1.6772000959313,-1.6636390055709,-1.64364926666656,-1.56120372012365,-1.53540663865066,
-1.52542898772208,-1.51801717690807,-1.50981563675015,-1.49810995219668,
-1.46536847004356,-1.40484166951035,-1.36333421682153,-1.3548606689335,
-1.34990125877571,-1.34527920866447,-1.33841487704988,-1.31833650282153,
-1.28203942000067,-1.20806208840535,-1.1926999558903,-1.18367771130796,
-1.17571266540575,-1.16559288782027,-1.14401382787951,-1.11369663955315,
-1.07539876741578,-1.03073039487558,-1.01995710283299,-1.01452415556432,
-1.01003293556814,-1.00409665429345,-0.99056026333586,-0.970620902600873,
-0.888820995130883,-0.862431544129402,-0.851298906545881,-0.843197568132834,
-0.834640384824886,-0.821127484121622,-0.761499315502669,-0.697519577552796,
-0.684544058961901,-0.67876561523136,-0.67427829789425,-0.668799256910654,
-0.65778942132117,-0.64278773401885,-0.600103559402819,-0.535928015486579,
-0.52004600642507,-0.510912491352526,-0.502961801435924,-0.493010086867018,
-0.472389476168545,-0.443974486443278,-0.37757160740112,-0.352080491709411,
-0.344459917436211,-0.339684332581721,-0.334928725731316,-0.327401144965952,
-0.300677559471162,-0.237623252380554,-0.193682918097719,-0.180635753336664,
-0.17217381440158,-0.164020425050653,-0.152579434675949,-0.122043130566837,
-0.0710903605481419,-0.021239433825702,-0.0106102094200809,-0.00529049879569223,
-0.00261560889277293,-0.000972523347507427),.UNSPECIFIED.);
#2270=B_SPLINE_CURVE_WITH_KNOTS('',3,(#53242,#53243,#53244,#53245,#53246,
#53247,#53248,#53249,#53250,#53251,#53252,#53253),.UNSPECIFIED.,.F.,.F.,
(4,2,2,2,2,4),(-4.2710288732429,-4.26942616966666,-4.26606147541147,-4.25584756501187,
-4.18561723202379,-4.15046929847984),.UNSPECIFIED.);
#2271=B_SPLINE_CURVE_WITH_KNOTS('',3,(#53255,#53256,#53257,#53258,#53259,
#53260,#53261,#53262,#53263,#53264,#53265,#53266,#53267),.UNSPECIFIED.,
 .F.,.F.,(4,3,3,3,4),(-10.4882942077004,-10.3977555936811,-10.3072163406073,
-10.2165955445259,-10.1336107524811),.UNSPECIFIED.);
#2272=B_SPLINE_CURVE_WITH_KNOTS('',3,(#53268,#53269,#53270,#53271,#53272,
#53273,#53274,#53275,#53276,#53277,#53278,#53279,#53280,#53281,#53282,#53283,
#53284,#53285,#53286,#53287,#53288,#53289,#53290,#53291,#53292,#53293,#53294,
#53295,#53296,#53297,#53298,#53299,#53300,#53301,#53302,#53303,#53304,#53305,
#53306,#53307,#53308,#53309,#53310,#53311,#53312,#53313,#53314,#53315,#53316,
#53317,#53318,#53319,#53320,#53321,#53322,#53323,#53324,#53325,#53326,#53327,
#53328,#53329,#53330,#53331,#53332,#53333,#53334,#53335,#53336,#53337,#53338,
#53339,#53340,#53341,#53342,#53343,#53344,#53345,#53346,#53347,#53348,#53349,
#53350,#53351,#53352,#53353,#53354,#53355,#53356,#53357,#53358,#53359,#53360,
#53361,#53362,#53363,#53364,#53365,#53366,#53367,#53368,#53369,#53370,#53371,
#53372,#53373,#53374,#53375,#53376,#53377,#53378,#53379,#53380,#53381,#53382,
#53383,#53384,#53385,#53386,#53387,#53388,#53389,#53390,#53391,#53392,#53393,
#53394,#53395,#53396,#53397,#53398,#53399,#53400,#53401,#53402,#53403,#53404,
#53405,#53406,#53407,#53408,#53409,#53410,#53411,#53412,#53413,#53414,#53415,
#53416,#53417,#53418,#53419,#53420,#53421,#53422,#53423,#53424,#53425,#53426,
#53427,#53428,#53429,#53430,#53431,#53432,#53433,#53434,#53435,#53436,#53437,
#53438,#53439,#53440,#53441,#53442,#53443),.UNSPECIFIED.,.F.,.F.,(4,2,2,
2,2,2,2,2,2,2,2,2,2,2,2,2,2,2,2,2,2,2,2,2,2,2,2,2,2,2,2,2,2,2,2,2,2,2,2,
2,2,2,2,2,2,2,2,2,2,2,2,2,2,2,2,2,2,2,2,2,2,2,2,2,2,2,2,2,2,2,2,2,2,2,2,
2,2,2,2,2,2,2,2,2,2,2,2,4),(1.42897696838616,1.46741399900062,1.4962817479625,
1.50747664149338,1.51555765934761,1.52403315896472,1.53728303602105,1.58537646119945,
1.64510865215483,1.67121576218021,1.67866660797506,1.68338860514827,1.68816973070354,
1.69581320288804,1.72155830573022,1.78120631517213,1.82889207245565,1.84216294039551,
1.85067949012597,1.85882195563953,1.87014297564165,1.89966061686505,1.94933774210726,
2.00176272089881,2.01246140564018,2.01788787305856,2.02238900944671,2.02836248149229,
2.04210041037211,2.06245363617006,2.15010509400306,2.17227445881266,2.18249818450072,
2.19047736960002,2.19944523199193,2.21493670413336,2.26438130308697,2.33884697895409,
2.34917345804516,2.35458322536127,2.35907669657421,2.365044492506,2.37877582324682,
2.39912186739911,2.48670846944777,2.50678412169201,2.51674076021563,2.52414497203279,
2.53234581491239,2.54406530112091,2.57695399226888,2.63803562873668,2.67894607028684,
2.68740441471095,2.69235881500317,2.69698225534397,2.70385339807908,2.72398463101445,
2.76043868950381,2.83408916429931,2.84948139257655,2.85851191435645,2.86568181947272,
2.87539621406065,2.89470112244532,2.97069396812108,3.01544306822901,3.02395342326548,
3.02892203382812,3.0335418016751,3.04038829051741,3.06030844694979,3.09612412908314,
3.17102746566376,3.18640753138475,3.19535063730725,3.20333113420022,3.21358891054149,
3.23597107785262,3.26793788023563,3.32626235462994,3.35340566644226,3.36119484109002,
3.36600727683016,3.37073089151171,3.37810455280796,3.3869574035366,3.44309910570526),
 .UNSPECIFIED.);
#2273=B_SPLINE_CURVE_WITH_KNOTS('',3,(#53446,#53447,#53448,#53449,#53450,
#53451,#53452,#53453,#53454,#53455,#53456,#53457,#53458,#53459,#53460,#53461,
#53462,#53463,#53464,#53465,#53466,#53467,#53468,#53469,#53470,#53471,#53472,
#53473,#53474,#53475,#53476,#53477,#53478,#53479,#53480,#53481,#53482,#53483,
#53484,#53485,#53486,#53487,#53488,#53489,#53490,#53491,#53492,#53493,#53494,
#53495,#53496,#53497,#53498,#53499,#53500,#53501,#53502,#53503,#53504,#53505,
#53506,#53507,#53508,#53509,#53510,#53511,#53512,#53513,#53514,#53515,#53516,
#53517,#53518,#53519,#53520,#53521,#53522,#53523,#53524,#53525,#53526,#53527,
#53528,#53529,#53530,#53531,#53532,#53533,#53534,#53535,#53536,#53537,#53538,
#53539,#53540,#53541,#53542,#53543,#53544,#53545,#53546,#53547,#53548,#53549,
#53550,#53551,#53552,#53553,#53554,#53555,#53556,#53557,#53558,#53559,#53560,
#53561,#53562,#53563,#53564,#53565,#53566,#53567,#53568,#53569,#53570,#53571,
#53572,#53573,#53574,#53575,#53576,#53577,#53578,#53579,#53580,#53581,#53582,
#53583,#53584,#53585,#53586,#53587,#53588,#53589,#53590),.UNSPECIFIED.,
 .F.,.F.,(4,3,3,3,3,3,3,3,3,3,3,3,3,3,3,3,3,3,3,3,3,3,3,3,3,3,3,3,3,3,3,
3,3,3,3,3,3,3,3,3,3,3,3,3,3,3,3,3,4),(17.9338702011125,18.0215425533029,
18.1091390113459,18.1966882365676,18.2842137661014,18.37173624473,18.4592763100473,
18.5469081112597,18.6345877412305,18.7224058161635,18.7919434588766,18.8797523806305,
18.9674503898695,19.0550604981952,19.1459995403529,19.2335108212493,19.3210091141967,
19.4085150829,19.4960493915041,19.5836806339246,19.6713694207407,19.7591838703614,
19.7825728354566,19.8703922597118,19.9581008960562,20.0457217423095,20.1366568010254,
20.2241790274407,20.3116883235665,20.3992053412126,20.4867507326539,20.574393052463,
20.6620929264883,20.749918393224,20.7732022120366,20.8610210912083,20.948729198936,
21.0363495336298,21.1272847905032,21.2148065516797,21.3023154005905,21.3898319896304,
21.4773769716732,21.565018912844,21.6527184257294,21.7405435598915,21.7638315886167,
21.8810158240277,21.9911485751285),.UNSPECIFIED.);
#2274=B_SPLINE_CURVE_WITH_KNOTS('',3,(#53591,#53592,#53593,#53594,#53595,
#53596,#53597,#53598,#53599,#53600,#53601,#53602,#53603,#53604,#53605,#53606,
#53607,#53608,#53609,#53610,#53611,#53612,#53613,#53614,#53615,#53616,#53617,
#53618,#53619,#53620,#53621,#53622,#53623,#53624,#53625,#53626,#53627,#53628,
#53629,#53630,#53631,#53632,#53633,#53634,#53635,#53636,#53637,#53638,#53639,
#53640,#53641,#53642,#53643,#53644,#53645,#53646,#53647,#53648,#53649,#53650,
#53651,#53652,#53653,#53654,#53655,#53656,#53657,#53658,#53659,#53660,#53661,
#53662,#53663,#53664,#53665,#53666,#53667,#53668,#53669,#53670,#53671,#53672),
 .UNSPECIFIED.,.F.,.F.,(4,3,3,3,3,3,3,3,3,3,3,3,3,3,3,3,3,3,3,3,3,3,3,3,
3,3,3,4),(21.991148575271,22.0776484880045,22.1640859049774,22.2504905972469,
22.3368842576987,22.4232885662622,22.5097777320238,22.5963104573412,22.6829796147006,
22.7544609651967,22.8422789538582,22.9299861494228,23.0176055515318,23.1085411503124,
23.1960619337185,23.2835697898192,23.3710853720355,23.4586293342593,23.5462702413632,
23.6339687106596,23.7217927951481,23.7450903417767,23.8329109525581,23.9206242639271,
24.0082359437503,24.0957889950546,24.183303645942,24.2166288630184),
 .UNSPECIFIED.);
#2275=B_SPLINE_CURVE_WITH_KNOTS('',3,(#53674,#53675,#53676,#53677,#53678,
#53679,#53680,#53681,#53682,#53683,#53684,#53685,#53686,#53687,#53688,#53689,
#53690,#53691,#53692,#53693,#53694,#53695,#53696,#53697,#53698,#53699,#53700,
#53701,#53702,#53703,#53704,#53705,#53706,#53707,#53708,#53709,#53710,#53711,
#53712,#53713,#53714,#53715,#53716,#53717,#53718,#53719,#53720,#53721,#53722,
#53723,#53724,#53725,#53726,#53727,#53728,#53729,#53730,#53731,#53732,#53733,
#53734,#53735,#53736,#53737,#53738,#53739,#53740,#53741,#53742,#53743,#53744,
#53745,#53746,#53747,#53748,#53749,#53750,#53751,#53752,#53753,#53754,#53755),
 .UNSPECIFIED.,.F.,.F.,(4,3,3,3,3,3,3,3,3,3,3,3,3,3,3,3,3,3,3,3,3,3,3,3,
3,3,3,4),(21.991148575328,22.0925750235656,22.1945818624572,22.297244987739,
22.3241606593577,22.4119800908502,22.4996887345,22.5873095881174,22.6782446440949,
22.7657668779734,22.8532761815859,22.940793206734,23.0283386056848,23.1159809329764,
23.2036808144772,23.2915062886212,23.3147900359377,23.4026142419743,23.4903263946006,
23.5810553110645,23.6686080538086,23.756125339587,23.8436278351851,23.931136191465,
24.0187081467531,24.1063183109976,24.1940259041244,24.2161577263113),
 .UNSPECIFIED.);
#2276=B_SPLINE_CURVE_WITH_KNOTS('',3,(#53756,#53757,#53758,#53759,#53760,
#53761,#53762,#53763,#53764,#53765,#53766,#53767,#53768,#53769,#53770,#53771,
#53772,#53773,#53774,#53775,#53776,#53777,#53778,#53779,#53780,#53781,#53782,
#53783,#53784,#53785,#53786,#53787,#53788,#53789,#53790,#53791,#53792,#53793,
#53794,#53795,#53796,#53797,#53798,#53799,#53800,#53801,#53802,#53803,#53804,
#53805,#53806,#53807,#53808,#53809,#53810,#53811,#53812,#53813,#53814,#53815,
#53816,#53817,#53818,#53819,#53820,#53821,#53822,#53823,#53824,#53825,#53826,
#53827,#53828,#53829,#53830,#53831,#53832,#53833,#53834,#53835,#53836,#53837,
#53838,#53839,#53840,#53841,#53842,#53843,#53844,#53845,#53846,#53847,#53848,
#53849,#53850,#53851,#53852,#53853,#53854,#53855,#53856,#53857,#53858,#53859,
#53860,#53861,#53862,#53863,#53864,#53865,#53866,#53867,#53868,#53869,#53870,
#53871,#53872,#53873,#53874,#53875,#53876,#53877,#53878,#53879,#53880,#53881,
#53882,#53883,#53884,#53885,#53886,#53887,#53888,#53889,#53890,#53891,#53892,
#53893,#53894,#53895,#53896,#53897,#53898,#53899,#53900,#53901,#53902,#53903),
 .UNSPECIFIED.,.F.,.F.,(4,3,3,3,3,3,3,3,3,3,3,3,3,3,3,3,3,3,3,3,3,3,3,3,
3,3,3,3,3,3,3,3,3,3,3,3,3,3,3,3,3,3,3,3,3,3,3,3,3,4),(17.9331346486732,
18.0208008418309,18.1085586009925,18.1963629732292,18.2843083139475,18.3616431530376,
18.449386361552,18.5370178462857,18.6245607041036,18.7155246822929,18.8029673258297,
18.8903965868309,18.9778332023575,19.0652979097325,19.1528595308134,19.2404786018306,
19.3282237282067,19.3522725296176,19.4400992041747,19.5278150523077,19.6154430629779,
19.7063754183804,19.7939046423309,19.8814208615799,19.9689447198792,20.0564968613797,
20.1441457617657,20.2318521252015,20.3196838973925,20.3429019061977,20.4307323340458,
20.5184522034034,20.6060844970501,20.6970153452661,20.7845494822013,20.8720708396058,
20.9596000566279,21.0471577729739,21.1348125427106,21.2225249541539,21.3103629916908,
21.3335312827777,21.4213282095817,21.5090165240303,21.5966170225215,21.6841504300686,
21.771642449676,21.8591099162917,21.9465917807573,21.9911485751285),
 .UNSPECIFIED.);
#2277=B_SPLINE_CURVE_WITH_KNOTS('',3,(#53906,#53907,#53908,#53909,#53910,
#53911,#53912,#53913,#53914,#53915,#53916,#53917,#53918,#53919,#53920,#53921,
#53922,#53923,#53924,#53925,#53926,#53927,#53928,#53929,#53930,#53931,#53932,
#53933,#53934,#53935,#53936,#53937,#53938,#53939,#53940,#53941,#53942,#53943,
#53944,#53945,#53946,#53947,#53948,#53949,#53950,#53951,#53952,#53953,#53954,
#53955,#53956,#53957,#53958,#53959,#53960,#53961,#53962,#53963,#53964,#53965,
#53966,#53967,#53968,#53969,#53970,#53971,#53972,#53973,#53974,#53975,#53976,
#53977,#53978,#53979,#53980,#53981,#53982,#53983,#53984,#53985,#53986,#53987,
#53988,#53989,#53990,#53991,#53992,#53993,#53994,#53995,#53996,#53997,#53998,
#53999,#54000,#54001,#54002,#54003,#54004,#54005,#54006,#54007,#54008,#54009,
#54010,#54011,#54012,#54013,#54014,#54015,#54016,#54017,#54018,#54019,#54020,
#54021,#54022,#54023,#54024,#54025,#54026,#54027,#54028,#54029,#54030,#54031,
#54032,#54033,#54034,#54035,#54036,#54037,#54038,#54039,#54040,#54041,#54042,
#54043,#54044,#54045,#54046,#54047,#54048,#54049,#54050,#54051,#54052,#54053,
#54054,#54055,#54056,#54057,#54058,#54059,#54060,#54061,#54062,#54063,#54064,
#54065,#54066,#54067,#54068,#54069,#54070,#54071,#54072,#54073,#54074,#54075,
#54076,#54077),.UNSPECIFIED.,.F.,.F.,(4,2,2,2,2,2,2,2,2,2,2,2,2,2,2,2,2,
2,2,2,2,2,2,2,2,2,2,2,2,2,2,2,2,2,2,2,2,2,2,2,2,2,2,2,2,2,2,2,2,2,2,2,2,
2,2,2,2,2,2,2,2,2,2,2,2,2,2,2,2,2,2,2,2,2,2,2,2,2,2,2,2,2,2,2,2,4),(-2.01551729291411,
-2.00485584560195,-1.9613915699149,-1.87982452303997,-1.86522737907853,
-1.85644500508538,-1.84842595738612,-1.83785420115296,-1.81353634332151,
-1.77736369470597,-1.70395574528014,-1.69333764465119,-1.68793362022894,
-1.68343796383025,-1.67745797292388,-1.6636625306281,-1.64318232872964,
-1.55366278916108,-1.53280190555801,-1.52280762463715,-1.51485391558332,
-1.50575061817829,-1.48957690053267,-1.43482754925375,-1.3707039488082,
-1.35908927001258,-1.35340586146658,-1.34884603156413,-1.34387258184106,
-1.33533020945826,-1.28751745267307,-1.20672559278948,-1.19202597681336,
-1.18322540000485,-1.17521692252114,-1.16469923606476,-1.14070480745836,
-1.10525773627288,-1.03012385305295,-1.01993357496737,-1.01455413556473,
-1.01005787674292,-1.00405044403608,-0.990084278654935,-0.969241387422245,
-0.873420503508213,-0.857034650446284,-0.847795136008765,-0.839855203327756,
-0.830050051574538,-0.810236190278846,-0.783370261830456,-0.741177824036141,
-0.69061076330626,-0.681987282930691,-0.676996515365108,-0.672392333456984,
-0.665621325643081,-0.646307595833169,-0.612265525127834,-0.534186499210383,
-0.51912275174109,-0.510247270411892,-0.502257491914246,-0.491889169034531,
-0.468821161619825,-0.435400792448215,-0.369554225159334,-0.350664203474423,
-0.343753450025736,-0.339169526250929,-0.334243640603721,-0.325921163238598,
-0.285642987253449,-0.198226315501195,-0.182821766418207,-0.173876946954676,
-0.165902457938223,-0.155663032031858,-0.133367585790185,-0.101577600200077,
-0.0380060262036244,-0.0150834299228487,-0.00785356191111222,-0.00370416980883594,
-0.000974342611802808),.UNSPECIFIED.);
#2278=B_SPLINE_CURVE_WITH_KNOTS('',3,(#54078,#54079,#54080,#54081,#54082,
#54083,#54084,#54085,#54086,#54087,#54088,#54089),.UNSPECIFIED.,.F.,.F.,
(4,2,2,2,2,4),(-4.27068267975062,-4.26906145758045,-4.26567463808812,-4.25535529738831,
-4.18692414937688,-4.15012784700328),.UNSPECIFIED.);
#2279=B_SPLINE_CURVE_WITH_KNOTS('',3,(#54091,#54092,#54093,#54094,#54095,
#54096,#54097,#54098,#54099,#54100,#54101,#54102,#54103),.UNSPECIFIED.,
 .F.,.F.,(4,3,3,3,4),(-10.4883010731468,-10.397763044796,-10.3072243768395,
-10.216604158493,-10.1336107525393),.UNSPECIFIED.);
#2280=B_SPLINE_CURVE_WITH_KNOTS('',3,(#54104,#54105,#54106,#54107,#54108,
#54109,#54110,#54111,#54112,#54113,#54114,#54115,#54116,#54117,#54118,#54119,
#54120,#54121,#54122,#54123,#54124,#54125,#54126,#54127,#54128,#54129,#54130,
#54131,#54132,#54133,#54134,#54135,#54136,#54137,#54138,#54139,#54140,#54141,
#54142,#54143,#54144,#54145,#54146,#54147,#54148,#54149,#54150,#54151,#54152,
#54153,#54154,#54155,#54156,#54157,#54158,#54159,#54160,#54161,#54162,#54163,
#54164,#54165,#54166,#54167,#54168,#54169,#54170,#54171,#54172,#54173,#54174,
#54175,#54176,#54177,#54178,#54179,#54180,#54181,#54182,#54183,#54184,#54185,
#54186,#54187,#54188,#54189,#54190,#54191,#54192,#54193,#54194,#54195,#54196,
#54197,#54198,#54199,#54200,#54201,#54202,#54203,#54204,#54205,#54206,#54207,
#54208,#54209,#54210,#54211,#54212,#54213,#54214,#54215,#54216,#54217,#54218,
#54219,#54220,#54221,#54222,#54223,#54224,#54225,#54226,#54227,#54228,#54229,
#54230,#54231,#54232,#54233,#54234,#54235,#54236,#54237,#54238,#54239,#54240,
#54241,#54242,#54243,#54244,#54245,#54246,#54247,#54248,#54249,#54250,#54251,
#54252,#54253,#54254,#54255,#54256,#54257,#54258,#54259,#54260,#54261,#54262,
#54263,#54264,#54265,#54266,#54267,#54268,#54269,#54270,#54271,#54272,#54273,
#54274,#54275,#54276,#54277,#54278,#54279,#54280,#54281),.UNSPECIFIED.,
 .F.,.F.,(4,2,2,2,2,2,2,2,2,2,2,2,2,2,2,2,2,2,2,2,2,2,2,2,2,2,2,2,2,2,2,
2,2,2,2,2,2,2,2,2,2,2,2,2,2,2,2,2,2,2,2,2,2,2,2,2,2,2,2,2,2,2,2,2,2,2,2,
2,2,2,2,2,2,2,2,2,2,2,2,2,2,2,2,2,2,2,2,2,4),(1.42896226070502,1.46760630807409,
1.49633027514612,1.50749839411284,1.51556752003582,1.52403673018617,1.53728897428289,
1.5856494956979,1.64518666713393,1.67125223828278,1.67869417368618,1.68341082794888,
1.68819106050374,1.69583157802488,1.72154498345669,1.78102501648932,1.82893172626393,
1.84221481544433,1.85073554231687,1.85887952965337,1.87019884611771,1.89969173097079,
1.94930855097605,2.00173087151417,2.01242740034867,2.01785537427144,2.02235773171005,
2.02833407399051,2.04209087049889,2.0624843409397,2.15077067139438,2.17245429937023,
2.18259343056372,2.19056201115673,2.19957597506071,2.21530130486682,2.26650589711478,
2.32319739803509,2.34463814477,2.3518667079049,2.35609493908851,2.36081086712881,
2.36816144281155,2.39291279821649,2.44623889947685,2.50134065548667,2.51480195401738,
2.52334346069836,2.53144130861827,2.54258691783137,2.57088859138895,2.61702655972888,
2.67526013133429,2.68567373581047,2.69109771876124,2.69558732092313,2.70152728280376,
2.71508756196999,2.73507475771854,2.81756899567094,2.84329917656217,2.85327126333096,
2.86068193557275,2.86888518304589,2.8805991291241,2.91341048992409,2.97421532664369,
3.01538147111956,3.023848666603,3.02880742911736,3.03343054553154,3.0403003236911,
3.06042763051094,3.09687264547184,3.17066339032726,3.18597708686976,3.19498813737077,
3.20295360792355,3.21308789873877,3.23475506836586,3.26525360577859,3.32507674682859,
3.35312000980341,3.36097522902233,3.36580074958091,3.37051004368903,3.37782039401938,
3.38657571455232,3.44294074553524),.UNSPECIFIED.);
#2281=B_SPLINE_CURVE_WITH_KNOTS('',3,(#54284,#54285,#54286,#54287,#54288,
#54289,#54290,#54291,#54292,#54293,#54294,#54295,#54296,#54297,#54298,#54299,
#54300,#54301,#54302,#54303,#54304,#54305,#54306,#54307,#54308,#54309,#54310,
#54311,#54312,#54313,#54314,#54315,#54316,#54317,#54318,#54319,#54320,#54321,
#54322,#54323,#54324,#54325,#54326,#54327,#54328,#54329,#54330,#54331,#54332,
#54333,#54334,#54335,#54336,#54337,#54338,#54339,#54340,#54341,#54342,#54343,
#54344,#54345,#54346,#54347,#54348,#54349,#54350,#54351,#54352,#54353,#54354,
#54355,#54356,#54357,#54358,#54359,#54360,#54361,#54362,#54363,#54364,#54365,
#54366,#54367,#54368,#54369,#54370,#54371,#54372,#54373,#54374,#54375,#54376,
#54377,#54378,#54379,#54380,#54381,#54382,#54383,#54384,#54385,#54386,#54387,
#54388,#54389,#54390,#54391,#54392,#54393,#54394,#54395,#54396,#54397,#54398,
#54399,#54400,#54401,#54402,#54403,#54404,#54405,#54406,#54407,#54408,#54409,
#54410,#54411,#54412,#54413,#54414,#54415,#54416,#54417,#54418,#54419,#54420,
#54421,#54422,#54423,#54424,#54425,#54426,#54427,#54428),.UNSPECIFIED.,
 .F.,.F.,(4,3,3,3,3,3,3,3,3,3,3,3,3,3,3,3,3,3,3,3,3,3,3,3,3,3,3,3,3,3,3,
3,3,3,3,3,3,3,3,3,3,3,3,3,3,3,3,3,4),(17.9338728552279,18.0215469755457,
18.1091452403261,18.1966963240079,18.2842237432648,18.3717481409769,18.4592901528567,
18.5469239325214,18.6346055615492,18.7224256501151,18.7919434588766,18.8797491078548,
18.9674437991789,19.0550505486975,19.1459908345424,19.2334986755925,19.3209935046125,
19.4084959889484,19.4960267963733,19.583654530042,19.6713397995486,19.7591507459476,
19.7825728354566,19.870393578819,19.9581035467,20.0457257352183,20.1366602948206,
20.2241838816509,20.3116945425309,20.3992129277918,20.4867596882313,20.5744033722082,
20.6621046091846,20.749931426706,20.7732022120367,20.8610213187728,20.9487296606754,
21.0363502358434,21.1272854049401,21.2148074208924,21.302316529447,21.3898333827436,
21.4773786334039,21.5650208483663,21.6527206383839,21.7405460525077,21.7638315886167,
21.8810147511443,21.9911485751285),.UNSPECIFIED.);
#2282=B_SPLINE_CURVE_WITH_KNOTS('',3,(#54429,#54430,#54431,#54432,#54433,
#54434,#54435,#54436,#54437,#54438,#54439,#54440,#54441,#54442,#54443,#54444,
#54445,#54446,#54447,#54448,#54449,#54450,#54451,#54452,#54453,#54454,#54455,
#54456,#54457,#54458,#54459,#54460,#54461,#54462,#54463,#54464,#54465,#54466,
#54467,#54468,#54469,#54470,#54471,#54472,#54473,#54474,#54475,#54476,#54477,
#54478,#54479,#54480,#54481,#54482,#54483,#54484,#54485,#54486,#54487,#54488,
#54489,#54490,#54491,#54492,#54493,#54494,#54495,#54496,#54497,#54498,#54499,
#54500,#54501,#54502,#54503,#54504,#54505,#54506,#54507,#54508,#54509,#54510),
 .UNSPECIFIED.,.F.,.F.,(4,3,3,3,3,3,3,3,3,3,3,3,3,3,3,3,3,3,3,3,3,3,3,3,
3,3,3,4),(21.9911485753201,22.0776479380628,22.1640847994147,22.2504889325943,
22.3368820308656,22.4232857745334,22.5097743736308,22.5963065304959,22.6829751209414,
22.7544609651967,22.842279178373,22.9299866007098,23.0176062315584,23.1085417453356,
23.1960627609244,23.283570850077,23.3710866659631,23.4586308622222,23.5462720027297,
23.6339707053352,23.721795021218,23.7450903417767,23.8329109711241,23.9206243019256,
24.0082360024787,24.0957890751796,24.1833037489021,24.2166325011217),
 .UNSPECIFIED.);
#2283=B_SPLINE_CURVE_WITH_KNOTS('',3,(#54512,#54513,#54514,#54515,#54516,
#54517,#54518,#54519,#54520,#54521,#54522,#54523,#54524,#54525,#54526,#54527,
#54528,#54529,#54530,#54531,#54532,#54533,#54534,#54535,#54536,#54537,#54538,
#54539,#54540,#54541,#54542,#54543,#54544,#54545,#54546,#54547,#54548,#54549,
#54550,#54551,#54552,#54553,#54554,#54555,#54556,#54557,#54558,#54559,#54560,
#54561,#54562,#54563,#54564,#54565,#54566,#54567,#54568,#54569,#54570,#54571,
#54572,#54573,#54574,#54575,#54576,#54577,#54578,#54579,#54580,#54581,#54582,
#54583,#54584,#54585,#54586,#54587,#54588,#54589,#54590,#54591,#54592,#54593),
 .UNSPECIFIED.,.F.,.F.,(4,3,3,3,3,3,3,3,3,3,3,3,3,3,3,3,3,3,3,3,3,3,3,3,
3,3,3,4),(21.9911485753333,22.0925692721343,22.1945701393998,22.2972272288129,
22.3241606593577,22.4119814005141,22.4996913661684,22.587313552442,22.678248112879,
22.7657716974341,22.8532823560317,22.9408007390053,23.0283474971554,23.1159911788507,
23.2036924135476,23.2915192288096,23.3147900359378,23.4026144670927,23.4903268514756,
23.5810561923767,23.6686091819928,23.7561267199653,23.8436294728221,23.9311380911715,
24.0187103151771,24.1063207518307,24.1940286226559,24.2161615786844),
 .UNSPECIFIED.);
#2284=B_SPLINE_CURVE_WITH_KNOTS('',3,(#54594,#54595,#54596,#54597,#54598,
#54599,#54600,#54601,#54602,#54603,#54604,#54605,#54606,#54607,#54608,#54609,
#54610,#54611,#54612,#54613,#54614,#54615,#54616,#54617,#54618,#54619,#54620,
#54621,#54622,#54623,#54624,#54625,#54626,#54627,#54628,#54629,#54630,#54631,
#54632,#54633,#54634,#54635,#54636,#54637,#54638,#54639,#54640,#54641,#54642,
#54643,#54644,#54645,#54646,#54647,#54648,#54649,#54650,#54651,#54652,#54653,
#54654,#54655,#54656,#54657,#54658,#54659,#54660,#54661,#54662,#54663,#54664,
#54665,#54666,#54667,#54668,#54669,#54670,#54671,#54672,#54673,#54674,#54675,
#54676,#54677,#54678,#54679,#54680,#54681,#54682,#54683,#54684,#54685,#54686,
#54687,#54688,#54689,#54690,#54691,#54692,#54693,#54694,#54695,#54696,#54697,
#54698,#54699,#54700,#54701,#54702,#54703,#54704,#54705,#54706,#54707,#54708,
#54709,#54710,#54711,#54712,#54713,#54714,#54715,#54716,#54717,#54718,#54719,
#54720,#54721,#54722,#54723,#54724,#54725,#54726,#54727,#54728,#54729,#54730,
#54731,#54732,#54733,#54734,#54735,#54736,#54737,#54738,#54739,#54740,#54741),
 .UNSPECIFIED.,.F.,.F.,(4,3,3,3,3,3,3,3,3,3,3,3,3,3,3,3,3,3,3,3,3,3,3,3,
3,3,3,3,3,3,3,3,3,3,3,3,3,3,3,3,3,3,3,3,3,3,3,3,3,4),(17.933138501431,18.0208128037283,
18.1085788187915,18.1963915332837,18.2843453074777,18.3616431530376,18.4493680107016,
18.5369809011481,18.6245049442856,18.7154758924521,18.8028992851819,18.8903091662094,
18.9777262923058,19.0651714204417,19.1527134250011,19.2403128340521,19.328038380529,
19.3522725296177,19.4401067268995,19.5278301686341,19.6154658340362,19.7063953430564,
19.7939323248959,19.881456326584,19.9689879833974,20.0565479310192,20.1442046095046,
20.2319187437788,20.31975821699,20.3429019061977,20.4307340263315,20.5184556296605,
20.6060896967071,20.697019894966,20.7845558931506,20.8720791412141,20.959610276429,
21.0471699366439,21.1348266789459,21.2225410820182,21.3103811242552,21.3335312827777,
21.4213251004975,21.509010264913,21.596607576048,21.6841377624944,21.7716265218872,
21.8590907051537,21.946569266503,21.9911485751285),.UNSPECIFIED.);
#2285=B_SPLINE_CURVE_WITH_KNOTS('',3,(#54744,#54745,#54746,#54747,#54748,
#54749,#54750,#54751,#54752,#54753,#54754,#54755,#54756,#54757,#54758,#54759,
#54760,#54761,#54762,#54763,#54764,#54765,#54766,#54767,#54768,#54769,#54770,
#54771,#54772,#54773,#54774,#54775,#54776,#54777,#54778,#54779,#54780,#54781,
#54782,#54783,#54784,#54785,#54786,#54787,#54788,#54789,#54790,#54791,#54792,
#54793,#54794,#54795,#54796,#54797,#54798,#54799,#54800,#54801,#54802,#54803,
#54804,#54805,#54806,#54807,#54808,#54809,#54810,#54811,#54812,#54813,#54814,
#54815,#54816,#54817,#54818,#54819,#54820,#54821,#54822,#54823,#54824,#54825,
#54826,#54827,#54828,#54829,#54830,#54831,#54832,#54833,#54834,#54835,#54836,
#54837,#54838,#54839,#54840,#54841,#54842,#54843,#54844,#54845,#54846,#54847,
#54848,#54849,#54850,#54851,#54852,#54853,#54854,#54855,#54856,#54857,#54858,
#54859,#54860,#54861,#54862,#54863,#54864,#54865,#54866,#54867,#54868,#54869,
#54870,#54871,#54872,#54873,#54874,#54875,#54876,#54877,#54878,#54879,#54880,
#54881,#54882,#54883,#54884,#54885,#54886,#54887,#54888,#54889,#54890,#54891,
#54892,#54893,#54894,#54895,#54896,#54897,#54898,#54899,#54900,#54901,#54902,
#54903,#54904,#54905,#54906,#54907,#54908,#54909,#54910,#54911,#54912,#54913,
#54914,#54915,#54916,#54917,#54918,#54919,#54920,#54921),.UNSPECIFIED.,
 .F.,.F.,(4,2,2,2,2,2,2,2,2,2,2,2,2,2,2,2,2,2,2,2,2,2,2,2,2,2,2,2,2,2,2,
2,2,2,2,2,2,2,2,2,2,2,2,2,2,2,2,2,2,2,2,2,2,2,2,2,2,2,2,2,2,2,2,2,2,2,2,
2,2,2,2,2,2,2,2,2,2,2,2,2,2,2,2,2,2,2,2,2,4),(-2.01509656764977,-2.00442233309338,
-1.9608583577495,-1.87948704543101,-1.86486657550063,-1.85607938554859,
-1.84806164739386,-1.83749996772665,-1.81324616040176,-1.77721781116714,
-1.70349473386971,-1.69305883332441,-1.68762595096638,-1.68313323006403,
-1.67719230258546,-1.66363146043247,-1.64364219553089,-1.56120202888727,
-1.53540039744752,-1.52542244956876,-1.51801059822966,-1.50980918998896,
-1.49810404406586,-1.46536688483646,-1.4048564047723,-1.36332861833298,
-1.35485467935966,-1.34989520288803,-1.34527322972197,-1.33840921159076,
-1.31833327766372,-1.2820434608007,-1.20805411918878,-1.19269330151755,
-1.18367137174265,-1.17570633079864,-1.16558618798958,-1.14400480293205,
-1.11368284458367,-1.07539126960149,-1.03072531611218,-1.01995220604332,
-1.01451931294949,-1.01002811585744,-1.00409183718097,-0.990555342435218,
-0.970615723187036,-0.888811585450084,-0.862426344445932,-0.85129421014968,
-0.843192989048181,-0.834635706030987,-0.821122162907508,-0.761468710728449,
-0.697439338488143,-0.684516130021924,-0.678746703584717,-0.674259955026725,
-0.668773483690929,-0.657725090667497,-0.642652460849895,-0.599590832733255,
-0.535943149624645,-0.520051552054786,-0.510916016790236,-0.502965578788175,
-0.493016829977024,-0.47241272073589,-0.444029850769972,-0.37785629362894,
-0.352121194415033,-0.344479781412078,-0.339699733192449,-0.334948449595917,
-0.327441082075921,-0.300958007167124,-0.239215749908723,-0.193873240375049,
-0.180734101219078,-0.172253508725591,-0.164111456249471,-0.152735532858041,
-0.122716224619186,-0.0713397715117924,-0.0212389669004389,-0.0106100332438987,
-0.00529042794641405,-0.00261557680526768,-0.000972528424130169),
 .UNSPECIFIED.);
#2286=B_SPLINE_CURVE_WITH_KNOTS('',3,(#54922,#54923,#54924,#54925,#54926,
#54927,#54928,#54929,#54930,#54931,#54932,#54933),.UNSPECIFIED.,.F.,.F.,
(4,2,2,2,2,4),(-4.27097705097338,-4.26723027831455,-4.26003241710359,-4.23690981860426,
-4.17261700115569,-4.15043685499169),.UNSPECIFIED.);
#2287=B_SPLINE_CURVE_WITH_KNOTS('',3,(#54935,#54936,#54937,#54938,#54939,
#54940,#54941,#54942,#54943,#54944,#54945,#54946,#54947),.UNSPECIFIED.,
 .F.,.F.,(4,3,3,3,4),(-10.4882942057671,-10.3977555924899,-10.3072163401549,
-10.2165955448043,-10.1336107524809),.UNSPECIFIED.);
#2288=B_SPLINE_CURVE_WITH_KNOTS('',3,(#54948,#54949,#54950,#54951,#54952,
#54953,#54954,#54955,#54956,#54957,#54958,#54959,#54960,#54961,#54962,#54963,
#54964,#54965,#54966,#54967,#54968,#54969,#54970,#54971,#54972,#54973,#54974,
#54975,#54976,#54977,#54978,#54979,#54980,#54981,#54982,#54983,#54984,#54985,
#54986,#54987,#54988,#54989,#54990,#54991,#54992,#54993,#54994,#54995,#54996,
#54997,#54998,#54999,#55000,#55001,#55002,#55003,#55004,#55005,#55006,#55007,
#55008,#55009,#55010,#55011,#55012,#55013,#55014,#55015,#55016,#55017,#55018,
#55019,#55020,#55021,#55022,#55023,#55024,#55025,#55026,#55027,#55028,#55029,
#55030,#55031,#55032,#55033,#55034,#55035,#55036,#55037,#55038,#55039,#55040,
#55041,#55042,#55043,#55044,#55045,#55046,#55047,#55048,#55049,#55050,#55051,
#55052,#55053,#55054,#55055,#55056,#55057,#55058,#55059,#55060,#55061,#55062,
#55063,#55064,#55065,#55066,#55067,#55068,#55069,#55070,#55071,#55072,#55073,
#55074,#55075,#55076,#55077,#55078,#55079,#55080,#55081,#55082,#55083,#55084,
#55085,#55086,#55087,#55088,#55089,#55090,#55091,#55092,#55093,#55094,#55095,
#55096,#55097,#55098,#55099,#55100,#55101,#55102,#55103,#55104,#55105,#55106,
#55107,#55108,#55109,#55110,#55111,#55112,#55113,#55114,#55115,#55116,#55117,
#55118,#55119,#55120,#55121,#55122,#55123),.UNSPECIFIED.,.F.,.F.,(4,2,2,
2,2,2,2,2,2,2,2,2,2,2,2,2,2,2,2,2,2,2,2,2,2,2,2,2,2,2,2,2,2,2,2,2,2,2,2,
2,2,2,2,2,2,2,2,2,2,2,2,2,2,2,2,2,2,2,2,2,2,2,2,2,2,2,2,2,2,2,2,2,2,2,2,
2,2,2,2,2,2,2,2,2,2,2,2,4),(1.42898336541552,1.46742042112348,1.49628767324879,
1.50748242560879,1.51556335490523,1.52403877281142,1.53728854434148,1.58538207353613,
1.64511336640643,1.67122017213511,1.67867093854414,1.68339288630674,1.68817396892759,
1.69581737063309,1.7215622074559,1.78120946774099,1.82889513342733,1.84216590412159,
1.85068238563881,1.8588247819375,1.87014569937684,1.89966303694102,1.94933960584668,
2.00176420693129,2.0124627931025,2.01788921483925,2.02239031356692,2.02836373761618,
2.04210157404567,2.0624546801884,2.15010624733382,2.17227476486632,2.18249828827888,
2.19047738888946,2.19944523224858,2.21493687033016,2.26438326886928,2.33884446341765,
2.34917154282268,2.35458140550876,2.35907481829952,2.36504235539273,2.37877234152408,
2.39911564013077,2.48666264161458,2.50894350254305,2.51918007663318,2.52715367372913,
2.53609874002411,2.55150650100293,2.60038497279164,2.67585417911298,2.68599672903178,
2.69136531045916,2.69586331645455,2.70188621777872,2.71593968890811,2.73696465367393,
2.82131097911041,2.84470522745123,2.85517774105293,2.86320851512811,2.87195340468667,
2.88636803507151,2.94862908948105,3.0128998568419,3.02278794986426,3.02810540927959,
3.03257077225844,3.03865180033539,3.05306208137573,3.07485511640371,3.12305130328204,
3.17486450111713,3.18824825716846,3.19678029661692,3.20489719519077,3.21611528228411,
3.24467251611403,3.29167571826644,3.34865407437406,3.35903110763528,3.36445108845531,
3.36894453296996,3.37490069007886,3.38161060650366,3.3934525021966,3.44312968008527),
 .UNSPECIFIED.);
#2289=B_SPLINE_CURVE_WITH_KNOTS('',3,(#55126,#55127,#55128,#55129,#55130,
#55131,#55132,#55133,#55134,#55135,#55136,#55137,#55138,#55139,#55140,#55141,
#55142,#55143,#55144,#55145,#55146,#55147,#55148,#55149,#55150,#55151,#55152,
#55153,#55154,#55155,#55156,#55157,#55158,#55159,#55160,#55161,#55162,#55163,
#55164,#55165,#55166,#55167,#55168,#55169,#55170,#55171,#55172,#55173,#55174,
#55175,#55176,#55177,#55178,#55179,#55180,#55181,#55182,#55183,#55184,#55185,
#55186,#55187,#55188,#55189,#55190,#55191,#55192,#55193,#55194,#55195,#55196,
#55197,#55198,#55199,#55200,#55201,#55202,#55203,#55204,#55205,#55206,#55207,
#55208,#55209,#55210,#55211,#55212,#55213,#55214,#55215,#55216,#55217,#55218,
#55219,#55220,#55221,#55222,#55223,#55224,#55225,#55226,#55227,#55228,#55229,
#55230,#55231,#55232,#55233,#55234,#55235,#55236,#55237,#55238,#55239,#55240,
#55241,#55242,#55243,#55244,#55245,#55246,#55247,#55248,#55249,#55250,#55251,
#55252,#55253,#55254,#55255,#55256,#55257,#55258,#55259,#55260,#55261,#55262,
#55263,#55264,#55265,#55266,#55267,#55268,#55269,#55270),.UNSPECIFIED.,
 .F.,.F.,(4,3,3,3,3,3,3,3,3,3,3,3,3,3,3,3,3,3,3,3,3,3,3,3,3,3,3,3,3,3,3,
3,3,3,3,3,3,3,3,3,3,3,3,3,3,3,3,3,4),(17.9338701936111,18.0215425484498,
18.1091390091939,18.1966882371871,18.2842137695347,18.3717362510166,18.4592763192238,
18.5469081233696,18.6345877563007,18.7224058342168,18.7919434588766,18.8797523761682,
18.9674503808827,19.0550604846278,19.1459995284814,19.2335108046853,19.3210090929069,
19.4085150568561,19.4960493606828,19.583680598315,19.6713693803307,19.7591838251699,
19.7825728354566,19.8703922614065,19.9581008994616,20.0457217474393,20.136656805514,
20.2241790336769,20.3116883315558,20.3992053509585,20.4867507441582,20.5743930657194,
20.6620929414952,20.7499184099657,20.7732022120367,20.8610210915467,20.948729199622,
21.0363495346721,21.1272847914152,21.2148065529677,21.302315402261,21.3898319916896,
21.4773769741273,21.5650189156996,21.652718428991,21.7405435635626,21.7638315886167,
21.8810158224684,21.9911485751285),.UNSPECIFIED.);
#2290=B_SPLINE_CURVE_WITH_KNOTS('',3,(#55271,#55272,#55273,#55274,#55275,
#55276,#55277,#55278,#55279,#55280,#55281,#55282,#55283,#55284,#55285,#55286,
#55287,#55288,#55289,#55290,#55291,#55292,#55293,#55294,#55295,#55296,#55297,
#55298,#55299,#55300,#55301,#55302,#55303,#55304,#55305,#55306,#55307,#55308,
#55309,#55310,#55311,#55312,#55313,#55314,#55315,#55316,#55317,#55318,#55319,
#55320,#55321,#55322,#55323,#55324,#55325,#55326,#55327,#55328,#55329,#55330,
#55331,#55332,#55333,#55334,#55335,#55336,#55337,#55338,#55339,#55340,#55341,
#55342,#55343,#55344,#55345,#55346,#55347,#55348,#55349,#55350,#55351,#55352),
 .UNSPECIFIED.,.F.,.F.,(4,3,3,3,3,3,3,3,3,3,3,3,3,3,3,3,3,3,3,3,3,3,3,3,
3,3,3,4),(21.9911485752709,22.0776484873086,22.1640859035787,22.2504905951409,
22.3368842548815,22.4232885627304,22.5097777277752,22.5963104523736,22.682979609016,
22.7544609651967,22.8422789541284,22.9299861499661,23.0176055523507,23.108541151029,
23.1960619347146,23.2835697910957,23.3710853735935,23.4586293360987,23.5462702434834,
23.6339687130605,23.7217927978273,23.7450903417767,23.8329109525895,23.9206242639913,
24.0082359438482,24.0957889951867,24.1833036461088,24.2166288571228),
 .UNSPECIFIED.);
#2291=B_SPLINE_CURVE_WITH_KNOTS('',3,(#55354,#55355,#55356,#55357,#55358,
#55359,#55360,#55361,#55362,#55363,#55364,#55365,#55366,#55367,#55368,#55369,
#55370,#55371,#55372,#55373,#55374,#55375,#55376,#55377,#55378,#55379,#55380,
#55381,#55382,#55383,#55384,#55385,#55386,#55387,#55388,#55389,#55390,#55391,
#55392,#55393,#55394,#55395,#55396,#55397,#55398,#55399,#55400,#55401,#55402,
#55403,#55404,#55405,#55406,#55407,#55408,#55409,#55410,#55411,#55412,#55413,
#55414,#55415,#55416,#55417,#55418,#55419,#55420,#55421,#55422,#55423,#55424,
#55425,#55426,#55427,#55428,#55429,#55430,#55431,#55432,#55433,#55434,#55435),
 .UNSPECIFIED.,.F.,.F.,(4,3,3,3,3,3,3,3,3,3,3,3,3,3,3,3,3,3,3,3,3,3,3,3,
3,3,3,4),(21.991148575328,22.0925750122967,22.1945818395017,22.2972449529874,
22.3241606593577,22.4119800933751,22.4996887395737,22.5873095957602,22.6782446507824,
22.7657668872646,22.853276193489,22.9407932212544,23.0283386228251,23.1159809527272,
23.203680836836,23.2915063135646,23.3147900359378,23.4026142424768,23.4903263956193,
23.5810553112597,23.6686080545512,23.7561253408872,23.8436278370528,23.9311361939092,
24.0187081497838,24.106318314622,24.1940259083462,24.2161577207422),
 .UNSPECIFIED.);
#2292=B_SPLINE_CURVE_WITH_KNOTS('',3,(#55436,#55437,#55438,#55439,#55440,
#55441,#55442,#55443,#55444,#55445,#55446,#55447,#55448,#55449,#55450,#55451,
#55452,#55453,#55454,#55455,#55456,#55457,#55458,#55459,#55460,#55461,#55462,
#55463,#55464,#55465,#55466,#55467,#55468,#55469,#55470,#55471,#55472,#55473,
#55474,#55475,#55476,#55477,#55478,#55479,#55480,#55481,#55482,#55483,#55484,
#55485,#55486,#55487,#55488,#55489,#55490,#55491,#55492,#55493,#55494,#55495,
#55496,#55497,#55498,#55499,#55500,#55501,#55502,#55503,#55504,#55505,#55506,
#55507,#55508,#55509,#55510,#55511,#55512,#55513,#55514,#55515,#55516,#55517,
#55518,#55519,#55520,#55521,#55522,#55523,#55524,#55525,#55526,#55527,#55528,
#55529,#55530,#55531,#55532,#55533,#55534,#55535,#55536,#55537,#55538,#55539,
#55540,#55541,#55542,#55543,#55544,#55545,#55546,#55547,#55548,#55549,#55550,
#55551,#55552,#55553,#55554,#55555,#55556,#55557,#55558,#55559,#55560,#55561,
#55562,#55563,#55564,#55565,#55566,#55567,#55568,#55569,#55570,#55571,#55572,
#55573,#55574,#55575,#55576,#55577,#55578,#55579,#55580,#55581,#55582,#55583),
 .UNSPECIFIED.,.F.,.F.,(4,3,3,3,3,3,3,3,3,3,3,3,3,3,3,3,3,3,3,3,3,3,3,3,
3,3,3,3,3,3,3,3,3,3,3,3,3,3,3,3,3,3,3,3,3,3,3,3,3,4),(17.9331346413009,
18.0208008549548,18.1085586349722,18.1963630282738,18.2843083902826,18.3616431530376,
18.4493863215626,18.5370177657643,18.6245605825582,18.7155245759407,18.8029671774752,
18.8903963961828,18.9778329691677,19.0652976337961,19.1528592120373,19.2404782401086,
19.328223323708,19.3522725296177,19.4400992198406,19.5278150837884,19.6154431104019,
19.7063754598764,19.7939046999881,19.8814209354505,19.9689448099973,20.0564969677625,
20.144145884356,20.2318522639848,20.3196840522245,20.3429019061977,20.4307323378319,
20.5184522110659,20.6060845086748,20.6970153554376,20.7845494965245,20.8720708581442,
20.9596000794408,21.047157800116,21.1348125742423,21.222524990115,21.3103630321082,
21.3335312827777,21.421328203082,21.5090165109469,21.5966170027785,21.6841504035972,
21.7716424163973,21.8591098761587,21.9465917337312,21.9911485751285),
 .UNSPECIFIED.);
#2293=B_SPLINE_CURVE_WITH_KNOTS('',3,(#55585,#55586,#55587,#55588,#55589,
#55590,#55591,#55592,#55593,#55594,#55595,#55596,#55597,#55598,#55599,#55600,
#55601,#55602,#55603,#55604,#55605,#55606,#55607,#55608,#55609,#55610,#55611,
#55612,#55613,#55614,#55615,#55616,#55617,#55618,#55619,#55620,#55621,#55622,
#55623,#55624,#55625,#55626,#55627,#55628,#55629,#55630,#55631,#55632,#55633,
#55634,#55635,#55636,#55637,#55638,#55639,#55640,#55641,#55642,#55643,#55644,
#55645,#55646,#55647,#55648,#55649,#55650,#55651,#55652,#55653,#55654,#55655,
#55656,#55657,#55658,#55659,#55660,#55661,#55662,#55663,#55664,#55665,#55666,
#55667,#55668,#55669,#55670,#55671,#55672,#55673,#55674,#55675,#55676,#55677,
#55678,#55679,#55680,#55681),.UNSPECIFIED.,.F.,.F.,(4,3,3,3,3,3,3,3,3,3,
3,3,3,3,3,3,3,3,3,3,3,3,3,3,3,3,3,3,3,3,3,3,4),(-0.760759816994444,-0.728264991811328,
-0.695770166628212,-0.679277258312604,-0.673133552693547,-0.639296875083126,
-0.609964780509387,-0.599335840102474,-0.591522810183719,-0.556929583326479,
-0.521819327675206,-0.48700557018393,-0.46641420726125,-0.455506208456746,
-0.450683812595539,-0.414689753833517,-0.404640118493211,-0.369640440894481,
-0.33464076329575,-0.314658074377986,-0.309087722362195,-0.304655337289647,
-0.268706903554133,-0.232146738196951,-0.195137918029292,-0.172257529468521,
-0.161271461718819,-0.155984382027272,-0.118128117568438,-0.0801985115663637,
-0.0429532259117857,-0.0149177406115184,-7.75271862796333E-5),
 .UNSPECIFIED.);
#2294=B_SPLINE_CURVE_WITH_KNOTS('',3,(#55682,#55683,#55684,#55685,#55686,
#55687,#55688,#55689,#55690,#55691,#55692,#55693,#55694,#55695,#55696,#55697,
#55698,#55699,#55700,#55701,#55702,#55703,#55704,#55705,#55706,#55707,#55708,
#55709,#55710,#55711,#55712,#55713,#55714,#55715,#55716,#55717,#55718,#55719,
#55720,#55721,#55722,#55723,#55724,#55725,#55726,#55727,#55728,#55729,#55730,
#55731,#55732,#55733,#55734,#55735,#55736,#55737,#55738,#55739,#55740,#55741,
#55742,#55743,#55744,#55745,#55746,#55747,#55748,#55749,#55750,#55751,#55752,
#55753,#55754,#55755,#55756,#55757,#55758,#55759,#55760,#55761,#55762,#55763,
#55764,#55765,#55766,#55767,#55768,#55769,#55770,#55771,#55772,#55773,#55774,
#55775,#55776,#55777,#55778,#55779,#55780,#55781),.UNSPECIFIED.,.F.,.F.,
(4,3,3,3,3,3,3,3,3,3,3,3,3,3,3,3,3,3,3,3,3,3,3,3,3,3,3,3,3,3,3,3,3,4),(-0.757763664684544,
-0.720381973657696,-0.682469288080949,-0.665926778923518,-0.657236479192177,
-0.619823586647078,-0.58844849796256,-0.574621441004157,-0.568708672760664,
-0.563214615962493,-0.526686992270663,-0.490320816525781,-0.45498363839703,
-0.433443448090507,-0.420354083330733,-0.414509335427944,-0.379623925576214,
-0.368822877170939,-0.33339680623558,-0.297701811576582,-0.279872858492725,
-0.274338169979935,-0.269571988414296,-0.234853323947987,-0.200243129273121,
-0.165977491882068,-0.146785125676167,-0.136607374511969,-0.130842930290342,
-0.0974426608405007,-0.0645413522423534,-0.0326213770037655,-0.0124385622348649,
0.),.UNSPECIFIED.);
#2295=B_SPLINE_CURVE_WITH_KNOTS('',3,(#56066,#56067,#56068,#56069,#56070,
#56071,#56072,#56073,#56074,#56075,#56076,#56077,#56078,#56079,#56080,#56081,
#56082,#56083,#56084,#56085,#56086,#56087,#56088,#56089,#56090,#56091,#56092,
#56093,#56094,#56095,#56096,#56097,#56098,#56099,#56100,#56101,#56102,#56103,
#56104,#56105,#56106,#56107,#56108,#56109,#56110,#56111,#56112,#56113,#56114,
#56115,#56116,#56117,#56118,#56119,#56120,#56121,#56122,#56123,#56124,#56125,
#56126,#56127,#56128,#56129,#56130,#56131,#56132,#56133,#56134,#56135,#56136,
#56137,#56138,#56139,#56140,#56141,#56142,#56143,#56144,#56145,#56146,#56147,
#56148,#56149,#56150,#56151,#56152,#56153,#56154,#56155,#56156,#56157,#56158,
#56159,#56160,#56161,#56162),.UNSPECIFIED.,.F.,.F.,(4,3,3,3,3,3,3,3,3,3,
3,3,3,3,3,3,3,3,3,3,3,3,3,3,3,3,3,3,3,3,3,3,4),(0.,0.0317312806353046,0.0642559409710066,
0.0977155979249547,0.129677601589085,0.134721269266439,0.168713657830876,
0.203412250787311,0.238085926099261,0.267345190569703,0.27293511481588,
0.277770698819479,0.313396265799393,0.348890032601819,0.355122983981029,
0.389870418620742,0.41193498250944,0.417350288416101,0.422249312177161,
0.457204205816802,0.493397395543351,0.529989879387874,0.55660407456938,
0.565580838002556,0.571298452925119,0.608611867141919,0.64218476056642,
0.656270742946784,0.66268483640152,0.700540820507026,0.7381751635799,0.742903440839923,
0.757686396975181),.UNSPECIFIED.);
#2296=B_SPLINE_CURVE_WITH_KNOTS('',3,(#56448,#56449,#56450,#56451),
 .UNSPECIFIED.,.F.,.F.,(4,4),(-0.0163901208212989,0.),.UNSPECIFIED.);
#2297=B_SPLINE_CURVE_WITH_KNOTS('',3,(#56452,#56453,#56454,#56455,#56456,
#56457,#56458,#56459,#56460,#56461,#56462,#56463,#56464,#56465,#56466,#56467,
#56468,#56469,#56470,#56471,#56472,#56473,#56474,#56475,#56476,#56477,#56478,
#56479,#56480,#56481,#56482,#56483,#56484,#56485,#56486,#56487,#56488,#56489,
#56490,#56491,#56492,#56493,#56494,#56495,#56496,#56497,#56498,#56499,#56500,
#56501,#56502,#56503,#56504,#56505,#56506,#56507,#56508,#56509,#56510,#56511,
#56512,#56513,#56514,#56515,#56516,#56517,#56518,#56519,#56520,#56521,#56522,
#56523,#56524,#56525,#56526,#56527,#56528,#56529,#56530,#56531,#56532,#56533,
#56534,#56535,#56536,#56537,#56538,#56539,#56540,#56541,#56542,#56543,#56544,
#56545,#56546,#56547,#56548),.UNSPECIFIED.,.F.,.F.,(4,3,3,3,3,3,3,3,3,3,
3,3,3,3,3,3,3,3,3,3,3,3,3,3,3,3,3,3,3,3,3,3,4),(0.,0.0369273503214421,0.075453949697969,
0.113980549074496,0.148593722241587,0.155414829285566,0.15991268003852,
0.196868730101154,0.233511857819008,0.269948573766588,0.300182913927748,
0.30668030757842,0.311558445745243,0.346837776429413,0.381907055493282,
0.390885934411227,0.426888021696901,0.446975199311113,0.453110029126761,
0.457477086043627,0.492330531618533,0.527975345133486,0.56362015864844,
0.586702996757923,0.593773585511785,0.59917438939843,0.633033686297888,
0.662014224183436,0.675195718914722,0.683250103205775,0.715766483365038,
0.7482828635243,0.760759816994426),.UNSPECIFIED.);
#2298=B_SPLINE_CURVE_WITH_KNOTS('',3,(#56550,#56551,#56552,#56553,#56554,
#56555,#56556,#56557,#56558,#56559,#56560,#56561,#56562,#56563,#56564,#56565,
#56566,#56567,#56568,#56569,#56570,#56571,#56572,#56573,#56574,#56575,#56576,
#56577,#56578,#56579,#56580,#56581,#56582,#56583,#56584,#56585,#56586,#56587,
#56588,#56589,#56590,#56591,#56592,#56593,#56594,#56595,#56596,#56597,#56598,
#56599,#56600,#56601,#56602,#56603,#56604,#56605,#56606,#56607,#56608,#56609,
#56610,#56611,#56612,#56613,#56614,#56615,#56616,#56617,#56618,#56619,#56620,
#56621,#56622,#56623,#56624,#56625,#56626,#56627,#56628,#56629,#56630,#56631,
#56632,#56633,#56634,#56635,#56636,#56637,#56638,#56639,#56640,#56641,#56642,
#56643,#56644,#56645,#56646),.UNSPECIFIED.,.F.,.F.,(4,3,3,3,3,3,3,3,3,3,
3,3,3,3,3,3,3,3,3,3,3,3,3,3,3,3,3,3,3,3,3,3,4),(-0.760759816994476,-0.72867719727751,
-0.695709509772144,-0.679296483390001,-0.67313674552237,-0.639623085494667,
-0.605457437465359,-0.599329771118666,-0.591523612514049,-0.556772239761969,
-0.521698252355195,-0.486799294770719,-0.466411345045984,-0.455503194092392,
-0.450680887225085,-0.414687271005122,-0.404640118493233,-0.369644644590622,
-0.334649170688011,-0.31466595630823,-0.309139237774412,-0.304706649237392,
-0.26876366107657,-0.23220698919768,-0.195198522951163,-0.172299540947597,
-0.161302847522944,-0.15637940503376,-0.118526813930542,-0.0805957826481643,
-0.0433462769323225,-0.0149177406115232,-7.70745645911542E-5),
 .UNSPECIFIED.);
#2299=B_SPLINE_CURVE_WITH_KNOTS('',3,(#56647,#56648,#56649,#56650,#56651,
#56652,#56653,#56654,#56655,#56656,#56657,#56658,#56659,#56660,#56661,#56662,
#56663,#56664,#56665,#56666,#56667,#56668,#56669,#56670,#56671,#56672,#56673,
#56674,#56675,#56676,#56677,#56678,#56679,#56680,#56681,#56682,#56683,#56684,
#56685,#56686,#56687,#56688,#56689,#56690,#56691,#56692,#56693,#56694,#56695,
#56696,#56697,#56698,#56699,#56700,#56701,#56702,#56703,#56704,#56705,#56706,
#56707,#56708,#56709,#56710,#56711,#56712,#56713,#56714,#56715,#56716,#56717,
#56718,#56719,#56720,#56721,#56722,#56723,#56724,#56725,#56726,#56727,#56728,
#56729,#56730,#56731,#56732,#56733,#56734,#56735,#56736,#56737,#56738,#56739,
#56740,#56741,#56742,#56743,#56744,#56745,#56746),.UNSPECIFIED.,.F.,.F.,
(4,3,3,3,3,3,3,3,3,3,3,3,3,3,3,3,3,3,3,3,3,3,3,3,3,3,3,3,3,3,3,3,3,4),(-0.757763664684541,
-0.720112840922623,-0.682462017160704,-0.665890632802888,-0.657236256652766,
-0.619823116120217,-0.588448296754926,-0.57462061065214,-0.568701943316166,
-0.563203084666934,-0.526652622723307,-0.490393340155699,-0.455008271985665,
-0.433438531484178,-0.420355266574036,-0.414509519578869,-0.379626370547332,
-0.368822877170946,-0.333397756276839,-0.297724697737825,-0.279872859743228,
-0.274339772740684,-0.269574604924806,-0.234866697539682,-0.200136844250274,
-0.166019399733717,-0.146788550715945,-0.136613171362025,-0.130388812283381,
-0.0969950806536839,-0.0641041103661313,-0.0321947839414556,-0.0124385622348649,
0.),.UNSPECIFIED.);
#2300=B_SPLINE_CURVE_WITH_KNOTS('',3,(#57031,#57032,#57033,#57034,#57035,
#57036,#57037,#57038,#57039,#57040,#57041,#57042,#57043,#57044,#57045,#57046,
#57047,#57048,#57049,#57050,#57051,#57052,#57053,#57054,#57055,#57056,#57057,
#57058,#57059,#57060,#57061,#57062,#57063,#57064,#57065,#57066,#57067,#57068,
#57069,#57070,#57071,#57072,#57073,#57074,#57075,#57076,#57077,#57078,#57079,
#57080,#57081,#57082,#57083,#57084,#57085,#57086,#57087,#57088,#57089,#57090,
#57091,#57092,#57093,#57094,#57095,#57096,#57097,#57098,#57099,#57100,#57101,
#57102,#57103,#57104,#57105,#57106,#57107,#57108,#57109,#57110,#57111,#57112,
#57113,#57114,#57115,#57116,#57117,#57118,#57119,#57120,#57121,#57122,#57123,
#57124),.UNSPECIFIED.,.F.,.F.,(4,3,3,3,3,3,3,3,3,3,3,3,3,3,3,3,3,3,3,3,
3,3,3,3,3,3,3,3,3,3,3,4),(7.37877496047656E-15,0.0324242548762023,0.0650764812389879,
0.0985463434422195,0.129697019504787,0.134733032820196,0.169300198334513,
0.203925126369526,0.238560097109361,0.273001694877465,0.278364300420405,
0.314020733983785,0.349481131532155,0.355122983981017,0.389954438528394,
0.411931265454395,0.417329657811387,0.422220055612132,0.457543827286333,
0.493520000679641,0.53011436736757,0.556569343667961,0.565759141712967,
0.571513495091189,0.608852677501213,0.637578888089422,0.651941993383527,
0.660700630375842,0.666305098677632,0.704604269758768,0.742903440839903,
0.757686857130631),.UNSPECIFIED.);
#2301=B_SPLINE_CURVE_WITH_KNOTS('',3,(#57410,#57411,#57412,#57413),
 .UNSPECIFIED.,.F.,.F.,(4,4),(-0.0162873320748038,0.),.UNSPECIFIED.);
#2302=B_SPLINE_CURVE_WITH_KNOTS('',3,(#57414,#57415,#57416,#57417,#57418,
#57419,#57420,#57421,#57422,#57423,#57424,#57425,#57426,#57427,#57428,#57429,
#57430,#57431,#57432,#57433,#57434,#57435,#57436,#57437,#57438,#57439,#57440,
#57441,#57442,#57443,#57444,#57445,#57446,#57447,#57448,#57449,#57450,#57451,
#57452,#57453,#57454,#57455,#57456,#57457,#57458,#57459,#57460,#57461,#57462,
#57463,#57464,#57465,#57466,#57467,#57468,#57469,#57470,#57471,#57472,#57473,
#57474,#57475,#57476,#57477,#57478,#57479,#57480,#57481,#57482,#57483,#57484,
#57485,#57486,#57487,#57488,#57489,#57490,#57491,#57492,#57493,#57494,#57495,
#57496,#57497,#57498,#57499,#57500,#57501,#57502,#57503,#57504,#57505,#57506,
#57507,#57508,#57509,#57510,#57511,#57512,#57513),.UNSPECIFIED.,.F.,.F.,
(4,3,3,3,3,3,3,3,3,3,3,3,3,3,3,3,3,3,3,3,3,3,3,3,3,3,3,3,3,3,3,3,3,4),(8.40311229217861E-15,
0.037154906704243,0.0748575402003926,0.112713526298086,0.148602209914868,
0.155563216342729,0.160137581649395,0.197101195136362,0.233889668479667,
0.269838109891337,0.300344302506693,0.307574466956952,0.312824195400226,
0.348077394899254,0.383139909542925,0.390885934411227,0.426911554808929,
0.446975445769724,0.453109734545746,0.457476473349302,0.492419953500651,
0.527549736956349,0.562225774259029,0.586701706612183,0.593769976980005,
0.599171096269385,0.633029003473375,0.662011207283425,0.673224422339548,
0.681404190977219,0.683249578743692,0.715766221134031,0.74828286352437,
0.7607598169945),.UNSPECIFIED.);
#2303=B_SPLINE_CURVE_WITH_KNOTS('',3,(#57515,#57516,#57517,#57518,#57519,
#57520,#57521,#57522,#57523,#57524,#57525,#57526,#57527,#57528,#57529,#57530,
#57531,#57532,#57533,#57534,#57535,#57536,#57537,#57538,#57539,#57540,#57541,
#57542,#57543,#57544,#57545,#57546,#57547,#57548,#57549,#57550,#57551,#57552,
#57553,#57554,#57555,#57556,#57557,#57558,#57559,#57560,#57561,#57562,#57563,
#57564,#57565,#57566,#57567,#57568,#57569,#57570,#57571,#57572,#57573,#57574,
#57575,#57576,#57577,#57578,#57579,#57580,#57581,#57582,#57583,#57584,#57585,
#57586,#57587,#57588,#57589,#57590,#57591,#57592,#57593,#57594,#57595,#57596,
#57597,#57598,#57599,#57600,#57601,#57602,#57603,#57604,#57605,#57606,#57607,
#57608,#57609,#57610,#57611),.UNSPECIFIED.,.F.,.F.,(4,3,3,3,3,3,3,3,3,3,
3,3,3,3,3,3,3,3,3,3,3,3,3,3,3,3,3,3,3,3,3,3,4),(-0.760759816994569,-0.728265012223969,
-0.695770207453369,-0.679277205036654,-0.673133543750063,-0.639296880860471,
-0.60996478556457,-0.599335856776469,-0.591522808027896,-0.556929595372945,
-0.521884160161627,-0.486981466865639,-0.466414215846013,-0.455506217424483,
-0.450683821468725,-0.414689761897011,-0.404640118493263,-0.369640429831607,
-0.334640741169951,-0.314658053635049,-0.309087585707408,-0.304655192905571,
-0.268706744459819,-0.232146569596101,-0.19513774849793,-0.17225741155648,
-0.161271373612937,-0.155984378195552,-0.118128111533916,-0.080198505595755,
-0.0429532188256224,-0.0149177406115174,-7.75300628616282E-5),
 .UNSPECIFIED.);
#2304=B_SPLINE_CURVE_WITH_KNOTS('',3,(#57612,#57613,#57614,#57615,#57616,
#57617,#57618,#57619,#57620,#57621,#57622,#57623,#57624,#57625,#57626,#57627,
#57628,#57629,#57630,#57631,#57632,#57633,#57634,#57635,#57636,#57637,#57638,
#57639,#57640,#57641,#57642,#57643,#57644,#57645,#57646,#57647,#57648,#57649,
#57650,#57651,#57652,#57653,#57654,#57655,#57656,#57657,#57658,#57659,#57660,
#57661,#57662,#57663,#57664,#57665,#57666,#57667,#57668,#57669,#57670,#57671,
#57672,#57673,#57674,#57675,#57676,#57677,#57678,#57679,#57680,#57681,#57682,
#57683,#57684,#57685,#57686,#57687,#57688,#57689,#57690,#57691,#57692,#57693,
#57694,#57695,#57696,#57697,#57698,#57699,#57700,#57701,#57702,#57703,#57704,
#57705,#57706,#57707,#57708,#57709,#57710,#57711),.UNSPECIFIED.,.F.,.F.,
(4,3,3,3,3,3,3,3,3,3,3,3,3,3,3,3,3,3,3,3,3,3,3,3,3,3,3,3,3,3,3,3,3,4),(-0.757763664684454,
-0.720381983678288,-0.682469301582833,-0.665926845916897,-0.657236479144063,
-0.619823586771666,-0.588448498071578,-0.574621442191374,-0.568708683306026,
-0.563214634116051,-0.526663060420545,-0.490401464824994,-0.455014148149494,
-0.433443455337693,-0.420354081977822,-0.414509335454218,-0.379623921634209,
-0.36882287717096,-0.333396805704032,-0.29770181177085,-0.279872858674851,
-0.274338167969609,-0.269571984980098,-0.234909244560119,-0.200298697723679,
-0.165977486809442,-0.14678512123762,-0.136607366744964,-0.130842926885658,
-0.0973672231254303,-0.0647374859486738,-0.0326213606334859,-0.0124385622348654,
0.),.UNSPECIFIED.);
#2305=B_SPLINE_CURVE_WITH_KNOTS('',3,(#57996,#57997,#57998,#57999,#58000,
#58001,#58002,#58003,#58004,#58005,#58006,#58007,#58008,#58009,#58010,#58011,
#58012,#58013,#58014,#58015,#58016,#58017,#58018,#58019,#58020,#58021,#58022,
#58023,#58024,#58025,#58026,#58027,#58028,#58029,#58030,#58031,#58032,#58033,
#58034,#58035,#58036,#58037,#58038,#58039,#58040,#58041,#58042,#58043,#58044,
#58045,#58046,#58047,#58048,#58049,#58050,#58051,#58052,#58053,#58054,#58055,
#58056,#58057,#58058,#58059,#58060,#58061,#58062,#58063,#58064,#58065,#58066,
#58067,#58068,#58069,#58070,#58071,#58072,#58073,#58074,#58075,#58076,#58077,
#58078,#58079,#58080,#58081,#58082,#58083,#58084,#58085,#58086,#58087,#58088,
#58089,#58090,#58091,#58092),.UNSPECIFIED.,.F.,.F.,(4,3,3,3,3,3,3,3,3,3,
3,3,3,3,3,3,3,3,3,3,3,3,3,3,3,3,3,3,3,3,3,3,4),(0.,0.0317312649685969,0.0642559110632862,
0.0974710776091265,0.12967756590561,0.134721247960768,0.168753867071307,
0.20335447753473,0.238023614120417,0.267345161024578,0.27293499338489,0.277770512668279,
0.3133960762696,0.348889848578609,0.355122983980998,0.389870425600039,0.411934989052527,
0.417350324507801,0.422249364155745,0.457397349687017,0.493693649725071,
0.529989949763124,0.556604136147715,0.56558068166977,0.571298424882708,
0.608725571359697,0.642184740832426,0.65627071778627,0.66268481658205,0.700540800689733,
0.738175144334356,0.74290344083985,0.757686395020893),.UNSPECIFIED.);
#2306=B_SPLINE_CURVE_WITH_KNOTS('',3,(#58378,#58379,#58380,#58381),
 .UNSPECIFIED.,.F.,.F.,(4,4),(-0.0163907070131913,0.),.UNSPECIFIED.);
#2307=B_SPLINE_CURVE_WITH_KNOTS('',3,(#58382,#58383,#58384,#58385,#58386,
#58387,#58388,#58389,#58390,#58391,#58392,#58393,#58394,#58395,#58396,#58397,
#58398,#58399,#58400,#58401,#58402,#58403,#58404,#58405,#58406,#58407,#58408,
#58409,#58410,#58411,#58412,#58413,#58414,#58415,#58416,#58417,#58418,#58419,
#58420,#58421,#58422,#58423,#58424,#58425,#58426,#58427,#58428,#58429,#58430,
#58431,#58432,#58433,#58434,#58435,#58436,#58437,#58438,#58439,#58440,#58441,
#58442,#58443,#58444,#58445,#58446,#58447,#58448,#58449,#58450,#58451,#58452,
#58453,#58454,#58455,#58456,#58457,#58458,#58459,#58460,#58461,#58462,#58463,
#58464,#58465,#58466,#58467,#58468,#58469,#58470,#58471,#58472,#58473,#58474,
#58475,#58476,#58477,#58478),.UNSPECIFIED.,.F.,.F.,(4,3,3,3,3,3,3,3,3,3,
3,3,3,3,3,3,3,3,3,3,3,3,3,3,3,3,3,3,3,3,3,3,4),(0.,0.0371488255941907,0.0748481542789714,
0.112705168174495,0.148593698835094,0.15541443824774,0.159912176538531,
0.196868224356431,0.233511365402667,0.269948093072399,0.300182553407106,
0.306678475117778,0.311556542095174,0.347097110787367,0.381905205719197,
0.39088593441123,0.426888020859033,0.446975198525616,0.453110029188261,
0.457477086646452,0.492330532691639,0.527975346805991,0.563620160920343,
0.586702998745845,0.593773594183896,0.599174397431784,0.633258020605501,
0.662014231335216,0.675195728621906,0.683250104575177,0.715766484049769,
0.74828286352436,0.760759816994485),.UNSPECIFIED.);
#2308=B_SPLINE_CURVE_WITH_KNOTS('',3,(#58480,#58481,#58482,#58483,#58484,
#58485,#58486,#58487,#58488,#58489,#58490,#58491,#58492,#58493,#58494,#58495,
#58496,#58497,#58498,#58499,#58500,#58501,#58502,#58503,#58504,#58505,#58506,
#58507,#58508,#58509,#58510,#58511,#58512,#58513,#58514,#58515,#58516,#58517,
#58518,#58519,#58520,#58521,#58522,#58523,#58524,#58525,#58526,#58527,#58528,
#58529,#58530,#58531,#58532,#58533,#58534,#58535,#58536,#58537,#58538,#58539,
#58540,#58541,#58542,#58543,#58544,#58545,#58546,#58547,#58548,#58549,#58550,
#58551,#58552,#58553,#58554,#58555,#58556,#58557,#58558,#58559,#58560,#58561,
#58562,#58563,#58564,#58565,#58566,#58567,#58568,#58569,#58570,#58571,#58572,
#58573,#58574,#58575,#58576),.UNSPECIFIED.,.F.,.F.,(4,3,3,3,3,3,3,3,3,3,
3,3,3,3,3,3,3,3,3,3,3,3,3,3,3,3,3,3,3,3,3,3,4),(-0.760759816994486,-0.728677168897516,
-0.695709459409064,-0.679296550858681,-0.673136756605015,-0.639623073529853,
-0.605457412994165,-0.599329749581528,-0.591523615338422,-0.5567722273375,
-0.52169823453926,-0.486799286134059,-0.466411335710125,-0.455503184191866,
-0.450680877744631,-0.414687263581558,-0.404640118493239,-0.370062588212486,
-0.334594449163023,-0.314665985300723,-0.309139425335693,-0.304706824750879,
-0.268763856298477,-0.232207196979931,-0.195198731916467,-0.17229968507175,
-0.161302955218476,-0.156379428357842,-0.118526840186713,-0.0805958087489636,
-0.0433463054005835,-0.0149177406115234,-7.70748816987286E-5),
 .UNSPECIFIED.);
#2309=B_SPLINE_CURVE_WITH_KNOTS('',3,(#58577,#58578,#58579,#58580,#58581,
#58582,#58583,#58584,#58585,#58586,#58587,#58588,#58589,#58590,#58591,#58592,
#58593,#58594,#58595,#58596,#58597,#58598,#58599,#58600,#58601,#58602,#58603,
#58604,#58605,#58606,#58607,#58608,#58609,#58610,#58611,#58612,#58613,#58614,
#58615,#58616,#58617,#58618,#58619,#58620,#58621,#58622,#58623,#58624,#58625,
#58626,#58627,#58628,#58629,#58630,#58631,#58632,#58633,#58634,#58635,#58636,
#58637,#58638,#58639,#58640,#58641,#58642,#58643,#58644,#58645,#58646,#58647,
#58648,#58649,#58650,#58651,#58652,#58653,#58654,#58655,#58656,#58657,#58658,
#58659,#58660,#58661,#58662,#58663,#58664,#58665,#58666,#58667,#58668,#58669,
#58670,#58671,#58672,#58673,#58674,#58675,#58676),.UNSPECIFIED.,.F.,.F.,
(4,3,3,3,3,3,3,3,3,3,3,3,3,3,3,3,3,3,3,3,3,3,3,3,3,3,3,3,3,3,3,3,3,4),(-0.75776366468452,
-0.72011282712767,-0.68246198957082,-0.665890495352086,-0.657236255224794,
-0.61982311437852,-0.588448295761168,-0.574620607209714,-0.568701916322679,
-0.563203038262648,-0.5266525809423,-0.490393307629812,-0.455008248392471,
-0.433438511839063,-0.420355271578355,-0.414509520573623,-0.379626380580655,
-0.368822877170925,-0.333217025002694,-0.297701813310625,-0.27987286011839,
-0.274339780902846,-0.26957461784756,-0.234866709644299,-0.200136856371557,
-0.166019419234261,-0.146788567732903,-0.136613199619544,-0.130845342725424,
-0.0974461208295118,-0.0645472684616144,-0.0326317837335634,-0.0124385622348647,
0.),.UNSPECIFIED.);
#2310=B_SPLINE_CURVE_WITH_KNOTS('',3,(#58961,#58962,#58963,#58964,#58965,
#58966,#58967,#58968,#58969,#58970,#58971,#58972,#58973,#58974,#58975,#58976,
#58977,#58978,#58979,#58980,#58981,#58982,#58983,#58984,#58985,#58986,#58987,
#58988,#58989,#58990,#58991,#58992,#58993,#58994,#58995,#58996,#58997,#58998,
#58999,#59000,#59001,#59002,#59003,#59004,#59005,#59006,#59007,#59008,#59009,
#59010,#59011,#59012,#59013,#59014,#59015,#59016,#59017,#59018,#59019,#59020,
#59021,#59022,#59023,#59024,#59025,#59026,#59027,#59028,#59029,#59030,#59031,
#59032,#59033,#59034,#59035,#59036,#59037,#59038,#59039,#59040,#59041,#59042,
#59043,#59044,#59045,#59046,#59047,#59048,#59049,#59050,#59051,#59052,#59053,
#59054),.UNSPECIFIED.,.F.,.F.,(4,3,3,3,3,3,3,3,3,3,3,3,3,3,3,3,3,3,3,3,
3,3,3,3,3,3,3,3,3,3,3,4),(7.37877496047521E-15,0.0324242735236978,0.0650765288202324,
0.0985464079585014,0.129697094094769,0.134733078671135,0.168898023091528,
0.203503086561803,0.238170057614052,0.267361263736785,0.273576206797938,
0.27836433821044,0.314020768760248,0.349481163000816,0.355122983981023,
0.3899544235958,0.411931250623808,0.417329575041924,0.42221994011044,0.457543689126243,
0.493519846720045,0.530114209763389,0.556569206240022,0.564438243045673,
0.572420851034514,0.609740985058124,0.647119750965754,0.656486576561947,
0.666305087445587,0.704604264142757,0.742903440839926,0.757686856778839),
 .UNSPECIFIED.);
#2311=B_SPLINE_CURVE_WITH_KNOTS('',3,(#59340,#59341,#59342,#59343),
 .UNSPECIFIED.,.F.,.F.,(4,4),(-0.0162873178926763,0.),.UNSPECIFIED.);
#2312=B_SPLINE_CURVE_WITH_KNOTS('',3,(#59344,#59345,#59346,#59347,#59348,
#59349,#59350,#59351,#59352,#59353,#59354,#59355,#59356,#59357,#59358,#59359,
#59360,#59361,#59362,#59363,#59364,#59365,#59366,#59367,#59368,#59369,#59370,
#59371,#59372,#59373,#59374,#59375,#59376,#59377,#59378,#59379,#59380,#59381,
#59382,#59383,#59384,#59385,#59386,#59387,#59388,#59389,#59390,#59391,#59392,
#59393,#59394,#59395,#59396,#59397,#59398,#59399,#59400,#59401,#59402,#59403,
#59404,#59405,#59406,#59407,#59408,#59409,#59410,#59411,#59412,#59413,#59414,
#59415,#59416,#59417,#59418,#59419,#59420,#59421,#59422,#59423,#59424,#59425,
#59426,#59427,#59428,#59429,#59430,#59431,#59432,#59433,#59434,#59435,#59436,
#59437,#59438,#59439,#59440),.UNSPECIFIED.,.F.,.F.,(4,3,3,3,3,3,3,3,3,3,
3,3,3,3,3,3,3,3,3,3,3,3,3,3,3,3,3,3,3,3,3,3,4),(8.4031122921758E-15,0.0371549281743425,
0.0748575730861908,0.11271355525129,0.148602239855083,0.155563764461372,
0.1601385507907,0.197102163001497,0.233890618711408,0.269839031867023,0.300344999315642,
0.307576069988628,0.312824559625132,0.34807774400219,0.383140250103658,
0.39088593441124,0.426911555703311,0.446975446515054,0.453109732596831,
0.457476469900029,0.492419949903742,0.527549734179228,0.562225766766138,
0.586701700129649,0.593769962691508,0.599171083400769,0.633028984861318,
0.662011195208229,0.675191763445889,0.683249576797649,0.715766220161021,
0.748282863524393,0.760759816994521),.UNSPECIFIED.);
#3941=LINE('',#20217,#4578);
#3942=LINE('',#20566,#4579);
#3943=LINE('',#21035,#4580);
#3944=LINE('',#21501,#4581);
#3945=LINE('',#21964,#4582);
#3946=LINE('',#22427,#4583);
#3947=LINE('',#22893,#4584);
#3948=LINE('',#23356,#4585);
#3949=LINE('',#23822,#4586);
#3950=LINE('',#24291,#4587);
#3951=LINE('',#24533,#4588);
#3952=LINE('',#24635,#4589);
#3953=LINE('',#24776,#4590);
#3954=LINE('',#25167,#4591);
#3955=LINE('',#25554,#4592);
#3956=LINE('',#25939,#4593);
#3957=LINE('',#26330,#4594);
#3958=LINE('',#26717,#4595);
#3959=LINE('',#27098,#4596);
#3960=LINE('',#27491,#4597);
#3961=LINE('',#27897,#4598);
#3962=LINE('',#28208,#4599);
#3963=LINE('',#28557,#4600);
#3964=LINE('',#29026,#4601);
#3965=LINE('',#29492,#4602);
#3966=LINE('',#29955,#4603);
#3967=LINE('',#30418,#4604);
#3968=LINE('',#30884,#4605);
#3969=LINE('',#31347,#4606);
#3970=LINE('',#31813,#4607);
#3971=LINE('',#32282,#4608);
#3972=LINE('',#32524,#4609);
#3973=LINE('',#32626,#4610);
#3974=LINE('',#32771,#4611);
#3975=LINE('',#33164,#4612);
#3976=LINE('',#33543,#4613);
#3977=LINE('',#33926,#4614);
#3978=LINE('',#34313,#4615);
#3979=LINE('',#34708,#4616);
#3980=LINE('',#35089,#4617);
#3981=LINE('',#35484,#4618);
#3982=LINE('',#35890,#4619);
#3983=LINE('',#36203,#4620);
#3984=LINE('',#36552,#4621);
#3985=LINE('',#37021,#4622);
#3986=LINE('',#37487,#4623);
#3987=LINE('',#37950,#4624);
#3988=LINE('',#38413,#4625);
#3989=LINE('',#38879,#4626);
#3990=LINE('',#39342,#4627);
#3991=LINE('',#39808,#4628);
#3992=LINE('',#40277,#4629);
#3993=LINE('',#40519,#4630);
#3994=LINE('',#40621,#4631);
#3995=LINE('',#40766,#4632);
#3996=LINE('',#41159,#4633);
#3997=LINE('',#41550,#4634);
#3998=LINE('',#41935,#4635);
#3999=LINE('',#42328,#4636);
#4000=LINE('',#42719,#4637);
#4001=LINE('',#43104,#4638);
#4002=LINE('',#43499,#4639);
#4003=LINE('',#43903,#4640);
#4004=LINE('',#44214,#4641);
#4005=LINE('',#44563,#4642);
#4006=LINE('',#45032,#4643);
#4007=LINE('',#45498,#4644);
#4008=LINE('',#45961,#4645);
#4009=LINE('',#46424,#4646);
#4010=LINE('',#46890,#4647);
#4011=LINE('',#47353,#4648);
#4012=LINE('',#47819,#4649);
#4013=LINE('',#48288,#4650);
#4014=LINE('',#48530,#4651);
#4015=LINE('',#48632,#4652);
#4016=LINE('',#48777,#4653);
#4017=LINE('',#49166,#4654);
#4018=LINE('',#49553,#4655);
#4019=LINE('',#49934,#4656);
#4020=LINE('',#50327,#4657);
#4021=LINE('',#50722,#4658);
#4022=LINE('',#51105,#4659);
#4023=LINE('',#51502,#4660);
#4024=LINE('',#51908,#4661);
#4025=LINE('',#59449,#4662);
#4026=LINE('',#59455,#4663);
#4027=LINE('',#59461,#4664);
#4028=LINE('',#59467,#4665);
#4029=LINE('',#59472,#4666);
#4030=LINE('',#59474,#4667);
#4031=LINE('',#59476,#4668);
#4032=LINE('',#59477,#4669);
#4033=LINE('',#59480,#4670);
#4034=LINE('',#59482,#4671);
#4035=LINE('',#59483,#4672);
#4036=LINE('',#59486,#4673);
#4037=LINE('',#59488,#4674);
#4038=LINE('',#59489,#4675);
#4039=LINE('',#59491,#4676);
#4040=LINE('',#59492,#4677);
#4578=VECTOR('',#17895,4.085);
#4579=VECTOR('',#17900,4.085);
#4580=VECTOR('',#17903,4.085);
#4581=VECTOR('',#17906,4.085);
#4582=VECTOR('',#17909,4.085);
#4583=VECTOR('',#17912,4.085);
#4584=VECTOR('',#17915,4.085);
#4585=VECTOR('',#17918,4.085);
#4586=VECTOR('',#17921,4.085);
#4587=VECTOR('',#17924,4.085);
#4588=VECTOR('',#17929,3.38975);
#4589=VECTOR('',#17932,3.38975);
#4590=VECTOR('',#17939,3.38975);
#4591=VECTOR('',#17942,3.38975);
#4592=VECTOR('',#17945,3.38975);
#4593=VECTOR('',#17948,3.38975);
#4594=VECTOR('',#17951,3.38975);
#4595=VECTOR('',#17954,3.38975);
#4596=VECTOR('',#17957,3.38975);
#4597=VECTOR('',#17960,3.38975);
#4598=VECTOR('',#17963,3.38975);
#4599=VECTOR('',#17968,4.085);
#4600=VECTOR('',#17973,4.085);
#4601=VECTOR('',#17976,4.085);
#4602=VECTOR('',#17979,4.085);
#4603=VECTOR('',#17982,4.085);
#4604=VECTOR('',#17985,4.085);
#4605=VECTOR('',#17988,4.085);
#4606=VECTOR('',#17991,4.085);
#4607=VECTOR('',#17994,4.085);
#4608=VECTOR('',#17997,4.085);
#4609=VECTOR('',#18002,3.38975);
#4610=VECTOR('',#18005,3.38975);
#4611=VECTOR('',#18012,3.38975);
#4612=VECTOR('',#18015,3.38975);
#4613=VECTOR('',#18018,3.38975);
#4614=VECTOR('',#18021,3.38975);
#4615=VECTOR('',#18024,3.38975);
#4616=VECTOR('',#18027,3.38975);
#4617=VECTOR('',#18030,3.38975);
#4618=VECTOR('',#18033,3.38975);
#4619=VECTOR('',#18036,3.38975);
#4620=VECTOR('',#18041,4.085);
#4621=VECTOR('',#18046,4.085);
#4622=VECTOR('',#18049,4.085);
#4623=VECTOR('',#18052,4.085);
#4624=VECTOR('',#18055,4.085);
#4625=VECTOR('',#18058,4.085);
#4626=VECTOR('',#18061,4.085);
#4627=VECTOR('',#18064,4.085);
#4628=VECTOR('',#18067,4.085);
#4629=VECTOR('',#18070,4.085);
#4630=VECTOR('',#18075,3.38975);
#4631=VECTOR('',#18078,3.38975);
#4632=VECTOR('',#18085,3.38975);
#4633=VECTOR('',#18088,3.38975);
#4634=VECTOR('',#18091,3.38975);
#4635=VECTOR('',#18094,3.38975);
#4636=VECTOR('',#18097,3.38975);
#4637=VECTOR('',#18100,3.38975);
#4638=VECTOR('',#18103,3.38975);
#4639=VECTOR('',#18106,3.38975);
#4640=VECTOR('',#18109,3.38975);
#4641=VECTOR('',#18114,4.085);
#4642=VECTOR('',#18119,4.085);
#4643=VECTOR('',#18122,4.085);
#4644=VECTOR('',#18125,4.085);
#4645=VECTOR('',#18128,4.085);
#4646=VECTOR('',#18131,4.085);
#4647=VECTOR('',#18134,4.085);
#4648=VECTOR('',#18137,4.085);
#4649=VECTOR('',#18140,4.085);
#4650=VECTOR('',#18143,4.085);
#4651=VECTOR('',#18148,3.38975);
#4652=VECTOR('',#18151,3.38975);
#4653=VECTOR('',#18158,3.38975);
#4654=VECTOR('',#18161,3.38975);
#4655=VECTOR('',#18164,3.38975);
#4656=VECTOR('',#18167,3.38975);
#4657=VECTOR('',#18170,3.38975);
#4658=VECTOR('',#18173,3.38975);
#4659=VECTOR('',#18176,3.38975);
#4660=VECTOR('',#18179,3.38975);
#4661=VECTOR('',#18182,3.38975);
#4662=VECTOR('',#18221,4.5);
#4663=VECTOR('',#18228,4.5);
#4664=VECTOR('',#18235,4.5);
#4665=VECTOR('',#18242,4.5);
#4666=VECTOR('',#18247,10.);
#4667=VECTOR('',#18248,10.);
#4668=VECTOR('',#18249,10.);
#4669=VECTOR('',#18250,10.);
#4670=VECTOR('',#18253,10.);
#4671=VECTOR('',#18254,10.);
#4672=VECTOR('',#18255,10.);
#4673=VECTOR('',#18258,10.);
#4674=VECTOR('',#18259,10.);
#4675=VECTOR('',#18260,10.);
#4676=VECTOR('',#18263,10.);
#4677=VECTOR('',#18264,10.);
#5215=VERTEX_POINT('',#20215);
#5216=VERTEX_POINT('',#20216);
#5217=VERTEX_POINT('',#20218);
#5218=VERTEX_POINT('',#20364);
#5219=VERTEX_POINT('',#20369);
#5220=VERTEX_POINT('',#20371);
#5221=VERTEX_POINT('',#20564);
#5222=VERTEX_POINT('',#20565);
#5223=VERTEX_POINT('',#20567);
#5224=VERTEX_POINT('',#20801);
#5225=VERTEX_POINT('',#21033);
#5226=VERTEX_POINT('',#21034);
#5227=VERTEX_POINT('',#21036);
#5228=VERTEX_POINT('',#21264);
#5229=VERTEX_POINT('',#21499);
#5230=VERTEX_POINT('',#21500);
#5231=VERTEX_POINT('',#21502);
#5232=VERTEX_POINT('',#21730);
#5233=VERTEX_POINT('',#21962);
#5234=VERTEX_POINT('',#21963);
#5235=VERTEX_POINT('',#21965);
#5236=VERTEX_POINT('',#22199);
#5237=VERTEX_POINT('',#22425);
#5238=VERTEX_POINT('',#22426);
#5239=VERTEX_POINT('',#22428);
#5240=VERTEX_POINT('',#22656);
#5241=VERTEX_POINT('',#22891);
#5242=VERTEX_POINT('',#22892);
#5243=VERTEX_POINT('',#22894);
#5244=VERTEX_POINT('',#23125);
#5245=VERTEX_POINT('',#23354);
#5246=VERTEX_POINT('',#23355);
#5247=VERTEX_POINT('',#23357);
#5248=VERTEX_POINT('',#23588);
#5249=VERTEX_POINT('',#23820);
#5250=VERTEX_POINT('',#23821);
#5251=VERTEX_POINT('',#23823);
#5252=VERTEX_POINT('',#24054);
#5253=VERTEX_POINT('',#24289);
#5254=VERTEX_POINT('',#24290);
#5255=VERTEX_POINT('',#24292);
#5256=VERTEX_POINT('',#24375);
#5257=VERTEX_POINT('',#24381);
#5258=VERTEX_POINT('',#24383);
#5259=VERTEX_POINT('',#24531);
#5260=VERTEX_POINT('',#24532);
#5261=VERTEX_POINT('',#24534);
#5262=VERTEX_POINT('',#24632);
#5263=VERTEX_POINT('',#24634);
#5264=VERTEX_POINT('',#24637);
#5265=VERTEX_POINT('',#24774);
#5266=VERTEX_POINT('',#24775);
#5267=VERTEX_POINT('',#24777);
#5268=VERTEX_POINT('',#25165);
#5269=VERTEX_POINT('',#25166);
#5270=VERTEX_POINT('',#25360);
#5271=VERTEX_POINT('',#25552);
#5272=VERTEX_POINT('',#25553);
#5273=VERTEX_POINT('',#25555);
#5274=VERTEX_POINT('',#25937);
#5275=VERTEX_POINT('',#25938);
#5276=VERTEX_POINT('',#26134);
#5277=VERTEX_POINT('',#26328);
#5278=VERTEX_POINT('',#26329);
#5279=VERTEX_POINT('',#26331);
#5280=VERTEX_POINT('',#26715);
#5281=VERTEX_POINT('',#26716);
#5282=VERTEX_POINT('',#26900);
#5283=VERTEX_POINT('',#27096);
#5284=VERTEX_POINT('',#27097);
#5285=VERTEX_POINT('',#27099);
#5286=VERTEX_POINT('',#27489);
#5287=VERTEX_POINT('',#27490);
#5288=VERTEX_POINT('',#27686);
#5289=VERTEX_POINT('',#27895);
#5290=VERTEX_POINT('',#27896);
#5291=VERTEX_POINT('',#27898);
#5292=VERTEX_POINT('',#28025);
#5293=VERTEX_POINT('',#28206);
#5294=VERTEX_POINT('',#28207);
#5295=VERTEX_POINT('',#28209);
#5296=VERTEX_POINT('',#28355);
#5297=VERTEX_POINT('',#28360);
#5298=VERTEX_POINT('',#28362);
#5299=VERTEX_POINT('',#28555);
#5300=VERTEX_POINT('',#28556);
#5301=VERTEX_POINT('',#28558);
#5302=VERTEX_POINT('',#28792);
#5303=VERTEX_POINT('',#29024);
#5304=VERTEX_POINT('',#29025);
#5305=VERTEX_POINT('',#29027);
#5306=VERTEX_POINT('',#29255);
#5307=VERTEX_POINT('',#29490);
#5308=VERTEX_POINT('',#29491);
#5309=VERTEX_POINT('',#29493);
#5310=VERTEX_POINT('',#29721);
#5311=VERTEX_POINT('',#29953);
#5312=VERTEX_POINT('',#29954);
#5313=VERTEX_POINT('',#29956);
#5314=VERTEX_POINT('',#30190);
#5315=VERTEX_POINT('',#30416);
#5316=VERTEX_POINT('',#30417);
#5317=VERTEX_POINT('',#30419);
#5318=VERTEX_POINT('',#30647);
#5319=VERTEX_POINT('',#30882);
#5320=VERTEX_POINT('',#30883);
#5321=VERTEX_POINT('',#30885);
#5322=VERTEX_POINT('',#31116);
#5323=VERTEX_POINT('',#31345);
#5324=VERTEX_POINT('',#31346);
#5325=VERTEX_POINT('',#31348);
#5326=VERTEX_POINT('',#31579);
#5327=VERTEX_POINT('',#31811);
#5328=VERTEX_POINT('',#31812);
#5329=VERTEX_POINT('',#31814);
#5330=VERTEX_POINT('',#32045);
#5331=VERTEX_POINT('',#32280);
#5332=VERTEX_POINT('',#32281);
#5333=VERTEX_POINT('',#32283);
#5334=VERTEX_POINT('',#32366);
#5335=VERTEX_POINT('',#32372);
#5336=VERTEX_POINT('',#32374);
#5337=VERTEX_POINT('',#32522);
#5338=VERTEX_POINT('',#32523);
#5339=VERTEX_POINT('',#32525);
#5340=VERTEX_POINT('',#32623);
#5341=VERTEX_POINT('',#32625);
#5342=VERTEX_POINT('',#32628);
#5343=VERTEX_POINT('',#32769);
#5344=VERTEX_POINT('',#32770);
#5345=VERTEX_POINT('',#32772);
#5346=VERTEX_POINT('',#33162);
#5347=VERTEX_POINT('',#33163);
#5348=VERTEX_POINT('',#33353);
#5349=VERTEX_POINT('',#33541);
#5350=VERTEX_POINT('',#33542);
#5351=VERTEX_POINT('',#33544);
#5352=VERTEX_POINT('',#33924);
#5353=VERTEX_POINT('',#33925);
#5354=VERTEX_POINT('',#34117);
#5355=VERTEX_POINT('',#34311);
#5356=VERTEX_POINT('',#34312);
#5357=VERTEX_POINT('',#34314);
#5358=VERTEX_POINT('',#34706);
#5359=VERTEX_POINT('',#34707);
#5360=VERTEX_POINT('',#34893);
#5361=VERTEX_POINT('',#35087);
#5362=VERTEX_POINT('',#35088);
#5363=VERTEX_POINT('',#35090);
#5364=VERTEX_POINT('',#35482);
#5365=VERTEX_POINT('',#35483);
#5366=VERTEX_POINT('',#35679);
#5367=VERTEX_POINT('',#35888);
#5368=VERTEX_POINT('',#35889);
#5369=VERTEX_POINT('',#35891);
#5370=VERTEX_POINT('',#36020);
#5371=VERTEX_POINT('',#36201);
#5372=VERTEX_POINT('',#36202);
#5373=VERTEX_POINT('',#36204);
#5374=VERTEX_POINT('',#36350);
#5375=VERTEX_POINT('',#36355);
#5376=VERTEX_POINT('',#36357);
#5377=VERTEX_POINT('',#36550);
#5378=VERTEX_POINT('',#36551);
#5379=VERTEX_POINT('',#36553);
#5380=VERTEX_POINT('',#36787);
#5381=VERTEX_POINT('',#37019);
#5382=VERTEX_POINT('',#37020);
#5383=VERTEX_POINT('',#37022);
#5384=VERTEX_POINT('',#37250);
#5385=VERTEX_POINT('',#37485);
#5386=VERTEX_POINT('',#37486);
#5387=VERTEX_POINT('',#37488);
#5388=VERTEX_POINT('',#37716);
#5389=VERTEX_POINT('',#37948);
#5390=VERTEX_POINT('',#37949);
#5391=VERTEX_POINT('',#37951);
#5392=VERTEX_POINT('',#38185);
#5393=VERTEX_POINT('',#38411);
#5394=VERTEX_POINT('',#38412);
#5395=VERTEX_POINT('',#38414);
#5396=VERTEX_POINT('',#38642);
#5397=VERTEX_POINT('',#38877);
#5398=VERTEX_POINT('',#38878);
#5399=VERTEX_POINT('',#38880);
#5400=VERTEX_POINT('',#39111);
#5401=VERTEX_POINT('',#39340);
#5402=VERTEX_POINT('',#39341);
#5403=VERTEX_POINT('',#39343);
#5404=VERTEX_POINT('',#39574);
#5405=VERTEX_POINT('',#39806);
#5406=VERTEX_POINT('',#39807);
#5407=VERTEX_POINT('',#39809);
#5408=VERTEX_POINT('',#40040);
#5409=VERTEX_POINT('',#40275);
#5410=VERTEX_POINT('',#40276);
#5411=VERTEX_POINT('',#40278);
#5412=VERTEX_POINT('',#40361);
#5413=VERTEX_POINT('',#40367);
#5414=VERTEX_POINT('',#40369);
#5415=VERTEX_POINT('',#40517);
#5416=VERTEX_POINT('',#40518);
#5417=VERTEX_POINT('',#40520);
#5418=VERTEX_POINT('',#40618);
#5419=VERTEX_POINT('',#40620);
#5420=VERTEX_POINT('',#40623);
#5421=VERTEX_POINT('',#40764);
#5422=VERTEX_POINT('',#40765);
#5423=VERTEX_POINT('',#40767);
#5424=VERTEX_POINT('',#41157);
#5425=VERTEX_POINT('',#41158);
#5426=VERTEX_POINT('',#41350);
#5427=VERTEX_POINT('',#41548);
#5428=VERTEX_POINT('',#41549);
#5429=VERTEX_POINT('',#41551);
#5430=VERTEX_POINT('',#41933);
#5431=VERTEX_POINT('',#41934);
#5432=VERTEX_POINT('',#42130);
#5433=VERTEX_POINT('',#42326);
#5434=VERTEX_POINT('',#42327);
#5435=VERTEX_POINT('',#42329);
#5436=VERTEX_POINT('',#42717);
#5437=VERTEX_POINT('',#42718);
#5438=VERTEX_POINT('',#42904);
#5439=VERTEX_POINT('',#43102);
#5440=VERTEX_POINT('',#43103);
#5441=VERTEX_POINT('',#43105);
#5442=VERTEX_POINT('',#43497);
#5443=VERTEX_POINT('',#43498);
#5444=VERTEX_POINT('',#43692);
#5445=VERTEX_POINT('',#43901);
#5446=VERTEX_POINT('',#43902);
#5447=VERTEX_POINT('',#43904);
#5448=VERTEX_POINT('',#44033);
#5449=VERTEX_POINT('',#44212);
#5450=VERTEX_POINT('',#44213);
#5451=VERTEX_POINT('',#44215);
#5452=VERTEX_POINT('',#44361);
#5453=VERTEX_POINT('',#44366);
#5454=VERTEX_POINT('',#44368);
#5455=VERTEX_POINT('',#44561);
#5456=VERTEX_POINT('',#44562);
#5457=VERTEX_POINT('',#44564);
#5458=VERTEX_POINT('',#44798);
#5459=VERTEX_POINT('',#45030);
#5460=VERTEX_POINT('',#45031);
#5461=VERTEX_POINT('',#45033);
#5462=VERTEX_POINT('',#45261);
#5463=VERTEX_POINT('',#45496);
#5464=VERTEX_POINT('',#45497);
#5465=VERTEX_POINT('',#45499);
#5466=VERTEX_POINT('',#45727);
#5467=VERTEX_POINT('',#45959);
#5468=VERTEX_POINT('',#45960);
#5469=VERTEX_POINT('',#45962);
#5470=VERTEX_POINT('',#46196);
#5471=VERTEX_POINT('',#46422);
#5472=VERTEX_POINT('',#46423);
#5473=VERTEX_POINT('',#46425);
#5474=VERTEX_POINT('',#46653);
#5475=VERTEX_POINT('',#46888);
#5476=VERTEX_POINT('',#46889);
#5477=VERTEX_POINT('',#46891);
#5478=VERTEX_POINT('',#47122);
#5479=VERTEX_POINT('',#47351);
#5480=VERTEX_POINT('',#47352);
#5481=VERTEX_POINT('',#47354);
#5482=VERTEX_POINT('',#47585);
#5483=VERTEX_POINT('',#47817);
#5484=VERTEX_POINT('',#47818);
#5485=VERTEX_POINT('',#47820);
#5486=VERTEX_POINT('',#48051);
#5487=VERTEX_POINT('',#48286);
#5488=VERTEX_POINT('',#48287);
#5489=VERTEX_POINT('',#48289);
#5490=VERTEX_POINT('',#48372);
#5491=VERTEX_POINT('',#48378);
#5492=VERTEX_POINT('',#48380);
#5493=VERTEX_POINT('',#48528);
#5494=VERTEX_POINT('',#48529);
#5495=VERTEX_POINT('',#48531);
#5496=VERTEX_POINT('',#48629);
#5497=VERTEX_POINT('',#48631);
#5498=VERTEX_POINT('',#48634);
#5499=VERTEX_POINT('',#48775);
#5500=VERTEX_POINT('',#48776);
#5501=VERTEX_POINT('',#48778);
#5502=VERTEX_POINT('',#49164);
#5503=VERTEX_POINT('',#49165);
#5504=VERTEX_POINT('',#49361);
#5505=VERTEX_POINT('',#49551);
#5506=VERTEX_POINT('',#49552);
#5507=VERTEX_POINT('',#49554);
#5508=VERTEX_POINT('',#49932);
#5509=VERTEX_POINT('',#49933);
#5510=VERTEX_POINT('',#50131);
#5511=VERTEX_POINT('',#50325);
#5512=VERTEX_POINT('',#50326);
#5513=VERTEX_POINT('',#50328);
#5514=VERTEX_POINT('',#50720);
#5515=VERTEX_POINT('',#50721);
#5516=VERTEX_POINT('',#50905);
#5517=VERTEX_POINT('',#51103);
#5518=VERTEX_POINT('',#51104);
#5519=VERTEX_POINT('',#51106);
#5520=VERTEX_POINT('',#51500);
#5521=VERTEX_POINT('',#51501);
#5522=VERTEX_POINT('',#51697);
#5523=VERTEX_POINT('',#51906);
#5524=VERTEX_POINT('',#51907);
#5525=VERTEX_POINT('',#51909);
#5526=VERTEX_POINT('',#52038);
#5527=VERTEX_POINT('',#52221);
#5528=VERTEX_POINT('',#52410);
#5529=VERTEX_POINT('',#52603);
#5530=VERTEX_POINT('',#52831);
#5531=VERTEX_POINT('',#53063);
#5532=VERTEX_POINT('',#53254);
#5533=VERTEX_POINT('',#53445);
#5534=VERTEX_POINT('',#53673);
#5535=VERTEX_POINT('',#53905);
#5536=VERTEX_POINT('',#54090);
#5537=VERTEX_POINT('',#54283);
#5538=VERTEX_POINT('',#54511);
#5539=VERTEX_POINT('',#54743);
#5540=VERTEX_POINT('',#54934);
#5541=VERTEX_POINT('',#55125);
#5542=VERTEX_POINT('',#55353);
#5543=VERTEX_POINT('',#56447);
#5544=VERTEX_POINT('',#57409);
#5545=VERTEX_POINT('',#58377);
#5546=VERTEX_POINT('',#59339);
#5547=VERTEX_POINT('',#59446);
#5548=VERTEX_POINT('',#59448);
#5549=VERTEX_POINT('',#59452);
#5550=VERTEX_POINT('',#59454);
#5551=VERTEX_POINT('',#59458);
#5552=VERTEX_POINT('',#59460);
#5553=VERTEX_POINT('',#59464);
#5554=VERTEX_POINT('',#59466);
#5555=VERTEX_POINT('',#59470);
#5556=VERTEX_POINT('',#59471);
#5557=VERTEX_POINT('',#59473);
#5558=VERTEX_POINT('',#59475);
#5559=VERTEX_POINT('',#59479);
#5560=VERTEX_POINT('',#59481);
#5561=VERTEX_POINT('',#59485);
#5562=VERTEX_POINT('',#59487);
#7392=EDGE_CURVE('',#5215,#5216,#3941,.T.);
#7393=EDGE_CURVE('',#5216,#5217,#1989,.T.);
#7394=EDGE_CURVE('',#5217,#5218,#1990,.T.);
#7395=EDGE_CURVE('',#5219,#5218,#1809,.T.);
#7396=EDGE_CURVE('',#5220,#5219,#1991,.T.);
#7397=EDGE_CURVE('',#5215,#5220,#1992,.T.);
#7398=EDGE_CURVE('',#5221,#5222,#3942,.T.);
#7399=EDGE_CURVE('',#5222,#5223,#1993,.T.);
#7400=EDGE_CURVE('',#5223,#5216,#1994,.T.);
#7401=EDGE_CURVE('',#5224,#5215,#1995,.T.);
#7402=EDGE_CURVE('',#5221,#5224,#1996,.T.);
#7403=EDGE_CURVE('',#5225,#5226,#3943,.T.);
#7404=EDGE_CURVE('',#5226,#5227,#1997,.T.);
#7405=EDGE_CURVE('',#5227,#5222,#1998,.T.);
#7406=EDGE_CURVE('',#5228,#5221,#1999,.T.);
#7407=EDGE_CURVE('',#5225,#5228,#2000,.T.);
#7408=EDGE_CURVE('',#5229,#5230,#3944,.T.);
#7409=EDGE_CURVE('',#5230,#5231,#2001,.T.);
#7410=EDGE_CURVE('',#5231,#5226,#2002,.T.);
#7411=EDGE_CURVE('',#5232,#5225,#2003,.T.);
#7412=EDGE_CURVE('',#5229,#5232,#2004,.T.);
#7413=EDGE_CURVE('',#5233,#5234,#3945,.T.);
#7414=EDGE_CURVE('',#5234,#5235,#2005,.T.);
#7415=EDGE_CURVE('',#5235,#5230,#2006,.T.);
#7416=EDGE_CURVE('',#5236,#5229,#2007,.T.);
#7417=EDGE_CURVE('',#5233,#5236,#2008,.T.);
#7418=EDGE_CURVE('',#5237,#5238,#3946,.T.);
#7419=EDGE_CURVE('',#5238,#5239,#2009,.T.);
#7420=EDGE_CURVE('',#5239,#5234,#2010,.T.);
#7421=EDGE_CURVE('',#5240,#5233,#2011,.T.);
#7422=EDGE_CURVE('',#5237,#5240,#2012,.T.);
#7423=EDGE_CURVE('',#5241,#5242,#3947,.T.);
#7424=EDGE_CURVE('',#5242,#5243,#2013,.T.);
#7425=EDGE_CURVE('',#5243,#5238,#2014,.T.);
#7426=EDGE_CURVE('',#5244,#5237,#2015,.T.);
#7427=EDGE_CURVE('',#5241,#5244,#2016,.T.);
#7428=EDGE_CURVE('',#5245,#5246,#3948,.T.);
#7429=EDGE_CURVE('',#5246,#5247,#2017,.T.);
#7430=EDGE_CURVE('',#5247,#5242,#2018,.T.);
#7431=EDGE_CURVE('',#5248,#5241,#2019,.T.);
#7432=EDGE_CURVE('',#5245,#5248,#2020,.T.);
#7433=EDGE_CURVE('',#5249,#5250,#3949,.T.);
#7434=EDGE_CURVE('',#5250,#5251,#2021,.T.);
#7435=EDGE_CURVE('',#5251,#5246,#2022,.T.);
#7436=EDGE_CURVE('',#5252,#5245,#2023,.T.);
#7437=EDGE_CURVE('',#5249,#5252,#2024,.T.);
#7438=EDGE_CURVE('',#5253,#5254,#3950,.T.);
#7439=EDGE_CURVE('',#5255,#5253,#2025,.T.);
#7440=EDGE_CURVE('',#5256,#5255,#2026,.T.);
#7441=EDGE_CURVE('',#5257,#5256,#1810,.T.);
#7442=EDGE_CURVE('',#5257,#5258,#2027,.T.);
#7443=EDGE_CURVE('',#5258,#5254,#2028,.T.);
#7444=EDGE_CURVE('',#5259,#5260,#3951,.T.);
#7445=EDGE_CURVE('',#5260,#5261,#2029,.T.);
#7446=EDGE_CURVE('',#5261,#5262,#1811,.T.);
#7447=EDGE_CURVE('',#5262,#5263,#3952,.T.);
#7448=EDGE_CURVE('',#5263,#5263,#1812,.F.);
#7449=EDGE_CURVE('',#5262,#5264,#1813,.T.);
#7450=EDGE_CURVE('',#5264,#5259,#2030,.T.);
#7451=EDGE_CURVE('',#5265,#5266,#3953,.T.);
#7452=EDGE_CURVE('',#5266,#5267,#2031,.T.);
#7453=EDGE_CURVE('',#5267,#5260,#2032,.T.);
#7454=EDGE_CURVE('',#5259,#5265,#2033,.T.);
#7455=EDGE_CURVE('',#5268,#5269,#3954,.T.);
#7456=EDGE_CURVE('',#5269,#5266,#2034,.T.);
#7457=EDGE_CURVE('',#5265,#5270,#2035,.T.);
#7458=EDGE_CURVE('',#5270,#5268,#2036,.T.);
#7459=EDGE_CURVE('',#5271,#5272,#3955,.T.);
#7460=EDGE_CURVE('',#5272,#5273,#2037,.T.);
#7461=EDGE_CURVE('',#5273,#5269,#2038,.T.);
#7462=EDGE_CURVE('',#5268,#5271,#2039,.T.);
#7463=EDGE_CURVE('',#5274,#5275,#3956,.T.);
#7464=EDGE_CURVE('',#5275,#5272,#2040,.T.);
#7465=EDGE_CURVE('',#5271,#5276,#2041,.T.);
#7466=EDGE_CURVE('',#5276,#5274,#2042,.T.);
#7467=EDGE_CURVE('',#5277,#5278,#3957,.T.);
#7468=EDGE_CURVE('',#5278,#5279,#2043,.T.);
#7469=EDGE_CURVE('',#5279,#5275,#2044,.T.);
#7470=EDGE_CURVE('',#5274,#5277,#2045,.T.);
#7471=EDGE_CURVE('',#5280,#5281,#3958,.T.);
#7472=EDGE_CURVE('',#5281,#5278,#2046,.T.);
#7473=EDGE_CURVE('',#5277,#5282,#2047,.T.);
#7474=EDGE_CURVE('',#5282,#5280,#2048,.T.);
#7475=EDGE_CURVE('',#5283,#5284,#3959,.T.);
#7476=EDGE_CURVE('',#5284,#5285,#2049,.T.);
#7477=EDGE_CURVE('',#5285,#5281,#2050,.T.);
#7478=EDGE_CURVE('',#5280,#5283,#2051,.T.);
#7479=EDGE_CURVE('',#5286,#5287,#3960,.T.);
#7480=EDGE_CURVE('',#5287,#5284,#2052,.T.);
#7481=EDGE_CURVE('',#5283,#5288,#2053,.T.);
#7482=EDGE_CURVE('',#5288,#5286,#2054,.T.);
#7483=EDGE_CURVE('',#5289,#5290,#3961,.T.);
#7484=EDGE_CURVE('',#5289,#5291,#2055,.F.);
#7485=EDGE_CURVE('',#5292,#5291,#1814,.T.);
#7486=EDGE_CURVE('',#5292,#5290,#2056,.T.);
#7487=EDGE_CURVE('',#5293,#5294,#3962,.T.);
#7488=EDGE_CURVE('',#5294,#5295,#2057,.T.);
#7489=EDGE_CURVE('',#5295,#5296,#2058,.T.);
#7490=EDGE_CURVE('',#5297,#5296,#1815,.T.);
#7491=EDGE_CURVE('',#5298,#5297,#2059,.T.);
#7492=EDGE_CURVE('',#5293,#5298,#2060,.T.);
#7493=EDGE_CURVE('',#5299,#5300,#3963,.T.);
#7494=EDGE_CURVE('',#5300,#5301,#2061,.T.);
#7495=EDGE_CURVE('',#5301,#5294,#2062,.T.);
#7496=EDGE_CURVE('',#5302,#5293,#2063,.T.);
#7497=EDGE_CURVE('',#5299,#5302,#2064,.T.);
#7498=EDGE_CURVE('',#5303,#5304,#3964,.T.);
#7499=EDGE_CURVE('',#5304,#5305,#2065,.T.);
#7500=EDGE_CURVE('',#5305,#5300,#2066,.T.);
#7501=EDGE_CURVE('',#5306,#5299,#2067,.T.);
#7502=EDGE_CURVE('',#5303,#5306,#2068,.T.);
#7503=EDGE_CURVE('',#5307,#5308,#3965,.T.);
#7504=EDGE_CURVE('',#5308,#5309,#2069,.T.);
#7505=EDGE_CURVE('',#5309,#5304,#2070,.T.);
#7506=EDGE_CURVE('',#5310,#5303,#2071,.T.);
#7507=EDGE_CURVE('',#5307,#5310,#2072,.T.);
#7508=EDGE_CURVE('',#5311,#5312,#3966,.T.);
#7509=EDGE_CURVE('',#5312,#5313,#2073,.T.);
#7510=EDGE_CURVE('',#5313,#5308,#2074,.T.);
#7511=EDGE_CURVE('',#5314,#5307,#2075,.T.);
#7512=EDGE_CURVE('',#5311,#5314,#2076,.T.);
#7513=EDGE_CURVE('',#5315,#5316,#3967,.T.);
#7514=EDGE_CURVE('',#5316,#5317,#2077,.T.);
#7515=EDGE_CURVE('',#5317,#5312,#2078,.T.);
#7516=EDGE_CURVE('',#5318,#5311,#2079,.T.);
#7517=EDGE_CURVE('',#5315,#5318,#2080,.T.);
#7518=EDGE_CURVE('',#5319,#5320,#3968,.T.);
#7519=EDGE_CURVE('',#5320,#5321,#2081,.T.);
#7520=EDGE_CURVE('',#5321,#5316,#2082,.T.);
#7521=EDGE_CURVE('',#5322,#5315,#2083,.T.);
#7522=EDGE_CURVE('',#5319,#5322,#2084,.T.);
#7523=EDGE_CURVE('',#5323,#5324,#3969,.T.);
#7524=EDGE_CURVE('',#5324,#5325,#2085,.T.);
#7525=EDGE_CURVE('',#5325,#5320,#2086,.T.);
#7526=EDGE_CURVE('',#5326,#5319,#2087,.T.);
#7527=EDGE_CURVE('',#5323,#5326,#2088,.T.);
#7528=EDGE_CURVE('',#5327,#5328,#3970,.T.);
#7529=EDGE_CURVE('',#5328,#5329,#2089,.T.);
#7530=EDGE_CURVE('',#5329,#5324,#2090,.T.);
#7531=EDGE_CURVE('',#5330,#5323,#2091,.T.);
#7532=EDGE_CURVE('',#5327,#5330,#2092,.T.);
#7533=EDGE_CURVE('',#5331,#5332,#3971,.T.);
#7534=EDGE_CURVE('',#5333,#5331,#2093,.T.);
#7535=EDGE_CURVE('',#5334,#5333,#2094,.T.);
#7536=EDGE_CURVE('',#5335,#5334,#1816,.T.);
#7537=EDGE_CURVE('',#5335,#5336,#2095,.T.);
#7538=EDGE_CURVE('',#5336,#5332,#2096,.T.);
#7539=EDGE_CURVE('',#5337,#5338,#3972,.T.);
#7540=EDGE_CURVE('',#5338,#5339,#2097,.T.);
#7541=EDGE_CURVE('',#5339,#5340,#1817,.T.);
#7542=EDGE_CURVE('',#5340,#5341,#3973,.T.);
#7543=EDGE_CURVE('',#5341,#5341,#1818,.F.);
#7544=EDGE_CURVE('',#5340,#5342,#1819,.T.);
#7545=EDGE_CURVE('',#5342,#5337,#2098,.T.);
#7546=EDGE_CURVE('',#5343,#5344,#3974,.T.);
#7547=EDGE_CURVE('',#5344,#5345,#2099,.T.);
#7548=EDGE_CURVE('',#5345,#5338,#2100,.T.);
#7549=EDGE_CURVE('',#5337,#5343,#2101,.T.);
#7550=EDGE_CURVE('',#5346,#5347,#3975,.T.);
#7551=EDGE_CURVE('',#5347,#5344,#2102,.T.);
#7552=EDGE_CURVE('',#5343,#5348,#2103,.T.);
#7553=EDGE_CURVE('',#5348,#5346,#2104,.T.);
#7554=EDGE_CURVE('',#5349,#5350,#3976,.T.);
#7555=EDGE_CURVE('',#5350,#5351,#2105,.T.);
#7556=EDGE_CURVE('',#5351,#5347,#2106,.T.);
#7557=EDGE_CURVE('',#5346,#5349,#2107,.T.);
#7558=EDGE_CURVE('',#5352,#5353,#3977,.T.);
#7559=EDGE_CURVE('',#5353,#5350,#2108,.T.);
#7560=EDGE_CURVE('',#5349,#5354,#2109,.T.);
#7561=EDGE_CURVE('',#5354,#5352,#2110,.T.);
#7562=EDGE_CURVE('',#5355,#5356,#3978,.T.);
#7563=EDGE_CURVE('',#5356,#5357,#2111,.T.);
#7564=EDGE_CURVE('',#5357,#5353,#2112,.T.);
#7565=EDGE_CURVE('',#5352,#5355,#2113,.T.);
#7566=EDGE_CURVE('',#5358,#5359,#3979,.T.);
#7567=EDGE_CURVE('',#5359,#5356,#2114,.T.);
#7568=EDGE_CURVE('',#5355,#5360,#2115,.T.);
#7569=EDGE_CURVE('',#5360,#5358,#2116,.T.);
#7570=EDGE_CURVE('',#5361,#5362,#3980,.T.);
#7571=EDGE_CURVE('',#5362,#5363,#2117,.T.);
#7572=EDGE_CURVE('',#5363,#5359,#2118,.T.);
#7573=EDGE_CURVE('',#5358,#5361,#2119,.T.);
#7574=EDGE_CURVE('',#5364,#5365,#3981,.T.);
#7575=EDGE_CURVE('',#5365,#5362,#2120,.T.);
#7576=EDGE_CURVE('',#5361,#5366,#2121,.T.);
#7577=EDGE_CURVE('',#5366,#5364,#2122,.T.);
#7578=EDGE_CURVE('',#5367,#5368,#3982,.T.);
#7579=EDGE_CURVE('',#5367,#5369,#2123,.F.);
#7580=EDGE_CURVE('',#5370,#5369,#1820,.T.);
#7581=EDGE_CURVE('',#5370,#5368,#2124,.T.);
#7582=EDGE_CURVE('',#5371,#5372,#3983,.T.);
#7583=EDGE_CURVE('',#5372,#5373,#2125,.T.);
#7584=EDGE_CURVE('',#5373,#5374,#2126,.T.);
#7585=EDGE_CURVE('',#5375,#5374,#1821,.T.);
#7586=EDGE_CURVE('',#5376,#5375,#2127,.T.);
#7587=EDGE_CURVE('',#5371,#5376,#2128,.T.);
#7588=EDGE_CURVE('',#5377,#5378,#3984,.T.);
#7589=EDGE_CURVE('',#5378,#5379,#2129,.T.);
#7590=EDGE_CURVE('',#5379,#5372,#2130,.T.);
#7591=EDGE_CURVE('',#5380,#5371,#2131,.T.);
#7592=EDGE_CURVE('',#5377,#5380,#2132,.T.);
#7593=EDGE_CURVE('',#5381,#5382,#3985,.T.);
#7594=EDGE_CURVE('',#5382,#5383,#2133,.T.);
#7595=EDGE_CURVE('',#5383,#5378,#2134,.T.);
#7596=EDGE_CURVE('',#5384,#5377,#2135,.T.);
#7597=EDGE_CURVE('',#5381,#5384,#2136,.T.);
#7598=EDGE_CURVE('',#5385,#5386,#3986,.T.);
#7599=EDGE_CURVE('',#5386,#5387,#2137,.T.);
#7600=EDGE_CURVE('',#5387,#5382,#2138,.T.);
#7601=EDGE_CURVE('',#5388,#5381,#2139,.T.);
#7602=EDGE_CURVE('',#5385,#5388,#2140,.T.);
#7603=EDGE_CURVE('',#5389,#5390,#3987,.T.);
#7604=EDGE_CURVE('',#5390,#5391,#2141,.T.);
#7605=EDGE_CURVE('',#5391,#5386,#2142,.T.);
#7606=EDGE_CURVE('',#5392,#5385,#2143,.T.);
#7607=EDGE_CURVE('',#5389,#5392,#2144,.T.);
#7608=EDGE_CURVE('',#5393,#5394,#3988,.T.);
#7609=EDGE_CURVE('',#5394,#5395,#2145,.T.);
#7610=EDGE_CURVE('',#5395,#5390,#2146,.T.);
#7611=EDGE_CURVE('',#5396,#5389,#2147,.T.);
#7612=EDGE_CURVE('',#5393,#5396,#2148,.T.);
#7613=EDGE_CURVE('',#5397,#5398,#3989,.T.);
#7614=EDGE_CURVE('',#5398,#5399,#2149,.T.);
#7615=EDGE_CURVE('',#5399,#5394,#2150,.T.);
#7616=EDGE_CURVE('',#5400,#5393,#2151,.T.);
#7617=EDGE_CURVE('',#5397,#5400,#2152,.T.);
#7618=EDGE_CURVE('',#5401,#5402,#3990,.T.);
#7619=EDGE_CURVE('',#5402,#5403,#2153,.T.);
#7620=EDGE_CURVE('',#5403,#5398,#2154,.T.);
#7621=EDGE_CURVE('',#5404,#5397,#2155,.T.);
#7622=EDGE_CURVE('',#5401,#5404,#2156,.T.);
#7623=EDGE_CURVE('',#5405,#5406,#3991,.T.);
#7624=EDGE_CURVE('',#5406,#5407,#2157,.T.);
#7625=EDGE_CURVE('',#5407,#5402,#2158,.T.);
#7626=EDGE_CURVE('',#5408,#5401,#2159,.T.);
#7627=EDGE_CURVE('',#5405,#5408,#2160,.T.);
#7628=EDGE_CURVE('',#5409,#5410,#3992,.T.);
#7629=EDGE_CURVE('',#5411,#5409,#2161,.T.);
#7630=EDGE_CURVE('',#5412,#5411,#2162,.T.);
#7631=EDGE_CURVE('',#5413,#5412,#1822,.T.);
#7632=EDGE_CURVE('',#5413,#5414,#2163,.T.);
#7633=EDGE_CURVE('',#5414,#5410,#2164,.T.);
#7634=EDGE_CURVE('',#5415,#5416,#3993,.T.);
#7635=EDGE_CURVE('',#5416,#5417,#2165,.T.);
#7636=EDGE_CURVE('',#5417,#5418,#1823,.T.);
#7637=EDGE_CURVE('',#5418,#5419,#3994,.T.);
#7638=EDGE_CURVE('',#5419,#5419,#1824,.F.);
#7639=EDGE_CURVE('',#5418,#5420,#1825,.T.);
#7640=EDGE_CURVE('',#5420,#5415,#2166,.T.);
#7641=EDGE_CURVE('',#5421,#5422,#3995,.T.);
#7642=EDGE_CURVE('',#5422,#5423,#2167,.T.);
#7643=EDGE_CURVE('',#5423,#5416,#2168,.T.);
#7644=EDGE_CURVE('',#5415,#5421,#2169,.T.);
#7645=EDGE_CURVE('',#5424,#5425,#3996,.T.);
#7646=EDGE_CURVE('',#5425,#5422,#2170,.T.);
#7647=EDGE_CURVE('',#5421,#5426,#2171,.T.);
#7648=EDGE_CURVE('',#5426,#5424,#2172,.T.);
#7649=EDGE_CURVE('',#5427,#5428,#3997,.T.);
#7650=EDGE_CURVE('',#5428,#5429,#2173,.T.);
#7651=EDGE_CURVE('',#5429,#5425,#2174,.T.);
#7652=EDGE_CURVE('',#5424,#5427,#2175,.T.);
#7653=EDGE_CURVE('',#5430,#5431,#3998,.T.);
#7654=EDGE_CURVE('',#5431,#5428,#2176,.T.);
#7655=EDGE_CURVE('',#5427,#5432,#2177,.T.);
#7656=EDGE_CURVE('',#5432,#5430,#2178,.T.);
#7657=EDGE_CURVE('',#5433,#5434,#3999,.T.);
#7658=EDGE_CURVE('',#5434,#5435,#2179,.T.);
#7659=EDGE_CURVE('',#5435,#5431,#2180,.T.);
#7660=EDGE_CURVE('',#5430,#5433,#2181,.T.);
#7661=EDGE_CURVE('',#5436,#5437,#4000,.T.);
#7662=EDGE_CURVE('',#5437,#5434,#2182,.T.);
#7663=EDGE_CURVE('',#5433,#5438,#2183,.T.);
#7664=EDGE_CURVE('',#5438,#5436,#2184,.T.);
#7665=EDGE_CURVE('',#5439,#5440,#4001,.T.);
#7666=EDGE_CURVE('',#5440,#5441,#2185,.T.);
#7667=EDGE_CURVE('',#5441,#5437,#2186,.T.);
#7668=EDGE_CURVE('',#5436,#5439,#2187,.T.);
#7669=EDGE_CURVE('',#5442,#5443,#4002,.T.);
#7670=EDGE_CURVE('',#5443,#5440,#2188,.T.);
#7671=EDGE_CURVE('',#5439,#5444,#2189,.T.);
#7672=EDGE_CURVE('',#5444,#5442,#2190,.T.);
#7673=EDGE_CURVE('',#5445,#5446,#4003,.T.);
#7674=EDGE_CURVE('',#5445,#5447,#2191,.F.);
#7675=EDGE_CURVE('',#5448,#5447,#1826,.T.);
#7676=EDGE_CURVE('',#5448,#5446,#2192,.T.);
#7677=EDGE_CURVE('',#5449,#5450,#4004,.T.);
#7678=EDGE_CURVE('',#5450,#5451,#2193,.T.);
#7679=EDGE_CURVE('',#5451,#5452,#2194,.T.);
#7680=EDGE_CURVE('',#5453,#5452,#1827,.T.);
#7681=EDGE_CURVE('',#5454,#5453,#2195,.T.);
#7682=EDGE_CURVE('',#5449,#5454,#2196,.T.);
#7683=EDGE_CURVE('',#5455,#5456,#4005,.T.);
#7684=EDGE_CURVE('',#5456,#5457,#2197,.T.);
#7685=EDGE_CURVE('',#5457,#5450,#2198,.T.);
#7686=EDGE_CURVE('',#5458,#5449,#2199,.T.);
#7687=EDGE_CURVE('',#5455,#5458,#2200,.T.);
#7688=EDGE_CURVE('',#5459,#5460,#4006,.T.);
#7689=EDGE_CURVE('',#5460,#5461,#2201,.T.);
#7690=EDGE_CURVE('',#5461,#5456,#2202,.T.);
#7691=EDGE_CURVE('',#5462,#5455,#2203,.T.);
#7692=EDGE_CURVE('',#5459,#5462,#2204,.T.);
#7693=EDGE_CURVE('',#5463,#5464,#4007,.T.);
#7694=EDGE_CURVE('',#5464,#5465,#2205,.T.);
#7695=EDGE_CURVE('',#5465,#5460,#2206,.T.);
#7696=EDGE_CURVE('',#5466,#5459,#2207,.T.);
#7697=EDGE_CURVE('',#5463,#5466,#2208,.T.);
#7698=EDGE_CURVE('',#5467,#5468,#4008,.T.);
#7699=EDGE_CURVE('',#5468,#5469,#2209,.T.);
#7700=EDGE_CURVE('',#5469,#5464,#2210,.T.);
#7701=EDGE_CURVE('',#5470,#5463,#2211,.T.);
#7702=EDGE_CURVE('',#5467,#5470,#2212,.T.);
#7703=EDGE_CURVE('',#5471,#5472,#4009,.T.);
#7704=EDGE_CURVE('',#5472,#5473,#2213,.T.);
#7705=EDGE_CURVE('',#5473,#5468,#2214,.T.);
#7706=EDGE_CURVE('',#5474,#5467,#2215,.T.);
#7707=EDGE_CURVE('',#5471,#5474,#2216,.T.);
#7708=EDGE_CURVE('',#5475,#5476,#4010,.T.);
#7709=EDGE_CURVE('',#5476,#5477,#2217,.T.);
#7710=EDGE_CURVE('',#5477,#5472,#2218,.T.);
#7711=EDGE_CURVE('',#5478,#5471,#2219,.T.);
#7712=EDGE_CURVE('',#5475,#5478,#2220,.T.);
#7713=EDGE_CURVE('',#5479,#5480,#4011,.T.);
#7714=EDGE_CURVE('',#5480,#5481,#2221,.T.);
#7715=EDGE_CURVE('',#5481,#5476,#2222,.T.);
#7716=EDGE_CURVE('',#5482,#5475,#2223,.T.);
#7717=EDGE_CURVE('',#5479,#5482,#2224,.T.);
#7718=EDGE_CURVE('',#5483,#5484,#4012,.T.);
#7719=EDGE_CURVE('',#5484,#5485,#2225,.T.);
#7720=EDGE_CURVE('',#5485,#5480,#2226,.T.);
#7721=EDGE_CURVE('',#5486,#5479,#2227,.T.);
#7722=EDGE_CURVE('',#5483,#5486,#2228,.T.);
#7723=EDGE_CURVE('',#5487,#5488,#4013,.T.);
#7724=EDGE_CURVE('',#5489,#5487,#2229,.T.);
#7725=EDGE_CURVE('',#5490,#5489,#2230,.T.);
#7726=EDGE_CURVE('',#5491,#5490,#1828,.T.);
#7727=EDGE_CURVE('',#5491,#5492,#2231,.T.);
#7728=EDGE_CURVE('',#5492,#5488,#2232,.T.);
#7729=EDGE_CURVE('',#5493,#5494,#4014,.T.);
#7730=EDGE_CURVE('',#5494,#5495,#2233,.T.);
#7731=EDGE_CURVE('',#5495,#5496,#1829,.T.);
#7732=EDGE_CURVE('',#5496,#5497,#4015,.T.);
#7733=EDGE_CURVE('',#5497,#5497,#1830,.F.);
#7734=EDGE_CURVE('',#5496,#5498,#1831,.T.);
#7735=EDGE_CURVE('',#5498,#5493,#2234,.T.);
#7736=EDGE_CURVE('',#5499,#5500,#4016,.T.);
#7737=EDGE_CURVE('',#5500,#5501,#2235,.T.);
#7738=EDGE_CURVE('',#5501,#5494,#2236,.T.);
#7739=EDGE_CURVE('',#5493,#5499,#2237,.T.);
#7740=EDGE_CURVE('',#5502,#5503,#4017,.T.);
#7741=EDGE_CURVE('',#5503,#5500,#2238,.T.);
#7742=EDGE_CURVE('',#5499,#5504,#2239,.T.);
#7743=EDGE_CURVE('',#5504,#5502,#2240,.T.);
#7744=EDGE_CURVE('',#5505,#5506,#4018,.T.);
#7745=EDGE_CURVE('',#5506,#5507,#2241,.T.);
#7746=EDGE_CURVE('',#5507,#5503,#2242,.T.);
#7747=EDGE_CURVE('',#5502,#5505,#2243,.T.);
#7748=EDGE_CURVE('',#5508,#5509,#4019,.T.);
#7749=EDGE_CURVE('',#5509,#5506,#2244,.T.);
#7750=EDGE_CURVE('',#5505,#5510,#2245,.T.);
#7751=EDGE_CURVE('',#5510,#5508,#2246,.T.);
#7752=EDGE_CURVE('',#5511,#5512,#4020,.T.);
#7753=EDGE_CURVE('',#5512,#5513,#2247,.T.);
#7754=EDGE_CURVE('',#5513,#5509,#2248,.T.);
#7755=EDGE_CURVE('',#5508,#5511,#2249,.T.);
#7756=EDGE_CURVE('',#5514,#5515,#4021,.T.);
#7757=EDGE_CURVE('',#5515,#5512,#2250,.T.);
#7758=EDGE_CURVE('',#5511,#5516,#2251,.T.);
#7759=EDGE_CURVE('',#5516,#5514,#2252,.T.);
#7760=EDGE_CURVE('',#5517,#5518,#4022,.T.);
#7761=EDGE_CURVE('',#5518,#5519,#2253,.T.);
#7762=EDGE_CURVE('',#5519,#5515,#2254,.T.);
#7763=EDGE_CURVE('',#5514,#5517,#2255,.T.);
#7764=EDGE_CURVE('',#5520,#5521,#4023,.T.);
#7765=EDGE_CURVE('',#5521,#5518,#2256,.T.);
#7766=EDGE_CURVE('',#5517,#5522,#2257,.T.);
#7767=EDGE_CURVE('',#5522,#5520,#2258,.T.);
#7768=EDGE_CURVE('',#5523,#5524,#4024,.T.);
#7769=EDGE_CURVE('',#5523,#5525,#2259,.F.);
#7770=EDGE_CURVE('',#5526,#5525,#1832,.T.);
#7771=EDGE_CURVE('',#5526,#5524,#2260,.T.);
#7772=EDGE_CURVE('',#5524,#5527,#2261,.T.);
#7773=EDGE_CURVE('',#5527,#5521,#2262,.T.);
#7774=EDGE_CURVE('',#5520,#5528,#2263,.T.);
#7775=EDGE_CURVE('',#5528,#5523,#2264,.F.);
#7776=EDGE_CURVE('',#5488,#5529,#2265,.T.);
#7777=EDGE_CURVE('',#5529,#5484,#2266,.T.);
#7778=EDGE_CURVE('',#5530,#5483,#2267,.T.);
#7779=EDGE_CURVE('',#5487,#5530,#2268,.T.);
#7780=EDGE_CURVE('',#5446,#5531,#2269,.T.);
#7781=EDGE_CURVE('',#5531,#5443,#2270,.T.);
#7782=EDGE_CURVE('',#5442,#5532,#2271,.T.);
#7783=EDGE_CURVE('',#5532,#5445,#2272,.F.);
#7784=EDGE_CURVE('',#5410,#5533,#2273,.T.);
#7785=EDGE_CURVE('',#5533,#5406,#2274,.T.);
#7786=EDGE_CURVE('',#5534,#5405,#2275,.T.);
#7787=EDGE_CURVE('',#5409,#5534,#2276,.T.);
#7788=EDGE_CURVE('',#5368,#5535,#2277,.T.);
#7789=EDGE_CURVE('',#5535,#5365,#2278,.T.);
#7790=EDGE_CURVE('',#5364,#5536,#2279,.T.);
#7791=EDGE_CURVE('',#5536,#5367,#2280,.F.);
#7792=EDGE_CURVE('',#5332,#5537,#2281,.T.);
#7793=EDGE_CURVE('',#5537,#5328,#2282,.T.);
#7794=EDGE_CURVE('',#5538,#5327,#2283,.T.);
#7795=EDGE_CURVE('',#5331,#5538,#2284,.T.);
#7796=EDGE_CURVE('',#5290,#5539,#2285,.T.);
#7797=EDGE_CURVE('',#5539,#5287,#2286,.T.);
#7798=EDGE_CURVE('',#5286,#5540,#2287,.T.);
#7799=EDGE_CURVE('',#5540,#5289,#2288,.F.);
#7800=EDGE_CURVE('',#5254,#5541,#2289,.T.);
#7801=EDGE_CURVE('',#5541,#5250,#2290,.T.);
#7802=EDGE_CURVE('',#5542,#5249,#2291,.T.);
#7803=EDGE_CURVE('',#5253,#5542,#2292,.T.);
#7804=EDGE_CURVE('',#5261,#5219,#2293,.T.);
#7805=EDGE_CURVE('',#5218,#5264,#2294,.T.);
#7806=EDGE_CURVE('',#5291,#5257,#2295,.T.);
#7807=EDGE_CURVE('',#5543,#5292,#2296,.T.);
#7808=EDGE_CURVE('',#5256,#5543,#2297,.T.);
#7809=EDGE_CURVE('',#5339,#5297,#2298,.T.);
#7810=EDGE_CURVE('',#5296,#5342,#2299,.T.);
#7811=EDGE_CURVE('',#5369,#5335,#2300,.T.);
#7812=EDGE_CURVE('',#5544,#5370,#2301,.T.);
#7813=EDGE_CURVE('',#5334,#5544,#2302,.T.);
#7814=EDGE_CURVE('',#5417,#5375,#2303,.T.);
#7815=EDGE_CURVE('',#5374,#5420,#2304,.T.);
#7816=EDGE_CURVE('',#5447,#5413,#2305,.T.);
#7817=EDGE_CURVE('',#5545,#5448,#2306,.T.);
#7818=EDGE_CURVE('',#5412,#5545,#2307,.T.);
#7819=EDGE_CURVE('',#5495,#5453,#2308,.T.);
#7820=EDGE_CURVE('',#5452,#5498,#2309,.T.);
#7821=EDGE_CURVE('',#5525,#5491,#2310,.T.);
#7822=EDGE_CURVE('',#5546,#5526,#2311,.T.);
#7823=EDGE_CURVE('',#5490,#5546,#2312,.T.);
#7824=EDGE_CURVE('',#5547,#5547,#1833,.T.);
#7825=EDGE_CURVE('',#5547,#5548,#4025,.T.);
#7826=EDGE_CURVE('',#5548,#5548,#1834,.T.);
#7827=EDGE_CURVE('',#5549,#5549,#1835,.T.);
#7828=EDGE_CURVE('',#5549,#5550,#4026,.T.);
#7829=EDGE_CURVE('',#5550,#5550,#1836,.T.);
#7830=EDGE_CURVE('',#5551,#5551,#1837,.T.);
#7831=EDGE_CURVE('',#5551,#5552,#4027,.T.);
#7832=EDGE_CURVE('',#5552,#5552,#1838,.T.);
#7833=EDGE_CURVE('',#5553,#5553,#1839,.T.);
#7834=EDGE_CURVE('',#5553,#5554,#4028,.T.);
#7835=EDGE_CURVE('',#5554,#5554,#1840,.T.);
#7836=EDGE_CURVE('',#5555,#5556,#4029,.F.);
#7837=EDGE_CURVE('',#5556,#5557,#4030,.T.);
#7838=EDGE_CURVE('',#5558,#5557,#4031,.F.);
#7839=EDGE_CURVE('',#5555,#5558,#4032,.T.);
#7840=EDGE_CURVE('',#5559,#5555,#4033,.F.);
#7841=EDGE_CURVE('',#5560,#5558,#4034,.F.);
#7842=EDGE_CURVE('',#5559,#5560,#4035,.F.);
#7843=EDGE_CURVE('',#5561,#5559,#4036,.F.);
#7844=EDGE_CURVE('',#5562,#5560,#4037,.F.);
#7845=EDGE_CURVE('',#5561,#5562,#4038,.F.);
#7846=EDGE_CURVE('',#5556,#5561,#4039,.F.);
#7847=EDGE_CURVE('',#5557,#5562,#4040,.F.);
#10161=ORIENTED_EDGE('',*,*,#7392,.T.);
#10162=ORIENTED_EDGE('',*,*,#7393,.T.);
#10163=ORIENTED_EDGE('',*,*,#7394,.T.);
#10164=ORIENTED_EDGE('',*,*,#7395,.F.);
#10165=ORIENTED_EDGE('',*,*,#7396,.F.);
#10166=ORIENTED_EDGE('',*,*,#7397,.F.);
#10167=ORIENTED_EDGE('',*,*,#7398,.T.);
#10168=ORIENTED_EDGE('',*,*,#7399,.T.);
#10169=ORIENTED_EDGE('',*,*,#7400,.T.);
#10170=ORIENTED_EDGE('',*,*,#7392,.F.);
#10171=ORIENTED_EDGE('',*,*,#7401,.F.);
#10172=ORIENTED_EDGE('',*,*,#7402,.F.);
#10173=ORIENTED_EDGE('',*,*,#7403,.T.);
#10174=ORIENTED_EDGE('',*,*,#7404,.T.);
#10175=ORIENTED_EDGE('',*,*,#7405,.T.);
#10176=ORIENTED_EDGE('',*,*,#7398,.F.);
#10177=ORIENTED_EDGE('',*,*,#7406,.F.);
#10178=ORIENTED_EDGE('',*,*,#7407,.F.);
#10179=ORIENTED_EDGE('',*,*,#7408,.T.);
#10180=ORIENTED_EDGE('',*,*,#7409,.T.);
#10181=ORIENTED_EDGE('',*,*,#7410,.T.);
#10182=ORIENTED_EDGE('',*,*,#7403,.F.);
#10183=ORIENTED_EDGE('',*,*,#7411,.F.);
#10184=ORIENTED_EDGE('',*,*,#7412,.F.);
#10185=ORIENTED_EDGE('',*,*,#7413,.T.);
#10186=ORIENTED_EDGE('',*,*,#7414,.T.);
#10187=ORIENTED_EDGE('',*,*,#7415,.T.);
#10188=ORIENTED_EDGE('',*,*,#7408,.F.);
#10189=ORIENTED_EDGE('',*,*,#7416,.F.);
#10190=ORIENTED_EDGE('',*,*,#7417,.F.);
#10191=ORIENTED_EDGE('',*,*,#7418,.T.);
#10192=ORIENTED_EDGE('',*,*,#7419,.T.);
#10193=ORIENTED_EDGE('',*,*,#7420,.T.);
#10194=ORIENTED_EDGE('',*,*,#7413,.F.);
#10195=ORIENTED_EDGE('',*,*,#7421,.F.);
#10196=ORIENTED_EDGE('',*,*,#7422,.F.);
#10197=ORIENTED_EDGE('',*,*,#7423,.T.);
#10198=ORIENTED_EDGE('',*,*,#7424,.T.);
#10199=ORIENTED_EDGE('',*,*,#7425,.T.);
#10200=ORIENTED_EDGE('',*,*,#7418,.F.);
#10201=ORIENTED_EDGE('',*,*,#7426,.F.);
#10202=ORIENTED_EDGE('',*,*,#7427,.F.);
#10203=ORIENTED_EDGE('',*,*,#7428,.T.);
#10204=ORIENTED_EDGE('',*,*,#7429,.T.);
#10205=ORIENTED_EDGE('',*,*,#7430,.T.);
#10206=ORIENTED_EDGE('',*,*,#7423,.F.);
#10207=ORIENTED_EDGE('',*,*,#7431,.F.);
#10208=ORIENTED_EDGE('',*,*,#7432,.F.);
#10209=ORIENTED_EDGE('',*,*,#7433,.T.);
#10210=ORIENTED_EDGE('',*,*,#7434,.T.);
#10211=ORIENTED_EDGE('',*,*,#7435,.T.);
#10212=ORIENTED_EDGE('',*,*,#7428,.F.);
#10213=ORIENTED_EDGE('',*,*,#7436,.F.);
#10214=ORIENTED_EDGE('',*,*,#7437,.F.);
#10215=ORIENTED_EDGE('',*,*,#7438,.F.);
#10216=ORIENTED_EDGE('',*,*,#7439,.F.);
#10217=ORIENTED_EDGE('',*,*,#7440,.F.);
#10218=ORIENTED_EDGE('',*,*,#7441,.F.);
#10219=ORIENTED_EDGE('',*,*,#7442,.T.);
#10220=ORIENTED_EDGE('',*,*,#7443,.T.);
#10221=ORIENTED_EDGE('',*,*,#7444,.T.);
#10222=ORIENTED_EDGE('',*,*,#7445,.T.);
#10223=ORIENTED_EDGE('',*,*,#7446,.T.);
#10224=ORIENTED_EDGE('',*,*,#7447,.T.);
#10225=ORIENTED_EDGE('',*,*,#7448,.T.);
#10226=ORIENTED_EDGE('',*,*,#7447,.F.);
#10227=ORIENTED_EDGE('',*,*,#7449,.T.);
#10228=ORIENTED_EDGE('',*,*,#7450,.T.);
#10229=ORIENTED_EDGE('',*,*,#7451,.T.);
#10230=ORIENTED_EDGE('',*,*,#7452,.T.);
#10231=ORIENTED_EDGE('',*,*,#7453,.T.);
#10232=ORIENTED_EDGE('',*,*,#7444,.F.);
#10233=ORIENTED_EDGE('',*,*,#7454,.T.);
#10234=ORIENTED_EDGE('',*,*,#7455,.T.);
#10235=ORIENTED_EDGE('',*,*,#7456,.T.);
#10236=ORIENTED_EDGE('',*,*,#7451,.F.);
#10237=ORIENTED_EDGE('',*,*,#7457,.T.);
#10238=ORIENTED_EDGE('',*,*,#7458,.T.);
#10239=ORIENTED_EDGE('',*,*,#7459,.T.);
#10240=ORIENTED_EDGE('',*,*,#7460,.T.);
#10241=ORIENTED_EDGE('',*,*,#7461,.T.);
#10242=ORIENTED_EDGE('',*,*,#7455,.F.);
#10243=ORIENTED_EDGE('',*,*,#7462,.T.);
#10244=ORIENTED_EDGE('',*,*,#7463,.T.);
#10245=ORIENTED_EDGE('',*,*,#7464,.T.);
#10246=ORIENTED_EDGE('',*,*,#7459,.F.);
#10247=ORIENTED_EDGE('',*,*,#7465,.T.);
#10248=ORIENTED_EDGE('',*,*,#7466,.T.);
#10249=ORIENTED_EDGE('',*,*,#7467,.T.);
#10250=ORIENTED_EDGE('',*,*,#7468,.T.);
#10251=ORIENTED_EDGE('',*,*,#7469,.T.);
#10252=ORIENTED_EDGE('',*,*,#7463,.F.);
#10253=ORIENTED_EDGE('',*,*,#7470,.T.);
#10254=ORIENTED_EDGE('',*,*,#7471,.T.);
#10255=ORIENTED_EDGE('',*,*,#7472,.T.);
#10256=ORIENTED_EDGE('',*,*,#7467,.F.);
#10257=ORIENTED_EDGE('',*,*,#7473,.T.);
#10258=ORIENTED_EDGE('',*,*,#7474,.T.);
#10259=ORIENTED_EDGE('',*,*,#7475,.T.);
#10260=ORIENTED_EDGE('',*,*,#7476,.T.);
#10261=ORIENTED_EDGE('',*,*,#7477,.T.);
#10262=ORIENTED_EDGE('',*,*,#7471,.F.);
#10263=ORIENTED_EDGE('',*,*,#7478,.T.);
#10264=ORIENTED_EDGE('',*,*,#7479,.T.);
#10265=ORIENTED_EDGE('',*,*,#7480,.T.);
#10266=ORIENTED_EDGE('',*,*,#7475,.F.);
#10267=ORIENTED_EDGE('',*,*,#7481,.T.);
#10268=ORIENTED_EDGE('',*,*,#7482,.T.);
#10269=ORIENTED_EDGE('',*,*,#7483,.F.);
#10270=ORIENTED_EDGE('',*,*,#7484,.T.);
#10271=ORIENTED_EDGE('',*,*,#7485,.F.);
#10272=ORIENTED_EDGE('',*,*,#7486,.T.);
#10273=ORIENTED_EDGE('',*,*,#7487,.T.);
#10274=ORIENTED_EDGE('',*,*,#7488,.T.);
#10275=ORIENTED_EDGE('',*,*,#7489,.T.);
#10276=ORIENTED_EDGE('',*,*,#7490,.F.);
#10277=ORIENTED_EDGE('',*,*,#7491,.F.);
#10278=ORIENTED_EDGE('',*,*,#7492,.F.);
#10279=ORIENTED_EDGE('',*,*,#7493,.T.);
#10280=ORIENTED_EDGE('',*,*,#7494,.T.);
#10281=ORIENTED_EDGE('',*,*,#7495,.T.);
#10282=ORIENTED_EDGE('',*,*,#7487,.F.);
#10283=ORIENTED_EDGE('',*,*,#7496,.F.);
#10284=ORIENTED_EDGE('',*,*,#7497,.F.);
#10285=ORIENTED_EDGE('',*,*,#7498,.T.);
#10286=ORIENTED_EDGE('',*,*,#7499,.T.);
#10287=ORIENTED_EDGE('',*,*,#7500,.T.);
#10288=ORIENTED_EDGE('',*,*,#7493,.F.);
#10289=ORIENTED_EDGE('',*,*,#7501,.F.);
#10290=ORIENTED_EDGE('',*,*,#7502,.F.);
#10291=ORIENTED_EDGE('',*,*,#7503,.T.);
#10292=ORIENTED_EDGE('',*,*,#7504,.T.);
#10293=ORIENTED_EDGE('',*,*,#7505,.T.);
#10294=ORIENTED_EDGE('',*,*,#7498,.F.);
#10295=ORIENTED_EDGE('',*,*,#7506,.F.);
#10296=ORIENTED_EDGE('',*,*,#7507,.F.);
#10297=ORIENTED_EDGE('',*,*,#7508,.T.);
#10298=ORIENTED_EDGE('',*,*,#7509,.T.);
#10299=ORIENTED_EDGE('',*,*,#7510,.T.);
#10300=ORIENTED_EDGE('',*,*,#7503,.F.);
#10301=ORIENTED_EDGE('',*,*,#7511,.F.);
#10302=ORIENTED_EDGE('',*,*,#7512,.F.);
#10303=ORIENTED_EDGE('',*,*,#7513,.T.);
#10304=ORIENTED_EDGE('',*,*,#7514,.T.);
#10305=ORIENTED_EDGE('',*,*,#7515,.T.);
#10306=ORIENTED_EDGE('',*,*,#7508,.F.);
#10307=ORIENTED_EDGE('',*,*,#7516,.F.);
#10308=ORIENTED_EDGE('',*,*,#7517,.F.);
#10309=ORIENTED_EDGE('',*,*,#7518,.T.);
#10310=ORIENTED_EDGE('',*,*,#7519,.T.);
#10311=ORIENTED_EDGE('',*,*,#7520,.T.);
#10312=ORIENTED_EDGE('',*,*,#7513,.F.);
#10313=ORIENTED_EDGE('',*,*,#7521,.F.);
#10314=ORIENTED_EDGE('',*,*,#7522,.F.);
#10315=ORIENTED_EDGE('',*,*,#7523,.T.);
#10316=ORIENTED_EDGE('',*,*,#7524,.T.);
#10317=ORIENTED_EDGE('',*,*,#7525,.T.);
#10318=ORIENTED_EDGE('',*,*,#7518,.F.);
#10319=ORIENTED_EDGE('',*,*,#7526,.F.);
#10320=ORIENTED_EDGE('',*,*,#7527,.F.);
#10321=ORIENTED_EDGE('',*,*,#7528,.T.);
#10322=ORIENTED_EDGE('',*,*,#7529,.T.);
#10323=ORIENTED_EDGE('',*,*,#7530,.T.);
#10324=ORIENTED_EDGE('',*,*,#7523,.F.);
#10325=ORIENTED_EDGE('',*,*,#7531,.F.);
#10326=ORIENTED_EDGE('',*,*,#7532,.F.);
#10327=ORIENTED_EDGE('',*,*,#7533,.F.);
#10328=ORIENTED_EDGE('',*,*,#7534,.F.);
#10329=ORIENTED_EDGE('',*,*,#7535,.F.);
#10330=ORIENTED_EDGE('',*,*,#7536,.F.);
#10331=ORIENTED_EDGE('',*,*,#7537,.T.);
#10332=ORIENTED_EDGE('',*,*,#7538,.T.);
#10333=ORIENTED_EDGE('',*,*,#7539,.T.);
#10334=ORIENTED_EDGE('',*,*,#7540,.T.);
#10335=ORIENTED_EDGE('',*,*,#7541,.T.);
#10336=ORIENTED_EDGE('',*,*,#7542,.T.);
#10337=ORIENTED_EDGE('',*,*,#7543,.T.);
#10338=ORIENTED_EDGE('',*,*,#7542,.F.);
#10339=ORIENTED_EDGE('',*,*,#7544,.T.);
#10340=ORIENTED_EDGE('',*,*,#7545,.T.);
#10341=ORIENTED_EDGE('',*,*,#7546,.T.);
#10342=ORIENTED_EDGE('',*,*,#7547,.T.);
#10343=ORIENTED_EDGE('',*,*,#7548,.T.);
#10344=ORIENTED_EDGE('',*,*,#7539,.F.);
#10345=ORIENTED_EDGE('',*,*,#7549,.T.);
#10346=ORIENTED_EDGE('',*,*,#7550,.T.);
#10347=ORIENTED_EDGE('',*,*,#7551,.T.);
#10348=ORIENTED_EDGE('',*,*,#7546,.F.);
#10349=ORIENTED_EDGE('',*,*,#7552,.T.);
#10350=ORIENTED_EDGE('',*,*,#7553,.T.);
#10351=ORIENTED_EDGE('',*,*,#7554,.T.);
#10352=ORIENTED_EDGE('',*,*,#7555,.T.);
#10353=ORIENTED_EDGE('',*,*,#7556,.T.);
#10354=ORIENTED_EDGE('',*,*,#7550,.F.);
#10355=ORIENTED_EDGE('',*,*,#7557,.T.);
#10356=ORIENTED_EDGE('',*,*,#7558,.T.);
#10357=ORIENTED_EDGE('',*,*,#7559,.T.);
#10358=ORIENTED_EDGE('',*,*,#7554,.F.);
#10359=ORIENTED_EDGE('',*,*,#7560,.T.);
#10360=ORIENTED_EDGE('',*,*,#7561,.T.);
#10361=ORIENTED_EDGE('',*,*,#7562,.T.);
#10362=ORIENTED_EDGE('',*,*,#7563,.T.);
#10363=ORIENTED_EDGE('',*,*,#7564,.T.);
#10364=ORIENTED_EDGE('',*,*,#7558,.F.);
#10365=ORIENTED_EDGE('',*,*,#7565,.T.);
#10366=ORIENTED_EDGE('',*,*,#7566,.T.);
#10367=ORIENTED_EDGE('',*,*,#7567,.T.);
#10368=ORIENTED_EDGE('',*,*,#7562,.F.);
#10369=ORIENTED_EDGE('',*,*,#7568,.T.);
#10370=ORIENTED_EDGE('',*,*,#7569,.T.);
#10371=ORIENTED_EDGE('',*,*,#7570,.T.);
#10372=ORIENTED_EDGE('',*,*,#7571,.T.);
#10373=ORIENTED_EDGE('',*,*,#7572,.T.);
#10374=ORIENTED_EDGE('',*,*,#7566,.F.);
#10375=ORIENTED_EDGE('',*,*,#7573,.T.);
#10376=ORIENTED_EDGE('',*,*,#7574,.T.);
#10377=ORIENTED_EDGE('',*,*,#7575,.T.);
#10378=ORIENTED_EDGE('',*,*,#7570,.F.);
#10379=ORIENTED_EDGE('',*,*,#7576,.T.);
#10380=ORIENTED_EDGE('',*,*,#7577,.T.);
#10381=ORIENTED_EDGE('',*,*,#7578,.F.);
#10382=ORIENTED_EDGE('',*,*,#7579,.T.);
#10383=ORIENTED_EDGE('',*,*,#7580,.F.);
#10384=ORIENTED_EDGE('',*,*,#7581,.T.);
#10385=ORIENTED_EDGE('',*,*,#7582,.T.);
#10386=ORIENTED_EDGE('',*,*,#7583,.T.);
#10387=ORIENTED_EDGE('',*,*,#7584,.T.);
#10388=ORIENTED_EDGE('',*,*,#7585,.F.);
#10389=ORIENTED_EDGE('',*,*,#7586,.F.);
#10390=ORIENTED_EDGE('',*,*,#7587,.F.);
#10391=ORIENTED_EDGE('',*,*,#7588,.T.);
#10392=ORIENTED_EDGE('',*,*,#7589,.T.);
#10393=ORIENTED_EDGE('',*,*,#7590,.T.);
#10394=ORIENTED_EDGE('',*,*,#7582,.F.);
#10395=ORIENTED_EDGE('',*,*,#7591,.F.);
#10396=ORIENTED_EDGE('',*,*,#7592,.F.);
#10397=ORIENTED_EDGE('',*,*,#7593,.T.);
#10398=ORIENTED_EDGE('',*,*,#7594,.T.);
#10399=ORIENTED_EDGE('',*,*,#7595,.T.);
#10400=ORIENTED_EDGE('',*,*,#7588,.F.);
#10401=ORIENTED_EDGE('',*,*,#7596,.F.);
#10402=ORIENTED_EDGE('',*,*,#7597,.F.);
#10403=ORIENTED_EDGE('',*,*,#7598,.T.);
#10404=ORIENTED_EDGE('',*,*,#7599,.T.);
#10405=ORIENTED_EDGE('',*,*,#7600,.T.);
#10406=ORIENTED_EDGE('',*,*,#7593,.F.);
#10407=ORIENTED_EDGE('',*,*,#7601,.F.);
#10408=ORIENTED_EDGE('',*,*,#7602,.F.);
#10409=ORIENTED_EDGE('',*,*,#7603,.T.);
#10410=ORIENTED_EDGE('',*,*,#7604,.T.);
#10411=ORIENTED_EDGE('',*,*,#7605,.T.);
#10412=ORIENTED_EDGE('',*,*,#7598,.F.);
#10413=ORIENTED_EDGE('',*,*,#7606,.F.);
#10414=ORIENTED_EDGE('',*,*,#7607,.F.);
#10415=ORIENTED_EDGE('',*,*,#7608,.T.);
#10416=ORIENTED_EDGE('',*,*,#7609,.T.);
#10417=ORIENTED_EDGE('',*,*,#7610,.T.);
#10418=ORIENTED_EDGE('',*,*,#7603,.F.);
#10419=ORIENTED_EDGE('',*,*,#7611,.F.);
#10420=ORIENTED_EDGE('',*,*,#7612,.F.);
#10421=ORIENTED_EDGE('',*,*,#7613,.T.);
#10422=ORIENTED_EDGE('',*,*,#7614,.T.);
#10423=ORIENTED_EDGE('',*,*,#7615,.T.);
#10424=ORIENTED_EDGE('',*,*,#7608,.F.);
#10425=ORIENTED_EDGE('',*,*,#7616,.F.);
#10426=ORIENTED_EDGE('',*,*,#7617,.F.);
#10427=ORIENTED_EDGE('',*,*,#7618,.T.);
#10428=ORIENTED_EDGE('',*,*,#7619,.T.);
#10429=ORIENTED_EDGE('',*,*,#7620,.T.);
#10430=ORIENTED_EDGE('',*,*,#7613,.F.);
#10431=ORIENTED_EDGE('',*,*,#7621,.F.);
#10432=ORIENTED_EDGE('',*,*,#7622,.F.);
#10433=ORIENTED_EDGE('',*,*,#7623,.T.);
#10434=ORIENTED_EDGE('',*,*,#7624,.T.);
#10435=ORIENTED_EDGE('',*,*,#7625,.T.);
#10436=ORIENTED_EDGE('',*,*,#7618,.F.);
#10437=ORIENTED_EDGE('',*,*,#7626,.F.);
#10438=ORIENTED_EDGE('',*,*,#7627,.F.);
#10439=ORIENTED_EDGE('',*,*,#7628,.F.);
#10440=ORIENTED_EDGE('',*,*,#7629,.F.);
#10441=ORIENTED_EDGE('',*,*,#7630,.F.);
#10442=ORIENTED_EDGE('',*,*,#7631,.F.);
#10443=ORIENTED_EDGE('',*,*,#7632,.T.);
#10444=ORIENTED_EDGE('',*,*,#7633,.T.);
#10445=ORIENTED_EDGE('',*,*,#7634,.T.);
#10446=ORIENTED_EDGE('',*,*,#7635,.T.);
#10447=ORIENTED_EDGE('',*,*,#7636,.T.);
#10448=ORIENTED_EDGE('',*,*,#7637,.T.);
#10449=ORIENTED_EDGE('',*,*,#7638,.T.);
#10450=ORIENTED_EDGE('',*,*,#7637,.F.);
#10451=ORIENTED_EDGE('',*,*,#7639,.T.);
#10452=ORIENTED_EDGE('',*,*,#7640,.T.);
#10453=ORIENTED_EDGE('',*,*,#7641,.T.);
#10454=ORIENTED_EDGE('',*,*,#7642,.T.);
#10455=ORIENTED_EDGE('',*,*,#7643,.T.);
#10456=ORIENTED_EDGE('',*,*,#7634,.F.);
#10457=ORIENTED_EDGE('',*,*,#7644,.T.);
#10458=ORIENTED_EDGE('',*,*,#7645,.T.);
#10459=ORIENTED_EDGE('',*,*,#7646,.T.);
#10460=ORIENTED_EDGE('',*,*,#7641,.F.);
#10461=ORIENTED_EDGE('',*,*,#7647,.T.);
#10462=ORIENTED_EDGE('',*,*,#7648,.T.);
#10463=ORIENTED_EDGE('',*,*,#7649,.T.);
#10464=ORIENTED_EDGE('',*,*,#7650,.T.);
#10465=ORIENTED_EDGE('',*,*,#7651,.T.);
#10466=ORIENTED_EDGE('',*,*,#7645,.F.);
#10467=ORIENTED_EDGE('',*,*,#7652,.T.);
#10468=ORIENTED_EDGE('',*,*,#7653,.T.);
#10469=ORIENTED_EDGE('',*,*,#7654,.T.);
#10470=ORIENTED_EDGE('',*,*,#7649,.F.);
#10471=ORIENTED_EDGE('',*,*,#7655,.T.);
#10472=ORIENTED_EDGE('',*,*,#7656,.T.);
#10473=ORIENTED_EDGE('',*,*,#7657,.T.);
#10474=ORIENTED_EDGE('',*,*,#7658,.T.);
#10475=ORIENTED_EDGE('',*,*,#7659,.T.);
#10476=ORIENTED_EDGE('',*,*,#7653,.F.);
#10477=ORIENTED_EDGE('',*,*,#7660,.T.);
#10478=ORIENTED_EDGE('',*,*,#7661,.T.);
#10479=ORIENTED_EDGE('',*,*,#7662,.T.);
#10480=ORIENTED_EDGE('',*,*,#7657,.F.);
#10481=ORIENTED_EDGE('',*,*,#7663,.T.);
#10482=ORIENTED_EDGE('',*,*,#7664,.T.);
#10483=ORIENTED_EDGE('',*,*,#7665,.T.);
#10484=ORIENTED_EDGE('',*,*,#7666,.T.);
#10485=ORIENTED_EDGE('',*,*,#7667,.T.);
#10486=ORIENTED_EDGE('',*,*,#7661,.F.);
#10487=ORIENTED_EDGE('',*,*,#7668,.T.);
#10488=ORIENTED_EDGE('',*,*,#7669,.T.);
#10489=ORIENTED_EDGE('',*,*,#7670,.T.);
#10490=ORIENTED_EDGE('',*,*,#7665,.F.);
#10491=ORIENTED_EDGE('',*,*,#7671,.T.);
#10492=ORIENTED_EDGE('',*,*,#7672,.T.);
#10493=ORIENTED_EDGE('',*,*,#7673,.F.);
#10494=ORIENTED_EDGE('',*,*,#7674,.T.);
#10495=ORIENTED_EDGE('',*,*,#7675,.F.);
#10496=ORIENTED_EDGE('',*,*,#7676,.T.);
#10497=ORIENTED_EDGE('',*,*,#7677,.T.);
#10498=ORIENTED_EDGE('',*,*,#7678,.T.);
#10499=ORIENTED_EDGE('',*,*,#7679,.T.);
#10500=ORIENTED_EDGE('',*,*,#7680,.F.);
#10501=ORIENTED_EDGE('',*,*,#7681,.F.);
#10502=ORIENTED_EDGE('',*,*,#7682,.F.);
#10503=ORIENTED_EDGE('',*,*,#7683,.T.);
#10504=ORIENTED_EDGE('',*,*,#7684,.T.);
#10505=ORIENTED_EDGE('',*,*,#7685,.T.);
#10506=ORIENTED_EDGE('',*,*,#7677,.F.);
#10507=ORIENTED_EDGE('',*,*,#7686,.F.);
#10508=ORIENTED_EDGE('',*,*,#7687,.F.);
#10509=ORIENTED_EDGE('',*,*,#7688,.T.);
#10510=ORIENTED_EDGE('',*,*,#7689,.T.);
#10511=ORIENTED_EDGE('',*,*,#7690,.T.);
#10512=ORIENTED_EDGE('',*,*,#7683,.F.);
#10513=ORIENTED_EDGE('',*,*,#7691,.F.);
#10514=ORIENTED_EDGE('',*,*,#7692,.F.);
#10515=ORIENTED_EDGE('',*,*,#7693,.T.);
#10516=ORIENTED_EDGE('',*,*,#7694,.T.);
#10517=ORIENTED_EDGE('',*,*,#7695,.T.);
#10518=ORIENTED_EDGE('',*,*,#7688,.F.);
#10519=ORIENTED_EDGE('',*,*,#7696,.F.);
#10520=ORIENTED_EDGE('',*,*,#7697,.F.);
#10521=ORIENTED_EDGE('',*,*,#7698,.T.);
#10522=ORIENTED_EDGE('',*,*,#7699,.T.);
#10523=ORIENTED_EDGE('',*,*,#7700,.T.);
#10524=ORIENTED_EDGE('',*,*,#7693,.F.);
#10525=ORIENTED_EDGE('',*,*,#7701,.F.);
#10526=ORIENTED_EDGE('',*,*,#7702,.F.);
#10527=ORIENTED_EDGE('',*,*,#7703,.T.);
#10528=ORIENTED_EDGE('',*,*,#7704,.T.);
#10529=ORIENTED_EDGE('',*,*,#7705,.T.);
#10530=ORIENTED_EDGE('',*,*,#7698,.F.);
#10531=ORIENTED_EDGE('',*,*,#7706,.F.);
#10532=ORIENTED_EDGE('',*,*,#7707,.F.);
#10533=ORIENTED_EDGE('',*,*,#7708,.T.);
#10534=ORIENTED_EDGE('',*,*,#7709,.T.);
#10535=ORIENTED_EDGE('',*,*,#7710,.T.);
#10536=ORIENTED_EDGE('',*,*,#7703,.F.);
#10537=ORIENTED_EDGE('',*,*,#7711,.F.);
#10538=ORIENTED_EDGE('',*,*,#7712,.F.);
#10539=ORIENTED_EDGE('',*,*,#7713,.T.);
#10540=ORIENTED_EDGE('',*,*,#7714,.T.);
#10541=ORIENTED_EDGE('',*,*,#7715,.T.);
#10542=ORIENTED_EDGE('',*,*,#7708,.F.);
#10543=ORIENTED_EDGE('',*,*,#7716,.F.);
#10544=ORIENTED_EDGE('',*,*,#7717,.F.);
#10545=ORIENTED_EDGE('',*,*,#7718,.T.);
#10546=ORIENTED_EDGE('',*,*,#7719,.T.);
#10547=ORIENTED_EDGE('',*,*,#7720,.T.);
#10548=ORIENTED_EDGE('',*,*,#7713,.F.);
#10549=ORIENTED_EDGE('',*,*,#7721,.F.);
#10550=ORIENTED_EDGE('',*,*,#7722,.F.);
#10551=ORIENTED_EDGE('',*,*,#7723,.F.);
#10552=ORIENTED_EDGE('',*,*,#7724,.F.);
#10553=ORIENTED_EDGE('',*,*,#7725,.F.);
#10554=ORIENTED_EDGE('',*,*,#7726,.F.);
#10555=ORIENTED_EDGE('',*,*,#7727,.T.);
#10556=ORIENTED_EDGE('',*,*,#7728,.T.);
#10557=ORIENTED_EDGE('',*,*,#7729,.T.);
#10558=ORIENTED_EDGE('',*,*,#7730,.T.);
#10559=ORIENTED_EDGE('',*,*,#7731,.T.);
#10560=ORIENTED_EDGE('',*,*,#7732,.T.);
#10561=ORIENTED_EDGE('',*,*,#7733,.T.);
#10562=ORIENTED_EDGE('',*,*,#7732,.F.);
#10563=ORIENTED_EDGE('',*,*,#7734,.T.);
#10564=ORIENTED_EDGE('',*,*,#7735,.T.);
#10565=ORIENTED_EDGE('',*,*,#7736,.T.);
#10566=ORIENTED_EDGE('',*,*,#7737,.T.);
#10567=ORIENTED_EDGE('',*,*,#7738,.T.);
#10568=ORIENTED_EDGE('',*,*,#7729,.F.);
#10569=ORIENTED_EDGE('',*,*,#7739,.T.);
#10570=ORIENTED_EDGE('',*,*,#7740,.T.);
#10571=ORIENTED_EDGE('',*,*,#7741,.T.);
#10572=ORIENTED_EDGE('',*,*,#7736,.F.);
#10573=ORIENTED_EDGE('',*,*,#7742,.T.);
#10574=ORIENTED_EDGE('',*,*,#7743,.T.);
#10575=ORIENTED_EDGE('',*,*,#7744,.T.);
#10576=ORIENTED_EDGE('',*,*,#7745,.T.);
#10577=ORIENTED_EDGE('',*,*,#7746,.T.);
#10578=ORIENTED_EDGE('',*,*,#7740,.F.);
#10579=ORIENTED_EDGE('',*,*,#7747,.T.);
#10580=ORIENTED_EDGE('',*,*,#7748,.T.);
#10581=ORIENTED_EDGE('',*,*,#7749,.T.);
#10582=ORIENTED_EDGE('',*,*,#7744,.F.);
#10583=ORIENTED_EDGE('',*,*,#7750,.T.);
#10584=ORIENTED_EDGE('',*,*,#7751,.T.);
#10585=ORIENTED_EDGE('',*,*,#7752,.T.);
#10586=ORIENTED_EDGE('',*,*,#7753,.T.);
#10587=ORIENTED_EDGE('',*,*,#7754,.T.);
#10588=ORIENTED_EDGE('',*,*,#7748,.F.);
#10589=ORIENTED_EDGE('',*,*,#7755,.T.);
#10590=ORIENTED_EDGE('',*,*,#7756,.T.);
#10591=ORIENTED_EDGE('',*,*,#7757,.T.);
#10592=ORIENTED_EDGE('',*,*,#7752,.F.);
#10593=ORIENTED_EDGE('',*,*,#7758,.T.);
#10594=ORIENTED_EDGE('',*,*,#7759,.T.);
#10595=ORIENTED_EDGE('',*,*,#7760,.T.);
#10596=ORIENTED_EDGE('',*,*,#7761,.T.);
#10597=ORIENTED_EDGE('',*,*,#7762,.T.);
#10598=ORIENTED_EDGE('',*,*,#7756,.F.);
#10599=ORIENTED_EDGE('',*,*,#7763,.T.);
#10600=ORIENTED_EDGE('',*,*,#7764,.T.);
#10601=ORIENTED_EDGE('',*,*,#7765,.T.);
#10602=ORIENTED_EDGE('',*,*,#7760,.F.);
#10603=ORIENTED_EDGE('',*,*,#7766,.T.);
#10604=ORIENTED_EDGE('',*,*,#7767,.T.);
#10605=ORIENTED_EDGE('',*,*,#7768,.F.);
#10606=ORIENTED_EDGE('',*,*,#7769,.T.);
#10607=ORIENTED_EDGE('',*,*,#7770,.F.);
#10608=ORIENTED_EDGE('',*,*,#7771,.T.);
#10609=ORIENTED_EDGE('',*,*,#7768,.T.);
#10610=ORIENTED_EDGE('',*,*,#7772,.T.);
#10611=ORIENTED_EDGE('',*,*,#7773,.T.);
#10612=ORIENTED_EDGE('',*,*,#7764,.F.);
#10613=ORIENTED_EDGE('',*,*,#7774,.T.);
#10614=ORIENTED_EDGE('',*,*,#7775,.T.);
#10615=ORIENTED_EDGE('',*,*,#7723,.T.);
#10616=ORIENTED_EDGE('',*,*,#7776,.T.);
#10617=ORIENTED_EDGE('',*,*,#7777,.T.);
#10618=ORIENTED_EDGE('',*,*,#7718,.F.);
#10619=ORIENTED_EDGE('',*,*,#7778,.F.);
#10620=ORIENTED_EDGE('',*,*,#7779,.F.);
#10621=ORIENTED_EDGE('',*,*,#7673,.T.);
#10622=ORIENTED_EDGE('',*,*,#7780,.T.);
#10623=ORIENTED_EDGE('',*,*,#7781,.T.);
#10624=ORIENTED_EDGE('',*,*,#7669,.F.);
#10625=ORIENTED_EDGE('',*,*,#7782,.T.);
#10626=ORIENTED_EDGE('',*,*,#7783,.T.);
#10627=ORIENTED_EDGE('',*,*,#7628,.T.);
#10628=ORIENTED_EDGE('',*,*,#7784,.T.);
#10629=ORIENTED_EDGE('',*,*,#7785,.T.);
#10630=ORIENTED_EDGE('',*,*,#7623,.F.);
#10631=ORIENTED_EDGE('',*,*,#7786,.F.);
#10632=ORIENTED_EDGE('',*,*,#7787,.F.);
#10633=ORIENTED_EDGE('',*,*,#7578,.T.);
#10634=ORIENTED_EDGE('',*,*,#7788,.T.);
#10635=ORIENTED_EDGE('',*,*,#7789,.T.);
#10636=ORIENTED_EDGE('',*,*,#7574,.F.);
#10637=ORIENTED_EDGE('',*,*,#7790,.T.);
#10638=ORIENTED_EDGE('',*,*,#7791,.T.);
#10639=ORIENTED_EDGE('',*,*,#7533,.T.);
#10640=ORIENTED_EDGE('',*,*,#7792,.T.);
#10641=ORIENTED_EDGE('',*,*,#7793,.T.);
#10642=ORIENTED_EDGE('',*,*,#7528,.F.);
#10643=ORIENTED_EDGE('',*,*,#7794,.F.);
#10644=ORIENTED_EDGE('',*,*,#7795,.F.);
#10645=ORIENTED_EDGE('',*,*,#7483,.T.);
#10646=ORIENTED_EDGE('',*,*,#7796,.T.);
#10647=ORIENTED_EDGE('',*,*,#7797,.T.);
#10648=ORIENTED_EDGE('',*,*,#7479,.F.);
#10649=ORIENTED_EDGE('',*,*,#7798,.T.);
#10650=ORIENTED_EDGE('',*,*,#7799,.T.);
#10651=ORIENTED_EDGE('',*,*,#7438,.T.);
#10652=ORIENTED_EDGE('',*,*,#7800,.T.);
#10653=ORIENTED_EDGE('',*,*,#7801,.T.);
#10654=ORIENTED_EDGE('',*,*,#7433,.F.);
#10655=ORIENTED_EDGE('',*,*,#7802,.F.);
#10656=ORIENTED_EDGE('',*,*,#7803,.F.);
#10657=ORIENTED_EDGE('',*,*,#7446,.F.);
#10658=ORIENTED_EDGE('',*,*,#7804,.T.);
#10659=ORIENTED_EDGE('',*,*,#7395,.T.);
#10660=ORIENTED_EDGE('',*,*,#7805,.T.);
#10661=ORIENTED_EDGE('',*,*,#7449,.F.);
#10662=ORIENTED_EDGE('',*,*,#7805,.F.);
#10663=ORIENTED_EDGE('',*,*,#7394,.F.);
#10664=ORIENTED_EDGE('',*,*,#7393,.F.);
#10665=ORIENTED_EDGE('',*,*,#7400,.F.);
#10666=ORIENTED_EDGE('',*,*,#7399,.F.);
#10667=ORIENTED_EDGE('',*,*,#7405,.F.);
#10668=ORIENTED_EDGE('',*,*,#7404,.F.);
#10669=ORIENTED_EDGE('',*,*,#7410,.F.);
#10670=ORIENTED_EDGE('',*,*,#7409,.F.);
#10671=ORIENTED_EDGE('',*,*,#7415,.F.);
#10672=ORIENTED_EDGE('',*,*,#7414,.F.);
#10673=ORIENTED_EDGE('',*,*,#7420,.F.);
#10674=ORIENTED_EDGE('',*,*,#7419,.F.);
#10675=ORIENTED_EDGE('',*,*,#7425,.F.);
#10676=ORIENTED_EDGE('',*,*,#7424,.F.);
#10677=ORIENTED_EDGE('',*,*,#7430,.F.);
#10678=ORIENTED_EDGE('',*,*,#7429,.F.);
#10679=ORIENTED_EDGE('',*,*,#7435,.F.);
#10680=ORIENTED_EDGE('',*,*,#7434,.F.);
#10681=ORIENTED_EDGE('',*,*,#7801,.F.);
#10682=ORIENTED_EDGE('',*,*,#7800,.F.);
#10683=ORIENTED_EDGE('',*,*,#7443,.F.);
#10684=ORIENTED_EDGE('',*,*,#7442,.F.);
#10685=ORIENTED_EDGE('',*,*,#7806,.F.);
#10686=ORIENTED_EDGE('',*,*,#7484,.F.);
#10687=ORIENTED_EDGE('',*,*,#7799,.F.);
#10688=ORIENTED_EDGE('',*,*,#7798,.F.);
#10689=ORIENTED_EDGE('',*,*,#7482,.F.);
#10690=ORIENTED_EDGE('',*,*,#7481,.F.);
#10691=ORIENTED_EDGE('',*,*,#7478,.F.);
#10692=ORIENTED_EDGE('',*,*,#7474,.F.);
#10693=ORIENTED_EDGE('',*,*,#7473,.F.);
#10694=ORIENTED_EDGE('',*,*,#7470,.F.);
#10695=ORIENTED_EDGE('',*,*,#7466,.F.);
#10696=ORIENTED_EDGE('',*,*,#7465,.F.);
#10697=ORIENTED_EDGE('',*,*,#7462,.F.);
#10698=ORIENTED_EDGE('',*,*,#7458,.F.);
#10699=ORIENTED_EDGE('',*,*,#7457,.F.);
#10700=ORIENTED_EDGE('',*,*,#7454,.F.);
#10701=ORIENTED_EDGE('',*,*,#7450,.F.);
#10702=ORIENTED_EDGE('',*,*,#7804,.F.);
#10703=ORIENTED_EDGE('',*,*,#7445,.F.);
#10704=ORIENTED_EDGE('',*,*,#7453,.F.);
#10705=ORIENTED_EDGE('',*,*,#7452,.F.);
#10706=ORIENTED_EDGE('',*,*,#7456,.F.);
#10707=ORIENTED_EDGE('',*,*,#7461,.F.);
#10708=ORIENTED_EDGE('',*,*,#7460,.F.);
#10709=ORIENTED_EDGE('',*,*,#7464,.F.);
#10710=ORIENTED_EDGE('',*,*,#7469,.F.);
#10711=ORIENTED_EDGE('',*,*,#7468,.F.);
#10712=ORIENTED_EDGE('',*,*,#7472,.F.);
#10713=ORIENTED_EDGE('',*,*,#7477,.F.);
#10714=ORIENTED_EDGE('',*,*,#7476,.F.);
#10715=ORIENTED_EDGE('',*,*,#7480,.F.);
#10716=ORIENTED_EDGE('',*,*,#7797,.F.);
#10717=ORIENTED_EDGE('',*,*,#7796,.F.);
#10718=ORIENTED_EDGE('',*,*,#7486,.F.);
#10719=ORIENTED_EDGE('',*,*,#7807,.F.);
#10720=ORIENTED_EDGE('',*,*,#7808,.F.);
#10721=ORIENTED_EDGE('',*,*,#7440,.T.);
#10722=ORIENTED_EDGE('',*,*,#7439,.T.);
#10723=ORIENTED_EDGE('',*,*,#7803,.T.);
#10724=ORIENTED_EDGE('',*,*,#7802,.T.);
#10725=ORIENTED_EDGE('',*,*,#7437,.T.);
#10726=ORIENTED_EDGE('',*,*,#7436,.T.);
#10727=ORIENTED_EDGE('',*,*,#7432,.T.);
#10728=ORIENTED_EDGE('',*,*,#7431,.T.);
#10729=ORIENTED_EDGE('',*,*,#7427,.T.);
#10730=ORIENTED_EDGE('',*,*,#7426,.T.);
#10731=ORIENTED_EDGE('',*,*,#7422,.T.);
#10732=ORIENTED_EDGE('',*,*,#7421,.T.);
#10733=ORIENTED_EDGE('',*,*,#7417,.T.);
#10734=ORIENTED_EDGE('',*,*,#7416,.T.);
#10735=ORIENTED_EDGE('',*,*,#7412,.T.);
#10736=ORIENTED_EDGE('',*,*,#7411,.T.);
#10737=ORIENTED_EDGE('',*,*,#7407,.T.);
#10738=ORIENTED_EDGE('',*,*,#7406,.T.);
#10739=ORIENTED_EDGE('',*,*,#7402,.T.);
#10740=ORIENTED_EDGE('',*,*,#7401,.T.);
#10741=ORIENTED_EDGE('',*,*,#7397,.T.);
#10742=ORIENTED_EDGE('',*,*,#7396,.T.);
#10743=ORIENTED_EDGE('',*,*,#7541,.F.);
#10744=ORIENTED_EDGE('',*,*,#7809,.T.);
#10745=ORIENTED_EDGE('',*,*,#7490,.T.);
#10746=ORIENTED_EDGE('',*,*,#7810,.T.);
#10747=ORIENTED_EDGE('',*,*,#7544,.F.);
#10748=ORIENTED_EDGE('',*,*,#7810,.F.);
#10749=ORIENTED_EDGE('',*,*,#7489,.F.);
#10750=ORIENTED_EDGE('',*,*,#7488,.F.);
#10751=ORIENTED_EDGE('',*,*,#7495,.F.);
#10752=ORIENTED_EDGE('',*,*,#7494,.F.);
#10753=ORIENTED_EDGE('',*,*,#7500,.F.);
#10754=ORIENTED_EDGE('',*,*,#7499,.F.);
#10755=ORIENTED_EDGE('',*,*,#7505,.F.);
#10756=ORIENTED_EDGE('',*,*,#7504,.F.);
#10757=ORIENTED_EDGE('',*,*,#7510,.F.);
#10758=ORIENTED_EDGE('',*,*,#7509,.F.);
#10759=ORIENTED_EDGE('',*,*,#7515,.F.);
#10760=ORIENTED_EDGE('',*,*,#7514,.F.);
#10761=ORIENTED_EDGE('',*,*,#7520,.F.);
#10762=ORIENTED_EDGE('',*,*,#7519,.F.);
#10763=ORIENTED_EDGE('',*,*,#7525,.F.);
#10764=ORIENTED_EDGE('',*,*,#7524,.F.);
#10765=ORIENTED_EDGE('',*,*,#7530,.F.);
#10766=ORIENTED_EDGE('',*,*,#7529,.F.);
#10767=ORIENTED_EDGE('',*,*,#7793,.F.);
#10768=ORIENTED_EDGE('',*,*,#7792,.F.);
#10769=ORIENTED_EDGE('',*,*,#7538,.F.);
#10770=ORIENTED_EDGE('',*,*,#7537,.F.);
#10771=ORIENTED_EDGE('',*,*,#7811,.F.);
#10772=ORIENTED_EDGE('',*,*,#7579,.F.);
#10773=ORIENTED_EDGE('',*,*,#7791,.F.);
#10774=ORIENTED_EDGE('',*,*,#7790,.F.);
#10775=ORIENTED_EDGE('',*,*,#7577,.F.);
#10776=ORIENTED_EDGE('',*,*,#7576,.F.);
#10777=ORIENTED_EDGE('',*,*,#7573,.F.);
#10778=ORIENTED_EDGE('',*,*,#7569,.F.);
#10779=ORIENTED_EDGE('',*,*,#7568,.F.);
#10780=ORIENTED_EDGE('',*,*,#7565,.F.);
#10781=ORIENTED_EDGE('',*,*,#7561,.F.);
#10782=ORIENTED_EDGE('',*,*,#7560,.F.);
#10783=ORIENTED_EDGE('',*,*,#7557,.F.);
#10784=ORIENTED_EDGE('',*,*,#7553,.F.);
#10785=ORIENTED_EDGE('',*,*,#7552,.F.);
#10786=ORIENTED_EDGE('',*,*,#7549,.F.);
#10787=ORIENTED_EDGE('',*,*,#7545,.F.);
#10788=ORIENTED_EDGE('',*,*,#7809,.F.);
#10789=ORIENTED_EDGE('',*,*,#7540,.F.);
#10790=ORIENTED_EDGE('',*,*,#7548,.F.);
#10791=ORIENTED_EDGE('',*,*,#7547,.F.);
#10792=ORIENTED_EDGE('',*,*,#7551,.F.);
#10793=ORIENTED_EDGE('',*,*,#7556,.F.);
#10794=ORIENTED_EDGE('',*,*,#7555,.F.);
#10795=ORIENTED_EDGE('',*,*,#7559,.F.);
#10796=ORIENTED_EDGE('',*,*,#7564,.F.);
#10797=ORIENTED_EDGE('',*,*,#7563,.F.);
#10798=ORIENTED_EDGE('',*,*,#7567,.F.);
#10799=ORIENTED_EDGE('',*,*,#7572,.F.);
#10800=ORIENTED_EDGE('',*,*,#7571,.F.);
#10801=ORIENTED_EDGE('',*,*,#7575,.F.);
#10802=ORIENTED_EDGE('',*,*,#7789,.F.);
#10803=ORIENTED_EDGE('',*,*,#7788,.F.);
#10804=ORIENTED_EDGE('',*,*,#7581,.F.);
#10805=ORIENTED_EDGE('',*,*,#7812,.F.);
#10806=ORIENTED_EDGE('',*,*,#7813,.F.);
#10807=ORIENTED_EDGE('',*,*,#7535,.T.);
#10808=ORIENTED_EDGE('',*,*,#7534,.T.);
#10809=ORIENTED_EDGE('',*,*,#7795,.T.);
#10810=ORIENTED_EDGE('',*,*,#7794,.T.);
#10811=ORIENTED_EDGE('',*,*,#7532,.T.);
#10812=ORIENTED_EDGE('',*,*,#7531,.T.);
#10813=ORIENTED_EDGE('',*,*,#7527,.T.);
#10814=ORIENTED_EDGE('',*,*,#7526,.T.);
#10815=ORIENTED_EDGE('',*,*,#7522,.T.);
#10816=ORIENTED_EDGE('',*,*,#7521,.T.);
#10817=ORIENTED_EDGE('',*,*,#7517,.T.);
#10818=ORIENTED_EDGE('',*,*,#7516,.T.);
#10819=ORIENTED_EDGE('',*,*,#7512,.T.);
#10820=ORIENTED_EDGE('',*,*,#7511,.T.);
#10821=ORIENTED_EDGE('',*,*,#7507,.T.);
#10822=ORIENTED_EDGE('',*,*,#7506,.T.);
#10823=ORIENTED_EDGE('',*,*,#7502,.T.);
#10824=ORIENTED_EDGE('',*,*,#7501,.T.);
#10825=ORIENTED_EDGE('',*,*,#7497,.T.);
#10826=ORIENTED_EDGE('',*,*,#7496,.T.);
#10827=ORIENTED_EDGE('',*,*,#7492,.T.);
#10828=ORIENTED_EDGE('',*,*,#7491,.T.);
#10829=ORIENTED_EDGE('',*,*,#7636,.F.);
#10830=ORIENTED_EDGE('',*,*,#7814,.T.);
#10831=ORIENTED_EDGE('',*,*,#7585,.T.);
#10832=ORIENTED_EDGE('',*,*,#7815,.T.);
#10833=ORIENTED_EDGE('',*,*,#7639,.F.);
#10834=ORIENTED_EDGE('',*,*,#7815,.F.);
#10835=ORIENTED_EDGE('',*,*,#7584,.F.);
#10836=ORIENTED_EDGE('',*,*,#7583,.F.);
#10837=ORIENTED_EDGE('',*,*,#7590,.F.);
#10838=ORIENTED_EDGE('',*,*,#7589,.F.);
#10839=ORIENTED_EDGE('',*,*,#7595,.F.);
#10840=ORIENTED_EDGE('',*,*,#7594,.F.);
#10841=ORIENTED_EDGE('',*,*,#7600,.F.);
#10842=ORIENTED_EDGE('',*,*,#7599,.F.);
#10843=ORIENTED_EDGE('',*,*,#7605,.F.);
#10844=ORIENTED_EDGE('',*,*,#7604,.F.);
#10845=ORIENTED_EDGE('',*,*,#7610,.F.);
#10846=ORIENTED_EDGE('',*,*,#7609,.F.);
#10847=ORIENTED_EDGE('',*,*,#7615,.F.);
#10848=ORIENTED_EDGE('',*,*,#7614,.F.);
#10849=ORIENTED_EDGE('',*,*,#7620,.F.);
#10850=ORIENTED_EDGE('',*,*,#7619,.F.);
#10851=ORIENTED_EDGE('',*,*,#7625,.F.);
#10852=ORIENTED_EDGE('',*,*,#7624,.F.);
#10853=ORIENTED_EDGE('',*,*,#7785,.F.);
#10854=ORIENTED_EDGE('',*,*,#7784,.F.);
#10855=ORIENTED_EDGE('',*,*,#7633,.F.);
#10856=ORIENTED_EDGE('',*,*,#7632,.F.);
#10857=ORIENTED_EDGE('',*,*,#7816,.F.);
#10858=ORIENTED_EDGE('',*,*,#7674,.F.);
#10859=ORIENTED_EDGE('',*,*,#7783,.F.);
#10860=ORIENTED_EDGE('',*,*,#7782,.F.);
#10861=ORIENTED_EDGE('',*,*,#7672,.F.);
#10862=ORIENTED_EDGE('',*,*,#7671,.F.);
#10863=ORIENTED_EDGE('',*,*,#7668,.F.);
#10864=ORIENTED_EDGE('',*,*,#7664,.F.);
#10865=ORIENTED_EDGE('',*,*,#7663,.F.);
#10866=ORIENTED_EDGE('',*,*,#7660,.F.);
#10867=ORIENTED_EDGE('',*,*,#7656,.F.);
#10868=ORIENTED_EDGE('',*,*,#7655,.F.);
#10869=ORIENTED_EDGE('',*,*,#7652,.F.);
#10870=ORIENTED_EDGE('',*,*,#7648,.F.);
#10871=ORIENTED_EDGE('',*,*,#7647,.F.);
#10872=ORIENTED_EDGE('',*,*,#7644,.F.);
#10873=ORIENTED_EDGE('',*,*,#7640,.F.);
#10874=ORIENTED_EDGE('',*,*,#7814,.F.);
#10875=ORIENTED_EDGE('',*,*,#7635,.F.);
#10876=ORIENTED_EDGE('',*,*,#7643,.F.);
#10877=ORIENTED_EDGE('',*,*,#7642,.F.);
#10878=ORIENTED_EDGE('',*,*,#7646,.F.);
#10879=ORIENTED_EDGE('',*,*,#7651,.F.);
#10880=ORIENTED_EDGE('',*,*,#7650,.F.);
#10881=ORIENTED_EDGE('',*,*,#7654,.F.);
#10882=ORIENTED_EDGE('',*,*,#7659,.F.);
#10883=ORIENTED_EDGE('',*,*,#7658,.F.);
#10884=ORIENTED_EDGE('',*,*,#7662,.F.);
#10885=ORIENTED_EDGE('',*,*,#7667,.F.);
#10886=ORIENTED_EDGE('',*,*,#7666,.F.);
#10887=ORIENTED_EDGE('',*,*,#7670,.F.);
#10888=ORIENTED_EDGE('',*,*,#7781,.F.);
#10889=ORIENTED_EDGE('',*,*,#7780,.F.);
#10890=ORIENTED_EDGE('',*,*,#7676,.F.);
#10891=ORIENTED_EDGE('',*,*,#7817,.F.);
#10892=ORIENTED_EDGE('',*,*,#7818,.F.);
#10893=ORIENTED_EDGE('',*,*,#7630,.T.);
#10894=ORIENTED_EDGE('',*,*,#7629,.T.);
#10895=ORIENTED_EDGE('',*,*,#7787,.T.);
#10896=ORIENTED_EDGE('',*,*,#7786,.T.);
#10897=ORIENTED_EDGE('',*,*,#7627,.T.);
#10898=ORIENTED_EDGE('',*,*,#7626,.T.);
#10899=ORIENTED_EDGE('',*,*,#7622,.T.);
#10900=ORIENTED_EDGE('',*,*,#7621,.T.);
#10901=ORIENTED_EDGE('',*,*,#7617,.T.);
#10902=ORIENTED_EDGE('',*,*,#7616,.T.);
#10903=ORIENTED_EDGE('',*,*,#7612,.T.);
#10904=ORIENTED_EDGE('',*,*,#7611,.T.);
#10905=ORIENTED_EDGE('',*,*,#7607,.T.);
#10906=ORIENTED_EDGE('',*,*,#7606,.T.);
#10907=ORIENTED_EDGE('',*,*,#7602,.T.);
#10908=ORIENTED_EDGE('',*,*,#7601,.T.);
#10909=ORIENTED_EDGE('',*,*,#7597,.T.);
#10910=ORIENTED_EDGE('',*,*,#7596,.T.);
#10911=ORIENTED_EDGE('',*,*,#7592,.T.);
#10912=ORIENTED_EDGE('',*,*,#7591,.T.);
#10913=ORIENTED_EDGE('',*,*,#7587,.T.);
#10914=ORIENTED_EDGE('',*,*,#7586,.T.);
#10915=ORIENTED_EDGE('',*,*,#7731,.F.);
#10916=ORIENTED_EDGE('',*,*,#7819,.T.);
#10917=ORIENTED_EDGE('',*,*,#7680,.T.);
#10918=ORIENTED_EDGE('',*,*,#7820,.T.);
#10919=ORIENTED_EDGE('',*,*,#7734,.F.);
#10920=ORIENTED_EDGE('',*,*,#7820,.F.);
#10921=ORIENTED_EDGE('',*,*,#7679,.F.);
#10922=ORIENTED_EDGE('',*,*,#7678,.F.);
#10923=ORIENTED_EDGE('',*,*,#7685,.F.);
#10924=ORIENTED_EDGE('',*,*,#7684,.F.);
#10925=ORIENTED_EDGE('',*,*,#7690,.F.);
#10926=ORIENTED_EDGE('',*,*,#7689,.F.);
#10927=ORIENTED_EDGE('',*,*,#7695,.F.);
#10928=ORIENTED_EDGE('',*,*,#7694,.F.);
#10929=ORIENTED_EDGE('',*,*,#7700,.F.);
#10930=ORIENTED_EDGE('',*,*,#7699,.F.);
#10931=ORIENTED_EDGE('',*,*,#7705,.F.);
#10932=ORIENTED_EDGE('',*,*,#7704,.F.);
#10933=ORIENTED_EDGE('',*,*,#7710,.F.);
#10934=ORIENTED_EDGE('',*,*,#7709,.F.);
#10935=ORIENTED_EDGE('',*,*,#7715,.F.);
#10936=ORIENTED_EDGE('',*,*,#7714,.F.);
#10937=ORIENTED_EDGE('',*,*,#7720,.F.);
#10938=ORIENTED_EDGE('',*,*,#7719,.F.);
#10939=ORIENTED_EDGE('',*,*,#7777,.F.);
#10940=ORIENTED_EDGE('',*,*,#7776,.F.);
#10941=ORIENTED_EDGE('',*,*,#7728,.F.);
#10942=ORIENTED_EDGE('',*,*,#7727,.F.);
#10943=ORIENTED_EDGE('',*,*,#7821,.F.);
#10944=ORIENTED_EDGE('',*,*,#7769,.F.);
#10945=ORIENTED_EDGE('',*,*,#7775,.F.);
#10946=ORIENTED_EDGE('',*,*,#7774,.F.);
#10947=ORIENTED_EDGE('',*,*,#7767,.F.);
#10948=ORIENTED_EDGE('',*,*,#7766,.F.);
#10949=ORIENTED_EDGE('',*,*,#7763,.F.);
#10950=ORIENTED_EDGE('',*,*,#7759,.F.);
#10951=ORIENTED_EDGE('',*,*,#7758,.F.);
#10952=ORIENTED_EDGE('',*,*,#7755,.F.);
#10953=ORIENTED_EDGE('',*,*,#7751,.F.);
#10954=ORIENTED_EDGE('',*,*,#7750,.F.);
#10955=ORIENTED_EDGE('',*,*,#7747,.F.);
#10956=ORIENTED_EDGE('',*,*,#7743,.F.);
#10957=ORIENTED_EDGE('',*,*,#7742,.F.);
#10958=ORIENTED_EDGE('',*,*,#7739,.F.);
#10959=ORIENTED_EDGE('',*,*,#7735,.F.);
#10960=ORIENTED_EDGE('',*,*,#7819,.F.);
#10961=ORIENTED_EDGE('',*,*,#7730,.F.);
#10962=ORIENTED_EDGE('',*,*,#7738,.F.);
#10963=ORIENTED_EDGE('',*,*,#7737,.F.);
#10964=ORIENTED_EDGE('',*,*,#7741,.F.);
#10965=ORIENTED_EDGE('',*,*,#7746,.F.);
#10966=ORIENTED_EDGE('',*,*,#7745,.F.);
#10967=ORIENTED_EDGE('',*,*,#7749,.F.);
#10968=ORIENTED_EDGE('',*,*,#7754,.F.);
#10969=ORIENTED_EDGE('',*,*,#7753,.F.);
#10970=ORIENTED_EDGE('',*,*,#7757,.F.);
#10971=ORIENTED_EDGE('',*,*,#7762,.F.);
#10972=ORIENTED_EDGE('',*,*,#7761,.F.);
#10973=ORIENTED_EDGE('',*,*,#7765,.F.);
#10974=ORIENTED_EDGE('',*,*,#7773,.F.);
#10975=ORIENTED_EDGE('',*,*,#7772,.F.);
#10976=ORIENTED_EDGE('',*,*,#7771,.F.);
#10977=ORIENTED_EDGE('',*,*,#7822,.F.);
#10978=ORIENTED_EDGE('',*,*,#7823,.F.);
#10979=ORIENTED_EDGE('',*,*,#7725,.T.);
#10980=ORIENTED_EDGE('',*,*,#7724,.T.);
#10981=ORIENTED_EDGE('',*,*,#7779,.T.);
#10982=ORIENTED_EDGE('',*,*,#7778,.T.);
#10983=ORIENTED_EDGE('',*,*,#7722,.T.);
#10984=ORIENTED_EDGE('',*,*,#7721,.T.);
#10985=ORIENTED_EDGE('',*,*,#7717,.T.);
#10986=ORIENTED_EDGE('',*,*,#7716,.T.);
#10987=ORIENTED_EDGE('',*,*,#7712,.T.);
#10988=ORIENTED_EDGE('',*,*,#7711,.T.);
#10989=ORIENTED_EDGE('',*,*,#7707,.T.);
#10990=ORIENTED_EDGE('',*,*,#7706,.T.);
#10991=ORIENTED_EDGE('',*,*,#7702,.T.);
#10992=ORIENTED_EDGE('',*,*,#7701,.T.);
#10993=ORIENTED_EDGE('',*,*,#7697,.T.);
#10994=ORIENTED_EDGE('',*,*,#7696,.T.);
#10995=ORIENTED_EDGE('',*,*,#7692,.T.);
#10996=ORIENTED_EDGE('',*,*,#7691,.T.);
#10997=ORIENTED_EDGE('',*,*,#7687,.T.);
#10998=ORIENTED_EDGE('',*,*,#7686,.T.);
#10999=ORIENTED_EDGE('',*,*,#7682,.T.);
#11000=ORIENTED_EDGE('',*,*,#7681,.T.);
#11001=ORIENTED_EDGE('',*,*,#7448,.F.);
#11002=ORIENTED_EDGE('',*,*,#7543,.F.);
#11003=ORIENTED_EDGE('',*,*,#7733,.F.);
#11004=ORIENTED_EDGE('',*,*,#7638,.F.);
#11005=ORIENTED_EDGE('',*,*,#7824,.F.);
#11006=ORIENTED_EDGE('',*,*,#7825,.T.);
#11007=ORIENTED_EDGE('',*,*,#7826,.F.);
#11008=ORIENTED_EDGE('',*,*,#7825,.F.);
#11009=ORIENTED_EDGE('',*,*,#7827,.F.);
#11010=ORIENTED_EDGE('',*,*,#7828,.T.);
#11011=ORIENTED_EDGE('',*,*,#7829,.F.);
#11012=ORIENTED_EDGE('',*,*,#7828,.F.);
#11013=ORIENTED_EDGE('',*,*,#7830,.F.);
#11014=ORIENTED_EDGE('',*,*,#7831,.T.);
#11015=ORIENTED_EDGE('',*,*,#7832,.F.);
#11016=ORIENTED_EDGE('',*,*,#7831,.F.);
#11017=ORIENTED_EDGE('',*,*,#7833,.F.);
#11018=ORIENTED_EDGE('',*,*,#7834,.T.);
#11019=ORIENTED_EDGE('',*,*,#7835,.F.);
#11020=ORIENTED_EDGE('',*,*,#7834,.F.);
#11021=ORIENTED_EDGE('',*,*,#7836,.T.);
#11022=ORIENTED_EDGE('',*,*,#7837,.T.);
#11023=ORIENTED_EDGE('',*,*,#7838,.F.);
#11024=ORIENTED_EDGE('',*,*,#7839,.F.);
#11025=ORIENTED_EDGE('',*,*,#7840,.T.);
#11026=ORIENTED_EDGE('',*,*,#7839,.T.);
#11027=ORIENTED_EDGE('',*,*,#7841,.F.);
#11028=ORIENTED_EDGE('',*,*,#7842,.F.);
#11029=ORIENTED_EDGE('',*,*,#7843,.T.);
#11030=ORIENTED_EDGE('',*,*,#7842,.T.);
#11031=ORIENTED_EDGE('',*,*,#7844,.F.);
#11032=ORIENTED_EDGE('',*,*,#7845,.F.);
#11033=ORIENTED_EDGE('',*,*,#7846,.T.);
#11034=ORIENTED_EDGE('',*,*,#7845,.T.);
#11035=ORIENTED_EDGE('',*,*,#7847,.F.);
#11036=ORIENTED_EDGE('',*,*,#7837,.F.);
#11037=ORIENTED_EDGE('',*,*,#7847,.T.);
#11038=ORIENTED_EDGE('',*,*,#7844,.T.);
#11039=ORIENTED_EDGE('',*,*,#7841,.T.);
#11040=ORIENTED_EDGE('',*,*,#7838,.T.);
#11041=ORIENTED_EDGE('',*,*,#7813,.T.);
#11042=ORIENTED_EDGE('',*,*,#7812,.T.);
#11043=ORIENTED_EDGE('',*,*,#7580,.T.);
#11044=ORIENTED_EDGE('',*,*,#7811,.T.);
#11045=ORIENTED_EDGE('',*,*,#7536,.T.);
#11046=ORIENTED_EDGE('',*,*,#7823,.T.);
#11047=ORIENTED_EDGE('',*,*,#7822,.T.);
#11048=ORIENTED_EDGE('',*,*,#7770,.T.);
#11049=ORIENTED_EDGE('',*,*,#7821,.T.);
#11050=ORIENTED_EDGE('',*,*,#7726,.T.);
#11051=ORIENTED_EDGE('',*,*,#7833,.T.);
#11052=ORIENTED_EDGE('',*,*,#7830,.T.);
#11053=ORIENTED_EDGE('',*,*,#7827,.T.);
#11054=ORIENTED_EDGE('',*,*,#7824,.T.);
#11055=ORIENTED_EDGE('',*,*,#7818,.T.);
#11056=ORIENTED_EDGE('',*,*,#7817,.T.);
#11057=ORIENTED_EDGE('',*,*,#7675,.T.);
#11058=ORIENTED_EDGE('',*,*,#7816,.T.);
#11059=ORIENTED_EDGE('',*,*,#7631,.T.);
#11060=ORIENTED_EDGE('',*,*,#7808,.T.);
#11061=ORIENTED_EDGE('',*,*,#7807,.T.);
#11062=ORIENTED_EDGE('',*,*,#7485,.T.);
#11063=ORIENTED_EDGE('',*,*,#7806,.T.);
#11064=ORIENTED_EDGE('',*,*,#7441,.T.);
#11065=ORIENTED_EDGE('',*,*,#7846,.F.);
#11066=ORIENTED_EDGE('',*,*,#7836,.F.);
#11067=ORIENTED_EDGE('',*,*,#7840,.F.);
#11068=ORIENTED_EDGE('',*,*,#7843,.F.);
#11069=ORIENTED_EDGE('',*,*,#7826,.T.);
#11070=ORIENTED_EDGE('',*,*,#7829,.T.);
#11071=ORIENTED_EDGE('',*,*,#7832,.T.);
#11072=ORIENTED_EDGE('',*,*,#7835,.T.);
#15699=CYLINDRICAL_SURFACE('',#17048,4.085);
#15700=CYLINDRICAL_SURFACE('',#17050,4.085);
#15701=CYLINDRICAL_SURFACE('',#17051,4.085);
#15702=CYLINDRICAL_SURFACE('',#17052,4.085);
#15703=CYLINDRICAL_SURFACE('',#17053,4.085);
#15704=CYLINDRICAL_SURFACE('',#17054,4.085);
#15705=CYLINDRICAL_SURFACE('',#17055,4.085);
#15706=CYLINDRICAL_SURFACE('',#17056,4.085);
#15707=CYLINDRICAL_SURFACE('',#17057,4.085);
#15708=CYLINDRICAL_SURFACE('',#17058,4.085);
#15709=CYLINDRICAL_SURFACE('',#17060,3.38975);
#15710=CYLINDRICAL_SURFACE('',#17064,3.38975);
#15711=CYLINDRICAL_SURFACE('',#17065,3.38975);
#15712=CYLINDRICAL_SURFACE('',#17066,3.38975);
#15713=CYLINDRICAL_SURFACE('',#17067,3.38975);
#15714=CYLINDRICAL_SURFACE('',#17068,3.38975);
#15715=CYLINDRICAL_SURFACE('',#17069,3.38975);
#15716=CYLINDRICAL_SURFACE('',#17070,3.38975);
#15717=CYLINDRICAL_SURFACE('',#17071,3.38975);
#15718=CYLINDRICAL_SURFACE('',#17072,3.38975);
#15719=CYLINDRICAL_SURFACE('',#17074,4.085);
#15720=CYLINDRICAL_SURFACE('',#17076,4.085);
#15721=CYLINDRICAL_SURFACE('',#17077,4.085);
#15722=CYLINDRICAL_SURFACE('',#17078,4.085);
#15723=CYLINDRICAL_SURFACE('',#17079,4.085);
#15724=CYLINDRICAL_SURFACE('',#17080,4.085);
#15725=CYLINDRICAL_SURFACE('',#17081,4.085);
#15726=CYLINDRICAL_SURFACE('',#17082,4.085);
#15727=CYLINDRICAL_SURFACE('',#17083,4.085);
#15728=CYLINDRICAL_SURFACE('',#17084,4.085);
#15729=CYLINDRICAL_SURFACE('',#17086,3.38975);
#15730=CYLINDRICAL_SURFACE('',#17090,3.38975);
#15731=CYLINDRICAL_SURFACE('',#17091,3.38975);
#15732=CYLINDRICAL_SURFACE('',#17092,3.38975);
#15733=CYLINDRICAL_SURFACE('',#17093,3.38975);
#15734=CYLINDRICAL_SURFACE('',#17094,3.38975);
#15735=CYLINDRICAL_SURFACE('',#17095,3.38975);
#15736=CYLINDRICAL_SURFACE('',#17096,3.38975);
#15737=CYLINDRICAL_SURFACE('',#17097,3.38975);
#15738=CYLINDRICAL_SURFACE('',#17098,3.38975);
#15739=CYLINDRICAL_SURFACE('',#17100,4.085);
#15740=CYLINDRICAL_SURFACE('',#17102,4.085);
#15741=CYLINDRICAL_SURFACE('',#17103,4.085);
#15742=CYLINDRICAL_SURFACE('',#17104,4.085);
#15743=CYLINDRICAL_SURFACE('',#17105,4.085);
#15744=CYLINDRICAL_SURFACE('',#17106,4.085);
#15745=CYLINDRICAL_SURFACE('',#17107,4.085);
#15746=CYLINDRICAL_SURFACE('',#17108,4.085);
#15747=CYLINDRICAL_SURFACE('',#17109,4.085);
#15748=CYLINDRICAL_SURFACE('',#17110,4.085);
#15749=CYLINDRICAL_SURFACE('',#17112,3.38975);
#15750=CYLINDRICAL_SURFACE('',#17116,3.38975);
#15751=CYLINDRICAL_SURFACE('',#17117,3.38975);
#15752=CYLINDRICAL_SURFACE('',#17118,3.38975);
#15753=CYLINDRICAL_SURFACE('',#17119,3.38975);
#15754=CYLINDRICAL_SURFACE('',#17120,3.38975);
#15755=CYLINDRICAL_SURFACE('',#17121,3.38975);
#15756=CYLINDRICAL_SURFACE('',#17122,3.38975);
#15757=CYLINDRICAL_SURFACE('',#17123,3.38975);
#15758=CYLINDRICAL_SURFACE('',#17124,3.38975);
#15759=CYLINDRICAL_SURFACE('',#17126,4.085);
#15760=CYLINDRICAL_SURFACE('',#17128,4.085);
#15761=CYLINDRICAL_SURFACE('',#17129,4.085);
#15762=CYLINDRICAL_SURFACE('',#17130,4.085);
#15763=CYLINDRICAL_SURFACE('',#17131,4.085);
#15764=CYLINDRICAL_SURFACE('',#17132,4.085);
#15765=CYLINDRICAL_SURFACE('',#17133,4.085);
#15766=CYLINDRICAL_SURFACE('',#17134,4.085);
#15767=CYLINDRICAL_SURFACE('',#17135,4.085);
#15768=CYLINDRICAL_SURFACE('',#17136,4.085);
#15769=CYLINDRICAL_SURFACE('',#17138,3.38975);
#15770=CYLINDRICAL_SURFACE('',#17142,3.38975);
#15771=CYLINDRICAL_SURFACE('',#17143,3.38975);
#15772=CYLINDRICAL_SURFACE('',#17144,3.38975);
#15773=CYLINDRICAL_SURFACE('',#17145,3.38975);
#15774=CYLINDRICAL_SURFACE('',#17146,3.38975);
#15775=CYLINDRICAL_SURFACE('',#17147,3.38975);
#15776=CYLINDRICAL_SURFACE('',#17148,3.38975);
#15777=CYLINDRICAL_SURFACE('',#17149,3.38975);
#15778=CYLINDRICAL_SURFACE('',#17150,3.38975);
#15779=CYLINDRICAL_SURFACE('',#17152,3.38975);
#15780=CYLINDRICAL_SURFACE('',#17153,4.085);
#15781=CYLINDRICAL_SURFACE('',#17154,3.38975);
#15782=CYLINDRICAL_SURFACE('',#17155,4.085);
#15783=CYLINDRICAL_SURFACE('',#17156,3.38975);
#15784=CYLINDRICAL_SURFACE('',#17157,4.085);
#15785=CYLINDRICAL_SURFACE('',#17158,3.38975);
#15786=CYLINDRICAL_SURFACE('',#17159,4.085);
#15787=CYLINDRICAL_SURFACE('',#17168,4.5);
#15788=CYLINDRICAL_SURFACE('',#17171,4.5);
#15789=CYLINDRICAL_SURFACE('',#17174,4.5);
#15790=CYLINDRICAL_SURFACE('',#17177,4.5);
#16191=ADVANCED_FACE('',(#423),#15699,.F.);
#16192=ADVANCED_FACE('',(#424),#15700,.F.);
#16193=ADVANCED_FACE('',(#425),#15701,.F.);
#16194=ADVANCED_FACE('',(#426),#15702,.F.);
#16195=ADVANCED_FACE('',(#427),#15703,.F.);
#16196=ADVANCED_FACE('',(#428),#15704,.F.);
#16197=ADVANCED_FACE('',(#429),#15705,.F.);
#16198=ADVANCED_FACE('',(#430),#15706,.F.);
#16199=ADVANCED_FACE('',(#431),#15707,.F.);
#16200=ADVANCED_FACE('',(#432),#15708,.F.);
#16201=ADVANCED_FACE('',(#433),#15709,.F.);
#16202=ADVANCED_FACE('',(#434),#15710,.F.);
#16203=ADVANCED_FACE('',(#435),#15711,.F.);
#16204=ADVANCED_FACE('',(#436),#15712,.F.);
#16205=ADVANCED_FACE('',(#437),#15713,.F.);
#16206=ADVANCED_FACE('',(#438),#15714,.F.);
#16207=ADVANCED_FACE('',(#439),#15715,.F.);
#16208=ADVANCED_FACE('',(#440),#15716,.F.);
#16209=ADVANCED_FACE('',(#441),#15717,.F.);
#16210=ADVANCED_FACE('',(#442),#15718,.F.);
#16211=ADVANCED_FACE('',(#443),#15719,.F.);
#16212=ADVANCED_FACE('',(#444),#15720,.F.);
#16213=ADVANCED_FACE('',(#445),#15721,.F.);
#16214=ADVANCED_FACE('',(#446),#15722,.F.);
#16215=ADVANCED_FACE('',(#447),#15723,.F.);
#16216=ADVANCED_FACE('',(#448),#15724,.F.);
#16217=ADVANCED_FACE('',(#449),#15725,.F.);
#16218=ADVANCED_FACE('',(#450),#15726,.F.);
#16219=ADVANCED_FACE('',(#451),#15727,.F.);
#16220=ADVANCED_FACE('',(#452),#15728,.F.);
#16221=ADVANCED_FACE('',(#453),#15729,.F.);
#16222=ADVANCED_FACE('',(#454),#15730,.F.);
#16223=ADVANCED_FACE('',(#455),#15731,.F.);
#16224=ADVANCED_FACE('',(#456),#15732,.F.);
#16225=ADVANCED_FACE('',(#457),#15733,.F.);
#16226=ADVANCED_FACE('',(#458),#15734,.F.);
#16227=ADVANCED_FACE('',(#459),#15735,.F.);
#16228=ADVANCED_FACE('',(#460),#15736,.F.);
#16229=ADVANCED_FACE('',(#461),#15737,.F.);
#16230=ADVANCED_FACE('',(#462),#15738,.F.);
#16231=ADVANCED_FACE('',(#463),#15739,.F.);
#16232=ADVANCED_FACE('',(#464),#15740,.F.);
#16233=ADVANCED_FACE('',(#465),#15741,.F.);
#16234=ADVANCED_FACE('',(#466),#15742,.F.);
#16235=ADVANCED_FACE('',(#467),#15743,.F.);
#16236=ADVANCED_FACE('',(#468),#15744,.F.);
#16237=ADVANCED_FACE('',(#469),#15745,.F.);
#16238=ADVANCED_FACE('',(#470),#15746,.F.);
#16239=ADVANCED_FACE('',(#471),#15747,.F.);
#16240=ADVANCED_FACE('',(#472),#15748,.F.);
#16241=ADVANCED_FACE('',(#473),#15749,.F.);
#16242=ADVANCED_FACE('',(#474),#15750,.F.);
#16243=ADVANCED_FACE('',(#475),#15751,.F.);
#16244=ADVANCED_FACE('',(#476),#15752,.F.);
#16245=ADVANCED_FACE('',(#477),#15753,.F.);
#16246=ADVANCED_FACE('',(#478),#15754,.F.);
#16247=ADVANCED_FACE('',(#479),#15755,.F.);
#16248=ADVANCED_FACE('',(#480),#15756,.F.);
#16249=ADVANCED_FACE('',(#481),#15757,.F.);
#16250=ADVANCED_FACE('',(#482),#15758,.F.);
#16251=ADVANCED_FACE('',(#483),#15759,.F.);
#16252=ADVANCED_FACE('',(#484),#15760,.F.);
#16253=ADVANCED_FACE('',(#485),#15761,.F.);
#16254=ADVANCED_FACE('',(#486),#15762,.F.);
#16255=ADVANCED_FACE('',(#487),#15763,.F.);
#16256=ADVANCED_FACE('',(#488),#15764,.F.);
#16257=ADVANCED_FACE('',(#489),#15765,.F.);
#16258=ADVANCED_FACE('',(#490),#15766,.F.);
#16259=ADVANCED_FACE('',(#491),#15767,.F.);
#16260=ADVANCED_FACE('',(#492),#15768,.F.);
#16261=ADVANCED_FACE('',(#493),#15769,.F.);
#16262=ADVANCED_FACE('',(#494),#15770,.F.);
#16263=ADVANCED_FACE('',(#495),#15771,.F.);
#16264=ADVANCED_FACE('',(#496),#15772,.F.);
#16265=ADVANCED_FACE('',(#497),#15773,.F.);
#16266=ADVANCED_FACE('',(#498),#15774,.F.);
#16267=ADVANCED_FACE('',(#499),#15775,.F.);
#16268=ADVANCED_FACE('',(#500),#15776,.F.);
#16269=ADVANCED_FACE('',(#501),#15777,.F.);
#16270=ADVANCED_FACE('',(#502),#15778,.F.);
#16271=ADVANCED_FACE('',(#503),#15779,.F.);
#16272=ADVANCED_FACE('',(#504),#15780,.F.);
#16273=ADVANCED_FACE('',(#505),#15781,.F.);
#16274=ADVANCED_FACE('',(#506),#15782,.F.);
#16275=ADVANCED_FACE('',(#507),#15783,.F.);
#16276=ADVANCED_FACE('',(#508),#15784,.F.);
#16277=ADVANCED_FACE('',(#509),#15785,.F.);
#16278=ADVANCED_FACE('',(#510),#15786,.F.);
#16279=ADVANCED_FACE('',(#511),#303,.T.);
#16280=ADVANCED_FACE('',(#512),#273,.F.);
#16281=ADVANCED_FACE('',(#513),#274,.F.);
#16282=ADVANCED_FACE('',(#514),#304,.T.);
#16283=ADVANCED_FACE('',(#515),#275,.F.);
#16284=ADVANCED_FACE('',(#516),#276,.F.);
#16285=ADVANCED_FACE('',(#517),#305,.T.);
#16286=ADVANCED_FACE('',(#518),#277,.F.);
#16287=ADVANCED_FACE('',(#519),#278,.F.);
#16288=ADVANCED_FACE('',(#520),#306,.T.);
#16289=ADVANCED_FACE('',(#521),#279,.F.);
#16290=ADVANCED_FACE('',(#522),#280,.F.);
#16291=ADVANCED_FACE('',(#523),#307,.F.);
#16292=ADVANCED_FACE('',(#524),#308,.F.);
#16293=ADVANCED_FACE('',(#525),#309,.F.);
#16294=ADVANCED_FACE('',(#526),#310,.F.);
#16295=ADVANCED_FACE('',(#527),#15787,.F.);
#16296=ADVANCED_FACE('',(#528),#15788,.F.);
#16297=ADVANCED_FACE('',(#529),#15789,.F.);
#16298=ADVANCED_FACE('',(#530),#15790,.F.);
#16299=ADVANCED_FACE('',(#531),#311,.T.);
#16300=ADVANCED_FACE('',(#532),#312,.T.);
#16301=ADVANCED_FACE('',(#533),#313,.T.);
#16302=ADVANCED_FACE('',(#534),#314,.T.);
#16303=ADVANCED_FACE('',(#535,#187,#188,#189,#190,#191,#192,#193,#194),
#315,.T.);
#16304=ADVANCED_FACE('',(#536,#195,#196,#197,#198),#316,.F.);
#16841=CLOSED_SHELL('',(#16191,#16192,#16193,#16194,#16195,#16196,#16197,
#16198,#16199,#16200,#16201,#16202,#16203,#16204,#16205,#16206,#16207,#16208,
#16209,#16210,#16211,#16212,#16213,#16214,#16215,#16216,#16217,#16218,#16219,
#16220,#16221,#16222,#16223,#16224,#16225,#16226,#16227,#16228,#16229,#16230,
#16231,#16232,#16233,#16234,#16235,#16236,#16237,#16238,#16239,#16240,#16241,
#16242,#16243,#16244,#16245,#16246,#16247,#16248,#16249,#16250,#16251,#16252,
#16253,#16254,#16255,#16256,#16257,#16258,#16259,#16260,#16261,#16262,#16263,
#16264,#16265,#16266,#16267,#16268,#16269,#16270,#16271,#16272,#16273,#16274,
#16275,#16276,#16277,#16278,#16279,#16280,#16281,#16282,#16283,#16284,#16285,
#16286,#16287,#16288,#16289,#16290,#16291,#16292,#16293,#16294,#16295,#16296,
#16297,#16298,#16299,#16300,#16301,#16302,#16303,#16304));
#17047=AXIS2_PLACEMENT_3D('',#20213,#17891,#17892);
#17048=AXIS2_PLACEMENT_3D('',#20214,#17893,#17894);
#17049=AXIS2_PLACEMENT_3D('',#20370,#17896,#17897);
#17050=AXIS2_PLACEMENT_3D('',#20563,#17898,#17899);
#17051=AXIS2_PLACEMENT_3D('',#21032,#17901,#17902);
#17052=AXIS2_PLACEMENT_3D('',#21498,#17904,#17905);
#17053=AXIS2_PLACEMENT_3D('',#21961,#17907,#17908);
#17054=AXIS2_PLACEMENT_3D('',#22424,#17910,#17911);
#17055=AXIS2_PLACEMENT_3D('',#22890,#17913,#17914);
#17056=AXIS2_PLACEMENT_3D('',#23353,#17916,#17917);
#17057=AXIS2_PLACEMENT_3D('',#23819,#17919,#17920);
#17058=AXIS2_PLACEMENT_3D('',#24288,#17922,#17923);
#17059=AXIS2_PLACEMENT_3D('',#24382,#17925,#17926);
#17060=AXIS2_PLACEMENT_3D('',#24530,#17927,#17928);
#17061=AXIS2_PLACEMENT_3D('',#24633,#17930,#17931);
#17062=AXIS2_PLACEMENT_3D('',#24636,#17933,#17934);
#17063=AXIS2_PLACEMENT_3D('',#24638,#17935,#17936);
#17064=AXIS2_PLACEMENT_3D('',#24773,#17937,#17938);
#17065=AXIS2_PLACEMENT_3D('',#25164,#17940,#17941);
#17066=AXIS2_PLACEMENT_3D('',#25551,#17943,#17944);
#17067=AXIS2_PLACEMENT_3D('',#25936,#17946,#17947);
#17068=AXIS2_PLACEMENT_3D('',#26327,#17949,#17950);
#17069=AXIS2_PLACEMENT_3D('',#26714,#17952,#17953);
#17070=AXIS2_PLACEMENT_3D('',#27095,#17955,#17956);
#17071=AXIS2_PLACEMENT_3D('',#27488,#17958,#17959);
#17072=AXIS2_PLACEMENT_3D('',#27894,#17961,#17962);
#17073=AXIS2_PLACEMENT_3D('',#28026,#17964,#17965);
#17074=AXIS2_PLACEMENT_3D('',#28205,#17966,#17967);
#17075=AXIS2_PLACEMENT_3D('',#28361,#17969,#17970);
#17076=AXIS2_PLACEMENT_3D('',#28554,#17971,#17972);
#17077=AXIS2_PLACEMENT_3D('',#29023,#17974,#17975);
#17078=AXIS2_PLACEMENT_3D('',#29489,#17977,#17978);
#17079=AXIS2_PLACEMENT_3D('',#29952,#17980,#17981);
#17080=AXIS2_PLACEMENT_3D('',#30415,#17983,#17984);
#17081=AXIS2_PLACEMENT_3D('',#30881,#17986,#17987);
#17082=AXIS2_PLACEMENT_3D('',#31344,#17989,#17990);
#17083=AXIS2_PLACEMENT_3D('',#31810,#17992,#17993);
#17084=AXIS2_PLACEMENT_3D('',#32279,#17995,#17996);
#17085=AXIS2_PLACEMENT_3D('',#32373,#17998,#17999);
#17086=AXIS2_PLACEMENT_3D('',#32521,#18000,#18001);
#17087=AXIS2_PLACEMENT_3D('',#32624,#18003,#18004);
#17088=AXIS2_PLACEMENT_3D('',#32627,#18006,#18007);
#17089=AXIS2_PLACEMENT_3D('',#32629,#18008,#18009);
#17090=AXIS2_PLACEMENT_3D('',#32768,#18010,#18011);
#17091=AXIS2_PLACEMENT_3D('',#33161,#18013,#18014);
#17092=AXIS2_PLACEMENT_3D('',#33540,#18016,#18017);
#17093=AXIS2_PLACEMENT_3D('',#33923,#18019,#18020);
#17094=AXIS2_PLACEMENT_3D('',#34310,#18022,#18023);
#17095=AXIS2_PLACEMENT_3D('',#34705,#18025,#18026);
#17096=AXIS2_PLACEMENT_3D('',#35086,#18028,#18029);
#17097=AXIS2_PLACEMENT_3D('',#35481,#18031,#18032);
#17098=AXIS2_PLACEMENT_3D('',#35887,#18034,#18035);
#17099=AXIS2_PLACEMENT_3D('',#36021,#18037,#18038);
#17100=AXIS2_PLACEMENT_3D('',#36200,#18039,#18040);
#17101=AXIS2_PLACEMENT_3D('',#36356,#18042,#18043);
#17102=AXIS2_PLACEMENT_3D('',#36549,#18044,#18045);
#17103=AXIS2_PLACEMENT_3D('',#37018,#18047,#18048);
#17104=AXIS2_PLACEMENT_3D('',#37484,#18050,#18051);
#17105=AXIS2_PLACEMENT_3D('',#37947,#18053,#18054);
#17106=AXIS2_PLACEMENT_3D('',#38410,#18056,#18057);
#17107=AXIS2_PLACEMENT_3D('',#38876,#18059,#18060);
#17108=AXIS2_PLACEMENT_3D('',#39339,#18062,#18063);
#17109=AXIS2_PLACEMENT_3D('',#39805,#18065,#18066);
#17110=AXIS2_PLACEMENT_3D('',#40274,#18068,#18069);
#17111=AXIS2_PLACEMENT_3D('',#40368,#18071,#18072);
#17112=AXIS2_PLACEMENT_3D('',#40516,#18073,#18074);
#17113=AXIS2_PLACEMENT_3D('',#40619,#18076,#18077);
#17114=AXIS2_PLACEMENT_3D('',#40622,#18079,#18080);
#17115=AXIS2_PLACEMENT_3D('',#40624,#18081,#18082);
#17116=AXIS2_PLACEMENT_3D('',#40763,#18083,#18084);
#17117=AXIS2_PLACEMENT_3D('',#41156,#18086,#18087);
#17118=AXIS2_PLACEMENT_3D('',#41547,#18089,#18090);
#17119=AXIS2_PLACEMENT_3D('',#41932,#18092,#18093);
#17120=AXIS2_PLACEMENT_3D('',#42325,#18095,#18096);
#17121=AXIS2_PLACEMENT_3D('',#42716,#18098,#18099);
#17122=AXIS2_PLACEMENT_3D('',#43101,#18101,#18102);
#17123=AXIS2_PLACEMENT_3D('',#43496,#18104,#18105);
#17124=AXIS2_PLACEMENT_3D('',#43900,#18107,#18108);
#17125=AXIS2_PLACEMENT_3D('',#44034,#18110,#18111);
#17126=AXIS2_PLACEMENT_3D('',#44211,#18112,#18113);
#17127=AXIS2_PLACEMENT_3D('',#44367,#18115,#18116);
#17128=AXIS2_PLACEMENT_3D('',#44560,#18117,#18118);
#17129=AXIS2_PLACEMENT_3D('',#45029,#18120,#18121);
#17130=AXIS2_PLACEMENT_3D('',#45495,#18123,#18124);
#17131=AXIS2_PLACEMENT_3D('',#45958,#18126,#18127);
#17132=AXIS2_PLACEMENT_3D('',#46421,#18129,#18130);
#17133=AXIS2_PLACEMENT_3D('',#46887,#18132,#18133);
#17134=AXIS2_PLACEMENT_3D('',#47350,#18135,#18136);
#17135=AXIS2_PLACEMENT_3D('',#47816,#18138,#18139);
#17136=AXIS2_PLACEMENT_3D('',#48285,#18141,#18142);
#17137=AXIS2_PLACEMENT_3D('',#48379,#18144,#18145);
#17138=AXIS2_PLACEMENT_3D('',#48527,#18146,#18147);
#17139=AXIS2_PLACEMENT_3D('',#48630,#18149,#18150);
#17140=AXIS2_PLACEMENT_3D('',#48633,#18152,#18153);
#17141=AXIS2_PLACEMENT_3D('',#48635,#18154,#18155);
#17142=AXIS2_PLACEMENT_3D('',#48774,#18156,#18157);
#17143=AXIS2_PLACEMENT_3D('',#49163,#18159,#18160);
#17144=AXIS2_PLACEMENT_3D('',#49550,#18162,#18163);
#17145=AXIS2_PLACEMENT_3D('',#49931,#18165,#18166);
#17146=AXIS2_PLACEMENT_3D('',#50324,#18168,#18169);
#17147=AXIS2_PLACEMENT_3D('',#50719,#18171,#18172);
#17148=AXIS2_PLACEMENT_3D('',#51102,#18174,#18175);
#17149=AXIS2_PLACEMENT_3D('',#51499,#18177,#18178);
#17150=AXIS2_PLACEMENT_3D('',#51905,#18180,#18181);
#17151=AXIS2_PLACEMENT_3D('',#52039,#18183,#18184);
#17152=AXIS2_PLACEMENT_3D('',#52220,#18185,#18186);
#17153=AXIS2_PLACEMENT_3D('',#52602,#18187,#18188);
#17154=AXIS2_PLACEMENT_3D('',#53062,#18189,#18190);
#17155=AXIS2_PLACEMENT_3D('',#53444,#18191,#18192);
#17156=AXIS2_PLACEMENT_3D('',#53904,#18193,#18194);
#17157=AXIS2_PLACEMENT_3D('',#54282,#18195,#18196);
#17158=AXIS2_PLACEMENT_3D('',#54742,#18197,#18198);
#17159=AXIS2_PLACEMENT_3D('',#55124,#18199,#18200);
#17160=AXIS2_PLACEMENT_3D('',#55584,#18201,#18202);
#17161=AXIS2_PLACEMENT_3D('',#56549,#18203,#18204);
#17162=AXIS2_PLACEMENT_3D('',#57514,#18205,#18206);
#17163=AXIS2_PLACEMENT_3D('',#58479,#18207,#18208);
#17164=AXIS2_PLACEMENT_3D('',#59441,#18209,#18210);
#17165=AXIS2_PLACEMENT_3D('',#59442,#18211,#18212);
#17166=AXIS2_PLACEMENT_3D('',#59443,#18213,#18214);
#17167=AXIS2_PLACEMENT_3D('',#59444,#18215,#18216);
#17168=AXIS2_PLACEMENT_3D('',#59445,#18217,#18218);
#17169=AXIS2_PLACEMENT_3D('',#59447,#18219,#18220);
#17170=AXIS2_PLACEMENT_3D('',#59450,#18222,#18223);
#17171=AXIS2_PLACEMENT_3D('',#59451,#18224,#18225);
#17172=AXIS2_PLACEMENT_3D('',#59453,#18226,#18227);
#17173=AXIS2_PLACEMENT_3D('',#59456,#18229,#18230);
#17174=AXIS2_PLACEMENT_3D('',#59457,#18231,#18232);
#17175=AXIS2_PLACEMENT_3D('',#59459,#18233,#18234);
#17176=AXIS2_PLACEMENT_3D('',#59462,#18236,#18237);
#17177=AXIS2_PLACEMENT_3D('',#59463,#18238,#18239);
#17178=AXIS2_PLACEMENT_3D('',#59465,#18240,#18241);
#17179=AXIS2_PLACEMENT_3D('',#59468,#18243,#18244);
#17180=AXIS2_PLACEMENT_3D('',#59469,#18245,#18246);
#17181=AXIS2_PLACEMENT_3D('',#59478,#18251,#18252);
#17182=AXIS2_PLACEMENT_3D('',#59484,#18256,#18257);
#17183=AXIS2_PLACEMENT_3D('',#59490,#18261,#18262);
#17184=AXIS2_PLACEMENT_3D('',#59493,#18265,#18266);
#17185=AXIS2_PLACEMENT_3D('',#59494,#18267,#18268);
#17891=DIRECTION('axis',(0.,0.,1.));
#17892=DIRECTION('refdir',(1.,0.,0.));
#17893=DIRECTION('center_axis',(0.,0.,-1.));
#17894=DIRECTION('ref_axis',(-0.608852061413682,-0.79328378737518,0.));
#17895=DIRECTION('',(0.,0.,-1.));
#17896=DIRECTION('center_axis',(0.,0.,1.));
#17897=DIRECTION('ref_axis',(1.,-4.78333543045355E-14,0.));
#17898=DIRECTION('center_axis',(0.,0.,-1.));
#17899=DIRECTION('ref_axis',(-0.608852061413682,-0.79328378737518,0.));
#17900=DIRECTION('',(0.,0.,-1.));
#17901=DIRECTION('center_axis',(0.,0.,-1.));
#17902=DIRECTION('ref_axis',(-0.608852061413682,-0.79328378737518,0.));
#17903=DIRECTION('',(0.,0.,-1.));
#17904=DIRECTION('center_axis',(0.,0.,-1.));
#17905=DIRECTION('ref_axis',(-0.608852061413682,-0.79328378737518,0.));
#17906=DIRECTION('',(0.,0.,-1.));
#17907=DIRECTION('center_axis',(0.,0.,-1.));
#17908=DIRECTION('ref_axis',(-0.608852061413682,-0.79328378737518,0.));
#17909=DIRECTION('',(0.,0.,-1.));
#17910=DIRECTION('center_axis',(0.,0.,-1.));
#17911=DIRECTION('ref_axis',(-0.608852061413682,-0.79328378737518,0.));
#17912=DIRECTION('',(0.,0.,-1.));
#17913=DIRECTION('center_axis',(0.,0.,-1.));
#17914=DIRECTION('ref_axis',(-0.608852061413682,-0.79328378737518,0.));
#17915=DIRECTION('',(0.,0.,-1.));
#17916=DIRECTION('center_axis',(0.,0.,-1.));
#17917=DIRECTION('ref_axis',(-0.608852061413682,-0.79328378737518,0.));
#17918=DIRECTION('',(0.,0.,-1.));
#17919=DIRECTION('center_axis',(0.,0.,-1.));
#17920=DIRECTION('ref_axis',(-0.608852061413682,-0.79328378737518,0.));
#17921=DIRECTION('',(0.,0.,-1.));
#17922=DIRECTION('center_axis',(0.,0.,-1.));
#17923=DIRECTION('ref_axis',(-0.608852061413682,-0.79328378737518,0.));
#17924=DIRECTION('',(0.,0.,-1.));
#17925=DIRECTION('center_axis',(0.,0.,-1.));
#17926=DIRECTION('ref_axis',(1.,-4.78333543045355E-14,0.));
#17927=DIRECTION('center_axis',(0.,0.,-1.));
#17928=DIRECTION('ref_axis',(0.937755906520935,-0.347295061561634,0.));
#17929=DIRECTION('',(0.,0.,-1.));
#17930=DIRECTION('center_axis',(0.,0.,1.));
#17931=DIRECTION('ref_axis',(1.,0.,0.));
#17932=DIRECTION('',(0.,0.,-1.));
#17933=DIRECTION('center_axis',(0.,0.,1.));
#17934=DIRECTION('ref_axis',(1.,0.,0.));
#17935=DIRECTION('center_axis',(0.,0.,1.));
#17936=DIRECTION('ref_axis',(1.,0.,0.));
#17937=DIRECTION('center_axis',(0.,0.,-1.));
#17938=DIRECTION('ref_axis',(0.937755906520935,-0.347295061561634,0.));
#17939=DIRECTION('',(0.,0.,-1.));
#17940=DIRECTION('center_axis',(0.,0.,-1.));
#17941=DIRECTION('ref_axis',(0.937755906520935,-0.347295061561634,0.));
#17942=DIRECTION('',(0.,0.,-1.));
#17943=DIRECTION('center_axis',(0.,0.,-1.));
#17944=DIRECTION('ref_axis',(0.937755906520935,-0.347295061561634,0.));
#17945=DIRECTION('',(0.,0.,-1.));
#17946=DIRECTION('center_axis',(0.,0.,-1.));
#17947=DIRECTION('ref_axis',(0.937755906520935,-0.347295061561634,0.));
#17948=DIRECTION('',(0.,0.,-1.));
#17949=DIRECTION('center_axis',(0.,0.,-1.));
#17950=DIRECTION('ref_axis',(0.937755906520935,-0.347295061561634,0.));
#17951=DIRECTION('',(0.,0.,-1.));
#17952=DIRECTION('center_axis',(0.,0.,-1.));
#17953=DIRECTION('ref_axis',(0.937755906520935,-0.347295061561634,0.));
#17954=DIRECTION('',(0.,0.,-1.));
#17955=DIRECTION('center_axis',(0.,0.,-1.));
#17956=DIRECTION('ref_axis',(0.937755906520935,-0.347295061561634,0.));
#17957=DIRECTION('',(0.,0.,-1.));
#17958=DIRECTION('center_axis',(0.,0.,-1.));
#17959=DIRECTION('ref_axis',(0.937755906520935,-0.347295061561634,0.));
#17960=DIRECTION('',(0.,0.,-1.));
#17961=DIRECTION('center_axis',(0.,0.,-1.));
#17962=DIRECTION('ref_axis',(0.857775286865319,-0.514024860530227,0.));
#17963=DIRECTION('',(0.,0.,-1.));
#17964=DIRECTION('center_axis',(0.,0.,-1.));
#17965=DIRECTION('ref_axis',(1.,0.,0.));
#17966=DIRECTION('center_axis',(0.,0.,-1.));
#17967=DIRECTION('ref_axis',(-0.608854967610821,-0.793281556835671,0.));
#17968=DIRECTION('',(0.,0.,-1.));
#17969=DIRECTION('center_axis',(0.,0.,1.));
#17970=DIRECTION('ref_axis',(1.,-4.56591109270566E-14,0.));
#17971=DIRECTION('center_axis',(0.,0.,-1.));
#17972=DIRECTION('ref_axis',(-0.608854967610821,-0.793281556835671,0.));
#17973=DIRECTION('',(0.,0.,-1.));
#17974=DIRECTION('center_axis',(0.,0.,-1.));
#17975=DIRECTION('ref_axis',(-0.608854967610821,-0.793281556835671,0.));
#17976=DIRECTION('',(0.,0.,-1.));
#17977=DIRECTION('center_axis',(0.,0.,-1.));
#17978=DIRECTION('ref_axis',(-0.608854967610821,-0.793281556835671,0.));
#17979=DIRECTION('',(0.,0.,-1.));
#17980=DIRECTION('center_axis',(0.,0.,-1.));
#17981=DIRECTION('ref_axis',(-0.608854967610821,-0.793281556835671,0.));
#17982=DIRECTION('',(0.,0.,-1.));
#17983=DIRECTION('center_axis',(0.,0.,-1.));
#17984=DIRECTION('ref_axis',(-0.608854967610821,-0.793281556835671,0.));
#17985=DIRECTION('',(0.,0.,-1.));
#17986=DIRECTION('center_axis',(0.,0.,-1.));
#17987=DIRECTION('ref_axis',(-0.608854967610821,-0.793281556835671,0.));
#17988=DIRECTION('',(0.,0.,-1.));
#17989=DIRECTION('center_axis',(0.,0.,-1.));
#17990=DIRECTION('ref_axis',(-0.608854967610821,-0.793281556835671,0.));
#17991=DIRECTION('',(0.,0.,-1.));
#17992=DIRECTION('center_axis',(0.,0.,-1.));
#17993=DIRECTION('ref_axis',(-0.608854967610821,-0.793281556835671,0.));
#17994=DIRECTION('',(0.,0.,-1.));
#17995=DIRECTION('center_axis',(0.,0.,-1.));
#17996=DIRECTION('ref_axis',(-0.608854967610821,-0.793281556835671,0.));
#17997=DIRECTION('',(0.,0.,-1.));
#17998=DIRECTION('center_axis',(0.,0.,-1.));
#17999=DIRECTION('ref_axis',(1.,-4.56591109270566E-14,0.));
#18000=DIRECTION('center_axis',(0.,0.,-1.));
#18001=DIRECTION('ref_axis',(0.937753558233112,-0.347301402273498,0.));
#18002=DIRECTION('',(0.,0.,-1.));
#18003=DIRECTION('center_axis',(0.,0.,1.));
#18004=DIRECTION('ref_axis',(1.,0.,0.));
#18005=DIRECTION('',(0.,0.,-1.));
#18006=DIRECTION('center_axis',(0.,0.,1.));
#18007=DIRECTION('ref_axis',(1.,0.,0.));
#18008=DIRECTION('center_axis',(0.,0.,1.));
#18009=DIRECTION('ref_axis',(1.,0.,0.));
#18010=DIRECTION('center_axis',(0.,0.,-1.));
#18011=DIRECTION('ref_axis',(0.937753558233112,-0.347301402273498,0.));
#18012=DIRECTION('',(0.,0.,-1.));
#18013=DIRECTION('center_axis',(0.,0.,-1.));
#18014=DIRECTION('ref_axis',(0.937753558233112,-0.347301402273498,0.));
#18015=DIRECTION('',(0.,0.,-1.));
#18016=DIRECTION('center_axis',(0.,0.,-1.));
#18017=DIRECTION('ref_axis',(0.937753558233112,-0.347301402273498,0.));
#18018=DIRECTION('',(0.,0.,-1.));
#18019=DIRECTION('center_axis',(0.,0.,-1.));
#18020=DIRECTION('ref_axis',(0.937753558233112,-0.347301402273498,0.));
#18021=DIRECTION('',(0.,0.,-1.));
#18022=DIRECTION('center_axis',(0.,0.,-1.));
#18023=DIRECTION('ref_axis',(0.937753558233112,-0.347301402273498,0.));
#18024=DIRECTION('',(0.,0.,-1.));
#18025=DIRECTION('center_axis',(0.,0.,-1.));
#18026=DIRECTION('ref_axis',(0.937753558233112,-0.347301402273498,0.));
#18027=DIRECTION('',(0.,0.,-1.));
#18028=DIRECTION('center_axis',(0.,0.,-1.));
#18029=DIRECTION('ref_axis',(0.937753558233112,-0.347301402273498,0.));
#18030=DIRECTION('',(0.,0.,-1.));
#18031=DIRECTION('center_axis',(0.,0.,-1.));
#18032=DIRECTION('ref_axis',(0.937753558233112,-0.347301402273498,0.));
#18033=DIRECTION('',(0.,0.,-1.));
#18034=DIRECTION('center_axis',(0.,0.,-1.));
#18035=DIRECTION('ref_axis',(0.85779647863907,-0.51398949525687,0.));
#18036=DIRECTION('',(0.,0.,-1.));
#18037=DIRECTION('center_axis',(0.,0.,-1.));
#18038=DIRECTION('ref_axis',(1.,0.,0.));
#18039=DIRECTION('center_axis',(0.,0.,-1.));
#18040=DIRECTION('ref_axis',(-0.608852066092606,-0.793283783784066,0.));
#18041=DIRECTION('',(0.,0.,-1.));
#18042=DIRECTION('center_axis',(0.,0.,1.));
#18043=DIRECTION('ref_axis',(1.,-4.78333543045355E-14,0.));
#18044=DIRECTION('center_axis',(0.,0.,-1.));
#18045=DIRECTION('ref_axis',(-0.608852066092606,-0.793283783784066,0.));
#18046=DIRECTION('',(0.,0.,-1.));
#18047=DIRECTION('center_axis',(0.,0.,-1.));
#18048=DIRECTION('ref_axis',(-0.608852066092606,-0.793283783784066,0.));
#18049=DIRECTION('',(0.,0.,-1.));
#18050=DIRECTION('center_axis',(0.,0.,-1.));
#18051=DIRECTION('ref_axis',(-0.608852066092606,-0.793283783784066,0.));
#18052=DIRECTION('',(0.,0.,-1.));
#18053=DIRECTION('center_axis',(0.,0.,-1.));
#18054=DIRECTION('ref_axis',(-0.608852066092606,-0.793283783784066,0.));
#18055=DIRECTION('',(0.,0.,-1.));
#18056=DIRECTION('center_axis',(0.,0.,-1.));
#18057=DIRECTION('ref_axis',(-0.608852066092606,-0.793283783784066,0.));
#18058=DIRECTION('',(0.,0.,-1.));
#18059=DIRECTION('center_axis',(0.,0.,-1.));
#18060=DIRECTION('ref_axis',(-0.608852066092606,-0.793283783784066,0.));
#18061=DIRECTION('',(0.,0.,-1.));
#18062=DIRECTION('center_axis',(0.,0.,-1.));
#18063=DIRECTION('ref_axis',(-0.608852066092606,-0.793283783784066,0.));
#18064=DIRECTION('',(0.,0.,-1.));
#18065=DIRECTION('center_axis',(0.,0.,-1.));
#18066=DIRECTION('ref_axis',(-0.608852066092606,-0.793283783784066,0.));
#18067=DIRECTION('',(0.,0.,-1.));
#18068=DIRECTION('center_axis',(0.,0.,-1.));
#18069=DIRECTION('ref_axis',(-0.608852066092606,-0.793283783784066,0.));
#18070=DIRECTION('',(0.,0.,-1.));
#18071=DIRECTION('center_axis',(0.,0.,-1.));
#18072=DIRECTION('ref_axis',(1.,-4.78333543045355E-14,0.));
#18073=DIRECTION('center_axis',(0.,0.,-1.));
#18074=DIRECTION('ref_axis',(0.937755905787258,-0.347295063542687,0.));
#18075=DIRECTION('',(0.,0.,-1.));
#18076=DIRECTION('center_axis',(0.,0.,1.));
#18077=DIRECTION('ref_axis',(1.,0.,0.));
#18078=DIRECTION('',(0.,0.,-1.));
#18079=DIRECTION('center_axis',(0.,0.,1.));
#18080=DIRECTION('ref_axis',(1.,0.,0.));
#18081=DIRECTION('center_axis',(0.,0.,1.));
#18082=DIRECTION('ref_axis',(1.,0.,0.));
#18083=DIRECTION('center_axis',(0.,0.,-1.));
#18084=DIRECTION('ref_axis',(0.937755905787258,-0.347295063542687,0.));
#18085=DIRECTION('',(0.,0.,-1.));
#18086=DIRECTION('center_axis',(0.,0.,-1.));
#18087=DIRECTION('ref_axis',(0.937755905787258,-0.347295063542687,0.));
#18088=DIRECTION('',(0.,0.,-1.));
#18089=DIRECTION('center_axis',(0.,0.,-1.));
#18090=DIRECTION('ref_axis',(0.937755905787258,-0.347295063542687,0.));
#18091=DIRECTION('',(0.,0.,-1.));
#18092=DIRECTION('center_axis',(0.,0.,-1.));
#18093=DIRECTION('ref_axis',(0.937755905787258,-0.347295063542687,0.));
#18094=DIRECTION('',(0.,0.,-1.));
#18095=DIRECTION('center_axis',(0.,0.,-1.));
#18096=DIRECTION('ref_axis',(0.937755905787258,-0.347295063542687,0.));
#18097=DIRECTION('',(0.,0.,-1.));
#18098=DIRECTION('center_axis',(0.,0.,-1.));
#18099=DIRECTION('ref_axis',(0.937755905787258,-0.347295063542687,0.));
#18100=DIRECTION('',(0.,0.,-1.));
#18101=DIRECTION('center_axis',(0.,0.,-1.));
#18102=DIRECTION('ref_axis',(0.937755905787258,-0.347295063542687,0.));
#18103=DIRECTION('',(0.,0.,-1.));
#18104=DIRECTION('center_axis',(0.,0.,-1.));
#18105=DIRECTION('ref_axis',(0.937755905787258,-0.347295063542687,0.));
#18106=DIRECTION('',(0.,0.,-1.));
#18107=DIRECTION('center_axis',(0.,0.,-1.));
#18108=DIRECTION('ref_axis',(0.857775134428094,-0.514025114908664,0.));
#18109=DIRECTION('',(0.,0.,-1.));
#18110=DIRECTION('center_axis',(0.,0.,-1.));
#18111=DIRECTION('ref_axis',(1.,0.,0.));
#18112=DIRECTION('center_axis',(0.,0.,-1.));
#18113=DIRECTION('ref_axis',(-0.60885499756405,-0.793281533846138,0.));
#18114=DIRECTION('',(0.,0.,-1.));
#18115=DIRECTION('center_axis',(0.,0.,1.));
#18116=DIRECTION('ref_axis',(1.,-4.78333543045355E-14,0.));
#18117=DIRECTION('center_axis',(0.,0.,-1.));
#18118=DIRECTION('ref_axis',(-0.60885499756405,-0.793281533846138,0.));
#18119=DIRECTION('',(0.,0.,-1.));
#18120=DIRECTION('center_axis',(0.,0.,-1.));
#18121=DIRECTION('ref_axis',(-0.60885499756405,-0.793281533846138,0.));
#18122=DIRECTION('',(0.,0.,-1.));
#18123=DIRECTION('center_axis',(0.,0.,-1.));
#18124=DIRECTION('ref_axis',(-0.60885499756405,-0.793281533846138,0.));
#18125=DIRECTION('',(0.,0.,-1.));
#18126=DIRECTION('center_axis',(0.,0.,-1.));
#18127=DIRECTION('ref_axis',(-0.60885499756405,-0.793281533846138,0.));
#18128=DIRECTION('',(0.,0.,-1.));
#18129=DIRECTION('center_axis',(0.,0.,-1.));
#18130=DIRECTION('ref_axis',(-0.60885499756405,-0.793281533846138,0.));
#18131=DIRECTION('',(0.,0.,-1.));
#18132=DIRECTION('center_axis',(0.,0.,-1.));
#18133=DIRECTION('ref_axis',(-0.60885499756405,-0.793281533846138,0.));
#18134=DIRECTION('',(0.,0.,-1.));
#18135=DIRECTION('center_axis',(0.,0.,-1.));
#18136=DIRECTION('ref_axis',(-0.60885499756405,-0.793281533846138,0.));
#18137=DIRECTION('',(0.,0.,-1.));
#18138=DIRECTION('center_axis',(0.,0.,-1.));
#18139=DIRECTION('ref_axis',(-0.60885499756405,-0.793281533846138,0.));
#18140=DIRECTION('',(0.,0.,-1.));
#18141=DIRECTION('center_axis',(0.,0.,-1.));
#18142=DIRECTION('ref_axis',(-0.60885499756405,-0.793281533846138,0.));
#18143=DIRECTION('',(0.,0.,-1.));
#18144=DIRECTION('center_axis',(0.,0.,-1.));
#18145=DIRECTION('ref_axis',(1.,-4.78333543045355E-14,0.));
#18146=DIRECTION('center_axis',(0.,0.,-1.));
#18147=DIRECTION('ref_axis',(0.93775354145692,-0.347301447571133,0.));
#18148=DIRECTION('',(0.,0.,-1.));
#18149=DIRECTION('center_axis',(0.,0.,1.));
#18150=DIRECTION('ref_axis',(1.,0.,0.));
#18151=DIRECTION('',(0.,0.,-1.));
#18152=DIRECTION('center_axis',(0.,0.,1.));
#18153=DIRECTION('ref_axis',(1.,0.,0.));
#18154=DIRECTION('center_axis',(0.,0.,1.));
#18155=DIRECTION('ref_axis',(1.,0.,0.));
#18156=DIRECTION('center_axis',(0.,0.,-1.));
#18157=DIRECTION('ref_axis',(0.93775354145692,-0.347301447571133,0.));
#18158=DIRECTION('',(0.,0.,-1.));
#18159=DIRECTION('center_axis',(0.,0.,-1.));
#18160=DIRECTION('ref_axis',(0.93775354145692,-0.347301447571133,0.));
#18161=DIRECTION('',(0.,0.,-1.));
#18162=DIRECTION('center_axis',(0.,0.,-1.));
#18163=DIRECTION('ref_axis',(0.93775354145692,-0.347301447571133,0.));
#18164=DIRECTION('',(0.,0.,-1.));
#18165=DIRECTION('center_axis',(0.,0.,-1.));
#18166=DIRECTION('ref_axis',(0.93775354145692,-0.347301447571133,0.));
#18167=DIRECTION('',(0.,0.,-1.));
#18168=DIRECTION('center_axis',(0.,0.,-1.));
#18169=DIRECTION('ref_axis',(0.93775354145692,-0.347301447571133,0.));
#18170=DIRECTION('',(0.,0.,-1.));
#18171=DIRECTION('center_axis',(0.,0.,-1.));
#18172=DIRECTION('ref_axis',(0.93775354145692,-0.347301447571133,0.));
#18173=DIRECTION('',(0.,0.,-1.));
#18174=DIRECTION('center_axis',(0.,0.,-1.));
#18175=DIRECTION('ref_axis',(0.93775354145692,-0.347301447571133,0.));
#18176=DIRECTION('',(0.,0.,-1.));
#18177=DIRECTION('center_axis',(0.,0.,-1.));
#18178=DIRECTION('ref_axis',(0.93775354145692,-0.347301447571133,0.));
#18179=DIRECTION('',(0.,0.,-1.));
#18180=DIRECTION('center_axis',(0.,0.,-1.));
#18181=DIRECTION('ref_axis',(0.857796441547725,-0.513989557158567,0.));
#18182=DIRECTION('',(0.,0.,-1.));
#18183=DIRECTION('center_axis',(0.,0.,-1.));
#18184=DIRECTION('ref_axis',(1.,0.,0.));
#18185=DIRECTION('center_axis',(0.,0.,-1.));
#18186=DIRECTION('ref_axis',(0.93775354145692,-0.347301447571133,0.));
#18187=DIRECTION('center_axis',(0.,0.,-1.));
#18188=DIRECTION('ref_axis',(-0.60885499756405,-0.793281533846138,0.));
#18189=DIRECTION('center_axis',(0.,0.,-1.));
#18190=DIRECTION('ref_axis',(0.937755905787258,-0.347295063542687,0.));
#18191=DIRECTION('center_axis',(0.,0.,-1.));
#18192=DIRECTION('ref_axis',(-0.608852066092606,-0.793283783784066,0.));
#18193=DIRECTION('center_axis',(0.,0.,-1.));
#18194=DIRECTION('ref_axis',(0.937753558233112,-0.347301402273498,0.));
#18195=DIRECTION('center_axis',(0.,0.,-1.));
#18196=DIRECTION('ref_axis',(-0.608854967610821,-0.793281556835671,0.));
#18197=DIRECTION('center_axis',(0.,0.,-1.));
#18198=DIRECTION('ref_axis',(0.937755906520935,-0.347295061561634,0.));
#18199=DIRECTION('center_axis',(0.,0.,-1.));
#18200=DIRECTION('ref_axis',(-0.608852061413682,-0.79328378737518,0.));
#18201=DIRECTION('center_axis',(0.,0.,1.));
#18202=DIRECTION('ref_axis',(1.,0.,0.));
#18203=DIRECTION('center_axis',(0.,0.,1.));
#18204=DIRECTION('ref_axis',(1.,0.,0.));
#18205=DIRECTION('center_axis',(0.,0.,1.));
#18206=DIRECTION('ref_axis',(1.,0.,0.));
#18207=DIRECTION('center_axis',(0.,0.,1.));
#18208=DIRECTION('ref_axis',(1.,0.,0.));
#18209=DIRECTION('center_axis',(0.,0.,-1.));
#18210=DIRECTION('ref_axis',(1.,0.,0.));
#18211=DIRECTION('center_axis',(0.,0.,-1.));
#18212=DIRECTION('ref_axis',(1.,0.,0.));
#18213=DIRECTION('center_axis',(0.,0.,-1.));
#18214=DIRECTION('ref_axis',(1.,0.,0.));
#18215=DIRECTION('center_axis',(0.,0.,-1.));
#18216=DIRECTION('ref_axis',(1.,0.,0.));
#18217=DIRECTION('center_axis',(0.,0.,-1.));
#18218=DIRECTION('ref_axis',(1.,0.,0.));
#18219=DIRECTION('center_axis',(0.,0.,-1.));
#18220=DIRECTION('ref_axis',(1.,0.,0.));
#18221=DIRECTION('',(0.,0.,-1.));
#18222=DIRECTION('center_axis',(0.,0.,1.));
#18223=DIRECTION('ref_axis',(1.,0.,0.));
#18224=DIRECTION('center_axis',(0.,0.,-1.));
#18225=DIRECTION('ref_axis',(1.,0.,0.));
#18226=DIRECTION('center_axis',(0.,0.,-1.));
#18227=DIRECTION('ref_axis',(1.,0.,0.));
#18228=DIRECTION('',(0.,0.,-1.));
#18229=DIRECTION('center_axis',(0.,0.,1.));
#18230=DIRECTION('ref_axis',(1.,0.,0.));
#18231=DIRECTION('center_axis',(0.,0.,-1.));
#18232=DIRECTION('ref_axis',(1.,0.,0.));
#18233=DIRECTION('center_axis',(0.,0.,-1.));
#18234=DIRECTION('ref_axis',(1.,0.,0.));
#18235=DIRECTION('',(0.,0.,-1.));
#18236=DIRECTION('center_axis',(0.,0.,1.));
#18237=DIRECTION('ref_axis',(1.,0.,0.));
#18238=DIRECTION('center_axis',(0.,0.,-1.));
#18239=DIRECTION('ref_axis',(1.,0.,0.));
#18240=DIRECTION('center_axis',(0.,0.,-1.));
#18241=DIRECTION('ref_axis',(1.,0.,0.));
#18242=DIRECTION('',(0.,0.,-1.));
#18243=DIRECTION('center_axis',(0.,0.,1.));
#18244=DIRECTION('ref_axis',(1.,0.,0.));
#18245=DIRECTION('center_axis',(0.,1.,0.));
#18246=DIRECTION('ref_axis',(-1.,0.,0.));
#18247=DIRECTION('',(1.,0.,0.));
#18248=DIRECTION('',(0.,0.,1.));
#18249=DIRECTION('',(1.,0.,0.));
#18250=DIRECTION('',(0.,0.,1.));
#18251=DIRECTION('center_axis',(1.,0.,0.));
#18252=DIRECTION('ref_axis',(0.,1.,0.));
#18253=DIRECTION('',(0.,-1.,0.));
#18254=DIRECTION('',(0.,-1.,0.));
#18255=DIRECTION('',(0.,0.,-1.));
#18256=DIRECTION('center_axis',(0.,-1.,0.));
#18257=DIRECTION('ref_axis',(1.,0.,0.));
#18258=DIRECTION('',(-1.,0.,0.));
#18259=DIRECTION('',(-1.,0.,0.));
#18260=DIRECTION('',(0.,0.,-1.));
#18261=DIRECTION('center_axis',(-1.,0.,0.));
#18262=DIRECTION('ref_axis',(0.,-1.,0.));
#18263=DIRECTION('',(0.,1.,0.));
#18264=DIRECTION('',(0.,1.,0.));
#18265=DIRECTION('center_axis',(0.,0.,1.));
#18266=DIRECTION('ref_axis',(1.,0.,0.));
#18267=DIRECTION('center_axis',(0.,0.,1.));
#18268=DIRECTION('ref_axis',(1.,0.,0.));
#20213=CARTESIAN_POINT('',(0.,0.,0.));
#20214=CARTESIAN_POINT('Origin',(130.,-35.,32.7603849714045));
#20215=CARTESIAN_POINT('',(132.487160670875,-31.7594357285724,18.0469660640533));
#20216=CARTESIAN_POINT('',(132.487160670875,-31.7594357285724,17.9425407188119));
#20217=CARTESIAN_POINT('',(132.487160670875,-31.7594357285724,32.7603849714045));
#20218=CARTESIAN_POINT('',(125.917570547331,-35.0058571788241,17.1353849828742));
#20219=CARTESIAN_POINT('Ctrl Pts',(132.487160670875,-31.7594357285724,17.9425407188119));
#20220=CARTESIAN_POINT('Ctrl Pts',(132.581704114026,-31.8319986262038,17.9367376621138));
#20221=CARTESIAN_POINT('Ctrl Pts',(132.673155474161,-31.9087684968269,17.9309346054157));
#20222=CARTESIAN_POINT('Ctrl Pts',(132.761122894562,-31.9894476651075,17.9251315487176));
#20223=CARTESIAN_POINT('Ctrl Pts',(132.849041174532,-32.0700817643262,17.9193317337277));
#20224=CARTESIAN_POINT('Ctrl Pts',(132.933479084742,-32.1546205419903,17.9135319187378));
#20225=CARTESIAN_POINT('Ctrl Pts',(133.014078024373,-32.2427262263259,17.907732103748));
#20226=CARTESIAN_POINT('Ctrl Pts',(133.094654120592,-32.3308069396815,17.901933932546));
#20227=CARTESIAN_POINT('Ctrl Pts',(133.171393133673,-32.4224522480155,17.8961357613441));
#20228=CARTESIAN_POINT('Ctrl Pts',(133.243973935598,-32.5172881550293,17.8903375901422));
#20229=CARTESIAN_POINT('Ctrl Pts',(133.316551380068,-32.6121196751058,17.8845396871532));
#20230=CARTESIAN_POINT('Ctrl Pts',(133.384970747326,-32.7101411753726,17.8787417841642));
#20231=CARTESIAN_POINT('Ctrl Pts',(133.448952172999,-32.8109468009291,17.8729438811751));
#20232=CARTESIAN_POINT('Ctrl Pts',(133.512945812966,-32.9117716706553,17.8671448713448));
#20233=CARTESIAN_POINT('Ctrl Pts',(133.572499607407,-33.0153813771399,17.8613458615145));
#20234=CARTESIAN_POINT('Ctrl Pts',(133.627378224929,-33.1213429761359,17.8555468516842));
#20235=CARTESIAN_POINT('Ctrl Pts',(133.682314579367,-33.2274160556359,17.8497417408083));
#20236=CARTESIAN_POINT('Ctrl Pts',(133.732565744311,-33.3358456058072,17.8439366299325));
#20237=CARTESIAN_POINT('Ctrl Pts',(133.777943289161,-33.4461758452515,17.8381315190567));
#20238=CARTESIAN_POINT('Ctrl Pts',(133.823345287127,-33.5565655396092,17.8323232799146));
#20239=CARTESIAN_POINT('Ctrl Pts',(133.863868294095,-33.6688575789527,17.8265150407725));
#20240=CARTESIAN_POINT('Ctrl Pts',(133.899373395709,-33.7825797271113,17.8207068016304));
#20241=CARTESIAN_POINT('Ctrl Pts',(133.934935743661,-33.896485234177,17.8148891976249));
#20242=CARTESIAN_POINT('Ctrl Pts',(133.965463916952,-34.0118250612506,17.8090715936195));
#20243=CARTESIAN_POINT('Ctrl Pts',(133.990869754237,-34.1281149131264,17.803253989614));
#20244=CARTESIAN_POINT('Ctrl Pts',(134.012612161228,-34.2276361869148,17.7982752631673));
#20245=CARTESIAN_POINT('Ctrl Pts',(134.030603812871,-34.3278529548629,17.7932965367205));
#20246=CARTESIAN_POINT('Ctrl Pts',(134.044819691244,-34.4284593931121,17.7883178102738));
#20247=CARTESIAN_POINT('Ctrl Pts',(134.06147525078,-34.546331569412,17.7824846515646));
#20248=CARTESIAN_POINT('Ctrl Pts',(134.073000536758,-34.6651195996746,17.7766514928553));
#20249=CARTESIAN_POINT('Ctrl Pts',(134.079303348713,-34.7843401076304,17.7708183341461));
#20250=CARTESIAN_POINT('Ctrl Pts',(134.085598203868,-34.903410109157,17.7649925393368));
#20251=CARTESIAN_POINT('Ctrl Pts',(134.086683677878,-35.0229110995942,17.7591667445275));
#20252=CARTESIAN_POINT('Ctrl Pts',(134.082518952074,-35.1423516981127,17.7533409497181));
#20253=CARTESIAN_POINT('Ctrl Pts',(134.078358408253,-35.2616723611382,17.7475210048424));
#20254=CARTESIAN_POINT('Ctrl Pts',(134.068958167338,-35.3809323485755,17.7417010599667));
#20255=CARTESIAN_POINT('Ctrl Pts',(134.05432940372,-35.4996379550549,17.735881115091));
#20256=CARTESIAN_POINT('Ctrl Pts',(134.039180744297,-35.6225622739632,17.7298543335333));
#20257=CARTESIAN_POINT('Ctrl Pts',(134.018424994074,-35.7448916310486,17.7238275519756));
#20258=CARTESIAN_POINT('Ctrl Pts',(133.992133470621,-35.8660804539682,17.7178007704178));
#20259=CARTESIAN_POINT('Ctrl Pts',(133.966773358858,-35.9829760039448,17.7119874954985));
#20260=CARTESIAN_POINT('Ctrl Pts',(133.936263133592,-36.0988100265722,17.7061742205792));
#20261=CARTESIAN_POINT('Ctrl Pts',(133.900719114567,-36.2131015576818,17.7003609456598));
#20262=CARTESIAN_POINT('Ctrl Pts',(133.86518073122,-36.3273749673099,17.6945485924637));
#20263=CARTESIAN_POINT('Ctrl Pts',(133.824610262327,-36.4401059834592,17.6887362392676));
#20264=CARTESIAN_POINT('Ctrl Pts',(133.779174025344,-36.5508283870779,17.6829238860714));
#20265=CARTESIAN_POINT('Ctrl Pts',(133.733734366207,-36.6615591300547,17.6771110951021));
#20266=CARTESIAN_POINT('Ctrl Pts',(133.683428364855,-36.7702805833146,17.6712983041329));
#20267=CARTESIAN_POINT('Ctrl Pts',(133.628470409577,-36.8765466918841,17.6654855131636));
#20268=CARTESIAN_POINT('Ctrl Pts',(133.573495461997,-36.9828456565877,17.659670924953));
#20269=CARTESIAN_POINT('Ctrl Pts',(133.513865886678,-37.0866874055096,17.6538563367424));
#20270=CARTESIAN_POINT('Ctrl Pts',(133.449841614988,-37.1876512134011,17.6480417485318));
#20271=CARTESIAN_POINT('Ctrl Pts',(133.385748439847,-37.2887236793802,17.6422209026132));
#20272=CARTESIAN_POINT('Ctrl Pts',(133.317251345423,-37.3869116779491,17.6364000566945));
#20273=CARTESIAN_POINT('Ctrl Pts',(133.244653204869,-37.4818240429435,17.6305792107758));
#20274=CARTESIAN_POINT('Ctrl Pts',(133.172008572249,-37.5767971900996,17.6247546371701));
#20275=CARTESIAN_POINT('Ctrl Pts',(133.095257923063,-37.6684902141337,17.6189300635644));
#20276=CARTESIAN_POINT('Ctrl Pts',(133.014742893228,-37.7565468049227,17.6131054899586));
#20277=CARTESIAN_POINT('Ctrl Pts',(132.934115448857,-37.8447263397244,17.6072727841229));
#20278=CARTESIAN_POINT('Ctrl Pts',(132.849713419676,-37.9292590201806,17.6014400782871));
#20279=CARTESIAN_POINT('Ctrl Pts',(132.761913655608,-38.0098268985053,17.5956073724513));
#20280=CARTESIAN_POINT('Ctrl Pts',(132.739991385184,-38.0299434766635,17.5941510342027));
#20281=CARTESIAN_POINT('Ctrl Pts',(132.717857442463,-38.049813083404,17.592694695954));
#20282=CARTESIAN_POINT('Ctrl Pts',(132.695517984647,-38.0694311841847,17.5912383577053));
#20283=CARTESIAN_POINT('Ctrl Pts',(132.606178986837,-38.1478870481142,17.585414232488));
#20284=CARTESIAN_POINT('Ctrl Pts',(132.513269708122,-38.2225640338864,17.5795901072706));
#20285=CARTESIAN_POINT('Ctrl Pts',(132.417143086002,-38.2931207542073,17.5737659820533));
#20286=CARTESIAN_POINT('Ctrl Pts',(132.321136103841,-38.363589659073,17.5679491055885));
#20287=CARTESIAN_POINT('Ctrl Pts',(132.221920069128,-38.4299482589507,17.5621322291238));
#20288=CARTESIAN_POINT('Ctrl Pts',(132.119882780823,-38.4918937549089,17.556315352659));
#20289=CARTESIAN_POINT('Ctrl Pts',(132.017945927415,-38.5537782781614,17.5505042017226));
#20290=CARTESIAN_POINT('Ctrl Pts',(131.91319369184,-38.6112581284909,17.5446930507863));
#20291=CARTESIAN_POINT('Ctrl Pts',(131.806044305422,-38.6640727294711,17.5388818998499));
#20292=CARTESIAN_POINT('Ctrl Pts',(131.694857351711,-38.7188774725572,17.5328517750702));
#20293=CARTESIAN_POINT('Ctrl Pts',(131.581089398034,-38.7686581968064,17.5268216502905));
#20294=CARTESIAN_POINT('Ctrl Pts',(131.465237969362,-38.8131748836292,17.5207915255108));
#20295=CARTESIAN_POINT('Ctrl Pts',(131.353714643256,-38.8560284680744,17.5149866806334));
#20296=CARTESIAN_POINT('Ctrl Pts',(131.240261138487,-38.8940041214257,17.509181835756));
#20297=CARTESIAN_POINT('Ctrl Pts',(131.125342649476,-38.9269363276312,17.5033769908786));
#20298=CARTESIAN_POINT('Ctrl Pts',(131.010439464464,-38.9598641481678,17.4975729190477));
#20299=CARTESIAN_POINT('Ctrl Pts',(130.894072075446,-38.987749744817,17.4917688472168));
#20300=CARTESIAN_POINT('Ctrl Pts',(130.776720674511,-39.0104775269021,17.485964775386));
#20301=CARTESIAN_POINT('Ctrl Pts',(130.65935724065,-39.0332076394386,17.4801601084197));
#20302=CARTESIAN_POINT('Ctrl Pts',(130.541009994955,-39.0507788081581,17.4743554414534));
#20303=CARTESIAN_POINT('Ctrl Pts',(130.422168519274,-39.0631267198223,17.4685507744871));
#20304=CARTESIAN_POINT('Ctrl Pts',(130.303286845885,-39.0754788081238,17.4627441441129));
#20305=CARTESIAN_POINT('Ctrl Pts',(130.18391101576,-39.0826040834041,17.4569375137386));
#20306=CARTESIAN_POINT('Ctrl Pts',(130.06453427578,-39.0844902163244,17.4511308833643));
#20307=CARTESIAN_POINT('Ctrl Pts',(129.945023028346,-39.0863784744404,17.4453177103833));
#20308=CARTESIAN_POINT('Ctrl Pts',(129.825511277327,-39.083015800483,17.4395045374023));
#20309=CARTESIAN_POINT('Ctrl Pts',(129.70649098094,-39.0744419809013,17.4336913644213));
#20310=CARTESIAN_POINT('Ctrl Pts',(129.587391143467,-39.0658624314486,17.4278743065054));
#20311=CARTESIAN_POINT('Ctrl Pts',(129.468783819143,-39.0520648478111,17.4220572485895));
#20312=CARTESIAN_POINT('Ctrl Pts',(129.351152907099,-39.0331405195001,17.4162401906737));
#20313=CARTESIAN_POINT('Ctrl Pts',(129.233351764959,-39.0141888047636,17.4104147145767));
#20314=CARTESIAN_POINT('Ctrl Pts',(129.11653025366,-38.9900956192539,17.4045892384796));
#20315=CARTESIAN_POINT('Ctrl Pts',(129.001159350494,-38.9610026958958,17.3987637623826));
#20316=CARTESIAN_POINT('Ctrl Pts',(128.970760316404,-38.9533370129145,17.3972288099674));
#20317=CARTESIAN_POINT('Ctrl Pts',(128.940461894974,-38.9453244773613,17.3956938575521));
#20318=CARTESIAN_POINT('Ctrl Pts',(128.910272476765,-38.9369682402966,17.3941589051369));
#20319=CARTESIAN_POINT('Ctrl Pts',(128.7966252111,-38.9055114070744,17.3883806174033));
#20320=CARTESIAN_POINT('Ctrl Pts',(128.684141526411,-38.8690742365292,17.3826023296697));
#20321=CARTESIAN_POINT('Ctrl Pts',(128.573294774159,-38.8277587696401,17.3768240419362));
#20322=CARTESIAN_POINT('Ctrl Pts',(128.462589215034,-38.7864959291011,17.3710531144048));
#20323=CARTESIAN_POINT('Ctrl Pts',(128.353516828246,-38.7403672904179,17.3652821868735));
#20324=CARTESIAN_POINT('Ctrl Pts',(128.246538336773,-38.6895253347269,17.3595112593422));
#20325=CARTESIAN_POINT('Ctrl Pts',(128.139667079847,-38.6387343426837,17.3537461165513));
#20326=CARTESIAN_POINT('Ctrl Pts',(128.03488591716,-38.583239606427,17.3479809737605));
#20327=CARTESIAN_POINT('Ctrl Pts',(127.932637365784,-38.5232423616104,17.3422158309696));
#20328=CARTESIAN_POINT('Ctrl Pts',(127.825383702245,-38.4603082249189,17.3361684818696));
#20329=CARTESIAN_POINT('Ctrl Pts',(127.72091732099,-38.3924197627085,17.3301211327695));
#20330=CARTESIAN_POINT('Ctrl Pts',(127.619722083475,-38.3198647623211,17.3240737836695));
#20331=CARTESIAN_POINT('Ctrl Pts',(127.523352525227,-38.2507696793152,17.3183148134289));
#20332=CARTESIAN_POINT('Ctrl Pts',(127.429949706546,-38.1774431219199,17.3125558431884));
#20333=CARTESIAN_POINT('Ctrl Pts',(127.339902590464,-38.1001785064379,17.3067968729478));
#20334=CARTESIAN_POINT('Ctrl Pts',(127.249865669562,-38.0229226388944,17.3010385547408));
#20335=CARTESIAN_POINT('Ctrl Pts',(127.163184011491,-37.941729869919,17.2952802365337));
#20336=CARTESIAN_POINT('Ctrl Pts',(127.080213109896,-37.8569335862734,17.2895219183267));
#20337=CARTESIAN_POINT('Ctrl Pts',(126.997231227526,-37.7721260802728,17.2837628380356));
#20338=CARTESIAN_POINT('Ctrl Pts',(126.917961368612,-37.6837144084915,17.2780037577445));
#20339=CARTESIAN_POINT('Ctrl Pts',(126.842721276515,-37.5920679123491,17.2722446774535));
#20340=CARTESIAN_POINT('Ctrl Pts',(126.767452749201,-37.5003867805764,17.2664834206539));
#20341=CARTESIAN_POINT('Ctrl Pts',(126.696217280093,-37.4054687147629,17.2607221638544));
#20342=CARTESIAN_POINT('Ctrl Pts',(126.629291074734,-37.3077145276516,17.2549609070549));
#20343=CARTESIAN_POINT('Ctrl Pts',(126.562282534711,-37.2098400803499,17.249192562581));
#20344=CARTESIAN_POINT('Ctrl Pts',(126.499594073982,-37.1091228910951,17.2434242181072));
#20345=CARTESIAN_POINT('Ctrl Pts',(126.441457524535,-37.0059911391414,17.2376558736334));
#20346=CARTESIAN_POINT('Ctrl Pts',(126.383279228692,-36.9027853308665,17.2318833870562));
#20347=CARTESIAN_POINT('Ctrl Pts',(126.329659537295,-36.7971618781968,17.2261109004791));
#20348=CARTESIAN_POINT('Ctrl Pts',(126.280782651279,-36.6895701562747,17.220338413902));
#20349=CARTESIAN_POINT('Ctrl Pts',(126.231828296463,-36.5818079038151,17.2145567780592));
#20350=CARTESIAN_POINT('Ctrl Pts',(126.18763190295,-36.4720715400648,17.2087751422165));
#20351=CARTESIAN_POINT('Ctrl Pts',(126.148328293113,-36.3608269773817,17.2029935063738));
#20352=CARTESIAN_POINT('Ctrl Pts',(126.134927030354,-36.3228961709946,17.2010221551053));
#20353=CARTESIAN_POINT('Ctrl Pts',(126.122094161038,-36.2847901185301,17.1990508038369));
#20354=CARTESIAN_POINT('Ctrl Pts',(126.10983366812,-36.2465275409332,17.1970794525685));
#20355=CARTESIAN_POINT('Ctrl Pts',(126.063947737475,-36.103326611438,17.1897015038852));
#20356=CARTESIAN_POINT('Ctrl Pts',(126.02595987326,-35.9575499236023,17.1823235552019));
#20357=CARTESIAN_POINT('Ctrl Pts',(125.996104768623,-35.8099678858821,17.1749456065186));
#20358=CARTESIAN_POINT('Ctrl Pts',(125.966727677199,-35.6647487996489,17.1676857869456));
#20359=CARTESIAN_POINT('Ctrl Pts',(125.945224957893,-35.5177815783573,17.1604259673726));
#20360=CARTESIAN_POINT('Ctrl Pts',(125.931774609395,-35.369820458114,17.1531661477996));
#20361=CARTESIAN_POINT('Ctrl Pts',(125.920793500128,-35.2490223071195,17.1472390989943));
#20362=CARTESIAN_POINT('Ctrl Pts',(125.915178823828,-35.1275620126132,17.141312050189));
#20363=CARTESIAN_POINT('Ctrl Pts',(125.915004204916,-35.0058612407387,17.1353850013836));
#20364=CARTESIAN_POINT('',(126.824949217806,-32.429732011932,17.));
#20365=CARTESIAN_POINT('Ctrl Pts',(125.919160822134,-35.0058546617942,17.1353849714045));
#20366=CARTESIAN_POINT('Ctrl Pts',(125.92665513971,-34.0801598293983,17.090256647603));
#20367=CARTESIAN_POINT('Ctrl Pts',(126.2419104066,-33.1499595688096,17.0451283238015));
#20368=CARTESIAN_POINT('Ctrl Pts',(126.824949217806,-32.429732011932,17.));
#20369=CARTESIAN_POINT('',(128.537425967084,-31.1858025486036,17.0000001263181));
#20370=CARTESIAN_POINT('Origin',(130.,-35.,17.));
#20371=CARTESIAN_POINT('',(125.915001286748,-34.9967576658375,17.239615028553));
#20372=CARTESIAN_POINT('Ctrl Pts',(125.915001286748,-34.9967576658375,17.239615028553));
#20373=CARTESIAN_POINT('Ctrl Pts',(125.915121830798,-34.84488488998,17.2322214958407));
#20374=CARTESIAN_POINT('Ctrl Pts',(125.923715533729,-34.6933711864996,17.2248279631283));
#20375=CARTESIAN_POINT('Ctrl Pts',(125.940640899099,-34.5430222216247,17.217434430416));
#20376=CARTESIAN_POINT('Ctrl Pts',(125.957898968693,-34.3897178265603,17.2098955620188));
#20377=CARTESIAN_POINT('Ctrl Pts',(125.983819475205,-34.2376241677412,17.2023566936216));
#20378=CARTESIAN_POINT('Ctrl Pts',(126.018203886763,-34.0875720781268,17.1948178252245));
#20379=CARTESIAN_POINT('Ctrl Pts',(126.025778474723,-34.0545169028373,17.1931570778334));
#20380=CARTESIAN_POINT('Ctrl Pts',(126.033763617093,-34.0215607216557,17.1914963304423));
#20381=CARTESIAN_POINT('Ctrl Pts',(126.042156880036,-33.9887122873517,17.1898355830512));
#20382=CARTESIAN_POINT('Ctrl Pts',(126.071413140095,-33.8742130344265,17.1840467428947));
#20383=CARTESIAN_POINT('Ctrl Pts',(126.105691644772,-33.7607909591982,17.1782579027383));
#20384=CARTESIAN_POINT('Ctrl Pts',(126.144897526267,-33.6489226828134,17.1724690625818));
#20385=CARTESIAN_POINT('Ctrl Pts',(126.184054424549,-33.5371941728955,17.1666874549112));
#20386=CARTESIAN_POINT('Ctrl Pts',(126.228126322497,-33.4270159884914,17.1609058472407));
#20387=CARTESIAN_POINT('Ctrl Pts',(126.27696771855,-33.3188528823207,17.1551242395702));
#20388=CARTESIAN_POINT('Ctrl Pts',(126.325761225946,-33.2107958293414,17.1493483007267));
#20389=CARTESIAN_POINT('Ctrl Pts',(126.379314761018,-33.1047502998445,17.1435723618833));
#20390=CARTESIAN_POINT('Ctrl Pts',(126.437433784762,-33.0011635979796,17.1377964230398));
#20391=CARTESIAN_POINT('Ctrl Pts',(126.495513134357,-32.8976476081448,17.1320244270612));
#20392=CARTESIAN_POINT('Ctrl Pts',(126.558151571977,-32.7965874670979,17.1262524310825));
#20393=CARTESIAN_POINT('Ctrl Pts',(126.625107719851,-32.6984077039163,17.1204804351039));
#20394=CARTESIAN_POINT('Ctrl Pts',(126.692039837253,-32.600263177322,17.1147105106869));
#20395=CARTESIAN_POINT('Ctrl Pts',(126.763286351737,-32.5049973150308,17.10894058627));
#20396=CARTESIAN_POINT('Ctrl Pts',(126.838561805029,-32.4130068536275,17.1031706618531));
#20397=CARTESIAN_POINT('Ctrl Pts',(126.913828561771,-32.3210270198548,17.0974014040338));
#20398=CARTESIAN_POINT('Ctrl Pts',(126.993123069758,-32.2323221546499,17.0916321462146));
#20399=CARTESIAN_POINT('Ctrl Pts',(127.076119165966,-32.1472564313688,17.0858628883953));
#20400=CARTESIAN_POINT('Ctrl Pts',(127.159125872678,-32.062179832995,17.0800928930144));
#20401=CARTESIAN_POINT('Ctrl Pts',(127.245834819185,-31.980743597332,17.0743228976335));
#20402=CARTESIAN_POINT('Ctrl Pts',(127.335883040552,-31.9032749837315,17.0685529022526));
#20403=CARTESIAN_POINT('Ctrl Pts',(127.426020987657,-31.8257291789507,17.0627771575401));
#20404=CARTESIAN_POINT('Ctrl Pts',(127.519504541578,-31.7521591633589,17.0570014128275));
#20405=CARTESIAN_POINT('Ctrl Pts',(127.615937561779,-31.6828519341666,17.0512256681149));
#20406=CARTESIAN_POINT('Ctrl Pts',(127.712418239099,-31.6135104533982,17.045447069034));
#20407=CARTESIAN_POINT('Ctrl Pts',(127.811850939971,-31.5484361819415,17.0396684699532));
#20408=CARTESIAN_POINT('Ctrl Pts',(127.913811980347,-31.4878717923949,17.0338898708723));
#20409=CARTESIAN_POINT('Ctrl Pts',(128.01593821576,-31.4272092777552,17.0281019094322));
#20410=CARTESIAN_POINT('Ctrl Pts',(128.120600610571,-31.3710714403544,17.022313947992));
#20411=CARTESIAN_POINT('Ctrl Pts',(128.227351924597,-31.3196543911246,17.0165259865519));
#20412=CARTESIAN_POINT('Ctrl Pts',(128.328951155668,-31.2707188561064,17.011017366474));
#20413=CARTESIAN_POINT('Ctrl Pts',(128.432442089675,-31.2260591674412,17.005508746396));
#20414=CARTESIAN_POINT('Ctrl Pts',(128.537425967084,-31.1858025486036,17.0000001263181));
#20415=CARTESIAN_POINT('Ctrl Pts',(132.487160670875,-31.7594357285724,18.0469660640533));
#20416=CARTESIAN_POINT('Ctrl Pts',(132.581995825681,-31.8322225173823,18.0411567048122));
#20417=CARTESIAN_POINT('Ctrl Pts',(132.673587188726,-31.9091404736677,18.035347345571));
#20418=CARTESIAN_POINT('Ctrl Pts',(132.761569405332,-31.9898572426657,18.0295379863299));
#20419=CARTESIAN_POINT('Ctrl Pts',(132.849596841011,-32.0706154966078,18.0237256413283));
#20420=CARTESIAN_POINT('Ctrl Pts',(132.934011145747,-32.1551761643168,18.0179132963266));
#20421=CARTESIAN_POINT('Ctrl Pts',(133.014484707895,-32.2431708529785,18.012100951325));
#20422=CARTESIAN_POINT('Ctrl Pts',(133.095089062964,-32.3313085585774,18.0062791595738));
#20423=CARTESIAN_POINT('Ctrl Pts',(133.171739614314,-32.4228911245167,18.0004573678227));
#20424=CARTESIAN_POINT('Ctrl Pts',(133.244149453117,-32.5175175074448,17.9946355760715));
#20425=CARTESIAN_POINT('Ctrl Pts',(133.31248306625,-32.6068170108013,17.989141515156));
#20426=CARTESIAN_POINT('Ctrl Pts',(133.377040197403,-32.6988267736018,17.9836474542405));
#20427=CARTESIAN_POINT('Ctrl Pts',(133.437616796849,-32.7931887806115,17.978153393325));
#20428=CARTESIAN_POINT('Ctrl Pts',(133.501837123684,-32.8932267323347,17.9723288605703));
#20429=CARTESIAN_POINT('Ctrl Pts',(133.561790445962,-32.9962314200498,17.9665043278156));
#20430=CARTESIAN_POINT('Ctrl Pts',(133.617191501953,-33.1018033194102,17.9606797950608));
#20431=CARTESIAN_POINT('Ctrl Pts',(133.672522646919,-33.2072419967683,17.9548626123294));
#20432=CARTESIAN_POINT('Ctrl Pts',(133.723312763425,-33.3152410840024,17.9490454295979));
#20433=CARTESIAN_POINT('Ctrl Pts',(133.769319907765,-33.4253722875156,17.9432282468664));
#20434=CARTESIAN_POINT('Ctrl Pts',(133.815280976368,-33.535393195628,17.9374168899907));
#20435=CARTESIAN_POINT('Ctrl Pts',(133.856468445744,-33.6475415975982,17.9316055331149));
#20436=CARTESIAN_POINT('Ctrl Pts',(133.892686630217,-33.7613653488906,17.9257941762391));
#20437=CARTESIAN_POINT('Ctrl Pts',(133.93026752783,-33.8794717312346,17.9197641664274));
#20438=CARTESIAN_POINT('Ctrl Pts',(133.962497647065,-33.9993816132568,17.9137341566156));
#20439=CARTESIAN_POINT('Ctrl Pts',(133.989213398485,-34.1205675345144,17.9077041468038));
#20440=CARTESIAN_POINT('Ctrl Pts',(134.014931373,-34.2372274174997,17.901899345126));
#20441=CARTESIAN_POINT('Ctrl Pts',(134.035539398504,-34.3550692997241,17.8960945434482));
#20442=CARTESIAN_POINT('Ctrl Pts',(134.050942750205,-34.4736086678504,17.8902897417704));
#20443=CARTESIAN_POINT('Ctrl Pts',(134.066343808017,-34.5921303829263,17.8844858045519));
#20444=CARTESIAN_POINT('Ctrl Pts',(134.076541680862,-34.7113489726554,17.8786818673334));
#20445=CARTESIAN_POINT('Ctrl Pts',(134.081493237234,-34.8307724773791,17.8728779301149));
#20446=CARTESIAN_POINT('Ctrl Pts',(134.086445223776,-34.9502063570867,17.867073488676));
#20447=CARTESIAN_POINT('Ctrl Pts',(134.086149970745,-35.0698447793198,17.8612690472372));
#20448=CARTESIAN_POINT('Ctrl Pts',(134.080616448311,-35.1891940849229,17.8554646057984));
#20449=CARTESIAN_POINT('Ctrl Pts',(134.075081140371,-35.3085819010752,17.8496582914351));
#20450=CARTESIAN_POINT('Ctrl Pts',(134.06430422041,-35.4276800075163,17.8438519770719));
#20451=CARTESIAN_POINT('Ctrl Pts',(134.048346612716,-35.545998812552,17.8380456627087));
#20452=CARTESIAN_POINT('Ctrl Pts',(134.032371385358,-35.664448259837,17.8322329372769));
#20453=CARTESIAN_POINT('Ctrl Pts',(134.011204106662,-35.7821162833686,17.8264202118451));
#20454=CARTESIAN_POINT('Ctrl Pts',(133.984957050805,-35.898522288671,17.8206074864133));
#20455=CARTESIAN_POINT('Ctrl Pts',(133.958692800776,-36.0150045503334,17.8147909531257));
#20456=CARTESIAN_POINT('Ctrl Pts',(133.927342253215,-36.1302227543044,17.8089744198381));
#20457=CARTESIAN_POINT('Ctrl Pts',(133.891067426887,-36.2437118956641,17.8031578865505));
#20458=CARTESIAN_POINT('Ctrl Pts',(133.854740775171,-36.3573631775373,17.7973330432548));
#20459=CARTESIAN_POINT('Ctrl Pts',(133.813475943363,-36.4692800845744,17.791508199959));
#20460=CARTESIAN_POINT('Ctrl Pts',(133.767482925139,-36.5790178620857,17.7856833566632));
#20461=CARTESIAN_POINT('Ctrl Pts',(133.755350927817,-36.6079643951529,17.7841468846943));
#20462=CARTESIAN_POINT('Ctrl Pts',(133.742890192233,-36.636759442064,17.7826104127255));
#20463=CARTESIAN_POINT('Ctrl Pts',(133.730105093327,-36.6653951461247,17.7810739407566));
#20464=CARTESIAN_POINT('Ctrl Pts',(133.681642147958,-36.7739410847745,17.775249820221));
#20465=CARTESIAN_POINT('Ctrl Pts',(133.628359278819,-36.8805444906622,17.7694256996854));
#20466=CARTESIAN_POINT('Ctrl Pts',(133.570434298946,-36.9847478219934,17.7636015791498));
#20467=CARTESIAN_POINT('Ctrl Pts',(133.512582285387,-37.0888198915968,17.7577847950796));
#20468=CARTESIAN_POINT('Ctrl Pts',(133.450099988354,-37.1904975462668,17.7519680110093));
#20469=CARTESIAN_POINT('Ctrl Pts',(133.383213025757,-37.2893437099631,17.746151226939));
#20470=CARTESIAN_POINT('Ctrl Pts',(133.316392895301,-37.3880911085112,17.7403402548853));
#20471=CARTESIAN_POINT('Ctrl Pts',(133.245177082164,-37.4840123082296,17.7345292828316));
#20472=CARTESIAN_POINT('Ctrl Pts',(133.169836506206,-37.5766958539816,17.7287183107778));
#20473=CARTESIAN_POINT('Ctrl Pts',(133.091654118015,-37.672875380892,17.7226881515033));
#20474=CARTESIAN_POINT('Ctrl Pts',(133.009029889101,-37.7655678070874,17.7166579922287));
#20475=CARTESIAN_POINT('Ctrl Pts',(132.92231541916,-37.8543471391786,17.7106278329541));
#20476=CARTESIAN_POINT('Ctrl Pts',(132.838846628786,-37.9398035049379,17.7048233795479));
#20477=CARTESIAN_POINT('Ctrl Pts',(132.751588597142,-38.0216341246567,17.6990189261418));
#20478=CARTESIAN_POINT('Ctrl Pts',(132.660894654302,-38.099494255311,17.6932144727356));
#20479=CARTESIAN_POINT('Ctrl Pts',(132.570213999643,-38.1773429781525,17.687410869779));
#20480=CARTESIAN_POINT('Ctrl Pts',(132.476098744603,-38.2512221029872,17.6816072668224));
#20481=CARTESIAN_POINT('Ctrl Pts',(132.378936721682,-38.3208259626536,17.6758036638659));
#20482=CARTESIAN_POINT('Ctrl Pts',(132.281766017736,-38.3904360411364,17.6699995423814));
#20483=CARTESIAN_POINT('Ctrl Pts',(132.181548336559,-38.455769857223,17.664195420897));
#20484=CARTESIAN_POINT('Ctrl Pts',(132.078701484019,-38.5165643944533,17.6583912994125));
#20485=CARTESIAN_POINT('Ctrl Pts',(131.975821184969,-38.5773787024889,17.6525852903875));
#20486=CARTESIAN_POINT('Ctrl Pts',(131.870310365345,-38.633650588177,17.6467792813625));
#20487=CARTESIAN_POINT('Ctrl Pts',(131.76261189896,-38.6851627228176,17.6409732723375));
#20488=CARTESIAN_POINT('Ctrl Pts',(131.654794083567,-38.7367319420424,17.6351608292244));
#20489=CARTESIAN_POINT('Ctrl Pts',(131.544784150796,-38.7835307053043,17.6293483861113));
#20490=CARTESIAN_POINT('Ctrl Pts',(131.433045588882,-38.8253895671142,17.6235359429982));
#20491=CARTESIAN_POINT('Ctrl Pts',(131.321233573453,-38.8672759456601,17.6177196789627));
#20492=CARTESIAN_POINT('Ctrl Pts',(131.207691053125,-38.9042158295528,17.6119034149272));
#20493=CARTESIAN_POINT('Ctrl Pts',(131.092895733437,-38.9360899273054,17.6060871508917));
#20494=CARTESIAN_POINT('Ctrl Pts',(130.977935983922,-38.9680096806858,17.600262555791));
#20495=CARTESIAN_POINT('Ctrl Pts',(130.861720249722,-38.9948490735882,17.5944379606904));
#20496=CARTESIAN_POINT('Ctrl Pts',(130.744735586478,-39.0165400416568,17.5886133655897));
#20497=CARTESIAN_POINT('Ctrl Pts',(130.713812817997,-39.0222736546375,17.5870737397892));
#20498=CARTESIAN_POINT('Ctrl Pts',(130.682836344301,-39.0276478222182,17.5855341139886));
#20499=CARTESIAN_POINT('Ctrl Pts',(130.651815190333,-39.0326618947851,17.5839944881881));
#20500=CARTESIAN_POINT('Ctrl Pts',(130.534583268297,-39.0516105568768,17.578176094327));
#20501=CARTESIAN_POINT('Ctrl Pts',(130.416333240764,-39.0654738601746,17.5723577004659));
#20502=CARTESIAN_POINT('Ctrl Pts',(130.297544301261,-39.0741492840576,17.5665393066048));
#20503=CARTESIAN_POINT('Ctrl Pts',(130.178905628137,-39.0828137336484,17.5607282729322));
#20504=CARTESIAN_POINT('Ctrl Pts',(130.059729803323,-39.0863033265891,17.5549172392596));
#20505=CARTESIAN_POINT('Ctrl Pts',(129.940505181167,-39.0845667293523,17.549106205587));
#20506=CARTESIAN_POINT('Ctrl Pts',(129.821400146662,-39.0828318740006,17.5433010006422));
#20507=CARTESIAN_POINT('Ctrl Pts',(129.702246818913,-39.0758812624831,17.5374957956974));
#20508=CARTESIAN_POINT('Ctrl Pts',(129.583537018591,-39.0637154901784,17.5316905907525));
#20509=CARTESIAN_POINT('Ctrl Pts',(129.460183081588,-39.0510737714122,17.5256582759553));
#20510=CARTESIAN_POINT('Ctrl Pts',(129.337308532162,-39.0328004820631,17.5196259611581));
#20511=CARTESIAN_POINT('Ctrl Pts',(129.215463760267,-39.0089559599159,17.5135936463609));
#20512=CARTESIAN_POINT('Ctrl Pts',(129.098338076859,-38.9860349440316,17.5077949651195));
#20513=CARTESIAN_POINT('Ctrl Pts',(128.98216432776,-38.9579662978657,17.501996283878));
#20514=CARTESIAN_POINT('Ctrl Pts',(128.867423787524,-38.9248561913697,17.4961976026366));
#20515=CARTESIAN_POINT('Ctrl Pts',(128.752699916642,-38.8917508950661,17.4903997638199));
#20516=CARTESIAN_POINT('Ctrl Pts',(128.639409233592,-38.853605708297,17.4846019250032));
#20517=CARTESIAN_POINT('Ctrl Pts',(128.528019260807,-38.8105770827324,17.4788040861865));
#20518=CARTESIAN_POINT('Ctrl Pts',(128.416619052904,-38.7675445034627,17.4730057146327));
#20519=CARTESIAN_POINT('Ctrl Pts',(128.307120284198,-38.7196277406865,17.4672073430789));
#20520=CARTESIAN_POINT('Ctrl Pts',(128.199971240297,-38.6670316966507,17.4614089715251));
#20521=CARTESIAN_POINT('Ctrl Pts',(128.09278693909,-38.61441834593,17.4556086920219));
#20522=CARTESIAN_POINT('Ctrl Pts',(127.987954267406,-38.5571228321082,17.4498084125187));
#20523=CARTESIAN_POINT('Ctrl Pts',(127.885897033814,-38.4953960645915,17.4440081330155));
#20524=CARTESIAN_POINT('Ctrl Pts',(127.783725552764,-38.4336001973551,17.4382013604186));
#20525=CARTESIAN_POINT('Ctrl Pts',(127.684336061771,-38.3673633867531,17.4323945878217));
#20526=CARTESIAN_POINT('Ctrl Pts',(127.588123611192,-38.2969800249788,17.4265878152247));
#20527=CARTESIAN_POINT('Ctrl Pts',(127.491847393984,-38.2265500152951,17.420777194079));
#20528=CARTESIAN_POINT('Ctrl Pts',(127.398752728922,-38.1519682368748,17.4149665729333));
#20529=CARTESIAN_POINT('Ctrl Pts',(127.309200486926,-38.0735684440798,17.4091559517876));
#20530=CARTESIAN_POINT('Ctrl Pts',(127.219518559403,-37.9950551162322,17.4033369159617));
#20531=CARTESIAN_POINT('Ctrl Pts',(127.133389588573,-37.9127130201863,17.3975178801359));
#20532=CARTESIAN_POINT('Ctrl Pts',(127.051136702445,-37.8269117871514,17.3916988443101));
#20533=CARTESIAN_POINT('Ctrl Pts',(127.028596767237,-37.803399490812,17.3901042414133));
#20534=CARTESIAN_POINT('Ctrl Pts',(127.006347661452,-37.7796276189105,17.3885096385165));
#20535=CARTESIAN_POINT('Ctrl Pts',(126.98439548147,-37.7556041783652,17.3869150356197));
#20536=CARTESIAN_POINT('Ctrl Pts',(126.904949694774,-37.6686624197412,17.3811441061854));
#20537=CARTESIAN_POINT('Ctrl Pts',(126.829126420265,-37.5781282483199,17.3753731767511));
#20538=CARTESIAN_POINT('Ctrl Pts',(126.757271904743,-37.4843388456957,17.3696022473168));
#20539=CARTESIAN_POINT('Ctrl Pts',(126.68553138207,-37.3906982342941,17.3638404731136));
#20540=CARTESIAN_POINT('Ctrl Pts',(126.617747338226,-37.2938129978376,17.3580786989103));
#20541=CARTESIAN_POINT('Ctrl Pts',(126.554228208451,-37.1940560067062,17.352316924707));
#20542=CARTESIAN_POINT('Ctrl Pts',(126.490766915311,-37.0943898481901,17.346560396823));
#20543=CARTESIAN_POINT('Ctrl Pts',(126.431563040174,-36.9918574813407,17.3408038689389));
#20544=CARTESIAN_POINT('Ctrl Pts',(126.376883772214,-36.8868634820651,17.3350473410549));
#20545=CARTESIAN_POINT('Ctrl Pts',(126.322240771507,-36.7819391224183,17.3292946313173));
#20546=CARTESIAN_POINT('Ctrl Pts',(126.272116603255,-36.6745567447501,17.3235419215796));
#20547=CARTESIAN_POINT('Ctrl Pts',(126.226733859034,-36.5651477979528,17.317789211842));
#20548=CARTESIAN_POINT('Ctrl Pts',(126.181369996407,-36.4557843710003,17.3120388955326));
#20549=CARTESIAN_POINT('Ctrl Pts',(126.140743793312,-36.3443964363891,17.3062885792231));
#20550=CARTESIAN_POINT('Ctrl Pts',(126.105030474364,-36.2314371256241,17.3005382629137));
#20551=CARTESIAN_POINT('Ctrl Pts',(126.069314010461,-36.1184678675355,17.2947874402249));
#20552=CARTESIAN_POINT('Ctrl Pts',(126.038511430088,-36.0039273512483,17.2890366175361));
#20553=CARTESIAN_POINT('Ctrl Pts',(126.012748532405,-35.8882852774671,17.2832857948474));
#20554=CARTESIAN_POINT('Ctrl Pts',(125.986984650957,-35.7726387878505,17.2775347525613));
#20555=CARTESIAN_POINT('Ctrl Pts',(125.966260918392,-35.6558910655558,17.2717837102753));
#20556=CARTESIAN_POINT('Ctrl Pts',(125.950652058164,-35.5385222799012,17.2660326679892));
#20557=CARTESIAN_POINT('Ctrl Pts',(125.935032572806,-35.4210735999719,17.2602777109029));
#20558=CARTESIAN_POINT('Ctrl Pts',(125.924534958788,-35.3030034268805,17.2545227538166));
#20559=CARTESIAN_POINT('Ctrl Pts',(125.919182065361,-35.1847971437223,17.2487677967303));
#20560=CARTESIAN_POINT('Ctrl Pts',(125.916344291963,-35.1221314750591,17.2457168740187));
#20561=CARTESIAN_POINT('Ctrl Pts',(125.914951544561,-35.0594275863794,17.2426659513071));
#20562=CARTESIAN_POINT('Ctrl Pts',(125.915001286747,-34.9967576667114,17.2396150285955));
#20563=CARTESIAN_POINT('Origin',(130.,-35.,32.7603849714045));
#20564=CARTESIAN_POINT('',(132.487160670875,-31.7594357285724,19.2967873947729));
#20565=CARTESIAN_POINT('',(132.487160670875,-31.7594357285724,19.1927515499128));
#20566=CARTESIAN_POINT('',(132.487160670875,-31.7594357285724,32.7603849714045));
#20567=CARTESIAN_POINT('',(125.915000065373,-34.9992691782955,18.3853849714449));
#20568=CARTESIAN_POINT('Ctrl Pts',(132.487160670875,-31.7594357285724,19.1927515499128));
#20569=CARTESIAN_POINT('Ctrl Pts',(132.581827177387,-31.8320930783806,19.1869279757759));
#20570=CARTESIAN_POINT('Ctrl Pts',(132.673193329814,-31.908814616929,19.1811044016391));
#20571=CARTESIAN_POINT('Ctrl Pts',(132.760910607467,-31.9892529801437,19.1752808275022));
#20572=CARTESIAN_POINT('Ctrl Pts',(132.798099032587,-32.0233554526232,19.1728118777524));
#20573=CARTESIAN_POINT('Ctrl Pts',(132.834632084745,-32.0581255579088,19.1703429280026));
#20574=CARTESIAN_POINT('Ctrl Pts',(132.870485381043,-32.0935350204725,19.1678739782528));
#20575=CARTESIAN_POINT('Ctrl Pts',(132.955052701829,-32.1770554687629,19.1620504560929));
#20576=CARTESIAN_POINT('Ctrl Pts',(133.03610818553,-32.2644045741462,19.156226933933));
#20577=CARTESIAN_POINT('Ctrl Pts',(133.113286012663,-32.355255172354,19.1504034117731));
#20578=CARTESIAN_POINT('Ctrl Pts',(133.190366466249,-32.4459911463853,19.1445872370215));
#20579=CARTESIAN_POINT('Ctrl Pts',(133.263578731991,-32.5402195179648,19.1387710622698));
#20580=CARTESIAN_POINT('Ctrl Pts',(133.332592945845,-32.6375755552185,19.1329548875181));
#20581=CARTESIAN_POINT('Ctrl Pts',(133.401538075306,-32.7348341374344,19.1271445348556));
#20582=CARTESIAN_POINT('Ctrl Pts',(133.466293278075,-32.8352138256769,19.1213341821931));
#20583=CARTESIAN_POINT('Ctrl Pts',(133.526568593771,-32.9383164759288,19.1155238295306));
#20584=CARTESIAN_POINT('Ctrl Pts',(133.589126503954,-33.0453235692901,19.1094934418703));
#20585=CARTESIAN_POINT('Ctrl Pts',(133.646858227866,-33.155263593993,19.1034630542101));
#20586=CARTESIAN_POINT('Ctrl Pts',(133.699488433033,-33.2676575587207,19.0974326665498));
#20587=CARTESIAN_POINT('Ctrl Pts',(133.750141208964,-33.3758286421019,19.0916288534359));
#20588=CARTESIAN_POINT('Ctrl Pts',(133.79606871103,-33.4862721897746,19.0858250403219));
#20589=CARTESIAN_POINT('Ctrl Pts',(133.837072401333,-33.5985363412033,19.0800212272079));
#20590=CARTESIAN_POINT('Ctrl Pts',(133.878070036958,-33.7107839155086,19.0742182710952));
#20591=CARTESIAN_POINT('Ctrl Pts',(133.914145166652,-33.8248511754843,19.0684153149826));
#20592=CARTESIAN_POINT('Ctrl Pts',(133.945147960975,-33.9402676913422,19.0626123588699));
#20593=CARTESIAN_POINT('Ctrl Pts',(133.976153494533,-34.0556944047638,19.0568088900402));
#20594=CARTESIAN_POINT('Ctrl Pts',(134.002085695723,-34.1724702167038,19.0510054212106));
#20595=CARTESIAN_POINT('Ctrl Pts',(134.022845199161,-34.2901116259668,19.0452019523809));
#20596=CARTESIAN_POINT('Ctrl Pts',(134.043611436343,-34.4077911944864,19.0393966010843));
#20597=CARTESIAN_POINT('Ctrl Pts',(134.059201567955,-34.5263365167954,19.0335912497877));
#20598=CARTESIAN_POINT('Ctrl Pts',(134.069567812193,-34.6452566815796,19.0277858984912));
#20599=CARTESIAN_POINT('Ctrl Pts',(134.079945538032,-34.7643085617543,19.021974117216));
#20600=CARTESIAN_POINT('Ctrl Pts',(134.08508779176,-34.8837357060798,19.0161623359409));
#20601=CARTESIAN_POINT('Ctrl Pts',(134.08499886531,-35.0030447355878,19.0103505546657));
#20602=CARTESIAN_POINT('Ctrl Pts',(134.084909880444,-35.1224321392741,19.0045349556277));
#20603=CARTESIAN_POINT('Ctrl Pts',(134.079582889975,-35.241700866618,18.9987193565897));
#20604=CARTESIAN_POINT('Ctrl Pts',(134.069074136742,-35.3603618593873,18.9929037575517));
#20605=CARTESIAN_POINT('Ctrl Pts',(134.058550328391,-35.4791928490312,18.9870798269328));
#20606=CARTESIAN_POINT('Ctrl Pts',(134.042829993951,-35.59741396297,18.9812558963139));
#20607=CARTESIAN_POINT('Ctrl Pts',(134.022020620761,-35.7145453982577,18.975431965695));
#20608=CARTESIAN_POINT('Ctrl Pts',(134.016497305201,-35.7456349401286,18.9738861523581));
#20609=CARTESIAN_POINT('Ctrl Pts',(134.01061573948,-35.7766477941407,18.9723403390213));
#20610=CARTESIAN_POINT('Ctrl Pts',(134.004378520275,-35.8075751769097,18.9707945256845));
#20611=CARTESIAN_POINT('Ctrl Pts',(133.980880487633,-35.9240906665762,18.9649708451222));
#20612=CARTESIAN_POINT('Ctrl Pts',(133.952254965274,-36.0397675904643,18.9591471645599));
#20613=CARTESIAN_POINT('Ctrl Pts',(133.91857506942,-36.1541206285814,18.9533234839977));
#20614=CARTESIAN_POINT('Ctrl Pts',(133.88493766735,-36.2683293879503,18.9475071511487));
#20615=CARTESIAN_POINT('Ctrl Pts',(133.846258690005,-36.3812171955832,18.9416908182998));
#20616=CARTESIAN_POINT('Ctrl Pts',(133.802662383301,-36.4923082116737,18.9358744854508));
#20617=CARTESIAN_POINT('Ctrl Pts',(133.759109719698,-36.6032880175059,18.9300639751778));
#20618=CARTESIAN_POINT('Ctrl Pts',(133.71064966797,-36.7124742322112,18.9242534649048));
#20619=CARTESIAN_POINT('Ctrl Pts',(133.65745629243,-36.8194060758835,18.9184429546318));
#20620=CARTESIAN_POINT('Ctrl Pts',(133.602250551807,-36.9303832711881,18.9124126262353));
#20621=CARTESIAN_POINT('Ctrl Pts',(133.541946407721,-37.0389317263569,18.9063822978388));
#20622=CARTESIAN_POINT('Ctrl Pts',(133.476793534076,-37.1445586309089,18.9003519694423));
#20623=CARTESIAN_POINT('Ctrl Pts',(133.414086297717,-37.2462206282868,18.8945480009153));
#20624=CARTESIAN_POINT('Ctrl Pts',(133.346888017009,-37.3451760749478,18.8887440323882));
#20625=CARTESIAN_POINT('Ctrl Pts',(133.275467795461,-37.4410112086788,18.8829400638611));
#20626=CARTESIAN_POINT('Ctrl Pts',(133.204058132901,-37.5368321738467,18.8771369534107));
#20627=CARTESIAN_POINT('Ctrl Pts',(133.12842801474,-37.6295334161818,18.8713338429603));
#20628=CARTESIAN_POINT('Ctrl Pts',(133.04888877558,-37.7187317326541,18.8655307325099));
#20629=CARTESIAN_POINT('Ctrl Pts',(132.969342525942,-37.8079379109431,18.8597271105814));
#20630=CARTESIAN_POINT('Ctrl Pts',(132.885886742036,-37.8936402447414,18.8539234886528));
#20631=CARTESIAN_POINT('Ctrl Pts',(132.798871353915,-37.975490572029,18.8481198667243));
#20632=CARTESIAN_POINT('Ctrl Pts',(132.711827762464,-38.0573674285532,18.8423143637323));
#20633=CARTESIAN_POINT('Ctrl Pts',(132.621222569546,-38.1353895159424,18.8365088607403));
#20634=CARTESIAN_POINT('Ctrl Pts',(132.527440179702,-38.2092477526714,18.8307033577483));
#20635=CARTESIAN_POINT('Ctrl Pts',(132.433553965407,-38.283187756254,18.8248914276097));
#20636=CARTESIAN_POINT('Ctrl Pts',(132.336483854118,-38.3529544550157,18.8190794974711));
#20637=CARTESIAN_POINT('Ctrl Pts',(132.236644859884,-38.4182809672049,18.8132675673325));
#20638=CARTESIAN_POINT('Ctrl Pts',(132.136740308358,-38.4836503747498,18.8074518209055));
#20639=CARTESIAN_POINT('Ctrl Pts',(132.034063603382,-38.5445735814209,18.8016360744785));
#20640=CARTESIAN_POINT('Ctrl Pts',(131.929054624238,-38.6008295234163,18.7958203280516));
#20641=CARTESIAN_POINT('Ctrl Pts',(131.82389526941,-38.6571660254343,18.7899962533192));
#20642=CARTESIAN_POINT('Ctrl Pts',(131.716397340927,-38.7088217463478,18.7841721785869));
#20643=CARTESIAN_POINT('Ctrl Pts',(131.607021068971,-38.7556235546025,18.7783481038545));
#20644=CARTESIAN_POINT('Ctrl Pts',(131.578018257175,-38.7680337786138,18.776803760275));
#20645=CARTESIAN_POINT('Ctrl Pts',(131.548883456525,-38.7801029826979,18.7752594166955));
#20646=CARTESIAN_POINT('Ctrl Pts',(131.519625411257,-38.791828531126,18.773715073116));
#20647=CARTESIAN_POINT('Ctrl Pts',(131.409293643512,-38.8360454456193,18.7678913704191));
#20648=CARTESIAN_POINT('Ctrl Pts',(131.296852532956,-38.8755141152904,18.7620676677222));
#20649=CARTESIAN_POINT('Ctrl Pts',(131.182748077146,-38.9100296656174,18.7562439650253));
#20650=CARTESIAN_POINT('Ctrl Pts',(131.068787554557,-38.9445016774661,18.750427608442));
#20651=CARTESIAN_POINT('Ctrl Pts',(130.953168247317,-38.9740328798198,18.7446112518587));
#20652=CARTESIAN_POINT('Ctrl Pts',(130.836356250139,-38.9984663588497,18.7387948952753));
#20653=CARTESIAN_POINT('Ctrl Pts',(130.719661158745,-39.0228753847833,18.7329843597185));
#20654=CARTESIAN_POINT('Ctrl Pts',(130.601776149403,-39.0421967537167,18.7271738241616));
#20655=CARTESIAN_POINT('Ctrl Pts',(130.483182028482,-39.0563234742008,18.7213632886047));
#20656=CARTESIAN_POINT('Ctrl Pts',(130.360102075995,-39.0709845389522,18.7153329691024));
#20657=CARTESIAN_POINT('Ctrl Pts',(130.236258737322,-39.0800500903439,18.7093026496));
#20658=CARTESIAN_POINT('Ctrl Pts',(130.112201044107,-39.083458818906,18.7032723300976));
#20659=CARTESIAN_POINT('Ctrl Pts',(129.992799321315,-39.0867396155442,18.6974683326275));
#20660=CARTESIAN_POINT('Ctrl Pts',(129.873199488605,-39.0847805341232,18.6916643351573));
#20661=CARTESIAN_POINT('Ctrl Pts',(129.753895122748,-39.0775798446374,18.6858603376872));
#20662=CARTESIAN_POINT('Ctrl Pts',(129.634608368584,-39.0703802181162,18.6800571970023));
#20663=CARTESIAN_POINT('Ctrl Pts',(129.515617401998,-39.0579405468999,18.6742540563174));
#20664=CARTESIAN_POINT('Ctrl Pts',(129.397413389351,-39.0403111732473,18.6684509156325));
#20665=CARTESIAN_POINT('Ctrl Pts',(129.279198932917,-39.0226802419705,18.6626472622174));
#20666=CARTESIAN_POINT('Ctrl Pts',(129.161771972536,-38.9998587568216,18.6568436088023));
#20667=CARTESIAN_POINT('Ctrl Pts',(129.045615522846,-38.9719485482276,18.6510399553872));
#20668=CARTESIAN_POINT('Ctrl Pts',(128.929421400574,-38.9440292876214,18.6452344196951));
#20669=CARTESIAN_POINT('Ctrl Pts',(128.814499005302,-38.9110181166276,18.6394288840031));
#20670=CARTESIAN_POINT('Ctrl Pts',(128.701317562576,-38.8730671213814,18.6336233483111));
#20671=CARTESIAN_POINT('Ctrl Pts',(128.588010788321,-38.8350741010814,18.6278113838561));
#20672=CARTESIAN_POINT('Ctrl Pts',(128.47644920212,-38.7921304675922,18.6219994194012));
#20673=CARTESIAN_POINT('Ctrl Pts',(128.367083513114,-38.7444370400442,18.6161874549463));
#20674=CARTESIAN_POINT('Ctrl Pts',(128.257645993281,-38.6967122876964,18.6103716732228));
#20675=CARTESIAN_POINT('Ctrl Pts',(128.150407608846,-38.6442317075111,18.6045558914993));
#20676=CARTESIAN_POINT('Ctrl Pts',(128.045794377579,-38.5872420304878,18.5987401097757));
#20677=CARTESIAN_POINT('Ctrl Pts',(127.941031317505,-38.5301707319026,18.592915998593));
#20678=CARTESIAN_POINT('Ctrl Pts',(127.838901263346,-38.4685776567739,18.5870918874104));
#20679=CARTESIAN_POINT('Ctrl Pts',(127.739801298729,-38.4027528312785,18.5812677762277));
#20680=CARTESIAN_POINT('Ctrl Pts',(127.713528536551,-38.3853017656568,18.5797237243343));
#20681=CARTESIAN_POINT('Ctrl Pts',(127.687468563015,-38.3675534882863,18.5781796724409));
#20682=CARTESIAN_POINT('Ctrl Pts',(127.661628371752,-38.3495138644596,18.5766356205475));
#20683=CARTESIAN_POINT('Ctrl Pts',(127.564645404129,-38.2818078542471,18.5708405111669));
#20684=CARTESIAN_POINT('Ctrl Pts',(127.470441320797,-38.2097715994423,18.5650454017863));
#20685=CARTESIAN_POINT('Ctrl Pts',(127.379429648083,-38.1336617607289,18.5592502924056));
#20686=CARTESIAN_POINT('Ctrl Pts',(127.288533132876,-38.0576482241601,18.5534625156047));
#20687=CARTESIAN_POINT('Ctrl Pts',(127.20082130956,-37.977571615792,18.5476747388038));
#20688=CARTESIAN_POINT('Ctrl Pts',(127.11667881418,-37.8937318361248,18.5418869620029));
#20689=CARTESIAN_POINT('Ctrl Pts',(127.032620266486,-37.8099757021282,18.5361049595787));
#20690=CARTESIAN_POINT('Ctrl Pts',(126.952124254574,-37.722464154091,18.5303229571545));
#20691=CARTESIAN_POINT('Ctrl Pts',(126.875541868502,-37.6315368864056,18.5245409547303));
#20692=CARTESIAN_POINT('Ctrl Pts',(126.798745396922,-37.5403554321999,18.5187427887601));
#20693=CARTESIAN_POINT('Ctrl Pts',(126.725884781323,-37.4457394066967,18.5129446227899));
#20694=CARTESIAN_POINT('Ctrl Pts',(126.65727658786,-37.3480683954962,18.5071464568196));
#20695=CARTESIAN_POINT('Ctrl Pts',(126.58893403817,-37.2507755562707,18.5013707407437));
#20696=CARTESIAN_POINT('Ctrl Pts',(126.524811277393,-37.1504516870973,18.4955950246677));
#20697=CARTESIAN_POINT('Ctrl Pts',(126.465180005024,-37.0475039934317,18.4898193085918));
#20698=CARTESIAN_POINT('Ctrl Pts',(126.405556722735,-36.9445700938754,18.4840443664124));
#20699=CARTESIAN_POINT('Ctrl Pts',(126.350423939006,-36.8390134261195,18.4782694242329));
#20700=CARTESIAN_POINT('Ctrl Pts',(126.300008586202,-36.7312678989178,18.4724944820535));
#20701=CARTESIAN_POINT('Ctrl Pts',(126.249587776293,-36.6235107090232,18.4667189147773));
#20702=CARTESIAN_POINT('Ctrl Pts',(126.203885587117,-36.5135645627699,18.4609433475011));
#20703=CARTESIAN_POINT('Ctrl Pts',(126.163081481472,-36.4018849033276,18.4551677802249));
#20704=CARTESIAN_POINT('Ctrl Pts',(126.121997131868,-36.2894382242567,18.4493525461599));
#20705=CARTESIAN_POINT('Ctrl Pts',(126.08587855545,-36.1752345254005,18.4435373120949));
#20706=CARTESIAN_POINT('Ctrl Pts',(126.054858042081,-36.0597546564499,18.4377220780299));
#20707=CARTESIAN_POINT('Ctrl Pts',(126.024004228695,-35.9448953604704,18.4319380942349));
#20708=CARTESIAN_POINT('Ctrl Pts',(125.998193853041,-35.8287739946131,18.4261541104399));
#20709=CARTESIAN_POINT('Ctrl Pts',(125.977505578191,-35.7118733219564,18.4203701266449));
#20710=CARTESIAN_POINT('Ctrl Pts',(125.956649638406,-35.5940252458205,18.4145392674449));
#20711=CARTESIAN_POINT('Ctrl Pts',(125.940999242795,-35.4753855999452,18.4087084082449));
#20712=CARTESIAN_POINT('Ctrl Pts',(125.930581536691,-35.3564524799731,18.4028775490449));
#20713=CARTESIAN_POINT('Ctrl Pts',(125.920163830587,-35.2375193600011,18.3970466898449));
#20714=CARTESIAN_POINT('Ctrl Pts',(125.914978771534,-35.1182931914366,18.3912158306449));
#20715=CARTESIAN_POINT('Ctrl Pts',(125.915000065373,-34.9992691782955,18.3853849714449));
#20716=CARTESIAN_POINT('Ctrl Pts',(125.915000065374,-34.9992691774698,18.3853849714045));
#20717=CARTESIAN_POINT('Ctrl Pts',(125.915007160825,-34.9596084944438,18.3834420369294));
#20718=CARTESIAN_POINT('Ctrl Pts',(125.915591831957,-34.9199536068433,18.3814991024543));
#20719=CARTESIAN_POINT('Ctrl Pts',(125.916753658639,-34.8803157664518,18.3795561679791));
#20720=CARTESIAN_POINT('Ctrl Pts',(125.920236584366,-34.7614893904925,18.3737316361649));
#20721=CARTESIAN_POINT('Ctrl Pts',(125.928916364881,-34.6426238185521,18.3679071043506));
#20722=CARTESIAN_POINT('Ctrl Pts',(125.942802846095,-34.5242098631234,18.3620825725364));
#20723=CARTESIAN_POINT('Ctrl Pts',(125.956671803865,-34.4059453350683,18.3562653907384));
#20724=CARTESIAN_POINT('Ctrl Pts',(125.975734346806,-34.2881316918524,18.3504482089403));
#20725=CARTESIAN_POINT('Ctrl Pts',(125.999948324585,-34.1712590308118,18.3446310271423));
#20726=CARTESIAN_POINT('Ctrl Pts',(126.024138052315,-34.0545034165374,18.3388196711919));
#20727=CARTESIAN_POINT('Ctrl Pts',(126.053468869069,-33.9386873070813,18.3330083152416));
#20728=CARTESIAN_POINT('Ctrl Pts',(126.087846978892,-33.8242943653134,18.3271969592912));
#20729=CARTESIAN_POINT('Ctrl Pts',(126.123518576595,-33.7055973508514,18.3211669491295));
#20730=CARTESIAN_POINT('Ctrl Pts',(126.164624688392,-33.588433146939,18.3151369389678));
#20731=CARTESIAN_POINT('Ctrl Pts',(126.211002501278,-33.4733294544416,18.3091069288061));
#20732=CARTESIAN_POINT('Ctrl Pts',(126.255648191268,-33.3625246654219,18.3033021280282));
#20733=CARTESIAN_POINT('Ctrl Pts',(126.305178700704,-33.2536296476363,18.2974973272503));
#20734=CARTESIAN_POINT('Ctrl Pts',(126.359398630354,-33.1470977717822,18.2916925264723));
#20735=CARTESIAN_POINT('Ctrl Pts',(126.413610485596,-33.0405817606087,18.2858885901428));
#20736=CARTESIAN_POINT('Ctrl Pts',(126.472510187143,-32.9364285551924,18.2800846538133));
#20737=CARTESIAN_POINT('Ctrl Pts',(126.535855549591,-32.8350685399535,18.2742807174837));
#20738=CARTESIAN_POINT('Ctrl Pts',(126.599206415331,-32.7336997187998,18.2684762769222));
#20739=CARTESIAN_POINT('Ctrl Pts',(126.66700349354,-32.6351249164702,18.2626718363606));
#20740=CARTESIAN_POINT('Ctrl Pts',(126.738960637975,-32.5397465010037,18.256867395799));
#20741=CARTESIAN_POINT('Ctrl Pts',(126.810941001048,-32.4443373094839,18.2510610823003));
#20742=CARTESIAN_POINT('Ctrl Pts',(126.887083854255,-32.3521268817277,18.2452547688016));
#20743=CARTESIAN_POINT('Ctrl Pts',(126.967062468593,-32.2634848930473,18.2394484553029));
#20744=CARTESIAN_POINT('Ctrl Pts',(127.047129392011,-32.1747450295463,18.2336357307128));
#20745=CARTESIAN_POINT('Ctrl Pts',(127.131040256969,-32.0895817732114,18.2278230061228));
#20746=CARTESIAN_POINT('Ctrl Pts',(127.218431033966,-32.0083283791175,18.2220102815327));
#20747=CARTESIAN_POINT('Ctrl Pts',(127.305879059942,-31.9270217565923,18.2161937490744));
#20748=CARTESIAN_POINT('Ctrl Pts',(127.396811227873,-31.8496303612636,18.2103772166162));
#20749=CARTESIAN_POINT('Ctrl Pts',(127.490831255007,-31.7764464935186,18.204560684158));
#20750=CARTESIAN_POINT('Ctrl Pts',(127.584985607785,-31.7031580685799,18.1987358416673));
#20751=CARTESIAN_POINT('Ctrl Pts',(127.682236293481,-31.6340894049455,18.1929109991767));
#20752=CARTESIAN_POINT('Ctrl Pts',(127.782158868308,-31.5694890009543,18.1870861566861));
#20753=CARTESIAN_POINT('Ctrl Pts',(127.808516504672,-31.5524486678726,18.185549676261));
#20754=CARTESIAN_POINT('Ctrl Pts',(127.835059925452,-31.5357189856054,18.1840131958358));
#20755=CARTESIAN_POINT('Ctrl Pts',(127.861781083475,-31.5193039683111,18.1824767154107));
#20756=CARTESIAN_POINT('Ctrl Pts',(127.963069165046,-31.4570819040853,18.1766525982635));
#20757=CARTESIAN_POINT('Ctrl Pts',(128.067238441947,-31.399184622791,18.1708284811163));
#20758=CARTESIAN_POINT('Ctrl Pts',(128.173883810515,-31.3458893472556,18.1650043639691));
#20759=CARTESIAN_POINT('Ctrl Pts',(128.280394840776,-31.2926612063475,18.1591875833059));
#20760=CARTESIAN_POINT('Ctrl Pts',(128.389375396946,-31.2440237218838,18.1533708026427));
#20761=CARTESIAN_POINT('Ctrl Pts',(128.500392476305,-31.2002102328055,18.1475540219795));
#20762=CARTESIAN_POINT('Ctrl Pts',(128.611298629235,-31.1564405214402,18.1417430533472));
#20763=CARTESIAN_POINT('Ctrl Pts',(128.724236879665,-31.1174853655095,18.1359320847149));
#20764=CARTESIAN_POINT('Ctrl Pts',(128.838751302399,-31.0835313786116,18.1301211160827));
#20765=CARTESIAN_POINT('Ctrl Pts',(128.95758525217,-31.0482966345749,18.124090955531));
#20766=CARTESIAN_POINT('Ctrl Pts',(129.078116222543,-31.0184479812632,18.1180607949793));
#20767=CARTESIAN_POINT('Ctrl Pts',(129.199813490375,-30.9941384759563,18.1120306344276));
#20768=CARTESIAN_POINT('Ctrl Pts',(129.316955595742,-30.9707388821707,18.1062261844567));
#20769=CARTESIAN_POINT('Ctrl Pts',(129.435177821768,-30.9524713116863,18.1004217344858));
#20770=CARTESIAN_POINT('Ctrl Pts',(129.553993896093,-30.9394207857404,18.0946172845148));
#20771=CARTESIAN_POINT('Ctrl Pts',(129.672792561881,-30.9263721719142,18.0888136849927));
#20772=CARTESIAN_POINT('Ctrl Pts',(129.79218449724,-30.9185391270626,18.0830100854705));
#20773=CARTESIAN_POINT('Ctrl Pts',(129.911677017859,-30.9159549401573,18.0772064859483));
#20774=CARTESIAN_POINT('Ctrl Pts',(130.031180214741,-30.9133705223633,18.0714023678936));
#20775=CARTESIAN_POINT('Ctrl Pts',(130.150783606583,-30.9160359037771,18.0655982498389));
#20776=CARTESIAN_POINT('Ctrl Pts',(130.269993853628,-30.9239322479866,18.0597941317842));
#20777=CARTESIAN_POINT('Ctrl Pts',(130.389242868866,-30.931831160155,18.0539881261806));
#20778=CARTESIAN_POINT('Ctrl Pts',(130.508098077894,-30.9449643913867,18.048182120577));
#20779=CARTESIAN_POINT('Ctrl Pts',(130.626071248985,-30.9632612431328,18.0423761149734));
#20780=CARTESIAN_POINT('Ctrl Pts',(130.744175155961,-30.9815783711422,18.036563675252));
#20781=CARTESIAN_POINT('Ctrl Pts',(130.861394670249,-31.0050704791497,18.0307512355306));
#20782=CARTESIAN_POINT('Ctrl Pts',(130.977251583454,-31.0336157091582,18.0249387958092));
#20783=CARTESIAN_POINT('Ctrl Pts',(131.093184657763,-31.0621797040047,18.0191225351521));
#20784=CARTESIAN_POINT('Ctrl Pts',(131.20775295628,-31.0958033215968,18.0133062744949));
#20785=CARTESIAN_POINT('Ctrl Pts',(131.320494855899,-31.1343152824441,18.0074900138378));
#20786=CARTESIAN_POINT('Ctrl Pts',(131.433398245051,-31.1728824071535,18.0016654220702));
#20787=CARTESIAN_POINT('Ctrl Pts',(131.544469634885,-31.2163517024487,17.9958408303027));
#20788=CARTESIAN_POINT('Ctrl Pts',(131.653268610582,-31.2645043299095,17.9900162385351));
#20789=CARTESIAN_POINT('Ctrl Pts',(131.682028269868,-31.2772328795179,17.9884765799708));
#20790=CARTESIAN_POINT('Ctrl Pts',(131.710629287558,-31.2902884296224,17.9869369214065));
#20791=CARTESIAN_POINT('Ctrl Pts',(131.739063847766,-31.3036664201683,17.9853972628422));
#20792=CARTESIAN_POINT('Ctrl Pts',(131.846528250602,-31.3542266452825,17.9795783408343));
#20793=CARTESIAN_POINT('Ctrl Pts',(131.951961127314,-31.4095597189194,17.9737594188264));
#20794=CARTESIAN_POINT('Ctrl Pts',(132.054908974376,-31.4694796265946,17.9679404968185));
#20795=CARTESIAN_POINT('Ctrl Pts',(132.157711772312,-31.5293151096759,17.9621297734234));
#20796=CARTESIAN_POINT('Ctrl Pts',(132.258036157374,-31.5937243625645,17.9563190500284));
#20797=CARTESIAN_POINT('Ctrl Pts',(132.355450161183,-31.6624740393248,17.9505083266334));
#20798=CARTESIAN_POINT('Ctrl Pts',(132.399974541707,-31.6938970036755,17.9478524573595));
#20799=CARTESIAN_POINT('Ctrl Pts',(132.443891228791,-31.7262260633449,17.9451965880857));
#20800=CARTESIAN_POINT('Ctrl Pts',(132.487160670875,-31.7594357285724,17.9425407188119));
#20801=CARTESIAN_POINT('',(125.915000466472,-35.0019521977367,18.4896150286331));
#20802=CARTESIAN_POINT('Ctrl Pts',(125.915000466472,-35.0019521969606,18.4896150285955));
#20803=CARTESIAN_POINT('Ctrl Pts',(125.914942432893,-34.8805161196803,18.4837275172242));
#20804=CARTESIAN_POINT('Ctrl Pts',(125.920303700108,-34.7590882866263,18.4778400058528));
#20805=CARTESIAN_POINT('Ctrl Pts',(125.931055605275,-34.6381761303638,18.4719524944815));
#20806=CARTESIAN_POINT('Ctrl Pts',(125.941810869229,-34.5172262023751,18.4660631439115));
#20807=CARTESIAN_POINT('Ctrl Pts',(125.957960089699,-34.3967926619571,18.4601737933416));
#20808=CARTESIAN_POINT('Ctrl Pts',(125.979422788629,-34.2773770779969,18.4542844427717));
#20809=CARTESIAN_POINT('Ctrl Pts',(126.000896647879,-34.1578993995112,18.4483920298173));
#20810=CARTESIAN_POINT('Ctrl Pts',(126.027689417893,-34.0394411165113,18.4424996168629));
#20811=CARTESIAN_POINT('Ctrl Pts',(126.0596697468,-33.9224924614117,18.4366072039085));
#20812=CARTESIAN_POINT('Ctrl Pts',(126.091695452381,-33.8053778686486,18.4307064302488));
#20813=CARTESIAN_POINT('Ctrl Pts',(126.128923314983,-33.689777560173,18.4248056565891));
#20814=CARTESIAN_POINT('Ctrl Pts',(126.171172249785,-33.5761660703631,18.4189048829295));
#20815=CARTESIAN_POINT('Ctrl Pts',(126.213453797143,-33.4624668822243,18.4129995543785));
#20816=CARTESIAN_POINT('Ctrl Pts',(126.260763988836,-33.3507599323557,18.4070942258275));
#20817=CARTESIAN_POINT('Ctrl Pts',(126.312874489663,-33.241497662491,18.4011888972765));
#20818=CARTESIAN_POINT('Ctrl Pts',(126.365076832098,-33.1320428244831,18.395273160941));
#20819=CARTESIAN_POINT('Ctrl Pts',(126.422096202377,-33.0250416198214,18.3893574246055));
#20820=CARTESIAN_POINT('Ctrl Pts',(126.483659068718,-32.9209205270143,18.3834416882701));
#20821=CARTESIAN_POINT('Ctrl Pts',(126.52226554126,-32.8556255147855,18.3797318916674));
#20822=CARTESIAN_POINT('Ctrl Pts',(126.562657934769,-32.7914625588259,18.3760220950646));
#20823=CARTESIAN_POINT('Ctrl Pts',(126.604760614246,-32.7285303186201,18.3723122984619));
#20824=CARTESIAN_POINT('Ctrl Pts',(126.670854132907,-32.6297381931789,18.3664885952195));
#20825=CARTESIAN_POINT('Ctrl Pts',(126.741369641896,-32.5336739181619,18.3606648919772));
#20826=CARTESIAN_POINT('Ctrl Pts',(126.816054726341,-32.4407584142282,18.3548411887348));
#20827=CARTESIAN_POINT('Ctrl Pts',(126.890645601849,-32.3479601153677,18.3490248316029));
#20828=CARTESIAN_POINT('Ctrl Pts',(126.969395338088,-32.2583030029975,18.3432084744711));
#20829=CARTESIAN_POINT('Ctrl Pts',(127.052007852507,-32.1721797620218,18.3373921173392));
#20830=CARTESIAN_POINT('Ctrl Pts',(127.134537688124,-32.0861427133913,18.3315815812315));
#20831=CARTESIAN_POINT('Ctrl Pts',(127.220922330196,-32.0036327932832,18.3257710451238));
#20832=CARTESIAN_POINT('Ctrl Pts',(127.310825365669,-31.9250097908984,18.3199605090161));
#20833=CARTESIAN_POINT('Ctrl Pts',(127.40412897821,-31.8434128780386,18.3139301897193));
#20834=CARTESIAN_POINT('Ctrl Pts',(127.501222124778,-31.7660030829177,18.3078998704225));
#20835=CARTESIAN_POINT('Ctrl Pts',(127.601686289747,-31.6931410149187,18.3018695511257));
#20836=CARTESIAN_POINT('Ctrl Pts',(127.698379978124,-31.6230135012949,18.2960655531024));
#20837=CARTESIAN_POINT('Ctrl Pts',(127.79819585213,-31.5570987701424,18.2902615550791));
#20838=CARTESIAN_POINT('Ctrl Pts',(127.900727523391,-31.4956769456922,18.2844575570558));
#20839=CARTESIAN_POINT('Ctrl Pts',(128.003244058942,-31.4342641883224,18.2786544158178));
#20840=CARTESIAN_POINT('Ctrl Pts',(128.10847524429,-31.3773432284515,18.2728512745798));
#20841=CARTESIAN_POINT('Ctrl Pts',(128.215987278031,-31.3251498523268,18.2670481333418));
#20842=CARTESIAN_POINT('Ctrl Pts',(128.323508810868,-31.2729518647198,18.2612444793744));
#20843=CARTESIAN_POINT('Ctrl Pts',(128.433311225432,-31.2254824696792,18.2554408254069));
#20844=CARTESIAN_POINT('Ctrl Pts',(128.544938375596,-31.1829303557327,18.2496371714394));
#20845=CARTESIAN_POINT('Ctrl Pts',(128.656601729342,-31.1403644410311,18.2438316351963));
#20846=CARTESIAN_POINT('Ctrl Pts',(128.770090614322,-31.1027191244947,18.2380260989532));
#20847=CARTESIAN_POINT('Ctrl Pts',(128.884931888289,-31.0701338310006,18.2322205627101));
#20848=CARTESIAN_POINT('Ctrl Pts',(128.999900331694,-31.0375124541951,18.2264085977088));
#20849=CARTESIAN_POINT('Ctrl Pts',(129.116223760316,-31.0099623964539,18.2205966327076));
#20850=CARTESIAN_POINT('Ctrl Pts',(129.233416797189,-30.987572406489,18.2147846677063));
#20851=CARTESIAN_POINT('Ctrl Pts',(129.350686805802,-30.9651677109024,18.2089688854385));
#20852=CARTESIAN_POINT('Ctrl Pts',(129.468827157024,-30.947929891404,18.2031531031708));
#20853=CARTESIAN_POINT('Ctrl Pts',(129.587346928516,-30.9358958622355,18.197337320903));
#20854=CARTESIAN_POINT('Ctrl Pts',(129.706036445829,-30.9238445977472,18.1915132091833));
#20855=CARTESIAN_POINT('Ctrl Pts',(129.82510606183,-30.9170120225813,18.1856890974636));
#20856=CARTESIAN_POINT('Ctrl Pts',(129.944064288009,-30.9153829804835,18.1798649857439));
#20857=CARTESIAN_POINT('Ctrl Pts',(129.975601637482,-30.9149511005572,18.1783209391271));
#20858=CARTESIAN_POINT('Ctrl Pts',(130.007131185099,-30.914884667119,18.1767768925103));
#20859=CARTESIAN_POINT('Ctrl Pts',(130.038643847061,-30.9151827882897,18.1752328458935));
#20860=CARTESIAN_POINT('Ctrl Pts',(130.157465221301,-30.9163068814317,18.1694108768983));
#20861=CARTESIAN_POINT('Ctrl Pts',(130.276429325207,-30.9226216024877,18.1635889079031));
#20862=CARTESIAN_POINT('Ctrl Pts',(130.395046111187,-30.9341466369241,18.1577669389079));
#20863=CARTESIAN_POINT('Ctrl Pts',(130.513522711005,-30.9456580506041,18.1519518505534));
#20864=CARTESIAN_POINT('Ctrl Pts',(130.631652406412,-30.9623674952217,18.1461367621989));
#20865=CARTESIAN_POINT('Ctrl Pts',(130.748944700955,-30.9842426822688,18.1403216738444));
#20866=CARTESIAN_POINT('Ctrl Pts',(130.866126084286,-31.0060971842101,18.1345120842186));
#20867=CARTESIAN_POINT('Ctrl Pts',(130.982471242487,-31.0331076396458,18.1287024945928));
#20868=CARTESIAN_POINT('Ctrl Pts',(131.097494992829,-31.0651899994134,18.122892904967));
#20869=CARTESIAN_POINT('Ctrl Pts',(131.212437145711,-31.0972496000637,18.1170874366443));
#20870=CARTESIAN_POINT('Ctrl Pts',(131.326059363574,-31.1343738378891,18.1112819683217));
#20871=CARTESIAN_POINT('Ctrl Pts',(131.437887480208,-31.1764277704924,18.1054764999991));
#20872=CARTESIAN_POINT('Ctrl Pts',(131.549670783362,-31.2184648505982,18.0996733581329));
#20873=CARTESIAN_POINT('Ctrl Pts',(131.659661033301,-31.2654275536267,18.0938702162667));
#20874=CARTESIAN_POINT('Ctrl Pts',(131.767400549396,-31.3171315122592,18.0880670744004));
#20875=CARTESIAN_POINT('Ctrl Pts',(131.875115307195,-31.3688235894393,18.0822652660831));
#20876=CARTESIAN_POINT('Ctrl Pts',(131.980579993813,-31.4252545745619,18.0764634577657));
#20877=CARTESIAN_POINT('Ctrl Pts',(132.083358870215,-31.4861928314297,18.0706616494483));
#20878=CARTESIAN_POINT('Ctrl Pts',(132.186158067372,-31.5471431366042,18.064858694036));
#20879=CARTESIAN_POINT('Ctrl Pts',(132.286270042872,-31.6126022843173,18.0590557386236));
#20880=CARTESIAN_POINT('Ctrl Pts',(132.383285852153,-31.6822939330125,18.0532527832113));
#20881=CARTESIAN_POINT('Ctrl Pts',(132.418320364943,-31.7074610988143,18.0511572101586));
#20882=CARTESIAN_POINT('Ctrl Pts',(132.452951391226,-31.7331798151592,18.049061637106));
#20883=CARTESIAN_POINT('Ctrl Pts',(132.487160670875,-31.7594357285724,18.0469660640533));
#20884=CARTESIAN_POINT('Ctrl Pts',(132.487160670875,-31.7594357285724,19.2967873947729));
#20885=CARTESIAN_POINT('Ctrl Pts',(132.581876164488,-31.8321306763978,19.2909824707339));
#20886=CARTESIAN_POINT('Ctrl Pts',(132.673459485987,-31.9090257878229,19.2851775466948));
#20887=CARTESIAN_POINT('Ctrl Pts',(132.761523547418,-31.9898151722764,19.2793726226558));
#20888=CARTESIAN_POINT('Ctrl Pts',(132.849563241322,-32.0705822021225,19.2735693048525));
#20889=CARTESIAN_POINT('Ctrl Pts',(132.93408531082,-32.15524108653,19.2677659870493));
#20890=CARTESIAN_POINT('Ctrl Pts',(133.01473686711,-32.2434466045282,19.261962669246));
#20891=CARTESIAN_POINT('Ctrl Pts',(133.095385140938,-32.3316485326231,19.2561595876337));
#20892=CARTESIAN_POINT('Ctrl Pts',(133.172162939408,-32.4233965057908,19.2503565060214));
#20893=CARTESIAN_POINT('Ctrl Pts',(133.244755719231,-32.5183099866179,19.2445534244092));
#20894=CARTESIAN_POINT('Ctrl Pts',(133.317362676565,-32.6132420042339,19.2387492094437));
#20895=CARTESIAN_POINT('Ctrl Pts',(133.385782741859,-32.7113404345906,19.2329449944782));
#20896=CARTESIAN_POINT('Ctrl Pts',(133.449743380949,-32.8121938829971,19.2271407795127));
#20897=CARTESIAN_POINT('Ctrl Pts',(133.513770830608,-32.9131526786342,19.2213305017107));
#20898=CARTESIAN_POINT('Ctrl Pts',(133.57332933159,-33.0168718945394,19.2155202239086));
#20899=CARTESIAN_POINT('Ctrl Pts',(133.628191087686,-33.1229133128067,19.2097099461066));
#20900=CARTESIAN_POINT('Ctrl Pts',(133.683082530687,-33.2290121124242,19.2038965242351));
#20901=CARTESIAN_POINT('Ctrl Pts',(133.73327199399,-33.3374352474132,19.1980831023636));
#20902=CARTESIAN_POINT('Ctrl Pts',(133.778579567858,-33.4477237844481,19.1922696804921));
#20903=CARTESIAN_POINT('Ctrl Pts',(133.823958924307,-33.5581870559732,19.1864470481864));
#20904=CARTESIAN_POINT('Ctrl Pts',(133.864440800237,-33.6705212498169,19.1806244158808));
#20905=CARTESIAN_POINT('Ctrl Pts',(133.899894794839,-33.784251017195,19.1748017835751));
#20906=CARTESIAN_POINT('Ctrl Pts',(133.928658559913,-33.8765197826057,19.170077891962));
#20907=CARTESIAN_POINT('Ctrl Pts',(133.954113889628,-33.9697067625727,19.1653540003488));
#20908=CARTESIAN_POINT('Ctrl Pts',(133.976216025045,-34.0635539939876,19.1606301087357));
#20909=CARTESIAN_POINT('Ctrl Pts',(134.00346347904,-34.1792486122797,19.1548065076683));
#20910=CARTESIAN_POINT('Ctrl Pts',(134.025701189129,-34.2963199975551,19.148982906601));
#20911=CARTESIAN_POINT('Ctrl Pts',(134.042793156588,-34.4142965826944,19.1431593055336));
#20912=CARTESIAN_POINT('Ctrl Pts',(134.059863559868,-34.5321243219905,19.1373430518463));
#20913=CARTESIAN_POINT('Ctrl Pts',(134.071801075234,-34.6508545890837,19.1315267981591));
#20914=CARTESIAN_POINT('Ctrl Pts',(134.078520127177,-34.7700031038992,19.1257105444718));
#20915=CARTESIAN_POINT('Ctrl Pts',(134.085232453251,-34.8890323493252,19.1199001129387));
#20916=CARTESIAN_POINT('Ctrl Pts',(134.086736685062,-35.0084786042326,19.1140896814056));
#20917=CARTESIAN_POINT('Ctrl Pts',(134.082998806176,-35.1278504938013,19.1082792498726));
#20918=CARTESIAN_POINT('Ctrl Pts',(134.079119447478,-35.2517406444073,19.1022488918015));
#20919=CARTESIAN_POINT('Ctrl Pts',(134.069593242568,-35.375550245363,19.0962185337304));
#20920=CARTESIAN_POINT('Ctrl Pts',(134.054441532247,-35.4987272416763,19.0901881756594));
#20921=CARTESIAN_POINT('Ctrl Pts',(134.039858835987,-35.6172783943498,19.0843842843343));
#20922=CARTESIAN_POINT('Ctrl Pts',(134.020065594749,-35.7352431580727,19.0785803930091));
#20923=CARTESIAN_POINT('Ctrl Pts',(133.995133781718,-35.8521332443793,19.072776501684));
#20924=CARTESIAN_POINT('Ctrl Pts',(133.970205651734,-35.9690060631193,19.0669734677377));
#20925=CARTESIAN_POINT('Ctrl Pts',(133.940140544713,-36.0848041209145,19.0611704337913));
#20926=CARTESIAN_POINT('Ctrl Pts',(133.905061562704,-36.1990492865157,19.055367399845));
#20927=CARTESIAN_POINT('Ctrl Pts',(133.869979484137,-36.3133045369806,19.0495638536424));
#20928=CARTESIAN_POINT('Ctrl Pts',(133.829882770461,-36.4260062323352,19.0437603074397));
#20929=CARTESIAN_POINT('Ctrl Pts',(133.784944217865,-36.5366919885432,19.0379567612371));
#20930=CARTESIAN_POINT('Ctrl Pts',(133.739991092992,-36.6474136369469,19.0321513331119));
#20931=CARTESIAN_POINT('Ctrl Pts',(133.690193160215,-36.7561176679729,19.0263459049867));
#20932=CARTESIAN_POINT('Ctrl Pts',(133.635770849495,-36.8623628352079,19.0205404768616));
#20933=CARTESIAN_POINT('Ctrl Pts',(133.581288272842,-36.9687256557357,19.0147286199477));
#20934=CARTESIAN_POINT('Ctrl Pts',(133.522171282718,-37.0726238137133,19.0089167630338));
#20935=CARTESIAN_POINT('Ctrl Pts',(133.458685731352,-37.1736416474993,19.0031049061199));
#20936=CARTESIAN_POINT('Ctrl Pts',(133.395158483429,-37.2747258285993,18.9972892320474));
#20937=CARTESIAN_POINT('Ctrl Pts',(133.327257191844,-37.3729255829226,18.9914735579748));
#20938=CARTESIAN_POINT('Ctrl Pts',(133.255289419488,-37.4678565183916,18.9856578839023));
#20939=CARTESIAN_POINT('Ctrl Pts',(133.183218563532,-37.5629234289266,18.9798338797037));
#20940=CARTESIAN_POINT('Ctrl Pts',(133.107069860903,-37.6547118622023,18.974009875505));
#20941=CARTESIAN_POINT('Ctrl Pts',(133.027189364268,-37.7428725002925,18.9681858713064));
#20942=CARTESIAN_POINT('Ctrl Pts',(133.005997570519,-37.7662609635338,18.9666407995933));
#20943=CARTESIAN_POINT('Ctrl Pts',(132.984543318965,-37.78939431269,18.9650957278803));
#20944=CARTESIAN_POINT('Ctrl Pts',(132.962833467165,-37.8122664962353,18.9635506561672));
#20945=CARTESIAN_POINT('Ctrl Pts',(132.881005718716,-37.8984752506235,18.9577270448116));
#20946=CARTESIAN_POINT('Ctrl Pts',(132.795280311605,-37.9812486725524,18.951903433456));
#20947=CARTESIAN_POINT('Ctrl Pts',(132.705977104063,-38.0602145206319,18.9460798221004));
#20948=CARTESIAN_POINT('Ctrl Pts',(132.616786563406,-38.1390807436659,18.9402635579406));
#20949=CARTESIAN_POINT('Ctrl Pts',(132.524027503426,-38.2141486792318,18.9344472937808));
#20950=CARTESIAN_POINT('Ctrl Pts',(132.428058055112,-38.285081289863,18.928631029621));
#20951=CARTESIAN_POINT('Ctrl Pts',(132.332184670638,-38.3559428981164,18.922820587446));
#20952=CARTESIAN_POINT('Ctrl Pts',(132.233107617269,-38.4226771749324,18.9170101452711));
#20953=CARTESIAN_POINT('Ctrl Pts',(132.13121922248,-38.4849863164338,18.9111997030961));
#20954=CARTESIAN_POINT('Ctrl Pts',(132.025474584566,-38.5496537166859,18.9051693489504));
#20955=CARTESIAN_POINT('Ctrl Pts',(131.91670193106,-38.6095541045878,18.8991389948047));
#20956=CARTESIAN_POINT('Ctrl Pts',(131.805374681896,-38.6644027150367,18.8931086406589));
#20957=CARTESIAN_POINT('Ctrl Pts',(131.698227993033,-38.7171916507418,18.8873047383418));
#20958=CARTESIAN_POINT('Ctrl Pts',(131.588715508498,-38.765301179574,18.8815008360246));
#20959=CARTESIAN_POINT('Ctrl Pts',(131.477285073716,-38.8085238362096,18.8756969337074));
#20960=CARTESIAN_POINT('Ctrl Pts',(131.365871097844,-38.8517401086123,18.8698938886598));
#20961=CARTESIAN_POINT('Ctrl Pts',(131.252540115701,-38.89007079666,18.8640908436121));
#20962=CARTESIAN_POINT('Ctrl Pts',(131.137759504369,-38.9233567656049,18.8582877985644));
#20963=CARTESIAN_POINT('Ctrl Pts',(131.022968759016,-38.9566456733799,18.8524842411637));
#20964=CARTESIAN_POINT('Ctrl Pts',(130.9067285222,-38.9848888627538,18.8466806837631));
#20965=CARTESIAN_POINT('Ctrl Pts',(130.789520240903,-39.0079773937991,18.8408771263625));
#20966=CARTESIAN_POINT('Ctrl Pts',(130.67227395072,-39.0310734121083,18.8350716869553));
#20967=CARTESIAN_POINT('Ctrl Pts',(130.554059392165,-39.049011368817,18.8292662475481));
#20968=CARTESIAN_POINT('Ctrl Pts',(130.435366444342,-39.0617337504003,18.823460808141));
#20969=CARTESIAN_POINT('Ctrl Pts',(130.316542057763,-39.0744702205544,18.817648939879));
#20970=CARTESIAN_POINT('Ctrl Pts',(130.197238630717,-39.0819795433496,18.8118370716169));
#20971=CARTESIAN_POINT('Ctrl Pts',(130.077949542718,-39.0842562197774,18.8060252033549));
#20972=CARTESIAN_POINT('Ctrl Pts',(129.958582106154,-39.0865343915166,18.8002095178826));
#20973=CARTESIAN_POINT('Ctrl Pts',(129.839229434664,-39.0835730825584,18.7943938324103));
#20974=CARTESIAN_POINT('Ctrl Pts',(129.720381619031,-39.0754188203207,18.7885781469381));
#20975=CARTESIAN_POINT('Ctrl Pts',(129.601363571389,-39.0672528783022,18.7827541313521));
#20976=CARTESIAN_POINT('Ctrl Pts',(129.482852227254,-39.0538791825038,18.7769301157661));
#20977=CARTESIAN_POINT('Ctrl Pts',(129.365329441072,-39.0353956784472,18.7711061001802));
#20978=CARTESIAN_POINT('Ctrl Pts',(129.334153588154,-39.0304924675669,18.7695611346531));
#20979=CARTESIAN_POINT('Ctrl Pts',(129.303047226244,-39.0252299498191,18.7680161691259));
#20980=CARTESIAN_POINT('Ctrl Pts',(129.27201917389,-39.0196105429278,18.7664712035988));
#20981=CARTESIAN_POINT('Ctrl Pts',(129.155063461701,-38.9984290092772,18.7606476816623));
#20982=CARTESIAN_POINT('Ctrl Pts',(129.038844346339,-38.9721046129996,18.7548241597257));
#20983=CARTESIAN_POINT('Ctrl Pts',(128.923848482773,-38.9407008148259,18.7490006377892));
#20984=CARTESIAN_POINT('Ctrl Pts',(128.808997706935,-38.9093366381272,18.743184463261));
#20985=CARTESIAN_POINT('Ctrl Pts',(128.695367503658,-38.8729059126443,18.7373682887328));
#20986=CARTESIAN_POINT('Ctrl Pts',(128.583436065122,-38.8315234070018,18.7315521142046));
#20987=CARTESIAN_POINT('Ctrl Pts',(128.471616671848,-38.7901823259472,18.7257417617654));
#20988=CARTESIAN_POINT('Ctrl Pts',(128.361493041206,-38.7438994664882,18.7199314093263));
#20989=CARTESIAN_POINT('Ctrl Pts',(128.253529297619,-38.6928397048511,18.7141210568872));
#20990=CARTESIAN_POINT('Ctrl Pts',(128.141477018012,-38.6398463341364,18.7080906691431));
#20991=CARTESIAN_POINT('Ctrl Pts',(128.031751879363,-38.5817072295166,18.7020602813991));
#20992=CARTESIAN_POINT('Ctrl Pts',(127.924851583423,-38.5186622527854,18.6960298936551));
#20993=CARTESIAN_POINT('Ctrl Pts',(127.821967765316,-38.4579860136645,18.6902260807628));
#20994=CARTESIAN_POINT('Ctrl Pts',(127.721700731998,-38.3927661261518,18.6844222678704));
#20995=CARTESIAN_POINT('Ctrl Pts',(127.624469484752,-38.3232634218679,18.6786184549781));
#20996=CARTESIAN_POINT('Ctrl Pts',(127.527252594828,-38.2537709804647,18.6728154990861));
#20997=CARTESIAN_POINT('Ctrl Pts',(127.433070931625,-38.1799972173488,18.6670125431941));
#20998=CARTESIAN_POINT('Ctrl Pts',(127.3423137808,-38.1022457930139,18.6612095873021));
#20999=CARTESIAN_POINT('Ctrl Pts',(127.251548611156,-38.0244874989774,18.6554061186918));
#21000=CARTESIAN_POINT('Ctrl Pts',(127.164208865598,-37.9427511106475,18.6496026500815));
#21001=CARTESIAN_POINT('Ctrl Pts',(127.080649560863,-37.85737957113,18.6437991814713));
#21002=CARTESIAN_POINT('Ctrl Pts',(126.997063152035,-37.7719803396865,18.6379938303926));
#21003=CARTESIAN_POINT('Ctrl Pts',(126.917259908267,-37.6829439037049,18.632188479314));
#21004=CARTESIAN_POINT('Ctrl Pts',(126.841556456764,-37.5906484485915,18.6263831282353));
#21005=CARTESIAN_POINT('Ctrl Pts',(126.765769156444,-37.4982507674301,18.6205713471749));
#21006=CARTESIAN_POINT('Ctrl Pts',(126.694090971559,-37.4025871778309,18.6147595661144));
#21007=CARTESIAN_POINT('Ctrl Pts',(126.6267969445,-37.3040673050859,18.6089477850539));
#21008=CARTESIAN_POINT('Ctrl Pts',(126.55945871193,-37.2054827145426,18.603132186229));
#21009=CARTESIAN_POINT('Ctrl Pts',(126.496510587499,-37.1040384503452,18.597316587404));
#21010=CARTESIAN_POINT('Ctrl Pts',(126.438182297114,-37.0001699056351,18.591500988579));
#21011=CARTESIAN_POINT('Ctrl Pts',(126.379770444036,-36.8961525560254,18.5856770581691));
#21012=CARTESIAN_POINT('Ctrl Pts',(126.325991818649,-36.7897043569867,18.5798531277592));
#21013=CARTESIAN_POINT('Ctrl Pts',(126.277028627127,-36.6812819979907,18.5740291973493));
#21014=CARTESIAN_POINT('Ctrl Pts',(126.264032582858,-36.6525040173584,18.5724833819097));
#21015=CARTESIAN_POINT('Ctrl Pts',(126.251375516676,-36.6235870446739,18.57093756647));
#21016=CARTESIAN_POINT('Ctrl Pts',(126.239060244978,-36.5945397953937,18.5693917510304));
#21017=CARTESIAN_POINT('Ctrl Pts',(126.18609618114,-36.4696168214741,18.5627436908306));
#21018=CARTESIAN_POINT('Ctrl Pts',(126.139308118626,-36.3419289321288,18.5560956306308));
#21019=CARTESIAN_POINT('Ctrl Pts',(126.098961571492,-36.2120743291181,18.549447570431));
#21020=CARTESIAN_POINT('Ctrl Pts',(126.059996554439,-36.0866661546856,18.5430271504086));
#21021=CARTESIAN_POINT('Ctrl Pts',(126.027039355238,-35.9592374719865,18.5366067303862));
#21022=CARTESIAN_POINT('Ctrl Pts',(126.000282119951,-35.8303504561443,18.5301863103638));
#21023=CARTESIAN_POINT('Ctrl Pts',(125.973599394212,-35.7018223455884,18.5237837689669));
#21024=CARTESIAN_POINT('Ctrl Pts',(125.953082273561,-35.5718442467167,18.51738122757));
#21025=CARTESIAN_POINT('Ctrl Pts',(125.938873294589,-35.4409930641106,18.5109786861731));
#21026=CARTESIAN_POINT('Ctrl Pts',(125.92472284485,-35.3106808800761,18.5046025179476));
#21027=CARTESIAN_POINT('Ctrl Pts',(125.916828774108,-35.1795030367883,18.4982263497221));
#21028=CARTESIAN_POINT('Ctrl Pts',(125.915282546399,-35.0480450231657,18.4918501814966));
#21029=CARTESIAN_POINT('Ctrl Pts',(125.915101870735,-35.0326842429822,18.4911051305421));
#21030=CARTESIAN_POINT('Ctrl Pts',(125.91500781049,-35.0173196526052,18.4903600795876));
#21031=CARTESIAN_POINT('Ctrl Pts',(125.915000466472,-35.0019521977368,18.4896150286331));
#21032=CARTESIAN_POINT('Origin',(130.,-35.,32.7603849714045));
#21033=CARTESIAN_POINT('',(132.487160670875,-31.7594357285724,20.546920387862));
#21034=CARTESIAN_POINT('',(132.487160670875,-31.7594357285724,20.4426725214427));
#21035=CARTESIAN_POINT('',(132.487160670875,-31.7594357285724,32.7603849714045));
#21036=CARTESIAN_POINT('',(125.915000768169,-34.9974948168759,19.6353849713624));
#21037=CARTESIAN_POINT('Ctrl Pts',(132.487160670875,-31.7594357285724,20.4426725214427));
#21038=CARTESIAN_POINT('Ctrl Pts',(132.581973816846,-31.8322056254144,20.4368690159672));
#21039=CARTESIAN_POINT('Ctrl Pts',(132.673580943561,-31.9091326155342,20.4310655104917));
#21040=CARTESIAN_POINT('Ctrl Pts',(132.761608938129,-31.9898935113773,20.4252620050163));
#21041=CARTESIAN_POINT('Ctrl Pts',(132.849664876522,-32.0706800441597,20.4194566572616));
#21042=CARTESIAN_POINT('Ctrl Pts',(132.934139122451,-32.1553026271649,20.4136513095069));
#21043=CARTESIAN_POINT('Ctrl Pts',(133.014694978785,-32.24340079357,20.4078459617522));
#21044=CARTESIAN_POINT('Ctrl Pts',(133.095339789209,-32.3315962426887,20.4020342034217));
#21045=CARTESIAN_POINT('Ctrl Pts',(133.172057297195,-32.4232746347158,20.3962224450911));
#21046=CARTESIAN_POINT('Ctrl Pts',(133.244550616061,-32.518041841647,20.3904106867605));
#21047=CARTESIAN_POINT('Ctrl Pts',(133.317091103821,-32.6128707103202,20.3845951469199));
#21048=CARTESIAN_POINT('Ctrl Pts',(133.385401695484,-32.7107920623311,20.3787796070793));
#21049=CARTESIAN_POINT('Ctrl Pts',(133.449229353136,-32.8113835718737,20.3729640672387));
#21050=CARTESIAN_POINT('Ctrl Pts',(133.513148928066,-32.9121199417804,20.3671401525241));
#21051=CARTESIAN_POINT('Ctrl Pts',(133.572572480076,-33.0155337916903,20.3613162378095));
#21052=CARTESIAN_POINT('Ctrl Pts',(133.627293255973,-33.1211789241196,20.3554923230949));
#21053=CARTESIAN_POINT('Ctrl Pts',(133.643396625479,-33.1522684431573,20.3537784466178));
#21054=CARTESIAN_POINT('Ctrl Pts',(133.65909304477,-33.1835510716237,20.3520645701407));
#21055=CARTESIAN_POINT('Ctrl Pts',(133.67437805383,-33.2150151492148,20.3503506936635));
#21056=CARTESIAN_POINT('Ctrl Pts',(133.726315092385,-33.3219271572154,20.3445271008662));
#21057=CARTESIAN_POINT('Ctrl Pts',(133.773665842176,-33.4312802395044,20.3387035080688));
#21058=CARTESIAN_POINT('Ctrl Pts',(133.816194276671,-33.5426440919575,20.3328799152715));
#21059=CARTESIAN_POINT('Ctrl Pts',(133.858669055222,-33.6538674423517,20.3270636698024));
#21060=CARTESIAN_POINT('Ctrl Pts',(133.896333475151,-33.7670961389996,20.3212474243333));
#21061=CARTESIAN_POINT('Ctrl Pts',(133.928997921894,-33.8818764246515,20.3154311788642));
#21062=CARTESIAN_POINT('Ctrl Pts',(133.961629671348,-33.9965418146112,20.3096207554886));
#21063=CARTESIAN_POINT('Ctrl Pts',(133.989271293318,-34.1127553132915,20.3038103321129));
#21064=CARTESIAN_POINT('Ctrl Pts',(134.011781924575,-34.2300449430975,20.2979999087373));
#21065=CARTESIAN_POINT('Ctrl Pts',(134.035144634565,-34.3517742528843,20.2919695475855));
#21066=CARTESIAN_POINT('Ctrl Pts',(134.052980079544,-34.4746623527927,20.2859391864338));
#21067=CARTESIAN_POINT('Ctrl Pts',(134.065188110948,-34.5981659265273,20.279908825282));
#21068=CARTESIAN_POINT('Ctrl Pts',(134.076937654409,-34.7170311685227,20.2741049419129));
#21069=CARTESIAN_POINT('Ctrl Pts',(134.083474806984,-34.8364660453647,20.2683010585438));
#21070=CARTESIAN_POINT('Ctrl Pts',(134.084762795524,-34.9559783655528,20.2624971751747));
#21071=CARTESIAN_POINT('Ctrl Pts',(134.086050593816,-35.0754730325862,20.2566941490967));
#21072=CARTESIAN_POINT('Ctrl Pts',(134.082090765608,-35.1950447120137,20.2508911230188));
#21073=CARTESIAN_POINT('Ctrl Pts',(134.072898649722,-35.3141999189945,20.2450880969408));
#21074=CARTESIAN_POINT('Ctrl Pts',(134.063705722259,-35.4333656462495,20.2392845585107));
#21075=CARTESIAN_POINT('Ctrl Pts',(134.049279620036,-35.5521144208015,20.2334810200806));
#21076=CARTESIAN_POINT('Ctrl Pts',(134.029687618902,-35.6699572330127,20.2276774816504));
#21077=CARTESIAN_POINT('Ctrl Pts',(134.010089264288,-35.7878382604115,20.2218720611937));
#21078=CARTESIAN_POINT('Ctrl Pts',(133.985321746008,-35.9048123385787,20.216066640737));
#21079=CARTESIAN_POINT('Ctrl Pts',(133.955503447826,-36.0204006439795,20.2102612202802));
#21080=CARTESIAN_POINT('Ctrl Pts',(133.925652128563,-36.1361169530231,20.204449370843));
#21081=CARTESIAN_POINT('Ctrl Pts',(133.890738966784,-36.2504440304432,20.1986375214057));
#21082=CARTESIAN_POINT('Ctrl Pts',(133.850932270891,-36.3629180624723,20.1928256719684));
#21083=CARTESIAN_POINT('Ctrl Pts',(133.811099429694,-36.4754659681972,20.1870100052696));
#21084=CARTESIAN_POINT('Ctrl Pts',(133.766366806055,-36.5861580269391,20.1811943385708));
#21085=CARTESIAN_POINT('Ctrl Pts',(133.716950257289,-36.6945517946766,20.175378671872));
#21086=CARTESIAN_POINT('Ctrl Pts',(133.667462924501,-36.8031008251138,20.1695546748408));
#21087=CARTESIAN_POINT('Ctrl Pts',(133.613278460185,-36.9093446313024,20.1637306778096));
#21088=CARTESIAN_POINT('Ctrl Pts',(133.554657961643,-37.0128665568614,20.1579066807784));
#21089=CARTESIAN_POINT('Ctrl Pts',(133.539105539269,-37.0403316373585,20.1563615342173));
#21090=CARTESIAN_POINT('Ctrl Pts',(133.523241105197,-37.0676052971867,20.1548163876562));
#21091=CARTESIAN_POINT('Ctrl Pts',(133.507070025072,-37.0946801281448,20.1532712410951));
#21092=CARTESIAN_POINT('Ctrl Pts',(133.446121885322,-37.1967240589228,20.1474476468881));
#21093=CARTESIAN_POINT('Ctrl Pts',(133.380618063255,-37.2962702566973,20.1416240526811));
#21094=CARTESIAN_POINT('Ctrl Pts',(133.31078907183,-37.3928854385135,20.1358004584741));
#21095=CARTESIAN_POINT('Ctrl Pts',(133.24104818012,-37.4893787258295,20.129984211602));
#21096=CARTESIAN_POINT('Ctrl Pts',(133.166993209679,-37.5829480242237,20.12416796473));
#21097=CARTESIAN_POINT('Ctrl Pts',(133.088899730329,-37.6731860122284,20.118351717858));
#21098=CARTESIAN_POINT('Ctrl Pts',(133.01088442307,-37.7633336714078,20.1125412930877));
#21099=CARTESIAN_POINT('Ctrl Pts',(132.928838914779,-37.8501563471065,20.1067308683174));
#21100=CARTESIAN_POINT('Ctrl Pts',(132.843080737952,-37.9332775043436,20.1009204435472));
#21101=CARTESIAN_POINT('Ctrl Pts',(132.754076447675,-38.0195449587201,20.0948900829213));
#21102=CARTESIAN_POINT('Ctrl Pts',(132.661073134648,-38.1018247753736,20.0888597222954));
#21103=CARTESIAN_POINT('Ctrl Pts',(132.564470314909,-38.1797353669689,20.0828293616696));
#21104=CARTESIAN_POINT('Ctrl Pts',(132.471495505345,-38.2547199526789,20.0770254769351));
#21105=CARTESIAN_POINT('Ctrl Pts',(132.375187025567,-38.3256572963924,20.0712215922007));
#21106=CARTESIAN_POINT('Ctrl Pts',(132.275936372773,-38.3922468405305,20.0654177074662));
#21107=CARTESIAN_POINT('Ctrl Pts',(132.176700380505,-38.4588265485846,20.059614680036));
#21108=CARTESIAN_POINT('Ctrl Pts',(132.074523418492,-38.5210595068002,20.0538116526058));
#21109=CARTESIAN_POINT('Ctrl Pts',(131.969826631532,-38.5786880335823,20.0480086251756));
#21110=CARTESIAN_POINT('Ctrl Pts',(131.865120601104,-38.6363216482714,20.0422050854077));
#21111=CARTESIAN_POINT('Ctrl Pts',(131.757894661149,-38.6893498263612,20.0364015456399));
#21112=CARTESIAN_POINT('Ctrl Pts',(131.648594683529,-38.7375607780262,20.030598005872));
#21113=CARTESIAN_POINT('Ctrl Pts',(131.539259261383,-38.7857873638604,20.0247925840935));
#21114=CARTESIAN_POINT('Ctrl Pts',(131.42784883737,-38.8291934517726,20.018987162315));
#21115=CARTESIAN_POINT('Ctrl Pts',(131.314828779498,-38.8676155807685,20.0131817405366));
#21116=CARTESIAN_POINT('Ctrl Pts',(131.201683562701,-38.9060802586044,20.0073698898076));
#21117=CARTESIAN_POINT('Ctrl Pts',(131.086925540826,-38.9395498291027,20.0015580390787));
#21118=CARTESIAN_POINT('Ctrl Pts',(130.971034895023,-38.9679108146036,19.9957461883498));
#21119=CARTESIAN_POINT('Ctrl Pts',(130.855068131805,-38.9962904277069,19.9899305203754));
#21120=CARTESIAN_POINT('Ctrl Pts',(130.73796766273,-39.0195546941866,19.984114852401));
#21121=CARTESIAN_POINT('Ctrl Pts',(130.620221860504,-39.0376416190337,19.9782991844266));
#21122=CARTESIAN_POINT('Ctrl Pts',(130.502307400478,-39.0557544513943,19.9724751861529));
#21123=CARTESIAN_POINT('Ctrl Pts',(130.383746166805,-39.0686750961732,19.9666511878792));
#21124=CARTESIAN_POINT('Ctrl Pts',(130.265029763085,-39.0763935316256,19.9608271896056));
#21125=CARTESIAN_POINT('Ctrl Pts',(130.233533751809,-39.0784412682687,19.9592820559126));
#21126=CARTESIAN_POINT('Ctrl Pts',(130.20202680599,-39.0801231235685,19.9577369222196));
#21127=CARTESIAN_POINT('Ctrl Pts',(130.170518062655,-39.0814395242743,19.9561917885266));
#21128=CARTESIAN_POINT('Ctrl Pts',(130.051761867813,-39.0864010277223,19.9503681923283));
#21129=CARTESIAN_POINT('Ctrl Pts',(129.932597446586,-39.0861831196748,19.94454459613));
#21130=CARTESIAN_POINT('Ctrl Pts',(129.813513543482,-39.0807410848442,19.9387209999317));
#21131=CARTESIAN_POINT('Ctrl Pts',(129.694579882059,-39.0753059159329,19.9329047510479));
#21132=CARTESIAN_POINT('Ctrl Pts',(129.575726941025,-39.0646597480532,19.9270885021641));
#21133=CARTESIAN_POINT('Ctrl Pts',(129.457446449946,-39.0488097813214,19.9212722532804));
#21134=CARTESIAN_POINT('Ctrl Pts',(129.339284358021,-39.0329756804576,19.9154618264805));
#21135=CARTESIAN_POINT('Ctrl Pts',(129.221693978482,-39.0119481973629,19.9096513996806));
#21136=CARTESIAN_POINT('Ctrl Pts',(129.105164294347,-38.9857865045544,19.9038409728807));
#21137=CARTESIAN_POINT('Ctrl Pts',(128.984223792851,-38.9586345537728,19.897810613009));
#21138=CARTESIAN_POINT('Ctrl Pts',(128.864426318758,-38.9259520597147,19.8917802531372));
#21139=CARTESIAN_POINT('Ctrl Pts',(128.746310020357,-38.8878639938842,19.8857498932654));
#21140=CARTESIAN_POINT('Ctrl Pts',(128.632629636571,-38.8512063437561,19.8799460064703));
#21141=CARTESIAN_POINT('Ctrl Pts',(128.520506854486,-38.8095419542711,19.8741421196751));
#21142=CARTESIAN_POINT('Ctrl Pts',(128.410407656527,-38.7630335078993,19.86833823288));
#21143=CARTESIAN_POINT('Ctrl Pts',(128.300324721403,-38.7165319313245,19.8625352033812));
#21144=CARTESIAN_POINT('Ctrl Pts',(128.192265152028,-38.6651878796574,19.8567321738825));
#21145=CARTESIAN_POINT('Ctrl Pts',(128.086675322317,-38.6092123348132,19.8509291443837));
#21146=CARTESIAN_POINT('Ctrl Pts',(127.981076170194,-38.5532318479493,19.8451256025418));
#21147=CARTESIAN_POINT('Ctrl Pts',(127.877947552067,-38.4926192461628,19.8393220607));
#21148=CARTESIAN_POINT('Ctrl Pts',(127.77771101376,-38.427631348561,19.8335185188581));
#21149=CARTESIAN_POINT('Ctrl Pts',(127.677441970036,-38.3626223762214,19.8277130950023));
#21150=CARTESIAN_POINT('Ctrl Pts',(127.580067213783,-38.2932355083157,19.8219076711466));
#21151=CARTESIAN_POINT('Ctrl Pts',(127.485978557059,-38.2197703620652,19.8161022472909));
#21152=CARTESIAN_POINT('Ctrl Pts',(127.39178570626,-38.1462238602805,19.8102903944905));
#21153=CARTESIAN_POINT('Ctrl Pts',(127.300886540859,-38.0685903166835,19.8044785416901));
#21154=CARTESIAN_POINT('Ctrl Pts',(127.213639188317,-37.9872091368231,19.7986666888897));
#21155=CARTESIAN_POINT('Ctrl Pts',(127.12633453142,-37.9057745055292,19.7928510188448));
#21156=CARTESIAN_POINT('Ctrl Pts',(127.042686749539,-37.8205876265996,19.7870353487999));
#21157=CARTESIAN_POINT('Ctrl Pts',(126.963015401848,-37.732022977683,19.7812196787549));
#21158=CARTESIAN_POINT('Ctrl Pts',(126.883229934067,-37.6433314700399,19.7753956784281));
#21159=CARTESIAN_POINT('Ctrl Pts',(126.807432527555,-37.55125284963,19.7695716781012));
#21160=CARTESIAN_POINT('Ctrl Pts',(126.735901043608,-37.4561927861793,19.7637476777744));
#21161=CARTESIAN_POINT('Ctrl Pts',(126.716923659215,-37.4309732427707,19.7622025638356));
#21162=CARTESIAN_POINT('Ctrl Pts',(126.698246285856,-37.4055439965965,19.7606574498969));
#21163=CARTESIAN_POINT('Ctrl Pts',(126.679873575016,-37.3799129232232,19.7591123359582));
#21164=CARTESIAN_POINT('Ctrl Pts',(126.61011205585,-37.2825912687329,19.7532455100666));
#21165=CARTESIAN_POINT('Ctrl Pts',(126.544521954487,-37.1820446244611,19.7473786841751));
#21166=CARTESIAN_POINT('Ctrl Pts',(126.483412467191,-37.078662340086,19.7415118582836));
#21167=CARTESIAN_POINT('Ctrl Pts',(126.422382088058,-36.9754138873468,19.7356526271837));
#21168=CARTESIAN_POINT('Ctrl Pts',(126.36582098778,-36.8693374369891,19.7297933960838));
#21169=CARTESIAN_POINT('Ctrl Pts',(126.313996697074,-36.7608533870868,19.7239341649839));
#21170=CARTESIAN_POINT('Ctrl Pts',(126.262227895367,-36.6524854925888,19.7180812074455));
#21171=CARTESIAN_POINT('Ctrl Pts',(126.215185984591,-36.5417154858371,19.7122282499071));
#21172=CARTESIAN_POINT('Ctrl Pts',(126.173093650344,-36.4289901297627,19.7063752923687));
#21173=CARTESIAN_POINT('Ctrl Pts',(126.130548943974,-36.3150532987387,19.7004594322883));
#21174=CARTESIAN_POINT('Ctrl Pts',(126.093061051907,-36.1991191920976,19.694543572208));
#21175=CARTESIAN_POINT('Ctrl Pts',(126.060811055506,-36.0816725288085,19.6886277121276));
#21176=CARTESIAN_POINT('Ctrl Pts',(126.028952031247,-35.9656496912095,19.6827835710159));
#21177=CARTESIAN_POINT('Ctrl Pts',(126.002204712301,-35.8481511652892,19.6769394299042));
#21178=CARTESIAN_POINT('Ctrl Pts',(125.980694158762,-35.7296612601705,19.6710952887925));
#21179=CARTESIAN_POINT('Ctrl Pts',(125.958787640782,-35.6089902029473,19.6651435692279));
#21180=CARTESIAN_POINT('Ctrl Pts',(125.942312718397,-35.4872913124443,19.6591918496632));
#21181=CARTESIAN_POINT('Ctrl Pts',(125.93134717999,-35.3650879760073,19.6532401300985));
#21182=CARTESIAN_POINT('Ctrl Pts',(125.920381641583,-35.2428846395704,19.6472884105338));
#21183=CARTESIAN_POINT('Ctrl Pts',(125.914925531444,-35.1201772941067,19.6413366909692));
#21184=CARTESIAN_POINT('Ctrl Pts',(125.915000768169,-34.9974948177444,19.6353849714045));
#21185=CARTESIAN_POINT('Ctrl Pts',(125.915000768169,-34.9974948168759,19.6353849713624));
#21186=CARTESIAN_POINT('Ctrl Pts',(125.915083357695,-34.8628227653834,19.6288515991363));
#21187=CARTESIAN_POINT('Ctrl Pts',(125.921829701158,-34.7283970455392,19.6223182269103));
#21188=CARTESIAN_POINT('Ctrl Pts',(125.935142558186,-34.5948346291612,19.6157848546842));
#21189=CARTESIAN_POINT('Ctrl Pts',(125.948507987138,-34.4607447803019,19.6092256824403));
#21190=CARTESIAN_POINT('Ctrl Pts',(125.968491780673,-34.3275252624722,19.6026665101964));
#21191=CARTESIAN_POINT('Ctrl Pts',(125.994945663311,-34.1957831385947,19.5961073379525));
#21192=CARTESIAN_POINT('Ctrl Pts',(126.021539621642,-34.0633434282967,19.5895134343004));
#21193=CARTESIAN_POINT('Ctrl Pts',(126.05467226789,-33.9323969920297,19.5829195306483));
#21194=CARTESIAN_POINT('Ctrl Pts',(126.09414425753,-33.8035402560003,19.5763256269961));
#21195=CARTESIAN_POINT('Ctrl Pts',(126.122663682811,-33.7104382844833,19.5715613791273));
#21196=CARTESIAN_POINT('Ctrl Pts',(126.154491475401,-33.6184268020555,19.5667971312585));
#21197=CARTESIAN_POINT('Ctrl Pts',(126.189537223219,-33.5277233864641,19.5620328833897));
#21198=CARTESIAN_POINT('Ctrl Pts',(126.23237555984,-33.4168516347736,19.5562092823351));
#21199=CARTESIAN_POINT('Ctrl Pts',(126.280125989455,-33.3076723261669,19.5503856812804));
#21200=CARTESIAN_POINT('Ctrl Pts',(126.332634487578,-33.2006514516925,19.5445620802257));
#21201=CARTESIAN_POINT('Ctrl Pts',(126.385076738051,-33.0937656007214,19.5387458265509));
#21202=CARTESIAN_POINT('Ctrl Pts',(126.44226493884,-32.9890331308576,19.5329295728761));
#21203=CARTESIAN_POINT('Ctrl Pts',(126.503996271198,-32.8869020542812,19.5271133192013));
#21204=CARTESIAN_POINT('Ctrl Pts',(126.5656658096,-32.7848732123888,19.5213028876804));
#21205=CARTESIAN_POINT('Ctrl Pts',(126.631869222394,-32.685440930835,19.5154924561596));
#21206=CARTESIAN_POINT('Ctrl Pts',(126.702357131409,-32.5890299646765,19.5096820246388));
#21207=CARTESIAN_POINT('Ctrl Pts',(126.775513028668,-32.4889698148787,19.5036516665631));
#21208=CARTESIAN_POINT('Ctrl Pts',(126.853283971756,-32.3921646170861,19.4976213084873));
#21209=CARTESIAN_POINT('Ctrl Pts',(126.935340631508,-32.2990579504334,19.4915909504116));
#21210=CARTESIAN_POINT('Ctrl Pts',(127.014315698788,-32.2094478531512,19.4857870590981));
#21211=CARTESIAN_POINT('Ctrl Pts',(127.097260097743,-32.1232638377191,19.4799831677846));
#21212=CARTESIAN_POINT('Ctrl Pts',(127.183838716184,-32.0408682652616,19.4741792764712));
#21213=CARTESIAN_POINT('Ctrl Pts',(127.270404544818,-31.9584848646717,19.4683762425362));
#21214=CARTESIAN_POINT('Ctrl Pts',(127.360603229571,-31.8798890755223,19.4625732086013));
#21215=CARTESIAN_POINT('Ctrl Pts',(127.454063195155,-31.8054060061196,19.4567701746663));
#21216=CARTESIAN_POINT('Ctrl Pts',(127.547531410817,-31.7309163618041,19.4509666284748));
#21217=CARTESIAN_POINT('Ctrl Pts',(127.64426116035,-31.6605404135621,19.4451630822833));
#21218=CARTESIAN_POINT('Ctrl Pts',(127.743848745869,-31.5945622133882,19.4393595360918));
#21219=CARTESIAN_POINT('Ctrl Pts',(127.843468624772,-31.5285626183855,19.4335541079775));
#21220=CARTESIAN_POINT('Ctrl Pts',(127.945947842454,-31.4669638329767,19.4277486798632));
#21221=CARTESIAN_POINT('Ctrl Pts',(128.050855322594,-31.4100055673388,19.4219432517489));
#21222=CARTESIAN_POINT('Ctrl Pts',(128.155878974712,-31.3529842275098,19.4161313948455));
#21223=CARTESIAN_POINT('Ctrl Pts',(128.263335897692,-31.3006138598848,19.410319537942));
#21224=CARTESIAN_POINT('Ctrl Pts',(128.372771973071,-31.2530874111643,19.4045076810385));
#21225=CARTESIAN_POINT('Ctrl Pts',(128.482279924769,-31.2055297476345,19.3986920069762));
#21226=CARTESIAN_POINT('Ctrl Pts',(128.593769237178,-31.1628224846373,19.3928763329138));
#21227=CARTESIAN_POINT('Ctrl Pts',(128.706769022905,-31.1251092092962,19.3870606588515));
#21228=CARTESIAN_POINT('Ctrl Pts',(128.819930664764,-31.0873419150481,19.3812366546626));
#21229=CARTESIAN_POINT('Ctrl Pts',(128.93460670701,-31.0545829975725,19.3754126504737));
#21230=CARTESIAN_POINT('Ctrl Pts',(129.050314299865,-31.026925363027,19.3695886462848));
#21231=CARTESIAN_POINT('Ctrl Pts',(129.081010799286,-31.0195879658703,19.3680435744636));
#21232=CARTESIAN_POINT('Ctrl Pts',(129.11177986451,-31.0126093186781,19.3664985026424));
#21233=CARTESIAN_POINT('Ctrl Pts',(129.142612418793,-31.005990543878,19.3649534308213));
#21234=CARTESIAN_POINT('Ctrl Pts',(129.258835029655,-30.9810412230756,19.3591293177954));
#21235=CARTESIAN_POINT('Ctrl Pts',(129.376334978398,-30.9611288626928,19.3533052047695));
#21236=CARTESIAN_POINT('Ctrl Pts',(129.494637967476,-30.9463801095708,19.3474810917436));
#21237=CARTESIAN_POINT('Ctrl Pts',(129.61278929623,-30.9316502638382,19.3416644450284));
#21238=CARTESIAN_POINT('Ctrl Pts',(129.731741215775,-30.9220709082435,19.3358477983132));
#21239=CARTESIAN_POINT('Ctrl Pts',(129.851007744688,-30.9177180024088,19.330031151598));
#21240=CARTESIAN_POINT('Ctrl Pts',(129.970134825831,-30.9133701860407,19.3242213057718));
#21241=CARTESIAN_POINT('Ctrl Pts',(130.089575378288,-30.9142366686104,19.3184114599455));
#21242=CARTESIAN_POINT('Ctrl Pts',(130.208837598351,-30.9203416984366,19.3126016141192));
#21243=CARTESIAN_POINT('Ctrl Pts',(130.32802135689,-30.9264427118196,19.3067955905373));
#21244=CARTESIAN_POINT('Ctrl Pts',(130.447026610071,-30.937775398331,19.3009895669555));
#21245=CARTESIAN_POINT('Ctrl Pts',(130.565361081706,-30.9543119438973,19.2951835433736));
#21246=CARTESIAN_POINT('Ctrl Pts',(130.683645629729,-30.9708415129327,19.2893799692696));
#21247=CARTESIAN_POINT('Ctrl Pts',(130.801259555445,-30.9925705175673,19.2835763951656));
#21248=CARTESIAN_POINT('Ctrl Pts',(130.917715872798,-31.0194193166304,19.2777728210616));
#21249=CARTESIAN_POINT('Ctrl Pts',(131.034150542079,-31.0462631247686,19.2719703257844));
#21250=CARTESIAN_POINT('Ctrl Pts',(131.149427633751,-31.0782247411371,19.2661678305072));
#21251=CARTESIAN_POINT('Ctrl Pts',(131.263071151461,-31.1151735860729,19.2603653352299));
#21252=CARTESIAN_POINT('Ctrl Pts',(131.37676782237,-31.1521397126744,19.2545601260171));
#21253=CARTESIAN_POINT('Ctrl Pts',(131.48882900263,-31.1940976062958,19.2487549168043));
#21254=CARTESIAN_POINT('Ctrl Pts',(131.598794675586,-31.2408670434104,19.2429497075916));
#21255=CARTESIAN_POINT('Ctrl Pts',(131.708783852424,-31.2876464769478,19.2371432575829));
#21256=CARTESIAN_POINT('Ctrl Pts',(131.816676258096,-31.3392393327794,19.2313368075742));
#21257=CARTESIAN_POINT('Ctrl Pts',(131.92203391114,-31.3954181040753,19.2255303575655));
#21258=CARTESIAN_POINT('Ctrl Pts',(132.027506882934,-31.4516583655951,19.2197175521328));
#21259=CARTESIAN_POINT('Ctrl Pts',(132.13043920323,-31.5124943695596,19.2139047467001));
#21260=CARTESIAN_POINT('Ctrl Pts',(132.23041920653,-31.5776535588658,19.2080919412675));
#21261=CARTESIAN_POINT('Ctrl Pts',(132.318370563582,-31.6349734121843,19.2029784774826));
#21262=CARTESIAN_POINT('Ctrl Pts',(132.404037533551,-31.6956380129049,19.1978650136977));
#21263=CARTESIAN_POINT('Ctrl Pts',(132.487160670875,-31.7594357285724,19.1927515499128));
#21264=CARTESIAN_POINT('',(125.915000261184,-35.0014607794641,19.7396150285596));
#21265=CARTESIAN_POINT('Ctrl Pts',(125.915000261184,-35.0014607794641,19.7396150285596));
#21266=CARTESIAN_POINT('Ctrl Pts',(125.914958122368,-34.8836216006865,19.7338448931807));
#21267=CARTESIAN_POINT('Ctrl Pts',(125.920019141927,-34.7655803622538,19.7280747578018));
#21268=CARTESIAN_POINT('Ctrl Pts',(125.930209565061,-34.647819910157,19.722304622423));
#21269=CARTESIAN_POINT('Ctrl Pts',(125.940387587582,-34.5302027594559,19.7165415086582));
#21270=CARTESIAN_POINT('Ctrl Pts',(125.95568256745,-34.4128661270332,19.7107783948935));
#21271=CARTESIAN_POINT('Ctrl Pts',(125.976068747181,-34.296293901839,19.7050152811287));
#21272=CARTESIAN_POINT('Ctrl Pts',(125.99643568078,-34.1798317298528,19.6992576081897));
#21273=CARTESIAN_POINT('Ctrl Pts',(126.021884184083,-34.0641329379567,19.6934999352506));
#21274=CARTESIAN_POINT('Ctrl Pts',(126.052336666458,-33.9496766188433,19.6877422623115));
#21275=CARTESIAN_POINT('Ctrl Pts',(126.082770032877,-33.8352921474657,19.6819882036401));
#21276=CARTESIAN_POINT('Ctrl Pts',(126.118201025278,-33.722148999268,19.6762341449686));
#21277=CARTESIAN_POINT('Ctrl Pts',(126.158501038491,-33.6107157494872,19.6704800862971));
#21278=CARTESIAN_POINT('Ctrl Pts',(126.198788206539,-33.4993180177683,19.6647278616654));
#21279=CARTESIAN_POINT('Ctrl Pts',(126.243941169215,-33.3896294924763,19.6589756370337));
#21280=CARTESIAN_POINT('Ctrl Pts',(126.293781763902,-33.2821026263431,19.653223412402));
#21281=CARTESIAN_POINT('Ctrl Pts',(126.343618775953,-33.1745834894454,19.6474716012511));
#21282=CARTESIAN_POINT('Ctrl Pts',(126.398142574666,-33.0692260805372,19.6417197901003));
#21283=CARTESIAN_POINT('Ctrl Pts',(126.457127560634,-32.9664612424684,19.6359679789494));
#21284=CARTESIAN_POINT('Ctrl Pts',(126.516122867989,-32.8636784222707,19.6302151613278));
#21285=CARTESIAN_POINT('Ctrl Pts',(126.579580706547,-32.763489435633,19.6244623437061));
#21286=CARTESIAN_POINT('Ctrl Pts',(126.647230782565,-32.6662983107046,19.6187095260844));
#21287=CARTESIAN_POINT('Ctrl Pts',(126.714949685685,-32.5690083036481,19.6129508555534));
#21288=CARTESIAN_POINT('Ctrl Pts',(126.78686910445,-32.4747225907782,19.6071921850223));
#21289=CARTESIAN_POINT('Ctrl Pts',(126.862676808916,-32.3838141895719,19.6014335144912));
#21290=CARTESIAN_POINT('Ctrl Pts',(126.938525657659,-32.2928564482559,19.5956717184686));
#21291=CARTESIAN_POINT('Ctrl Pts',(127.018266713885,-32.2052799760541,19.589909922446));
#21292=CARTESIAN_POINT('Ctrl Pts',(127.10155029257,-32.1214214804004,19.5841481264234));
#21293=CARTESIAN_POINT('Ctrl Pts',(127.184962488869,-32.0374334792696,19.5783774322667));
#21294=CARTESIAN_POINT('Ctrl Pts',(127.271927827314,-31.9571752034551,19.57260673811));
#21295=CARTESIAN_POINT('Ctrl Pts',(127.362062681455,-31.8809437800148,19.5668360439533));
#21296=CARTESIAN_POINT('Ctrl Pts',(127.424785193379,-31.8278963056356,19.5628203672597));
#21297=CARTESIAN_POINT('Ctrl Pts',(127.489041833148,-31.7767979365938,19.5588046905661));
#21298=CARTESIAN_POINT('Ctrl Pts',(127.554695457865,-31.7277361511926,19.5547890138725));
#21299=CARTESIAN_POINT('Ctrl Pts',(127.649907355974,-31.6565859940937,19.5489654176607));
#21300=CARTESIAN_POINT('Ctrl Pts',(127.748380713119,-31.5894800720813,19.5431418214489));
#21301=CARTESIAN_POINT('Ctrl Pts',(127.849737400708,-31.5267312580099,19.5373182252371));
#21302=CARTESIAN_POINT('Ctrl Pts',(127.95096621208,-31.4640616107024,19.5315019763397));
#21303=CARTESIAN_POINT('Ctrl Pts',(128.055070774387,-31.4057383507268,19.5256857274423));
#21304=CARTESIAN_POINT('Ctrl Pts',(128.161641181523,-31.352033188949,19.5198694785449));
#21305=CARTESIAN_POINT('Ctrl Pts',(128.268104911339,-31.2983817862112,19.5140590517314));
#21306=CARTESIAN_POINT('Ctrl Pts',(128.377029213014,-31.249339468026,19.5082486249179));
#21307=CARTESIAN_POINT('Ctrl Pts',(128.487977101229,-31.2051334998985,19.5024381981043));
#21308=CARTESIAN_POINT('Ctrl Pts',(128.603124527375,-31.159254271983,19.4964078382377));
#21309=CARTESIAN_POINT('Ctrl Pts',(128.720451377084,-31.118584989689,19.490377478371));
#21310=CARTESIAN_POINT('Ctrl Pts',(128.83944293416,-31.083326373448,19.4843471185043));
#21311=CARTESIAN_POINT('Ctrl Pts',(128.953965706223,-31.0493919114555,19.4785432316955));
#21312=CARTESIAN_POINT('Ctrl Pts',(129.070029976031,-31.0204691704228,19.4727393448867));
#21313=CARTESIAN_POINT('Ctrl Pts',(129.18715929488,-30.996686998485,19.4669354580779));
#21314=CARTESIAN_POINT('Ctrl Pts',(129.30427131247,-30.9729083394294,19.4611324285656));
#21315=CARTESIAN_POINT('Ctrl Pts',(129.422447666179,-30.9542688206558,19.4553293990532));
#21316=CARTESIAN_POINT('Ctrl Pts',(129.541200818743,-30.9408463553004,19.4495263695409));
#21317=CARTESIAN_POINT('Ctrl Pts',(129.659964455893,-30.9274227048903,19.4437228276854));
#21318=CARTESIAN_POINT('Ctrl Pts',(129.779304587376,-30.9192170695619,19.4379192858299));
#21319=CARTESIAN_POINT('Ctrl Pts',(129.898728285557,-30.9162555124183,19.4321157439744));
#21320=CARTESIAN_POINT('Ctrl Pts',(130.018190711304,-30.9132929948799,19.4263103201051));
#21321=CARTESIAN_POINT('Ctrl Pts',(130.137736349643,-30.9155779477278,19.4205048962358));
#21322=CARTESIAN_POINT('Ctrl Pts',(130.25687264739,-30.9230843223066,19.4146994723666));
#21323=CARTESIAN_POINT('Ctrl Pts',(130.376140877046,-30.9305990094679,19.4088876195528));
#21324=CARTESIAN_POINT('Ctrl Pts',(130.494998453504,-30.9433466344716,19.403075766739));
#21325=CARTESIAN_POINT('Ctrl Pts',(130.61295815825,-30.9612492901599,19.3972639139252));
#21326=CARTESIAN_POINT('Ctrl Pts',(130.730995339327,-30.9791637043725,19.391448243867));
#21327=CARTESIAN_POINT('Ctrl Pts',(130.848133074523,-31.0022398135148,19.3856325738087));
#21328=CARTESIAN_POINT('Ctrl Pts',(130.96389617366,-31.0303489868247,19.3798169037505));
#21329=CARTESIAN_POINT('Ctrl Pts',(131.079825090187,-31.0584984233081,19.3739929034105));
#21330=CARTESIAN_POINT('Ctrl Pts',(131.194375049813,-31.0916952000503,19.3681689030705));
#21331=CARTESIAN_POINT('Ctrl Pts',(131.307087664496,-31.1297613978822,19.3623449027305));
#21332=CARTESIAN_POINT('Ctrl Pts',(131.336990447327,-31.1398604027732,19.3607997889217));
#21333=CARTESIAN_POINT('Ctrl Pts',(131.36676402913,-31.1503018823635,19.3592546751129));
#21334=CARTESIAN_POINT('Ctrl Pts',(131.396400123974,-31.1610819631353,19.3577095613041));
#21335=CARTESIAN_POINT('Ctrl Pts',(131.508084011257,-31.2017067935042,19.3518867861588));
#21336=CARTESIAN_POINT('Ctrl Pts',(131.618173684181,-31.2472749228511,19.3460640110134));
#21337=CARTESIAN_POINT('Ctrl Pts',(131.726200384617,-31.297641666161,19.340241235868));
#21338=CARTESIAN_POINT('Ctrl Pts',(131.834107403958,-31.3479526089421,19.3344249116844));
#21339=CARTESIAN_POINT('Ctrl Pts',(131.939955626777,-31.4030514283356,19.3286085875007));
#21340=CARTESIAN_POINT('Ctrl Pts',(132.043293084972,-31.4627442319075,19.3227922633171));
#21341=CARTESIAN_POINT('Ctrl Pts',(132.146519156579,-31.5223726931019,19.316982208501));
#21342=CARTESIAN_POINT('Ctrl Pts',(132.247239497912,-31.5865850807773,19.3111721536849));
#21343=CARTESIAN_POINT('Ctrl Pts',(132.345024568614,-31.6551405451656,19.3053620988688));
#21344=CARTESIAN_POINT('Ctrl Pts',(132.393129567781,-31.6888661490192,19.3025038641702));
#21345=CARTESIAN_POINT('Ctrl Pts',(132.440524554963,-31.723642112516,19.2996456294715));
#21346=CARTESIAN_POINT('Ctrl Pts',(132.487160670875,-31.7594357285724,19.2967873947729));
#21347=CARTESIAN_POINT('Ctrl Pts',(132.487160670875,-31.7594357285724,20.546920387862));
#21348=CARTESIAN_POINT('Ctrl Pts',(132.523548068931,-31.7873633664098,20.5446756841462));
#21349=CARTESIAN_POINT('Ctrl Pts',(132.55944402042,-31.8158878360481,20.5424309804305));
#21350=CARTESIAN_POINT('Ctrl Pts',(132.594828390306,-31.8449895998809,20.5401862767148));
#21351=CARTESIAN_POINT('Ctrl Pts',(132.686628563226,-31.9204903636558,20.5343626831361));
#21352=CARTESIAN_POINT('Ctrl Pts',(132.775278808919,-32.0001228172305,20.5285390895573));
#21353=CARTESIAN_POINT('Ctrl Pts',(132.860385118183,-32.0835943396574,20.5227154959786));
#21354=CARTESIAN_POINT('Ctrl Pts',(132.945384053196,-32.1669605503598,20.5168992497283));
#21355=CARTESIAN_POINT('Ctrl Pts',(133.026847655943,-32.2541559127918,20.5110830034779));
#21356=CARTESIAN_POINT('Ctrl Pts',(133.104414314979,-32.3448471303985,20.5052667572275));
#21357=CARTESIAN_POINT('Ctrl Pts',(133.181903329363,-32.4354475655976,20.4994563330716));
#21358=CARTESIAN_POINT('Ctrl Pts',(133.255502896433,-32.5295365858737,20.4936459089157));
#21359=CARTESIAN_POINT('Ctrl Pts',(133.324888111438,-32.6267439989716,20.4878354847598));
#21360=CARTESIAN_POINT('Ctrl Pts',(133.396899701905,-32.7276309159011,20.481805123901));
#21361=CARTESIAN_POINT('Ctrl Pts',(133.464371272422,-32.8318766516566,20.4757747630421));
#21362=CARTESIAN_POINT('Ctrl Pts',(133.526985163046,-32.9390291948563,20.4697444021832));
#21363=CARTESIAN_POINT('Ctrl Pts',(133.587247521362,-33.0421575085327,20.4639405180413));
#21364=CARTESIAN_POINT('Ctrl Pts',(133.643010266103,-33.1479778462274,20.4581366338994));
#21365=CARTESIAN_POINT('Ctrl Pts',(133.694034661689,-33.2560582239541,20.4523327497575));
#21366=CARTESIAN_POINT('Ctrl Pts',(133.745051520432,-33.3641226370634,20.4465297229109));
#21367=CARTESIAN_POINT('Ctrl Pts',(133.791331247631,-33.4744460571622,20.4407266960642));
#21368=CARTESIAN_POINT('Ctrl Pts',(133.83268192967,-33.586573586641,20.4349236692176));
#21369=CARTESIAN_POINT('Ctrl Pts',(133.874036262546,-33.6987110158207,20.4291201300237));
#21370=CARTESIAN_POINT('Ctrl Pts',(133.910460543719,-33.8126524879418,20.4233165908298));
#21371=CARTESIAN_POINT('Ctrl Pts',(133.941811928845,-33.9279255074333,20.4175130516359));
#21372=CARTESIAN_POINT('Ctrl Pts',(133.973173480865,-34.0432359086363,20.4117076304211));
#21373=CARTESIAN_POINT('Ctrl Pts',(133.999458758033,-34.1598783221522,20.4059022092063));
#21374=CARTESIAN_POINT('Ctrl Pts',(134.020575614019,-34.2773681906033,20.4000967879916));
#21375=CARTESIAN_POINT('Ctrl Pts',(134.041715854976,-34.3949881682423,20.3942849378085));
#21376=CARTESIAN_POINT('Ctrl Pts',(134.057676177778,-34.5134570719638,20.3884730876255));
#21377=CARTESIAN_POINT('Ctrl Pts',(134.068416070864,-34.6322831601186,20.3826612374424));
#21378=CARTESIAN_POINT('Ctrl Pts',(134.079163017972,-34.7511872939037,20.3768455700041));
#21379=CARTESIAN_POINT('Ctrl Pts',(134.084682687972,-34.8704486723726,20.3710299025658));
#21380=CARTESIAN_POINT('Ctrl Pts',(134.084986697936,-34.9895751408295,20.3652142351274));
#21381=CARTESIAN_POINT('Ctrl Pts',(134.085291143361,-35.1088722451291,20.3593902373715));
#21382=CARTESIAN_POINT('Ctrl Pts',(134.080365034102,-35.2280336471716,20.3535662396156));
#21383=CARTESIAN_POINT('Ctrl Pts',(134.070271860316,-35.346571757529,20.3477422418597));
#21384=CARTESIAN_POINT('Ctrl Pts',(134.067594084757,-35.3780205824025,20.3461971026219));
#21385=CARTESIAN_POINT('Ctrl Pts',(134.064552893826,-35.4094255905554,20.3446519633841));
#21386=CARTESIAN_POINT('Ctrl Pts',(134.061150073727,-35.4407778109978,20.3431068241463));
#21387=CARTESIAN_POINT('Ctrl Pts',(134.048324924255,-35.5589435975309,20.3372832304498));
#21388=CARTESIAN_POINT('Ctrl Pts',(134.030317473101,-35.6767397176403,20.3314596367534));
#21389=CARTESIAN_POINT('Ctrl Pts',(134.007156478494,-35.7936762292395,20.3256360430569));
#21390=CARTESIAN_POINT('Ctrl Pts',(133.984024704926,-35.9104652080444,20.3198197966897));
#21391=CARTESIAN_POINT('Ctrl Pts',(133.955752398789,-36.0263963384068,20.3140035503225));
#21392=CARTESIAN_POINT('Ctrl Pts',(133.922420097489,-36.1409844779025,20.3081873039553));
#21393=CARTESIAN_POINT('Ctrl Pts',(133.889121162011,-36.2554579140226,20.3023768796835));
#21394=CARTESIAN_POINT('Ctrl Pts',(133.850772421123,-36.368590643845,20.2965664554118));
#21395=CARTESIAN_POINT('Ctrl Pts',(133.807505391999,-36.479908000485,20.2907560311401));
#21396=CARTESIAN_POINT('Ctrl Pts',(133.762600616579,-36.595438948679,20.284725670325));
#21397=CARTESIAN_POINT('Ctrl Pts',(133.712397948556,-36.7090139373482,20.2786953095099));
#21398=CARTESIAN_POINT('Ctrl Pts',(133.657101307584,-36.820119508732,20.2726649486948));
#21399=CARTESIAN_POINT('Ctrl Pts',(133.603881390285,-36.9270523931991,20.2668610644404));
#21400=CARTESIAN_POINT('Ctrl Pts',(133.545943417351,-37.0316976001409,20.2610571801859));
#21401=CARTESIAN_POINT('Ctrl Pts',(133.483517821578,-37.1336186601058,20.2552532959315));
#21402=CARTESIAN_POINT('Ctrl Pts',(133.421101446741,-37.2355246652257,20.2494502689736));
#21403=CARTESIAN_POINT('Ctrl Pts',(133.354198980525,-37.3347069754688,20.2436472420158));
#21404=CARTESIAN_POINT('Ctrl Pts',(133.283085686113,-37.4307557215072,20.237844215058));
#21405=CARTESIAN_POINT('Ctrl Pts',(133.211966113151,-37.5268129476313,20.2320406757544));
#21406=CARTESIAN_POINT('Ctrl Pts',(133.136635215813,-37.6197357312892,20.2262371364508));
#21407=CARTESIAN_POINT('Ctrl Pts',(133.057409873698,-37.7091455967172,20.2204335971472));
#21408=CARTESIAN_POINT('Ctrl Pts',(132.978158839741,-37.7985844567084,20.2146281758244));
#21409=CARTESIAN_POINT('Ctrl Pts',(132.895011120008,-37.8845078274006,20.2088227545015));
#21410=CARTESIAN_POINT('Ctrl Pts',(132.808321473052,-37.9665730235404,20.2030173331787));
#21411=CARTESIAN_POINT('Ctrl Pts',(132.721535825356,-38.0487290992693,20.1972054828905));
#21412=CARTESIAN_POINT('Ctrl Pts',(132.631200717793,-38.1270181911431,20.1913936326023));
#21413=CARTESIAN_POINT('Ctrl Pts',(132.537705221933,-38.2011368615813,20.1855817823141));
#21414=CARTESIAN_POINT('Ctrl Pts',(132.444148317742,-38.2753042135501,20.1797661147722));
#21415=CARTESIAN_POINT('Ctrl Pts',(132.347427221373,-38.3452954501526,20.1739504472303));
#21416=CARTESIAN_POINT('Ctrl Pts',(132.247959924876,-38.4108505062744,20.1681347796885));
#21417=CARTESIAN_POINT('Ctrl Pts',(132.148350152239,-38.4764994629209,20.1623107818321));
#21418=CARTESIAN_POINT('Ctrl Pts',(132.045986677384,-38.5376993473583,20.1564867839757));
#21419=CARTESIAN_POINT('Ctrl Pts',(131.941312109039,-38.5942359821383,20.1506627861194));
#21420=CARTESIAN_POINT('Ctrl Pts',(131.913541379025,-38.6092354576102,20.1491176479389));
#21421=CARTESIAN_POINT('Ctrl Pts',(131.885608085202,-38.6239069646692,20.1475725097584));
#21422=CARTESIAN_POINT('Ctrl Pts',(131.857520709763,-38.6382470796802,20.1460273715779));
#21423=CARTESIAN_POINT('Ctrl Pts',(131.751659969621,-38.6922946781139,20.1402037775663));
#21424=CARTESIAN_POINT('Ctrl Pts',(131.643267658643,-38.7418053106816,20.1343801835548));
#21425=CARTESIAN_POINT('Ctrl Pts',(131.53276931453,-38.7865344615405,20.1285565895432));
#21426=CARTESIAN_POINT('Ctrl Pts',(131.422410380457,-38.8312071799459,20.1227403428587));
#21427=CARTESIAN_POINT('Ctrl Pts',(131.309951073269,-38.8711102633735,20.1169240961742));
#21428=CARTESIAN_POINT('Ctrl Pts',(131.19584129982,-38.9060451335903,20.1111078494896));
#21429=CARTESIAN_POINT('Ctrl Pts',(131.081845750858,-38.9409450338173,20.1052974248988));
#21430=CARTESIAN_POINT('Ctrl Pts',(130.966203410539,-38.9708864955649,20.0994870003079));
#21431=CARTESIAN_POINT('Ctrl Pts',(130.849383369527,-38.9957193209197,20.093676575717));
#21432=CARTESIAN_POINT('Ctrl Pts',(130.728141458058,-39.0214921180109,20.0876462150209));
#21433=CARTESIAN_POINT('Ctrl Pts',(130.60563134316,-39.0417617250352,20.0816158543247));
#21434=CARTESIAN_POINT('Ctrl Pts',(130.482394247349,-39.056417235705,20.0755854936286));
#21435=CARTESIAN_POINT('Ctrl Pts',(130.363785441738,-39.0705223442743,20.0697816090525));
#21436=CARTESIAN_POINT('Ctrl Pts',(130.244503717389,-39.0794273851999,20.0639777244764));
#21437=CARTESIAN_POINT('Ctrl Pts',(130.12504043967,-39.0830858291796,20.0581738399004));
#21438=CARTESIAN_POINT('Ctrl Pts',(130.005594807964,-39.0867437327677,20.0523708126206));
#21439=CARTESIAN_POINT('Ctrl Pts',(129.885968084255,-39.0851565681025,20.0465677853408));
#21440=CARTESIAN_POINT('Ctrl Pts',(129.766653960719,-39.0783298819433,20.040764758061));
#21441=CARTESIAN_POINT('Ctrl Pts',(129.647329303011,-39.0715025930602,20.0349612184354));
#21442=CARTESIAN_POINT('Ctrl Pts',(129.528317708041,-39.0594348862607,20.0291576788098));
#21443=CARTESIAN_POINT('Ctrl Pts',(129.410109423915,-39.0421843238831,20.0233541391843));
#21444=CARTESIAN_POINT('Ctrl Pts',(129.291862806249,-39.0249281673533,20.0175487175398));
#21445=CARTESIAN_POINT('Ctrl Pts',(129.174420421361,-39.0024858715713,20.0117432958954));
#21446=CARTESIAN_POINT('Ctrl Pts',(129.05826334707,-38.9749662987915,20.005937874251));
#21447=CARTESIAN_POINT('Ctrl Pts',(128.941977639649,-38.9474162506505,20.0001260236433));
#21448=CARTESIAN_POINT('Ctrl Pts',(128.82698048155,-38.9147777964909,19.9943141730357));
#21449=CARTESIAN_POINT('Ctrl Pts',(128.713738934119,-38.8772100111288,19.988502322428));
#21450=CARTESIAN_POINT('Ctrl Pts',(128.600423009067,-38.8396175510559,19.9826866545676));
#21451=CARTESIAN_POINT('Ctrl Pts',(128.488865371773,-38.7970894571204,19.9768709867071));
#21452=CARTESIAN_POINT('Ctrl Pts',(128.379512661255,-38.7498327676002,19.9710553188467));
#21453=CARTESIAN_POINT('Ctrl Pts',(128.270003314891,-38.7025083880196,19.9652313206755));
#21454=CARTESIAN_POINT('Ctrl Pts',(128.162705565199,-38.6504420715526,19.9594073225043));
#21455=CARTESIAN_POINT('Ctrl Pts',(128.058041166046,-38.5938865991053,19.9535833243331));
#21456=CARTESIAN_POINT('Ctrl Pts',(128.030273190693,-38.5788821565466,19.9520381892252));
#21457=CARTESIAN_POINT('Ctrl Pts',(128.002690406367,-38.5635619712292,19.9504930541173));
#21458=CARTESIAN_POINT('Ctrl Pts',(127.97530032608,-38.5479312606687,19.9489479190094));
#21459=CARTESIAN_POINT('Ctrl Pts',(127.872067493333,-38.489019329336,19.943124326216));
#21460=CARTESIAN_POINT('Ctrl Pts',(127.771241531577,-38.4255030674034,19.9373007334226));
#21461=CARTESIAN_POINT('Ctrl Pts',(127.673260210972,-38.3576043474708,19.9314771406292));
#21462=CARTESIAN_POINT('Ctrl Pts',(127.575402508372,-38.2897912918693,19.9256608951641));
#21463=CARTESIAN_POINT('Ctrl Pts',(127.480382641277,-38.2176070060932,19.9198446496989));
#21464=CARTESIAN_POINT('Ctrl Pts',(127.388613317249,-38.1413189257303,19.9140284042337));
#21465=CARTESIAN_POINT('Ctrl Pts',(127.296935854815,-38.0651072101519,19.908217980862));
#21466=CARTESIAN_POINT('Ctrl Pts',(127.208502774595,-37.9848001317203,19.9024075574903));
#21467=CARTESIAN_POINT('Ctrl Pts',(127.123696836121,-37.9007076911436,19.8965971341186));
#21468=CARTESIAN_POINT('Ctrl Pts',(127.035680799385,-37.8134321598283,19.8905667729653));
#21469=CARTESIAN_POINT('Ctrl Pts',(126.951572289504,-37.7220792902935,19.8845364118121));
#21470=CARTESIAN_POINT('Ctrl Pts',(126.871760744005,-37.6270409508138,19.8785060506589));
#21471=CARTESIAN_POINT('Ctrl Pts',(126.794946621351,-37.5355718955536,19.8727021672936));
#21472=CARTESIAN_POINT('Ctrl Pts',(126.722112814015,-37.4406895438645,19.8668982839284));
#21473=CARTESIAN_POINT('Ctrl Pts',(126.653567586273,-37.3427793537506,19.8610944005632));
#21474=CARTESIAN_POINT('Ctrl Pts',(126.585032483341,-37.2448836259423,19.8552913744891));
#21475=CARTESIAN_POINT('Ctrl Pts',(126.520784934362,-37.1439612835512,19.849488348415));
#21476=CARTESIAN_POINT('Ctrl Pts',(126.461090924169,-37.0404282768574,19.8436853223409));
#21477=CARTESIAN_POINT('Ctrl Pts',(126.40139164356,-36.9368861291808,19.8378817839146));
#21478=CARTESIAN_POINT('Ctrl Pts',(126.346246905051,-36.8307332126852,19.8320782454883));
#21479=CARTESIAN_POINT('Ctrl Pts',(126.29587730123,-36.7224111101761,19.826274707062));
#21480=CARTESIAN_POINT('Ctrl Pts',(126.245491363076,-36.6140538799459,19.8204692866091));
#21481=CARTESIAN_POINT('Ctrl Pts',(126.199883811363,-36.5035264347844,19.8146638661562));
#21482=CARTESIAN_POINT('Ctrl Pts',(126.159227306094,-36.3912908084738,19.8088584457033));
#21483=CARTESIAN_POINT('Ctrl Pts',(126.118525777404,-36.2789308913088,19.8030465962698));
#21484=CARTESIAN_POINT('Ctrl Pts',(126.082786378527,-36.1648594012373,19.7972347468362));
#21485=CARTESIAN_POINT('Ctrl Pts',(126.052132089805,-36.0495541737595,19.7914228974027));
#21486=CARTESIAN_POINT('Ctrl Pts',(126.021457667142,-35.9341732130374,19.7856072307076));
#21487=CARTESIAN_POINT('Ctrl Pts',(125.995875093492,-35.8175572990579,19.7797915640125));
#21488=CARTESIAN_POINT('Ctrl Pts',(125.975456039167,-35.7001934784911,19.7739758973174));
#21489=CARTESIAN_POINT('Ctrl Pts',(125.955007736688,-35.5826615465633,19.7681519002899));
#21490=CARTESIAN_POINT('Ctrl Pts',(125.939737768042,-35.464379973335,19.7623279032623));
#21491=CARTESIAN_POINT('Ctrl Pts',(125.929665904588,-35.345840066687,19.7565039062348));
#21492=CARTESIAN_POINT('Ctrl Pts',(125.926993769716,-35.3143906115087,19.7549587596368));
#21493=CARTESIAN_POINT('Ctrl Pts',(125.92468723338,-35.2829229658023,19.7534136130389));
#21494=CARTESIAN_POINT('Ctrl Pts',(125.922746050153,-35.2514462734928,19.751868466441));
#21495=CARTESIAN_POINT('Ctrl Pts',(125.917614677707,-35.1682399953501,19.7477839871591));
#21496=CARTESIAN_POINT('Ctrl Pts',(125.91503008981,-35.0848750595345,19.7436995078773));
#21497=CARTESIAN_POINT('Ctrl Pts',(125.915000261185,-35.0014607801979,19.7396150285955));
#21498=CARTESIAN_POINT('Origin',(130.,-35.,32.7603849714045));
#21499=CARTESIAN_POINT('',(132.487160670875,-31.7594357285724,21.7969524316048));
#21500=CARTESIAN_POINT('',(132.487160670875,-31.7594357285724,21.6925409193069));
#21501=CARTESIAN_POINT('',(132.487160670875,-31.7594357285724,32.7603849714045));
#21502=CARTESIAN_POINT('',(125.915001474033,-35.0034702810671,20.8853849714288));
#21503=CARTESIAN_POINT('Ctrl Pts',(132.487160670875,-31.7594357285724,21.6925409193069));
#21504=CARTESIAN_POINT('Ctrl Pts',(132.581750072248,-31.8320338995304,21.686731190181));
#21505=CARTESIAN_POINT('Ctrl Pts',(132.673252096067,-31.9088490454524,21.6809214610551));
#21506=CARTESIAN_POINT('Ctrl Pts',(132.7612728889,-31.9895852390367,21.6751117319293));
#21507=CARTESIAN_POINT('Ctrl Pts',(132.851093333724,-32.0719721454453,21.669183218477));
#21508=CARTESIAN_POINT('Ctrl Pts',(132.937288272235,-32.1584419595542,21.6632547050247));
#21509=CARTESIAN_POINT('Ctrl Pts',(133.019473900383,-32.2486362717907,21.6573261915724));
#21510=CARTESIAN_POINT('Ctrl Pts',(133.099929339428,-32.3369317944248,21.6515224864303));
#21511=CARTESIAN_POINT('Ctrl Pts',(133.176542332567,-32.4287962210242,21.6457187812882));
#21512=CARTESIAN_POINT('Ctrl Pts',(133.248990082593,-32.5238561343873,21.6399150761461));
#21513=CARTESIAN_POINT('Ctrl Pts',(133.321429231274,-32.6189047617812,21.6341120600478));
#21514=CARTESIAN_POINT('Ctrl Pts',(133.389703872855,-32.7171477967207,21.6283090439495));
#21515=CARTESIAN_POINT('Ctrl Pts',(133.453532313997,-32.8181797608012,21.6225060278511));
#21516=CARTESIAN_POINT('Ctrl Pts',(133.517368240634,-32.9192235734274,21.6167023312028));
#21517=CARTESIAN_POINT('Ctrl Pts',(133.576756711935,-33.0230566203116,21.6108986345545));
#21518=CARTESIAN_POINT('Ctrl Pts',(133.631460429976,-33.1292461023645,21.6050949379061));
#21519=CARTESIAN_POINT('Ctrl Pts',(133.688224574743,-33.2394352329726,21.5990726438368));
#21520=CARTESIAN_POINT('Ctrl Pts',(133.739943902747,-33.3521613770866,21.5930503497675));
#21521=CARTESIAN_POINT('Ctrl Pts',(133.786407175595,-33.4669162773674,21.5870280556982));
#21522=CARTESIAN_POINT('Ctrl Pts',(133.831250903433,-33.5776712285531,21.5812156774551));
#21523=CARTESIAN_POINT('Ctrl Pts',(133.871198788336,-33.6903154573991,21.5754032992121));
#21524=CARTESIAN_POINT('Ctrl Pts',(133.906111585419,-33.8043757771527,21.569590920969));
#21525=CARTESIAN_POINT('Ctrl Pts',(133.941048496566,-33.9185148777014,21.5637745281504));
#21526=CARTESIAN_POINT('Ctrl Pts',(133.970943292541,-34.0340716227221,21.5579581353317));
#21527=CARTESIAN_POINT('Ctrl Pts',(133.995707688656,-34.1505619111331,21.552141742513));
#21528=CARTESIAN_POINT('Ctrl Pts',(134.020506523705,-34.2672141983023,21.5463172610509));
#21529=CARTESIAN_POINT('Ctrl Pts',(134.040160655904,-34.3848022184481,21.5404927795887));
#21530=CARTESIAN_POINT('Ctrl Pts',(134.054633516296,-34.502835994338,21.5346682981265));
#21531=CARTESIAN_POINT('Ctrl Pts',(134.056158283232,-34.5152712693208,21.5340546684424));
#21532=CARTESIAN_POINT('Ctrl Pts',(134.05762558901,-34.5277114917279,21.5334410387583));
#21533=CARTESIAN_POINT('Ctrl Pts',(134.059035424522,-34.540156089013,21.5328274090742));
#21534=CARTESIAN_POINT('Ctrl Pts',(134.072415333228,-34.6582603459497,21.5270038154121));
#21535=CARTESIAN_POINT('Ctrl Pts',(134.080657885567,-34.7771395049127,21.52118022175));
#21536=CARTESIAN_POINT('Ctrl Pts',(134.083683781112,-34.896309229528,21.515356628088));
#21537=CARTESIAN_POINT('Ctrl Pts',(134.086705859041,-35.0153286038346,21.5095403817543));
#21538=CARTESIAN_POINT('Ctrl Pts',(134.084524360526,-35.134637410044,21.5037241354207));
#21539=CARTESIAN_POINT('Ctrl Pts',(134.077111557626,-35.2537446485602,21.497907889087));
#21540=CARTESIAN_POINT('Ctrl Pts',(134.069706174982,-35.3727326600739,21.492097464848));
#21541=CARTESIAN_POINT('Ctrl Pts',(134.057079930669,-35.4915191000857,21.486287040609));
#21542=CARTESIAN_POINT('Ctrl Pts',(134.039257132993,-35.6096120188813,21.48047661637));
#21543=CARTESIAN_POINT('Ctrl Pts',(134.020759705521,-35.7321749991799,21.4744462555423));
#21544=CARTESIAN_POINT('Ctrl Pts',(133.996664539723,-35.8539904703923,21.4684158947146));
#21545=CARTESIAN_POINT('Ctrl Pts',(133.967058086598,-35.9745127693146,21.462385533887));
#21546=CARTESIAN_POINT('Ctrl Pts',(133.938563535254,-36.0905087253357,21.4565816496629));
#21547=CARTESIAN_POINT('Ctrl Pts',(133.904964301935,-36.2053064581143,21.4507777654389));
#21548=CARTESIAN_POINT('Ctrl Pts',(133.866389576652,-36.3184296119088,21.4449738812149));
#21549=CARTESIAN_POINT('Ctrl Pts',(133.827820549268,-36.431536056205,21.4391708542865));
#21550=CARTESIAN_POINT('Ctrl Pts',(133.784277623227,-36.5429680270441,21.4333678273582));
#21551=CARTESIAN_POINT('Ctrl Pts',(133.735939558198,-36.652265298761,21.4275648004299));
#21552=CARTESIAN_POINT('Ctrl Pts',(133.687597225423,-36.7615722202854,21.4217612611549));
#21553=CARTESIAN_POINT('Ctrl Pts',(133.634459077087,-36.8687436944971,21.4159577218799));
#21554=CARTESIAN_POINT('Ctrl Pts',(133.576751357031,-36.9733410070182,21.4101541826049));
#21555=CARTESIAN_POINT('Ctrl Pts',(133.519024923033,-37.0779722392296,21.4043487613097));
#21556=CARTESIAN_POINT('Ctrl Pts',(133.456726167387,-37.1800272922317,21.3985433400145));
#21557=CARTESIAN_POINT('Ctrl Pts',(133.390126134966,-37.2790940719986,21.3927379187193));
#21558=CARTESIAN_POINT('Ctrl Pts',(133.323452349172,-37.3782705590576,21.3869260684572));
#21559=CARTESIAN_POINT('Ctrl Pts',(133.25246800667,-37.4744518282846,21.3811142181951));
#21560=CARTESIAN_POINT('Ctrl Pts',(133.177486231656,-37.5672565605406,21.375302367933));
#21561=CARTESIAN_POINT('Ctrl Pts',(133.102455208208,-37.6601222474446,21.3694867004164));
#21562=CARTESIAN_POINT('Ctrl Pts',(133.023421793118,-37.749606675364,21.3636710328997));
#21563=CARTESIAN_POINT('Ctrl Pts',(132.94073683228,-37.8353645062447,21.3578553653831));
#21564=CARTESIAN_POINT('Ctrl Pts',(132.857933434161,-37.9212451759609,21.3520313675505));
#21565=CARTESIAN_POINT('Ctrl Pts',(132.771468345601,-38.0033883141385,21.3462073697179));
#21566=CARTESIAN_POINT('Ctrl Pts',(132.681726486139,-38.0814879609596,21.3403833718853));
#21567=CARTESIAN_POINT('Ctrl Pts',(132.657917480281,-38.102208224166,21.3388382334254));
#21568=CARTESIAN_POINT('Ctrl Pts',(132.633877994583,-38.1226441118969,21.3372930949656));
#21569=CARTESIAN_POINT('Ctrl Pts',(132.609615554879,-38.1427904250415,21.3357479565057));
#21570=CARTESIAN_POINT('Ctrl Pts',(132.51817094072,-38.2187214466004,21.3299243628355));
#21571=CARTESIAN_POINT('Ctrl Pts',(132.423262109218,-38.2907805045869,21.3241007691653));
#21572=CARTESIAN_POINT('Ctrl Pts',(132.325250675735,-38.3586357788534,21.3182771754951));
#21573=CARTESIAN_POINT('Ctrl Pts',(132.227362898235,-38.4264054436113,21.3124609291534));
#21574=CARTESIAN_POINT('Ctrl Pts',(132.126380637163,-38.4899816431958,21.3066446828117));
#21575=CARTESIAN_POINT('Ctrl Pts',(132.022699350964,-38.5490720386617,21.30082843647));
#21576=CARTESIAN_POINT('Ctrl Pts',(131.919121850306,-38.6081032843147,21.2950180122231));
#21577=CARTESIAN_POINT('Ctrl Pts',(131.812851052025,-38.662657457747,21.2892075879762));
#21578=CARTESIAN_POINT('Ctrl Pts',(131.704311733594,-38.7124852208099,21.2833971637292));
#21579=CARTESIAN_POINT('Ctrl Pts',(131.591663977427,-38.7641990677833,21.2773668029046));
#21580=CARTESIAN_POINT('Ctrl Pts',(131.476572940032,-38.810821370695,21.2713364420799));
#21581=CARTESIAN_POINT('Ctrl Pts',(131.359542387655,-38.852125321971,21.2653060812552));
#21582=CARTESIAN_POINT('Ctrl Pts',(131.246907041727,-38.8918780595738,21.2595021970237));
#21583=CARTESIAN_POINT('Ctrl Pts',(131.13247565441,-38.9267045661159,21.2536983127921));
#21584=CARTESIAN_POINT('Ctrl Pts',(131.016717453162,-38.9564517715292,21.2478944285605));
#21585=CARTESIAN_POINT('Ctrl Pts',(130.90097635064,-38.9861945829617,21.2420914016247));
#21586=CARTESIAN_POINT('Ctrl Pts',(130.783909219319,-39.010859483706,21.236288374689));
#21587=CARTESIAN_POINT('Ctrl Pts',(130.665998968207,-39.030343704245,21.2304853477532));
#21588=CARTESIAN_POINT('Ctrl Pts',(130.548078306854,-39.0498296450367,21.2246818084709));
#21589=CARTESIAN_POINT('Ctrl Pts',(130.429314780602,-39.0641339296251,21.2188782691887));
#21590=CARTESIAN_POINT('Ctrl Pts',(130.310199336132,-39.0732052945884,21.2130747299064));
#21591=CARTESIAN_POINT('Ctrl Pts',(130.191045263914,-39.0822796012895,21.2072693086041));
#21592=CARTESIAN_POINT('Ctrl Pts',(130.071539453462,-39.0861175824741,21.2014638873018));
#21593=CARTESIAN_POINT('Ctrl Pts',(129.952175145256,-39.0847200373182,21.1956584659995));
#21594=CARTESIAN_POINT('Ctrl Pts',(129.832678652129,-39.0833209445104,21.1898466157305));
#21595=CARTESIAN_POINT('Ctrl Pts',(129.713324382588,-39.0766747571188,21.1840347654616));
#21596=CARTESIAN_POINT('Ctrl Pts',(129.594602904237,-39.0648343379217,21.1782229151926));
#21597=CARTESIAN_POINT('Ctrl Pts',(129.475803448983,-39.0529861418737,21.1724072476693));
#21598=CARTESIAN_POINT('Ctrl Pts',(129.357638015862,-39.035936977912,21.1665915801459));
#21599=CARTESIAN_POINT('Ctrl Pts',(129.240587756598,-39.0137909816745,21.1607759126225));
#21600=CARTESIAN_POINT('Ctrl Pts',(129.123369835479,-38.9916132636891,21.1549519147835));
#21601=CARTESIAN_POINT('Ctrl Pts',(129.007270672566,-38.9643242348053,21.1491279169445));
#21602=CARTESIAN_POINT('Ctrl Pts',(128.892757162696,-38.9320781145903,21.1433039191054));
#21603=CARTESIAN_POINT('Ctrl Pts',(128.862376103999,-38.9235230430346,21.141758780716));
#21604=CARTESIAN_POINT('Ctrl Pts',(128.83210654808,-38.9146193205452,21.1402136423267));
#21605=CARTESIAN_POINT('Ctrl Pts',(128.801956968712,-38.9053703915485,21.1386685039373));
#21606=CARTESIAN_POINT('Ctrl Pts',(128.688323845553,-38.8705113749443,21.1328449102228));
#21607=CARTESIAN_POINT('Ctrl Pts',(128.576030163275,-38.830632517438,21.1270213165083));
#21608=CARTESIAN_POINT('Ctrl Pts',(128.465551671052,-38.7858543719732,21.1211977227938));
#21609=CARTESIAN_POINT('Ctrl Pts',(128.355212563853,-38.7411327207887,21.1153814764076));
#21610=CARTESIAN_POINT('Ctrl Pts',(128.246684466789,-38.6915242278978,21.1095652300214));
#21611=CARTESIAN_POINT('Ctrl Pts',(128.14042865964,-38.6371993937798,21.1037489836352));
#21612=CARTESIAN_POINT('Ctrl Pts',(128.034279215138,-38.5829289391193,21.0979385593436));
#21613=CARTESIAN_POINT('Ctrl Pts',(127.930397897051,-38.5239517200571,21.092128135052));
#21614=CARTESIAN_POINT('Ctrl Pts',(127.829226092157,-38.4604863301319,21.0863177107604));
#21615=CARTESIAN_POINT('Ctrl Pts',(127.724224726253,-38.3946186445961,21.0802873499524));
#21616=CARTESIAN_POINT('Ctrl Pts',(127.622142463111,-38.3239164701803,21.0742569891444));
#21617=CARTESIAN_POINT('Ctrl Pts',(127.523445144338,-38.2486768147812,21.0682266283365));
#21618=CARTESIAN_POINT('Ctrl Pts',(127.428454506996,-38.1762628636363,21.06242274406));
#21619=CARTESIAN_POINT('Ctrl Pts',(127.336599502754,-38.0996463748078,21.0566188597836));
#21620=CARTESIAN_POINT('Ctrl Pts',(127.248265368406,-38.0191358891715,21.0508149755071));
#21621=CARTESIAN_POINT('Ctrl Pts',(127.159944281955,-37.9386372957963,21.0450119485266));
#21622=CARTESIAN_POINT('Ctrl Pts',(127.075143332853,-37.854246124464,21.039208921546));
#21623=CARTESIAN_POINT('Ctrl Pts',(126.994213187693,-37.7663099318341,21.0334058945654));
#21624=CARTESIAN_POINT('Ctrl Pts',(126.91327589725,-37.6783659753601,21.0276023552384));
#21625=CARTESIAN_POINT('Ctrl Pts',(126.836210366766,-37.5868766757659,21.0217988159114));
#21626=CARTESIAN_POINT('Ctrl Pts',(126.763328590582,-37.4922245459543,21.0159952765844));
#21627=CARTESIAN_POINT('Ctrl Pts',(126.69042317969,-37.3975417215643,21.0101898552374));
#21628=CARTESIAN_POINT('Ctrl Pts',(126.621704470347,-37.2996943505045,21.0043844338905));
#21629=CARTESIAN_POINT('Ctrl Pts',(126.557442170616,-37.1990954029655,20.9985790125435));
#21630=CARTESIAN_POINT('Ctrl Pts',(126.493108706341,-37.0983850514128,20.9927671622303));
#21631=CARTESIAN_POINT('Ctrl Pts',(126.433241722433,-36.9949173853986,20.9869553119172));
#21632=CARTESIAN_POINT('Ctrl Pts',(126.378065917287,-36.8891316789677,20.981143461604));
#21633=CARTESIAN_POINT('Ctrl Pts',(126.322853872378,-36.7832764919218,20.9753277940366));
#21634=CARTESIAN_POINT('Ctrl Pts',(126.272339314874,-36.6751006014944,20.9695121264692));
#21635=CARTESIAN_POINT('Ctrl Pts',(126.226698898587,-36.5650635124743,20.9636964589018));
#21636=CARTESIAN_POINT('Ctrl Pts',(126.180993107338,-36.4548688072199,20.9578724610193));
#21637=CARTESIAN_POINT('Ctrl Pts',(126.140175531616,-36.3428079645657,20.9520484631368));
#21638=CARTESIAN_POINT('Ctrl Pts',(126.104373121373,-36.2293560194356,20.9462244652543));
#21639=CARTESIAN_POINT('Ctrl Pts',(126.094874549378,-36.1992566082064,20.9446793272925));
#21640=CARTESIAN_POINT('Ctrl Pts',(126.08572870053,-36.1690593369959,20.9431341893307));
#21641=CARTESIAN_POINT('Ctrl Pts',(126.076937339023,-36.1387731811246,20.9415890513689));
#21642=CARTESIAN_POINT('Ctrl Pts',(126.035980316619,-35.997676632698,20.9343905929649));
#21643=CARTESIAN_POINT('Ctrl Pts',(126.002614949914,-35.8542850934519,20.927192134561));
#21644=CARTESIAN_POINT('Ctrl Pts',(125.977056286364,-35.7093298787686,20.919993676157));
#21645=CARTESIAN_POINT('Ctrl Pts',(125.951848625687,-35.5663653666423,20.9128940758009));
#21646=CARTESIAN_POINT('Ctrl Pts',(125.934234725755,-35.4218797790436,20.9057944754448));
#21647=CARTESIAN_POINT('Ctrl Pts',(125.924374885708,-35.2765952417385,20.8986948750887));
#21648=CARTESIAN_POINT('Ctrl Pts',(125.918213340713,-35.185805004833,20.8942582405354));
#21649=CARTESIAN_POINT('Ctrl Pts',(125.915078978048,-35.0947031752966,20.8898216059821));
#21650=CARTESIAN_POINT('Ctrl Pts',(125.915001474033,-35.0034702810671,20.8853849714288));
#21651=CARTESIAN_POINT('Ctrl Pts',(125.915001474033,-35.003470280567,20.8853849714045));
#21652=CARTESIAN_POINT('Ctrl Pts',(125.914898933796,-34.8827662892301,20.8795151642127));
#21653=CARTESIAN_POINT('Ctrl Pts',(125.920150846961,-34.7619569650232,20.8736453570208));
#21654=CARTESIAN_POINT('Ctrl Pts',(125.930756371625,-34.6415571273887,20.867775549829));
#21655=CARTESIAN_POINT('Ctrl Pts',(125.941161880961,-34.5234279754281,20.8620164445065));
#21656=CARTESIAN_POINT('Ctrl Pts',(125.956720796162,-34.4056934311284,20.8562573391841));
#21657=CARTESIAN_POINT('Ctrl Pts',(125.977379782769,-34.2888378610145,20.8504982338616));
#21658=CARTESIAN_POINT('Ctrl Pts',(125.998035648516,-34.1719999437465,20.8447399985413));
#21659=CARTESIAN_POINT('Ctrl Pts',(126.023789981672,-34.0560411455548,20.838981763221));
#21660=CARTESIAN_POINT('Ctrl Pts',(126.054537987098,-33.9414375291237,20.8332235279008));
#21661=CARTESIAN_POINT('Ctrl Pts',(126.085288892143,-33.8268231052669,20.8274647495636));
#21662=CARTESIAN_POINT('Ctrl Pts',(126.121034297585,-33.7135645182732,20.8217059712264));
#21663=CARTESIAN_POINT('Ctrl Pts',(126.161619205863,-33.6021237968987,20.8159471928892));
#21664=CARTESIAN_POINT('Ctrl Pts',(126.203573824735,-33.4869220337182,20.8099940600485));
#21665=CARTESIAN_POINT('Ctrl Pts',(126.250700225609,-33.3736634602182,20.8040409272077));
#21666=CARTESIAN_POINT('Ctrl Pts',(126.302773206644,-33.2628359206759,20.798087794367));
#21667=CARTESIAN_POINT('Ctrl Pts',(126.353220680837,-33.1554679665127,20.7923204941399));
#21668=CARTESIAN_POINT('Ctrl Pts',(126.408310257633,-33.0503818750327,20.7865531939128));
#21669=CARTESIAN_POINT('Ctrl Pts',(126.467791010027,-32.9479949680485,20.7807858936857));
#21670=CARTESIAN_POINT('Ctrl Pts',(126.530146624985,-32.8406594302205,20.7747398445382));
#21671=CARTESIAN_POINT('Ctrl Pts',(126.597328220364,-32.7362909643389,20.7686937953906));
#21672=CARTESIAN_POINT('Ctrl Pts',(126.668997397386,-32.6353337103565,20.7626477462431));
#21673=CARTESIAN_POINT('Ctrl Pts',(126.740666574408,-32.534376456374,20.7566016970955));
#21674=CARTESIAN_POINT('Ctrl Pts',(126.816822954776,-32.43683077537,20.750555647948));
#21675=CARTESIAN_POINT('Ctrl Pts',(126.897082912047,-32.3430975657186,20.7445095988004));
#21676=CARTESIAN_POINT('Ctrl Pts',(126.9743898227,-32.2528131311135,20.7386860051039));
#21677=CARTESIAN_POINT('Ctrl Pts',(127.055765126528,-32.1657599626625,20.7328624114074));
#21678=CARTESIAN_POINT('Ctrl Pts',(127.140908444355,-32.0823261874503,20.7270388177108));
#21679=CARTESIAN_POINT('Ctrl Pts',(127.225944341228,-31.9989976763494,20.7212225713435));
#21680=CARTESIAN_POINT('Ctrl Pts',(127.314738507605,-31.9192797592956,20.7154063249762));
#21681=CARTESIAN_POINT('Ctrl Pts',(127.406950539366,-31.8435273651268,20.7095900786089));
#21682=CARTESIAN_POINT('Ctrl Pts',(127.49907026636,-31.767850799533,20.7037796543371));
#21683=CARTESIAN_POINT('Ctrl Pts',(127.594600738773,-31.6961321176856,20.6979692300653));
#21684=CARTESIAN_POINT('Ctrl Pts',(127.693165392179,-31.6286888170687,20.6921588057936));
#21685=CARTESIAN_POINT('Ctrl Pts',(127.795460921015,-31.5586926484149,20.6861284449785));
#21686=CARTESIAN_POINT('Ctrl Pts',(127.901024549233,-31.4933022337859,20.6800980841634));
#21687=CARTESIAN_POINT('Ctrl Pts',(128.009398053128,-31.4328262042469,20.6740677233484));
#21688=CARTESIAN_POINT('Ctrl Pts',(128.113701475784,-31.3746214157803,20.6682638390938));
#21689=CARTESIAN_POINT('Ctrl Pts',(128.220607135908,-31.3209687562226,20.6624599548393));
#21690=CARTESIAN_POINT('Ctrl Pts',(128.329678398803,-31.2720983451041,20.6566560705848));
#21691=CARTESIAN_POINT('Ctrl Pts',(128.438733550691,-31.2232351526749,20.6508530436268));
#21692=CARTESIAN_POINT('Ctrl Pts',(128.549953296664,-31.1791529708189,20.6450500166689));
#21693=CARTESIAN_POINT('Ctrl Pts',(128.662879021698,-31.1400346517897,20.639246989711));
#21694=CARTESIAN_POINT('Ctrl Pts',(128.775814716876,-31.1009128790277,20.6334434504073));
#21695=CARTESIAN_POINT('Ctrl Pts',(128.890456304722,-31.0667559741176,20.6276399111036));
#21696=CARTESIAN_POINT('Ctrl Pts',(129.006328549081,-31.0376973806095,20.6218363717999));
#21697=CARTESIAN_POINT('Ctrl Pts',(129.12223836944,-31.0086293637427,20.616030950477));
#21698=CARTESIAN_POINT('Ctrl Pts',(129.239379244138,-30.9846630456388,20.6102255291541));
#21699=CARTESIAN_POINT('Ctrl Pts',(129.357264883258,-30.9658809425469,20.6044201078312));
#21700=CARTESIAN_POINT('Ctrl Pts',(129.475281069784,-30.9470780400187,20.5986082575429));
#21701=CARTESIAN_POINT('Ctrl Pts',(129.594043263529,-30.9334708763901,20.5927964072546));
#21702=CARTESIAN_POINT('Ctrl Pts',(129.713059015976,-30.9250902007913,20.5869845569663));
#21703=CARTESIAN_POINT('Ctrl Pts',(129.832152938592,-30.9167040207209,20.5811688894243));
#21704=CARTESIAN_POINT('Ctrl Pts',(129.95150034432,-30.9135511759163,20.5753532218823));
#21705=CARTESIAN_POINT('Ctrl Pts',(130.070609405729,-30.9156102889388,20.5695375543403));
#21706=CARTESIAN_POINT('Ctrl Pts',(130.18988907798,-30.9176723514179,20.5637135564838));
#21707=CARTESIAN_POINT('Ctrl Pts',(130.308929318364,-30.9249612477197,20.5578895586274));
#21708=CARTESIAN_POINT('Ctrl Pts',(130.427243892803,-30.9374038280844,20.5520655607709));
#21709=CARTESIAN_POINT('Ctrl Pts',(130.458633390305,-30.9407049120561,20.5505204225913));
#21710=CARTESIAN_POINT('Ctrl Pts',(130.489971870862,-30.9443684702231,20.5489752844116));
#21711=CARTESIAN_POINT('Ctrl Pts',(130.521250400698,-30.9483925387851,20.547430146232));
#21712=CARTESIAN_POINT('Ctrl Pts',(130.639133823985,-30.9635585641743,20.5416067849992));
#21713=CARTESIAN_POINT('Ctrl Pts',(130.756544892001,-30.9838981252513,20.5357834237664));
#21714=CARTESIAN_POINT('Ctrl Pts',(130.872994388123,-31.0093727562818,20.5299600625335));
#21715=CARTESIAN_POINT('Ctrl Pts',(130.989303093239,-31.0348165877036,20.5241437419227));
#21716=CARTESIAN_POINT('Ctrl Pts',(131.104652142935,-31.0653830568798,20.5183274213119));
#21717=CARTESIAN_POINT('Ctrl Pts',(131.218558069123,-31.1009820169465,20.5125111007011));
#21718=CARTESIAN_POINT('Ctrl Pts',(131.332533733271,-31.1366027721814,20.5066912190963));
#21719=CARTESIAN_POINT('Ctrl Pts',(131.445064099874,-31.1772621231237,20.5008713374914));
#21720=CARTESIAN_POINT('Ctrl Pts',(131.555674906802,-31.2228184337596,20.4950514558865));
#21721=CARTESIAN_POINT('Ctrl Pts',(131.666021155679,-31.2682657831728,20.4892454942283));
#21722=CARTESIAN_POINT('Ctrl Pts',(131.774456630174,-31.318586560334,20.4834395325702));
#21723=CARTESIAN_POINT('Ctrl Pts',(131.880526439234,-31.3735905758807,20.477633570912));
#21724=CARTESIAN_POINT('Ctrl Pts',(131.986977706055,-31.4287924018014,20.4718067293338));
#21725=CARTESIAN_POINT('Ctrl Pts',(132.091045869467,-31.4887110738161,20.4659798877556));
#21726=CARTESIAN_POINT('Ctrl Pts',(132.192293101711,-31.5531063323345,20.4601530461774));
#21727=CARTESIAN_POINT('Ctrl Pts',(132.293540333954,-31.617501590853,20.4543262045991));
#21728=CARTESIAN_POINT('Ctrl Pts',(132.391966277858,-31.6863732213768,20.4484993630209));
#21729=CARTESIAN_POINT('Ctrl Pts',(132.487160670875,-31.7594357285724,20.4426725214427));
#21730=CARTESIAN_POINT('',(125.915001496759,-34.9965030704355,20.9896150285509));
#21731=CARTESIAN_POINT('Ctrl Pts',(125.915001496759,-34.9965030704355,20.9896150285509));
#21732=CARTESIAN_POINT('Ctrl Pts',(125.91512689229,-34.8500201210564,20.9824905061118));
#21733=CARTESIAN_POINT('Ctrl Pts',(125.923135046557,-34.7038771894251,20.9753659836726));
#21734=CARTESIAN_POINT('Ctrl Pts',(125.938894207772,-34.5588143878878,20.9682414612335));
#21735=CARTESIAN_POINT('Ctrl Pts',(125.954891578428,-34.41155887264,20.9610092472438));
#21736=CARTESIAN_POINT('Ctrl Pts',(125.978876003809,-34.2654163169503,20.953777033254));
#21737=CARTESIAN_POINT('Ctrl Pts',(126.010660788167,-34.1211384335784,20.9465448192643));
#21738=CARTESIAN_POINT('Ctrl Pts',(126.028532809329,-34.0400135357117,20.9424782734601));
#21739=CARTESIAN_POINT('Ctrl Pts',(126.048870132568,-33.9594777781739,20.9384117276559));
#21740=CARTESIAN_POINT('Ctrl Pts',(126.071632971449,-33.8796618863085,20.9343451818516));
#21741=CARTESIAN_POINT('Ctrl Pts',(126.104231036441,-33.7653596393831,20.9285215881815));
#21742=CARTESIAN_POINT('Ctrl Pts',(126.14187452446,-33.6522969932765,20.9226979945113));
#21743=CARTESIAN_POINT('Ctrl Pts',(126.184452343526,-33.540951994904,20.9168744008411));
#21744=CARTESIAN_POINT('Ctrl Pts',(126.226976444347,-33.4297474747878,20.9110581544995));
#21745=CARTESIAN_POINT('Ctrl Pts',(126.274422349496,-33.3202566701994,20.9052419081578));
#21746=CARTESIAN_POINT('Ctrl Pts',(126.32662874226,-33.2129441522971,20.8994256618162));
#21747=CARTESIAN_POINT('Ctrl Pts',(126.378782876136,-33.1057390548189,20.8936152375693));
#21748=CARTESIAN_POINT('Ctrl Pts',(126.435687840096,-33.0007082713178,20.8878048133224));
#21749=CARTESIAN_POINT('Ctrl Pts',(126.497133839223,-32.8982974378659,20.8819943890755));
#21750=CARTESIAN_POINT('Ctrl Pts',(126.56090569653,-32.7920101425102,20.8759640282508));
#21751=CARTESIAN_POINT('Ctrl Pts',(126.629568996516,-32.6885454758239,20.8699336674261));
#21752=CARTESIAN_POINT('Ctrl Pts',(126.702836030425,-32.5883750793839,20.8639033066015));
#21753=CARTESIAN_POINT('Ctrl Pts',(126.773351443211,-32.4919666883655,20.8580994223699));
#21754=CARTESIAN_POINT('Ctrl Pts',(126.84813076695,-32.3986099494432,20.8522955381384));
#21755=CARTESIAN_POINT('Ctrl Pts',(126.926873163261,-32.3086961440013,20.8464916539068));
#21756=CARTESIAN_POINT('Ctrl Pts',(127.005603928477,-32.2187956197913,20.8406886269711));
#21757=CARTESIAN_POINT('Ctrl Pts',(127.088296333163,-32.1323373248072,20.8348856000354));
#21758=CARTESIAN_POINT('Ctrl Pts',(127.174609845076,-32.0496787509732,20.8290825730997));
#21759=CARTESIAN_POINT('Ctrl Pts',(127.260930977569,-31.9670128792525,20.8232790338174));
#21760=CARTESIAN_POINT('Ctrl Pts',(127.350873558013,-31.8881476781286,20.8174754945352));
#21761=CARTESIAN_POINT('Ctrl Pts',(127.444061337675,-31.8134026682948,20.811671955253));
#21762=CARTESIAN_POINT('Ctrl Pts',(127.537279337046,-31.738633419527,20.8058665339507));
#21763=CARTESIAN_POINT('Ctrl Pts',(127.633744310213,-31.6679872746706,20.8000611126484));
#21764=CARTESIAN_POINT('Ctrl Pts',(127.733048718335,-31.6017420806308,20.7942556913462));
#21765=CARTESIAN_POINT('Ctrl Pts',(127.832463096895,-31.5354235261713,20.7884438410772));
#21766=CARTESIAN_POINT('Ctrl Pts',(127.934722847032,-31.4735158774813,20.7826319908083));
#21767=CARTESIAN_POINT('Ctrl Pts',(128.039393238387,-31.416252502433,20.7768201405394));
#21768=CARTESIAN_POINT('Ctrl Pts',(128.144132377816,-31.3589515164932,20.7710044730161));
#21769=CARTESIAN_POINT('Ctrl Pts',(128.251284946046,-31.3063010587736,20.7651888054928));
#21770=CARTESIAN_POINT('Ctrl Pts',(128.360395032915,-31.2584868633254,20.7593731379695));
#21771=CARTESIAN_POINT('Ctrl Pts',(128.4696614082,-31.2106041792058,20.7535491401305));
#21772=CARTESIAN_POINT('Ctrl Pts',(128.580890519145,-31.1675717309309,20.7477251422915));
#21773=CARTESIAN_POINT('Ctrl Pts',(128.693609942556,-31.1295258665364,20.7419011444524));
#21774=CARTESIAN_POINT('Ctrl Pts',(128.723515020338,-31.1194320912171,20.7403560060627));
#21775=CARTESIAN_POINT('Ctrl Pts',(128.753524935726,-31.1096890286293,20.738810867673));
#21776=CARTESIAN_POINT('Ctrl Pts',(128.783630750152,-31.1002986206603,20.7372657292832));
#21777=CARTESIAN_POINT('Ctrl Pts',(128.897101478,-31.0649055762484,20.7314420044961));
#21778=CARTESIAN_POINT('Ctrl Pts',(129.012301234534,-31.0344121028999,20.725618279709));
#21779=CARTESIAN_POINT('Ctrl Pts',(129.128769267185,-31.0089873452721,20.7197945549218));
#21780=CARTESIAN_POINT('Ctrl Pts',(129.245089716674,-30.9835948047774,20.7139782097023));
#21781=CARTESIAN_POINT('Ctrl Pts',(129.362674850251,-30.9632582911488,20.7081618644827));
#21782=CARTESIAN_POINT('Ctrl Pts',(129.481047661269,-30.9480975492831,20.7023455192632));
#21783=CARTESIAN_POINT('Ctrl Pts',(129.599301329125,-30.9329520668231,20.6965350282407));
#21784=CARTESIAN_POINT('Ctrl Pts',(129.718340694462,-30.9229720438498,20.6907245372182));
#21785=CARTESIAN_POINT('Ctrl Pts',(129.837678020972,-30.9182262954538,20.6849140461958));
#21786=CARTESIAN_POINT('Ctrl Pts',(129.956926128198,-30.9134840950867,20.6791078992278));
#21787=CARTESIAN_POINT('Ctrl Pts',(130.076471346678,-30.9139683982542,20.6733017522598));
#21788=CARTESIAN_POINT('Ctrl Pts',(130.195820874261,-30.9196961895953,20.6674956052919));
#21789=CARTESIAN_POINT('Ctrl Pts',(130.315122580259,-30.9254216858953,20.6616917847609));
#21790=CARTESIAN_POINT('Ctrl Pts',(130.434228344077,-30.9363864729506,20.6558879642299));
#21791=CARTESIAN_POINT('Ctrl Pts',(130.552645896452,-30.9525554342111,20.6500841436989));
#21792=CARTESIAN_POINT('Ctrl Pts',(130.671043947322,-30.9687217326982,20.6442812789658));
#21793=CARTESIAN_POINT('Ctrl Pts',(130.788753607799,-30.9900904452799,20.6384784142326));
#21794=CARTESIAN_POINT('Ctrl Pts',(130.905288900095,-31.0165747142233,20.6326755494995));
#21795=CARTESIAN_POINT('Ctrl Pts',(131.021832502884,-31.0430608718421,20.6268722709461));
#21796=CARTESIAN_POINT('Ctrl Pts',(131.137201172975,-31.0746632200958,20.6210689923927));
#21797=CARTESIAN_POINT('Ctrl Pts',(131.250920904946,-31.1112441720303,20.6152657138392));
#21798=CARTESIAN_POINT('Ctrl Pts',(131.364740372975,-31.1478572066988,20.609457345614));
#21799=CARTESIAN_POINT('Ctrl Pts',(131.476907624376,-31.1894574428983,20.6036489773887));
#21800=CARTESIAN_POINT('Ctrl Pts',(131.586965380306,-31.2358578823707,20.5978406091634));
#21801=CARTESIAN_POINT('Ctrl Pts',(131.697070883064,-31.2822784519451,20.5920297210688));
#21802=CARTESIAN_POINT('Ctrl Pts',(131.8050646971,-31.3335032005729,20.5862188329742));
#21803=CARTESIAN_POINT('Ctrl Pts',(131.910512544768,-31.3892982930898,20.5804079448795));
#21804=CARTESIAN_POINT('Ctrl Pts',(132.016116110585,-31.4451757799725,20.5745884756639));
#21805=CARTESIAN_POINT('Ctrl Pts',(132.119165843915,-31.5056368914197,20.5687690064483));
#21806=CARTESIAN_POINT('Ctrl Pts',(132.21925449863,-31.5704031621328,20.5629495372327));
#21807=CARTESIAN_POINT('Ctrl Pts',(132.311149248095,-31.6298672466273,20.5576064874425));
#21808=CARTESIAN_POINT('Ctrl Pts',(132.400548046593,-31.6929598019526,20.5522634376522));
#21809=CARTESIAN_POINT('Ctrl Pts',(132.487160670875,-31.7594357285724,20.546920387862));
#21810=CARTESIAN_POINT('Ctrl Pts',(132.487160670875,-31.7594357285724,21.7969524316048));
#21811=CARTESIAN_POINT('Ctrl Pts',(132.581957158607,-31.8321928400738,21.7911469930517));
#21812=CARTESIAN_POINT('Ctrl Pts',(132.673521068581,-31.9090843242138,21.7853415544986));
#21813=CARTESIAN_POINT('Ctrl Pts',(132.761485630824,-31.9897803882855,21.7795361159454));
#21814=CARTESIAN_POINT('Ctrl Pts',(132.849547669554,-32.0705658743763,21.7737242441909));
#21815=CARTESIAN_POINT('Ctrl Pts',(132.934002098028,-32.1551640796059,21.7679123724363));
#21816=CARTESIAN_POINT('Ctrl Pts',(133.014518887018,-32.2432082269764,21.7621005006818));
#21817=CARTESIAN_POINT('Ctrl Pts',(133.095088674169,-32.3313103272023,21.7562848034082));
#21818=CARTESIAN_POINT('Ctrl Pts',(133.171715398641,-32.4228625743367,21.7504691061346));
#21819=CARTESIAN_POINT('Ctrl Pts',(133.244110264468,-32.5174662959045,21.744653408861));
#21820=CARTESIAN_POINT('Ctrl Pts',(133.316608699753,-32.6122053593371,21.7388293915414));
#21821=CARTESIAN_POINT('Ctrl Pts',(133.384862959886,-32.7100042767398,21.7330053742217));
#21822=CARTESIAN_POINT('Ctrl Pts',(133.448628295567,-32.8104366008229,21.7271813569022));
#21823=CARTESIAN_POINT('Ctrl Pts',(133.465118347645,-32.8364089294683,21.7256752353099));
#21824=CARTESIAN_POINT('Ctrl Pts',(133.481308438933,-32.8625572522097,21.7241691137177));
#21825=CARTESIAN_POINT('Ctrl Pts',(133.497194851732,-32.8888739570981,21.7226629921254));
#21826=CARTESIAN_POINT('Ctrl Pts',(133.558621507787,-32.9906305462117,21.7168393984549));
#21827=CARTESIAN_POINT('Ctrl Pts',(133.615702371735,-33.0952344137982,21.7110158047843));
#21828=CARTESIAN_POINT('Ctrl Pts',(133.668163334243,-33.2022784550113,21.7051922111138));
#21829=CARTESIAN_POINT('Ctrl Pts',(133.720558109454,-33.3091874442664,21.6993759647716));
#21830=CARTESIAN_POINT('Ctrl Pts',(133.768344398241,-33.4185301203645,21.6935597184295));
#21831=CARTESIAN_POINT('Ctrl Pts',(133.811292182914,-33.5298718095139,21.6877434720874));
#21832=CARTESIAN_POINT('Ctrl Pts',(133.854196976617,-33.6411020450188,21.6819330478399));
#21833=CARTESIAN_POINT('Ctrl Pts',(133.892272755379,-33.754326934,21.6761226235925));
#21834=CARTESIAN_POINT('Ctrl Pts',(133.925336397826,-33.8690892325637,21.670312199345));
#21835=CARTESIAN_POINT('Ctrl Pts',(133.959651567534,-33.9881955215219,21.6642818385205));
#21836=CARTESIAN_POINT('Ctrl Pts',(133.988567467094,-34.1089575054924,21.658251477696));
#21837=CARTESIAN_POINT('Ctrl Pts',(134.011935046681,-34.2308432011541,21.6522211168715));
#21838=CARTESIAN_POINT('Ctrl Pts',(134.03442503205,-34.3481513503324,21.6464172326392));
#21839=CARTESIAN_POINT('Ctrl Pts',(134.051775844246,-34.4664998918664,21.6406133484068));
#21840=CARTESIAN_POINT('Ctrl Pts',(134.063906187566,-34.5854020035479,21.6348094641745));
#21841=CARTESIAN_POINT('Ctrl Pts',(134.076034739105,-34.7042865521161,21.6290064372379));
#21842=CARTESIAN_POINT('Ctrl Pts',(134.082944313849,-34.823724102102,21.6232034103013));
#21843=CARTESIAN_POINT('Ctrl Pts',(134.084605395569,-34.943221813292,21.6174003833647));
#21844=CARTESIAN_POINT('Ctrl Pts',(134.086266623946,-35.0627300748804,21.6115968440815));
#21845=CARTESIAN_POINT('Ctrl Pts',(134.082678432297,-35.182298099916,21.6057933047983));
#21846=CARTESIAN_POINT('Ctrl Pts',(134.073863433233,-35.3014327907893,21.5999897655151));
#21847=CARTESIAN_POINT('Ctrl Pts',(134.065045575568,-35.4206061156535,21.5941843442118));
#21848=CARTESIAN_POINT('Ctrl Pts',(134.050997569646,-35.5393454198682,21.5883789229085));
#21849=CARTESIAN_POINT('Ctrl Pts',(134.031793849582,-35.6571631110081,21.5825735016052));
#21850=CARTESIAN_POINT('Ctrl Pts',(134.012568863176,-35.7751112743365,21.5767616513352));
#21851=CARTESIAN_POINT('Ctrl Pts',(133.988176831755,-35.8921353841254,21.5709498010651));
#21852=CARTESIAN_POINT('Ctrl Pts',(133.958743270378,-36.0077582642874,21.565137950795));
#21853=CARTESIAN_POINT('Ctrl Pts',(133.92929037688,-36.1234570861776,21.5593222832705));
#21854=CARTESIAN_POINT('Ctrl Pts',(133.894789476611,-36.2377524555536,21.553506615746));
#21855=CARTESIAN_POINT('Ctrl Pts',(133.855415376923,-36.350184162025,21.5476909482214));
#21856=CARTESIAN_POINT('Ctrl Pts',(133.81598487809,-36.4627769147761,21.5418669503811));
#21857=CARTESIAN_POINT('Ctrl Pts',(133.771667398671,-36.5735002987015,21.5360429525408));
#21858=CARTESIAN_POINT('Ctrl Pts',(133.722685139917,-36.6819156783392,21.5302189547005));
#21859=CARTESIAN_POINT('Ctrl Pts',(133.709689879603,-36.7106788696696,21.5286738163193));
#21860=CARTESIAN_POINT('Ctrl Pts',(133.696366524453,-36.7392797522863,21.5271286779382));
#21861=CARTESIAN_POINT('Ctrl Pts',(133.682719745472,-36.7677104616737,21.525583539557));
#21862=CARTESIAN_POINT('Ctrl Pts',(133.631285325959,-36.8748652002156,21.5197599458861));
#21863=CARTESIAN_POINT('Ctrl Pts',(133.575087319942,-36.9799460179862,21.5139363522152));
#21864=CARTESIAN_POINT('Ctrl Pts',(133.514315961416,-37.0825004978007,21.5081127585444));
#21865=CARTESIAN_POINT('Ctrl Pts',(133.453621274985,-37.1849255899053,21.502296512202));
#21866=CARTESIAN_POINT('Ctrl Pts',(133.3883649187,-37.2848303354245,21.4964802658595));
#21867=CARTESIAN_POINT('Ctrl Pts',(133.318784353857,-37.3817840818588,21.4906640195171));
#21868=CARTESIAN_POINT('Ctrl Pts',(133.249273439543,-37.4786407770581,21.4848535952694));
#21869=CARTESIAN_POINT('Ctrl Pts',(133.175447164514,-37.5725520198836,21.4790431710217));
#21870=CARTESIAN_POINT('Ctrl Pts',(133.0975875739,-37.663114008453,21.4732327467739));
#21871=CARTESIAN_POINT('Ctrl Pts',(133.01678083673,-37.7571039556174,21.4672023859495));
#21872=CARTESIAN_POINT('Ctrl Pts',(132.931629640789,-37.8474857007242,21.4611720251251));
#21873=CARTESIAN_POINT('Ctrl Pts',(132.842497217892,-37.933842968919,21.4551416643007));
#21874=CARTESIAN_POINT('Ctrl Pts',(132.756712257601,-38.0169569983845,21.4493377800681));
#21875=CARTESIAN_POINT('Ctrl Pts',(132.667240035614,-38.0963430768909,21.4435338958355));
#21876=CARTESIAN_POINT('Ctrl Pts',(132.574443152638,-38.1716663528558,21.4377300116029));
#21877=CARTESIAN_POINT('Ctrl Pts',(132.481659976753,-38.2469785027672,21.4319269846661));
#21878=CARTESIAN_POINT('Ctrl Pts',(132.385553433452,-38.3182287863131,21.4261239577293));
#21879=CARTESIAN_POINT('Ctrl Pts',(132.286519540347,-38.385122359917,21.4203209307924));
#21880=CARTESIAN_POINT('Ctrl Pts',(132.187476903585,-38.452021839524,21.414517391509));
#21881=CARTESIAN_POINT('Ctrl Pts',(132.085506741543,-38.5145636158361,21.4087138522256));
#21882=CARTESIAN_POINT('Ctrl Pts',(131.981033862242,-38.5724963032383,21.4029103129422));
#21883=CARTESIAN_POINT('Ctrl Pts',(131.876527103605,-38.6304477775353,21.3971048916386));
#21884=CARTESIAN_POINT('Ctrl Pts',(131.769516370539,-38.6837869924312,21.3912994703351));
#21885=CARTESIAN_POINT('Ctrl Pts',(131.660450273352,-38.732308922065,21.3854940490315));
#21886=CARTESIAN_POINT('Ctrl Pts',(131.551263395557,-38.7808845852445,21.3796821987613));
#21887=CARTESIAN_POINT('Ctrl Pts',(131.440016983603,-38.8246321485716,21.373870348491));
#21888=CARTESIAN_POINT('Ctrl Pts',(131.327178936584,-38.8633950186705,21.3680584982208));
#21889=CARTESIAN_POINT('Ctrl Pts',(131.21426677693,-38.9021833484305,21.362242830696));
#21890=CARTESIAN_POINT('Ctrl Pts',(131.099761291015,-38.9359803494343,21.3564271631713));
#21891=CARTESIAN_POINT('Ctrl Pts',(130.984143208555,-38.9646799549341,21.3506114956466));
#21892=CARTESIAN_POINT('Ctrl Pts',(130.868359515676,-38.9934206695197,21.3447874978061));
#21893=CARTESIAN_POINT('Ctrl Pts',(130.751460444186,-39.0170493346535,21.3389634999656));
#21894=CARTESIAN_POINT('Ctrl Pts',(130.63393465876,-39.0355113490638,21.3331395021252));
#21895=CARTESIAN_POINT('Ctrl Pts',(130.602754427149,-39.0404094221398,21.3315943637463));
#21896=CARTESIAN_POINT('Ctrl Pts',(130.571530096223,-39.0449441144374,21.3300492253674));
#21897=CARTESIAN_POINT('Ctrl Pts',(130.540270804112,-39.0491150216096,21.3285040869885));
#21898=CARTESIAN_POINT('Ctrl Pts',(130.422455197195,-39.0648350820046,21.3226804933117));
#21899=CARTESIAN_POINT('Ctrl Pts',(130.303762933154,-39.0754341682595,21.316856899635));
#21900=CARTESIAN_POINT('Ctrl Pts',(130.184676680017,-39.0808233879767,21.3110333059582));
#21901=CARTESIAN_POINT('Ctrl Pts',(130.065740671876,-39.0862058083928,21.3052170596099));
#21902=CARTESIAN_POINT('Ctrl Pts',(129.946412067634,-39.0863914175571,21.2994008132615));
#21903=CARTESIAN_POINT('Ctrl Pts',(129.827181220251,-39.0813427532328,21.2935845669132));
#21904=CARTESIAN_POINT('Ctrl Pts',(129.708069723603,-39.0762991426494,21.2877741426595));
#21905=CARTESIAN_POINT('Ctrl Pts',(129.589056194769,-39.0660316991624,21.2819637184058));
#21906=CARTESIAN_POINT('Ctrl Pts',(129.470632968861,-39.050554967698,21.2761532941521));
#21907=CARTESIAN_POINT('Ctrl Pts',(129.347727179064,-39.0344924099563,21.2701229333299));
#21908=CARTESIAN_POINT('Ctrl Pts',(129.2254577113,-39.0128183873161,21.2640925725078));
#21909=CARTESIAN_POINT('Ctrl Pts',(129.104371836293,-38.9856085096726,21.2580622116856));
#21910=CARTESIAN_POINT('Ctrl Pts',(128.987833469488,-38.9594205277848,21.2522583274471));
#21911=CARTESIAN_POINT('Ctrl Pts',(128.872391830741,-38.9281050996682,21.2464544432085));
#21912=CARTESIAN_POINT('Ctrl Pts',(128.758525744755,-38.8917819406493,21.24065055897));
#21913=CARTESIAN_POINT('Ctrl Pts',(128.644676478008,-38.8554641469495,21.2348475320272));
#21914=CARTESIAN_POINT('Ctrl Pts',(128.53240269012,-38.8141402174323,21.2290445050844));
#21915=CARTESIAN_POINT('Ctrl Pts',(128.422168062184,-38.7679797472927,21.2232414781417));
#21916=CARTESIAN_POINT('Ctrl Pts',(128.311923701683,-38.7218152016666,21.2174379388524));
#21917=CARTESIAN_POINT('Ctrl Pts',(128.203719235756,-38.6708134241352,21.211634399563));
#21918=CARTESIAN_POINT('Ctrl Pts',(128.097997780361,-38.6151919114329,21.2058308602737));
#21919=CARTESIAN_POINT('Ctrl Pts',(127.992242040732,-38.5595523613225,21.2000254389642));
#21920=CARTESIAN_POINT('Ctrl Pts',(127.888971274208,-38.4992902866326,21.1942200176547));
#21921=CARTESIAN_POINT('Ctrl Pts',(127.788602870336,-38.4346685043705,21.1884145963453));
#21922=CARTESIAN_POINT('Ctrl Pts',(127.688123317749,-38.3699751594673,21.1826027460692));
#21923=CARTESIAN_POINT('Ctrl Pts',(127.590552886961,-38.3009126911278,21.1767908957931));
#21924=CARTESIAN_POINT('Ctrl Pts',(127.496279033396,-38.2277865978695,21.170979045517));
#21925=CARTESIAN_POINT('Ctrl Pts',(127.401943260257,-38.1546124750005,21.1651633779864));
#21926=CARTESIAN_POINT('Ctrl Pts',(127.310908687054,-38.077369675391,21.1593477104559));
#21927=CARTESIAN_POINT('Ctrl Pts',(127.223527543474,-37.9964021255757,21.1535320429253));
#21928=CARTESIAN_POINT('Ctrl Pts',(127.136021235844,-37.91531859849,21.1477080450792));
#21929=CARTESIAN_POINT('Ctrl Pts',(127.052179088948,-37.830499961599,21.141884047233));
#21930=CARTESIAN_POINT('Ctrl Pts',(126.972314637893,-37.7423249895085,21.1360600493868));
#21931=CARTESIAN_POINT('Ctrl Pts',(126.951126164413,-37.7189316895732,21.1345149110645));
#21932=CARTESIAN_POINT('Ctrl Pts',(126.930217438473,-37.695302314154,21.1329697727423));
#21933=CARTESIAN_POINT('Ctrl Pts',(126.909593807446,-37.6714442844691,21.1314246344201));
#21934=CARTESIAN_POINT('Ctrl Pts',(126.830727378882,-37.5802092545508,21.1255159008441));
#21935=CARTESIAN_POINT('Ctrl Pts',(126.755762331177,-37.4853140262217,21.119607167268));
#21936=CARTESIAN_POINT('Ctrl Pts',(126.685059339014,-37.3871307911681,21.113698433692));
#21937=CARTESIAN_POINT('Ctrl Pts',(126.616054083285,-37.2913051544312,21.1079315819793));
#21938=CARTESIAN_POINT('Ctrl Pts',(126.551108816856,-37.1923479642437,21.1021647302665));
#21939=CARTESIAN_POINT('Ctrl Pts',(126.490521185757,-37.0906418756876,21.0963978785538));
#21940=CARTESIAN_POINT('Ctrl Pts',(126.429989538292,-36.9890297646709,21.0906363554752));
#21941=CARTESIAN_POINT('Ctrl Pts',(126.373807733833,-36.8846741590728,21.0848748323965));
#21942=CARTESIAN_POINT('Ctrl Pts',(126.322231234452,-36.7779881628293,21.0791133093179));
#21943=CARTESIAN_POINT('Ctrl Pts',(126.270689699326,-36.6713744901527,21.0733556920368));
#21944=CARTESIAN_POINT('Ctrl Pts',(126.223747441912,-36.5624339410496,21.0675980747557));
#21945=CARTESIAN_POINT('Ctrl Pts',(126.181614543349,-36.451605147564,21.0618404574746));
#21946=CARTESIAN_POINT('Ctrl Pts',(126.137570475,-36.3357491034337,21.0558216717347));
#21947=CARTESIAN_POINT('Ctrl Pts',(126.09878257563,-36.2178298937377,21.0498028859948));
#21948=CARTESIAN_POINT('Ctrl Pts',(126.065434963677,-36.0983728760976,21.0437841002549));
#21949=CARTESIAN_POINT('Ctrl Pts',(126.033547892699,-35.9841477733897,21.038028922092));
#21950=CARTESIAN_POINT('Ctrl Pts',(126.006634741561,-35.8685171588103,21.0322737439292));
#21951=CARTESIAN_POINT('Ctrl Pts',(125.984805368353,-35.7519554973474,21.0265185657663));
#21952=CARTESIAN_POINT('Ctrl Pts',(125.962975205303,-35.6353896183894,21.0207631793666));
#21953=CARTESIAN_POINT('Ctrl Pts',(125.946229255171,-35.5178930355523,21.0150077929669));
#21954=CARTESIAN_POINT('Ctrl Pts',(125.934625988469,-35.3999489296956,21.0092524065672));
#21955=CARTESIAN_POINT('Ctrl Pts',(125.923016652512,-35.2819431314981,21.0034940097308));
#21956=CARTESIAN_POINT('Ctrl Pts',(125.916555398921,-35.1634897576063,20.9977356128944));
#21957=CARTESIAN_POINT('Ctrl Pts',(125.915248694863,-35.0450752169156,20.9919772160581));
#21958=CARTESIAN_POINT('Ctrl Pts',(125.915070017821,-35.0288833640235,20.9911898202372));
#21959=CARTESIAN_POINT('Ctrl Pts',(125.91498763816,-35.0126922353489,20.9904024244164));
#21960=CARTESIAN_POINT('Ctrl Pts',(125.915001496758,-34.9965030713517,20.9896150285955));
#21961=CARTESIAN_POINT('Origin',(130.,-35.,32.7603849714045));
#21962=CARTESIAN_POINT('',(132.487160670875,-31.7594357285724,23.0467792200739));
#21963=CARTESIAN_POINT('',(132.487160670875,-31.7594357285724,22.9427607399423));
#21964=CARTESIAN_POINT('',(132.487160670875,-31.7594357285724,32.7603849714045));
#21965=CARTESIAN_POINT('',(125.915000225098,-34.9986438840781,22.1353849714387));
#21966=CARTESIAN_POINT('Ctrl Pts',(132.487160670875,-31.7594357285724,22.9427607399423));
#21967=CARTESIAN_POINT('Ctrl Pts',(132.581883176809,-31.8321360584143,22.9369379462702));
#21968=CARTESIAN_POINT('Ctrl Pts',(132.673310070028,-31.9089120318643,22.931115152598));
#21969=CARTESIAN_POINT('Ctrl Pts',(132.761090344536,-31.9894178122312,22.9252923589258));
#21970=CARTESIAN_POINT('Ctrl Pts',(132.825958200078,-32.0489099630639,22.920989431635));
#21971=CARTESIAN_POINT('Ctrl Pts',(132.888835410539,-32.1104381248282,22.9166865043441));
#21972=CARTESIAN_POINT('Ctrl Pts',(132.949594421577,-32.1738510746601,22.9123835770533));
#21973=CARTESIAN_POINT('Ctrl Pts',(133.031825834812,-32.2596743359825,22.9065599833817));
#21974=CARTESIAN_POINT('Ctrl Pts',(133.110440991607,-32.3492279582961,22.9007363897102));
#21975=CARTESIAN_POINT('Ctrl Pts',(133.185083236696,-32.4421747957844,22.8949127960386));
#21976=CARTESIAN_POINT('Ctrl Pts',(133.259631309504,-32.535004367031,22.8890965496955));
#21977=CARTESIAN_POINT('Ctrl Pts',(133.330216186761,-32.6312183229795,22.8832803033524));
#21978=CARTESIAN_POINT('Ctrl Pts',(133.396518192138,-32.7304429572103,22.8774640570093));
#21979=CARTESIAN_POINT('Ctrl Pts',(133.462753828841,-32.8295682670347,22.8716536327609));
#21980=CARTESIAN_POINT('Ctrl Pts',(133.524714896913,-32.9316979221826,22.8658432085125));
#21981=CARTESIAN_POINT('Ctrl Pts',(133.582122530858,-33.0364259184035,22.8600327842641));
#21982=CARTESIAN_POINT('Ctrl Pts',(133.641703162486,-33.145118085894,22.8540024234399));
#21983=CARTESIAN_POINT('Ctrl Pts',(133.696378554533,-33.2566088367296,22.8479720626158));
#21984=CARTESIAN_POINT('Ctrl Pts',(133.74588670753,-33.3704117776715,22.8419417017917));
#21985=CARTESIAN_POINT('Ctrl Pts',(133.79353552938,-33.4799407285751,22.8361378175583));
#21986=CARTESIAN_POINT('Ctrl Pts',(133.836398057633,-33.5916109199558,22.830333933325));
#21987=CARTESIAN_POINT('Ctrl Pts',(133.874288296302,-33.70496517532,22.8245300490917));
#21988=CARTESIAN_POINT('Ctrl Pts',(133.912172938179,-33.8183026870484,22.8187270221542));
#21989=CARTESIAN_POINT('Ctrl Pts',(133.945086621664,-33.9333233808971,22.8129239952166));
#21990=CARTESIAN_POINT('Ctrl Pts',(133.972892553101,-34.0495528623264,22.8071209682791));
#21991=CARTESIAN_POINT('Ctrl Pts',(134.000700939511,-34.1657926056034,22.8013174289949));
#21992=CARTESIAN_POINT('Ctrl Pts',(134.023400582241,-34.2832409515025,22.7955138897108));
#21993=CARTESIAN_POINT('Ctrl Pts',(134.040905493144,-34.4014118314883,22.7897103504266));
#21994=CARTESIAN_POINT('Ctrl Pts',(134.058416080684,-34.5196210329124,22.7839049291224));
#21995=CARTESIAN_POINT('Ctrl Pts',(134.070728526322,-34.6385528306901,22.7780995078181));
#21996=CARTESIAN_POINT('Ctrl Pts',(134.077808610295,-34.7577151721628,22.7722940865139));
#21997=CARTESIAN_POINT('Ctrl Pts',(134.084896534807,-34.877009474899,22.7664822362429));
#21998=CARTESIAN_POINT('Ctrl Pts',(134.086740507389,-34.9965344230827,22.7606703859719));
#21999=CARTESIAN_POINT('Ctrl Pts',(134.083358430272,-35.1157969340037,22.7548585357009));
#22000=CARTESIAN_POINT('Ctrl Pts',(134.079974131789,-35.2351377771821,22.7490428681754));
#22001=CARTESIAN_POINT('Ctrl Pts',(134.071356977106,-35.3542154334826,22.74322720065));
#22002=CARTESIAN_POINT('Ctrl Pts',(134.057576680408,-35.4725425722714,22.7374115331245));
#22003=CARTESIAN_POINT('Ctrl Pts',(134.043776644923,-35.5910392019093,22.7315875352833));
#22004=CARTESIAN_POINT('Ctrl Pts',(134.024798770866,-35.7087827666205,22.7257635374421));
#22005=CARTESIAN_POINT('Ctrl Pts',(134.000763742125,-35.825296601048,22.7199395396009));
#22006=CARTESIAN_POINT('Ctrl Pts',(133.994387117992,-35.856208356401,22.7183944012289));
#22007=CARTESIAN_POINT('Ctrl Pts',(133.987654806676,-35.8870336423118,22.7168492628569));
#22008=CARTESIAN_POINT('Ctrl Pts',(133.980569642328,-35.9177637618566,22.7153041244849));
#22009=CARTESIAN_POINT('Ctrl Pts',(133.953865808544,-36.0335849290374,22.7094805308135));
#22010=CARTESIAN_POINT('Ctrl Pts',(133.9220597084,-36.1484264117011,22.7036569371421));
#22011=CARTESIAN_POINT('Ctrl Pts',(133.885237815503,-36.261805102616,22.6978333434707));
#22012=CARTESIAN_POINT('Ctrl Pts',(133.848462378892,-36.3750407494713,22.6920170971278));
#22013=CARTESIAN_POINT('Ctrl Pts',(133.806683861123,-36.4868168903464,22.6862008507848));
#22014=CARTESIAN_POINT('Ctrl Pts',(133.760039584541,-36.5966613049366,22.6803846044419));
#22015=CARTESIAN_POINT('Ctrl Pts',(133.713441999138,-36.7063957646617,22.6745741801936));
#22016=CARTESIAN_POINT('Ctrl Pts',(133.661988503165,-36.8142019712026,22.6687637559454));
#22017=CARTESIAN_POINT('Ctrl Pts',(133.605865802954,-36.9196241327626,22.6629533316971));
#22018=CARTESIAN_POINT('Ctrl Pts',(133.547618742458,-37.0290367411901,22.6569229708729));
#22019=CARTESIAN_POINT('Ctrl Pts',(133.48434215393,-37.1358808302264,22.6508926100487));
#22020=CARTESIAN_POINT('Ctrl Pts',(133.416299224074,-37.2396706480178,22.6448622492245));
#22021=CARTESIAN_POINT('Ctrl Pts',(133.350811718553,-37.3395625292177,22.6390583649913));
#22022=CARTESIAN_POINT('Ctrl Pts',(133.280909669463,-37.436625042598,22.6332544807582));
#22023=CARTESIAN_POINT('Ctrl Pts',(133.206873489809,-37.5304520189804,22.627450596525));
#22024=CARTESIAN_POINT('Ctrl Pts',(133.132848246089,-37.624265136115,22.6216475695876));
#22025=CARTESIAN_POINT('Ctrl Pts',(133.054690339081,-37.7148433462175,22.6158445426502));
#22026=CARTESIAN_POINT('Ctrl Pts',(132.972721553387,-37.8018121932118,22.6100415157128));
#22027=CARTESIAN_POINT('Ctrl Pts',(132.890745530706,-37.8887887186459,22.6042379764288));
#22028=CARTESIAN_POINT('Ctrl Pts',(132.804958240457,-37.9721549502126,22.5984344371448));
#22029=CARTESIAN_POINT('Ctrl Pts',(132.715719080768,-38.0515725248392,22.5926308978609));
#22030=CARTESIAN_POINT('Ctrl Pts',(132.62645098186,-38.131015853659,22.5868254765568));
#22031=CARTESIAN_POINT('Ctrl Pts',(132.533729092154,-38.2065077075828,22.5810200552527));
#22032=CARTESIAN_POINT('Ctrl Pts',(132.437946192269,-38.277749740844,22.5752146339485));
#22033=CARTESIAN_POINT('Ctrl Pts',(132.342057221687,-38.3490706680631,22.5694027836777));
#22034=CARTESIAN_POINT('Ctrl Pts',(132.243100802464,-38.4161321366339,22.5635909334068));
#22035=CARTESIAN_POINT('Ctrl Pts',(132.141499148098,-38.478678829483,22.557779083136));
#22036=CARTESIAN_POINT('Ctrl Pts',(132.039830761221,-38.5412666033358,22.5519634156107));
#22037=CARTESIAN_POINT('Ctrl Pts',(131.935514035084,-38.5993334977942,22.5461477480854));
#22038=CARTESIAN_POINT('Ctrl Pts',(131.828994773743,-38.652670682887,22.5403320805601));
#22039=CARTESIAN_POINT('Ctrl Pts',(131.722322935062,-38.706084267738,22.534508082719));
#22040=CARTESIAN_POINT('Ctrl Pts',(131.613442635645,-38.7547544550479,22.5286840848779));
#22041=CARTESIAN_POINT('Ctrl Pts',(131.502818699154,-38.798520890751,22.5228600870369));
#22042=CARTESIAN_POINT('Ctrl Pts',(131.473469565799,-38.8101323647112,22.5213149486634));
#22043=CARTESIAN_POINT('Ctrl Pts',(131.443997778231,-38.8213989527745,22.5197698102899));
#22044=CARTESIAN_POINT('Ctrl Pts',(131.414412163886,-38.8323182580068,22.5182246719164));
#22045=CARTESIAN_POINT('Ctrl Pts',(131.302904612573,-38.8734728872218,22.5124010782451));
#22046=CARTESIAN_POINT('Ctrl Pts',(131.189419564544,-38.9098231007079,22.5065774845737));
#22047=CARTESIAN_POINT('Ctrl Pts',(131.07440847843,-38.9411764007054,22.5007538909024));
#22048=CARTESIAN_POINT('Ctrl Pts',(130.959542495885,-38.9724901438579,22.4949376445594));
#22049=CARTESIAN_POINT('Ctrl Pts',(130.843154695165,-38.9988194062718,22.4891213982165));
#22050=CARTESIAN_POINT('Ctrl Pts',(130.725715302816,-39.0200201864243,22.4833051518736));
#22051=CARTESIAN_POINT('Ctrl Pts',(130.608393467947,-39.0411997444788,22.4774947276254));
#22052=CARTESIAN_POINT('Ctrl Pts',(130.490022535097,-39.0572609608853,22.4716843033772));
#22053=CARTESIAN_POINT('Ctrl Pts',(130.371086060982,-39.0681101429711,22.4658738791289));
#22054=CARTESIAN_POINT('Ctrl Pts',(130.247647595317,-39.0793699890391,22.4598435183047));
#22055=CARTESIAN_POINT('Ctrl Pts',(130.123600361081,-39.0850153142089,22.4538131574805));
#22056=CARTESIAN_POINT('Ctrl Pts',(129.999494896475,-39.0849999687724,22.4477827966563));
#22057=CARTESIAN_POINT('Ctrl Pts',(129.880050344106,-39.08498519965,22.4419789124232));
#22058=CARTESIAN_POINT('Ctrl Pts',(129.760552301349,-39.0797272772828,22.4361750281901));
#22059=CARTESIAN_POINT('Ctrl Pts',(129.641494188579,-39.069238083865,22.4303711439569));
#22060=CARTESIAN_POINT('Ctrl Pts',(129.522453661967,-39.0587504398133,22.4245681170196));
#22061=CARTESIAN_POINT('Ctrl Pts',(129.403853342764,-39.0430330972231,22.4187650900822));
#22062=CARTESIAN_POINT('Ctrl Pts',(129.286182805827,-39.0221499242697,22.4129620631449));
#22063=CARTESIAN_POINT('Ctrl Pts',(129.168501879813,-39.0012649075506,22.4071585238609));
#22064=CARTESIAN_POINT('Ctrl Pts',(129.051751301354,-38.9752132250104,22.401354984577));
#22065=CARTESIAN_POINT('Ctrl Pts',(128.936411076525,-38.9441099885602,22.395551445293));
#22066=CARTESIAN_POINT('Ctrl Pts',(128.821033448205,-38.9129966656931,22.389746023989));
#22067=CARTESIAN_POINT('Ctrl Pts',(128.707067477154,-38.8768286372472,22.3839406026849));
#22068=CARTESIAN_POINT('Ctrl Pts',(128.59497799919,-38.8357708713164,22.3781351813808));
#22069=CARTESIAN_POINT('Ctrl Pts',(128.482764392504,-38.7946676377102,22.37232333111));
#22070=CARTESIAN_POINT('Ctrl Pts',(128.372431810508,-38.7486639984812,22.3665114808392));
#22071=CARTESIAN_POINT('Ctrl Pts',(128.264425235097,-38.6979731252989,22.3606996305684));
#22072=CARTESIAN_POINT('Ctrl Pts',(128.156347720388,-38.647248958079,22.3548839630431));
#22073=CARTESIAN_POINT('Ctrl Pts',(128.050599615636,-38.5918316148993,22.3490682955179));
#22074=CARTESIAN_POINT('Ctrl Pts',(127.947599953748,-38.5319794804252,22.3432526279926));
#22075=CARTESIAN_POINT('Ctrl Pts',(127.844452755967,-38.4720416142313,22.3374286301516));
#22076=CARTESIAN_POINT('Ctrl Pts',(127.744062201284,-38.4076564974399,22.3316046323106));
#22077=CARTESIAN_POINT('Ctrl Pts',(127.646817204616,-38.3391249948913,22.3257806344696));
#22078=CARTESIAN_POINT('Ctrl Pts',(127.621017576917,-38.3209432136995,22.3242354960957));
#22079=CARTESIAN_POINT('Ctrl Pts',(127.595439167258,-38.3024697941764,22.3226903577218));
#22080=CARTESIAN_POINT('Ctrl Pts',(127.570088819245,-38.2837108054217,22.321145219348));
#22081=CARTESIAN_POINT('Ctrl Pts',(127.475346633759,-38.2136025926574,22.315370553598));
#22082=CARTESIAN_POINT('Ctrl Pts',(127.383475506378,-38.1392680574956,22.309595887848));
#22083=CARTESIAN_POINT('Ctrl Pts',(127.29488013663,-38.0609723168952,22.303821222098));
#22084=CARTESIAN_POINT('Ctrl Pts',(127.206396987134,-37.9827757504145,22.2980538708889));
#22085=CARTESIAN_POINT('Ctrl Pts',(127.121181654222,-37.9006282275451,22.2922865196798));
#22086=CARTESIAN_POINT('Ctrl Pts',(127.039608898642,-37.814837389087,22.2865191684706));
#22087=CARTESIAN_POINT('Ctrl Pts',(126.95811726467,-37.7291318669908,22.2807575527157));
#22088=CARTESIAN_POINT('Ctrl Pts',(126.88026128903,-37.6397905344547,22.2749959369607));
#22089=CARTESIAN_POINT('Ctrl Pts',(126.806381191527,-37.5471599687034,22.2692343212057));
#22090=CARTESIAN_POINT('Ctrl Pts',(126.732553088088,-37.4545945928993,22.2634767602617));
#22091=CARTESIAN_POINT('Ctrl Pts',(126.662695556031,-37.35874491222,22.2577191993176));
#22092=CARTESIAN_POINT('Ctrl Pts',(126.597110128043,-37.2599923715208,22.2519616383735));
#22093=CARTESIAN_POINT('Ctrl Pts',(126.53154875107,-37.1612760446406,22.2462061888007));
#22094=CARTESIAN_POINT('Ctrl Pts',(126.470256594023,-37.0596593197758,22.2404507392278));
#22095=CARTESIAN_POINT('Ctrl Pts',(126.413492877872,-36.955554055229,22.2346952896549));
#22096=CARTESIAN_POINT('Ctrl Pts',(126.356735998231,-36.8514613289169,22.2289405332572));
#22097=CARTESIAN_POINT('Ctrl Pts',(126.304506673962,-36.7448810241795,22.2231857768594));
#22098=CARTESIAN_POINT('Ctrl Pts',(126.257018645826,-36.6362504644172,22.2174310204617));
#22099=CARTESIAN_POINT('Ctrl Pts',(126.209524641704,-36.5276062343738,22.2116755398742));
#22100=CARTESIAN_POINT('Ctrl Pts',(126.166773285701,-36.4169116179162,22.2059200592867));
#22101=CARTESIAN_POINT('Ctrl Pts',(126.128930263853,-36.3046241213032,22.2001645786991));
#22102=CARTESIAN_POINT('Ctrl Pts',(126.091051218587,-36.1922297363084,22.1944036193716));
#22103=CARTESIAN_POINT('Ctrl Pts',(126.058089971144,-36.0782398380018,22.188642660044));
#22104=CARTESIAN_POINT('Ctrl Pts',(126.030162393893,-35.9631273961087,22.1828817007164));
#22105=CARTESIAN_POINT('Ctrl Pts',(126.002220875286,-35.8479574904619,22.1771178655368));
#22106=CARTESIAN_POINT('Ctrl Pts',(125.979318111483,-35.7316643332545,22.1713540303573));
#22107=CARTESIAN_POINT('Ctrl Pts',(125.961518545287,-35.6147296478435,22.1655901951777));
#22108=CARTESIAN_POINT('Ctrl Pts',(125.943692203764,-35.4976190612692,22.1598176896424));
#22109=CARTESIAN_POINT('Ctrl Pts',(125.930984437041,-35.3798654324984,22.1540451841071));
#22110=CARTESIAN_POINT('Ctrl Pts',(125.923407691792,-35.2619544858525,22.1482726785719));
#22111=CARTESIAN_POINT('Ctrl Pts',(125.917769073044,-35.1742050825885,22.1439767761941));
#22112=CARTESIAN_POINT('Ctrl Pts',(125.914971102718,-35.0863686220552,22.1396808738164));
#22113=CARTESIAN_POINT('Ctrl Pts',(125.915000225098,-34.9986438840781,22.1353849714387));
#22114=CARTESIAN_POINT('Ctrl Pts',(125.915000225098,-34.9986438833803,22.1353849714045));
#22115=CARTESIAN_POINT('Ctrl Pts',(125.915025803142,-34.921595712626,22.1316119031962));
#22116=CARTESIAN_POINT('Ctrl Pts',(125.917231078305,-34.8445868960673,22.1278388349879));
#22117=CARTESIAN_POINT('Ctrl Pts',(125.921610227948,-34.7677030623887,22.1240657667795));
#22118=CARTESIAN_POINT('Ctrl Pts',(125.928369286289,-34.6490356589768,22.118242173109));
#22119=CARTESIAN_POINT('Ctrl Pts',(125.940322775489,-34.5304721391276,22.1124185794384));
#22120=CARTESIAN_POINT('Ctrl Pts',(125.957467056685,-34.4125032747234,22.1065949857679));
#22121=CARTESIAN_POINT('Ctrl Pts',(125.974589707823,-34.2946832455644,22.1007787394257));
#22122=CARTESIAN_POINT('Ctrl Pts',(125.99689006703,-34.1774567801585,22.0949624930836));
#22123=CARTESIAN_POINT('Ctrl Pts',(126.024312538453,-34.0613125077557,22.0891462467415));
#22124=CARTESIAN_POINT('Ctrl Pts',(126.05170755983,-33.9452844964101,22.083335822494));
#22125=CARTESIAN_POINT('Ctrl Pts',(126.084214400078,-33.8303369181398,22.0775253982466));
#22126=CARTESIAN_POINT('Ctrl Pts',(126.121726014143,-33.716950550204,22.0717149739991));
#22127=CARTESIAN_POINT('Ctrl Pts',(126.160657520395,-33.5992722736939,22.0656846131746));
#22128=CARTESIAN_POINT('Ctrl Pts',(126.204980104197,-33.4832761764104,22.0596542523501));
#22129=CARTESIAN_POINT('Ctrl Pts',(126.254516398774,-33.3694854821411,22.0536238915256));
#22130=CARTESIAN_POINT('Ctrl Pts',(126.302192305306,-33.2599683179982,22.0478200072933));
#22131=CARTESIAN_POINT('Ctrl Pts',(126.354697194335,-33.1524942997649,22.0420161230609));
#22132=CARTESIAN_POINT('Ctrl Pts',(126.41182327944,-33.0475111211504,22.0362122388286));
#22133=CARTESIAN_POINT('Ctrl Pts',(126.468940926411,-32.9425434496741,22.030409211892));
#22134=CARTESIAN_POINT('Ctrl Pts',(126.530678216865,-32.8400662447102,22.0246061849554));
#22135=CARTESIAN_POINT('Ctrl Pts',(126.596781231034,-32.7405029297297,22.0188031580188));
#22136=CARTESIAN_POINT('Ctrl Pts',(126.662890081408,-32.6409308243493,22.0129996187356));
#22137=CARTESIAN_POINT('Ctrl Pts',(126.73336519599,-32.544273460662,22.0071960794524));
#22138=CARTESIAN_POINT('Ctrl Pts',(126.807909486029,-32.4509250402118,22.0013925401692));
#22139=CARTESIAN_POINT('Ctrl Pts',(126.882477949913,-32.3575463479574,21.9955871188659));
#22140=CARTESIAN_POINT('Ctrl Pts',(126.961117958938,-32.2674790519153,21.9897816975626));
#22141=CARTESIAN_POINT('Ctrl Pts',(127.043492762845,-32.1810835491896,21.9839762762592));
#22142=CARTESIAN_POINT('Ctrl Pts',(127.125958789223,-32.094592371441,21.9781644259892));
#22143=CARTESIAN_POINT('Ctrl Pts',(127.212167584225,-32.0117813991429,21.9723525757191));
#22144=CARTESIAN_POINT('Ctrl Pts',(127.301746120357,-31.932973589779,21.966540725449));
#22145=CARTESIAN_POINT('Ctrl Pts',(127.391383492153,-31.8541140190227,21.9607250579245));
#22146=CARTESIAN_POINT('Ctrl Pts',(127.484394695461,-31.7792631029338,21.9549093903999));
#22147=CARTESIAN_POINT('Ctrl Pts',(127.580375599858,-31.70870196393,21.9490937228754));
#22148=CARTESIAN_POINT('Ctrl Pts',(127.676493986537,-31.6380397537135,21.9432697250351));
#22149=CARTESIAN_POINT('Ctrl Pts',(127.775590226525,-31.5716798113531,21.9374457271948));
#22150=CARTESIAN_POINT('Ctrl Pts',(127.877233255865,-31.5098586919733,21.9316217293544));
#22151=CARTESIAN_POINT('Ctrl Pts',(127.904199705735,-31.4934572119356,21.9300765909733));
#22152=CARTESIAN_POINT('Ctrl Pts',(127.931345296024,-31.4773749482052,21.9285314525922));
#22153=CARTESIAN_POINT('Ctrl Pts',(127.958661730927,-31.4616157541588,21.9269863142111));
#22154=CARTESIAN_POINT('Ctrl Pts',(128.061616792655,-31.4022196872256,21.9211627205402));
#22155=CARTESIAN_POINT('Ctrl Pts',(128.167332366969,-31.3472250375658,21.9153391268693));
#22156=CARTESIAN_POINT('Ctrl Pts',(128.275395991733,-31.2968977850092,21.9095155331985));
#22157=CARTESIAN_POINT('Ctrl Pts',(128.383323278183,-31.2466340277573,21.903699286856));
#22158=CARTESIAN_POINT('Ctrl Pts',(128.493592356012,-31.2010261261643,21.8978830405136));
#22159=CARTESIAN_POINT('Ctrl Pts',(128.605764074192,-31.1602954302203,21.8920667941712));
#22160=CARTESIAN_POINT('Ctrl Pts',(128.717823507863,-31.1196055059278,21.8862563699235));
#22161=CARTESIAN_POINT('Ctrl Pts',(128.831781411402,-31.0837832134984,21.8804459456757));
#22162=CARTESIAN_POINT('Ctrl Pts',(128.94717699838,-31.0530025681208,21.874635521428));
#22163=CARTESIAN_POINT('Ctrl Pts',(129.066940547023,-31.0210568116458,21.8686051606036));
#22164=CARTESIAN_POINT('Ctrl Pts',(129.188252361851,-30.9945421062579,21.8625747997792));
#22165=CARTESIAN_POINT('Ctrl Pts',(129.31057760758,-30.9735969197273,21.8565444389548));
#22166=CARTESIAN_POINT('Ctrl Pts',(129.428308799065,-30.9534383518746,21.8507405547222));
#22167=CARTESIAN_POINT('Ctrl Pts',(129.546978234582,-30.9384385838142,21.8449366704896));
#22168=CARTESIAN_POINT('Ctrl Pts',(129.666097575084,-30.928669238365,21.839132786257));
#22169=CARTESIAN_POINT('Ctrl Pts',(129.785199320386,-30.9189013359527,21.8333297593202));
#22170=CARTESIAN_POINT('Ctrl Pts',(129.904750431653,-30.9143623530833,21.8275267323834));
#22171=CARTESIAN_POINT('Ctrl Pts',(130.024257580144,-30.9150720239145,21.8217237054465));
#22172=CARTESIAN_POINT('Ctrl Pts',(130.143775279866,-30.9157817574023,21.8159201661631));
#22173=CARTESIAN_POINT('Ctrl Pts',(130.263248600744,-30.9217410635192,21.8101166268797));
#22174=CARTESIAN_POINT('Ctrl Pts',(130.382184990751,-30.9329175527358,21.8043130875963));
#22175=CARTESIAN_POINT('Ctrl Pts',(130.501159950442,-30.9440976663574,21.7985076662927));
#22176=CARTESIAN_POINT('Ctrl Pts',(130.619597226637,-30.9604982896458,21.7927022449892));
#22177=CARTESIAN_POINT('Ctrl Pts',(130.737010799371,-30.9820353309654,21.7868968236857));
#22178=CARTESIAN_POINT('Ctrl Pts',(130.854554396769,-31.0035962225649,21.7810849734154));
#22179=CARTESIAN_POINT('Ctrl Pts',(130.971071625956,-31.0303048124299,21.7752731231451));
#22180=CARTESIAN_POINT('Ctrl Pts',(131.086087894523,-31.0620261446564,21.7694612728749));
#22181=CARTESIAN_POINT('Ctrl Pts',(131.201179706394,-31.0937683116242,21.7636456053501));
#22182=CARTESIAN_POINT('Ctrl Pts',(131.314768206717,-31.1305296524004,21.7578299378254));
#22183=CARTESIAN_POINT('Ctrl Pts',(131.426396743237,-31.1721262650287,21.7520142703007));
#22184=CARTESIAN_POINT('Ctrl Pts',(131.538185175581,-31.213782460313,21.7461902724602));
#22185=CARTESIAN_POINT('Ctrl Pts',(131.648007665952,-31.2602875927179,21.7403662746197));
#22186=CARTESIAN_POINT('Ctrl Pts',(131.755430072907,-31.3114108036901,21.7345422767793));
#22187=CARTESIAN_POINT('Ctrl Pts',(131.783929823127,-31.3249740702793,21.7329971384004));
#22188=CARTESIAN_POINT('Ctrl Pts',(131.812260788292,-31.3388621474973,21.7314520000215));
#22189=CARTESIAN_POINT('Ctrl Pts',(131.84041519809,-31.353070209253,21.7299068616426));
#22190=CARTESIAN_POINT('Ctrl Pts',(131.946546836178,-31.4066293099055,21.7240822654817));
#22191=CARTESIAN_POINT('Ctrl Pts',(132.050509721292,-31.4649115473487,21.7182576693207));
#22192=CARTESIAN_POINT('Ctrl Pts',(132.15185506879,-31.5277176435486,21.7124330731598));
#22193=CARTESIAN_POINT('Ctrl Pts',(132.253060538421,-31.5904370541431,21.706616516165));
#22194=CARTESIAN_POINT('Ctrl Pts',(132.351655314945,-31.6576676858431,21.7007999591702));
#22195=CARTESIAN_POINT('Ctrl Pts',(132.447213477537,-31.7291635327704,21.6949834021754));
#22196=CARTESIAN_POINT('Ctrl Pts',(132.460589040624,-31.7391710212468,21.6941692412192));
#22197=CARTESIAN_POINT('Ctrl Pts',(132.473905147975,-31.7492620018798,21.6933550802631));
#22198=CARTESIAN_POINT('Ctrl Pts',(132.487160670875,-31.7594357285724,21.6925409193069));
#22199=CARTESIAN_POINT('',(125.915000722565,-35.0024296824293,22.2396150286373));
#22200=CARTESIAN_POINT('Ctrl Pts',(125.915000722565,-35.0024296815665,22.2396150285955));
#22201=CARTESIAN_POINT('Ctrl Pts',(125.914929010373,-34.8818606921115,22.233766442302));
#22202=CARTESIAN_POINT('Ctrl Pts',(125.920199535175,-34.7612723331104,22.2279178560086));
#22203=CARTESIAN_POINT('Ctrl Pts',(125.930790852349,-34.6411658981193,22.2220692697151));
#22204=CARTESIAN_POINT('Ctrl Pts',(125.941383317302,-34.5210464472191,22.2162200496115));
#22205=CARTESIAN_POINT('Ctrl Pts',(125.957297687507,-34.4014094220477,22.210370829508));
#22206=CARTESIAN_POINT('Ctrl Pts',(125.978460616568,-34.282751097943,22.2045216094045));
#22207=CARTESIAN_POINT('Ctrl Pts',(125.999630529126,-34.164053618095,22.1986704591324));
#22208=CARTESIAN_POINT('Ctrl Pts',(126.026052377497,-34.0463358750143,22.1928193088603));
#22209=CARTESIAN_POINT('Ctrl Pts',(126.057601774298,-33.930083540654,22.1869681585883));
#22210=CARTESIAN_POINT('Ctrl Pts',(126.089190817938,-33.8136851167277,22.1811096554144));
#22211=CARTESIAN_POINT('Ctrl Pts',(126.125920177321,-33.6987561662663,22.1752511522405));
#22212=CARTESIAN_POINT('Ctrl Pts',(126.167615514837,-33.5857672900539,22.1693926490666));
#22213=CARTESIAN_POINT('Ctrl Pts',(126.209337132696,-33.4727071975717,22.1635304533102));
#22214=CARTESIAN_POINT('Ctrl Pts',(126.25603081164,-33.3615899841467,22.1576682575538));
#22215=CARTESIAN_POINT('Ctrl Pts',(126.307474687368,-33.2528646830963,22.1518060617975));
#22216=CARTESIAN_POINT('Ctrl Pts',(126.359011363295,-33.1439432512265,22.1459332911588));
#22217=CARTESIAN_POINT('Ctrl Pts',(126.415315175187,-33.0374227087894,22.1400605205202));
#22218=CARTESIAN_POINT('Ctrl Pts',(126.476118646657,-32.9337267345384,22.1341877498816));
#22219=CARTESIAN_POINT('Ctrl Pts',(126.536050842734,-32.8315166581898,22.1283991323418));
#22220=CARTESIAN_POINT('Ctrl Pts',(126.600354320998,-32.7320509915407,22.1226105148021));
#22221=CARTESIAN_POINT('Ctrl Pts',(126.668734188096,-32.635704525564,22.1168218972623));
#22222=CARTESIAN_POINT('Ctrl Pts',(126.73752722176,-32.5387759125289,22.110998303591));
#22223=CARTESIAN_POINT('Ctrl Pts',(126.81066514483,-32.4446959552825,22.1051747099196));
#22224=CARTESIAN_POINT('Ctrl Pts',(126.887884046831,-32.3538784430739,22.0993511162483));
#22225=CARTESIAN_POINT('Ctrl Pts',(126.965005525716,-32.2631755106467,22.0935348699054));
#22226=CARTESIAN_POINT('Ctrl Pts',(127.046197480592,-32.1757271448576,22.0877186235624));
#22227=CARTESIAN_POINT('Ctrl Pts',(127.131153127975,-32.091917706654,22.0819023772195));
#22228=CARTESIAN_POINT('Ctrl Pts',(127.216023734286,-32.0081921621603,22.0760919529713));
#22229=CARTESIAN_POINT('Ctrl Pts',(127.304650249154,-31.928098583899,22.0702815287231));
#22230=CARTESIAN_POINT('Ctrl Pts',(127.396686480553,-31.8519873381029,22.0644711044748));
#22231=CARTESIAN_POINT('Ctrl Pts',(127.492206473676,-31.7729951242263,22.0584407436506));
#22232=CARTESIAN_POINT('Ctrl Pts',(127.591399122868,-31.6982930200788,22.0524103828264));
#22233=CARTESIAN_POINT('Ctrl Pts',(127.693836109116,-31.6282299739775,22.0463800220022));
#22234=CARTESIAN_POINT('Ctrl Pts',(127.792425965794,-31.5607982198177,22.0405761377691));
#22235=CARTESIAN_POINT('Ctrl Pts',(127.894020497765,-31.4976636093088,22.0347722535359));
#22236=CARTESIAN_POINT('Ctrl Pts',(127.998205759725,-31.4390949437533,22.0289683693028));
#22237=CARTESIAN_POINT('Ctrl Pts',(128.102375632409,-31.380534929416,22.0231653423654));
#22238=CARTESIAN_POINT('Ctrl Pts',(128.209135118203,-31.3265397188316,22.0173623154281));
#22239=CARTESIAN_POINT('Ctrl Pts',(128.318044091939,-31.2773330362037,22.0115592884907));
#22240=CARTESIAN_POINT('Ctrl Pts',(128.426962681199,-31.2281220091405,22.0057557492068));
#22241=CARTESIAN_POINT('Ctrl Pts',(128.538030763587,-31.1837005187533,21.9999522099228));
#22242=CARTESIAN_POINT('Ctrl Pts',(128.650787176772,-31.1442445931261,21.9941486706389));
#22243=CARTESIAN_POINT('Ctrl Pts',(128.763580155547,-31.1047758724024,21.9883432493348));
#22244=CARTESIAN_POINT('Ctrl Pts',(128.87806216876,-31.0702760537098,21.9825378280308));
#22245=CARTESIAN_POINT('Ctrl Pts',(128.993756423474,-31.0408714513545,21.9767324067267));
#22246=CARTESIAN_POINT('Ctrl Pts',(129.109578798866,-31.0114342861237,21.9709205564559));
#22247=CARTESIAN_POINT('Ctrl Pts',(129.226615699404,-30.9871037007483,21.9651087061851));
#22248=CARTESIAN_POINT('Ctrl Pts',(129.344379500266,-30.9679550150911,21.9592968559143));
#22249=CARTESIAN_POINT('Ctrl Pts',(129.462220649026,-30.9487937524743,21.953481188389));
#22250=CARTESIAN_POINT('Ctrl Pts',(129.580789244328,-30.9348212154102,21.9476655208637));
#22251=CARTESIAN_POINT('Ctrl Pts',(129.699593548547,-30.926060755985,21.9418498533384));
#22252=CARTESIAN_POINT('Ctrl Pts',(129.818568027102,-30.9172877481478,21.9360258554974));
#22253=CARTESIAN_POINT('Ctrl Pts',(129.937778481752,-30.9137417312552,21.9302018576564));
#22254=CARTESIAN_POINT('Ctrl Pts',(130.05673404596,-30.9153939910893,21.9243778598154));
#22255=CARTESIAN_POINT('Ctrl Pts',(130.088293605571,-30.9158323446298,21.9228327214416));
#22256=CARTESIAN_POINT('Ctrl Pts',(130.119835259209,-30.91663630686,21.9212875830677));
#22257=CARTESIAN_POINT('Ctrl Pts',(130.151349931726,-30.9178047329695,21.9197424446939));
#22258=CARTESIAN_POINT('Ctrl Pts',(130.27011093384,-30.9222078710817,21.9139196908137));
#22259=CARTESIAN_POINT('Ctrl Pts',(130.388871112727,-30.9318049791032,21.9080969369335));
#22260=CARTESIAN_POINT('Ctrl Pts',(130.507139933393,-30.9466021552334,21.9022741830532));
#22261=CARTESIAN_POINT('Ctrl Pts',(130.625268256982,-30.9613817531045,21.8964583462953));
#22262=CARTESIAN_POINT('Ctrl Pts',(130.742905981611,-30.9813490860618,21.8906425095373));
#22263=CARTESIAN_POINT('Ctrl Pts',(130.859563574337,-31.006458280965,21.8848266727793));
#22264=CARTESIAN_POINT('Ctrl Pts',(130.97611012843,-31.0315435760891,21.8790163717311));
#22265=CARTESIAN_POINT('Ctrl Pts',(131.091678009264,-31.0617609139633,21.8732060706829));
#22266=CARTESIAN_POINT('Ctrl Pts',(131.205784439581,-31.0970128253781,21.8673957696346));
#22267=CARTESIAN_POINT('Ctrl Pts',(131.321068739188,-31.1326286263979,21.8615254914655));
#22268=CARTESIAN_POINT('Ctrl Pts',(131.434860824508,-31.1733834844684,21.8556552132963));
#22269=CARTESIAN_POINT('Ctrl Pts',(131.546674675407,-31.2191241162327,21.8497849351272));
#22270=CARTESIAN_POINT('Ctrl Pts',(131.65721808492,-31.2643450378611,21.8439813557102));
#22271=CARTESIAN_POINT('Ctrl Pts',(131.765827598369,-31.3144388528637,21.8381777762933));
#22272=CARTESIAN_POINT('Ctrl Pts',(131.872050994275,-31.3692080650586,21.8323741968764));
#22273=CARTESIAN_POINT('Ctrl Pts',(131.980105579379,-31.4249214458048,21.8264705693311));
#22274=CARTESIAN_POINT('Ctrl Pts',(132.085690609827,-31.4854727630239,21.8205669417858));
#22275=CARTESIAN_POINT('Ctrl Pts',(132.188354523964,-31.5506044765137,21.8146633142406));
#22276=CARTESIAN_POINT('Ctrl Pts',(132.2910184381,-31.6157361900034,21.8087596866953));
#22277=CARTESIAN_POINT('Ctrl Pts',(132.390760863858,-31.6854480558678,21.80285605915));
#22278=CARTESIAN_POINT('Ctrl Pts',(132.487160670875,-31.7594357285724,21.7969524316048));
#22279=CARTESIAN_POINT('Ctrl Pts',(132.487160670875,-31.7594357285724,23.0467792200739));
#22280=CARTESIAN_POINT('Ctrl Pts',(132.583414813671,-31.8333116027474,23.0408775737182));
#22281=CARTESIAN_POINT('Ctrl Pts',(132.676442847798,-31.9115320435499,23.0349759273624));
#22282=CARTESIAN_POINT('Ctrl Pts',(132.765836767039,-31.9937777896347,23.0290742810067));
#22283=CARTESIAN_POINT('Ctrl Pts',(132.853746479267,-32.0746580098064,23.0232706196704));
#22284=CARTESIAN_POINT('Ctrl Pts',(132.938141520463,-32.1594306027935,23.0174669583341));
#22285=CARTESIAN_POINT('Ctrl Pts',(133.018667701034,-32.2477517715999,23.0116632969978));
#22286=CARTESIAN_POINT('Ctrl Pts',(133.099184936904,-32.3360631298518,23.0058602803216));
#22287=CARTESIAN_POINT('Ctrl Pts',(133.175833891759,-32.4279219783005,23.0000572636454));
#22288=CARTESIAN_POINT('Ctrl Pts',(133.248298528059,-32.522948996769,22.9942542469692));
#22289=CARTESIAN_POINT('Ctrl Pts',(133.320772216772,-32.6179878861828,22.9884505053698));
#22290=CARTESIAN_POINT('Ctrl Pts',(133.389060299958,-32.7161954078661,22.9826467637704));
#22291=CARTESIAN_POINT('Ctrl Pts',(133.452888584027,-32.8171611543005,22.976843022171));
#22292=CARTESIAN_POINT('Ctrl Pts',(133.51860336843,-32.9211110310011,22.9708677459514));
#22293=CARTESIAN_POINT('Ctrl Pts',(133.579590374359,-33.0279843254672,22.9648924697318));
#22294=CARTESIAN_POINT('Ctrl Pts',(133.635600506457,-33.1373046525406,22.9589171935123));
#22295=CARTESIAN_POINT('Ctrl Pts',(133.690084466923,-33.2436462046002,22.9531047324249));
#22296=CARTESIAN_POINT('Ctrl Pts',(133.739859151942,-33.3523027579522,22.9472922713375));
#22297=CARTESIAN_POINT('Ctrl Pts',(133.784744129264,-33.4628152759022,22.9414798102501));
#22298=CARTESIAN_POINT('Ctrl Pts',(133.831515042701,-33.5779712082205,22.9354231264644));
#22299=CARTESIAN_POINT('Ctrl Pts',(133.872976211536,-33.6951419989656,22.9293664426788));
#22300=CARTESIAN_POINT('Ctrl Pts',(133.908981331102,-33.8137917749825,22.9233097588931));
#22301=CARTESIAN_POINT('Ctrl Pts',(133.944986450668,-33.9324415509994,22.9172530751074));
#22302=CARTESIAN_POINT('Ctrl Pts',(133.975535465614,-34.0525698163222,22.9111963913218));
#22303=CARTESIAN_POINT('Ctrl Pts',(134.00054240192,-34.1736311414126,22.9051397075361));
#22304=CARTESIAN_POINT('Ctrl Pts',(134.024586951902,-34.2900334486165,22.8993161138646));
#22305=CARTESIAN_POINT('Ctrl Pts',(134.043585686199,-34.4076737573641,22.8934925201931));
#22306=CARTESIAN_POINT('Ctrl Pts',(134.057415670364,-34.5260769283036,22.8876689265217));
#22307=CARTESIAN_POINT('Ctrl Pts',(134.071228205949,-34.6443307160558,22.8818526801786));
#22308=CARTESIAN_POINT('Ctrl Pts',(134.079884914853,-34.7633450496769,22.8760364338356));
#22309=CARTESIAN_POINT('Ctrl Pts',(134.083313617438,-34.882633473061,22.8702201874926));
#22310=CARTESIAN_POINT('Ctrl Pts',(134.086738887873,-35.0018024880749,22.8644097632442));
#22311=CARTESIAN_POINT('Ctrl Pts',(134.084946551254,-35.1212446412136,22.8585993389959));
#22312=CARTESIAN_POINT('Ctrl Pts',(134.077916163162,-35.2404678070435,22.8527889147475));
#22313=CARTESIAN_POINT('Ctrl Pts',(134.070619660339,-35.3642038162958,22.8467585539234));
#22314=CARTESIAN_POINT('Ctrl Pts',(134.057680676829,-35.4877034872399,22.8407281930992));
#22315=CARTESIAN_POINT('Ctrl Pts',(134.039135779025,-35.6104155622194,22.834697832275));
#22316=CARTESIAN_POINT('Ctrl Pts',(134.021287354509,-35.7285190551891,22.8288939480418));
#22317=CARTESIAN_POINT('Ctrl Pts',(133.998246560815,-35.845892603303,22.8230900638086));
#22318=CARTESIAN_POINT('Ctrl Pts',(133.970098817708,-35.962050091022,22.8172861795753));
#22319=CARTESIAN_POINT('Ctrl Pts',(133.941955232323,-36.0781904210379,22.8114831526379));
#22320=CARTESIAN_POINT('Ctrl Pts',(133.90870629383,-36.1931146511323,22.8056801257004));
#22321=CARTESIAN_POINT('Ctrl Pts',(133.870488251105,-36.3063482300135,22.7998770987629));
#22322=CARTESIAN_POINT('Ctrl Pts',(133.832266834126,-36.4195918062359,22.7940735594788));
#22323=CARTESIAN_POINT('Ctrl Pts',(133.789075571221,-36.5311440475533,22.7882700201948));
#22324=CARTESIAN_POINT('Ctrl Pts',(133.74109995193,-36.6405475152117,22.7824664809107));
#22325=CARTESIAN_POINT('Ctrl Pts',(133.693108774706,-36.749986461139,22.7766610596065));
#22326=CARTESIAN_POINT('Ctrl Pts',(133.640330319394,-36.857274873817,22.7708556383023));
#22327=CARTESIAN_POINT('Ctrl Pts',(133.582997107867,-36.9619777585432,22.7650502169981));
#22328=CARTESIAN_POINT('Ctrl Pts',(133.525600405114,-37.0667965920228,22.7592383667271));
#22329=CARTESIAN_POINT('Ctrl Pts',(133.463639074183,-37.1690238239237,22.7534265164562));
#22330=CARTESIAN_POINT('Ctrl Pts',(133.397390335889,-37.2682512880201,22.7476146661853));
#22331=CARTESIAN_POINT('Ctrl Pts',(133.331098085069,-37.3675439252471,22.7417989986599));
#22332=CARTESIAN_POINT('Ctrl Pts',(133.260513059629,-37.4638325422687,22.7359833311345));
#22333=CARTESIAN_POINT('Ctrl Pts',(133.18595331224,-37.5567413815683,22.7301676636092));
#22334=CARTESIAN_POINT('Ctrl Pts',(133.111286766065,-37.649783302748,22.724343665768));
#22335=CARTESIAN_POINT('Ctrl Pts',(133.032634402642,-37.7394354776361,22.7185196679269));
#22336=CARTESIAN_POINT('Ctrl Pts',(132.950351781853,-37.8253582716739,22.7126956700858));
#22337=CARTESIAN_POINT('Ctrl Pts',(132.928521754051,-37.8481540572805,22.7111505317131));
#22338=CARTESIAN_POINT('Ctrl Pts',(132.906436386135,-37.8706875610478,22.7096053933404));
#22339=CARTESIAN_POINT('Ctrl Pts',(132.884102700967,-37.8929529222359,22.7080602549676));
#22340=CARTESIAN_POINT('Ctrl Pts',(132.799927516468,-37.9768705951102,22.7022366612962));
#22341=CARTESIAN_POINT('Ctrl Pts',(132.711950970825,-38.0572467206934,22.6964130676247));
#22342=CARTESIAN_POINT('Ctrl Pts',(132.620503068697,-38.1337180260751,22.6905894739533));
#22343=CARTESIAN_POINT('Ctrl Pts',(132.529170541681,-38.2100928515462,22.6847732276103));
#22344=CARTESIAN_POINT('Ctrl Pts',(132.434375679651,-38.2825723958932,22.6789569812673));
#22345=CARTESIAN_POINT('Ctrl Pts',(132.336485774208,-38.3508296326316,22.6731407349243));
#22346=CARTESIAN_POINT('Ctrl Pts',(132.238693857101,-38.4190185434996,22.667330310676));
#22347=CARTESIAN_POINT('Ctrl Pts',(132.137813393003,-38.4829933227504,22.6615198864277));
#22348=CARTESIAN_POINT('Ctrl Pts',(132.03424477454,-38.5424671060233,22.6557094621793));
#22349=CARTESIAN_POINT('Ctrl Pts',(131.926755869651,-38.6041920950062,22.6496791013552));
#22350=CARTESIAN_POINT('Ctrl Pts',(131.816371628909,-38.6610683239017,22.643648740531));
#22351=CARTESIAN_POINT('Ctrl Pts',(131.703573152674,-38.7128241964153,22.6376183797068));
#22352=CARTESIAN_POINT('Ctrl Pts',(131.595010942745,-38.7626363222924,22.6318144954736));
#22353=CARTESIAN_POINT('Ctrl Pts',(131.484212969969,-38.8077055712292,22.6260106112404));
#22354=CARTESIAN_POINT('Ctrl Pts',(131.371632631363,-38.8478369150188,22.6202067270071));
#22355=CARTESIAN_POINT('Ctrl Pts',(131.259068922076,-38.8879623309797,22.6144037000697));
#22356=CARTESIAN_POINT('Ctrl Pts',(131.144723755054,-38.9231511552312,22.6086006731322));
#22357=CARTESIAN_POINT('Ctrl Pts',(131.029068717973,-38.9532572106668,22.6027976461948));
#22358=CARTESIAN_POINT('Ctrl Pts',(130.913403469762,-38.9833659241523,22.5969941069107));
#22359=CARTESIAN_POINT('Ctrl Pts',(130.796428516745,-39.0083908737169,22.5911905676267));
#22360=CARTESIAN_POINT('Ctrl Pts',(130.678628126105,-39.0282364461956,22.5853870283426));
#22361=CARTESIAN_POINT('Ctrl Pts',(130.560789534173,-39.0480884543621,22.5795816070385));
#22362=CARTESIAN_POINT('Ctrl Pts',(130.442125374718,-39.0627576772734,22.5737761857343));
#22363=CARTESIAN_POINT('Ctrl Pts',(130.32312692478,-39.0722001412605,22.5679707644302));
#22364=CARTESIAN_POINT('Ctrl Pts',(130.203996695073,-39.0816530619025,22.5621589141593));
#22365=CARTESIAN_POINT('Ctrl Pts',(130.084531843238,-39.0858676376548,22.5563470638883));
#22366=CARTESIAN_POINT('Ctrl Pts',(129.965225710083,-39.0848519861509,22.5505352136174));
#22367=CARTESIAN_POINT('Ctrl Pts',(129.845841216019,-39.0838356675615,22.5447195460921));
#22368=CARTESIAN_POINT('Ctrl Pts',(129.726616055086,-39.0775823016849,22.5389038785667));
#22369=CARTESIAN_POINT('Ctrl Pts',(129.608038844918,-39.0661519220151,22.5330882110413));
#22370=CARTESIAN_POINT('Ctrl Pts',(129.489291785701,-39.0547051695606,22.5272642132002));
#22371=CARTESIAN_POINT('Ctrl Pts',(129.371194932633,-39.0380666591171,22.5214402153591));
#22372=CARTESIAN_POINT('Ctrl Pts',(129.254227251238,-39.016347595416,22.515616217518));
#22373=CARTESIAN_POINT('Ctrl Pts',(129.223195087791,-39.0105854094289,22.5140710791451));
#22374=CARTESIAN_POINT('Ctrl Pts',(129.192242321156,-39.0044658909861,22.5125259407721));
#22375=CARTESIAN_POINT('Ctrl Pts',(129.161377702765,-38.9979917011646,22.5109808023992));
#22376=CARTESIAN_POINT('Ctrl Pts',(129.045049612359,-38.9735906173953,22.5051572087276));
#22377=CARTESIAN_POINT('Ctrl Pts',(128.929599802197,-38.9440688376213,22.4993336150561));
#22378=CARTESIAN_POINT('Ctrl Pts',(128.815512999793,-38.9095032352386,22.4935100213846));
#22379=CARTESIAN_POINT('Ctrl Pts',(128.701570134837,-38.8749812424978,22.4876937750415));
#22380=CARTESIAN_POINT('Ctrl Pts',(128.588987244671,-38.8354282014207,22.4818775286984));
#22381=CARTESIAN_POINT('Ctrl Pts',(128.478239180689,-38.7909720400987,22.4760612823553));
#22382=CARTESIAN_POINT('Ctrl Pts',(128.36760197613,-38.7465603796394,22.4702508581068));
#22383=CARTESIAN_POINT('Ctrl Pts',(128.258796320694,-38.6972555141347,22.4644404338584));
#22384=CARTESIAN_POINT('Ctrl Pts',(128.152281620109,-38.6432350718299,22.45863000961));
#22385=CARTESIAN_POINT('Ctrl Pts',(128.041735117798,-38.5871698440516,22.4525996487858));
#22386=CARTESIAN_POINT('Ctrl Pts',(127.933656860859,-38.5260251272367,22.4465692879617));
#22387=CARTESIAN_POINT('Ctrl Pts',(127.82853772629,-38.4600544206492,22.4405389271376));
#22388=CARTESIAN_POINT('Ctrl Pts',(127.727366452209,-38.3965613138534,22.4347350429043));
#22389=CARTESIAN_POINT('Ctrl Pts',(127.62893641979,-38.3285984071376,22.4289311586709));
#22390=CARTESIAN_POINT('Ctrl Pts',(127.533659280727,-38.2564380013221,22.4231272744376));
#22391=CARTESIAN_POINT('Ctrl Pts',(127.438396215116,-38.1842882543705,22.4173242475001));
#22392=CARTESIAN_POINT('Ctrl Pts',(127.346285442124,-38.1079424878032,22.4115212205626));
#22393=CARTESIAN_POINT('Ctrl Pts',(127.257707727253,-38.027714994981,22.405718193625));
#22394=CARTESIAN_POINT('Ctrl Pts',(127.169122191896,-37.9474804189099,22.3999146543409));
#22395=CARTESIAN_POINT('Ctrl Pts',(127.084070637522,-37.8633637093151,22.3941111150568));
#22396=CARTESIAN_POINT('Ctrl Pts',(127.002898489856,-37.7757174816415,22.3883075757726));
#22397=CARTESIAN_POINT('Ctrl Pts',(126.921700019007,-37.6880428313175,22.3825021544683));
#22398=CARTESIAN_POINT('Ctrl Pts',(126.844383734154,-37.5968366860366,22.3766967331641));
#22399=CARTESIAN_POINT('Ctrl Pts',(126.771255713783,-37.5024858309735,22.3708913118598));
#22400=CARTESIAN_POINT('Ctrl Pts',(126.698046710899,-37.4080304910724,22.3650794615888));
#22401=CARTESIAN_POINT('Ctrl Pts',(126.629035480868,-37.3104238130077,22.3592676113178));
#22402=CARTESIAN_POINT('Ctrl Pts',(126.564485665799,-37.210082862587,22.3534557610468));
#22403=CARTESIAN_POINT('Ctrl Pts',(126.499893454065,-37.1096760076916,22.3476400935213));
#22404=CARTESIAN_POINT('Ctrl Pts',(126.439768698188,-37.0065316558561,22.3418244259959));
#22405=CARTESIAN_POINT('Ctrl Pts',(126.384329030278,-36.9010913809467,22.3360087584704));
#22406=CARTESIAN_POINT('Ctrl Pts',(126.32880995103,-36.795500074229,22.3301847606292));
#22407=CARTESIAN_POINT('Ctrl Pts',(126.277989527687,-36.6876066485449,22.324360762788));
#22408=CARTESIAN_POINT('Ctrl Pts',(126.232037303275,-36.5778726552195,22.3185367649468));
#22409=CARTESIAN_POINT('Ctrl Pts',(126.219845927668,-36.5487596286653,22.3169916265748));
#22410=CARTESIAN_POINT('Ctrl Pts',(126.207996937055,-36.5195171306766,22.3154464882028));
#22411=CARTESIAN_POINT('Ctrl Pts',(126.196492903007,-36.4901539394042,22.3139013498308));
#22412=CARTESIAN_POINT('Ctrl Pts',(126.147593400051,-36.3653415951119,22.307333523443));
#22413=CARTESIAN_POINT('Ctrl Pts',(126.104798671117,-36.2380114730377,22.3007656970552));
#22414=CARTESIAN_POINT('Ctrl Pts',(126.068343047717,-36.1087373943196,22.2941978706675));
#22415=CARTESIAN_POINT('Ctrl Pts',(126.03200196934,-35.9798694999168,22.2876506806524));
#22416=CARTESIAN_POINT('Ctrl Pts',(126.001960341602,-35.8490700312458,22.2811034906373));
#22417=CARTESIAN_POINT('Ctrl Pts',(125.978403669589,-35.7169295329545,22.2745563006222));
#22418=CARTESIAN_POINT('Ctrl Pts',(125.954985042458,-35.5855633935992,22.2680474779143));
#22419=CARTESIAN_POINT('Ctrl Pts',(125.937975683309,-35.4528720958563,22.2615386552065));
#22420=CARTESIAN_POINT('Ctrl Pts',(125.927510148756,-35.319454866162,22.2550298324986));
#22421=CARTESIAN_POINT('Ctrl Pts',(125.919248328881,-35.2141311376499,22.2498915645449));
#22422=CARTESIAN_POINT('Ctrl Pts',(125.915063725241,-35.1083554127925,22.2447532965911));
#22423=CARTESIAN_POINT('Ctrl Pts',(125.915000722565,-35.0024296824293,22.2396150286373));
#22424=CARTESIAN_POINT('Origin',(130.,-35.,32.7603849714045));
#22425=CARTESIAN_POINT('',(132.487160670875,-31.7594357285724,24.2969444293292));
#22426=CARTESIAN_POINT('',(132.487160670875,-31.7594357285724,24.1926561452238));
#22427=CARTESIAN_POINT('',(132.487160670875,-31.7594357285724,32.7603849714045));
#22428=CARTESIAN_POINT('',(125.915000507333,-34.997964094252,23.3853849713659));
#22429=CARTESIAN_POINT('Ctrl Pts',(132.487160670875,-31.7594357285724,24.1926561452238));
#22430=CARTESIAN_POINT('Ctrl Pts',(132.581972317179,-31.8322044744069,24.186852936304));
#22431=CARTESIAN_POINT('Ctrl Pts',(132.673586441412,-31.9091366288103,24.1810497273843));
#22432=CARTESIAN_POINT('Ctrl Pts',(132.761628074101,-31.989911067703,24.1752465184646));
#22433=CARTESIAN_POINT('Ctrl Pts',(132.84969112169,-32.0707051538523,24.1694418979952));
#22434=CARTESIAN_POINT('Ctrl Pts',(132.93417964885,-32.1553431070645,24.1636372775258));
#22435=CARTESIAN_POINT('Ctrl Pts',(133.014754835976,-32.2434662565174,24.1578326570563));
#22436=CARTESIAN_POINT('Ctrl Pts',(133.095416138222,-32.3316835880113,24.1520218328708));
#22437=CARTESIAN_POINT('Ctrl Pts',(133.172155473104,-32.4233932517347,24.1462110086852));
#22438=CARTESIAN_POINT('Ctrl Pts',(133.244673563067,-32.5182025729052,24.1404001844997));
#22439=CARTESIAN_POINT('Ctrl Pts',(133.317234011662,-32.613067273267,24.1345859661463));
#22440=CARTESIAN_POINT('Ctrl Pts',(133.385568070478,-32.711034903007,24.128771747793));
#22441=CARTESIAN_POINT('Ctrl Pts',(133.449420121027,-32.81168424841,24.1229575294397));
#22442=CARTESIAN_POINT('Ctrl Pts',(133.513369618591,-32.9124871985645,24.117134437789));
#22443=CARTESIAN_POINT('Ctrl Pts',(133.572823243656,-33.0159796845002,24.1113113461384));
#22444=CARTESIAN_POINT('Ctrl Pts',(133.627571421346,-33.1217160536719,24.1054882544877));
#22445=CARTESIAN_POINT('Ctrl Pts',(133.660879131881,-33.1860439733586,24.1019456004798));
#22446=CARTESIAN_POINT('Ctrl Pts',(133.692446162948,-33.2512019997072,24.0984029464718));
#22447=CARTESIAN_POINT('Ctrl Pts',(133.722234217902,-33.3170866252006,24.0948602924639));
#22448=CARTESIAN_POINT('Ctrl Pts',(133.771201327851,-33.425391101791,24.0890366987924));
#22449=CARTESIAN_POINT('Ctrl Pts',(133.81551653434,-33.5360091682225,24.083213105121));
#22450=CARTESIAN_POINT('Ctrl Pts',(133.854955774648,-33.6485041711093,24.0773895114495));
#22451=CARTESIAN_POINT('Ctrl Pts',(133.894345256496,-33.7608572448401,24.0715732651064));
#22452=CARTESIAN_POINT('Ctrl Pts',(133.928870873956,-33.875082163117,24.0657570187634));
#22453=CARTESIAN_POINT('Ctrl Pts',(133.958355605774,-33.9907201090709,24.0599407724204));
#22454=CARTESIAN_POINT('Ctrl Pts',(133.987810823214,-34.1062423008031,24.054130348172));
#22455=CARTESIAN_POINT('Ctrl Pts',(134.012235093006,-34.223174312939,24.0483199239236));
#22456=CARTESIAN_POINT('Ctrl Pts',(134.03150062945,-34.341040460466,24.0425094996753));
#22457=CARTESIAN_POINT('Ctrl Pts',(134.051495406297,-34.4633680854653,24.0364791388511));
#22458=CARTESIAN_POINT('Ctrl Pts',(134.065933047646,-34.5867015380635,24.030448778027));
#22459=CARTESIAN_POINT('Ctrl Pts',(134.074728435545,-34.7104949455294,24.0244184172028));
#22460=CARTESIAN_POINT('Ctrl Pts',(134.08319350333,-34.8296391603986,24.0186145329696));
#22461=CARTESIAN_POINT('Ctrl Pts',(134.086432445026,-34.9492089610494,24.0128106487363));
#22462=CARTESIAN_POINT('Ctrl Pts',(134.084422083151,-35.0687113285592,24.007006764503));
#22463=CARTESIAN_POINT('Ctrl Pts',(134.082412018227,-35.1881960442914,24.0012037375656));
#22464=CARTESIAN_POINT('Ctrl Pts',(134.075154198583,-35.3076129385223,23.9954007106281));
#22465=CARTESIAN_POINT('Ctrl Pts',(134.062677574554,-35.4264691374727,23.9895976836906));
#22466=CARTESIAN_POINT('Ctrl Pts',(134.050199848969,-35.5453358301824,23.9837941444065));
#22467=CARTESIAN_POINT('Ctrl Pts',(134.032502445518,-35.6636413230609,23.9779906051225));
#22468=CARTESIAN_POINT('Ctrl Pts',(134.009666108294,-35.7808986489905,23.9721870658384));
#22469=CARTESIAN_POINT('Ctrl Pts',(133.986822365513,-35.898194000104,23.9663816445342));
#22470=CARTESIAN_POINT('Ctrl Pts',(133.958836452693,-36.0144401076672,23.96057622323));
#22471=CARTESIAN_POINT('Ctrl Pts',(133.925839921304,-36.1291615970682,23.9547708019258));
#22472=CARTESIAN_POINT('Ctrl Pts',(133.892806849311,-36.2440101298999,23.9489589516549));
#22473=CARTESIAN_POINT('Ctrl Pts',(133.854752195815,-36.3573302817714,23.9431471013839));
#22474=CARTESIAN_POINT('Ctrl Pts',(133.811857003735,-36.4686630597519,23.937335251113));
#22475=CARTESIAN_POINT('Ctrl Pts',(133.768933637861,-36.5800689616986,23.9315195835876));
#22476=CARTESIAN_POINT('Ctrl Pts',(133.721163564773,-36.6894845168158,23.9257039160622));
#22477=CARTESIAN_POINT('Ctrl Pts',(133.668774768512,-36.7964734058513,23.9198882485368));
#22478=CARTESIAN_POINT('Ctrl Pts',(133.616310930957,-36.9036155449176,23.9140642506957));
#22479=CARTESIAN_POINT('Ctrl Pts',(133.559215360202,-37.0083237228902,23.9082402528545));
#22480=CARTESIAN_POINT('Ctrl Pts',(133.497760551461,-37.1101886466956,23.9024162550134));
#22481=CARTESIAN_POINT('Ctrl Pts',(133.481456255725,-37.1372139662253,23.9008711166408));
#22482=CARTESIAN_POINT('Ctrl Pts',(133.464845352462,-37.1640393303555,23.8993259782681));
#22483=CARTESIAN_POINT('Ctrl Pts',(133.447933409605,-37.1906574818822,23.8977808398955));
#22484=CARTESIAN_POINT('Ctrl Pts',(133.384192656586,-37.2909807289924,23.891957246224));
#22485=CARTESIAN_POINT('Ctrl Pts',(133.315966879741,-37.3886814839588,23.8861336525526));
#22486=CARTESIAN_POINT('Ctrl Pts',(133.243498460342,-37.4833329897058,23.8803100588811));
#22487=CARTESIAN_POINT('Ctrl Pts',(133.171121470617,-37.577865078519,23.8744938125381));
#22488=CARTESIAN_POINT('Ctrl Pts',(133.094512730825,-37.6693552485036,23.8686775661951));
#22489=CARTESIAN_POINT('Ctrl Pts',(133.013958945554,-37.7574039374957,23.8628613198521));
#22490=CARTESIAN_POINT('Ctrl Pts',(132.933485795066,-37.8453644892642,23.8570508956037));
#22491=CARTESIAN_POINT('Ctrl Pts',(132.849075729214,-37.9298901137807,23.8512404713554));
#22492=CARTESIAN_POINT('Ctrl Pts',(132.761056549752,-38.0106131815746,23.845430047107));
#22493=CARTESIAN_POINT('Ctrl Pts',(132.669705662293,-38.0943917844485,23.8393996862829));
#22494=CARTESIAN_POINT('Ctrl Pts',(132.574467310381,-38.1740739175952,23.8333693254587));
#22495=CARTESIAN_POINT('Ctrl Pts',(132.475751387658,-38.249289163265,23.8273389646345));
#22496=CARTESIAN_POINT('Ctrl Pts',(132.380742846018,-38.3216796206806,23.8215350804013));
#22497=CARTESIAN_POINT('Ctrl Pts',(132.28251358474,-38.3899323876553,23.815731196168));
#22498=CARTESIAN_POINT('Ctrl Pts',(132.181463245574,-38.4537578241979,23.8099273119348));
#22499=CARTESIAN_POINT('Ctrl Pts',(132.080427832625,-38.517573833041,23.8041242849973));
#22500=CARTESIAN_POINT('Ctrl Pts',(131.976572515624,-38.5769635939797,23.7983212580599));
#22501=CARTESIAN_POINT('Ctrl Pts',(131.870325389499,-38.6316811447861,23.7925182311224));
#22502=CARTESIAN_POINT('Ctrl Pts',(131.764068882864,-38.68640352658,23.7867146918383));
#22503=CARTESIAN_POINT('Ctrl Pts',(131.655420510286,-38.7364526911104,23.7809111525543));
#22504=CARTESIAN_POINT('Ctrl Pts',(131.544831817982,-38.7816292327712,23.7751076132702));
#22505=CARTESIAN_POINT('Ctrl Pts',(131.434207263055,-38.8268204246576,23.7693021919661));
#22506=CARTESIAN_POINT('Ctrl Pts',(131.321641514837,-38.8671356968009,23.7634967706619));
#22507=CARTESIAN_POINT('Ctrl Pts',(131.207604274662,-38.9024244920072,23.7576913493577));
#22508=CARTESIAN_POINT('Ctrl Pts',(131.093440748798,-38.9377523662879,23.7518794990868));
#22509=CARTESIAN_POINT('Ctrl Pts',(130.977802868591,-38.9680425319206,23.7460676488159));
#22510=CARTESIAN_POINT('Ctrl Pts',(130.861173763618,-38.9931948047717,23.7402557985449));
#22511=CARTESIAN_POINT('Ctrl Pts',(130.744468056023,-39.0183635977706,23.7344401310196));
#22512=CARTESIAN_POINT('Ctrl Pts',(130.626770228723,-39.0383877090663,23.7286244634942));
#22513=CARTESIAN_POINT('Ctrl Pts',(130.508570179099,-39.0532186436129,23.7228087959689));
#22514=CARTESIAN_POINT('Ctrl Pts',(130.390200820667,-39.0680708218719,23.7169847981277));
#22515=CARTESIAN_POINT('Ctrl Pts',(130.271328209625,-39.0777149433084,23.7111608002866));
#22516=CARTESIAN_POINT('Ctrl Pts',(130.152444038842,-39.0821545555039,23.7053368024455));
#22517=CARTESIAN_POINT('Ctrl Pts',(130.120903420318,-39.0833324088189,23.7037916640727));
#22518=CARTESIAN_POINT('Ctrl Pts',(130.089361967641,-39.0841442161781,23.7022465256999));
#22519=CARTESIAN_POINT('Ctrl Pts',(130.057828802667,-39.084590656306,23.7007013873271));
#22520=CARTESIAN_POINT('Ctrl Pts',(129.938980974395,-39.0862732796548,23.6948777936556));
#22521=CARTESIAN_POINT('Ctrl Pts',(129.81986799618,-39.0827672038154,23.6890541999842));
#22522=CARTESIAN_POINT('Ctrl Pts',(129.70097965991,-39.0740412168033,23.6832306063127));
#22523=CARTESIAN_POINT('Ctrl Pts',(129.582241318934,-39.06532623892,23.6774143599697));
#22524=CARTESIAN_POINT('Ctrl Pts',(129.463727459842,-39.05140447828,23.6715981136266));
#22525=CARTESIAN_POINT('Ctrl Pts',(129.345929425908,-39.0322967009022,23.6657818672836));
#22526=CARTESIAN_POINT('Ctrl Pts',(129.228249308457,-39.0132080505151,23.6599714430352));
#22527=CARTESIAN_POINT('Ctrl Pts',(129.111283991439,-38.9889437757074,23.6541610187869));
#22528=CARTESIAN_POINT('Ctrl Pts',(128.995520638518,-38.9595765193207,23.6483505945385));
#22529=CARTESIAN_POINT('Ctrl Pts',(128.875375403249,-38.929097651538,23.6423202337143));
#22530=CARTESIAN_POINT('Ctrl Pts',(128.75652537064,-38.8931218851609,23.6362898728902));
#22531=CARTESIAN_POINT('Ctrl Pts',(128.639505036172,-38.8517889938831,23.630259512066));
#22532=CARTESIAN_POINT('Ctrl Pts',(128.526879524368,-38.8120084031364,23.6244556278328));
#22533=CARTESIAN_POINT('Ctrl Pts',(128.415949176261,-38.7672659642247,23.6186517435995));
#22534=CARTESIAN_POINT('Ctrl Pts',(128.307175307434,-38.7177371558837,23.6128478593663));
#22535=CARTESIAN_POINT('Ctrl Pts',(128.19841750567,-38.6682156634772,23.6070448324288));
#22536=CARTESIAN_POINT('Ctrl Pts',(128.091815921246,-38.6139093768061,23.6012418054913));
#22537=CARTESIAN_POINT('Ctrl Pts',(127.987810935918,-38.5550415145804,23.5954387785538));
#22538=CARTESIAN_POINT('Ctrl Pts',(127.883796768038,-38.4961684549381,23.5896352392697));
#22539=CARTESIAN_POINT('Ctrl Pts',(127.782380010442,-38.4327332201464,23.5838316999857));
#22540=CARTESIAN_POINT('Ctrl Pts',(127.683974961418,-38.3650041635426,23.5780281607016));
#22541=CARTESIAN_POINT('Ctrl Pts',(127.585538000782,-38.2972531431953,23.5722227393974));
#22542=CARTESIAN_POINT('Ctrl Pts',(127.490115027271,-38.2252057631852,23.5664173180931));
#22543=CARTESIAN_POINT('Ctrl Pts',(127.398089435739,-38.1491723381845,23.5606118967889));
#22544=CARTESIAN_POINT('Ctrl Pts',(127.305961934383,-38.0730547132036,23.554800046518));
#22545=CARTESIAN_POINT('Ctrl Pts',(127.217239639829,-37.9929424924006,23.548988196247));
#22546=CARTESIAN_POINT('Ctrl Pts',(127.132271177233,-37.90918483412,23.5431763459761));
#22547=CARTESIAN_POINT('Ctrl Pts',(127.047246906896,-37.8253721633599,23.5373606784507));
#22548=CARTESIAN_POINT('Ctrl Pts',(126.965981656001,-37.7379095851817,23.5315450109253));
#22549=CARTESIAN_POINT('Ctrl Pts',(126.888784528308,-37.6471802524019,23.5257293433999));
#22550=CARTESIAN_POINT('Ctrl Pts',(126.811476824066,-37.5563209596498,23.5199053455588));
#22551=CARTESIAN_POINT('Ctrl Pts',(126.738249123523,-37.4621858938798,23.5140813477176));
#22552=CARTESIAN_POINT('Ctrl Pts',(126.669367987707,-37.3651882374751,23.5082573498765));
#22553=CARTESIAN_POINT('Ctrl Pts',(126.651093446919,-37.3394542305172,23.5067122115038));
#22554=CARTESIAN_POINT('Ctrl Pts',(126.633124599154,-37.3135188728382,23.5051670731312));
#22555=CARTESIAN_POINT('Ctrl Pts',(126.615465877015,-37.287390165746,23.5036219347586));
#22556=CARTESIAN_POINT('Ctrl Pts',(126.547946051236,-37.1874845362868,23.4977139492936));
#22557=CARTESIAN_POINT('Ctrl Pts',(126.484750138235,-37.0844341712422,23.4918059638286));
#22558=CARTESIAN_POINT('Ctrl Pts',(126.426178854133,-36.9786428220761,23.4858979783636));
#22559=CARTESIAN_POINT('Ctrl Pts',(126.367686936567,-36.8729948246073,23.4799979984658));
#22560=CARTESIAN_POINT('Ctrl Pts',(126.313807367995,-36.7646135732641,23.4740980185679));
#22561=CARTESIAN_POINT('Ctrl Pts',(126.264798248164,-36.6539325479227,23.46819803867));
#22562=CARTESIAN_POINT('Ctrl Pts',(126.215845205528,-36.5433781659803,23.4623048096448));
#22563=CARTESIAN_POINT('Ctrl Pts',(126.171751679283,-36.4305296035708,23.4564115806196));
#22564=CARTESIAN_POINT('Ctrl Pts',(126.132730166999,-36.3158453703833,23.4505183515944));
#22565=CARTESIAN_POINT('Ctrl Pts',(126.093751609521,-36.2012873813831,23.4446316098245));
#22566=CARTESIAN_POINT('Ctrl Pts',(126.059834070597,-36.0848981168303,23.4387448680547));
#22567=CARTESIAN_POINT('Ctrl Pts',(126.031141913439,-35.9671558761317,23.4328581262849));
#22568=CARTESIAN_POINT('Ctrl Pts',(126.002468405445,-35.849490164864,23.4269752107459));
#22569=CARTESIAN_POINT('Ctrl Pts',(125.979013612725,-35.7304736079775,23.4210922952069));
#22570=CARTESIAN_POINT('Ctrl Pts',(125.960892007609,-35.6105993987934,23.415209379668));
#22571=CARTESIAN_POINT('Ctrl Pts',(125.942777952188,-35.4907751307492,23.4093289150274));
#22572=CARTESIAN_POINT('Ctrl Pts',(125.929992721259,-35.3700943092338,23.4034484503869));
#22573=CARTESIAN_POINT('Ctrl Pts',(125.922599567219,-35.2490596530117,23.3975679857463));
#22574=CARTESIAN_POINT('Ctrl Pts',(125.917493910484,-35.1654740271159,23.3935069809657));
#22575=CARTESIAN_POINT('Ctrl Pts',(125.914958764663,-35.0817198648688,23.3894459761851));
#22576=CARTESIAN_POINT('Ctrl Pts',(125.915000507333,-34.9979640950484,23.3853849714045));
#22577=CARTESIAN_POINT('Ctrl Pts',(125.915000507333,-34.997964094252,23.3853849713659));
#22578=CARTESIAN_POINT('Ctrl Pts',(125.915068041878,-34.8624575358967,23.3788147639346));
#22579=CARTESIAN_POINT('Ctrl Pts',(125.921882638121,-34.7271788853975,23.3722445565033));
#22580=CARTESIAN_POINT('Ctrl Pts',(125.935349060719,-34.5927681964749,23.365674349072));
#22581=CARTESIAN_POINT('Ctrl Pts',(125.948524496332,-34.461261898893,23.359246112891));
#22582=CARTESIAN_POINT('Ctrl Pts',(125.968067066152,-34.3305866411253,23.3528178767101));
#22583=CARTESIAN_POINT('Ctrl Pts',(125.993836675524,-34.2013258376368,23.3463896405291));
#22584=CARTESIAN_POINT('Ctrl Pts',(126.020459989605,-34.0677828366577,23.3397484474726));
#22585=CARTESIAN_POINT('Ctrl Pts',(126.053729887508,-33.9357499211089,23.3331072544161));
#22586=CARTESIAN_POINT('Ctrl Pts',(126.093437848864,-33.8058487703357,23.3264660613596));
#22587=CARTESIAN_POINT('Ctrl Pts',(126.133145810219,-33.6759476195625,23.3198248683031));
#22588=CARTESIAN_POINT('Ctrl Pts',(126.179291657194,-33.5481784751308,23.3131836752467));
#22589=CARTESIAN_POINT('Ctrl Pts',(126.231614536202,-33.4231372931558,23.3065424821902));
#22590=CARTESIAN_POINT('Ctrl Pts',(126.277495928968,-33.3134899707806,23.3007188885187));
#22591=CARTESIAN_POINT('Ctrl Pts',(126.328240832554,-33.2056699869784,23.2948952948472));
#22592=CARTESIAN_POINT('Ctrl Pts',(126.38368242305,-33.1001389043826,23.2890717011758));
#22593=CARTESIAN_POINT('Ctrl Pts',(126.439054065743,-32.9947409649228,23.2832554548327));
#22594=CARTESIAN_POINT('Ctrl Pts',(126.499110421294,-32.8916265412262,23.2774392084897));
#22595=CARTESIAN_POINT('Ctrl Pts',(126.563636386211,-32.791237877492,23.2716229621467));
#22596=CARTESIAN_POINT('Ctrl Pts',(126.628097760281,-32.6909497033638,23.2658125378984));
#22597=CARTESIAN_POINT('Ctrl Pts',(126.697019623524,-32.5933822027085,23.26000211365));
#22598=CARTESIAN_POINT('Ctrl Pts',(126.770140972508,-32.4989530867004,23.2541916894017));
#22599=CARTESIAN_POINT('Ctrl Pts',(126.846030115791,-32.4009496333386,23.2481613285775));
#22600=CARTESIAN_POINT('Ctrl Pts',(126.926442736365,-32.3063272444975,23.2421309677533));
#22601=CARTESIAN_POINT('Ctrl Pts',(127.0110373891,-32.2155202441672,23.2361006069292));
#22602=CARTESIAN_POINT('Ctrl Pts',(127.09245500001,-32.1281235969596,23.2302967226959));
#22603=CARTESIAN_POINT('Ctrl Pts',(127.177745883189,-32.0442612501205,23.2244928384627));
#22604=CARTESIAN_POINT('Ctrl Pts',(127.26656505548,-31.9642861788243,23.2186889542295));
#22605=CARTESIAN_POINT('Ctrl Pts',(127.355371108229,-31.8843229207015,23.212885927292));
#22606=CARTESIAN_POINT('Ctrl Pts',(127.447704110287,-31.8082460693953,23.2070829003545));
#22607=CARTESIAN_POINT('Ctrl Pts',(127.54318365727,-31.7363703552494,23.2012798734171));
#22608=CARTESIAN_POINT('Ctrl Pts',(127.638671634099,-31.6644882952296,23.195476334133));
#22609=CARTESIAN_POINT('Ctrl Pts',(127.737306381951,-31.5968083554373,23.1896727948489));
#22610=CARTESIAN_POINT('Ctrl Pts',(127.838676519037,-31.5336033391087,23.1838692555648));
#22611=CARTESIAN_POINT('Ctrl Pts',(127.940079529277,-31.4703778261305,23.1780638342607));
#22612=CARTESIAN_POINT('Ctrl Pts',(128.044219346579,-31.4116303385915,23.1722584129565));
#22613=CARTESIAN_POINT('Ctrl Pts',(128.150658444779,-31.3575885992749,23.1664529916523));
#22614=CARTESIAN_POINT('Ctrl Pts',(128.257215414428,-31.3034870137343,23.1606411413814));
#22615=CARTESIAN_POINT('Ctrl Pts',(128.366076383178,-31.2541017633487,23.1548292911105));
#22616=CARTESIAN_POINT('Ctrl Pts',(128.476782081958,-31.2096131893757,23.1490174408395));
#22617=CARTESIAN_POINT('Ctrl Pts',(128.587560492835,-31.1650953950685,23.1432017733142));
#22618=CARTESIAN_POINT('Ctrl Pts',(128.700185662413,-31.1254808174235,23.1373861057888));
#22619=CARTESIAN_POINT('Ctrl Pts',(128.814182921209,-31.0908999941613,23.1315704382634));
#22620=CARTESIAN_POINT('Ctrl Pts',(128.92834346877,-31.0562696376038,23.1257464404223));
#22621=CARTESIAN_POINT('Ctrl Pts',(129.043879634147,-31.0266875277395,23.1199224425811));
#22622=CARTESIAN_POINT('Ctrl Pts',(129.160306188627,-31.0022332105109,23.11409844474));
#22623=CARTESIAN_POINT('Ctrl Pts',(129.19119478815,-30.9957453468543,23.1125533063673));
#22624=CARTESIAN_POINT('Ctrl Pts',(129.222146031755,-30.9896181299174,23.1110081679945));
#22625=CARTESIAN_POINT('Ctrl Pts',(129.253150813995,-30.9838524313263,23.1094630296218));
#22626=CARTESIAN_POINT('Ctrl Pts',(129.370019603658,-30.962119325424,23.1036388167605));
#22627=CARTESIAN_POINT('Ctrl Pts',(129.488026301746,-30.9454566790275,23.0978146038993));
#22628=CARTESIAN_POINT('Ctrl Pts',(129.606693270705,-30.9339780107959,23.0919903910381));
#22629=CARTESIAN_POINT('Ctrl Pts',(129.725207575952,-30.922514109741,23.0861736709608));
#22630=CARTESIAN_POINT('Ctrl Pts',(129.844380059347,-30.9162209598086,23.0803569508835));
#22631=CARTESIAN_POINT('Ctrl Pts',(129.963722808182,-30.9151610845281,23.0745402308062));
#22632=CARTESIAN_POINT('Ctrl Pts',(130.082924450892,-30.9141024624019,23.0687303881876));
#22633=CARTESIAN_POINT('Ctrl Pts',(130.202295552223,-30.9182647994427,23.062920545569));
#22634=CARTESIAN_POINT('Ctrl Pts',(130.321343825436,-30.9276587635791,23.0571107029504));
#22635=CARTESIAN_POINT('Ctrl Pts',(130.440313011485,-30.9370464870371,23.0513047199759));
#22636=CARTESIAN_POINT('Ctrl Pts',(130.558959390375,-30.9516588939429,23.0454987370015));
#22637=CARTESIAN_POINT('Ctrl Pts',(130.676791649195,-30.9714545970562,23.0396927540271));
#22638=CARTESIAN_POINT('Ctrl Pts',(130.794573438416,-30.9912418213266,23.0338892578558));
#22639=CARTESIAN_POINT('Ctrl Pts',(130.911541399294,-31.0162078577871,23.0280857616846));
#22640=CARTESIAN_POINT('Ctrl Pts',(131.027210946426,-31.0462596605818,23.0222822655134));
#22641=CARTESIAN_POINT('Ctrl Pts',(131.142858248281,-31.0763056838893,23.016479885456));
#22642=CARTESIAN_POINT('Ctrl Pts',(131.257207238655,-31.1114354235755,23.0106775053986));
#22643=CARTESIAN_POINT('Ctrl Pts',(131.369785731835,-31.1515052229657,23.0048751253412));
#22644=CARTESIAN_POINT('Ctrl Pts',(131.482409236857,-31.1915910433152,22.9990704253397));
#22645=CARTESIAN_POINT('Ctrl Pts',(131.593260444397,-31.2366207354387,22.9932657253382));
#22646=CARTESIAN_POINT('Ctrl Pts',(131.701884602897,-31.2864015027977,22.9874610253367));
#22647=CARTESIAN_POINT('Ctrl Pts',(131.810531700828,-31.3361927829424,22.9816550994889));
#22648=CARTESIAN_POINT('Ctrl Pts',(131.916950446232,-31.3907369569506,22.9758491736412));
#22649=CARTESIAN_POINT('Ctrl Pts',(132.020709414005,-31.4497945884568,22.9700432477934));
#22650=CARTESIAN_POINT('Ctrl Pts',(132.124565043882,-31.5089072381948,22.9642319131312));
#22651=CARTESIAN_POINT('Ctrl Pts',(132.225755598332,-31.5725415309082,22.958420578469));
#22652=CARTESIAN_POINT('Ctrl Pts',(132.323877385357,-31.6404138799805,22.9526092438067));
#22653=CARTESIAN_POINT('Ctrl Pts',(132.379306579903,-31.678755106278,22.9493264091853));
#22654=CARTESIAN_POINT('Ctrl Pts',(132.433757040346,-31.7184479874236,22.9460435745638));
#22655=CARTESIAN_POINT('Ctrl Pts',(132.487160670875,-31.7594357285724,22.9427607399423));
#22656=CARTESIAN_POINT('',(125.915000083441,-35.0008256610612,23.4896150285496));
#22657=CARTESIAN_POINT('Ctrl Pts',(125.915000083441,-35.0008256610612,23.4896150285496));
#22658=CARTESIAN_POINT('Ctrl Pts',(125.914976188112,-34.8826023086113,23.4838237303786));
#22659=CARTESIAN_POINT('Ctrl Pts',(125.920088782344,-34.7641789032467,23.4780324322077));
#22660=CARTESIAN_POINT('Ctrl Pts',(125.930363891994,-34.6460410356922,23.4722411340368));
#22661=CARTESIAN_POINT('Ctrl Pts',(125.940626165892,-34.5280507469398,23.4664570704035));
#22662=CARTESIAN_POINT('Ctrl Pts',(125.956038095578,-34.4103456948175,23.4606730067702));
#22663=CARTESIAN_POINT('Ctrl Pts',(125.976573711133,-34.2934124979475,23.454888943137));
#22664=CARTESIAN_POINT('Ctrl Pts',(125.997089184842,-34.1765939920917,23.4491105526584));
#22665=CARTESIAN_POINT('Ctrl Pts',(126.022718277938,-34.0605462405633,23.4433321621799));
#22666=CARTESIAN_POINT('Ctrl Pts',(126.053383190379,-33.9457510929488,23.4375537717014));
#22667=CARTESIAN_POINT('Ctrl Pts',(126.0840271413,-33.8310344155049,23.4317793311397));
#22668=CARTESIAN_POINT('Ctrl Pts',(126.119699958342,-33.7175690369885,23.4260048905781));
#22669=CARTESIAN_POINT('Ctrl Pts',(126.160272822346,-33.6058263375076,23.4202304500164));
#22670=CARTESIAN_POINT('Ctrl Pts',(126.200831076437,-33.4941238755415,23.4144580887775));
#22671=CARTESIAN_POINT('Ctrl Pts',(126.246285729108,-33.3841432475703,23.4086857275386));
#22672=CARTESIAN_POINT('Ctrl Pts',(126.296458370552,-33.276339824981,23.4029133662996));
#22673=CARTESIAN_POINT('Ctrl Pts',(126.346625133143,-33.1685490339875,23.3971416814227));
#22674=CARTESIAN_POINT('Ctrl Pts',(126.401508610812,-33.0629353158185,23.3913699965457));
#22675=CARTESIAN_POINT('Ctrl Pts',(126.46088288993,-32.9599325792491,23.3855983116687));
#22676=CARTESIAN_POINT('Ctrl Pts',(126.520264635338,-32.8569168901294,23.3798259010049));
#22677=CARTESIAN_POINT('Ctrl Pts',(126.584138098127,-32.7565131933276,23.374053490341));
#22678=CARTESIAN_POINT('Ctrl Pts',(126.652232561365,-32.6591287568908,23.3682810796771));
#22679=CARTESIAN_POINT('Ctrl Pts',(126.720394941295,-32.5616471902553,23.3625029116723));
#22680=CARTESIAN_POINT('Ctrl Pts',(126.792786493865,-32.4671912387105,23.3567247436676));
#22681=CARTESIAN_POINT('Ctrl Pts',(126.869094375303,-32.3761373951285,23.3509465756629));
#22682=CARTESIAN_POINT('Ctrl Pts',(126.945439758011,-32.2850388034211,23.3451655679956));
#22683=CARTESIAN_POINT('Ctrl Pts',(127.025705024388,-32.1973459552064,23.3393845603283));
#22684=CARTESIAN_POINT('Ctrl Pts',(127.109539652373,-32.1133992346024,23.3336035526611));
#22685=CARTESIAN_POINT('Ctrl Pts',(127.193510877075,-32.0293157346422,23.3278131256562));
#22686=CARTESIAN_POINT('Ctrl Pts',(127.281062779314,-31.9489908384644,23.3220226986513));
#22687=CARTESIAN_POINT('Ctrl Pts',(127.37181044764,-31.872725679307,23.3162322716463));
#22688=CARTESIAN_POINT('Ctrl Pts',(127.460271975996,-31.7983818128054,23.3105877186552));
#22689=CARTESIAN_POINT('Ctrl Pts',(127.551769842018,-31.7278957223704,23.3049431656641));
#22690=CARTESIAN_POINT('Ctrl Pts',(127.645922334693,-31.6615058266181,23.299298612673));
#22691=CARTESIAN_POINT('Ctrl Pts',(127.743061268699,-31.5930100967773,23.2934750190015));
#22692=CARTESIAN_POINT('Ctrl Pts',(127.8433488203,-31.5286470550448,23.28765142533));
#22693=CARTESIAN_POINT('Ctrl Pts',(127.946398371878,-31.4687190209535,23.2818278316586));
#22694=CARTESIAN_POINT('Ctrl Pts',(128.04931791114,-31.4088665949787,23.2760115853155));
#22695=CARTESIAN_POINT('Ctrl Pts',(128.154992169571,-31.3534382509531,23.2701953389725));
#22696=CARTESIAN_POINT('Ctrl Pts',(128.263003899946,-31.3026942852399,23.2643790926294));
#22697=CARTESIAN_POINT('Ctrl Pts',(128.370907509983,-31.2520011145162,23.2585686683811));
#22698=CARTESIAN_POINT('Ctrl Pts',(128.481143569719,-31.2059831663763,23.2527582441327));
#22699=CARTESIAN_POINT('Ctrl Pts',(128.593268989437,-31.1648555615309,23.2469478198844));
#22700=CARTESIAN_POINT('Ctrl Pts',(128.709638588206,-31.1221711917759,23.2409174590602));
#22701=CARTESIAN_POINT('Ctrl Pts',(128.828043017953,-31.0847549248083,23.234887098236));
#22702=CARTESIAN_POINT('Ctrl Pts',(128.947962219258,-31.0527932017828,23.2288567374119));
#22703=CARTESIAN_POINT('Ctrl Pts',(129.063377727884,-31.0220318351343,23.2230528531786));
#22704=CARTESIAN_POINT('Ctrl Pts',(129.180195852158,-30.9963228131408,23.2172489689454));
#22705=CARTESIAN_POINT('Ctrl Pts',(129.297936769714,-30.9757817876413,23.2114450847121));
#22706=CARTESIAN_POINT('Ctrl Pts',(129.415660295676,-30.9552437962709,23.2056420577747));
#22707=CARTESIAN_POINT('Ctrl Pts',(129.534305941696,-30.9398723534553,23.1998390308372));
#22708=CARTESIAN_POINT('Ctrl Pts',(129.653384206572,-30.9297318894517,23.1940360038997));
#22709=CARTESIAN_POINT('Ctrl Pts',(129.772472984814,-30.9195905301512,23.1882324646156));
#22710=CARTESIAN_POINT('Ctrl Pts',(129.891994050969,-30.914681102563,23.1824289253315));
#22711=CARTESIAN_POINT('Ctrl Pts',(130.011453946277,-30.9150160579123,23.1766253860475));
#22712=CARTESIAN_POINT('Ctrl Pts',(130.130952581035,-30.9153511218836,23.1708199647433));
#22713=CARTESIAN_POINT('Ctrl Pts',(130.250389597369,-30.9209339499411,23.1650145434391));
#22714=CARTESIAN_POINT('Ctrl Pts',(130.369273348815,-30.9317249117279,23.1592091221349));
#22715=CARTESIAN_POINT('Ctrl Pts',(130.488288753011,-30.9425278235061,23.153397271864));
#22716=CARTESIAN_POINT('Ctrl Pts',(130.606749262431,-30.9585503445551,23.147585421593));
#22717=CARTESIAN_POINT('Ctrl Pts',(130.724169994246,-30.9797011529696,23.1417735713221));
#22718=CARTESIAN_POINT('Ctrl Pts',(130.841667848627,-31.0008658533486,23.1359579037967));
#22719=CARTESIAN_POINT('Ctrl Pts',(130.958124167937,-31.0271654593772,23.1301422362714));
#22720=CARTESIAN_POINT('Ctrl Pts',(131.073067492797,-31.0584582767776,23.124326568746));
#22721=CARTESIAN_POINT('Ctrl Pts',(131.188175461558,-31.08979591776,23.1185025709048));
#22722=CARTESIAN_POINT('Ctrl Pts',(131.30176572272,-31.1261409215911,23.1126785730637));
#22723=CARTESIAN_POINT('Ctrl Pts',(131.41338497273,-31.1673027880015,23.1068545752225));
#22724=CARTESIAN_POINT('Ctrl Pts',(131.442998168172,-31.1782232555251,23.1053094368499));
#22725=CARTESIAN_POINT('Ctrl Pts',(131.472472757079,-31.1894825129043,23.1037642984772));
#22726=CARTESIAN_POINT('Ctrl Pts',(131.501800563169,-31.2010764592501,23.1022191601045));
#22727=CARTESIAN_POINT('Ctrl Pts',(131.612327895284,-31.2447704182979,23.0963960166496));
#22728=CARTESIAN_POINT('Ctrl Pts',(131.721124991535,-31.2933624212854,23.0905728731948));
#22729=CARTESIAN_POINT('Ctrl Pts',(131.827727178127,-31.3466948714436,23.0847497297399));
#22730=CARTESIAN_POINT('Ctrl Pts',(131.934210987089,-31.3999680979665,23.078933052662));
#22731=CARTESIAN_POINT('Ctrl Pts',(132.038504368934,-31.4579711278646,23.0731163755841));
#22732=CARTESIAN_POINT('Ctrl Pts',(132.140160799607,-31.5204976287083,23.0672996985061));
#22733=CARTESIAN_POINT('Ctrl Pts',(132.241707615468,-31.5829567080364,23.0614892934757));
#22734=CARTESIAN_POINT('Ctrl Pts',(132.340622792912,-31.6499293386126,23.0556788884453));
#22735=CARTESIAN_POINT('Ctrl Pts',(132.43648352961,-31.7211628570575,23.0498684834149));
#22736=CARTESIAN_POINT('Ctrl Pts',(132.453472538016,-31.7337872837555,23.0488387289679));
#22737=CARTESIAN_POINT('Ctrl Pts',(132.470365674088,-31.7465454255331,23.0478089745209));
#22738=CARTESIAN_POINT('Ctrl Pts',(132.487160670875,-31.7594357285724,23.0467792200739));
#22739=CARTESIAN_POINT('Ctrl Pts',(132.487160670875,-31.7594357285724,24.2969444293292));
#22740=CARTESIAN_POINT('Ctrl Pts',(132.553405700193,-31.8102793526328,24.2928615780578));
#22741=CARTESIAN_POINT('Ctrl Pts',(132.618025634951,-31.8631049026459,24.2887787267865));
#22742=CARTESIAN_POINT('Ctrl Pts',(132.680900483629,-31.9177933883531,24.2846958755152));
#22743=CARTESIAN_POINT('Ctrl Pts',(132.770582312949,-31.9957985612347,24.2788722818436));
#22744=CARTESIAN_POINT('Ctrl Pts',(132.857001403455,-32.077846930771,24.2730486881721));
#22745=CARTESIAN_POINT('Ctrl Pts',(132.939771970637,-32.1636351150355,24.2672250945006));
#22746=CARTESIAN_POINT('Ctrl Pts',(133.022438110453,-32.2493150647627,24.2614088481575));
#22747=CARTESIAN_POINT('Ctrl Pts',(133.101464601485,-32.3387251532974,24.2555926018144));
#22748=CARTESIAN_POINT('Ctrl Pts',(133.176499167056,-32.4315222325874,24.2497763554713));
#22749=CARTESIAN_POINT('Ctrl Pts',(133.251458622613,-32.5242264214889,24.2439659312229));
#22750=CARTESIAN_POINT('Ctrl Pts',(133.322433846866,-32.6203105406738,24.2381555069745));
#22751=CARTESIAN_POINT('Ctrl Pts',(133.389110273962,-32.7193955733341,24.232345082726));
#22752=CARTESIAN_POINT('Ctrl Pts',(133.458310541732,-32.8222311794219,24.2263147219019));
#22753=CARTESIAN_POINT('Ctrl Pts',(133.522879834287,-32.9282990467355,24.2202843610778));
#22754=CARTESIAN_POINT('Ctrl Pts',(133.58251308558,-33.0371385704409,24.2142540002536));
#22755=CARTESIAN_POINT('Ctrl Pts',(133.63990674693,-33.1418905105017,24.2084501160203));
#22756=CARTESIAN_POINT('Ctrl Pts',(133.692728223576,-33.2492092860081,24.202646231787));
#22757=CARTESIAN_POINT('Ctrl Pts',(133.740750791123,-33.3586564897268,24.1968423475537));
#22758=CARTESIAN_POINT('Ctrl Pts',(133.788766265222,-33.4680875269231,24.1910393206161));
#22759=CARTESIAN_POINT('Ctrl Pts',(133.831984075877,-33.5796459932815,24.1852362936786));
#22760=CARTESIAN_POINT('Ctrl Pts',(133.870224935108,-33.6928718686883,24.179433266741));
#22761=CARTESIAN_POINT('Ctrl Pts',(133.908469170607,-33.8061077407558,24.1736297274569));
#22762=CARTESIAN_POINT('Ctrl Pts',(133.941735450357,-33.9210109276833,24.1678261881727));
#22763=CARTESIAN_POINT('Ctrl Pts',(133.969894022572,-34.0371051721276,24.1620226488886));
#22764=CARTESIAN_POINT('Ctrl Pts',(133.998061726284,-34.1532370645816,24.1562172275843));
#22765=CARTESIAN_POINT('Ctrl Pts',(134.021118332114,-34.2705603860818,24.1504118062801));
#22766=CARTESIAN_POINT('Ctrl Pts',(134.038985099818,-34.3885882210449,24.1446063849758));
#22767=CARTESIAN_POINT('Ctrl Pts',(134.056871653315,-34.5067467609107,24.1387945347048));
#22768=CARTESIAN_POINT('Ctrl Pts',(134.069556835499,-34.6256109675757,24.1329826844338));
#22769=CARTESIAN_POINT('Ctrl Pts',(134.077013719479,-34.7446881687441,24.1271708341628));
#22770=CARTESIAN_POINT('Ctrl Pts',(134.084475501181,-34.8638435804575,24.1213551666374));
#22771=CARTESIAN_POINT('Ctrl Pts',(134.086702138233,-34.983211857953,24.1155394991119));
#22772=CARTESIAN_POINT('Ctrl Pts',(134.083718823924,-35.1023013544955,24.1097238315864));
#22773=CARTESIAN_POINT('Ctrl Pts',(134.080731236339,-35.2215614338824,24.1038998337452));
#22774=CARTESIAN_POINT('Ctrl Pts',(134.072518830281,-35.3405415293661,24.098075835904));
#22775=CARTESIAN_POINT('Ctrl Pts',(134.059158526398,-35.4587559891402,24.0922518380628));
#22776=CARTESIAN_POINT('Ctrl Pts',(134.055613964955,-35.4901189296677,24.0907066996908));
#22777=CARTESIAN_POINT('Ctrl Pts',(134.051707336022,-35.5214280420399,24.0891615613188));
#22778=CARTESIAN_POINT('Ctrl Pts',(134.047440672667,-35.5526744079872,24.0876164229467));
#22779=CARTESIAN_POINT('Ctrl Pts',(134.031359709197,-35.6704412968824,24.0817928292753));
#22780=CARTESIAN_POINT('Ctrl Pts',(134.010108618132,-35.7876956583175,24.0759692356038));
#22781=CARTESIAN_POINT('Ctrl Pts',(133.983729666343,-35.9039485303376,24.0701456419324));
#22782=CARTESIAN_POINT('Ctrl Pts',(133.95738399552,-36.0200547320917,24.0643293955894));
#22783=CARTESIAN_POINT('Ctrl Pts',(133.925923421333,-36.1351615628538,24.0585131492464));
#22784=CARTESIAN_POINT('Ctrl Pts',(133.88944183767,-36.2487862873119,24.0526969029033));
#22785=CARTESIAN_POINT('Ctrl Pts',(133.852996772274,-36.362297272794,24.046886478655));
#22786=CARTESIAN_POINT('Ctrl Pts',(133.811540820233,-36.4743287168497,24.0410760544067));
#22787=CARTESIAN_POINT('Ctrl Pts',(133.765218546725,-36.584409762467,24.0352656301584));
#22788=CARTESIAN_POINT('Ctrl Pts',(133.717142879353,-36.6986576033481,24.0292352693342));
#22789=CARTESIAN_POINT('Ctrl Pts',(133.663825310019,-36.8108040380569,24.02320490851));
#22790=CARTESIAN_POINT('Ctrl Pts',(133.605483849221,-36.9203414313629,24.0171745476859));
#22791=CARTESIAN_POINT('Ctrl Pts',(133.549333463805,-37.0257650317899,24.0113706634526));
#22792=CARTESIAN_POINT('Ctrl Pts',(133.488529946167,-37.128771634557,24.0055667792194));
#22793=CARTESIAN_POINT('Ctrl Pts',(133.423315685409,-37.2289312950451,23.9997628949862));
#22794=CARTESIAN_POINT('Ctrl Pts',(133.358111057496,-37.3290761608802,23.9939598680487));
#22795=CARTESIAN_POINT('Ctrl Pts',(133.288497204863,-37.4263745786227,23.9881568411113));
#22796=CARTESIAN_POINT('Ctrl Pts',(133.21476059592,-37.5204244307099,23.9823538141738));
#22797=CARTESIAN_POINT('Ctrl Pts',(133.141017476806,-37.6144825864156,23.9765502748897));
#22798=CARTESIAN_POINT('Ctrl Pts',(133.063151129624,-37.7052912848461,23.9707467356057));
#22799=CARTESIAN_POINT('Ctrl Pts',(132.981488757071,-37.7924809384234,23.9649431963216));
#22800=CARTESIAN_POINT('Ctrl Pts',(132.899799902363,-37.8796988665885,23.9591377750175));
#22801=CARTESIAN_POINT('Ctrl Pts',(132.814312853083,-37.9632951179704,23.9533323537133));
#22802=CARTESIAN_POINT('Ctrl Pts',(132.725391688841,-38.0429369271146,23.9475269324092));
#22803=CARTESIAN_POINT('Ctrl Pts',(132.63637205264,-38.1226669321908,23.9417150821382));
#22804=CARTESIAN_POINT('Ctrl Pts',(132.543911014788,-38.1984334812215,23.9359032318673));
#22805=CARTESIAN_POINT('Ctrl Pts',(132.448405871834,-38.2699439883226,23.9300913815964));
#22806=CARTESIAN_POINT('Ctrl Pts',(132.352838000591,-38.3415014639086,23.9242757140711));
#22807=CARTESIAN_POINT('Ctrl Pts',(132.254222378933,-38.4087971008361,23.9184600465457));
#22808=CARTESIAN_POINT('Ctrl Pts',(132.152984016047,-38.4715824672108,23.9126443790203));
#22809=CARTESIAN_POINT('Ctrl Pts',(132.051600640138,-38.5344577668432,23.9068203811792));
#22810=CARTESIAN_POINT('Ctrl Pts',(131.947587379506,-38.5928097020869,23.9009963833381));
#22811=CARTESIAN_POINT('Ctrl Pts',(131.841392584403,-38.6464363905196,23.895172385497));
#22812=CARTESIAN_POINT('Ctrl Pts',(131.813218526412,-38.660663843271,23.8936272471241));
#22813=CARTESIAN_POINT('Ctrl Pts',(131.784891016527,-38.674558966587,23.8920821087512));
#22814=CARTESIAN_POINT('Ctrl Pts',(131.756418628183,-38.6881185721951,23.8905369703783));
#22815=CARTESIAN_POINT('Ctrl Pts',(131.649106801957,-38.7392244373993,23.8847133767068));
#22816=CARTESIAN_POINT('Ctrl Pts',(131.539389563275,-38.7857252081775,23.8788897830354));
#22817=CARTESIAN_POINT('Ctrl Pts',(131.427699034966,-38.827388204188,23.8730661893639));
#22818=CARTESIAN_POINT('Ctrl Pts',(131.316149420849,-38.8689986361404,23.8672499430209));
#22819=CARTESIAN_POINT('Ctrl Pts',(131.202631848071,-38.9057832917305,23.8614336966779));
#22820=CARTESIAN_POINT('Ctrl Pts',(131.087601531726,-38.9375560831799,23.8556174503348));
#22821=CARTESIAN_POINT('Ctrl Pts',(130.972686361363,-38.9692970698898,23.8498070260865));
#22822=CARTESIAN_POINT('Ctrl Pts',(130.856261851211,-38.9960360648757,23.8439966018381));
#22823=CARTESIAN_POINT('Ctrl Pts',(130.738801057855,-39.0176358716181,23.8381861775898));
#22824=CARTESIAN_POINT('Ctrl Pts',(130.616894130519,-39.0400532757217,23.8321558167656));
#22825=CARTESIAN_POINT('Ctrl Pts',(130.493871338942,-39.0569345899523,23.8261254559415));
#22826=CARTESIAN_POINT('Ctrl Pts',(130.370276759998,-39.0681838848565,23.8200950951173));
#22827=CARTESIAN_POINT('Ctrl Pts',(130.251323906434,-39.0790107005699,23.8142912108841));
#22828=CARTESIAN_POINT('Ctrl Pts',(130.13184188237,-39.0846208606734,23.8084873266508));
#22829=CARTESIAN_POINT('Ctrl Pts',(130.012323149957,-39.0849814124394,23.8026834424176));
#22830=CARTESIAN_POINT('Ctrl Pts',(129.892822071738,-39.085341910948,23.7968804154801));
#22831=CARTESIAN_POINT('Ctrl Pts',(129.773284704179,-39.0804543419596,23.7910773885427));
#22832=CARTESIAN_POINT('Ctrl Pts',(129.654204398353,-39.0703378731847,23.7852743616052));
#22833=CARTESIAN_POINT('Ctrl Pts',(129.535113578981,-39.0602205112314,23.7794708223211));
#22834=CARTESIAN_POINT('Ctrl Pts',(129.416480308468,-39.044873366173,23.773667283037));
#22835=CARTESIAN_POINT('Ctrl Pts',(129.298793059799,-39.0243675064554,23.767863743753));
#22836=CARTESIAN_POINT('Ctrl Pts',(129.181067646528,-39.0038549969266,23.7620583224488));
#22837=CARTESIAN_POINT('Ctrl Pts',(129.064289267295,-38.9781805157527,23.7562529011446));
#22838=CARTESIAN_POINT('Ctrl Pts',(128.948935812706,-38.9474661587135,23.7504474798405));
#22839=CARTESIAN_POINT('Ctrl Pts',(128.833454614843,-38.9167177883667,23.7446356295695));
#22840=CARTESIAN_POINT('Ctrl Pts',(128.719401886215,-38.880918506736,23.7388237792986));
#22841=CARTESIAN_POINT('Ctrl Pts',(128.607240120711,-38.8402402162679,23.7330119290277));
#22842=CARTESIAN_POINT('Ctrl Pts',(128.495004686756,-38.7995352080802,23.7271962615023));
#22843=CARTESIAN_POINT('Ctrl Pts',(128.384663065915,-38.7539449646649,23.7213805939769));
#22844=CARTESIAN_POINT('Ctrl Pts',(128.276656014011,-38.7036887701256,23.7155649264515));
#22845=CARTESIAN_POINT('Ctrl Pts',(128.168494253667,-38.6533605890145,23.7097409286104));
#22846=CARTESIAN_POINT('Ctrl Pts',(128.062674097762,-38.5983533046016,23.7039169307692));
#22847=CARTESIAN_POINT('Ctrl Pts',(127.959610164208,-38.5389312395121,23.6980929329281));
#22848=CARTESIAN_POINT('Ctrl Pts',(127.932266740854,-38.5231662417456,23.6965477945554));
#22849=CARTESIAN_POINT('Ctrl Pts',(127.905117151511,-38.5070907303505,23.6950026561826));
#22850=CARTESIAN_POINT('Ctrl Pts',(127.878168762405,-38.4907101282068,23.6934575178099));
#22851=CARTESIAN_POINT('Ctrl Pts',(127.776600856886,-38.42897198704,23.6876339241384));
#22852=CARTESIAN_POINT('Ctrl Pts',(127.677565959971,-38.3626976832694,23.6818103304669));
#22853=CARTESIAN_POINT('Ctrl Pts',(127.581495552781,-38.2921210850732,23.6759867367955));
#22854=CARTESIAN_POINT('Ctrl Pts',(127.48554635268,-38.221633529739,23.6701704904524));
#22855=CARTESIAN_POINT('Ctrl Pts',(127.392554529426,-38.1468547157337,23.6643542441094));
#22856=CARTESIAN_POINT('Ctrl Pts',(127.302925253799,-38.0680633652851,23.6585379977664));
#22857=CARTESIAN_POINT('Ctrl Pts',(127.213385697572,-37.9893508854131,23.652727573518));
#22858=CARTESIAN_POINT('Ctrl Pts',(127.127202297796,-37.9066341276188,23.6469171492697));
#22859=CARTESIAN_POINT('Ctrl Pts',(127.04474911407,-37.8202335366442,23.6411067250213));
#22860=CARTESIAN_POINT('Ctrl Pts',(126.959174906799,-37.7305625045942,23.6350763641972));
#22861=CARTESIAN_POINT('Ctrl Pts',(126.877619249222,-37.6369235130641,23.629046003373));
#22862=CARTESIAN_POINT('Ctrl Pts',(126.800460617092,-37.5397190272199,23.6230156425488));
#22863=CARTESIAN_POINT('Ctrl Pts',(126.726199759155,-37.4461651588457,23.6172117583156));
#22864=CARTESIAN_POINT('Ctrl Pts',(126.656011889451,-37.3493091269353,23.6114078740823));
#22865=CARTESIAN_POINT('Ctrl Pts',(126.590194518506,-37.2495447491381,23.6056039898491));
#22866=CARTESIAN_POINT('Ctrl Pts',(126.524386869491,-37.1497951076065,23.5998009629116));
#22867=CARTESIAN_POINT('Ctrl Pts',(126.462948660205,-37.0471383152667,23.5939979359741));
#22868=CARTESIAN_POINT('Ctrl Pts',(126.406134296419,-36.9419975037632,23.5881949090366));
#22869=CARTESIAN_POINT('Ctrl Pts',(126.349314916518,-36.8368474094255,23.5823913697525));
#22870=CARTESIAN_POINT('Ctrl Pts',(126.297120387922,-36.7292132191378,23.5765878304684));
#22871=CARTESIAN_POINT('Ctrl Pts',(126.249759034134,-36.6195424347449,23.5707842911843));
#22872=CARTESIAN_POINT('Ctrl Pts',(126.202382321611,-36.5098360853956,23.5649788698802));
#22873=CARTESIAN_POINT('Ctrl Pts',(126.159842062791,-36.3980922031492,23.559173448576));
#22874=CARTESIAN_POINT('Ctrl Pts',(126.122298102512,-36.2847774103789,23.5533680272718));
#22875=CARTESIAN_POINT('Ctrl Pts',(126.084712565772,-36.171337131964,23.5475561770008));
#22876=CARTESIAN_POINT('Ctrl Pts',(126.052134500294,-36.0563228584039,23.5417443267299));
#22877=CARTESIAN_POINT('Ctrl Pts',(126.024673654136,-35.9402156369025,23.535932476459));
#22878=CARTESIAN_POINT('Ctrl Pts',(125.997194771546,-35.8240321555548,23.5301168089336));
#22879=CARTESIAN_POINT('Ctrl Pts',(125.97483987811,-35.7067546968341,23.5243011414082));
#22880=CARTESIAN_POINT('Ctrl Pts',(125.957667177219,-35.588872099752,23.5184854738828));
#22881=CARTESIAN_POINT('Ctrl Pts',(125.940469878288,-35.4708206485788,23.5126614760416));
#22882=CARTESIAN_POINT('Ctrl Pts',(125.92846962861,-35.3521627337903,23.5068374782005));
#22883=CARTESIAN_POINT('Ctrl Pts',(125.921672634806,-35.2333900218802,23.5010134803594));
#22884=CARTESIAN_POINT('Ctrl Pts',(125.919869355301,-35.2018789740052,23.4994683419867));
#22885=CARTESIAN_POINT('Ctrl Pts',(125.91843203318,-35.1703598310429,23.497923203614));
#22886=CARTESIAN_POINT('Ctrl Pts',(125.917360170799,-35.1388417265164,23.4963780652414));
#22887=CARTESIAN_POINT('Ctrl Pts',(125.915796331449,-35.0928570432683,23.4941237196927));
#22888=CARTESIAN_POINT('Ctrl Pts',(125.91500938505,-35.0468457909017,23.4918693741441));
#22889=CARTESIAN_POINT('Ctrl Pts',(125.915000083442,-35.0008256619992,23.4896150285955));
#22890=CARTESIAN_POINT('Origin',(130.,-35.,32.7603849714045));
#22891=CARTESIAN_POINT('',(132.487160670875,-31.7594357285724,25.5469383396565));
#22892=CARTESIAN_POINT('',(132.487160670875,-31.7594357285724,25.4425452647471));
#22893=CARTESIAN_POINT('',(132.487160670875,-31.7594357285724,32.7603849714045));
#22894=CARTESIAN_POINT('',(125.915001572211,-35.0035839873014,24.6353849714487));
#22895=CARTESIAN_POINT('Ctrl Pts',(132.487160670875,-31.7594357285724,25.4425452647471));
#22896=CARTESIAN_POINT('Ctrl Pts',(132.581714430403,-31.8320065441103,25.4367339326408));
#22897=CARTESIAN_POINT('Ctrl Pts',(132.673191712905,-31.9087977384192,25.4309226005346));
#22898=CARTESIAN_POINT('Ctrl Pts',(132.761197144929,-31.9895157653901,25.4251112684283));
#22899=CARTESIAN_POINT('Ctrl Pts',(132.849133405474,-32.070170348716,25.419304503977));
#22900=CARTESIAN_POINT('Ctrl Pts',(132.933602945501,-32.154745348426,25.4134977395256));
#22901=CARTESIAN_POINT('Ctrl Pts',(133.014243150667,-32.2429067428431,25.4076909750742));
#22902=CARTESIAN_POINT('Ctrl Pts',(133.094848361656,-32.3310298792302,25.4018867304942));
#22903=CARTESIAN_POINT('Ctrl Pts',(133.171627266642,-32.4227360152345,25.3960824859141));
#22904=CARTESIAN_POINT('Ctrl Pts',(133.244254186697,-32.5176543810142,25.3902782413341));
#22905=CARTESIAN_POINT('Ctrl Pts',(133.316866721276,-32.6125539459704,25.3844751464217));
#22906=CARTESIAN_POINT('Ctrl Pts',(133.385328658296,-32.7106641513093,25.3786720515093));
#22907=CARTESIAN_POINT('Ctrl Pts',(133.449355108616,-32.8115817733659,25.372868956597));
#22908=CARTESIAN_POINT('Ctrl Pts',(133.513383987267,-32.9125032229253,25.3670656415906));
#22909=CARTESIAN_POINT('Ctrl Pts',(133.572976826082,-33.0162319560225,25.3612623265843));
#22910=CARTESIAN_POINT('Ctrl Pts',(133.62789286766,-33.12233700021,25.3554590115779));
#22911=CARTESIAN_POINT('Ctrl Pts',(133.682823952171,-33.2284711093287,25.3496541068927));
#22912=CARTESIAN_POINT('Ctrl Pts',(133.73307550409,-33.336982461524,25.3438492022074));
#22913=CARTESIAN_POINT('Ctrl Pts',(133.778453683459,-33.4474173896512,25.3380442975221));
#22914=CARTESIAN_POINT('Ctrl Pts',(133.82388104049,-33.5579719993444,25.3322331018916));
#22915=CARTESIAN_POINT('Ctrl Pts',(133.864424325119,-33.6704539689137,25.3264219062611));
#22916=CARTESIAN_POINT('Ctrl Pts',(133.899938573092,-33.7843914585251,25.3206107106306));
#22917=CARTESIAN_POINT('Ctrl Pts',(133.935474542879,-33.8983986364736,25.3147959606603));
#22918=CARTESIAN_POINT('Ctrl Pts',(133.9659752453,-34.0138627134301,25.30898121069));
#22919=CARTESIAN_POINT('Ctrl Pts',(133.991346549699,-34.1303002125992,25.3031664607196));
#22920=CARTESIAN_POINT('Ctrl Pts',(134.016755656369,-34.2469111991799,25.2973430469947));
#22921=CARTESIAN_POINT('Ctrl Pts',(134.037020035604,-34.3644981023516,25.2915196332697));
#22922=CARTESIAN_POINT('Ctrl Pts',(134.05209720878,-34.4825705742856,25.2856962195447));
#22923=CARTESIAN_POINT('Ctrl Pts',(134.059311378333,-34.539066233128,25.2829098156547));
#22924=CARTESIAN_POINT('Ctrl Pts',(134.065338727097,-34.5956730301281,25.2801234117646));
#22925=CARTESIAN_POINT('Ctrl Pts',(134.07017882144,-34.6523372877341,25.2773370078746));
#22926=CARTESIAN_POINT('Ctrl Pts',(134.080294635191,-34.7707657801741,25.2715134142026));
#22927=CARTESIAN_POINT('Ctrl Pts',(134.085253665983,-34.8898271179956,25.2656898205305));
#22928=CARTESIAN_POINT('Ctrl Pts',(134.084990008492,-35.009034961019,25.2598662268584));
#22929=CARTESIAN_POINT('Ctrl Pts',(134.084726683644,-35.1280924056418,25.2540499805148));
#22930=CARTESIAN_POINT('Ctrl Pts',(134.079253777168,-35.2472955830911,25.2482337341712));
#22931=CARTESIAN_POINT('Ctrl Pts',(134.068557120453,-35.3661529156075,25.2424174878276));
#22932=CARTESIAN_POINT('Ctrl Pts',(134.057871171151,-35.4848912712785,25.2366070635786));
#22933=CARTESIAN_POINT('Ctrl Pts',(134.041971910454,-35.6032840663682,25.2307966393297));
#22934=CARTESIAN_POINT('Ctrl Pts',(134.020897212403,-35.7208402092625,25.2249862150807));
#22935=CARTESIAN_POINT('Ctrl Pts',(133.999024793444,-35.8428460952959,25.2189558542568));
#22936=CARTESIAN_POINT('Ctrl Pts',(133.971577394719,-35.9639502914226,25.2129254934329));
#22937=CARTESIAN_POINT('Ctrl Pts',(133.938656491478,-36.0836097277777,25.2068951326089));
#22938=CARTESIAN_POINT('Ctrl Pts',(133.90697196764,-36.1987752272179,25.2010912483751));
#22939=CARTESIAN_POINT('Ctrl Pts',(133.87021776973,-36.3126020997472,25.1952873641412));
#22940=CARTESIAN_POINT('Ctrl Pts',(133.828536183256,-36.4246177359195,25.1894834799073));
#22941=CARTESIAN_POINT('Ctrl Pts',(133.786860753598,-36.5366168261844,25.1836804529692));
#22942=CARTESIAN_POINT('Ctrl Pts',(133.740259525162,-36.6468048295454,25.1778774260311));
#22943=CARTESIAN_POINT('Ctrl Pts',(133.688923889136,-36.7547266283285,25.172074399093));
#22944=CARTESIAN_POINT('Ctrl Pts',(133.637583720709,-36.8626579554779,25.1662708598084));
#22945=CARTESIAN_POINT('Ctrl Pts',(133.581508489022,-36.9683223114745,25.1604673205237));
#22946=CARTESIAN_POINT('Ctrl Pts',(133.520936457764,-37.0712873920311,25.154663781239));
#22947=CARTESIAN_POINT('Ctrl Pts',(133.460344783703,-37.1742858629626,25.1488583599342));
#22948=CARTESIAN_POINT('Ctrl Pts',(133.395253616862,-37.2745829658215,25.1430529386293));
#22949=CARTESIAN_POINT('Ctrl Pts',(133.325945270333,-37.3717742427873,25.1372475173245));
#22950=CARTESIAN_POINT('Ctrl Pts',(133.256560171226,-37.4690731500963,25.131435667053));
#22951=CARTESIAN_POINT('Ctrl Pts',(133.182948807663,-37.5632590334871,25.1256238167814));
#22952=CARTESIAN_POINT('Ctrl Pts',(133.105434706826,-37.6539593594549,25.1198119665099));
#22953=CARTESIAN_POINT('Ctrl Pts',(133.027869694312,-37.7447192578837,25.1139962989839));
#22954=CARTESIAN_POINT('Ctrl Pts',(132.946397117582,-37.8319887418307,25.1081806314578));
#22955=CARTESIAN_POINT('Ctrl Pts',(132.861377218281,-37.9154322860769,25.1023649639318));
#22956=CARTESIAN_POINT('Ctrl Pts',(132.776235537155,-37.99899535419,25.0965409660901));
#22957=CARTESIAN_POINT('Ctrl Pts',(132.687536694358,-38.0787212723311,25.0907169682483));
#22958=CARTESIAN_POINT('Ctrl Pts',(132.595673905588,-38.1543148187598,25.0848929704065));
#22959=CARTESIAN_POINT('Ctrl Pts',(132.571302207098,-38.1743701985937,25.0833478320398));
#22960=CARTESIAN_POINT('Ctrl Pts',(132.546707963692,-38.194134951354,25.081802693673));
#22961=CARTESIAN_POINT('Ctrl Pts',(132.521898841803,-38.2136040875807,25.0802575553062));
#22962=CARTESIAN_POINT('Ctrl Pts',(132.428393788576,-38.286982848314,25.0744339616348));
#22963=CARTESIAN_POINT('Ctrl Pts',(132.331532681142,-38.3563955273654,25.0686103679635));
#22964=CARTESIAN_POINT('Ctrl Pts',(132.231686153495,-38.4215204094524,25.0627867742921));
#22965=CARTESIAN_POINT('Ctrl Pts',(132.131965597074,-38.486563126827,25.0569705279492));
#22966=CARTESIAN_POINT('Ctrl Pts',(132.029267451023,-38.547328585876,25.0511542816063));
#22967=CARTESIAN_POINT('Ctrl Pts',(131.92399509008,-38.6035354713597,25.0453380352634));
#22968=CARTESIAN_POINT('Ctrl Pts',(131.818828107351,-38.6596860934409,25.0395276110152));
#22969=CARTESIAN_POINT('Ctrl Pts',(131.711092394101,-38.711287028576,25.033717186767));
#22970=CARTESIAN_POINT('Ctrl Pts',(131.601219446355,-38.7581007549844,25.0279067625187));
#22971=CARTESIAN_POINT('Ctrl Pts',(131.487187580277,-38.8066864777663,25.0218764016945));
#22972=CARTESIAN_POINT('Ctrl Pts',(131.37085386077,-38.8501151747698,25.0158460408703));
#22973=CARTESIAN_POINT('Ctrl Pts',(131.252728120834,-38.8881740258469,25.0098156800461));
#22974=CARTESIAN_POINT('Ctrl Pts',(131.139038718239,-38.9248035364411,25.004011795813));
#22975=CARTESIAN_POINT('Ctrl Pts',(131.023689893896,-38.9564591314116,24.9982079115799));
#22976=CARTESIAN_POINT('Ctrl Pts',(130.907154920439,-38.983000746965,24.9924040273467));
#22977=CARTESIAN_POINT('Ctrl Pts',(130.790637160444,-39.0095384420378,24.9866010004094));
#22978=CARTESIAN_POINT('Ctrl Pts',(130.672933997801,-39.0309635692697,24.980797973472));
#22979=CARTESIAN_POINT('Ctrl Pts',(130.554530993478,-39.0471867237963,24.9749949465347));
#22980=CARTESIAN_POINT('Ctrl Pts',(130.436117535408,-39.0634113106577,24.9691914072507));
#22981=CARTESIAN_POINT('Ctrl Pts',(130.317004517384,-39.074432956221,24.9633878679668));
#22982=CARTESIAN_POINT('Ctrl Pts',(130.197684113715,-39.0802139638975,24.9575843286828));
#22983=CARTESIAN_POINT('Ctrl Pts',(130.078325015831,-39.0859968462875,24.9517789073787));
#22984=CARTESIAN_POINT('Ctrl Pts',(129.9587588062,-39.0865356911628,24.9459734860747));
#22985=CARTESIAN_POINT('Ctrl Pts',(129.839478515428,-39.0818449080031,24.9401680647706));
#22986=CARTESIAN_POINT('Ctrl Pts',(129.720066132774,-39.0771489302352,24.9343562144998));
#22987=CARTESIAN_POINT('Ctrl Pts',(129.60094070926,-39.067211780499,24.928544364229));
#22988=CARTESIAN_POINT('Ctrl Pts',(129.482591166976,-39.0520998382949,24.9227325139582));
#22989=CARTESIAN_POINT('Ctrl Pts',(129.364163892078,-39.0369779704859,24.9169168464329));
#22990=CARTESIAN_POINT('Ctrl Pts',(129.246513914762,-39.0166746106328,24.9111011789076));
#22991=CARTESIAN_POINT('Ctrl Pts',(129.130119329986,-38.9913071317472,24.9052855113824));
#22992=CARTESIAN_POINT('Ctrl Pts',(129.013558022536,-38.9659033166873,24.8994615135414));
#22993=CARTESIAN_POINT('Ctrl Pts',(128.898256090138,-38.935421008393,24.8936375157003));
#22994=CARTESIAN_POINT('Ctrl Pts',(128.784675994262,-38.900027251325,24.8878135178593));
#22995=CARTESIAN_POINT('Ctrl Pts',(128.7545425757,-38.8906370946432,24.8862683794854));
#22996=CARTESIAN_POINT('Ctrl Pts',(128.724530238221,-38.880901496636,24.8847232411116));
#22997=CARTESIAN_POINT('Ctrl Pts',(128.694647357324,-38.8708241342457,24.8831781027377));
#22998=CARTESIAN_POINT('Ctrl Pts',(128.582019414727,-38.832842769707,24.8773545090663));
#22999=CARTESIAN_POINT('Ctrl Pts',(128.470868921731,-38.7898804367451,24.8715309153949));
#23000=CARTESIAN_POINT('Ctrl Pts',(128.361668119773,-38.7420707703399,24.8657073217235));
#23001=CARTESIAN_POINT('Ctrl Pts',(128.252605090847,-38.6943214229304,24.8598910753806));
#23002=CARTESIAN_POINT('Ctrl Pts',(128.145487231185,-38.6417370682485,24.8540748290376));
#23003=CARTESIAN_POINT('Ctrl Pts',(128.040770940075,-38.584500870518,24.8482585826947));
#23004=CARTESIAN_POINT('Ctrl Pts',(127.93615947055,-38.5273219665372,24.8424481584464));
#23005=CARTESIAN_POINT('Ctrl Pts',(127.833945143398,-38.4655006777978,24.8366377341981));
#23006=CARTESIAN_POINT('Ctrl Pts',(127.734563145387,-38.3992676943364,24.8308273099498));
#23007=CARTESIAN_POINT('Ctrl Pts',(127.631419333192,-38.3305276554567,24.8247969491256));
#23008=CARTESIAN_POINT('Ctrl Pts',(127.531326916346,-38.257035519091,24.8187665883015));
#23009=CARTESIAN_POINT('Ctrl Pts',(127.434743363361,-38.1791010345973,24.8127362274773));
#23010=CARTESIAN_POINT('Ctrl Pts',(127.341787108056,-38.1040934622545,24.8069323432441));
#23011=CARTESIAN_POINT('Ctrl Pts',(127.252081257698,-38.0249714780642,24.8011284590109));
#23012=CARTESIAN_POINT('Ctrl Pts',(127.166002388424,-37.9420541357325,24.7953245747778));
#23013=CARTESIAN_POINT('Ctrl Pts',(127.079936233919,-37.8591490411788,24.7895215478404));
#23014=CARTESIAN_POINT('Ctrl Pts',(126.99749628908,-37.7724499865799,24.783718520903));
#23015=CARTESIAN_POINT('Ctrl Pts',(126.919023496393,-37.6823140726292,24.7779154939656));
#23016=CARTESIAN_POINT('Ctrl Pts',(126.84054377538,-37.59217020062,24.7721119546816));
#23017=CARTESIAN_POINT('Ctrl Pts',(126.766032171054,-37.4985891739393,24.7663084153976));
#23018=CARTESIAN_POINT('Ctrl Pts',(126.695790003784,-37.4019619690804,24.7605048761136));
#23019=CARTESIAN_POINT('Ctrl Pts',(126.625525057799,-37.3053034291459,24.7546994548095));
#23020=CARTESIAN_POINT('Ctrl Pts',(126.55953254236,-37.2055970765615,24.7488940335054));
#23021=CARTESIAN_POINT('Ctrl Pts',(126.498070667217,-37.1032631666515,24.7430886122013));
#23022=CARTESIAN_POINT('Ctrl Pts',(126.436540728735,-37.0008159314082,24.7372767619305));
#23023=CARTESIAN_POINT('Ctrl Pts',(126.379551655806,-36.8957356809368,24.7314649116596));
#23024=CARTESIAN_POINT('Ctrl Pts',(126.327315939811,-36.7884677223906,24.7256530613888));
#23025=CARTESIAN_POINT('Ctrl Pts',(126.275045915117,-36.6811293096734,24.7198373938634));
#23026=CARTESIAN_POINT('Ctrl Pts',(126.227535627083,-36.5716007010129,24.7140217263381));
#23027=CARTESIAN_POINT('Ctrl Pts',(126.184948982551,-36.4603461008479,24.7082060588128));
#23028=CARTESIAN_POINT('Ctrl Pts',(126.142301337249,-36.3489321404818,24.7023820609718));
#23029=CARTESIAN_POINT('Ctrl Pts',(126.104591540684,-36.2357876400545,24.6965580631307));
#23030=CARTESIAN_POINT('Ctrl Pts',(126.071933386223,-36.1213909566845,24.6907340652897));
#23031=CARTESIAN_POINT('Ctrl Pts',(126.063268999827,-36.0910408930177,24.6891889269162));
#23032=CARTESIAN_POINT('Ctrl Pts',(126.054959902828,-36.0606027397222,24.6876437885428));
#23033=CARTESIAN_POINT('Ctrl Pts',(126.047007611079,-36.0300855173897,24.6860986501693));
#23034=CARTESIAN_POINT('Ctrl Pts',(126.008453455647,-35.882132478141,24.6786075385628));
#23035=CARTESIAN_POINT('Ctrl Pts',(125.978189862158,-35.7319372299234,24.6711164269563));
#23036=CARTESIAN_POINT('Ctrl Pts',(125.956429349327,-35.5803114620726,24.6636253153498));
#23037=CARTESIAN_POINT('Ctrl Pts',(125.935075376487,-35.4315184371298,24.6562741561642));
#23038=CARTESIAN_POINT('Ctrl Pts',(125.921909712316,-35.2813476384019,24.6489229969786));
#23039=CARTESIAN_POINT('Ctrl Pts',(125.917087813763,-35.1305874399659,24.6415718377929));
#23040=CARTESIAN_POINT('Ctrl Pts',(125.915735081896,-35.0882932849811,24.6395095490115));
#23041=CARTESIAN_POINT('Ctrl Pts',(125.915038744708,-35.0459528841619,24.6374472602301));
#23042=CARTESIAN_POINT('Ctrl Pts',(125.915001572211,-35.0035839873014,24.6353849714487));
#23043=CARTESIAN_POINT('Ctrl Pts',(125.915001572211,-35.0035839863923,24.6353849714045));
#23044=CARTESIAN_POINT('Ctrl Pts',(125.914897993777,-34.8855261338114,24.629638553561));
#23045=CARTESIAN_POINT('Ctrl Pts',(125.919916516331,-34.7673454041149,24.6238921357174));
#23046=CARTESIAN_POINT('Ctrl Pts',(125.930062305213,-34.6495258061531,24.6181457178739));
#23047=CARTESIAN_POINT('Ctrl Pts',(125.940202397681,-34.5317723587141,24.6124025263913));
#23048=CARTESIAN_POINT('Ctrl Pts',(125.955463997557,-34.414380055344,24.6066593349087));
#23049=CARTESIAN_POINT('Ctrl Pts',(125.975800204933,-34.2978312101882,24.600916143426));
#23050=CARTESIAN_POINT('Ctrl Pts',(125.996130870098,-34.1813141280032,24.5951745171312));
#23051=CARTESIAN_POINT('Ctrl Pts',(126.021533322221,-34.0656404586676,24.5894328908363));
#23052=CARTESIAN_POINT('Ctrl Pts',(126.051909088729,-33.9512849975634,24.5836912645414));
#23053=CARTESIAN_POINT('Ctrl Pts',(126.082284131011,-33.8369322629426,24.5779497751394));
#23054=CARTESIAN_POINT('Ctrl Pts',(126.11763214416,-33.7238980780043,24.5722082857373));
#23055=CARTESIAN_POINT('Ctrl Pts',(126.157804255104,-33.6126439325464,24.5664667963353));
#23056=CARTESIAN_POINT('Ctrl Pts',(126.197985399101,-33.5013647706106,24.5607240159087));
#23057=CARTESIAN_POINT('Ctrl Pts',(126.242992654503,-33.3918668366453,24.554981235482));
#23058=CARTESIAN_POINT('Ctrl Pts',(126.292628585109,-33.2845927037431,24.5492384550554));
#23059=CARTESIAN_POINT('Ctrl Pts',(126.34231651387,-33.1772061914231,24.5434896585436));
#23060=CARTESIAN_POINT('Ctrl Pts',(126.396642621412,-33.0720485102871,24.5377408620317));
#23061=CARTESIAN_POINT('Ctrl Pts',(126.455362953409,-32.9695386711551,24.5319920655199));
#23062=CARTESIAN_POINT('Ctrl Pts',(126.514117959328,-32.8669683007208,24.5262398743862));
#23063=CARTESIAN_POINT('Ctrl Pts',(126.577272131778,-32.7670492373216,24.5204876832525));
#23064=CARTESIAN_POINT('Ctrl Pts',(126.644538532043,-32.6701709639857,24.5147354921189));
#23065=CARTESIAN_POINT('Ctrl Pts',(126.711905430002,-32.5731479520721,24.5089747070669));
#23066=CARTESIAN_POINT('Ctrl Pts',(126.783396567165,-32.4791751304812,24.503213922015));
#23067=CARTESIAN_POINT('Ctrl Pts',(126.858685058136,-32.388608524939,24.4974531369631));
#23068=CARTESIAN_POINT('Ctrl Pts',(126.895426495388,-32.3444112351312,24.4946418238423));
#23069=CARTESIAN_POINT('Ctrl Pts',(126.933071724442,-32.3010245830182,24.4918305107216));
#23070=CARTESIAN_POINT('Ctrl Pts',(126.971579748943,-32.2584865889459,24.4890191976008));
#23071=CARTESIAN_POINT('Ctrl Pts',(127.051348553824,-32.1703697615288,24.4831956039294));
#23072=CARTESIAN_POINT('Ctrl Pts',(127.135095038229,-32.0855952341228,24.4773720102579));
#23073=CARTESIAN_POINT('Ctrl Pts',(127.222508227281,-32.0045426972705,24.4715484165865));
#23074=CARTESIAN_POINT('Ctrl Pts',(127.30981113161,-31.9235924202328,24.4657321702435));
#23075=CARTESIAN_POINT('Ctrl Pts',(127.400771242611,-31.8463550690165,24.4599159239005));
#23076=CARTESIAN_POINT('Ctrl Pts',(127.495038491786,-31.7731760441003,24.4540996775575));
#23077=CARTESIAN_POINT('Ctrl Pts',(127.589211378925,-31.7000702717917,24.4482892533091));
#23078=CARTESIAN_POINT('Ctrl Pts',(127.686684497781,-31.6310149930845,24.4424788290608));
#23079=CARTESIAN_POINT('Ctrl Pts',(127.787072666214,-31.5663171935396,24.4366684048125));
#23080=CARTESIAN_POINT('Ctrl Pts',(127.89126073446,-31.4991704484638,24.4306380439883));
#23081=CARTESIAN_POINT('Ctrl Pts',(127.998588565236,-31.436717884397,24.4246076831641));
#23082=CARTESIAN_POINT('Ctrl Pts',(128.108589592872,-31.379255370534,24.4185773223399));
#23083=CARTESIAN_POINT('Ctrl Pts',(128.21445941535,-31.3239509222704,24.4127734381067));
#23084=CARTESIAN_POINT('Ctrl Pts',(128.322804871712,-31.2732686763006,24.4069695538735));
#23085=CARTESIAN_POINT('Ctrl Pts',(128.433183143552,-31.2274266159093,24.4011656696403));
#23086=CARTESIAN_POINT('Ctrl Pts',(128.54354511134,-31.1815913268806,24.3953626427028));
#23087=CARTESIAN_POINT('Ctrl Pts',(128.655938920462,-31.1405949582032,24.3895596157653));
#23088=CARTESIAN_POINT('Ctrl Pts',(128.769901084859,-31.104607637353,24.3837565888279));
#23089=CARTESIAN_POINT('Ctrl Pts',(128.883873310923,-31.0686171391988,24.3779530495438));
#23090=CARTESIAN_POINT('Ctrl Pts',(128.99941377817,-31.0376366911317,24.3721495102598));
#23091=CARTESIAN_POINT('Ctrl Pts',(129.116043749136,-31.0117865720905,24.3663459709757));
#23092=CARTESIAN_POINT('Ctrl Pts',(129.232711541842,-30.9859280701569,24.3605405496715));
#23093=CARTESIAN_POINT('Ctrl Pts',(129.35046914247,-30.9652032942997,24.3547351283673));
#23094=CARTESIAN_POINT('Ctrl Pts',(129.468828169307,-30.949681310529,24.3489297070631));
#23095=CARTESIAN_POINT('Ctrl Pts',(129.587318267811,-30.934142137598,24.3431178567922));
#23096=CARTESIAN_POINT('Ctrl Pts',(129.706410716854,-30.9238173105492,24.3373060065213));
#23097=CARTESIAN_POINT('Ctrl Pts',(129.825612406945,-30.9187239780446,24.3314941562504));
#23098=CARTESIAN_POINT('Ctrl Pts',(129.944892389345,-30.9136273002118,24.325678488725));
#23099=CARTESIAN_POINT('Ctrl Pts',(130.064281348287,-30.9137689594673,24.3198628211996));
#23100=CARTESIAN_POINT('Ctrl Pts',(130.183288233521,-30.9191140148918,24.3140471536742));
#23101=CARTESIAN_POINT('Ctrl Pts',(130.302465583268,-30.924466726531,24.3082231558331));
#23102=CARTESIAN_POINT('Ctrl Pts',(130.421259361681,-30.9350376746623,24.302399157992));
#23103=CARTESIAN_POINT('Ctrl Pts',(130.539185538356,-30.9507403201045,24.2965751601509));
#23104=CARTESIAN_POINT('Ctrl Pts',(130.570471995823,-30.9549063175326,24.2950300217781));
#23105=CARTESIAN_POINT('Ctrl Pts',(130.601697453545,-30.9594332434423,24.2934848834052));
#23106=CARTESIAN_POINT('Ctrl Pts',(130.632853035338,-30.964318888259,24.2919397450324));
#23107=CARTESIAN_POINT('Ctrl Pts',(130.750277186332,-30.9827326896275,24.2861161798426));
#23108=CARTESIAN_POINT('Ctrl Pts',(130.86708635909,-31.0063053840004,24.2802926146528));
#23109=CARTESIAN_POINT('Ctrl Pts',(130.98279253345,-31.0349850143794,24.274469049463));
#23110=CARTESIAN_POINT('Ctrl Pts',(131.098358075083,-31.0636297866824,24.2686525624076));
#23111=CARTESIAN_POINT('Ctrl Pts',(131.212822891391,-31.0973690542092,24.2628360753522));
#23112=CARTESIAN_POINT('Ctrl Pts',(131.325706145032,-31.1360993520763,24.2570195882968));
#23113=CARTESIAN_POINT('Ctrl Pts',(131.438460699241,-31.1747854931074,24.2512097326819));
#23114=CARTESIAN_POINT('Ctrl Pts',(131.549636896169,-31.2184512054732,24.245399877067));
#23115=CARTESIAN_POINT('Ctrl Pts',(131.658766976281,-31.2669426580348,24.2395900214521));
#23116=CARTESIAN_POINT('Ctrl Pts',(131.76782430422,-31.3154017835011,24.2337840390096));
#23117=CARTESIAN_POINT('Ctrl Pts',(131.874837856293,-31.3686800860968,24.2279780565671));
#23118=CARTESIAN_POINT('Ctrl Pts',(131.979358124371,-31.4265749741338,24.2221720741247));
#23119=CARTESIAN_POINT('Ctrl Pts',(132.083838706939,-31.4844478799449,24.2163682961673));
#23120=CARTESIAN_POINT('Ctrl Pts',(132.185827530777,-31.5469336892226,24.2105645182099));
#23121=CARTESIAN_POINT('Ctrl Pts',(132.284898567803,-31.6137833006653,24.2047607402525));
#23122=CARTESIAN_POINT('Ctrl Pts',(132.353774094002,-31.6602580555742,24.200725875243));
#23123=CARTESIAN_POINT('Ctrl Pts',(132.421239867495,-31.7088409506797,24.1966910102334));
#23124=CARTESIAN_POINT('Ctrl Pts',(132.487160670875,-31.7594357285724,24.1926561452238));
#23125=CARTESIAN_POINT('',(125.915001332191,-34.9967009094887,24.7396150285626));
#23126=CARTESIAN_POINT('Ctrl Pts',(125.915001332191,-34.9967009094887,24.7396150285626));
#23127=CARTESIAN_POINT('Ctrl Pts',(125.915116126591,-34.8545602292439,24.7327077308601));
#23128=CARTESIAN_POINT('Ctrl Pts',(125.922653598402,-34.712731699299,24.7258004331577));
#23129=CARTESIAN_POINT('Ctrl Pts',(125.93749319404,-34.5719071928536,24.7188931354552));
#23130=CARTESIAN_POINT('Ctrl Pts',(125.952505705087,-34.4294417571279,24.7119053518535));
#23131=CARTESIAN_POINT('Ctrl Pts',(125.974991434025,-34.2880039252054,24.7049175682517));
#23132=CARTESIAN_POINT('Ctrl Pts',(126.00477616189,-34.148289084606,24.69792978465));
#23133=CARTESIAN_POINT('Ctrl Pts',(126.031877926699,-34.0211595446883,24.691571449984));
#23134=CARTESIAN_POINT('Ctrl Pts',(126.065022300518,-33.8954563164075,24.685213115318));
#23135=CARTESIAN_POINT('Ctrl Pts',(126.104043775727,-33.7716881102292,24.6788547806521));
#23136=CARTESIAN_POINT('Ctrl Pts',(126.139783513885,-33.6583289084763,24.6730311869807));
#23137=CARTESIAN_POINT('Ctrl Pts',(126.180532547933,-33.546348060245,24.6672075933094));
#23138=CARTESIAN_POINT('Ctrl Pts',(126.226166636842,-33.4362203649119,24.661383999638));
#23139=CARTESIAN_POINT('Ctrl Pts',(126.271743151569,-33.3262316120246,24.6555677532951));
#23140=CARTESIAN_POINT('Ctrl Pts',(126.322192307714,-33.218091735661,24.6497515069522));
#23141=CARTESIAN_POINT('Ctrl Pts',(126.377340030494,-33.1122606786577,24.6439352606093));
#23142=CARTESIAN_POINT('Ctrl Pts',(126.4324325501,-33.0065355591265,24.6381248363611));
#23143=CARTESIAN_POINT('Ctrl Pts',(126.49221409211,-32.9031150212668,24.6323144121129));
#23144=CARTESIAN_POINT('Ctrl Pts',(126.556462644498,-32.8024387423191,24.6265039878647));
#23145=CARTESIAN_POINT('Ctrl Pts',(126.623143137484,-32.6979516579758,24.6204736270405));
#23146=CARTESIAN_POINT('Ctrl Pts',(126.694635322155,-32.5964211032217,24.6144432662162));
#23147=CARTESIAN_POINT('Ctrl Pts',(126.770638584713,-32.4983106009231,24.608412905392));
#23148=CARTESIAN_POINT('Ctrl Pts',(126.843787464204,-32.4038847425054,24.6026090211589));
#23149=CARTESIAN_POINT('Ctrl Pts',(126.921114422887,-32.3126270336183,24.5968051369258));
#23150=CARTESIAN_POINT('Ctrl Pts',(127.002307939814,-32.2249203052349,24.5910012526927));
#23151=CARTESIAN_POINT('Ctrl Pts',(127.08348946359,-32.1372265320732,24.5851982257553));
#23152=CARTESIAN_POINT('Ctrl Pts',(127.168536132488,-32.0530829958835,24.579395198818));
#23153=CARTESIAN_POINT('Ctrl Pts',(127.257097679211,-31.9728376557226,24.5735921718806));
#23154=CARTESIAN_POINT('Ctrl Pts',(127.345667044993,-31.8925852307372,24.5677886325967));
#23155=CARTESIAN_POINT('Ctrl Pts',(127.437751602994,-31.8162319602679,24.5619850933127));
#23156=CARTESIAN_POINT('Ctrl Pts',(127.532966430816,-31.7440868610295,24.5561815540288));
#23157=CARTESIAN_POINT('Ctrl Pts',(127.628212135697,-31.6719183659768,24.5503761327247));
#23158=CARTESIAN_POINT('Ctrl Pts',(127.72658980393,-31.6039610026355,24.5445707114206));
#23159=CARTESIAN_POINT('Ctrl Pts',(127.827684384881,-31.5404812663739,24.5387652901166));
#23160=CARTESIAN_POINT('Ctrl Pts',(127.928890918723,-31.47693123218,24.5329534398458));
#23161=CARTESIAN_POINT('Ctrl Pts',(128.032820024944,-31.4178689400449,24.527141589575));
#23162=CARTESIAN_POINT('Ctrl Pts',(128.139030699115,-31.3635156729112,24.5213297393041));
#23163=CARTESIAN_POINT('Ctrl Pts',(128.245311133026,-31.3091267062598,24.5155140717789));
#23164=CARTESIAN_POINT('Ctrl Pts',(128.353875748818,-31.2594530937282,24.5096984042536));
#23165=CARTESIAN_POINT('Ctrl Pts',(128.46426368474,-31.2146679181355,24.5038827367283));
#23166=CARTESIAN_POINT('Ctrl Pts',(128.574809739461,-31.1698185926148,24.4980587388873));
#23167=CARTESIAN_POINT('Ctrl Pts',(128.687183943758,-31.1298718162454,24.4922347410463));
#23168=CARTESIAN_POINT('Ctrl Pts',(128.800910291907,-31.0949508489719,24.4864107432053));
#23169=CARTESIAN_POINT('Ctrl Pts',(128.831082511994,-31.0856861259998,24.4848656048314));
#23170=CARTESIAN_POINT('Ctrl Pts',(128.861349852103,-31.0767748751189,24.4833204664575));
#23171=CARTESIAN_POINT('Ctrl Pts',(128.891703323487,-31.068218790824,24.4817753280836));
#23172=CARTESIAN_POINT('Ctrl Pts',(129.006109646572,-31.0359697563784,24.4759514933801));
#23173=CARTESIAN_POINT('Ctrl Pts',(129.122109200103,-31.0086663253676,24.4701276586767));
#23174=CARTESIAN_POINT('Ctrl Pts',(129.239236713014,-30.9864648723135,24.4643038239732));
#23175=CARTESIAN_POINT('Ctrl Pts',(129.356215278894,-30.9642916520838,24.4584873952401));
#23176=CARTESIAN_POINT('Ctrl Pts',(129.474318553343,-30.947207580189,24.4526709665069));
#23177=CARTESIAN_POINT('Ctrl Pts',(129.593066386045,-30.9353191965625,24.4468545377738));
#23178=CARTESIAN_POINT('Ctrl Pts',(129.711694163114,-30.9234428322493,24.4410439895272));
#23179=CARTESIAN_POINT('Ctrl Pts',(129.830964797952,-30.9167517461088,24.4352334412805));
#23180=CARTESIAN_POINT('Ctrl Pts',(129.950388826314,-30.9153012679702,24.4294228930339));
#23181=CARTESIAN_POINT('Ctrl Pts',(130.069721285963,-30.9138519019899,24.4236168000416));
#23182=CARTESIAN_POINT('Ctrl Pts',(130.189206498132,-30.9176351517947,24.4178107070493));
#23183=CARTESIAN_POINT('Ctrl Pts',(130.308351393327,-30.9266543949435,24.412004614057));
#23184=CARTESIAN_POINT('Ctrl Pts',(130.427447782068,-30.9356699661641,24.4062008848502));
#23185=CARTESIAN_POINT('Ctrl Pts',(130.546203722889,-30.9499172606221,24.4003971556435));
#23186=CARTESIAN_POINT('Ctrl Pts',(130.664128126284,-30.9693475922776,24.3945934264368));
#23187=CARTESIAN_POINT('Ctrl Pts',(130.782032350306,-30.9887745989902,24.3887906903715));
#23188=CARTESIAN_POINT('Ctrl Pts',(130.899104917337,-31.0133828118102,24.3829879543062));
#23189=CARTESIAN_POINT('Ctrl Pts',(131.014862463637,-31.0430720021839,24.377185218241));
#23190=CARTESIAN_POINT('Ctrl Pts',(131.130627519586,-31.0727631186128,24.3713821057292));
#23191=CARTESIAN_POINT('Ctrl Pts',(131.245076990013,-31.1075357655392,24.3655789932175));
#23192=CARTESIAN_POINT('Ctrl Pts',(131.357740886636,-31.147239342399,24.3597758807058));
#23193=CARTESIAN_POINT('Ctrl Pts',(131.470494548954,-31.1869745533434,24.3539681445262));
#23194=CARTESIAN_POINT('Ctrl Pts',(131.581459410504,-31.2316484049158,24.3481604083467));
#23195=CARTESIAN_POINT('Ctrl Pts',(131.69018367221,-31.2810614210241,24.3423526721671));
#23196=CARTESIAN_POINT('Ctrl Pts',(131.798954822992,-31.3304957472854,24.3365424313085));
#23197=CARTESIAN_POINT('Ctrl Pts',(131.905483084001,-31.3846731267033,24.3307321904498));
#23198=CARTESIAN_POINT('Ctrl Pts',(132.009340932909,-31.4433479203983,24.3249219495912));
#23199=CARTESIAN_POINT('Ctrl Pts',(132.113332546551,-31.5020982848682,24.319104225376));
#23200=CARTESIAN_POINT('Ctrl Pts',(132.214646531498,-31.5653574180558,24.3132865011608));
#23201=CARTESIAN_POINT('Ctrl Pts',(132.312883826761,-31.6328359998496,24.3074687769456));
#23202=CARTESIAN_POINT('Ctrl Pts',(132.372121391485,-31.6735259114135,24.3039606610735));
#23203=CARTESIAN_POINT('Ctrl Pts',(132.43024083144,-31.7157492671488,24.3004525452013));
#23204=CARTESIAN_POINT('Ctrl Pts',(132.487160670875,-31.7594357285724,24.2969444293292));
#23205=CARTESIAN_POINT('Ctrl Pts',(132.487160670875,-31.7594357285724,25.5469383396565));
#23206=CARTESIAN_POINT('Ctrl Pts',(132.581965719039,-31.8321994102783,25.5411336436149));
#23207=CARTESIAN_POINT('Ctrl Pts',(132.67354602429,-31.909104676569,25.5353289475733));
#23208=CARTESIAN_POINT('Ctrl Pts',(132.761532853475,-31.9898237096175,25.5295242515317));
#23209=CARTESIAN_POINT('Ctrl Pts',(132.849614083683,-32.0706293460753,25.5237133276347));
#23210=CARTESIAN_POINT('Ctrl Pts',(132.934093838299,-32.1552566430948,25.5179024037377));
#23211=CARTESIAN_POINT('Ctrl Pts',(133.014639827328,-32.2433404795867,25.5120914798407));
#23212=CARTESIAN_POINT('Ctrl Pts',(133.095233471736,-32.3314764312567,25.5062771178857));
#23213=CARTESIAN_POINT('Ctrl Pts',(133.171888452797,-32.4230726831881,25.5004627559307));
#23214=CARTESIAN_POINT('Ctrl Pts',(133.244313495104,-32.5177318949217,25.4946483939758));
#23215=CARTESIAN_POINT('Ctrl Pts',(133.316848344028,-32.6125346234227,25.4888252166249));
#23216=CARTESIAN_POINT('Ctrl Pts',(133.385140213338,-32.7104092514028,25.483002039274));
#23217=CARTESIAN_POINT('Ctrl Pts',(133.448941585321,-32.8109301196535,25.477178861923));
#23218=CARTESIAN_POINT('Ctrl Pts',(133.485485999684,-32.8685068793262,25.4738434382573));
#23219=CARTESIAN_POINT('Ctrl Pts',(133.520558010519,-32.9269513631098,25.4705080145915));
#23220=CARTESIAN_POINT('Ctrl Pts',(133.554118108444,-32.9861803776824,25.4671725909258));
#23221=CARTESIAN_POINT('Ctrl Pts',(133.612713475523,-33.089593241923,25.4613489972493));
#23222=CARTESIAN_POINT('Ctrl Pts',(133.666886136784,-33.1957323814797,25.4555254035728));
#23223=CARTESIAN_POINT('Ctrl Pts',(133.716373321031,-33.3041832826833,25.4497018098963));
#23224=CARTESIAN_POINT('Ctrl Pts',(133.765798069845,-33.4124973569673,25.4438855635481));
#23225=CARTESIAN_POINT('Ctrl Pts',(133.810548931312,-33.5231170235738,25.4380693172));
#23226=CARTESIAN_POINT('Ctrl Pts',(133.850407969835,-33.6356014270622,25.4322530708519));
#23227=CARTESIAN_POINT('Ctrl Pts',(133.89022710924,-33.7479732330426,25.4264426465984));
#23228=CARTESIAN_POINT('Ctrl Pts',(133.925164031561,-33.862205679837,25.4206322223449));
#23229=CARTESIAN_POINT('Ctrl Pts',(133.955048302462,-33.9778366445668,25.4148217980914));
#23230=CARTESIAN_POINT('Ctrl Pts',(133.986063754792,-34.0978444803334,25.4087914372692));
#23231=CARTESIAN_POINT('Ctrl Pts',(134.011636305304,-34.2193583917457,25.4027610764469));
#23232=CARTESIAN_POINT('Ctrl Pts',(134.031631640618,-34.3418424851396,25.3967307156247));
#23233=CARTESIAN_POINT('Ctrl Pts',(134.05087602995,-34.4597265587583,25.3909268313862));
#23234=CARTESIAN_POINT('Ctrl Pts',(134.064954494204,-34.578508816858,25.3851229471477));
#23235=CARTESIAN_POINT('Ctrl Pts',(134.073799202137,-34.6977003793139,25.3793190629091));
#23236=CARTESIAN_POINT('Ctrl Pts',(134.082642603612,-34.816874335902,25.3735160359664));
#23237=CARTESIAN_POINT('Ctrl Pts',(134.086253755971,-34.9364570695058,25.3677130090236));
#23238=CARTESIAN_POINT('Ctrl Pts',(134.084616753787,-35.0559551131028,25.3619099820808));
#23239=CARTESIAN_POINT('Ctrl Pts',(134.082979607073,-35.1754637071277,25.3561064427914));
#23240=CARTESIAN_POINT('Ctrl Pts',(134.076093390145,-35.2948871879604,25.350302903502));
#23241=CARTESIAN_POINT('Ctrl Pts',(134.063994313666,-35.4137332697378,25.3444993642127));
#23242=CARTESIAN_POINT('Ctrl Pts',(134.051891313598,-35.5326178919144,25.3386939429031));
#23243=CARTESIAN_POINT('Ctrl Pts',(134.034572133353,-35.6509243366218,25.3328885215936));
#23244=CARTESIAN_POINT('Ctrl Pts',(134.012124633458,-35.7681672510609,25.327083100284));
#23245=CARTESIAN_POINT('Ctrl Pts',(133.989652275034,-35.8855400011756,25.3212712500078));
#23246=CARTESIAN_POINT('Ctrl Pts',(133.962040337742,-36.0018464688193,25.3154593997315));
#23247=CARTESIAN_POINT('Ctrl Pts',(133.929427456171,-36.1166131231056,25.3096475494552));
#23248=CARTESIAN_POINT('Ctrl Pts',(133.896793154284,-36.2314551567464,25.3038318819244));
#23249=CARTESIAN_POINT('Ctrl Pts',(133.859151495107,-36.3447549762657,25.2980162143937));
#23250=CARTESIAN_POINT('Ctrl Pts',(133.816689918593,-36.4560573701981,25.292200546863));
#23251=CARTESIAN_POINT('Ctrl Pts',(133.774167520457,-36.5675191927906,25.2863765490165));
#23252=CARTESIAN_POINT('Ctrl Pts',(133.726811586517,-36.6769775057666,25.28055255117));
#23253=CARTESIAN_POINT('Ctrl Pts',(133.674856337231,-36.7839999721731,25.2747285533236));
#23254=CARTESIAN_POINT('Ctrl Pts',(133.661072326862,-36.8123936149122,25.2731834150015));
#23255=CARTESIAN_POINT('Ctrl Pts',(133.646964825407,-36.8406159572215,25.2716382766794));
#23256=CARTESIAN_POINT('Ctrl Pts',(133.632538719108,-36.8686592664739,25.2700931383574));
#23257=CARTESIAN_POINT('Ctrl Pts',(133.578167029443,-36.9743539061957,25.2642695446866));
#23258=CARTESIAN_POINT('Ctrl Pts',(133.519090795536,-37.0778439672222,25.2584459510158));
#23259=CARTESIAN_POINT('Ctrl Pts',(133.455512663061,-37.1786824540134,25.252622357345));
#23260=CARTESIAN_POINT('Ctrl Pts',(133.392014743844,-37.2793937180753,25.2468061110026));
#23261=CARTESIAN_POINT('Ctrl Pts',(133.324026438936,-37.3774597193653,25.2409898646602));
#23262=CARTESIAN_POINT('Ctrl Pts',(133.251797002751,-37.4724565219435,25.2351736183179));
#23263=CARTESIAN_POINT('Ctrl Pts',(133.17963986863,-37.567358232198,25.2293631940702));
#23264=CARTESIAN_POINT('Ctrl Pts',(133.103250294646,-37.6591965324894,25.2235527698225));
#23265=CARTESIAN_POINT('Ctrl Pts',(133.022921361146,-37.7475755575285,25.2177423455749));
#23266=CARTESIAN_POINT('Ctrl Pts',(132.939551811351,-37.8392999114788,25.2117119847504));
#23267=CARTESIAN_POINT('Ctrl Pts',(132.851939022809,-37.927297555214,25.205681623926));
#23268=CARTESIAN_POINT('Ctrl Pts',(132.760457575815,-38.0111623955089,25.1996512631016));
#23269=CARTESIAN_POINT('Ctrl Pts',(132.672411811516,-38.0918776028455,25.193847378869));
#23270=CARTESIAN_POINT('Ctrl Pts',(132.58078305967,-38.1687645315343,25.1880434946364));
#23271=CARTESIAN_POINT('Ctrl Pts',(132.485943022891,-38.2414984632021,25.1822396104038));
#23272=CARTESIAN_POINT('Ctrl Pts',(132.391116994998,-38.3142216512904,25.176436583467));
#23273=CARTESIAN_POINT('Ctrl Pts',(132.293080949419,-38.3827928138722,25.1706335565301));
#23274=CARTESIAN_POINT('Ctrl Pts',(132.192238888955,-38.4469281474602,25.1648305295933));
#23275=CARTESIAN_POINT('Ctrl Pts',(132.091387925192,-38.5110691435275,25.1590269903099));
#23276=CARTESIAN_POINT('Ctrl Pts',(131.987730798546,-38.5707733127841,25.1532234510265));
#23277=CARTESIAN_POINT('Ctrl Pts',(131.881699092075,-38.6258010876057,25.147419911743));
#23278=CARTESIAN_POINT('Ctrl Pts',(131.775633000759,-38.6808467072931,25.1416144904395));
#23279=CARTESIAN_POINT('Ctrl Pts',(131.667191160414,-38.7312127285709,25.1358090691359));
#23280=CARTESIAN_POINT('Ctrl Pts',(131.556827668056,-38.7767065827219,25.1300036478324));
#23281=CARTESIAN_POINT('Ctrl Pts',(131.446341958346,-38.8222508171055,25.1241917975621));
#23282=CARTESIAN_POINT('Ctrl Pts',(131.333930726594,-38.8629119588209,25.1183799472918));
#23283=CARTESIAN_POINT('Ctrl Pts',(131.2200660148,-38.898546385453,25.1125680970215));
#23284=CARTESIAN_POINT('Ctrl Pts',(131.106126516053,-38.9342042169678,25.1067524294967));
#23285=CARTESIAN_POINT('Ctrl Pts',(130.990732029815,-38.9648286537308,25.1009367619719));
#23286=CARTESIAN_POINT('Ctrl Pts',(130.874366029577,-38.9903269347664,25.0951210944472));
#23287=CARTESIAN_POINT('Ctrl Pts',(130.757833347608,-39.0158617393362,25.0892970966067));
#23288=CARTESIAN_POINT('Ctrl Pts',(130.640326774998,-39.0362556630418,25.0834730987662));
#23289=CARTESIAN_POINT('Ctrl Pts',(130.522336297021,-39.0514676097452,25.0776491009256));
#23290=CARTESIAN_POINT('Ctrl Pts',(130.491032779942,-39.0555034221396,25.0761039625467));
#23291=CARTESIAN_POINT('Ctrl Pts',(130.459695207567,-39.0591747752407,25.0745588241678));
#23292=CARTESIAN_POINT('Ctrl Pts',(130.428332725701,-39.0624815170156,25.0730136857889));
#23293=CARTESIAN_POINT('Ctrl Pts',(130.310128198923,-39.0749445564,25.0671900921183));
#23294=CARTESIAN_POINT('Ctrl Pts',(130.191188658355,-39.0822643809855,25.0613664984476));
#23295=CARTESIAN_POINT('Ctrl Pts',(130.071999041145,-39.084365451092,25.055542904777));
#23296=CARTESIAN_POINT('Ctrl Pts',(129.952959799342,-39.0864638703865,25.0497266584348));
#23297=CARTESIAN_POINT('Ctrl Pts',(129.833671513113,-39.0833566239554,25.0439104120926));
#23298=CARTESIAN_POINT('Ctrl Pts',(129.714625382435,-39.0750197947556,25.0380941657504));
#23299=CARTESIAN_POINT('Ctrl Pts',(129.59569841759,-39.0666913107677,25.0322837415029));
#23300=CARTESIAN_POINT('Ctrl Pts',(129.477013531071,-39.0531436864415,25.0264733172554));
#23301=CARTESIAN_POINT('Ctrl Pts',(129.359062469155,-39.0344050467887,25.0206628930078));
#23302=CARTESIAN_POINT('Ctrl Pts',(129.236646715557,-39.0149571108631,25.0146325321834));
#23303=CARTESIAN_POINT('Ctrl Pts',(129.115021885921,-38.9899174056844,25.0086021713589));
#23304=CARTESIAN_POINT('Ctrl Pts',(128.994732956178,-38.9593766138883,25.0025718105344));
#23305=CARTESIAN_POINT('Ctrl Pts',(128.878961604681,-38.9299828138971,24.9967679263021));
#23306=CARTESIAN_POINT('Ctrl Pts',(128.764428051713,-38.8954937835913,24.9909640420697));
#23307=CARTESIAN_POINT('Ctrl Pts',(128.651607636185,-38.8560424055248,24.9851601578373));
#23308=CARTESIAN_POINT('Ctrl Pts',(128.538803885439,-38.8165968548488,24.9793571309008));
#23309=CARTESIAN_POINT('Ctrl Pts',(128.427713154244,-38.7721905488504,24.9735541039642));
#23310=CARTESIAN_POINT('Ctrl Pts',(128.318794267271,-38.7230058130816,24.9677510770276));
#23311=CARTESIAN_POINT('Ctrl Pts',(128.209865763899,-38.673816734815,24.9619475377444));
#23312=CARTESIAN_POINT('Ctrl Pts',(128.103109858166,-38.6198485560297,24.9561439984613));
#23313=CARTESIAN_POINT('Ctrl Pts',(127.998963495633,-38.5613309180965,24.9503404591781));
#23314=CARTESIAN_POINT('Ctrl Pts',(127.894783359649,-38.5027943035756,24.9445350378748));
#23315=CARTESIAN_POINT('Ctrl Pts',(127.793214805662,-38.4397054957163,24.9387296165715));
#23316=CARTESIAN_POINT('Ctrl Pts',(127.694667812035,-38.3723387290031,24.9329241952682));
#23317=CARTESIAN_POINT('Ctrl Pts',(127.596011686735,-38.3048973598316,24.9271123449982));
#23318=CARTESIAN_POINT('Ctrl Pts',(127.500384138194,-38.2331688060413,24.9213004947282));
#23319=CARTESIAN_POINT('Ctrl Pts',(127.408164044286,-38.1574691413643,24.9154886444582));
#23320=CARTESIAN_POINT('Ctrl Pts',(127.315883379725,-38.0817197567409,24.9096729769337));
#23321=CARTESIAN_POINT('Ctrl Pts',(127.227014930152,-38.001994338893,24.9038573094093));
#23322=CARTESIAN_POINT('Ctrl Pts',(127.141901300726,-37.9186464029085,24.8980416418848));
#23323=CARTESIAN_POINT('Ctrl Pts',(127.056665755218,-37.8351790800058,24.8922176440446));
#23324=CARTESIAN_POINT('Ctrl Pts',(126.975196042748,-37.7480791794289,24.8863936462043));
#23325=CARTESIAN_POINT('Ctrl Pts',(126.897795127024,-37.6577339833181,24.8805696483641));
#23326=CARTESIAN_POINT('Ctrl Pts',(126.877260242069,-37.6337649102004,24.8790245099829));
#23327=CARTESIAN_POINT('Ctrl Pts',(126.857011512478,-37.6095675709048,24.8774793716017));
#23328=CARTESIAN_POINT('Ctrl Pts',(126.837054078806,-37.5851495313814,24.8759342332205));
#23329=CARTESIAN_POINT('Ctrl Pts',(126.762195742137,-37.4935599085143,24.8701385737665));
#23330=CARTESIAN_POINT('Ctrl Pts',(126.691190191979,-37.3985584741059,24.8643429143124));
#23331=CARTESIAN_POINT('Ctrl Pts',(126.624365980108,-37.3005042846615,24.8585472548584));
#23332=CARTESIAN_POINT('Ctrl Pts',(126.557622092833,-37.2025679591328,24.8527585619513));
#23333=CARTESIAN_POINT('Ctrl Pts',(126.495049783104,-37.1015865096678,24.8469698690443));
#23334=CARTESIAN_POINT('Ctrl Pts',(126.436938220602,-36.9979528913849,24.8411811761372));
#23335=CARTESIAN_POINT('Ctrl Pts',(126.378882465277,-36.8944187971804,24.8353980423753));
#23336=CARTESIAN_POINT('Ctrl Pts',(126.325279140324,-36.7882379553403,24.8296149086134));
#23337=CARTESIAN_POINT('Ctrl Pts',(126.27637444219,-36.6798326420283,24.8238317748515));
#23338=CARTESIAN_POINT('Ctrl Pts',(126.22750489271,-36.5715052414952,24.8180527975282));
#23339=CARTESIAN_POINT('Ctrl Pts',(126.183327422775,-36.4609569235521,24.8122738202048));
#23340=CARTESIAN_POINT('Ctrl Pts',(126.144042212232,-36.3486343236595,24.8064948428815));
#23341=CARTESIAN_POINT('Ctrl Pts',(126.104770622542,-36.2363506679293,24.8007178692282));
#23342=CARTESIAN_POINT('Ctrl Pts',(126.070388060113,-36.1222943403461,24.7949408955749));
#23343=CARTESIAN_POINT('Ctrl Pts',(126.041046289914,-36.006931239657,24.7891639219216));
#23344=CARTESIAN_POINT('Ctrl Pts',(126.011711368871,-35.8915950678071,24.7833882967688));
#23345=CARTESIAN_POINT('Ctrl Pts',(125.98741499763,-35.7749531300053,24.777612671616));
#23346=CARTESIAN_POINT('Ctrl Pts',(125.968258611742,-35.6574848881995,24.7718370464631));
#23347=CARTESIAN_POINT('Ctrl Pts',(125.949095050159,-35.5399726445438,24.7660592578473));
#23348=CARTESIAN_POINT('Ctrl Pts',(125.93507538937,-35.4216338854961,24.7602814692315));
#23349=CARTESIAN_POINT('Ctrl Pts',(125.926249593192,-35.302956470529,24.7545036806157));
#23350=CARTESIAN_POINT('Ctrl Pts',(125.918668595408,-35.2010174270874,24.749540796609));
#23351=CARTESIAN_POINT('Ctrl Pts',(125.914918852587,-35.0988287956417,24.7445779126023));
#23352=CARTESIAN_POINT('Ctrl Pts',(125.91500133219,-34.9967009101661,24.7396150285955));
#23353=CARTESIAN_POINT('Origin',(130.,-35.,32.7603849714045));
#23354=CARTESIAN_POINT('',(132.487160670875,-31.7594357285724,26.7967734504842));
#23355=CARTESIAN_POINT('',(132.487160670875,-31.7594357285724,26.6927660718219));
#23356=CARTESIAN_POINT('',(132.487160670875,-31.7594357285724,32.7603849714045));
#23357=CARTESIAN_POINT('',(125.91500046357,-34.998053885216,25.8853849714464));
#23358=CARTESIAN_POINT('Ctrl Pts',(132.487160670875,-31.7594357285724,26.6927660718219));
#23359=CARTESIAN_POINT('Ctrl Pts',(132.584486290898,-31.8341339706419,26.6867872558272));
#23360=CARTESIAN_POINT('Ctrl Pts',(132.678341578341,-31.9131420984798,26.6808084398325));
#23361=CARTESIAN_POINT('Ctrl Pts',(132.768344329939,-31.9960867737405,26.6748296238378));
#23362=CARTESIAN_POINT('Ctrl Pts',(132.858347081536,-32.0790314490012,26.6688508078431));
#23363=CARTESIAN_POINT('Ctrl Pts',(132.944497017134,-32.1659122971067,26.6628719918484));
#23364=CARTESIAN_POINT('Ctrl Pts',(133.026456729518,-32.2563191394852,26.6568931758537));
#23365=CARTESIAN_POINT('Ctrl Pts',(133.106288598545,-32.3443788335715,26.6510695822667));
#23366=CARTESIAN_POINT('Ctrl Pts',(133.182402651789,-32.4360676801457,26.6452459886798));
#23367=CARTESIAN_POINT('Ctrl Pts',(133.254451673081,-32.5310388201556,26.6394223950928));
#23368=CARTESIAN_POINT('Ctrl Pts',(133.326409793813,-32.6258901399413,26.6336061488357));
#23369=CARTESIAN_POINT('Ctrl Pts',(133.394312838722,-32.7240151941611,26.6277899025786));
#23370=CARTESIAN_POINT('Ctrl Pts',(133.457851565361,-32.8250315974873,26.6219736563214));
#23371=CARTESIAN_POINT('Ctrl Pts',(133.521326689369,-32.9259468828127,26.6161632321602));
#23372=CARTESIAN_POINT('Ctrl Pts',(133.58044596995,-33.0297474158179,26.6103528079991));
#23373=CARTESIAN_POINT('Ctrl Pts',(133.634941851182,-33.1360196517866,26.6045423838379));
#23374=CARTESIAN_POINT('Ctrl Pts',(133.691500515386,-33.2463145139389,26.5985120229815));
#23375=CARTESIAN_POINT('Ctrl Pts',(133.743078583024,-33.3592715373707,26.5924816621252));
#23376=CARTESIAN_POINT('Ctrl Pts',(133.789427576039,-33.4743972843641,26.5864513012688));
#23377=CARTESIAN_POINT('Ctrl Pts',(133.834035882578,-33.5851993596284,26.5806474171254));
#23378=CARTESIAN_POINT('Ctrl Pts',(133.873800632321,-33.6980097857414,26.5748435329819));
#23379=CARTESIAN_POINT('Ctrl Pts',(133.908548515549,-33.8123664278925,26.5690396488385));
#23380=CARTESIAN_POINT('Ctrl Pts',(133.943291266139,-33.9267061783283,26.5632366219916));
#23381=CARTESIAN_POINT('Ctrl Pts',(133.973018505237,-34.0425913000075,26.5574335951448));
#23382=CARTESIAN_POINT('Ctrl Pts',(133.997606581839,-34.159543804331,26.5516305682979));
#23383=CARTESIAN_POINT('Ctrl Pts',(134.022196829308,-34.2765066343234,26.5458270291052));
#23384=CARTESIAN_POINT('Ctrl Pts',(134.041646928132,-34.3945366347084,26.5400234899125));
#23385=CARTESIAN_POINT('Ctrl Pts',(134.055884335606,-34.5131455492763,26.5342199507197));
#23386=CARTESIAN_POINT('Ctrl Pts',(134.070126360103,-34.6317929273198,26.5284145295075));
#23387=CARTESIAN_POINT('Ctrl Pts',(134.079152282757,-34.7510191876909,26.5226091082953));
#23388=CARTESIAN_POINT('Ctrl Pts',(134.082941474662,-34.8703315208451,26.5168036870831));
#23389=CARTESIAN_POINT('Ctrl Pts',(134.086734862746,-34.9897759813572,26.5109918369046));
#23390=CARTESIAN_POINT('Ctrl Pts',(134.085279931424,-35.1093062965414,26.5051799867261));
#23391=CARTESIAN_POINT('Ctrl Pts',(134.078608182357,-35.2284300654614,26.4993681365476));
#23392=CARTESIAN_POINT('Ctrl Pts',(134.071932051251,-35.3476320755059,26.493552469115));
#23393=CARTESIAN_POINT('Ctrl Pts',(134.060032319177,-35.4664266021361,26.4877368016825));
#23394=CARTESIAN_POINT('Ctrl Pts',(134.042992121299,-35.5843284240144,26.4819211342499));
#23395=CARTESIAN_POINT('Ctrl Pts',(134.025927515177,-35.7023991275269,26.4760971365014));
#23396=CARTESIAN_POINT('Ctrl Pts',(134.003707822585,-35.8195741743018,26.470273138753));
#23397=CARTESIAN_POINT('Ctrl Pts',(133.976466834679,-35.9353804106881,26.4644491410045));
#23398=CARTESIAN_POINT('Ctrl Pts',(133.969239647932,-35.9661044541676,26.4629040017647));
#23399=CARTESIAN_POINT('Ctrl Pts',(133.961659295106,-35.9967322461004,26.461358862525));
#23400=CARTESIAN_POINT('Ctrl Pts',(133.953728849266,-36.0272551710664,26.4598137232852));
#23401=CARTESIAN_POINT('Ctrl Pts',(133.923839184084,-36.1422953624942,26.4539901295726));
#23402=CARTESIAN_POINT('Ctrl Pts',(133.888876229056,-36.2562154491357,26.4481665358599));
#23403=CARTESIAN_POINT('Ctrl Pts',(133.848939755854,-36.3685348938938,26.4423429421472));
#23404=CARTESIAN_POINT('Ctrl Pts',(133.809053668442,-36.4807126309992,26.4365266957625));
#23405=CARTESIAN_POINT('Ctrl Pts',(133.764206678942,-36.5912933615056,26.4307104493778));
#23406=CARTESIAN_POINT('Ctrl Pts',(133.714549087987,-36.6998088342318,26.4248942029931));
#23407=CARTESIAN_POINT('Ctrl Pts',(133.664941204552,-36.8082156823799,26.4190837787026));
#23408=CARTESIAN_POINT('Ctrl Pts',(133.610532468316,-36.9145610162808,26.4132733544121));
#23409=CARTESIAN_POINT('Ctrl Pts',(133.551522091763,-37.0183943697208,26.4074629301217));
#23410=CARTESIAN_POINT('Ctrl Pts',(133.490278051005,-37.1261580292921,26.4014325693131));
#23411=CARTESIAN_POINT('Ctrl Pts',(133.424077273874,-37.2312153614181,26.3954022085046));
#23412=CARTESIAN_POINT('Ctrl Pts',(133.353196250816,-37.3330880616707,26.389371847696));
#23413=CARTESIAN_POINT('Ctrl Pts',(133.284977239009,-37.4311348256938,26.3835679634199));
#23414=CARTESIAN_POINT('Ctrl Pts',(133.212423438938,-37.5262314831677,26.3777640791437));
#23415=CARTESIAN_POINT('Ctrl Pts',(133.135826364774,-37.6179797573683,26.3719601948675));
#23416=CARTESIAN_POINT('Ctrl Pts',(133.059240604813,-37.7097144793713,26.3661571678869));
#23417=CARTESIAN_POINT('Ctrl Pts',(132.978613020091,-37.7981014883151,26.3603541409062));
#23418=CARTESIAN_POINT('Ctrl Pts',(132.894275605525,-37.8827753501207,26.3545511139256));
#23419=CARTESIAN_POINT('Ctrl Pts',(132.809930744844,-37.9674566877454,26.3487475745982));
#23420=CARTESIAN_POINT('Ctrl Pts',(132.721875691268,-38.0484239370961,26.3429440352708));
#23421=CARTESIAN_POINT('Ctrl Pts',(132.630479042952,-38.1253487812709,26.3371404959433));
#23422=CARTESIAN_POINT('Ctrl Pts',(132.539052755767,-38.2022985712772,26.3313350745957));
#23423=CARTESIAN_POINT('Ctrl Pts',(132.444283030975,-38.275203086206,26.325529653248));
#23424=CARTESIAN_POINT('Ctrl Pts',(132.346570732266,-38.3437749323889,26.3197242319004));
#23425=CARTESIAN_POINT('Ctrl Pts',(132.248750226231,-38.4124227155436,26.313912381586));
#23426=CARTESIAN_POINT('Ctrl Pts',(132.14798097622,-38.476728017972,26.3081005312716));
#23427=CARTESIAN_POINT('Ctrl Pts',(132.044692080248,-38.5364472704922,26.3022886809572));
#23428=CARTESIAN_POINT('Ctrl Pts',(131.941335343575,-38.5962057469382,26.2964730133883));
#23429=CARTESIAN_POINT('Ctrl Pts',(131.835456026431,-38.6513719864717,26.2906573458195));
#23430=CARTESIAN_POINT('Ctrl Pts',(131.727505525628,-38.7017495402748,26.2848416782506));
#23431=CARTESIAN_POINT('Ctrl Pts',(131.619400397396,-38.7521992544809,26.2790176803662));
#23432=CARTESIAN_POINT('Ctrl Pts',(131.509218539945,-38.7978464364833,26.2731936824819));
#23433=CARTESIAN_POINT('Ctrl Pts',(131.397429024793,-38.8385436197425,26.2673696845975));
#23434=CARTESIAN_POINT('Ctrl Pts',(131.367770665218,-38.8493408013311,26.2658245466373));
#23435=CARTESIAN_POINT('Ctrl Pts',(131.33799921507,-38.8597898439868,26.264279408677));
#23436=CARTESIAN_POINT('Ctrl Pts',(131.308123564557,-38.8698885952765,26.2627342707168));
#23437=CARTESIAN_POINT('Ctrl Pts',(131.195522843021,-38.9079505842978,26.2569106770474));
#23438=CARTESIAN_POINT('Ctrl Pts',(131.081077952104,-38.9411554195207,26.251087083378));
#23439=CARTESIAN_POINT('Ctrl Pts',(130.965245490355,-38.9693231341563,26.2452634897087));
#23440=CARTESIAN_POINT('Ctrl Pts',(130.849559168462,-38.9974553110362,26.2394472433676));
#23441=CARTESIAN_POINT('Ctrl Pts',(130.732489150969,-39.0205629117897,26.2336309970266));
#23442=CARTESIAN_POINT('Ctrl Pts',(130.61450945898,-39.0385149652842,26.2278147506856));
#23443=CARTESIAN_POINT('Ctrl Pts',(130.496647865311,-39.0564490486743,26.2220043264392));
#23444=CARTESIAN_POINT('Ctrl Pts',(130.37787881002,-39.0692377903677,26.2161939021928));
#23445=CARTESIAN_POINT('Ctrl Pts',(130.258688251069,-39.0768008767609,26.2103834779464));
#23446=CARTESIAN_POINT('Ctrl Pts',(130.134986082877,-39.0846502416209,26.2043531171215));
#23447=CARTESIAN_POINT('Ctrl Pts',(130.010830306499,-39.0868704250375,26.1983227562966));
#23448=CARTESIAN_POINT('Ctrl Pts',(129.886772523961,-39.0834304865725,26.1922923954717));
#23449=CARTESIAN_POINT('Ctrl Pts',(129.767373862958,-39.0801197386432,26.1864885112402));
#23450=CARTESIAN_POINT('Ctrl Pts',(129.648066412888,-39.0715663580064,26.1806846270087));
#23451=CARTESIAN_POINT('Ctrl Pts',(129.529343078356,-39.0577958379037,26.1748807427773));
#23452=CARTESIAN_POINT('Ctrl Pts',(129.410637280528,-39.0440273518539,26.1690777158415));
#23453=CARTESIAN_POINT('Ctrl Pts',(129.292515832161,-39.0250433059067,26.1632746889057));
#23454=CARTESIAN_POINT('Ctrl Pts',(129.175466359289,-39.0009210533746,26.1574716619699));
#23455=CARTESIAN_POINT('Ctrl Pts',(129.058406552172,-38.9767966710997,26.1516681226875));
#23456=CARTESIAN_POINT('Ctrl Pts',(128.942419308677,-38.9475332626986,26.145864583405));
#23457=CARTESIAN_POINT('Ctrl Pts',(128.827981275665,-38.913259141663,26.1400610441226));
#23458=CARTESIAN_POINT('Ctrl Pts',(128.713506131733,-38.8789739059292,26.13425562282));
#23459=CARTESIAN_POINT('Ctrl Pts',(128.600581588395,-38.839674843065,26.1284502015173));
#23460=CARTESIAN_POINT('Ctrl Pts',(128.489667752291,-38.7955396851478,26.1226447802147));
#23461=CARTESIAN_POINT('Ctrl Pts',(128.378631089378,-38.7513556516274,26.1168329299452));
#23462=CARTESIAN_POINT('Ctrl Pts',(128.269609957953,-38.7023249840245,26.1110210796757));
#23463=CARTESIAN_POINT('Ctrl Pts',(128.163043288153,-38.6486730517819,26.1052092294062));
#23464=CARTESIAN_POINT('Ctrl Pts',(128.05640662479,-38.5949858806616,26.0993935618822));
#23465=CARTESIAN_POINT('Ctrl Pts',(127.952227989091,-38.5366715990711,26.0935778943582));
#23466=CARTESIAN_POINT('Ctrl Pts',(127.850919124464,-38.4740000561894,26.0877622268341));
#23467=CARTESIAN_POINT('Ctrl Pts',(127.749465145825,-38.4112387430886,26.0819382289943));
#23468=CARTESIAN_POINT('Ctrl Pts',(127.650889479176,-38.3441079404169,26.0761142311544));
#23469=CARTESIAN_POINT('Ctrl Pts',(127.555572589189,-38.2729191302681,26.0702902333145));
#23470=CARTESIAN_POINT('Ctrl Pts',(127.530284498455,-38.2540323506999,26.0687450949258));
#23471=CARTESIAN_POINT('Ctrl Pts',(127.505225589072,-38.2348601481981,26.0671999565371));
#23472=CARTESIAN_POINT('Ctrl Pts',(127.480402534567,-38.2154087783959,26.0656548181484));
#23473=CARTESIAN_POINT('Ctrl Pts',(127.387890871815,-38.1429165489286,26.0598963277298));
#23474=CARTESIAN_POINT('Ctrl Pts',(127.298344601786,-38.0662984777782,26.0541378373113));
#23475=CARTESIAN_POINT('Ctrl Pts',(127.212159759073,-37.9858284932445,26.0483793468928));
#23476=CARTESIAN_POINT('Ctrl Pts',(127.126084184856,-37.9054605316861,26.0426281573123));
#23477=CARTESIAN_POINT('Ctrl Pts',(127.043361868387,-37.8212506484488,26.0368769677319));
#23478=CARTESIAN_POINT('Ctrl Pts',(126.964357841702,-37.7335145301908,26.0311257781514));
#23479=CARTESIAN_POINT('Ctrl Pts',(126.88543220804,-37.6458654695144,26.0253802952818));
#23480=CARTESIAN_POINT('Ctrl Pts',(126.810217805869,-37.5546974406822,26.0196348124122));
#23481=CARTESIAN_POINT('Ctrl Pts',(126.73904413004,-37.460364162919,26.0138893295426));
#23482=CARTESIAN_POINT('Ctrl Pts',(126.667920512358,-37.3660972320024,26.0081478876082));
#23483=CARTESIAN_POINT('Ctrl Pts',(126.60083221996,-37.2686698127851,26.0024064456739));
#23484=CARTESIAN_POINT('Ctrl Pts',(126.538069144986,-37.1684694498891,25.9966650037395));
#23485=CARTESIAN_POINT('Ctrl Pts',(126.475328663353,-37.0683051569421,25.9909256285992));
#23486=CARTESIAN_POINT('Ctrl Pts',(126.416910526328,-36.9653702585504,25.985186253459));
#23487=CARTESIAN_POINT('Ctrl Pts',(126.363061503257,-36.8600815495317,25.9794468783187));
#23488=CARTESIAN_POINT('Ctrl Pts',(126.309218443453,-36.7548045002363,25.9737081387597));
#23489=CARTESIAN_POINT('Ctrl Pts',(126.259943681615,-36.6471745313558,25.9679693992006));
#23490=CARTESIAN_POINT('Ctrl Pts',(126.215437817401,-36.537632623887,25.9622306596416));
#23491=CARTESIAN_POINT('Ctrl Pts',(126.170925788961,-36.4280755444595,25.9564911252459));
#23492=CARTESIAN_POINT('Ctrl Pts',(126.13118412738,-36.3166063882113,25.9507515908502));
#23493=CARTESIAN_POINT('Ctrl Pts',(126.096364826132,-36.2036849377379,25.9450120564546));
#23494=CARTESIAN_POINT('Ctrl Pts',(126.061513761251,-36.0906604755645,25.939267286214));
#23495=CARTESIAN_POINT('Ctrl Pts',(126.031594144116,-35.9761814747901,25.9335225159735));
#23496=CARTESIAN_POINT('Ctrl Pts',(126.006707715966,-35.860721635765,25.927777745733));
#23497=CARTESIAN_POINT('Ctrl Pts',(125.981808406243,-35.7452020330715,25.922030001917));
#23498=CARTESIAN_POINT('Ctrl Pts',(125.961947542635,-35.6287009933682,25.916282258101));
#23499=CARTESIAN_POINT('Ctrl Pts',(125.947175220414,-35.5116994293291,25.910534514285));
#23500=CARTESIAN_POINT('Ctrl Pts',(125.932382690922,-35.3945378171746,25.904778908048));
#23501=CARTESIAN_POINT('Ctrl Pts',(125.922692631631,-35.2768747301239,25.8990233018109));
#23502=CARTESIAN_POINT('Ctrl Pts',(125.918103075061,-35.159193260448,25.8932676955738));
#23503=CARTESIAN_POINT('Ctrl Pts',(125.916007830481,-35.1054687975995,25.8906401208647));
#23504=CARTESIAN_POINT('Ctrl Pts',(125.914974887006,-35.0517404675829,25.8880125461556));
#23505=CARTESIAN_POINT('Ctrl Pts',(125.91500046357,-34.998053885216,25.8853849714464));
#23506=CARTESIAN_POINT('Ctrl Pts',(125.91500046357,-34.9980538843595,25.8853849714045));
#23507=CARTESIAN_POINT('Ctrl Pts',(125.915055004632,-34.8835693136621,25.879781769463));
#23508=CARTESIAN_POINT('Ctrl Pts',(125.919921914211,-34.7692049072162,25.8741785675215));
#23509=CARTESIAN_POINT('Ctrl Pts',(125.92957331797,-34.6552513579166,25.8685753655799));
#23510=CARTESIAN_POINT('Ctrl Pts',(125.939604342104,-34.536815653468,25.8627517719035));
#23511=CARTESIAN_POINT('Ctrl Pts',(125.954824952508,-34.4186271295216,25.856928178227));
#23512=CARTESIAN_POINT('Ctrl Pts',(125.975217969216,-34.3011762706659,25.8511045845505));
#23513=CARTESIAN_POINT('Ctrl Pts',(125.995585257105,-34.183873593513,25.8452883382024));
#23514=CARTESIAN_POINT('Ctrl Pts',(126.021111902477,-34.0673071291332,25.8394720918543));
#23515=CARTESIAN_POINT('Ctrl Pts',(126.051728847284,-33.9519637865835,25.8336558455062));
#23516=CARTESIAN_POINT('Ctrl Pts',(126.082315144362,-33.8367359033547,25.8278454212527));
#23517=CARTESIAN_POINT('Ctrl Pts',(126.117981500013,-33.7227290986611,25.8220349969993));
#23518=CARTESIAN_POINT('Ctrl Pts',(126.158607643251,-33.6104210128559,25.8162245727458));
#23519=CARTESIAN_POINT('Ctrl Pts',(126.20077156999,-33.4938618338497,25.8101942119235));
#23520=CARTESIAN_POINT('Ctrl Pts',(126.248278102886,-33.3791329563222,25.8041638511013));
#23521=CARTESIAN_POINT('Ctrl Pts',(126.300935504727,-33.2667525105132,25.798133490279));
#23522=CARTESIAN_POINT('Ctrl Pts',(126.351615302105,-33.1585926313008,25.7923296060405));
#23523=CARTESIAN_POINT('Ctrl Pts',(126.407065864033,-33.0526083722017,25.786525721802));
#23524=CARTESIAN_POINT('Ctrl Pts',(126.467067129435,-32.9492415227334,25.7807218375636));
#23525=CARTESIAN_POINT('Ctrl Pts',(126.527059532009,-32.8458899416535,25.7749188106208));
#23526=CARTESIAN_POINT('Ctrl Pts',(126.591601096351,-32.7451553543973,25.7691157836781));
#23527=CARTESIAN_POINT('Ctrl Pts',(126.660426315324,-32.6474540164702,25.7633127567353));
#23528=CARTESIAN_POINT('Ctrl Pts',(126.729257610845,-32.5497440525362,25.757509217446));
#23529=CARTESIAN_POINT('Ctrl Pts',(126.802373077782,-32.4550682042312,25.7517056781566));
#23530=CARTESIAN_POINT('Ctrl Pts',(126.879464862814,-32.3638123250448,25.7459021388673));
#23531=CARTESIAN_POINT('Ctrl Pts',(126.956581647812,-32.2725268526405,25.7400967175577));
#23532=CARTESIAN_POINT('Ctrl Pts',(127.037677051999,-32.1846638667855,25.7342912962482));
#23533=CARTESIAN_POINT('Ctrl Pts',(127.122404508452,-32.1005743349722,25.7284858749387));
#23534=CARTESIAN_POINT('Ctrl Pts',(127.20722579272,-32.0163916817859,25.7226740246625));
#23535=CARTESIAN_POINT('Ctrl Pts',(127.295686867836,-31.9359911116015,25.7168621743862));
#23536=CARTESIAN_POINT('Ctrl Pts',(127.387405936575,-31.8596851655038,25.71105032411));
#23537=CARTESIAN_POINT('Ctrl Pts',(127.479185246891,-31.783329101251,25.7052346565793));
#23538=CARTESIAN_POINT('Ctrl Pts',(127.574226488116,-31.7110732635981,25.6994189890486));
#23539=CARTESIAN_POINT('Ctrl Pts',(127.67211792635,-31.6431875162321,25.6936033215179));
#23540=CARTESIAN_POINT('Ctrl Pts',(127.770149583498,-31.5752045298638,25.6877793236714));
#23541=CARTESIAN_POINT('Ctrl Pts',(127.871039242098,-31.5116043447514,25.681955325825));
#23542=CARTESIAN_POINT('Ctrl Pts',(127.974349474773,-31.4526115310488,25.6761313279786));
#23543=CARTESIAN_POINT('Ctrl Pts',(128.001758241707,-31.4369604165395,25.6745861896562));
#23544=CARTESIAN_POINT('Ctrl Pts',(128.029337272293,-31.4216333400051,25.6730410513338));
#23545=CARTESIAN_POINT('Ctrl Pts',(128.057078167553,-31.406633924438,25.6714959130115));
#23546=CARTESIAN_POINT('Ctrl Pts',(128.161633015309,-31.3501014442725,25.6656723193407));
#23547=CARTESIAN_POINT('Ctrl Pts',(128.268825870595,-31.2980448796578,25.6598487256699));
#23548=CARTESIAN_POINT('Ctrl Pts',(128.378237088824,-31.2507187275515,25.6540251319991));
#23549=CARTESIAN_POINT('Ctrl Pts',(128.487510268548,-31.2034522844158,25.6482088856567));
#23550=CARTESIAN_POINT('Ctrl Pts',(128.598995873004,-31.1609045440246,25.6423926393143));
#23551=CARTESIAN_POINT('Ctrl Pts',(128.712248810399,-31.1232846540299,25.636576392972));
#23552=CARTESIAN_POINT('Ctrl Pts',(128.825388380978,-31.0857024217527,25.6307659687243));
#23553=CARTESIAN_POINT('Ctrl Pts',(128.940291379782,-31.0530383546505,25.6249555444766));
#23554=CARTESIAN_POINT('Ctrl Pts',(129.056492394029,-31.0254536865858,25.6191451202289));
#23555=CARTESIAN_POINT('Ctrl Pts',(129.177091857028,-30.9968248817756,25.6131147594045));
#23556=CARTESIAN_POINT('Ctrl Pts',(129.299089130788,-30.9736677832049,25.6070843985801));
#23557=CARTESIAN_POINT('Ctrl Pts',(129.42194576277,-30.9561060475304,25.6010540377557));
#23558=CARTESIAN_POINT('Ctrl Pts',(129.540188383732,-30.9392038614513,25.5952501535231));
#23559=CARTESIAN_POINT('Ctrl Pts',(129.659226538169,-30.9274844008765,25.5894462692905));
#23560=CARTESIAN_POINT('Ctrl Pts',(129.778570096611,-30.9210057859952,25.5836423850579));
#23561=CARTESIAN_POINT('Ctrl Pts',(129.897896026732,-30.9145281280745,25.5778393581211));
#23562=CARTESIAN_POINT('Ctrl Pts',(130.01752686352,-30.9132897984775,25.5720363311842));
#23563=CARTESIAN_POINT('Ctrl Pts',(130.136968921539,-30.9172969108038,25.5662333042474));
#23564=CARTESIAN_POINT('Ctrl Pts',(130.256421525043,-30.9213043769162,25.560429764964));
#23565=CARTESIAN_POINT('Ctrl Pts',(130.375684908512,-30.9305581920495,25.5546262256806));
#23566=CARTESIAN_POINT('Ctrl Pts',(130.494267601245,-30.9450123873975,25.5488226863971));
#23567=CARTESIAN_POINT('Ctrl Pts',(130.612888748962,-30.9594712700724,25.5430172650936));
#23568=CARTESIAN_POINT('Ctrl Pts',(130.730828361811,-30.9791338374944,25.53721184379));
#23569=CARTESIAN_POINT('Ctrl Pts',(130.847602925348,-31.0039026186863,25.5314064224865));
#23570=CARTESIAN_POINT('Ctrl Pts',(130.964506805905,-31.0286988290109,25.5255945722162));
#23571=CARTESIAN_POINT('Ctrl Pts',(131.080242662143,-31.0586124555127,25.5197827219459));
#23572=CARTESIAN_POINT('Ctrl Pts',(131.194339806386,-31.0934954976499,25.5139708716756));
#23573=CARTESIAN_POINT('Ctrl Pts',(131.308511890247,-31.1284014511566,25.5081552041508));
#23574=CARTESIAN_POINT('Ctrl Pts',(131.421042734608,-31.1682831844245,25.502339536626));
#23575=CARTESIAN_POINT('Ctrl Pts',(131.531480935743,-31.2129442645434,25.4965238691012));
#23576=CARTESIAN_POINT('Ctrl Pts',(131.642077327677,-31.2576693168372,25.4906998712607));
#23577=CARTESIAN_POINT('Ctrl Pts',(131.750574723407,-31.3071872110837,25.4848758734202));
#23578=CARTESIAN_POINT('Ctrl Pts',(131.856545517183,-31.3612551968259,25.4790518755796));
#23579=CARTESIAN_POINT('Ctrl Pts',(131.884660146513,-31.3755997282159,25.4775067372008));
#23580=CARTESIAN_POINT('Ctrl Pts',(131.91259709215,-31.3902642890495,25.4759615988219));
#23581=CARTESIAN_POINT('Ctrl Pts',(131.940348719913,-31.4052438406572,25.474416460443));
#23582=CARTESIAN_POINT('Ctrl Pts',(132.044926391124,-31.4616919393519,25.4685938479916));
#23583=CARTESIAN_POINT('Ctrl Pts',(132.147207370064,-31.5227983537948,25.4627712355401));
#23584=CARTESIAN_POINT('Ctrl Pts',(132.246748991077,-31.588351722247,25.4569486230886));
#23585=CARTESIAN_POINT('Ctrl Pts',(132.328827476711,-31.6424047018551,25.4521475036415));
#23586=CARTESIAN_POINT('Ctrl Pts',(132.409043659943,-31.6994802575364,25.4473463841943));
#23587=CARTESIAN_POINT('Ctrl Pts',(132.487160670875,-31.7594357285724,25.4425452647471));
#23588=CARTESIAN_POINT('',(125.915000988625,-35.0028420178004,25.9896150286367));
#23589=CARTESIAN_POINT('Ctrl Pts',(125.915000988624,-35.0028420169516,25.9896150285955));
#23590=CARTESIAN_POINT('Ctrl Pts',(125.914917631215,-34.8830274839136,25.98379925565));
#23591=CARTESIAN_POINT('Ctrl Pts',(125.920109897602,-34.7631670310304,25.9779834827044));
#23592=CARTESIAN_POINT('Ctrl Pts',(125.930563220774,-34.6437566844379,25.9721677097589));
#23593=CARTESIAN_POINT('Ctrl Pts',(125.941015823111,-34.5243545720863,25.9663523378546));
#23594=CARTESIAN_POINT('Ctrl Pts',(125.956728725648,-34.4054029082059,25.9605369659503));
#23595=CARTESIAN_POINT('Ctrl Pts',(125.977635392704,-34.2873935406028,25.954721594046));
#23596=CARTESIAN_POINT('Ctrl Pts',(125.998545461785,-34.16936497,25.948905275839));
#23597=CARTESIAN_POINT('Ctrl Pts',(126.024650905997,-34.0522793999723,25.943088957632));
#23598=CARTESIAN_POINT('Ctrl Pts',(126.05583399618,-33.9366188198428,25.937272639425));
#23599=CARTESIAN_POINT('Ctrl Pts',(126.087029385142,-33.820912622558,25.9314540272308));
#23600=CARTESIAN_POINT('Ctrl Pts',(126.123306298709,-33.7066329244786,25.9256354150366));
#23601=CARTESIAN_POINT('Ctrl Pts',(126.164497225102,-33.5942463004665,25.9198168028424));
#23602=CARTESIAN_POINT('Ctrl Pts',(126.205738353575,-33.4817227035156,25.9139910991244));
#23603=CARTESIAN_POINT('Ctrl Pts',(126.251905311348,-33.3710971675099,25.9081653954065));
#23604=CARTESIAN_POINT('Ctrl Pts',(126.302782435853,-33.2628162781789,25.9023396916885));
#23605=CARTESIAN_POINT('Ctrl Pts',(126.353695625483,-33.1544586320743,25.8965098583201));
#23606=CARTESIAN_POINT('Ctrl Pts',(126.409325443941,-33.0484493010495,25.8906800249518));
#23607=CARTESIAN_POINT('Ctrl Pts',(126.469411107928,-32.9452087514349,25.8848501915834));
#23608=CARTESIAN_POINT('Ctrl Pts',(126.529589512802,-32.8418088523261,25.8790113599967));
#23609=CARTESIAN_POINT('Ctrl Pts',(126.594237274589,-32.7411866060431,25.8731725284101));
#23610=CARTESIAN_POINT('Ctrl Pts',(126.663051158471,-32.6437323095588,25.8673336968235));
#23611=CARTESIAN_POINT('Ctrl Pts',(126.686630918682,-32.6103386277456,25.8653329632365));
#23612=CARTESIAN_POINT('Ctrl Pts',(126.710699509638,-32.5773166148935,25.8633322296496));
#23613=CARTESIAN_POINT('Ctrl Pts',(126.735243706803,-32.5446810093122,25.8613314960627));
#23614=CARTESIAN_POINT('Ctrl Pts',(126.80668521814,-32.4496875992438,25.8555079023934));
#23615=CARTESIAN_POINT('Ctrl Pts',(126.882391357813,-32.3576616542344,25.849684308724));
#23616=CARTESIAN_POINT('Ctrl Pts',(126.962086897633,-32.2690095235488,25.8438607150547));
#23617=CARTESIAN_POINT('Ctrl Pts',(127.041681889693,-32.1804692406932,25.8380444687137));
#23618=CARTESIAN_POINT('Ctrl Pts',(127.125256000357,-32.0952946069411,25.8322282223727));
#23619=CARTESIAN_POINT('Ctrl Pts',(127.212491956808,-32.0138613714127,25.8264119760317));
#23620=CARTESIAN_POINT('Ctrl Pts',(127.299640589586,-31.9325096510016,25.8206015517854));
#23621=CARTESIAN_POINT('Ctrl Pts',(127.390443479258,-31.8548921553197,25.814791127539));
#23622=CARTESIAN_POINT('Ctrl Pts',(127.484544897526,-31.7813495642682,25.8089807032927));
#23623=CARTESIAN_POINT('Ctrl Pts',(127.582208249156,-31.7050232339974,25.8029503424677));
#23624=CARTESIAN_POINT('Ctrl Pts',(127.683424475912,-31.6330867240478,25.7969199816428));
#23625=CARTESIAN_POINT('Ctrl Pts',(127.78775579291,-31.5658770307111,25.7908896208179));
#23626=CARTESIAN_POINT('Ctrl Pts',(127.888168836698,-31.5011914686559,25.7850857365864));
#23627=CARTESIAN_POINT('Ctrl Pts',(127.991466835099,-31.4408843257239,25.779281852355));
#23628=CARTESIAN_POINT('Ctrl Pts',(128.097228583065,-31.3852128783433,25.7734779681235));
#23629=CARTESIAN_POINT('Ctrl Pts',(128.202974708891,-31.3295496542302,25.7676749411878));
#23630=CARTESIAN_POINT('Ctrl Pts',(128.31118349932,-31.2785209540833,25.761871914252));
#23631=CARTESIAN_POINT('Ctrl Pts',(128.421408823274,-31.2323382719833,25.7560688873162));
#23632=CARTESIAN_POINT('Ctrl Pts',(128.531643878972,-31.1861515124349,25.7502653480338));
#23633=CARTESIAN_POINT('Ctrl Pts',(128.643895445546,-31.144811779412,25.7444618087514));
#23634=CARTESIAN_POINT('Ctrl Pts',(128.757697678905,-31.1084823085327,25.738658269469));
#23635=CARTESIAN_POINT('Ctrl Pts',(128.871536817004,-31.0721410564291,25.7328528481664));
#23636=CARTESIAN_POINT('Ctrl Pts',(128.986927233173,-31.040813421886,25.7270474268638));
#23637=CARTESIAN_POINT('Ctrl Pts',(129.103388830485,-31.0146125143595,25.7212420055612));
#23638=CARTESIAN_POINT('Ctrl Pts',(129.219979398238,-30.9883825917524,25.7154301552918));
#23639=CARTESIAN_POINT('Ctrl Pts',(129.337643116341,-30.9672908183684,25.7096183050223));
#23640=CARTESIAN_POINT('Ctrl Pts',(129.455890467262,-30.9513990297408,25.7038064547528));
#23641=CARTESIAN_POINT('Ctrl Pts',(129.57421548368,-30.9354968033008,25.6979907872288));
#23642=CARTESIAN_POINT('Ctrl Pts',(129.693124490572,-30.9248013999251,25.6921751197048));
#23643=CARTESIAN_POINT('Ctrl Pts',(129.812125293178,-30.9193225936694,25.6863594521808));
#23644=CARTESIAN_POINT('Ctrl Pts',(129.931296551588,-30.9138359396153,25.680535454341));
#23645=CARTESIAN_POINT('Ctrl Pts',(130.050559461267,-30.9135807976808,25.6747114565011));
#23646=CARTESIAN_POINT('Ctrl Pts',(130.169424134947,-30.9185149194812,25.6688874586613));
#23647=CARTESIAN_POINT('Ctrl Pts',(130.200959581122,-30.9198239689039,25.6673423202723));
#23648=CARTESIAN_POINT('Ctrl Pts',(130.232467039439,-30.9214979936995,25.6657971818832));
#23649=CARTESIAN_POINT('Ctrl Pts',(130.263937469796,-30.9235355990714,25.6642520434942));
#23650=CARTESIAN_POINT('Ctrl Pts',(130.382535283496,-30.9312144118348,25.6584291159803));
#23651=CARTESIAN_POINT('Ctrl Pts',(130.500988941927,-30.9440855038667,25.6526061884664));
#23652=CARTESIAN_POINT('Ctrl Pts',(130.618807884703,-30.9621414336521,25.6467832609524));
#23653=CARTESIAN_POINT('Ctrl Pts',(130.736486110336,-30.9801757983241,25.6409672880564));
#23654=CARTESIAN_POINT('Ctrl Pts',(130.853530727798,-31.0033826262588,25.6351513151604));
#23655=CARTESIAN_POINT('Ctrl Pts',(130.969453622283,-31.0317025471566,25.6293353422643));
#23656=CARTESIAN_POINT('Ctrl Pts',(131.085265436093,-31.0599953310862,25.623524942402));
#23657=CARTESIAN_POINT('Ctrl Pts',(131.199957270419,-31.0933913669269,25.6177145425396));
#23658=CARTESIAN_POINT('Ctrl Pts',(131.313049197558,-31.1317798918892,25.6119041426772));
#23659=CARTESIAN_POINT('Ctrl Pts',(131.426056890353,-31.170139823898,25.6060980705793));
#23660=CARTESIAN_POINT('Ctrl Pts',(131.537466661935,-31.2134847146107,25.6002919984813));
#23661=CARTESIAN_POINT('Ctrl Pts',(131.646812448055,-31.2616536060806,25.5944859263834));
#23662=CARTESIAN_POINT('Ctrl Pts',(131.75610939188,-31.3098009815934,25.5886824477269));
#23663=CARTESIAN_POINT('Ctrl Pts',(131.863343811697,-31.3627679059948,25.5828789690703));
#23664=CARTESIAN_POINT('Ctrl Pts',(131.968068894647,-31.4203450130042,25.5770754904138));
#23665=CARTESIAN_POINT('Ctrl Pts',(132.072791333078,-31.477920666076,25.5712721583068));
#23666=CARTESIAN_POINT('Ctrl Pts',(132.175004198702,-31.5401060813459,25.5654688261997));
#23667=CARTESIAN_POINT('Ctrl Pts',(132.274284934959,-31.6066457546229,25.5596654940927));
#23668=CARTESIAN_POINT('Ctrl Pts',(132.346861702901,-31.6552879646674,25.5554231092806));
#23669=CARTESIAN_POINT('Ctrl Pts',(132.417872030513,-31.7062561071201,25.5511807244686));
#23670=CARTESIAN_POINT('Ctrl Pts',(132.487160670875,-31.7594357285724,25.5469383396565));
#23671=CARTESIAN_POINT('Ctrl Pts',(132.487160670875,-31.7594357285724,26.7967734504842));
#23672=CARTESIAN_POINT('Ctrl Pts',(132.581820842687,-31.8320882164445,26.7909668279223));
#23673=CARTESIAN_POINT('Ctrl Pts',(132.673369442088,-31.9089489675386,26.7851602053605));
#23674=CARTESIAN_POINT('Ctrl Pts',(132.76141620503,-31.9897167006079,26.7793535827986));
#23675=CARTESIAN_POINT('Ctrl Pts',(132.849425873815,-32.0704504061804,26.7735494065705));
#23676=CARTESIAN_POINT('Ctrl Pts',(132.933936338899,-32.1550875457114,26.7677452303424));
#23677=CARTESIAN_POINT('Ctrl Pts',(133.014590944703,-32.2432870232625,26.7619410541143));
#23678=CARTESIAN_POINT('Ctrl Pts',(133.095230284945,-32.3314698072271,26.7561379764474));
#23679=CARTESIAN_POINT('Ctrl Pts',(133.172014941736,-32.4232132872004,26.7503348987804));
#23680=CARTESIAN_POINT('Ctrl Pts',(133.244626084105,-32.5181405006837,26.7445318211134));
#23681=CARTESIAN_POINT('Ctrl Pts',(133.317240619587,-32.6130721501085,26.7387284722691));
#23682=CARTESIAN_POINT('Ctrl Pts',(133.385681004865,-32.7111875044315,26.7329251234247));
#23683=CARTESIAN_POINT('Ctrl Pts',(133.449669970158,-32.8120781327959,26.7271217745804));
#23684=CARTESIAN_POINT('Ctrl Pts',(133.513677026994,-32.9129972858761,26.7213167849605));
#23685=CARTESIAN_POINT('Ctrl Pts',(133.573229942324,-33.0166929287383,26.7155117953405));
#23686=CARTESIAN_POINT('Ctrl Pts',(133.628096220153,-33.1227299562102,26.7097068057206));
#23687=CARTESIAN_POINT('Ctrl Pts',(133.683022189654,-33.2288823464814,26.7038955005724));
#23688=CARTESIAN_POINT('Ctrl Pts',(133.733251154285,-33.3373808439128,26.6980841954241));
#23689=CARTESIAN_POINT('Ctrl Pts',(133.778597736247,-33.4477680110159,26.6922728902759));
#23690=CARTESIAN_POINT('Ctrl Pts',(133.82397241188,-33.5582235665286,26.6864579848367));
#23691=CARTESIAN_POINT('Ctrl Pts',(133.864458542072,-33.6705697386857,26.6806430793975));
#23692=CARTESIAN_POINT('Ctrl Pts',(133.899920380554,-33.7843330944115,26.6748281739584));
#23693=CARTESIAN_POINT('Ctrl Pts',(133.935434693245,-33.8982647900363,26.6690046639858));
#23694=CARTESIAN_POINT('Ctrl Pts',(133.965909766219,-34.0136174623106,26.6631811540132));
#23695=CARTESIAN_POINT('Ctrl Pts',(133.991260715997,-34.1299063861051,26.6573576440406));
#23696=CARTESIAN_POINT('Ctrl Pts',(134.002446048264,-34.1812153217859,26.6547881981392));
#23697=CARTESIAN_POINT('Ctrl Pts',(134.012634521584,-34.2327064385346,26.6522187522379));
#23698=CARTESIAN_POINT('Ctrl Pts',(134.021822060174,-34.2843378476543,26.6496493063365));
#23699=CARTESIAN_POINT('Ctrl Pts',(134.042645419241,-34.4013593285178,26.6438257123361));
#23700=CARTESIAN_POINT('Ctrl Pts',(134.058390721628,-34.5194791038513,26.6380021183358));
#23701=CARTESIAN_POINT('Ctrl Pts',(134.068948190858,-34.6382188228866,26.6321785243355));
#23702=CARTESIAN_POINT('Ctrl Pts',(134.079492340279,-34.7568087342102,26.62636227766));
#23703=CARTESIAN_POINT('Ctrl Pts',(134.084861638985,-34.8760166304091,26.6205460309846));
#23704=CARTESIAN_POINT('Ctrl Pts',(134.084997358261,-34.9953542488175,26.6147297843091));
#23705=CARTESIAN_POINT('Ctrl Pts',(134.08513294168,-35.1145724096823,26.6089193597252));
#23706=CARTESIAN_POINT('Ctrl Pts',(134.080045367229,-35.2339196284414,26.6031089351413));
#23707=CARTESIAN_POINT('Ctrl Pts',(134.06972777815,-35.3529034028614,26.5972985105574));
#23708=CARTESIAN_POINT('Ctrl Pts',(134.059019647824,-35.4763909495606,26.5912681498578));
#23709=CARTESIAN_POINT('Ctrl Pts',(134.042677707291,-35.5994865476445,26.5852377891583));
#23710=CARTESIAN_POINT('Ctrl Pts',(134.020753720595,-35.7216401584744,26.5792074284587));
#23711=CARTESIAN_POINT('Ctrl Pts',(133.999653110775,-35.839206170349,26.5734035438842));
#23712=CARTESIAN_POINT('Ctrl Pts',(133.973382250749,-35.9558992354687,26.5675996593098));
#23713=CARTESIAN_POINT('Ctrl Pts',(133.94203994179,-36.0712357804576,26.5617957747353));
#23714=CARTESIAN_POINT('Ctrl Pts',(133.910702262416,-36.1865552890363,26.5559927474551));
#23715=CARTESIAN_POINT('Ctrl Pts',(133.874294730895,-36.3005182820209,26.5501897201749));
#23716=CARTESIAN_POINT('Ctrl Pts',(133.832966639145,-36.412654148474,26.5443866928947));
#23717=CARTESIAN_POINT('Ctrl Pts',(133.791634898549,-36.5247999153723,26.5385831532667));
#23718=CARTESIAN_POINT('Ctrl Pts',(133.745381875178,-36.6351178518403,26.5327796136388));
#23719=CARTESIAN_POINT('Ctrl Pts',(133.694405610657,-36.7431558117236,26.5269760740109));
#23720=CARTESIAN_POINT('Ctrl Pts',(133.643412815122,-36.8512288070687,26.5211706523622));
#23721=CARTESIAN_POINT('Ctrl Pts',(133.587693906403,-36.957019986286,26.5153652307134));
#23722=CARTESIAN_POINT('Ctrl Pts',(133.527493321216,-37.0601009365497,26.5095598090647));
#23723=CARTESIAN_POINT('Ctrl Pts',(133.467226069464,-37.1632960394077,26.5037479584497));
#23724=CARTESIAN_POINT('Ctrl Pts',(133.402467440639,-37.2637745695883,26.4979361078348));
#23725=CARTESIAN_POINT('Ctrl Pts',(133.333505813073,-37.3611361659615,26.4921242572199));
#23726=CARTESIAN_POINT('Ctrl Pts',(133.264498891141,-37.4585617099506,26.4863085893505));
#23727=CARTESIAN_POINT('Ctrl Pts',(133.191283722595,-37.5528659212446,26.4804929214811));
#23728=CARTESIAN_POINT('Ctrl Pts',(133.114188607779,-37.6436819618065,26.4746772536117));
#23729=CARTESIAN_POINT('Ctrl Pts',(133.036983062576,-37.7346280864924,26.4688532554291));
#23730=CARTESIAN_POINT('Ctrl Pts',(132.955886755106,-37.8220757695081,26.4630292572465));
#23731=CARTESIAN_POINT('Ctrl Pts',(132.871264481853,-37.9056953170025,26.4572052590639));
#23732=CARTESIAN_POINT('Ctrl Pts',(132.848813780388,-37.9278799904371,26.4556601239653));
#23733=CARTESIAN_POINT('Ctrl Pts',(132.826115074573,-37.9497954371215,26.4541149888666));
#23734=CARTESIAN_POINT('Ctrl Pts',(132.803175546273,-37.9714359923744,26.452569853768));
#23735=CARTESIAN_POINT('Ctrl Pts',(132.71671676846,-38.0529989580071,26.4467462600813));
#23736=CARTESIAN_POINT('Ctrl Pts',(132.62655580342,-38.1309168291375,26.4409226663946));
#23737=CARTESIAN_POINT('Ctrl Pts',(132.533032554403,-38.2048355774258,26.4350990727079));
#23738=CARTESIAN_POINT('Ctrl Pts',(132.43962729884,-38.2786610662467,26.4292828263486));
#23739=CARTESIAN_POINT('Ctrl Pts',(132.34286851411,-38.3484972166099,26.4234665799893));
#23740=CARTESIAN_POINT('Ctrl Pts',(132.243132376016,-38.4140272617056,26.4176503336301));
#23741=CARTESIAN_POINT('Ctrl Pts',(132.143496074328,-38.4794917108768,26.4118399093644));
#23742=CARTESIAN_POINT('Ctrl Pts',(132.040888687611,-38.5406584069209,26.4060294850987));
#23743=CARTESIAN_POINT('Ctrl Pts',(131.935718371841,-38.5972516432571,26.400219060833));
#23744=CARTESIAN_POINT('Ctrl Pts',(131.826567142526,-38.6559870504088,26.394188700015));
#23745=CARTESIAN_POINT('Ctrl Pts',(131.714655477881,-38.7097956491854,26.3881583391969));
#23746=CARTESIAN_POINT('Ctrl Pts',(131.600471789566,-38.758419222333,26.3821279783788));
#23747=CARTESIAN_POINT('Ctrl Pts',(131.490576390177,-38.8052166858733,26.3763240941258));
#23748=CARTESIAN_POINT('Ctrl Pts',(131.378576955514,-38.8472113842628,26.3705202098727));
#23749=CARTESIAN_POINT('Ctrl Pts',(131.264932091607,-38.8842208747216,26.3647163256197));
#23750=CARTESIAN_POINT('Ctrl Pts',(131.151304014243,-38.9212248984886,26.3589132986615));
#23751=CARTESIAN_POINT('Ctrl Pts',(131.036031379141,-38.9532450523193,26.3531102717033));
#23752=CARTESIAN_POINT('Ctrl Pts',(130.919589628053,-38.9801482278901,26.3473072447451));
#23753=CARTESIAN_POINT('Ctrl Pts',(130.803137596359,-39.0070537787339,26.3415037054395));
#23754=CARTESIAN_POINT('Ctrl Pts',(130.685516641328,-39.0288413611504,26.3357001661339));
#23755=CARTESIAN_POINT('Ctrl Pts',(130.567213484114,-39.0454287613848,26.3298966268282));
#23756=CARTESIAN_POINT('Ctrl Pts',(130.448871962547,-39.0620215407223,26.3240912055016));
#23757=CARTESIAN_POINT('Ctrl Pts',(130.329848202995,-39.0734107274202,26.318285784175));
#23758=CARTESIAN_POINT('Ctrl Pts',(130.210634508843,-39.0795659209877,26.3124803628483));
#23759=CARTESIAN_POINT('Ctrl Pts',(130.091288796536,-39.0857279308636,26.3066685125538));
#23760=CARTESIAN_POINT('Ctrl Pts',(129.971753137817,-39.0866443569019,26.3008566622593));
#23761=CARTESIAN_POINT('Ctrl Pts',(129.852520461635,-39.0823369270264,26.2950448119648));
#23762=CARTESIAN_POINT('Ctrl Pts',(129.733209472777,-39.0780266680074,26.2892291444151));
#23763=CARTESIAN_POINT('Ctrl Pts',(129.614202268867,-39.0684857525945,26.2834134768654));
#23764=CARTESIAN_POINT('Ctrl Pts',(129.495985624897,-39.0537876744705,26.2775978093158));
#23765=CARTESIAN_POINT('Ctrl Pts',(129.377599648333,-39.0390685429347,26.2717738114495));
#23766=CARTESIAN_POINT('Ctrl Pts',(129.260006893091,-39.0191775723406,26.2659498135832));
#23767=CARTESIAN_POINT('Ctrl Pts',(129.143683073694,-38.9942391417792,26.2601258157169));
#23768=CARTESIAN_POINT('Ctrl Pts',(129.112821734483,-38.987622841103,26.2585806775445));
#23769=CARTESIAN_POINT('Ctrl Pts',(129.082049622154,-38.9806515350318,26.2570355393721));
#23770=CARTESIAN_POINT('Ctrl Pts',(129.051375411372,-38.9733281251176,26.2554904011996));
#23771=CARTESIAN_POINT('Ctrl Pts',(128.935764949884,-38.9457263456983,26.2496668076131));
#23772=CARTESIAN_POINT('Ctrl Pts',(128.82117373593,-38.9130300558571,26.2438432140266));
#23773=CARTESIAN_POINT('Ctrl Pts',(128.708084191167,-38.8753294753978,26.23801962044));
#23774=CARTESIAN_POINT('Ctrl Pts',(128.595137325691,-38.8376764598303,26.2322033741833));
#23775=CARTESIAN_POINT('Ctrl Pts',(128.483688745096,-38.7950318393624,26.2263871279266));
#23776=CARTESIAN_POINT('Ctrl Pts',(128.374209589866,-38.7475365965281,26.2205708816699));
#23777=CARTESIAN_POINT('Ctrl Pts',(128.264840023901,-38.7000888967052,26.2147604575092));
#23778=CARTESIAN_POINT('Ctrl Pts',(128.157436333883,-38.6478003955138,26.2089500333485));
#23779=CARTESIAN_POINT('Ctrl Pts',(128.052452849073,-38.5908613305049,26.2031396091877));
#23780=CARTESIAN_POINT('Ctrl Pts',(127.943495519992,-38.531767002907,26.1971092483312));
#23781=CARTESIAN_POINT('Ctrl Pts',(127.837145661117,-38.4676632298352,26.1910788874747));
#23782=CARTESIAN_POINT('Ctrl Pts',(127.733886967421,-38.3988169594102,26.1850485266182));
#23783=CARTESIAN_POINT('Ctrl Pts',(127.634506265465,-38.3325562850112,26.1792446424752));
#23784=CARTESIAN_POINT('Ctrl Pts',(127.537989102031,-38.2619031554098,26.1734407583322));
#23785=CARTESIAN_POINT('Ctrl Pts',(127.444739458112,-38.1871411269462,26.1676368741892));
#23786=CARTESIAN_POINT('Ctrl Pts',(127.351503588177,-38.1123901416446,26.1618338473428));
#23787=CARTESIAN_POINT('Ctrl Pts',(127.261534596423,-38.0335317198258,26.1560308204964));
#23788=CARTESIAN_POINT('Ctrl Pts',(127.175204430662,-37.9508905420987,26.15022779365));
#23789=CARTESIAN_POINT('Ctrl Pts',(127.08886664286,-37.86824206803,26.1444242544578));
#23790=CARTESIAN_POINT('Ctrl Pts',(127.006168614799,-37.7818104564063,26.1386207152655));
#23791=CARTESIAN_POINT('Ctrl Pts',(126.927445910499,-37.6919577201531,26.1328171760733));
#23792=CARTESIAN_POINT('Ctrl Pts',(126.848697677352,-37.6020758457143,26.1270117548615));
#23793=CARTESIAN_POINT('Ctrl Pts',(126.773927600746,-37.508770947214,26.1212063336498));
#23794=CARTESIAN_POINT('Ctrl Pts',(126.703430969558,-37.4124381085387,26.115400912438));
#23795=CARTESIAN_POINT('Ctrl Pts',(126.632856269881,-37.3159985901676,26.10958906226));
#23796=CARTESIAN_POINT('Ctrl Pts',(126.566564703279,-37.2165247681411,26.103777212082));
#23797=CARTESIAN_POINT('Ctrl Pts',(126.504808302838,-37.114440824448,26.0979653619039));
#23798=CARTESIAN_POINT('Ctrl Pts',(126.443011340466,-37.0122898314788,26.0921496944719));
#23799=CARTESIAN_POINT('Ctrl Pts',(126.385755671832,-36.9075256601811,26.0863340270398));
#23800=CARTESIAN_POINT('Ctrl Pts',(126.333246661262,-36.8005957216576,26.0805183596078));
#23801=CARTESIAN_POINT('Ctrl Pts',(126.280662437201,-36.6935126175377,26.0746943618598));
#23802=CARTESIAN_POINT('Ctrl Pts',(126.232838604949,-36.584257927056,26.0688703641118));
#23803=CARTESIAN_POINT('Ctrl Pts',(126.189931906797,-36.4732977041844,26.0630463663638));
#23804=CARTESIAN_POINT('Ctrl Pts',(126.178548519299,-36.4438593351597,26.0615012271196));
#23805=CARTESIAN_POINT('Ctrl Pts',(126.167510959477,-36.4143009917256,26.0599560878754));
#23806=CARTESIAN_POINT('Ctrl Pts',(126.156821555698,-36.3846315196659,26.0584109486312));
#23807=CARTESIAN_POINT('Ctrl Pts',(126.110323273239,-36.2555710481221,26.0516896831143));
#23808=CARTESIAN_POINT('Ctrl Pts',(126.070293444533,-36.1240650790749,26.0449684175974));
#23809=CARTESIAN_POINT('Ctrl Pts',(126.03695945865,-35.9907243146395,26.0382471520806));
#23810=CARTESIAN_POINT('Ctrl Pts',(126.003758284155,-35.8579148149631,26.0315526658575));
#23811=CARTESIAN_POINT('Ctrl Pts',(125.977199802155,-35.7232852451568,26.0248581796344));
#23812=CARTESIAN_POINT('Ctrl Pts',(125.957461778018,-35.5874604019115,26.0181636934114));
#23813=CARTESIAN_POINT('Ctrl Pts',(125.937867450406,-35.4526243890526,26.0115179443062));
#23814=CARTESIAN_POINT('Ctrl Pts',(125.924994719631,-35.316610591759,26.004872195201));
#23815=CARTESIAN_POINT('Ctrl Pts',(125.91896982726,-35.1800492410075,25.9982264460959));
#23816=CARTESIAN_POINT('Ctrl Pts',(125.916367519001,-35.1210648294937,25.9953559736095));
#23817=CARTESIAN_POINT('Ctrl Pts',(125.915042131088,-35.0619784943742,25.9924855011231));
#23818=CARTESIAN_POINT('Ctrl Pts',(125.915000988625,-35.0028420178004,25.9896150286367));
#23819=CARTESIAN_POINT('Origin',(130.,-35.,32.7603849714045));
#23820=CARTESIAN_POINT('',(132.487160670875,-31.7594357285724,28.0469635236591));
#23821=CARTESIAN_POINT('',(132.487160670875,-31.7594357285724,27.9426397368634));
#23822=CARTESIAN_POINT('',(132.487160670875,-31.7594357285724,32.7603849714045));
#23823=CARTESIAN_POINT('',(125.915000279441,-34.9984890288179,27.1353849713731));
#23824=CARTESIAN_POINT('Ctrl Pts',(132.487160670875,-31.7594357285724,27.9426397368634));
#23825=CARTESIAN_POINT('Ctrl Pts',(132.581967877144,-31.8322010666427,27.9368366816923));
#23826=CARTESIAN_POINT('Ctrl Pts',(132.673586253723,-31.9091358676846,27.9310336265213));
#23827=CARTESIAN_POINT('Ctrl Pts',(132.761639006081,-31.989921097364,27.9252305713502));
#23828=CARTESIAN_POINT('Ctrl Pts',(132.849706643262,-32.0707199833336,27.9194265352053));
#23829=CARTESIAN_POINT('Ctrl Pts',(132.934207156769,-32.1553703162151,27.9136224990603));
#23830=CARTESIAN_POINT('Ctrl Pts',(133.014799632995,-32.2435152507423,27.9078184629153));
#23831=CARTESIAN_POINT('Ctrl Pts',(133.095475188514,-32.3317510500642,27.9020084436409));
#23832=CARTESIAN_POINT('Ctrl Pts',(133.172234383558,-32.4234883449647,27.8961984243665));
#23833=CARTESIAN_POINT('Ctrl Pts',(133.244775576362,-32.5183359496006,27.890388405092));
#23834=CARTESIAN_POINT('Ctrl Pts',(133.317354314023,-32.6132326441337,27.884575378749));
#23835=CARTESIAN_POINT('Ctrl Pts',(133.385710466145,-32.7112425208822,27.8787623524061));
#23836=CARTESIAN_POINT('Ctrl Pts',(133.449585855986,-32.8119455166326,27.8729493260631));
#23837=CARTESIAN_POINT('Ctrl Pts',(133.513564534955,-32.9128113532636,27.8671268998177));
#23838=CARTESIAN_POINT('Ctrl Pts',(133.573047769814,-33.0163786564525,27.8613044735724));
#23839=CARTESIAN_POINT('Ctrl Pts',(133.627823176215,-33.1222023532567,27.855482047327));
#23840=CARTESIAN_POINT('Ctrl Pts',(133.6783490715,-33.2198161798754,27.8501113286395));
#23841=CARTESIAN_POINT('Ctrl Pts',(133.724869706477,-33.3193493960304,27.8447406099519));
#23842=CARTESIAN_POINT('Ctrl Pts',(133.767255489786,-33.4204395944825,27.8393698912643));
#23843=CARTESIAN_POINT('Ctrl Pts',(133.813215309588,-33.5300538788457,27.8335463050565));
#23844=CARTESIAN_POINT('Ctrl Pts',(133.854461171478,-33.6418525051197,27.8277227188486));
#23845=CARTESIAN_POINT('Ctrl Pts',(133.890781146522,-33.7553928049892,27.8218991326408));
#23846=CARTESIAN_POINT('Ctrl Pts',(133.927055297774,-33.8687898545676,27.8160828938718));
#23847=CARTESIAN_POINT('Ctrl Pts',(133.958415800033,-33.9839238216377,27.8102666551029));
#23848=CARTESIAN_POINT('Ctrl Pts',(133.984698359438,-34.1003311807697,27.804450416334));
#23849=CARTESIAN_POINT('Ctrl Pts',(134.010954609366,-34.2166220133285,27.7986399997603));
#23850=CARTESIAN_POINT('Ctrl Pts',(134.032142939308,-34.3341833060769,27.7928295831866));
#23851=CARTESIAN_POINT('Ctrl Pts',(134.048148737625,-34.4525360303471,27.7870191666129));
#23852=CARTESIAN_POINT('Ctrl Pts',(134.064760418275,-34.575368870098,27.7809888029497));
#23853=CARTESIAN_POINT('Ctrl Pts',(134.075789319628,-34.6990538159745,27.7749584392865));
#23854=CARTESIAN_POINT('Ctrl Pts',(134.081165417872,-34.8230428527432,27.7689280756233));
#23855=CARTESIAN_POINT('Ctrl Pts',(134.086339601592,-34.9423751317172,27.7631241992668));
#23856=CARTESIAN_POINT('Ctrl Pts',(134.086277919101,-35.0619886269096,27.7573203229102));
#23857=CARTESIAN_POINT('Ctrl Pts',(134.080970805523,-35.181389868696,27.7515164465537));
#23858=CARTESIAN_POINT('Ctrl Pts',(134.075664475921,-35.3007734723626,27.7457134275539));
#23859=CARTESIAN_POINT('Ctrl Pts',(134.065114274316,-35.4199444771519,27.7399104085542));
#23860=CARTESIAN_POINT('Ctrl Pts',(134.049362739796,-35.5384109968717,27.7341073895544));
#23861=CARTESIAN_POINT('Ctrl Pts',(134.033609814721,-35.6568879748883,27.7283038582606));
#23862=CARTESIAN_POINT('Ctrl Pts',(134.0126546976,-35.7746599393862,27.7225003269668));
#23863=CARTESIAN_POINT('Ctrl Pts',(133.986591538575,-35.8912423377291,27.7166967956729));
#23864=CARTESIAN_POINT('Ctrl Pts',(133.960519927758,-36.0078625415514,27.7108913824031));
#23865=CARTESIAN_POINT('Ctrl Pts',(133.929337069791,-36.1232920137451,27.7050859691332));
#23866=CARTESIAN_POINT('Ctrl Pts',(133.893187582972,-36.2370591917086,27.6992805558633));
#23867=CARTESIAN_POINT('Ctrl Pts',(133.856998064044,-36.3509523559731,27.6934687136518));
#23868=CARTESIAN_POINT('Ctrl Pts',(133.815831061387,-36.4631791621531,27.6876568714403));
#23869=CARTESIAN_POINT('Ctrl Pts',(133.769880213874,-36.5732857887369,27.6818450292288));
#23870=CARTESIAN_POINT('Ctrl Pts',(133.723899185746,-36.6834647335877,27.676029369787));
#23871=CARTESIAN_POINT('Ctrl Pts',(133.673128228562,-36.7915203568409,27.6702137103452));
#23872=CARTESIAN_POINT('Ctrl Pts',(133.617807278788,-36.8970227973193,27.6643980509033));
#23873=CARTESIAN_POINT('Ctrl Pts',(133.562407087369,-37.0026763593348,27.6585740611197));
#23874=CARTESIAN_POINT('Ctrl Pts',(133.502444099556,-37.1057690873322,27.652750071336));
#23875=CARTESIAN_POINT('Ctrl Pts',(133.43820200028,-37.2058993642659,27.6469260815523));
#23876=CARTESIAN_POINT('Ctrl Pts',(133.421157360228,-37.2324658144272,27.6453808672669));
#23877=CARTESIAN_POINT('Ctrl Pts',(133.403811717253,-37.258823904402,27.6438356529814));
#23878=CARTESIAN_POINT('Ctrl Pts',(133.386170838292,-37.2849665323374,27.6422904386959));
#23879=CARTESIAN_POINT('Ctrl Pts',(133.31968597873,-37.3834927424374,27.636466842548));
#23880=CARTESIAN_POINT('Ctrl Pts',(133.248790165754,-37.4792736942146,27.6306432464));
#23881=CARTESIAN_POINT('Ctrl Pts',(133.173737464888,-37.571889481289,27.6248196502521));
#23882=CARTESIAN_POINT('Ctrl Pts',(133.098779453809,-37.6643884202153,27.6190034014091));
#23883=CARTESIAN_POINT('Ctrl Pts',(133.019675240873,-37.7537298225903,27.613187152566));
#23884=CARTESIAN_POINT('Ctrl Pts',(132.936722447597,-37.8395221896964,27.607370903723));
#23885=CARTESIAN_POINT('Ctrl Pts',(132.853852690199,-37.9252286785066,27.6015604769543));
#23886=CARTESIAN_POINT('Ctrl Pts',(132.767142298611,-38.0073929076184,27.5957500501856));
#23887=CARTESIAN_POINT('Ctrl Pts',(132.676929094683,-38.0856564329233,27.5899396234168));
#23888=CARTESIAN_POINT('Ctrl Pts',(132.583301189555,-38.1668823466824,27.5839092635298));
#23889=CARTESIAN_POINT('Ctrl Pts',(132.485900341863,-38.2439060792931,27.5778789036427));
#23890=CARTESIAN_POINT('Ctrl Pts',(132.385146510296,-38.3163686653362,27.5718485437557));
#23891=CARTESIAN_POINT('Ctrl Pts',(132.288176537885,-38.3861098837109,27.5660446569677));
#23892=CARTESIAN_POINT('Ctrl Pts',(132.188101247147,-38.4516261097104,27.5602407701796));
#23893=CARTESIAN_POINT('Ctrl Pts',(132.085328120449,-38.5126388413934,27.5544368833916));
#23894=CARTESIAN_POINT('Ctrl Pts',(131.982570174288,-38.5736425609341,27.5486338538911));
#23895=CARTESIAN_POINT('Ctrl Pts',(131.877115535678,-38.630143900653,27.5428308243906));
#23896=CARTESIAN_POINT('Ctrl Pts',(131.769398924054,-38.6819088048941,27.5370277948901));
#23897=CARTESIAN_POINT('Ctrl Pts',(131.661672802084,-38.7336782794812,27.5312242530376));
#23898=CARTESIAN_POINT('Ctrl Pts',(131.551684678089,-38.7807103102658,27.5254207111851));
#23899=CARTESIAN_POINT('Ctrl Pts',(131.439891429161,-38.8228180276112,27.5196171693326));
#23900=CARTESIAN_POINT('Ctrl Pts',(131.328061926951,-38.8649394000114,27.5138117454573));
#23901=CARTESIAN_POINT('Ctrl Pts',(131.214426517548,-38.9021331392433,27.5080063215821));
#23902=CARTESIAN_POINT('Ctrl Pts',(131.099458878302,-38.9342617064606,27.5022008977068));
#23903=CARTESIAN_POINT('Ctrl Pts',(130.984363923273,-38.9664258530264,27.4963890448739));
#23904=CARTESIAN_POINT('Ctrl Pts',(130.86793418704,-38.9935135211693,27.4905771920409));
#23905=CARTESIAN_POINT('Ctrl Pts',(130.750655380073,-39.015437896465,27.484765339208));
#23906=CARTESIAN_POINT('Ctrl Pts',(130.633299543836,-39.0373766717931,27.4789496691228));
#23907=CARTESIAN_POINT('Ctrl Pts',(130.515093929603,-39.0541453432434,27.4731339990377));
#23908=CARTESIAN_POINT('Ctrl Pts',(130.396529586751,-39.0657089525482,27.4673183289526));
#23909=CARTESIAN_POINT('Ctrl Pts',(130.277795413823,-39.0772891254219,27.4614943285746));
#23910=CARTESIAN_POINT('Ctrl Pts',(130.158701892992,-39.0836493333476,27.4556703281966));
#23911=CARTESIAN_POINT('Ctrl Pts',(130.039740432367,-39.0848066904121,27.4498463278186));
#23912=CARTESIAN_POINT('Ctrl Pts',(130.008179822116,-39.0851137385522,27.4483012139216));
#23913=CARTESIAN_POINT('Ctrl Pts',(129.976628478564,-39.0850548687037,27.4467561000245));
#23914=CARTESIAN_POINT('Ctrl Pts',(129.945095500927,-39.0846310109949,27.4452109861274));
#23915=CARTESIAN_POINT('Ctrl Pts',(129.826246487294,-39.0830334748794,27.4393873920245));
#23916=CARTESIAN_POINT('Ctrl Pts',(129.707275603482,-39.0762418978146,27.4335637979216));
#23917=CARTESIAN_POINT('Ctrl Pts',(129.588673316219,-39.0642385952611,27.4277402038187));
#23918=CARTESIAN_POINT('Ctrl Pts',(129.470220663076,-39.0522504366281,27.4219239570309));
#23919=CARTESIAN_POINT('Ctrl Pts',(129.352136084213,-39.0350636714838,27.4161077102431));
#23920=CARTESIAN_POINT('Ctrl Pts',(129.234910162847,-39.012712616309,27.4102914634554));
#23921=CARTESIAN_POINT('Ctrl Pts',(129.117801585011,-38.9903839346133,27.4044810387495));
#23922=CARTESIAN_POINT('Ctrl Pts',(129.001550353571,-38.9629013229485,27.3986706140437));
#23923=CARTESIAN_POINT('Ctrl Pts',(128.886641442207,-38.9303508395295,27.3928601893378));
#23924=CARTESIAN_POINT('Ctrl Pts',(128.767383003563,-38.8965682565809,27.3868298286804));
#23925=CARTESIAN_POINT('Ctrl Pts',(128.649570957648,-38.857326608824,27.3807994680229));
#23926=CARTESIAN_POINT('Ctrl Pts',(128.533735739328,-38.8127803658061,27.3747691073655));
#23927=CARTESIAN_POINT('Ctrl Pts',(128.422250822954,-38.7699070993704,27.3689652226458));
#23928=CARTESIAN_POINT('Ctrl Pts',(128.312597343979,-38.722120650378,27.3631613379261));
#23929=CARTESIAN_POINT('Ctrl Pts',(128.205231600146,-38.6696091605081,27.3573574532065));
#23930=CARTESIAN_POINT('Ctrl Pts',(128.097881715197,-38.6171054270566,27.3515544257726));
#23931=CARTESIAN_POINT('Ctrl Pts',(127.99281926009,-38.5598782200485,27.3457513983388));
#23932=CARTESIAN_POINT('Ctrl Pts',(127.890478289355,-38.4981628253007,27.339948370905));
#23933=CARTESIAN_POINT('Ctrl Pts',(127.788128282817,-38.4364419816295,27.3341448311152));
#23934=CARTESIAN_POINT('Ctrl Pts',(127.688500588084,-38.370232373222,27.3283412913254));
#23935=CARTESIAN_POINT('Ctrl Pts',(127.592001940681,-38.2998136835764,27.3225377515357));
#23936=CARTESIAN_POINT('Ctrl Pts',(127.495471999748,-38.2293721578649,27.3167323297169));
#23937=CARTESIAN_POINT('Ctrl Pts',(127.402073453869,-38.1547190768931,27.3109269078981));
#23938=CARTESIAN_POINT('Ctrl Pts',(127.312180989011,-38.0761752167533,27.3051214860793));
#23939=CARTESIAN_POINT('Ctrl Pts',(127.222188976412,-37.9975443764219,27.2993096352831));
#23940=CARTESIAN_POINT('Ctrl Pts',(127.135711102645,-37.9150144252529,27.2934977844868));
#23941=CARTESIAN_POINT('Ctrl Pts',(127.053086225347,-37.828944008771,27.2876859336906));
#23942=CARTESIAN_POINT('Ctrl Pts',(126.970407079494,-37.7428170606814,27.2818702656331));
#23943=CARTESIAN_POINT('Ctrl Pts',(126.891586238974,-37.653145322177,27.2760545975756));
#23944=CARTESIAN_POINT('Ctrl Pts',(126.81692211702,-37.5603203297405,27.2702389295181));
#23945=CARTESIAN_POINT('Ctrl Pts',(126.742151046706,-37.4673623754414,27.2644149311388));
#23946=CARTESIAN_POINT('Ctrl Pts',(126.671548819799,-37.3712424800554,27.2585909327595));
#23947=CARTESIAN_POINT('Ctrl Pts',(126.605370494355,-37.272381024257,27.2527669343802));
#23948=CARTESIAN_POINT('Ctrl Pts',(126.587813079664,-37.2461526244792,27.2512218007732));
#23949=CARTESIAN_POINT('Ctrl Pts',(126.570566795795,-37.2197313872462,27.2496766671661));
#23950=CARTESIAN_POINT('Ctrl Pts',(126.553635852833,-37.1931254330573,27.248131533559));
#23951=CARTESIAN_POINT('Ctrl Pts',(126.488371803247,-37.0905669212635,27.2421754756729));
#23952=CARTESIAN_POINT('Ctrl Pts',(126.427594206521,-36.9849433324307,27.2362194177869));
#23953=CARTESIAN_POINT('Ctrl Pts',(126.371595291619,-36.8766737255578,27.2302633599008));
#23954=CARTESIAN_POINT('Ctrl Pts',(126.315676623236,-36.7685592691748,27.2243158370535));
#23955=CARTESIAN_POINT('Ctrl Pts',(126.26452318171,-36.6578066792033,27.2183683142063));
#23956=CARTESIAN_POINT('Ctrl Pts',(126.21838365865,-36.5448633748115,27.212420791359));
#23957=CARTESIAN_POINT('Ctrl Pts',(126.172301362931,-36.4320601552009,27.2064806452876));
#23958=CARTESIAN_POINT('Ctrl Pts',(126.131220750067,-36.3170719829805,27.2005404992162));
#23959=CARTESIAN_POINT('Ctrl Pts',(126.095344190135,-36.2003699456776,27.1946003531448));
#23960=CARTESIAN_POINT('Ctrl Pts',(126.059514012327,-36.083818783723,27.1886678866446));
#23961=CARTESIAN_POINT('Ctrl Pts',(126.028874593329,-35.9655585367119,27.1827354201444));
#23962=CARTESIAN_POINT('Ctrl Pts',(126.003579608631,-35.8460786343174,27.1768029536441));
#23963=CARTESIAN_POINT('Ctrl Pts',(125.97830389398,-35.726689753263,27.1708750065739));
#23964=CARTESIAN_POINT('Ctrl Pts',(125.958364588432,-35.6060834401769,27.1649470595037));
#23965=CARTESIAN_POINT('Ctrl Pts',(125.943865134624,-35.4847627810422,27.1590191124334));
#23966=CARTESIAN_POINT('Ctrl Pts',(125.929375293527,-35.3635225539295,27.1530950954174));
#23967=CARTESIAN_POINT('Ctrl Pts',(125.920318164864,-35.2415693042346,27.1471710784014));
#23968=CARTESIAN_POINT('Ctrl Pts',(125.91674575583,-35.1194143101378,27.1412470613853));
#23969=CARTESIAN_POINT('Ctrl Pts',(125.915567400943,-35.0791216300713,27.1392930313917));
#23970=CARTESIAN_POINT('Ctrl Pts',(125.914985366504,-35.0388070499743,27.1373390013981));
#23971=CARTESIAN_POINT('Ctrl Pts',(125.915000279441,-34.9984890294654,27.1353849714045));
#23972=CARTESIAN_POINT('Ctrl Pts',(125.915000279441,-34.9984890288179,27.1353849713731));
#23973=CARTESIAN_POINT('Ctrl Pts',(125.915048271955,-34.8687384366259,27.1290965537963));
#23974=CARTESIAN_POINT('Ctrl Pts',(125.921282283113,-34.7391739314318,27.1228081362194));
#23975=CARTESIAN_POINT('Ctrl Pts',(125.933624288931,-34.6103673827449,27.1165197186425));
#23976=CARTESIAN_POINT('Ctrl Pts',(125.946018781103,-34.4810130636042,27.1102045585639));
#23977=CARTESIAN_POINT('Ctrl Pts',(125.96457324065,-34.3524234430616,27.1038893984853));
#23978=CARTESIAN_POINT('Ctrl Pts',(125.989158035434,-34.2251634138238,27.0975742384067));
#23979=CARTESIAN_POINT('Ctrl Pts',(126.013796778806,-34.0976241266608,27.0912452204144));
#23980=CARTESIAN_POINT('Ctrl Pts',(126.044492226841,-33.9714205392625,27.0849162024222));
#23981=CARTESIAN_POINT('Ctrl Pts',(126.081064803441,-33.8471028124032,27.0785871844299));
#23982=CARTESIAN_POINT('Ctrl Pts',(126.117752826942,-33.7223926577274,27.0722381879295));
#23983=CARTESIAN_POINT('Ctrl Pts',(126.160355004743,-33.5995805477314,27.0658891914291));
#23984=CARTESIAN_POINT('Ctrl Pts',(126.208642673094,-33.4791993491208,27.0595401949288));
#23985=CARTESIAN_POINT('Ctrl Pts',(126.230161623936,-33.4255525862153,27.056710823616));
#23986=CARTESIAN_POINT('Ctrl Pts',(126.252809073796,-33.3723882700398,27.0538814523033));
#23987=CARTESIAN_POINT('Ctrl Pts',(126.276561884102,-33.3197519239476,27.0510520809905));
#23988=CARTESIAN_POINT('Ctrl Pts',(126.325451445864,-33.211412411272,27.0452284869921));
#23989=CARTESIAN_POINT('Ctrl Pts',(126.379152242892,-33.1050337467732,27.0394048929937));
#23990=CARTESIAN_POINT('Ctrl Pts',(126.437484778255,-33.0010727139704,27.0335812989953));
#23991=CARTESIAN_POINT('Ctrl Pts',(126.495743718499,-32.897242843382,27.0277650523218));
#23992=CARTESIAN_POINT('Ctrl Pts',(126.558622576199,-32.7958248906842,27.0219488056483));
#23993=CARTESIAN_POINT('Ctrl Pts',(126.625894126307,-32.6972549960733,27.0161325589748));
#23994=CARTESIAN_POINT('Ctrl Pts',(126.693098337262,-32.5987837704124,27.0103221343928));
#23995=CARTESIAN_POINT('Ctrl Pts',(126.764686264268,-32.5031552666232,27.0045117098109));
#23996=CARTESIAN_POINT('Ctrl Pts',(126.840385476788,-32.4107798346396,26.9987012852289));
#23997=CARTESIAN_POINT('Ctrl Pts',(126.918950054951,-32.3149078089642,26.9926709245286));
#23998=CARTESIAN_POINT('Ctrl Pts',(127.001943089565,-32.2225403823583,26.9866405638283));
#23999=CARTESIAN_POINT('Ctrl Pts',(127.089011280693,-32.1341022914157,26.9806102031281));
#24000=CARTESIAN_POINT('Ctrl Pts',(127.17280954026,-32.0489855799698,26.9748063185556));
#24001=CARTESIAN_POINT('Ctrl Pts',(127.260382071063,-31.9675087036601,26.9690024339831));
#24002=CARTESIAN_POINT('Ctrl Pts',(127.35137428117,-31.8900149837096,26.9631985494106));
#24003=CARTESIAN_POINT('Ctrl Pts',(127.442353050778,-31.8125327103898,26.9573955221324));
#24004=CARTESIAN_POINT('Ctrl Pts',(127.536750184372,-31.7390326880646,26.9515924948542));
#24005=CARTESIAN_POINT('Ctrl Pts',(127.634176737621,-31.6698190302651,26.945789467576));
#24006=CARTESIAN_POINT('Ctrl Pts',(127.731611892633,-31.6005992616106,26.9399859279501));
#24007=CARTESIAN_POINT('Ctrl Pts',(127.832076666188,-31.5356668464153,26.9341823883242));
#24008=CARTESIAN_POINT('Ctrl Pts',(127.935152305295,-31.4752831322686,26.9283788486983));
#24009=CARTESIAN_POINT('Ctrl Pts',(128.03826137064,-31.4148798363808,26.9225734270515));
#24010=CARTESIAN_POINT('Ctrl Pts',(128.143982633231,-31.3590283814611,26.9167680054048));
#24011=CARTESIAN_POINT('Ctrl Pts',(128.251872449618,-31.3079443303769,26.910962583758));
#24012=CARTESIAN_POINT('Ctrl Pts',(128.359881743972,-31.2568037084433,26.9051507331451));
#24013=CARTESIAN_POINT('Ctrl Pts',(128.470064016391,-31.2104412034413,26.8993388825322));
#24014=CARTESIAN_POINT('Ctrl Pts',(128.58195519626,-31.1690244147754,26.8935270319193));
#24015=CARTESIAN_POINT('Ctrl Pts',(128.693919866853,-31.1275804233417,26.8877113640519));
#24016=CARTESIAN_POINT('Ctrl Pts',(128.807595292322,-31.0910887419833,26.8818956961845));
#24017=CARTESIAN_POINT('Ctrl Pts',(128.922503381796,-31.0596667605696,26.8760800283171));
#24018=CARTESIAN_POINT('Ctrl Pts',(129.037576064641,-31.028199770577,26.8702560301365));
#24019=CARTESIAN_POINT('Ctrl Pts',(129.153884538841,-31.0018170646865,26.8644320319559));
#24020=CARTESIAN_POINT('Ctrl Pts',(129.270941565394,-30.9805847690329,26.8586080337753));
#24021=CARTESIAN_POINT('Ctrl Pts',(129.301997365361,-30.9749517374578,26.8570628986576));
#24022=CARTESIAN_POINT('Ctrl Pts',(129.333105833546,-30.9696809423615,26.8555177635399));
#24023=CARTESIAN_POINT('Ctrl Pts',(129.364257843974,-30.9647730037764,26.8539726284221));
#24024=CARTESIAN_POINT('Ctrl Pts',(129.481684253281,-30.946272701638,26.8481482958581));
#24025=CARTESIAN_POINT('Ctrl Pts',(129.600108263132,-30.9328725377778,26.8423239632941));
#24026=CARTESIAN_POINT('Ctrl Pts',(129.719049255623,-30.9246728132291,26.8364996307302));
#24027=CARTESIAN_POINT('Ctrl Pts',(129.841350909668,-30.9162414065793,26.8305107324423));
#24028=CARTESIAN_POINT('Ctrl Pts',(129.964198789592,-30.9133088376121,26.8245218341545));
#24029=CARTESIAN_POINT('Ctrl Pts',(130.087058565302,-30.9159277912594,26.8185329358666));
#24030=CARTESIAN_POINT('Ctrl Pts',(130.206242809622,-30.9184683950457,26.8127232043038));
#24031=CARTESIAN_POINT('Ctrl Pts',(130.325437801707,-30.9262331086285,26.8069134727409));
#24032=CARTESIAN_POINT('Ctrl Pts',(130.444151130485,-30.9392174678655,26.801103741178));
#24033=CARTESIAN_POINT('Ctrl Pts',(130.562785662325,-30.9521932086283,26.7952978658718));
#24034=CARTESIAN_POINT('Ctrl Pts',(130.680938762273,-30.9703816604703,26.7894919905656));
#24035=CARTESIAN_POINT('Ctrl Pts',(130.79812060953,-30.9937263582421,26.7836861152593));
#24036=CARTESIAN_POINT('Ctrl Pts',(130.915252332796,-31.0170610704281,26.7778827233893));
#24037=CARTESIAN_POINT('Ctrl Pts',(131.031413230179,-31.0455475608967,26.7720793315192));
#24038=CARTESIAN_POINT('Ctrl Pts',(131.14612180951,-31.0790779403606,26.7662759396491));
#24039=CARTESIAN_POINT('Ctrl Pts',(131.26080839399,-31.1126018905265,26.7604736605531));
#24040=CARTESIAN_POINT('Ctrl Pts',(131.374042823382,-31.1511676892085,26.7546713814571));
#24041=CARTESIAN_POINT('Ctrl Pts',(131.485357570412,-31.1946172481577,26.7488691023611));
#24042=CARTESIAN_POINT('Ctrl Pts',(131.596710416444,-31.2380816783154,26.7430648373553));
#24043=CARTESIAN_POINT('Ctrl Pts',(131.706141886445,-31.286433060929,26.7372605723496));
#24044=CARTESIAN_POINT('Ctrl Pts',(131.813203480861,-31.3394647745183,26.7314563073438));
#24045=CARTESIAN_POINT('Ctrl Pts',(131.920288081564,-31.392507884004,26.7256507950693));
#24046=CARTESIAN_POINT('Ctrl Pts',(132.025001431504,-31.4502331367428,26.7198452827947));
#24047=CARTESIAN_POINT('Ctrl Pts',(132.126919781745,-31.5123880316151,26.7140397705201));
#24048=CARTESIAN_POINT('Ctrl Pts',(132.228918116506,-31.5745917050384,26.7082297021366));
#24049=CARTESIAN_POINT('Ctrl Pts',(132.328116731462,-31.6412317367213,26.702419633753));
#24050=CARTESIAN_POINT('Ctrl Pts',(132.42412112861,-31.712012507045,26.6966095653694));
#24051=CARTESIAN_POINT('Ctrl Pts',(132.445290832453,-31.7276202082552,26.6953284008536));
#24052=CARTESIAN_POINT('Ctrl Pts',(132.466305349192,-31.7434290916029,26.6940472363378));
#24053=CARTESIAN_POINT('Ctrl Pts',(132.487160670875,-31.7594357285724,26.6927660718219));
#24054=CARTESIAN_POINT('',(125.915000003014,-35.0001569306028,27.2396150285593));
#24055=CARTESIAN_POINT('Ctrl Pts',(125.915000003014,-35.0001569306028,27.2396150285593));
#24056=CARTESIAN_POINT('Ctrl Pts',(125.914995442009,-34.8814311542579,27.233798040467));
#24057=CARTESIAN_POINT('Ctrl Pts',(125.92017111884,-34.7625116039888,27.2279810523747));
#24058=CARTESIAN_POINT('Ctrl Pts',(125.930551771801,-34.6438874924847,27.2221640642824));
#24059=CARTESIAN_POINT('Ctrl Pts',(125.94091932464,-34.5254130816157,27.2163544170823));
#24060=CARTESIAN_POINT('Ctrl Pts',(125.956478754177,-34.4072337721956,27.2105447698822));
#24061=CARTESIAN_POINT('Ctrl Pts',(125.977202804404,-34.2898396497237,27.2047351226821));
#24062=CARTESIAN_POINT('Ctrl Pts',(125.997906137868,-34.1725628800947,27.1989312830863));
#24063=CARTESIAN_POINT('Ctrl Pts',(126.023763750967,-34.0560701368371,27.1931274434906));
#24064=CARTESIAN_POINT('Ctrl Pts',(126.054696570661,-33.9408466350681,27.1873236038948));
#24065=CARTESIAN_POINT('Ctrl Pts',(126.086567252157,-33.822129636033,27.1813437958773));
#24066=CARTESIAN_POINT('Ctrl Pts',(126.123825766704,-33.7047605122388,27.1753639878597));
#24067=CARTESIAN_POINT('Ctrl Pts',(126.166328678678,-33.5892593434404,27.1693841798421));
#24068=CARTESIAN_POINT('Ctrl Pts',(126.207534872779,-33.4772819903711,27.1635868092992));
#24069=CARTESIAN_POINT('Ctrl Pts',(126.253669957725,-33.3670606804676,27.1577894387562));
#24070=CARTESIAN_POINT('Ctrl Pts',(126.304552755601,-33.2590535149335,27.1519920682133));
#24071=CARTESIAN_POINT('Ctrl Pts',(126.355428250343,-33.1510618515125,27.1461955297586));
#24072=CARTESIAN_POINT('Ctrl Pts',(126.411049928465,-33.045284070752,27.1403989913039));
#24073=CARTESIAN_POINT('Ctrl Pts',(126.47118915546,-32.9421567058065,27.1346024528492));
#24074=CARTESIAN_POINT('Ctrl Pts',(126.531334034412,-32.8390196488263,27.1288053696288));
#24075=CARTESIAN_POINT('Ctrl Pts',(126.595997100056,-32.7385338565421,27.1230082864084));
#24076=CARTESIAN_POINT('Ctrl Pts',(126.664904942831,-32.641109167501,27.1172112031881));
#24077=CARTESIAN_POINT('Ctrl Pts',(126.73383562791,-32.5436521830885,27.1114121982889));
#24078=CARTESIAN_POINT('Ctrl Pts',(126.80701365207,-32.4492586539039,27.1056131933898));
#24079=CARTESIAN_POINT('Ctrl Pts',(126.88412407846,-32.358306936534,27.0998141884906));
#24080=CARTESIAN_POINT('Ctrl Pts',(126.961320033087,-32.2672543386412,27.0940087515343));
#24081=CARTESIAN_POINT('Ctrl Pts',(127.042456830683,-32.1796514845169,27.088203314578));
#24082=CARTESIAN_POINT('Ctrl Pts',(127.127181197167,-32.0958414082406,27.0823978776217));
#24083=CARTESIAN_POINT('Ctrl Pts',(127.211961991813,-32.011975512739,27.0765885741256));
#24084=CARTESIAN_POINT('Ctrl Pts',(127.300334810834,-31.9319076995307,27.0707792706295));
#24085=CARTESIAN_POINT('Ctrl Pts',(127.391912963374,-31.8559409977894,27.0649699671334));
#24086=CARTESIAN_POINT('Ctrl Pts',(127.483621027563,-31.779866530612,27.0591524226302));
#24087=CARTESIAN_POINT('Ctrl Pts',(127.57854317475,-31.7079050316072,27.0533348781271));
#24088=CARTESIAN_POINT('Ctrl Pts',(127.676263350047,-31.6403165354951,27.0475173336239));
#24089=CARTESIAN_POINT('Ctrl Pts',(127.6970313371,-31.6259522856575,27.0462809595738));
#24090=CARTESIAN_POINT('Ctrl Pts',(127.717925614027,-31.6117853855417,27.0450445855236));
#24091=CARTESIAN_POINT('Ctrl Pts',(127.738942050042,-31.5978180608714,27.0438082114734));
#24092=CARTESIAN_POINT('Ctrl Pts',(127.837934092804,-31.5320288851969,27.0379846173701));
#24093=CARTESIAN_POINT('Ctrl Pts',(127.939959515866,-31.4704577087745,27.0321610232669));
#24094=CARTESIAN_POINT('Ctrl Pts',(128.044623506418,-31.4133960675386,27.0263374291637));
#24095=CARTESIAN_POINT('Ctrl Pts',(128.149155448049,-31.3564064179026,27.0205211823755));
#24096=CARTESIAN_POINT('Ctrl Pts',(128.256318980633,-31.3039151810317,27.0147049355874));
#24097=CARTESIAN_POINT('Ctrl Pts',(128.365689833025,-31.2561710404826,27.0088886887992));
#24098=CARTESIAN_POINT('Ctrl Pts',(128.474951204838,-31.2084746919733,27.003078264093));
#24099=CARTESIAN_POINT('Ctrl Pts',(128.586415128783,-31.1655161489778,26.9972678393867));
#24100=CARTESIAN_POINT('Ctrl Pts',(128.699632747665,-31.1274982234923,26.9914574146805));
#24101=CARTESIAN_POINT('Ctrl Pts',(128.817135875086,-31.0880412450935,26.9854270540232));
#24102=CARTESIAN_POINT('Ctrl Pts',(128.936527688634,-31.0539065129513,26.9793966933659));
#24103=CARTESIAN_POINT('Ctrl Pts',(129.057283182286,-31.0252660464379,26.9733663327086));
#24104=CARTESIAN_POINT('Ctrl Pts',(129.17350358838,-30.9977011999184,26.9675624479884));
#24105=CARTESIAN_POINT('Ctrl Pts',(129.29098666009,-30.9752254791916,26.9617585632682));
#24106=CARTESIAN_POINT('Ctrl Pts',(129.40924956635,-30.9579412516463,26.955954678548));
#24107=CARTESIAN_POINT('Ctrl Pts',(129.527495004119,-30.9406595771364,26.9501516511137));
#24108=CARTESIAN_POINT('Ctrl Pts',(129.646519643429,-30.9285679298605,26.9443486236793));
#24109=CARTESIAN_POINT('Ctrl Pts',(129.7658323915,-30.9217172080483,26.938545596245));
#24110=CARTESIAN_POINT('Ctrl Pts',(129.885155673832,-30.9148658813779,26.9327420564546));
#24111=CARTESIAN_POINT('Ctrl Pts',(130.004766707816,-30.9132564235935,26.9269385166643));
#24112=CARTESIAN_POINT('Ctrl Pts',(130.124171878948,-30.9168876644796,26.9211349768739));
#24113=CARTESIAN_POINT('Ctrl Pts',(130.243615771964,-30.9205200829403,26.9153295550545));
#24114=CARTESIAN_POINT('Ctrl Pts',(130.362853261423,-30.9293965675983,26.9095241332352));
#24115=CARTESIAN_POINT('Ctrl Pts',(130.481393981588,-30.9434639364982,26.9037187114158));
#24116=CARTESIAN_POINT('Ctrl Pts',(130.600065974837,-30.9575468837317,26.8979068606189));
#24117=CARTESIAN_POINT('Ctrl Pts',(130.718039252864,-30.9768321414227,26.8920950098221));
#24118=CARTESIAN_POINT('Ctrl Pts',(130.834831637392,-31.0012150423897,26.8862831590252));
#24119=CARTESIAN_POINT('Ctrl Pts',(130.951700731915,-31.0256139582044,26.880467490967));
#24120=CARTESIAN_POINT('Ctrl Pts',(131.067386993512,-31.0551170845753,26.8746518229088));
#24121=CARTESIAN_POINT('Ctrl Pts',(131.181423052239,-31.0895697715419,26.8688361548507));
#24122=CARTESIAN_POINT('Ctrl Pts',(131.295622455409,-31.1240718082937,26.8630121564707));
#24123=CARTESIAN_POINT('Ctrl Pts',(131.408166553851,-31.1635374216842,26.8571881580907));
#24124=CARTESIAN_POINT('Ctrl Pts',(131.518607473302,-31.2077636753452,26.8513641597107));
#24125=CARTESIAN_POINT('Ctrl Pts',(131.547907958044,-31.219497104196,26.8498190261087));
#24126=CARTESIAN_POINT('Ctrl Pts',(131.577060541274,-31.2315653670552,26.8482738925068));
#24127=CARTESIAN_POINT('Ctrl Pts',(131.606057163059,-31.2439641390173,26.8467287589049));
#24128=CARTESIAN_POINT('Ctrl Pts',(131.71534415369,-31.2906945645586,26.8409052183997));
#24129=CARTESIAN_POINT('Ctrl Pts',(131.822766155584,-31.3422740861352,26.8350816778945));
#24130=CARTESIAN_POINT('Ctrl Pts',(131.927862926942,-31.3985323082215,26.8292581373893));
#24131=CARTESIAN_POINT('Ctrl Pts',(132.032811661674,-31.4547112864148,26.8234427997744));
#24132=CARTESIAN_POINT('Ctrl Pts',(132.135441326964,-31.5155556592987,26.8176274621594));
#24133=CARTESIAN_POINT('Ctrl Pts',(132.235311565566,-31.5808470047619,26.8118121245445));
#24134=CARTESIAN_POINT('Ctrl Pts',(132.321400919049,-31.6371289341695,26.806799233191));
#24135=CARTESIAN_POINT('Ctrl Pts',(132.405439988716,-31.6967144091857,26.8017863418376));
#24136=CARTESIAN_POINT('Ctrl Pts',(132.487160670875,-31.7594357285724,26.7967734504842));
#24137=CARTESIAN_POINT('Ctrl Pts',(132.487160670875,-31.7594357285724,28.0469635236591));
#24138=CARTESIAN_POINT('Ctrl Pts',(132.583285464304,-31.8332123260063,28.0410441738779));
#24139=CARTESIAN_POINT('Ctrl Pts',(132.675995739581,-31.9111704788722,28.0351248240968));
#24140=CARTESIAN_POINT('Ctrl Pts',(132.764929491174,-31.9929433146618,28.0292054743156));
#24141=CARTESIAN_POINT('Ctrl Pts',(132.852423570101,-32.0733923997447,28.0233819478403));
#24142=CARTESIAN_POINT('Ctrl Pts',(132.936544708698,-32.1577930401039,28.017558421365));
#24143=CARTESIAN_POINT('Ctrl Pts',(133.016915641834,-32.2458313395763,28.0117348948897));
#24144=CARTESIAN_POINT('Ctrl Pts',(133.097185160871,-32.3337585500728,28.0059187166889));
#24145=CARTESIAN_POINT('Ctrl Pts',(133.1737136136,-32.4253139911846,28.0001025384881));
#24146=CARTESIAN_POINT('Ctrl Pts',(133.246158326206,-32.5201449394763,27.9942863602873));
#24147=CARTESIAN_POINT('Ctrl Pts',(133.318530509731,-32.6148809463805,27.9884760050381));
#24148=CARTESIAN_POINT('Ctrl Pts',(133.386826840217,-32.7128856140347,27.982665649789));
#24149=CARTESIAN_POINT('Ctrl Pts',(133.450743329231,-32.8137714035883,27.9768552945399));
#24150=CARTESIAN_POINT('Ctrl Pts',(133.517080258284,-32.9184776158247,27.9708249081735));
#24151=CARTESIAN_POINT('Ctrl Pts',(133.57869876802,-33.0262871414312,27.9647945218072));
#24152=CARTESIAN_POINT('Ctrl Pts',(133.635306602846,-33.1367311242586,27.9587641354408));
#24153=CARTESIAN_POINT('Ctrl Pts',(133.689787576045,-33.2430255212621,27.9529603219047));
#24154=CARTESIAN_POINT('Ctrl Pts',(133.739627399038,-33.3517595880501,27.9471565083687));
#24155=CARTESIAN_POINT('Ctrl Pts',(133.784611529896,-33.4624888397864,27.9413526948326));
#24156=CARTESIAN_POINT('Ctrl Pts',(133.829589012122,-33.5732017257961,27.9355497390972));
#24157=CARTESIAN_POINT('Ctrl Pts',(133.869712075777,-33.6859088320985,27.9297467833618));
#24158=CARTESIAN_POINT('Ctrl Pts',(133.904814193391,-33.8001453775171,27.9239438276264));
#24159=CARTESIAN_POINT('Ctrl Pts',(133.939919407601,-33.9143920005167,27.9181403599728));
#24160=CARTESIAN_POINT('Ctrl Pts',(133.970002675169,-34.0301679405346,27.9123368923193));
#24161=CARTESIAN_POINT('Ctrl Pts',(133.994947433845,-34.1469935517149,27.9065334246658));
#24162=CARTESIAN_POINT('Ctrl Pts',(134.019900280401,-34.2638570414536,27.9007280753445));
#24163=CARTESIAN_POINT('Ctrl Pts',(134.039711219411,-34.3817704800661,27.8949227260232));
#24164=CARTESIAN_POINT('Ctrl Pts',(134.054314974779,-34.5002449747268,27.8891173767019));
#24165=CARTESIAN_POINT('Ctrl Pts',(134.068934902246,-34.6188506672473,27.8833055985757));
#24166=CARTESIAN_POINT('Ctrl Pts',(134.078336085858,-34.7380182504821,27.8774938204496));
#24167=CARTESIAN_POINT('Ctrl Pts',(134.082505201968,-34.8572545065437,27.8716820423234));
#24168=CARTESIAN_POINT('Ctrl Pts',(134.086677056282,-34.976569074918,27.8658664471218));
#24169=CARTESIAN_POINT('Ctrl Pts',(134.085610003201,-35.09595199855,27.8600508519202));
#24170=CARTESIAN_POINT('Ctrl Pts',(134.079342791129,-35.214912522814,27.8542352567186));
#24171=CARTESIAN_POINT('Ctrl Pts',(134.073066601531,-35.3340434531873,27.8484113309136));
#24172=CARTESIAN_POINT('Ctrl Pts',(134.061575424321,-35.4527503715008,27.8425874051085));
#24173=CARTESIAN_POINT('Ctrl Pts',(134.044959550162,-35.5705499430857,27.8367634793035));
#24174=CARTESIAN_POINT('Ctrl Pts',(134.040549271268,-35.6018169687812,27.835217660118));
#24175=CARTESIAN_POINT('Ctrl Pts',(134.035778229449,-35.6330201415283,27.8336718409326));
#24176=CARTESIAN_POINT('Ctrl Pts',(134.030648706208,-35.6641505907097,27.8321260217471));
#24177=CARTESIAN_POINT('Ctrl Pts',(134.011324098236,-35.7814292729995,27.8263024103989));
#24178=CARTESIAN_POINT('Ctrl Pts',(133.986845442312,-35.8980529423074,27.8204787990506));
#24179=CARTESIAN_POINT('Ctrl Pts',(133.957268484404,-36.013533986771,27.8146551877024));
#24180=CARTESIAN_POINT('Ctrl Pts',(133.927728841429,-36.1288693378441,27.8088389235485));
#24181=CARTESIAN_POINT('Ctrl Pts',(133.893103790243,-36.2430645392233,27.8030226593946));
#24182=CARTESIAN_POINT('Ctrl Pts',(133.853500512317,-36.3556396282095,27.7972063952408));
#24183=CARTESIAN_POINT('Ctrl Pts',(133.813936876611,-36.4681020314088,27.7913959530703));
#24184=CARTESIAN_POINT('Ctrl Pts',(133.7694050622,-36.5789471654182,27.7855855108999));
#24185=CARTESIAN_POINT('Ctrl Pts',(133.720062574716,-36.6877083397909,27.7797750687295));
#24186=CARTESIAN_POINT('Ctrl Pts',(133.668852586673,-36.8005858764355,27.7737447145815));
#24187=CARTESIAN_POINT('Ctrl Pts',(133.612460696619,-36.9112181565411,27.7677143604336));
#24188=CARTESIAN_POINT('Ctrl Pts',(133.551118839586,-37.0191037583881,27.7616840062856));
#24189=CARTESIAN_POINT('Ctrl Pts',(133.492080491692,-37.1229380406002,27.7558801039695));
#24190=CARTESIAN_POINT('Ctrl Pts',(133.428457455569,-37.2242278244811,27.7500762016534));
#24191=CARTESIAN_POINT('Ctrl Pts',(133.36050389423,-37.3225500160098,27.7442722993372));
#24192=CARTESIAN_POINT('Ctrl Pts',(133.292560370003,-37.4208576848121,27.7384692542893));
#24193=CARTESIAN_POINT('Ctrl Pts',(133.220287824704,-37.5161982971386,27.7326662092413));
#24194=CARTESIAN_POINT('Ctrl Pts',(133.143983715939,-37.6081777918516,27.7268631641934));
#24195=CARTESIAN_POINT('Ctrl Pts',(133.06767287024,-37.7001654074883,27.7210596067912));
#24196=CARTESIAN_POINT('Ctrl Pts',(132.987330014086,-37.7887910012047,27.715256049389));
#24197=CARTESIAN_POINT('Ctrl Pts',(132.903292426176,-37.8736941535434,27.7094524919868));
#24198=CARTESIAN_POINT('Ctrl Pts',(132.819227586119,-37.9586248387187,27.7036470525767));
#24199=CARTESIAN_POINT('Ctrl Pts',(132.731465918567,-38.0398303917396,27.6978416131667));
#24200=CARTESIAN_POINT('Ctrl Pts',(132.640380548991,-38.1169882188601,27.6920361737567));
#24201=CARTESIAN_POINT('Ctrl Pts',(132.549194312839,-38.1942314894038,27.6862243054899));
#24202=CARTESIAN_POINT('Ctrl Pts',(132.454677339591,-38.2674178227229,27.6804124372231));
#24203=CARTESIAN_POINT('Ctrl Pts',(132.357234850278,-38.3362657059409,27.6746005689564));
#24204=CARTESIAN_POINT('Ctrl Pts',(132.259728361135,-38.405158808168,27.6687848834782));
#24205=CARTESIAN_POINT('Ctrl Pts',(132.159292871994,-38.4697075652274,27.662969198));
#24206=CARTESIAN_POINT('Ctrl Pts',(132.056360087618,-38.5296753660996,27.6571535125219));
#24207=CARTESIAN_POINT('Ctrl Pts',(131.953279867147,-38.5897290620387,27.6513294969285));
#24208=CARTESIAN_POINT('Ctrl Pts',(131.847695572142,-38.6451885160911,27.645505481335));
#24209=CARTESIAN_POINT('Ctrl Pts',(131.740060955099,-38.695864293036,27.6396814657416));
#24210=CARTESIAN_POINT('Ctrl Pts',(131.711508186047,-38.7093073078893,27.6381365002207));
#24211=CARTESIAN_POINT('Ctrl Pts',(131.682811226506,-38.7224139605503,27.6365915346997));
#24212=CARTESIAN_POINT('Ctrl Pts',(131.653978731678,-38.7351813015111,27.6350465691787));
#24213=CARTESIAN_POINT('Ctrl Pts',(131.545297395498,-38.7833065741717,27.6292229691686));
#24214=CARTESIAN_POINT('Ctrl Pts',(131.434338636625,-38.8267621156396,27.6233993691585));
#24215=CARTESIAN_POINT('Ctrl Pts',(131.32154083558,-38.8653272590938,27.6175757691484));
#24216=CARTESIAN_POINT('Ctrl Pts',(131.208885342653,-38.9038437479384,27.6117595163166));
#24217=CARTESIAN_POINT('Ctrl Pts',(131.0943958053,-38.9374819794818,27.6059432634847));
#24218=CARTESIAN_POINT('Ctrl Pts',(130.978532401663,-38.966068499017,27.6001270106529));
#24219=CARTESIAN_POINT('Ctrl Pts',(130.862784974987,-38.9946264040154,27.5943165797744));
#24220=CARTESIAN_POINT('Ctrl Pts',(130.745666812013,-39.0181425593596,27.5885061488959));
#24221=CARTESIAN_POINT('Ctrl Pts',(130.627654576307,-39.0364928753611,27.5826957180173));
#24222=CARTESIAN_POINT('Ctrl Pts',(130.505175522547,-39.0555377593652,27.5766653596254));
#24223=CARTESIAN_POINT('Ctrl Pts',(130.381733800796,-39.0690178737889,27.5706350012334));
#24224=CARTESIAN_POINT('Ctrl Pts',(130.257875926543,-39.076852340533,27.5646046428414));
#24225=CARTESIAN_POINT('Ctrl Pts',(130.138669475346,-39.0843925876366,27.5588007516663));
#24226=CARTESIAN_POINT('Ctrl Pts',(130.019078008971,-39.086703551476,27.5529968604911));
#24227=CARTESIAN_POINT('Ctrl Pts',(129.899594712356,-39.0837658819052,27.5471929693159));
#24228=CARTESIAN_POINT('Ctrl Pts',(129.780129062552,-39.0808286462068,27.5413899353331));
#24229=CARTESIAN_POINT('Ctrl Pts',(129.660771958839,-39.07264432873,27.5355869013503));
#24230=CARTESIAN_POINT('Ctrl Pts',(129.542016036404,-39.0592457044491,27.5297838673675));
#24231=CARTESIAN_POINT('Ctrl Pts',(129.423249627108,-39.0458458969894,27.5239803209419));
#24232=CARTESIAN_POINT('Ctrl Pts',(129.305084910422,-39.0272309130128,27.5181767745164));
#24233=CARTESIAN_POINT('Ctrl Pts',(129.18800821304,-39.0034852738469,27.5123732280909));
#24234=CARTESIAN_POINT('Ctrl Pts',(129.070893547304,-38.979731933893,27.5065677995564));
#24235=CARTESIAN_POINT('Ctrl Pts',(128.954868002589,-38.9508447107762,27.5007623710218));
#24236=CARTESIAN_POINT('Ctrl Pts',(128.840405919094,-38.9169588416945,27.4949569424873));
#24237=CARTESIAN_POINT('Ctrl Pts',(128.725817077699,-38.8830354466347,27.4891450848899));
#24238=CARTESIAN_POINT('Ctrl Pts',(128.612795545343,-38.8441024720326,27.4833332272925));
#24239=CARTESIAN_POINT('Ctrl Pts',(128.50179889693,-38.8003445179036,27.4775213696951));
#24240=CARTESIAN_POINT('Ctrl Pts',(128.39072934418,-38.7565578228647,27.4717056947785));
#24241=CARTESIAN_POINT('Ctrl Pts',(128.281687696141,-38.7079400028129,27.465890019862));
#24242=CARTESIAN_POINT('Ctrl Pts',(128.175108490418,-38.6547224215056,27.4600743449455));
#24243=CARTESIAN_POINT('Ctrl Pts',(128.06837662097,-38.6014286114995,27.4542503396742));
#24244=CARTESIAN_POINT('Ctrl Pts',(127.964114589634,-38.5435220871408,27.4484263344029));
#24245=CARTESIAN_POINT('Ctrl Pts',(127.86272956321,-38.4812785122744,27.4426023291316));
#24246=CARTESIAN_POINT('Ctrl Pts',(127.835832772996,-38.4647656953982,27.4410572582911));
#24247=CARTESIAN_POINT('Ctrl Pts',(127.809138293843,-38.4479478588015,27.4395121874507));
#24248=CARTESIAN_POINT('Ctrl Pts',(127.782653338569,-38.4308306258164,27.4379671166102));
#24249=CARTESIAN_POINT('Ctrl Pts',(127.682827870727,-38.3663134018596,27.4321435304308));
#24250=CARTESIAN_POINT('Ctrl Pts',(127.585659606409,-38.2973316490775,27.4263199442514));
#24251=CARTESIAN_POINT('Ctrl Pts',(127.491573408628,-38.22413105126,27.4204963580719));
#24252=CARTESIAN_POINT('Ctrl Pts',(127.397605916506,-38.1510228083828,27.4146801193319));
#24253=CARTESIAN_POINT('Ctrl Pts',(127.306713076136,-38.0737065559006,27.4088638805918));
#24254=CARTESIAN_POINT('Ctrl Pts',(127.219292212636,-37.9924720886408,27.4030476418517));
#24255=CARTESIAN_POINT('Ctrl Pts',(127.131958859535,-37.9113189390471,27.3972372253073));
#24256=CARTESIAN_POINT('Ctrl Pts',(127.048090866573,-37.8262556538245,27.3914268087628));
#24257=CARTESIAN_POINT('Ctrl Pts',(126.968053308347,-37.737612876024,27.3856163922184));
#24258=CARTESIAN_POINT('Ctrl Pts',(126.884986013602,-37.6456146202838,27.3795860285444));
#24259=CARTESIAN_POINT('Ctrl Pts',(126.806045231511,-37.5497607967383,27.3735556648704));
#24260=CARTESIAN_POINT('Ctrl Pts',(126.731598189897,-37.4504641616877,27.3675253011963));
#24261=CARTESIAN_POINT('Ctrl Pts',(126.659947217293,-37.3548968923447,27.3617214248698));
#24262=CARTESIAN_POINT('Ctrl Pts',(126.592458789477,-37.256141112707,27.3559175485433));
#24263=CARTESIAN_POINT('Ctrl Pts',(126.529419436531,-37.154598698707,27.3501136722168));
#24264=CARTESIAN_POINT('Ctrl Pts',(126.46638939585,-37.0530712846997,27.3443106532473));
#24265=CARTESIAN_POINT('Ctrl Pts',(126.407807338344,-36.9487584017903,27.3385076342779));
#24266=CARTESIAN_POINT('Ctrl Pts',(126.353915896904,-36.8420900393705,27.3327046153084));
#24267=CARTESIAN_POINT('Ctrl Pts',(126.300019697896,-36.7354122602064,27.326901084045));
#24268=CARTESIAN_POINT('Ctrl Pts',(126.250815122409,-36.6263789525728,27.3210975527817));
#24269=CARTESIAN_POINT('Ctrl Pts',(126.206498066165,-36.5154431952367,27.3152940215184));
#24270=CARTESIAN_POINT('Ctrl Pts',(126.162166638734,-36.404471463524,27.3094886082791));
#24271=CARTESIAN_POINT('Ctrl Pts',(126.122726034021,-36.2915964341819,27.3036831950399));
#24272=CARTESIAN_POINT('Ctrl Pts',(126.088323159943,-36.1772889615392,27.2978777818007));
#24273=CARTESIAN_POINT('Ctrl Pts',(126.053882187963,-36.0628549042724,27.29206593962));
#24274=CARTESIAN_POINT('Ctrl Pts',(126.024490200144,-35.9469856285703,27.2862540974393));
#24275=CARTESIAN_POINT('Ctrl Pts',(126.000243628667,-35.8301650257512,27.2804422552586));
#24276=CARTESIAN_POINT('Ctrl Pts',(125.975981131991,-35.7132676949128,27.2746265958477));
#24277=CARTESIAN_POINT('Ctrl Pts',(125.956870847267,-35.595418194732,27.2688109364367));
#24278=CARTESIAN_POINT('Ctrl Pts',(125.942957466631,-35.4771067830487,27.2629952770258));
#24279=CARTESIAN_POINT('Ctrl Pts',(125.929024156488,-35.3586259022743,27.2571712872729));
#24280=CARTESIAN_POINT('Ctrl Pts',(125.920302638081,-35.2396821951967,27.25134729752));
#24281=CARTESIAN_POINT('Ctrl Pts',(125.91678554855,-35.12076731126,27.2455233077671));
#24282=CARTESIAN_POINT('Ctrl Pts',(125.915852398212,-35.0892169446464,27.243978093192));
#24283=CARTESIAN_POINT('Ctrl Pts',(125.915285325465,-35.0576685843124,27.2424328786169));
#24284=CARTESIAN_POINT('Ctrl Pts',(125.915083580701,-35.0261313479364,27.2408876640418));
#24285=CARTESIAN_POINT('Ctrl Pts',(125.915028195182,-35.0174733476091,27.2404634522263));
#24286=CARTESIAN_POINT('Ctrl Pts',(125.915000335634,-35.0088151710232,27.2400392404109));
#24287=CARTESIAN_POINT('Ctrl Pts',(125.915000003014,-35.0001569313426,27.2396150285955));
#24288=CARTESIAN_POINT('Origin',(130.,-35.,32.7603849714045));
#24289=CARTESIAN_POINT('',(132.487160670875,-31.7594357285724,29.296931249476));
#24290=CARTESIAN_POINT('',(132.487160670875,-31.7594357285724,29.1925548588025));
#24291=CARTESIAN_POINT('',(132.487160670875,-31.7594357285724,32.7603849714045));
#24292=CARTESIAN_POINT('',(125.917751433657,-35.0038808860531,29.7396160660207));
#24293=CARTESIAN_POINT('Ctrl Pts',(125.915001825726,-35.0038621470065,29.7396150285955));
#24294=CARTESIAN_POINT('Ctrl Pts',(125.914889706146,-34.88527311404,29.7338556330042));
#24295=CARTESIAN_POINT('Ctrl Pts',(125.919945886409,-34.7666043470561,29.7280962374129));
#24296=CARTESIAN_POINT('Ctrl Pts',(125.930164310688,-34.6483432611132,29.7223368418217));
#24297=CARTESIAN_POINT('Ctrl Pts',(125.940380151039,-34.5301120797944,29.716578902606));
#24298=CARTESIAN_POINT('Ctrl Pts',(125.955755605104,-34.4122887877864,29.7108209633903));
#24299=CARTESIAN_POINT('Ctrl Pts',(125.976232588964,-34.2953576638563,29.7050630241746));
#24300=CARTESIAN_POINT('Ctrl Pts',(125.99670941053,-34.1784274666885,29.6993051305947));
#24301=CARTESIAN_POINT('Ctrl Pts',(126.022287609829,-34.0623898323388,29.6935472370148));
#24302=CARTESIAN_POINT('Ctrl Pts',(126.052857746502,-33.9477200797059,29.6877893434349));
#24303=CARTESIAN_POINT('Ctrl Pts',(126.083435129142,-33.8330231471781,29.6820300850753));
#24304=CARTESIAN_POINT('Ctrl Pts',(126.11900669447,-33.7196951418414,29.6762708267158));
#24305=CARTESIAN_POINT('Ctrl Pts',(126.159412985297,-33.6081967155889,29.6705115683562));
#24306=CARTESIAN_POINT('Ctrl Pts',(126.199864385646,-33.4965738126658,29.6647458803696));
#24307=CARTESIAN_POINT('Ctrl Pts',(126.245161147391,-33.3867849580306,29.6589801923829));
#24308=CARTESIAN_POINT('Ctrl Pts',(126.295095376145,-33.2792714542557,29.6532145043962));
#24309=CARTESIAN_POINT('Ctrl Pts',(126.345059189201,-33.1716942524512,29.647445400439));
#24310=CARTESIAN_POINT('Ctrl Pts',(126.399665748915,-33.0663954535246,29.6416762964818));
#24311=CARTESIAN_POINT('Ctrl Pts',(126.458661736905,-32.9637907017352,29.6359071925245));
#24312=CARTESIAN_POINT('Ctrl Pts',(126.517754586706,-32.8610174896421,29.6301286166375));
#24313=CARTESIAN_POINT('Ctrl Pts',(126.581251035677,-32.7609475085123,29.6243500407505));
#24314=CARTESIAN_POINT('Ctrl Pts',(126.648854860074,-32.6639667701102,29.6185714648635));
#24315=CARTESIAN_POINT('Ctrl Pts',(126.698499254289,-32.5927496451699,29.6143280081967));
#24316=CARTESIAN_POINT('Ctrl Pts',(126.750357702169,-32.5231977812645,29.6100845515299));
#24317=CARTESIAN_POINT('Ctrl Pts',(126.804299925717,-32.4554517031058,29.6058410948631));
#24318=CARTESIAN_POINT('Ctrl Pts',(126.878347621069,-32.362455148147,29.6000160070964));
#24319=CARTESIAN_POINT('Ctrl Pts',(126.956578253727,-32.2725425605472,29.5941909193296));
#24320=CARTESIAN_POINT('Ctrl Pts',(127.038705676932,-32.1861128430297,29.5883658315628));
#24321=CARTESIAN_POINT('Ctrl Pts',(127.120728387972,-32.0997933230852,29.5825481707616));
#24322=CARTESIAN_POINT('Ctrl Pts',(127.206637728886,-32.0169481340628,29.5767305099604));
#24323=CARTESIAN_POINT('Ctrl Pts',(127.296106343381,-31.9379444659358,29.5709128491592));
#24324=CARTESIAN_POINT('Ctrl Pts',(127.385484176038,-31.8590209610953,29.5651010914106));
#24325=CARTESIAN_POINT('Ctrl Pts',(127.478413793455,-31.7839314912864,29.559289333662));
#24326=CARTESIAN_POINT('Ctrl Pts',(127.574530335048,-31.7130071639266,29.5534775759134));
#24327=CARTESIAN_POINT('Ctrl Pts',(127.674253428406,-31.6394215645971,29.5474477453459));
#24328=CARTESIAN_POINT('Ctrl Pts',(127.777406988163,-31.5703201313939,29.5414179147785));
#24329=CARTESIAN_POINT('Ctrl Pts',(127.883544615322,-31.5060278185615,29.535388084211));
#24330=CARTESIAN_POINT('Ctrl Pts',(127.985724855635,-31.4441326721242,29.5295830784565));
#24331=CARTESIAN_POINT('Ctrl Pts',(128.090670241815,-31.3866946760441,29.523778072702));
#24332=CARTESIAN_POINT('Ctrl Pts',(128.197952699211,-31.3339598303184,29.5179730669474));
#24333=CARTESIAN_POINT('Ctrl Pts',(128.305217823592,-31.281233504661,29.5121689990746));
#24334=CARTESIAN_POINT('Ctrl Pts',(128.414818902106,-31.2332089981539,29.5063649312017));
#24335=CARTESIAN_POINT('Ctrl Pts',(128.526304156129,-31.1900858855144,29.5005608633288));
#24336=CARTESIAN_POINT('Ctrl Pts',(128.637797675485,-31.1469595757983,29.4947563651519));
#24337=CARTESIAN_POINT('Ctrl Pts',(128.751175267391,-31.1087355295797,29.488951866975));
#24338=CARTESIAN_POINT('Ctrl Pts',(128.865966722983,-31.0755645595043,29.4831473687981));
#24339=CARTESIAN_POINT('Ctrl Pts',(128.98079374545,-31.0423833117676,29.4773410721611));
#24340=CARTESIAN_POINT('Ctrl Pts',(129.097035110911,-31.0142583670542,29.4715347755241));
#24341=CARTESIAN_POINT('Ctrl Pts',(129.214207684855,-30.9912900532143,29.4657284788871));
#24342=CARTESIAN_POINT('Ctrl Pts',(129.331507394359,-30.9682968181035,29.4599158822538));
#24343=CARTESIAN_POINT('Ctrl Pts',(129.44973992843,-30.9504714607943,29.4541032856206));
#24344=CARTESIAN_POINT('Ctrl Pts',(129.568414095604,-30.9378628030153,29.4482906889873));
#24345=CARTESIAN_POINT('Ctrl Pts',(129.687164680749,-30.9252460261311,29.442474349443));
#24346=CARTESIAN_POINT('Ctrl Pts',(129.806357058913,-30.917852664184,29.4366580098987));
#24347=CARTESIAN_POINT('Ctrl Pts',(129.925498726576,-30.9156794248911,29.4308416703545));
#24348=CARTESIAN_POINT('Ctrl Pts',(130.044808685338,-30.9135031158339,29.4250171150601));
#24349=CARTESIAN_POINT('Ctrl Pts',(130.164067384022,-30.9165616364723,29.4191925597657));
#24350=CARTESIAN_POINT('Ctrl Pts',(130.282785995545,-30.9247997496168,29.4133680044714));
#24351=CARTESIAN_POINT('Ctrl Pts',(130.314082285943,-30.9269714594944,29.4118325504125));
#24352=CARTESIAN_POINT('Ctrl Pts',(130.345341092885,-30.9295028438761,29.4102970963536));
#24353=CARTESIAN_POINT('Ctrl Pts',(130.376553582223,-30.9323923001702,29.4087616422947));
#24354=CARTESIAN_POINT('Ctrl Pts',(130.495101758289,-30.9433667460012,29.4029298332344));
#24355=CARTESIAN_POINT('Ctrl Pts',(130.613354428765,-30.9595451065276,29.3970980241742));
#24356=CARTESIAN_POINT('Ctrl Pts',(130.730820038436,-30.9809046949071,29.3912662151139));
#24357=CARTESIAN_POINT('Ctrl Pts',(130.848147694306,-31.0022391981878,29.3854412550389));
#24358=CARTESIAN_POINT('Ctrl Pts',(130.964689730705,-31.0287427564402,29.3796162949639));
#24359=CARTESIAN_POINT('Ctrl Pts',(131.079958684508,-31.0603408472616,29.3737913348889));
#24360=CARTESIAN_POINT('Ctrl Pts',(131.195119236869,-31.0919092225481,29.3679718527336));
#24361=CARTESIAN_POINT('Ctrl Pts',(131.309008697878,-31.1285624933226,29.3621523705783));
#24362=CARTESIAN_POINT('Ctrl Pts',(131.421149399369,-31.1701750190547,29.3563328884229));
#24363=CARTESIAN_POINT('Ctrl Pts',(131.533206474952,-31.2117565133665,29.3505177459897));
#24364=CARTESIAN_POINT('Ctrl Pts',(131.643517006468,-31.2582897605415,29.3447026035565));
#24365=CARTESIAN_POINT('Ctrl Pts',(131.751618760839,-31.3095993826311,29.3388874611232));
#24366=CARTESIAN_POINT('Ctrl Pts',(131.859673816909,-31.3608868397502,29.3330748307424));
#24367=CARTESIAN_POINT('Ctrl Pts',(131.965521627783,-31.4169463914047,29.3272622003616));
#24368=CARTESIAN_POINT('Ctrl Pts',(132.068720680817,-31.477554862775,29.3214495699808));
#24369=CARTESIAN_POINT('Ctrl Pts',(132.171910341834,-31.5381578182435,29.3156374686003));
#24370=CARTESIAN_POINT('Ctrl Pts',(132.272451372145,-31.603308666982,29.3098253672197));
#24371=CARTESIAN_POINT('Ctrl Pts',(132.369927990263,-31.6727389160201,29.3040132658392));
#24372=CARTESIAN_POINT('Ctrl Pts',(132.409519580254,-31.7009390526884,29.3016525937181));
#24373=CARTESIAN_POINT('Ctrl Pts',(132.448605957911,-31.7298446580891,29.2992919215971));
#24374=CARTESIAN_POINT('Ctrl Pts',(132.487160670875,-31.7594357285724,29.296931249476));
#24375=CARTESIAN_POINT('',(128.942095577027,-38.9456385074984,30.));
#24376=CARTESIAN_POINT('Ctrl Pts',(128.942095577027,-38.9456385074984,30.));
#24377=CARTESIAN_POINT('Ctrl Pts',(127.639207105396,-38.596308107828,29.9343068491439));
#24378=CARTESIAN_POINT('Ctrl Pts',(126.178813349621,-37.2185119668352,29.8475123998799));
#24379=CARTESIAN_POINT('Ctrl Pts',(125.916229787505,-35.4379239995562,29.7607179506158));
#24380=CARTESIAN_POINT('Ctrl Pts',(125.919305073524,-35.0038914743736,29.739616652208));
#24381=CARTESIAN_POINT('',(131.058681718482,-38.9454300169882,29.999999873734));
#24382=CARTESIAN_POINT('Origin',(130.,-35.,30.));
#24383=CARTESIAN_POINT('',(125.915000700056,-34.9976084607349,29.6353849714475));
#24384=CARTESIAN_POINT('Ctrl Pts',(131.058681718482,-38.9454300169882,29.999999873734));
#24385=CARTESIAN_POINT('Ctrl Pts',(130.944553579868,-38.9760541500725,29.9942106257328));
#24386=CARTESIAN_POINT('Ctrl Pts',(130.828900823923,-39.0017743570889,29.9884213777316));
#24387=CARTESIAN_POINT('Ctrl Pts',(130.712185167928,-39.0224392209931,29.9826321297304));
#24388=CARTESIAN_POINT('Ctrl Pts',(130.595617050571,-39.0430779627302,29.976850199837));
#24389=CARTESIAN_POINT('Ctrl Pts',(130.477989108527,-39.0586739970541,29.9710682699437));
#24390=CARTESIAN_POINT('Ctrl Pts',(130.359777597801,-39.0691258373416,29.9652863400504));
#24391=CARTESIAN_POINT('Ctrl Pts',(130.241683728729,-39.0795672761734,29.9595101642143));
#24392=CARTESIAN_POINT('Ctrl Pts',(130.123007855757,-39.0848746667639,29.9537339883782));
#24393=CARTESIAN_POINT('Ctrl Pts',(130.004235129155,-39.0849978046115,29.9479578125421));
#24394=CARTESIAN_POINT('Ctrl Pts',(129.88554614853,-39.0851208556354,29.9421857094549));
#24395=CARTESIAN_POINT('Ctrl Pts',(129.766760862474,-39.0800669244702,29.9364136063676));
#24396=CARTESIAN_POINT('Ctrl Pts',(129.648367584554,-39.0698377909209,29.9306415032804));
#24397=CARTESIAN_POINT('Ctrl Pts',(129.530018417893,-39.0596124685672,29.9248715507774));
#24398=CARTESIAN_POINT('Ctrl Pts',(129.412061380663,-39.0442158123201,29.9191015982745));
#24399=CARTESIAN_POINT('Ctrl Pts',(129.294982237339,-39.0237016482752,29.9133316457716));
#24400=CARTESIAN_POINT('Ctrl Pts',(129.177918221597,-39.0031901348279,29.9075624387937));
#24401=CARTESIAN_POINT('Ctrl Pts',(129.061732281649,-38.9775624998559,29.9017932318157));
#24402=CARTESIAN_POINT('Ctrl Pts',(128.946901819112,-38.9469240202227,29.8960240248378));
#24403=CARTESIAN_POINT('Ctrl Pts',(128.832058246409,-38.9162820426015,29.8902541591908));
#24404=CARTESIAN_POINT('Ctrl Pts',(128.718570858412,-38.8806281901078,29.8844842935439));
#24405=CARTESIAN_POINT('Ctrl Pts',(128.606902986808,-38.8401179294176,29.8787144278969));
#24406=CARTESIAN_POINT('Ctrl Pts',(128.495126237423,-38.799568170641,29.872938936548));
#24407=CARTESIAN_POINT('Ctrl Pts',(128.385172937777,-38.7541526867095,29.8671634451991));
#24408=CARTESIAN_POINT('Ctrl Pts',(128.27748764131,-38.7040756166905,29.8613879538502));
#24409=CARTESIAN_POINT('Ctrl Pts',(128.169750388419,-38.65397438529,29.8556096759195));
#24410=CARTESIAN_POINT('Ctrl Pts',(128.064283685775,-38.5992072781454,29.8498313979889));
#24411=CARTESIAN_POINT('Ctrl Pts',(127.961507016297,-38.5400242026565,29.8440531200582));
#24412=CARTESIAN_POINT('Ctrl Pts',(127.85856581443,-38.480746382583,29.8382655918388));
#24413=CARTESIAN_POINT('Ctrl Pts',(127.758323599919,-38.4170386909014,29.8324780636193));
#24414=CARTESIAN_POINT('Ctrl Pts',(127.661170868142,-38.3491944243311,29.8266905353998));
#24415=CARTESIAN_POINT('Ctrl Pts',(127.568698601784,-38.2846186478772,29.8211818292494));
#24416=CARTESIAN_POINT('Ctrl Pts',(127.479025300208,-38.2162957863241,29.8156731230991));
#24417=CARTESIAN_POINT('Ctrl Pts',(127.392457740908,-38.1445108311233,29.8101644169487));
#24418=CARTESIAN_POINT('Ctrl Pts',(127.302025730489,-38.0695213331038,29.8044097973659));
#24419=CARTESIAN_POINT('Ctrl Pts',(127.21467127379,-37.990494710053,29.7986551777831));
#24420=CARTESIAN_POINT('Ctrl Pts',(127.130781940669,-37.9077160672954,29.7929005582002));
#24421=CARTESIAN_POINT('Ctrl Pts',(127.046997022695,-37.8250404572341,29.7871531012616));
#24422=CARTESIAN_POINT('Ctrl Pts',(126.966668949469,-37.7386224034269,29.7814056443231));
#24423=CARTESIAN_POINT('Ctrl Pts',(126.890153059589,-37.6487878373355,29.7756581873845));
#24424=CARTESIAN_POINT('Ctrl Pts',(126.812342342182,-37.5574330606155,29.7698134700538));
#24425=CARTESIAN_POINT('Ctrl Pts',(126.738474361781,-37.4625453450967,29.7639687527231));
#24426=CARTESIAN_POINT('Ctrl Pts',(126.668884865751,-37.3645077632303,29.7581240353924));
#24427=CARTESIAN_POINT('Ctrl Pts',(126.600566624001,-37.2682611225644,29.7523860888007));
#24428=CARTESIAN_POINT('Ctrl Pts',(126.536372134257,-37.1689790755732,29.7466481422091));
#24429=CARTESIAN_POINT('Ctrl Pts',(126.47657871807,-37.0670576842563,29.7409101956174));
#24430=CARTESIAN_POINT('Ctrl Pts',(126.416805277182,-36.9651703420097,29.7351741659124));
#24431=CARTESIAN_POINT('Ctrl Pts',(126.361430199031,-36.8606457691834,29.7294381362073));
#24432=CARTESIAN_POINT('Ctrl Pts',(126.310686761419,-36.7539078731891,29.7237021065022));
#24433=CARTESIAN_POINT('Ctrl Pts',(126.259947595204,-36.6471789619982,29.7179665596351));
#24434=CARTESIAN_POINT('Ctrl Pts',(126.213839473349,-36.5382374769035,29.7122310127679));
#24435=CARTESIAN_POINT('Ctrl Pts',(126.172548747324,-36.4275300026224,29.7064954659007));
#24436=CARTESIAN_POINT('Ctrl Pts',(126.129887835005,-36.3131488253476,29.7005695913629));
#24437=CARTESIAN_POINT('Ctrl Pts',(126.092369787723,-36.1968828533769,29.6946437168251));
#24438=CARTESIAN_POINT('Ctrl Pts',(126.060144891387,-36.0792435884163,29.6887178422874));
#24439=CARTESIAN_POINT('Ctrl Pts',(126.028921932286,-35.9652619662481,29.6829762151801));
#24440=CARTESIAN_POINT('Ctrl Pts',(126.002667897363,-35.8499916120652,29.6772345880728));
#24441=CARTESIAN_POINT('Ctrl Pts',(125.981467567398,-35.7339087737072,29.6714929609655));
#24442=CARTESIAN_POINT('Ctrl Pts',(125.959246767212,-35.6122383298786,29.6654749627125));
#24443=CARTESIAN_POINT('Ctrl Pts',(125.942578393723,-35.4896757557052,29.6594569644595));
#24444=CARTESIAN_POINT('Ctrl Pts',(125.931498881111,-35.3667746523376,29.6534389662065));
#24445=CARTESIAN_POINT('Ctrl Pts',(125.920419368499,-35.2438735489701,29.6474209679535));
#24446=CARTESIAN_POINT('Ctrl Pts',(125.914928675205,-35.1206344422539,29.6414029697005));
#24447=CARTESIAN_POINT('Ctrl Pts',(125.915000700056,-34.9976084607349,29.6353849714475));
#24448=CARTESIAN_POINT('Ctrl Pts',(125.915000700057,-34.9976084598567,29.6353849714045));
#24449=CARTESIAN_POINT('Ctrl Pts',(125.915089664039,-34.845648725259,29.6279516357298));
#24450=CARTESIAN_POINT('Ctrl Pts',(125.923657510955,-34.693945020907,29.6205183000551));
#24451=CARTESIAN_POINT('Ctrl Pts',(125.940621229176,-34.543196984482,29.6130849643803));
#24452=CARTESIAN_POINT('Ctrl Pts',(125.953900069263,-34.4251946077035,29.6072663063214));
#24453=CARTESIAN_POINT('Ctrl Pts',(125.972350285853,-34.307578263497,29.6014476482625));
#24454=CARTESIAN_POINT('Ctrl Pts',(125.995942018589,-34.1908370488571,29.5956289902035));
#24455=CARTESIAN_POINT('Ctrl Pts',(126.019503712228,-34.0742444795399,29.5898177409788));
#24456=CARTESIAN_POINT('Ctrl Pts',(126.048193821194,-33.9585252210092,29.5840064917541));
#24457=CARTESIAN_POINT('Ctrl Pts',(126.081930718129,-33.8441634620494,29.5781952425294));
#24458=CARTESIAN_POINT('Ctrl Pts',(126.115633495392,-33.7299173623876,29.5723898704878));
#24459=CARTESIAN_POINT('Ctrl Pts',(126.154372792127,-33.6170264213218,29.5665844984463));
#24460=CARTESIAN_POINT('Ctrl Pts',(126.198016026887,-33.5059642346352,29.5607791264047));
#24461=CARTESIAN_POINT('Ctrl Pts',(126.24336474875,-33.390561968021,29.5547468924634));
#24462=CARTESIAN_POINT('Ctrl Pts',(126.29400840197,-33.2771347374572,29.548714658522));
#24463=CARTESIAN_POINT('Ctrl Pts',(126.349741154889,-33.1661964762586,29.5426824245806));
#24464=CARTESIAN_POINT('Ctrl Pts',(126.4033164962,-33.0595526286651,29.5368836980625));
#24465=CARTESIAN_POINT('Ctrl Pts',(126.461594070909,-32.9552090404644,29.5310849715443));
#24466=CARTESIAN_POINT('Ctrl Pts',(126.524342428739,-32.8536008182687,29.5252862450261));
#24467=CARTESIAN_POINT('Ctrl Pts',(126.587081183805,-32.7520081457994,29.5194884059225));
#24468=CARTESIAN_POINT('Ctrl Pts',(126.654289146494,-32.6531503549122,29.5136905668188));
#24469=CARTESIAN_POINT('Ctrl Pts',(126.725690118207,-32.5574358149699,29.5078927277152));
#24470=CARTESIAN_POINT('Ctrl Pts',(126.797097096589,-32.4617132229587,29.5020944008633));
#24471=CARTESIAN_POINT('Ctrl Pts',(126.872697540618,-32.3691347355745,29.4962960740114));
#24472=CARTESIAN_POINT('Ctrl Pts',(126.952173738435,-32.2800771923975,29.4904977471595));
#24473=CARTESIAN_POINT('Ctrl Pts',(127.03167547094,-32.1909910361686,29.4846975573792));
#24474=CARTESIAN_POINT('Ctrl Pts',(127.115055161299,-32.105428378916,29.4788973675989));
#24475=CARTESIAN_POINT('Ctrl Pts',(127.20195734371,-32.0237301376421,29.4730971778186));
#24476=CARTESIAN_POINT('Ctrl Pts',(127.288955816632,-31.9419413719968,29.4672905612349));
#24477=CARTESIAN_POINT('Ctrl Pts',(127.379484274045,-31.8640258497032,29.4614839446512));
#24478=CARTESIAN_POINT('Ctrl Pts',(127.473153080475,-31.790285114642,29.4556773280675));
#24479=CARTESIAN_POINT('Ctrl Pts',(127.566883344002,-31.7164959975027,29.4498669017011));
#24480=CARTESIAN_POINT('Ctrl Pts',(127.663757728217,-31.6468873605511,29.4440564753347));
#24481=CARTESIAN_POINT('Ctrl Pts',(127.763357846448,-31.5817172619934,29.4382460489683));
#24482=CARTESIAN_POINT('Ctrl Pts',(127.863101256293,-31.5164534052278,29.4324272633209));
#24483=CARTESIAN_POINT('Ctrl Pts',(127.965577876409,-31.4556410400234,29.4266084776736));
#24484=CARTESIAN_POINT('Ctrl Pts',(128.070344885655,-31.3994922386303,29.4207896920263));
#24485=CARTESIAN_POINT('Ctrl Pts',(128.099057878545,-31.3841038053175,29.4191949652881));
#24486=CARTESIAN_POINT('Ctrl Pts',(128.127942793974,-31.3690653801131,29.41760023855));
#24487=CARTESIAN_POINT('Ctrl Pts',(128.156990278416,-31.3543806882578,29.4160055118119));
#24488=CARTESIAN_POINT('Ctrl Pts',(128.263076116259,-31.3007499567556,29.4101813268474));
#24489=CARTESIAN_POINT('Ctrl Pts',(128.371675762737,-31.2516672333729,29.4043571418829));
#24490=CARTESIAN_POINT('Ctrl Pts',(128.482362616791,-31.2073753450827,29.3985329569184));
#24491=CARTESIAN_POINT('Ctrl Pts',(128.592909797229,-31.163139347876,29.3927161213811));
#24492=CARTESIAN_POINT('Ctrl Pts',(128.705538570954,-31.1236823117551,29.3868992858438));
#24493=CARTESIAN_POINT('Ctrl Pts',(128.819798154847,-31.0892010273222,29.3810824503064));
#24494=CARTESIAN_POINT('Ctrl Pts',(128.933943320326,-31.0547542721054,29.3752714396905));
#24495=CARTESIAN_POINT('Ctrl Pts',(129.049715658567,-31.025273473399,29.3694604290746));
#24496=CARTESIAN_POINT('Ctrl Pts',(129.166645398469,-31.0009069643096,29.3636494184587));
#24497=CARTESIAN_POINT('Ctrl Pts',(129.287984481213,-30.9756216103437,29.3576192784914));
#24498=CARTESIAN_POINT('Ctrl Pts',(129.410569557824,-30.9558440186323,29.3515891385241));
#24499=CARTESIAN_POINT('Ctrl Pts',(129.533859097536,-30.9416829030927,29.3455589985568));
#24500=CARTESIAN_POINT('Ctrl Pts',(129.652534477305,-30.9280517729211,29.3397545389704));
#24501=CARTESIAN_POINT('Ctrl Pts',(129.771862096122,-30.9196243260056,29.3339500793841));
#24502=CARTESIAN_POINT('Ctrl Pts',(129.891350325346,-30.9164451456852,29.3281456197977));
#24503=CARTESIAN_POINT('Ctrl Pts',(130.010820801379,-30.9132664377176,29.3223420226199));
#24504=CARTESIAN_POINT('Ctrl Pts',(130.130451432377,-30.9153344564683,29.3165384254422));
#24505=CARTESIAN_POINT('Ctrl Pts',(130.249748468838,-30.9226417005231,29.3107348282645));
#24506=CARTESIAN_POINT('Ctrl Pts',(130.369055918311,-30.9299495824011,29.3049307245115));
#24507=CARTESIAN_POINT('Ctrl Pts',(130.488029307856,-30.9424975738677,29.2991266207586));
#24508=CARTESIAN_POINT('Ctrl Pts',(130.606178536407,-30.960226171925,29.2933225170056));
#24509=CARTESIAN_POINT('Ctrl Pts',(130.724365944667,-30.9779604989467,29.287516537667));
#24510=CARTESIAN_POINT('Ctrl Pts',(130.841728258753,-31.0008787014336,29.2817105583284));
#24511=CARTESIAN_POINT('Ctrl Pts',(130.957784748129,-31.0288700126725,29.2759045789898));
#24512=CARTESIAN_POINT('Ctrl Pts',(131.073969498395,-31.0568922587649,29.2700921831201));
#24513=CARTESIAN_POINT('Ctrl Pts',(131.188845146208,-31.0899987090927,29.2642797872503));
#24514=CARTESIAN_POINT('Ctrl Pts',(131.301945173453,-31.1280284394999,29.2584673913806));
#24515=CARTESIAN_POINT('Ctrl Pts',(131.415119349703,-31.166083102409,29.2526511848719));
#24516=CARTESIAN_POINT('Ctrl Pts',(131.526515207018,-31.2090673269266,29.2468349783632));
#24517=CARTESIAN_POINT('Ctrl Pts',(131.635686834075,-31.2567723044366,29.2410187718545));
#24518=CARTESIAN_POINT('Ctrl Pts',(131.745014562896,-31.3045454940943,29.2351942488984));
#24519=CARTESIAN_POINT('Ctrl Pts',(131.852111348333,-31.3570527305047,29.2293697259423));
#24520=CARTESIAN_POINT('Ctrl Pts',(131.956556340386,-31.4140395586544,29.2235452029863));
#24521=CARTESIAN_POINT('Ctrl Pts',(131.984166408778,-31.4291040456322,29.2220054884053));
#24522=CARTESIAN_POINT('Ctrl Pts',(132.011591328512,-31.4444813395595,29.2204657738244));
#24523=CARTESIAN_POINT('Ctrl Pts',(132.038823685636,-31.4601662498232,29.2189260592434));
#24524=CARTESIAN_POINT('Ctrl Pts',(132.141833733249,-31.5194965290832,29.2131018820864));
#24525=CARTESIAN_POINT('Ctrl Pts',(132.242417377746,-31.5834223086336,29.2072777049293));
#24526=CARTESIAN_POINT('Ctrl Pts',(132.340137746395,-31.6517197954921,29.2014535277723));
#24527=CARTESIAN_POINT('Ctrl Pts',(132.389906219477,-31.6865033486382,29.1984873047823));
#24528=CARTESIAN_POINT('Ctrl Pts',(132.438932337297,-31.7224200719,29.1955210817924));
#24529=CARTESIAN_POINT('Ctrl Pts',(132.487160670875,-31.7594357285724,29.1925548588025));
#24530=CARTESIAN_POINT('Origin',(130.,-35.,23.));
#24531=CARTESIAN_POINT('',(126.821241975899,-33.8227564029848,17.9148966234937));
#24532=CARTESIAN_POINT('',(126.821241915871,-33.8227565650715,17.5703600952825));
#24533=CARTESIAN_POINT('',(126.821241915871,-33.8227565650715,23.));
#24534=CARTESIAN_POINT('',(133.378768828602,-35.2726284383002,17.));
#24535=CARTESIAN_POINT('Ctrl Pts',(126.821241915871,-33.8227565650715,17.5703600952825));
#24536=CARTESIAN_POINT('Ctrl Pts',(126.857212086853,-33.7256309677594,17.5642667500865));
#24537=CARTESIAN_POINT('Ctrl Pts',(126.897684653908,-33.6300288363987,17.5581734048904));
#24538=CARTESIAN_POINT('Ctrl Pts',(126.942506928975,-33.536394457808,17.5520800596944));
#24539=CARTESIAN_POINT('Ctrl Pts',(126.987285654953,-33.4428510538928,17.5459926347609));
#24540=CARTESIAN_POINT('Ctrl Pts',(127.036405501013,-33.3512719845787,17.5399052098273));
#24541=CARTESIAN_POINT('Ctrl Pts',(127.089665306779,-33.2620825577905,17.5338177848938));
#24542=CARTESIAN_POINT('Ctrl Pts',(127.142891448156,-33.1729495057405,17.527734207692));
#24543=CARTESIAN_POINT('Ctrl Pts',(127.200252127707,-33.086203459193,17.5216506304902));
#24544=CARTESIAN_POINT('Ctrl Pts',(127.261500154244,-33.0022453460714,17.5155670532884));
#24545=CARTESIAN_POINT('Ctrl Pts',(127.322728683129,-32.9183139601134,17.5094854127281));
#24546=CARTESIAN_POINT('Ctrl Pts',(127.387841847681,-32.8371690887653,17.5034037721677));
#24547=CARTESIAN_POINT('Ctrl Pts',(127.456549491797,-32.7591821638473,17.4973221316074));
#24548=CARTESIAN_POINT('Ctrl Pts',(127.525253041812,-32.6811998859558,17.4912408534353));
#24549=CARTESIAN_POINT('Ctrl Pts',(127.59755036266,-32.6063755009931,17.4851595752632));
#24550=CARTESIAN_POINT('Ctrl Pts',(127.673112026926,-32.5350461620416,17.4790782970911));
#24551=CARTESIAN_POINT('Ctrl Pts',(127.74868874015,-32.4637026170487,17.472995807764));
#24552=CARTESIAN_POINT('Ctrl Pts',(127.827530777778,-32.3958557947502,17.4669133184368));
#24553=CARTESIAN_POINT('Ctrl Pts',(127.909273677431,-32.3318042600632,17.4608308291097));
#24554=CARTESIAN_POINT('Ctrl Pts',(127.991104779775,-32.2676836121229,17.4547417766201));
#24555=CARTESIAN_POINT('Ctrl Pts',(128.075842656886,-32.2073666928101,17.4486527241306));
#24556=CARTESIAN_POINT('Ctrl Pts',(128.163091785404,-32.1511101682148,17.442563671641));
#24557=CARTESIAN_POINT('Ctrl Pts',(128.250391702938,-32.0948208958592,17.4364710746234));
#24558=CARTESIAN_POINT('Ctrl Pts',(128.34020541377,-32.0425969403403,17.4303784776057));
#24559=CARTESIAN_POINT('Ctrl Pts',(128.432112321585,-31.9946492234062,17.4242858805881));
#24560=CARTESIAN_POINT('Ctrl Pts',(128.524167018222,-31.946624405231,17.4181834865077));
#24561=CARTESIAN_POINT('Ctrl Pts',(128.618321246487,-31.9028897387552,17.4120810924273));
#24562=CARTESIAN_POINT('Ctrl Pts',(128.714133823855,-31.8636082452048,17.4059786983469));
#24563=CARTESIAN_POINT('Ctrl Pts',(128.775993963582,-31.8382466617216,17.4020387672769));
#24564=CARTESIAN_POINT('Ctrl Pts',(128.838545020091,-31.8147403681239,17.3980988362069));
#24565=CARTESIAN_POINT('Ctrl Pts',(128.901665374432,-31.7931220614469,17.3941589051368));
#24566=CARTESIAN_POINT('Ctrl Pts',(128.998656182998,-31.7599033467185,17.3881048025551));
#24567=CARTESIAN_POINT('Ctrl Pts',(129.097333999467,-31.7310277136576,17.3820506999734));
#24568=CARTESIAN_POINT('Ctrl Pts',(129.19727047136,-31.70666880403,17.3759965973917));
#24569=CARTESIAN_POINT('Ctrl Pts',(129.297074246778,-31.6823422383642,17.3699505334975));
#24570=CARTESIAN_POINT('Ctrl Pts',(129.398132937558,-31.6625205801586,17.3639044696033));
#24571=CARTESIAN_POINT('Ctrl Pts',(129.500000401422,-31.6473286078231,17.3578584057091));
#24572=CARTESIAN_POINT('Ctrl Pts',(129.601762953542,-31.6321522814676,17.3518185685636));
#24573=CARTESIAN_POINT('Ctrl Pts',(129.704332195085,-31.621596227296,17.3457787314182));
#24574=CARTESIAN_POINT('Ctrl Pts',(129.807250029976,-31.6157345683951,17.3397388942727));
#24575=CARTESIAN_POINT('Ctrl Pts',(129.910098444688,-31.6098768633027,17.3337031311206));
#24576=CARTESIAN_POINT('Ctrl Pts',(130.013294552223,-31.6087072854238,17.3276673679685));
#24577=CARTESIAN_POINT('Ctrl Pts',(130.116374231673,-31.6122482232751,17.3216316048163));
#24578=CARTESIAN_POINT('Ctrl Pts',(130.219418282801,-31.6157879372414,17.3155979278573));
#24579=CARTESIAN_POINT('Ctrl Pts',(130.322345551185,-31.624034917913,17.3095642508982));
#24580=CARTESIAN_POINT('Ctrl Pts',(130.424691943871,-31.6369594389435,17.3035305739392));
#24581=CARTESIAN_POINT('Ctrl Pts',(130.52703055245,-31.6498829769805,17.2974973558804));
#24582=CARTESIAN_POINT('Ctrl Pts',(130.628787941222,-31.6674832938503,17.2914641378216));
#24583=CARTESIAN_POINT('Ctrl Pts',(130.729506183834,-31.6896788992232,17.2854309197627));
#24584=CARTESIAN_POINT('Ctrl Pts',(130.830243919015,-31.7118788002366,17.2793965340612));
#24585=CARTESIAN_POINT('Ctrl Pts',(130.929941683416,-31.7386756626943,17.2733621483597));
#24586=CARTESIAN_POINT('Ctrl Pts',(131.028153768648,-31.7699373240577,17.2673277626582));
#24587=CARTESIAN_POINT('Ctrl Pts',(131.126480044199,-31.8012353330771,17.26128636083));
#24588=CARTESIAN_POINT('Ctrl Pts',(131.223316775647,-31.8370083746529,17.2552449590019));
#24589=CARTESIAN_POINT('Ctrl Pts',(131.318235456208,-31.8770750338031,17.2492035571737));
#24590=CARTESIAN_POINT('Ctrl Pts',(131.41321041572,-31.9171654491783,17.2431585732924));
#24591=CARTESIAN_POINT('Ctrl Pts',(131.506264667989,-31.9615543620595,17.2371135894111));
#24592=CARTESIAN_POINT('Ctrl Pts',(131.596993644016,-32.010013986074,17.2310686055298));
#24593=CARTESIAN_POINT('Ctrl Pts',(131.687886896195,-32.0585613522949,17.2250126764496));
#24594=CARTESIAN_POINT('Ctrl Pts',(131.776446088358,-32.1111939292309,17.2189567473694));
#24595=CARTESIAN_POINT('Ctrl Pts',(131.862294784052,-32.16763999467,17.2129008182892));
#24596=CARTESIAN_POINT('Ctrl Pts',(131.937055875936,-32.2167958898257,17.2076270297157));
#24597=CARTESIAN_POINT('Ctrl Pts',(132.009761740428,-32.2688430573262,17.2023532411421));
#24598=CARTESIAN_POINT('Ctrl Pts',(132.0801854484,-32.3235782165803,17.1970794525685));
#24599=CARTESIAN_POINT('Ctrl Pts',(132.163725198345,-32.3885075088443,17.1908234488535));
#24600=CARTESIAN_POINT('Ctrl Pts',(132.244340954018,-32.4574437278421,17.1845674451385));
#24601=CARTESIAN_POINT('Ctrl Pts',(132.321637206882,-32.5301000542288,17.1783114414236));
#24602=CARTESIAN_POINT('Ctrl Pts',(132.398820375414,-32.60265008449,17.1720645902352));
#24603=CARTESIAN_POINT('Ctrl Pts',(132.472693415881,-32.6789091177425,17.1658177390467));
#24604=CARTESIAN_POINT('Ctrl Pts',(132.542892921555,-32.7585494312818,17.1595708878583));
#24605=CARTESIAN_POINT('Ctrl Pts',(132.613005970988,-32.8380916614787,17.153331730161));
#24606=CARTESIAN_POINT('Ctrl Pts',(132.679454227142,-32.9210065833029,17.1470925724636));
#24607=CARTESIAN_POINT('Ctrl Pts',(132.741910682205,-33.0069292854214,17.1408534147663));
#24608=CARTESIAN_POINT('Ctrl Pts',(132.804294288443,-33.0927517678289,17.1346215343841));
#24609=CARTESIAN_POINT('Ctrl Pts',(132.862695133877,-33.1815747181818,17.1283896540019));
#24610=CARTESIAN_POINT('Ctrl Pts',(132.916826607734,-33.273000404484,17.1221577736197));
#24611=CARTESIAN_POINT('Ctrl Pts',(132.970921300909,-33.3643639698258,17.1159301276099));
#24612=CARTESIAN_POINT('Ctrl Pts',(133.020752191913,-33.4583264071137,17.1097024816));
#24613=CARTESIAN_POINT('Ctrl Pts',(133.066076207699,-33.5544614321713,17.1034748355901));
#24614=CARTESIAN_POINT('Ctrl Pts',(133.111378919699,-33.6505512705878,17.0972501167798));
#24615=CARTESIAN_POINT('Ctrl Pts',(133.15217880271,-33.7488113013554,17.0910253979695));
#24616=CARTESIAN_POINT('Ctrl Pts',(133.18827920759,-33.8487916101105,17.0848006791592));
#24617=CARTESIAN_POINT('Ctrl Pts',(133.224370200206,-33.9487458515422,17.078577583286));
#24618=CARTESIAN_POINT('Ctrl Pts',(133.255764019014,-34.050419100345,17.0723544874129));
#24619=CARTESIAN_POINT('Ctrl Pts',(133.282312756489,-34.1533430263166,17.0661313915397));
#24620=CARTESIAN_POINT('Ctrl Pts',(133.308867658179,-34.2562908496664,17.0599068507579));
#24621=CARTESIAN_POINT('Ctrl Pts',(133.330575125734,-34.3604895427839,17.0536823099761));
#24622=CARTESIAN_POINT('Ctrl Pts',(133.34733763752,-34.4654573890282,17.0474577691943));
#24623=CARTESIAN_POINT('Ctrl Pts',(133.364101852332,-34.5704358997268,17.0412325960156));
#24624=CARTESIAN_POINT('Ctrl Pts',(133.375920054006,-34.6761833216448,17.035007422837));
#24625=CARTESIAN_POINT('Ctrl Pts',(133.382746348089,-34.7822106361798,17.0287822496584));
#24626=CARTESIAN_POINT('Ctrl Pts',(133.38957746019,-34.8883127850986,17.0225526827346));
#24627=CARTESIAN_POINT('Ctrl Pts',(133.391409607669,-34.994694819922,17.0163231158108));
#24628=CARTESIAN_POINT('Ctrl Pts',(133.388248988362,-35.1008655311097,17.010093548887));
#24629=CARTESIAN_POINT('Ctrl Pts',(133.386541974809,-35.1582070914918,17.0067290325913));
#24630=CARTESIAN_POINT('Ctrl Pts',(133.383379494437,-35.2154870259768,17.0033645162957));
#24631=CARTESIAN_POINT('Ctrl Pts',(133.378768828602,-35.2726284383002,17.));
#24632=CARTESIAN_POINT('',(126.821241915871,-33.8227565650715,17.));
#24633=CARTESIAN_POINT('Origin',(130.,-35.,17.));
#24634=CARTESIAN_POINT('',(126.821241915871,-33.8227565650715,16.));
#24635=CARTESIAN_POINT('',(126.821241915871,-33.8227565650715,23.));
#24636=CARTESIAN_POINT('Origin',(130.,-35.,16.));
#24637=CARTESIAN_POINT('',(129.213983878817,-38.3003700508738,16.998298898493));
#24638=CARTESIAN_POINT('Origin',(130.,-35.,17.));
#24639=CARTESIAN_POINT('Ctrl Pts',(129.214786760262,-38.2975513992415,16.9966191224731));
#24640=CARTESIAN_POINT('Ctrl Pts',(129.246653588405,-38.3051395312634,16.9986057882608));
#24641=CARTESIAN_POINT('Ctrl Pts',(129.278627725152,-38.3122650918281,17.0006144214925));
#24642=CARTESIAN_POINT('Ctrl Pts',(129.562948150419,-38.371315022687,17.0185812798767));
#24643=CARTESIAN_POINT('Ctrl Pts',(129.820339259371,-38.3947753103289,17.0355059067697));
#24644=CARTESIAN_POINT('Ctrl Pts',(130.186419839379,-38.3863602280712,17.0588775137659));
#24645=CARTESIAN_POINT('Ctrl Pts',(130.294764342428,-38.3786543348929,17.0657189329248));
#24646=CARTESIAN_POINT('Ctrl Pts',(130.47777413777,-38.356765566798,17.077099281972));
#24647=CARTESIAN_POINT('Ctrl Pts',(130.552669845413,-38.3452504522162,17.0817067208494));
#24648=CARTESIAN_POINT('Ctrl Pts',(130.661059909158,-38.324845485086,17.0883038359326));
#24649=CARTESIAN_POINT('Ctrl Pts',(130.694899655733,-38.3179379594991,17.0903534317222));
#24650=CARTESIAN_POINT('Ctrl Pts',(130.754814885438,-38.3047508944395,17.0939658163127));
#24651=CARTESIAN_POINT('Ctrl Pts',(130.780932103144,-38.2986768705901,17.0955348410941));
#24652=CARTESIAN_POINT('Ctrl Pts',(130.83611855973,-38.285150101204,17.0988393862245));
#24653=CARTESIAN_POINT('Ctrl Pts',(130.86516655488,-38.2776199212549,17.1005723354365));
#24654=CARTESIAN_POINT('Ctrl Pts',(130.943853737324,-38.2561026555034,17.1052516552153));
#24655=CARTESIAN_POINT('Ctrl Pts',(130.993280849296,-38.2413666750523,17.10817448793));
#24656=CARTESIAN_POINT('Ctrl Pts',(131.268952899463,-38.15228056572,17.1244180377395));
#24657=CARTESIAN_POINT('Ctrl Pts',(131.487204870787,-38.0553798822507,17.136996498997));
#24658=CARTESIAN_POINT('Ctrl Pts',(131.842051924174,-37.8507285068452,17.1588181106744));
#24659=CARTESIAN_POINT('Ctrl Pts',(131.983862781221,-37.753921631808,17.1679974824299));
#24660=CARTESIAN_POINT('Ctrl Pts',(132.141492708805,-37.6278014531061,17.179470787434));
#24661=CARTESIAN_POINT('Ctrl Pts',(132.165001097274,-37.6084672921821,17.1812181425926));
#24662=CARTESIAN_POINT('Ctrl Pts',(132.201356071569,-37.5777376172861,17.1839833503402));
#24663=CARTESIAN_POINT('Ctrl Pts',(132.214382372257,-37.5665561477482,17.1849871056437));
#24664=CARTESIAN_POINT('Ctrl Pts',(132.23893598053,-37.5451538400591,17.1869050866599));
#24665=CARTESIAN_POINT('Ctrl Pts',(132.25047933074,-37.5349526902266,17.1878180019822));
#24666=CARTESIAN_POINT('Ctrl Pts',(132.275884266371,-37.5121914263325,17.1898516986653));
#24667=CARTESIAN_POINT('Ctrl Pts',(132.28971212245,-37.499594630796,17.1909750023959));
#24668=CARTESIAN_POINT('Ctrl Pts',(132.33741636256,-37.4554093833093,17.1949053798742));
#24669=CARTESIAN_POINT('Ctrl Pts',(132.370747660348,-37.4232427825009,17.19774951986));
#24670=CARTESIAN_POINT('Ctrl Pts',(132.550534164409,-37.2424783328038,17.2135896489576));
#24671=CARTESIAN_POINT('Ctrl Pts',(132.683682891899,-37.0812912981307,17.2271676473973));
#24672=CARTESIAN_POINT('Ctrl Pts',(132.892770772903,-36.7744701147091,17.2509959832686));
#24673=CARTESIAN_POINT('Ctrl Pts',(132.974590106743,-36.6336128830552,17.2612963397486));
#24674=CARTESIAN_POINT('Ctrl Pts',(133.073909781551,-36.4302216959482,17.2751714707825));
#24675=CARTESIAN_POINT('Ctrl Pts',(133.100221104257,-36.3722555726456,17.2790221057876));
#24676=CARTESIAN_POINT('Ctrl Pts',(133.137407413537,-36.283792757709,17.2847463889883));
#24677=CARTESIAN_POINT('Ctrl Pts',(133.149502540497,-36.2538273319791,17.2866597683682));
#24678=CARTESIAN_POINT('Ctrl Pts',(133.169818863107,-36.2013441392698,17.28996767964));
#24679=CARTESIAN_POINT('Ctrl Pts',(133.178232960908,-36.1789040060696,17.2913684474965));
#24680=CARTESIAN_POINT('Ctrl Pts',(133.196759108508,-36.1278549787408,17.2945251990383));
#24681=CARTESIAN_POINT('Ctrl Pts',(133.206726507739,-36.0991955427724,17.2962763900253));
#24682=CARTESIAN_POINT('Ctrl Pts',(133.232770263813,-36.0209403912586,17.301003672655));
#24683=CARTESIAN_POINT('Ctrl Pts',(133.248089773987,-35.9711004502343,17.3039555377369));
#24684=CARTESIAN_POINT('Ctrl Pts',(133.339695926222,-35.6465978698149,17.3228374367854));
#24685=CARTESIAN_POINT('Ctrl Pts',(133.382225693376,-35.3636102281896,17.3376348850357));
#24686=CARTESIAN_POINT('Ctrl Pts',(133.39203495278,-34.9408405567215,17.3602397627774));
#24687=CARTESIAN_POINT('Ctrl Pts',(133.386825023489,-34.8029984839704,17.367711907507));
#24688=CARTESIAN_POINT('Ctrl Pts',(133.370491590856,-34.6381019210267,17.3771552266791));
#24689=CARTESIAN_POINT('Ctrl Pts',(133.367398216467,-34.6103682135816,17.3787608947107));
#24690=CARTESIAN_POINT('Ctrl Pts',(133.36193445253,-34.5663258502553,17.3813428951952));
#24691=CARTESIAN_POINT('Ctrl Pts',(133.359786859501,-34.5499902608899,17.3823076295064));
#24692=CARTESIAN_POINT('Ctrl Pts',(133.355428641472,-34.5186115206496,17.3841754447154));
#24693=CARTESIAN_POINT('Ctrl Pts',(133.35323576391,-34.5035666072459,17.3850775920919));
#24694=CARTESIAN_POINT('Ctrl Pts',(133.34749503266,-34.4659551448432,17.3873487369644));
#24695=CARTESIAN_POINT('Ctrl Pts',(133.34382016177,-34.443408979409,17.388724418097));
#24696=CARTESIAN_POINT('Ctrl Pts',(133.329315865579,-34.3597561471504,17.3938773108535));
#24697=CARTESIAN_POINT('Ctrl Pts',(133.317037395229,-34.2989163673974,17.3977217156788));
#24698=CARTESIAN_POINT('Ctrl Pts',(133.259119330531,-34.0477057062228,17.4139080375364));
#24699=CARTESIAN_POINT('Ctrl Pts',(133.198703243129,-33.8611331160025,17.4266587307535));
#24700=CARTESIAN_POINT('Ctrl Pts',(133.061601489316,-33.5366100299174,17.4492664527907));
#24701=CARTESIAN_POINT('Ctrl Pts',(132.990753741091,-33.3967796417927,17.4591699197234));
#24702=CARTESIAN_POINT('Ctrl Pts',(132.878227077439,-33.2083041914475,17.472623776482));
#24703=CARTESIAN_POINT('Ctrl Pts',(132.844469017732,-33.1551797439451,17.4764303505179));
#24704=CARTESIAN_POINT('Ctrl Pts',(132.791354519797,-33.07652201559,17.4820907619841));
#24705=CARTESIAN_POINT('Ctrl Pts',(132.773084780329,-33.0502747582276,17.483983884035));
#24706=CARTESIAN_POINT('Ctrl Pts',(132.74062458761,-33.0050202367912,17.4872565678502));
#24707=CARTESIAN_POINT('Ctrl Pts',(132.726601223124,-32.9858964280754,17.4886423094046));
#24708=CARTESIAN_POINT('Ctrl Pts',(132.694380940432,-32.9429105986351,17.4917642271968));
#24709=CARTESIAN_POINT('Ctrl Pts',(132.676065395201,-32.9191397111135,17.4934956756242));
#24710=CARTESIAN_POINT('Ctrl Pts',(132.625480575953,-32.8552607617076,17.4981648705749));
#24711=CARTESIAN_POINT('Ctrl Pts',(132.59260884792,-32.8156386724102,17.5010787857782));
#24712=CARTESIAN_POINT('Ctrl Pts',(132.399350179993,-32.5932049948419,17.5175754641937));
#24713=CARTESIAN_POINT('Ctrl Pts',(132.220563895338,-32.4273261407114,17.5303624326294));
#24714=CARTESIAN_POINT('Ctrl Pts',(131.882756521121,-32.1755799866038,17.5527002228185));
#24715=CARTESIAN_POINT('Ctrl Pts',(131.731811098369,-32.0805931202618,17.5621884574029));
#24716=CARTESIAN_POINT('Ctrl Pts',(131.547882638817,-31.9841514626025,17.5739916659524));
#24717=CARTESIAN_POINT('Ctrl Pts',(131.521461893255,-31.9707366168401,17.5756929030975));
#24718=CARTESIAN_POINT('Ctrl Pts',(131.479840105132,-31.9502854642561,17.5783870928013));
#24719=CARTESIAN_POINT('Ctrl Pts',(131.46475638466,-31.9430122352426,17.5793663367062));
#24720=CARTESIAN_POINT('Ctrl Pts',(131.435881510991,-31.9293518061251,17.5812475193309));
#24721=CARTESIAN_POINT('Ctrl Pts',(131.422100313304,-31.9229451241244,17.582148290383));
#24722=CARTESIAN_POINT('Ctrl Pts',(131.391501006749,-31.9089694032447,17.5841541577313));
#24723=CARTESIAN_POINT('Ctrl Pts',(131.374663247239,-31.9014445099043,17.5852617574366));
#24724=CARTESIAN_POINT('Ctrl Pts',(131.324175077923,-31.8793735642484,17.5885925128912));
#24725=CARTESIAN_POINT('Ctrl Pts',(131.290350204207,-31.8652360356505,17.5908366212593));
#24726=CARTESIAN_POINT('Ctrl Pts',(131.056094103312,-31.7717594643386,17.606432860539));
#24727=CARTESIAN_POINT('Ctrl Pts',(130.848730782378,-31.7111522455224,17.620475932065));
#24728=CARTESIAN_POINT('Ctrl Pts',(130.440723554191,-31.6330853269384,17.6471676354725));
#24729=CARTESIAN_POINT('Ctrl Pts',(130.241457003235,-31.6129553756024,17.6597912237735));
#24730=CARTESIAN_POINT('Ctrl Pts',(129.996504147064,-31.6099524303263,17.6746053971701));
#24731=CARTESIAN_POINT('Ctrl Pts',(129.951447474415,-31.6102982888666,17.6773029781026));
#24732=CARTESIAN_POINT('Ctrl Pts',(129.877901061925,-31.612329671128,17.6816634435273));
#24733=CARTESIAN_POINT('Ctrl Pts',(129.84940317427,-31.613476845188,17.6833425559684));
#24734=CARTESIAN_POINT('Ctrl Pts',(129.793965853927,-31.6164096454853,17.6865895372866));
#24735=CARTESIAN_POINT('Ctrl Pts',(129.767026665636,-31.6181577145443,17.6881584330661));
#24736=CARTESIAN_POINT('Ctrl Pts',(129.703130681684,-31.6230710291277,17.6918597855181));
#24737=CARTESIAN_POINT('Ctrl Pts',(129.666198903818,-31.6265214321399,17.6939833455082));
#24738=CARTESIAN_POINT('Ctrl Pts',(129.541890723164,-31.6401965635318,17.7010842142481));
#24739=CARTESIAN_POINT('Ctrl Pts',(129.454854740657,-31.6532162297086,17.705976729016));
#24740=CARTESIAN_POINT('Ctrl Pts',(129.102215377666,-31.7200913790053,17.7256267014328));
#24741=CARTESIAN_POINT('Ctrl Pts',(128.843043375157,-31.8023039745643,17.7395819899753));
#24742=CARTESIAN_POINT('Ctrl Pts',(128.536169557994,-31.9418979547433,17.7578435251758));
#24743=CARTESIAN_POINT('Ctrl Pts',(128.4767287526,-31.9710675944567,17.7614733431461));
#24744=CARTESIAN_POINT('Ctrl Pts',(128.378398845571,-32.022948073835,17.767695627102));
#24745=CARTESIAN_POINT('Ctrl Pts',(128.339038193529,-32.0447277699912,17.7702471671157));
#24746=CARTESIAN_POINT('Ctrl Pts',(128.283021520079,-32.0771964229438,17.7739835673084));
#24747=CARTESIAN_POINT('Ctrl Pts',(128.266005979289,-32.0872589291292,17.7751328041374));
#24748=CARTESIAN_POINT('Ctrl Pts',(128.23626218091,-32.1052015532937,17.7771686632877));
#24749=CARTESIAN_POINT('Ctrl Pts',(128.223496593929,-32.1130180502889,17.7780513348182));
#24750=CARTESIAN_POINT('Ctrl Pts',(128.195387319012,-32.130486680041,17.7800151047999));
#24751=CARTESIAN_POINT('Ctrl Pts',(128.180069212159,-32.1401773627175,17.7810985249039));
#24752=CARTESIAN_POINT('Ctrl Pts',(128.134522445272,-32.1695057047648,17.7843580694332));
#24753=CARTESIAN_POINT('Ctrl Pts',(128.104529448348,-32.1895026015404,17.7865551929456));
#24754=CARTESIAN_POINT('Ctrl Pts',(127.950109119443,-32.2960536835067,17.7981105954731));
#24755=CARTESIAN_POINT('Ctrl Pts',(127.831279267454,-32.3903982079125,17.8078311676037));
#24756=CARTESIAN_POINT('Ctrl Pts',(127.620274920782,-32.5823182342661,17.8262058188554));
#24757=CARTESIAN_POINT('Ctrl Pts',(127.526783218911,-32.6780443680471,17.8348355513102));
#24758=CARTESIAN_POINT('Ctrl Pts',(127.345737839644,-32.8867938804341,17.8523767568404));
#24759=CARTESIAN_POINT('Ctrl Pts',(127.259173822995,-33.0003430635596,17.8612498184799));
#24760=CARTESIAN_POINT('Ctrl Pts',(127.15662883227,-33.1540797984807,17.8723963115759));
#24761=CARTESIAN_POINT('Ctrl Pts',(127.133899371468,-33.1895723115996,17.8749145222812));
#24762=CARTESIAN_POINT('Ctrl Pts',(127.097225588055,-33.2492616416814,17.8790606277824));
#24763=CARTESIAN_POINT('Ctrl Pts',(127.082908266727,-33.2732226619712,17.8807018318563));
#24764=CARTESIAN_POINT('Ctrl Pts',(127.055322196428,-33.3207123116181,17.8839103644606));
#24765=CARTESIAN_POINT('Ctrl Pts',(127.042035519745,-33.3442280644754,17.8854782469751));
#24766=CARTESIAN_POINT('Ctrl Pts',(127.013287952726,-33.3965582904307,17.8889227133214));
#24767=CARTESIAN_POINT('Ctrl Pts',(126.997959980009,-33.4254429217099,17.8907945805525));
#24768=CARTESIAN_POINT('Ctrl Pts',(126.94586323027,-33.5271432253532,17.8972881061284));
#24769=CARTESIAN_POINT('Ctrl Pts',(126.911305318637,-33.6010628842526,17.901835336003));
#24770=CARTESIAN_POINT('Ctrl Pts',(126.858897982631,-33.7245975362169,17.9092034732774));
#24771=CARTESIAN_POINT('Ctrl Pts',(126.839492810672,-33.7734760436544,17.9120614947518));
#24772=CARTESIAN_POINT('Ctrl Pts',(126.821241975899,-33.822756402985,17.9148966234937));
#24773=CARTESIAN_POINT('Origin',(130.,-35.,23.));
#24774=CARTESIAN_POINT('',(126.821241915874,-33.8227565650612,19.1602708352289));
#24775=CARTESIAN_POINT('',(126.821241893434,-33.8227566256554,18.8206072661261));
#24776=CARTESIAN_POINT('',(126.821241915871,-33.8227565650715,23.));
#24777=CARTESIAN_POINT('',(126.610251067749,-34.9973094977347,17.6410178032139));
#24778=CARTESIAN_POINT('Ctrl Pts',(126.821241893434,-33.8227566256554,18.8206072661261));
#24779=CARTESIAN_POINT('Ctrl Pts',(126.872479374406,-33.6844066790341,18.8127841894891));
#24780=CARTESIAN_POINT('Ctrl Pts',(126.932705550863,-33.5495191200307,18.8049941367639));
#24781=CARTESIAN_POINT('Ctrl Pts',(127.037869634602,-33.3500747900148,18.7926713874759));
#24782=CARTESIAN_POINT('Ctrl Pts',(127.076552171449,-33.2824667254386,18.7883412995881));
#24783=CARTESIAN_POINT('Ctrl Pts',(127.130542146319,-33.1952206221931,18.7824701353746));
#24784=CARTESIAN_POINT('Ctrl Pts',(127.143788586656,-33.17432936633,18.7810420946335));
#24785=CARTESIAN_POINT('Ctrl Pts',(127.164997311195,-33.1416764330164,18.778771873033));
#24786=CARTESIAN_POINT('Ctrl Pts',(127.172807166187,-33.1298162150347,18.7779392259102));
#24787=CARTESIAN_POINT('Ctrl Pts',(127.189336970124,-33.1050538545283,18.7761830540479));
#24788=CARTESIAN_POINT('Ctrl Pts',(127.198071642585,-33.0921622158202,18.7752584997376));
#24789=CARTESIAN_POINT('Ctrl Pts',(127.220391478412,-33.0597039032994,18.7729054933203));
#24790=CARTESIAN_POINT('Ctrl Pts',(127.234094501365,-33.0402196095835,18.7714696213604));
#24791=CARTESIAN_POINT('Ctrl Pts',(127.292175730443,-32.9594566312733,18.7654249352887));
#24792=CARTESIAN_POINT('Ctrl Pts',(127.338391257065,-32.8995317784167,18.7607139581683));
#24793=CARTESIAN_POINT('Ctrl Pts',(127.482307380556,-32.7253071129506,18.7464425807166));
#24794=CARTESIAN_POINT('Ctrl Pts',(127.585646593267,-32.6159070946926,18.7367079120512));
#24795=CARTESIAN_POINT('Ctrl Pts',(127.843950841067,-32.3765290529526,18.7140381619089));
#24796=CARTESIAN_POINT('Ctrl Pts',(128.003976365774,-32.2528090965189,18.7012126145115));
#24797=CARTESIAN_POINT('Ctrl Pts',(128.218745824074,-32.1154984803714,18.68569093999));
#24798=CARTESIAN_POINT('Ctrl Pts',(128.264076154793,-32.0879930745865,18.6824993711428));
#24799=CARTESIAN_POINT('Ctrl Pts',(128.336414855755,-32.0463893949651,18.6775352697771));
#24800=CARTESIAN_POINT('Ctrl Pts',(128.362998427676,-32.0315732986999,18.6757376260792));
#24801=CARTESIAN_POINT('Ctrl Pts',(128.41306159038,-32.0045481783305,18.6724005284951));
#24802=CARTESIAN_POINT('Ctrl Pts',(128.436491426823,-31.9922523157666,18.6708581275333));
#24803=CARTESIAN_POINT('Ctrl Pts',(128.489529453397,-31.965205471087,18.6674087726325));
#24804=CARTESIAN_POINT('Ctrl Pts',(128.519214639358,-31.9506108921657,18.6655073023659));
#24805=CARTESIAN_POINT('Ctrl Pts',(128.610903353846,-31.907187279465,18.6597189049237));
#24806=CARTESIAN_POINT('Ctrl Pts',(128.673571120008,-31.8797969116484,18.6558801290074));
#24807=CARTESIAN_POINT('Ctrl Pts',(128.82433161832,-31.8192674497629,18.646883010352));
#24808=CARTESIAN_POINT('Ctrl Pts',(128.913060561971,-31.7878636476055,18.6417756905233));
#24809=CARTESIAN_POINT('Ctrl Pts',(129.210783131956,-31.6962428785311,18.6250580347284));
#24810=CARTESIAN_POINT('Ctrl Pts',(129.424239369143,-31.6524387938148,18.6137671149021));
#24811=CARTESIAN_POINT('Ctrl Pts',(129.728490527445,-31.619980136382,18.5971368694424));
#24812=CARTESIAN_POINT('Ctrl Pts',(129.816899630509,-31.6140402425482,18.592236964465));
#24813=CARTESIAN_POINT('Ctrl Pts',(129.931168232004,-31.6108511249035,18.5857050149143));
#24814=CARTESIAN_POINT('Ctrl Pts',(129.956910556111,-31.610426114622,18.5842204741831));
#24815=CARTESIAN_POINT('Ctrl Pts',(129.998628748054,-31.6102126365942,18.5817899669335));
#24816=CARTESIAN_POINT('Ctrl Pts',(130.014603132038,-31.6102438177388,18.5808534404523));
#24817=CARTESIAN_POINT('Ctrl Pts',(130.046312340625,-31.6105298538767,18.5789817673671));
#24818=CARTESIAN_POINT('Ctrl Pts',(130.062046732567,-31.6107813761176,18.5780468085892));
#24819=CARTESIAN_POINT('Ctrl Pts',(130.102436165932,-31.6117083624268,18.5756318280374));
#24820=CARTESIAN_POINT('Ctrl Pts',(130.127086269569,-31.612543374149,18.5741436011085));
#24821=CARTESIAN_POINT('Ctrl Pts',(130.236231515571,-31.6174335860123,18.5674969431972));
#24822=CARTESIAN_POINT('Ctrl Pts',(130.320561165176,-31.6243816574958,18.5622103125906));
#24823=CARTESIAN_POINT('Ctrl Pts',(130.590819805894,-31.6568667108661,18.5449544077272));
#24824=CARTESIAN_POINT('Ctrl Pts',(130.774921413269,-31.6946852726754,18.5327380604987));
#24825=CARTESIAN_POINT('Ctrl Pts',(131.119304909335,-31.7957991067441,18.5097810698537));
#24826=CARTESIAN_POINT('Ctrl Pts',(131.279784417032,-31.856449069798,18.4990356839066));
#24827=CARTESIAN_POINT('Ctrl Pts',(131.475321083837,-31.9478183744436,18.48598938053));
#24828=CARTESIAN_POINT('Ctrl Pts',(131.515259950041,-31.9674478500741,18.4833259867266));
#24829=CARTESIAN_POINT('Ctrl Pts',(131.580010039091,-32.0008704467106,18.4790084581413));
#24830=CARTESIAN_POINT('Ctrl Pts',(131.605054064868,-32.0141983784849,18.4773386153349));
#24831=CARTESIAN_POINT('Ctrl Pts',(131.653591554047,-32.0408162650525,18.4741014986323));
#24832=CARTESIAN_POINT('Ctrl Pts',(131.677099357026,-32.0540754909154,18.4725333070905));
#24833=CARTESIAN_POINT('Ctrl Pts',(131.732712194422,-32.0863245478238,18.4688210940066));
#24834=CARTESIAN_POINT('Ctrl Pts',(131.764667424581,-32.1055665103633,18.4666862025069));
#24835=CARTESIAN_POINT('Ctrl Pts',(131.877453589975,-32.1760434378618,18.4591373253655));
#24836=CARTESIAN_POINT('Ctrl Pts',(131.956427944607,-32.2301706697105,18.4538273535168));
#24837=CARTESIAN_POINT('Ctrl Pts',(132.159303587464,-32.3822293628704,18.4399913404817));
#24838=CARTESIAN_POINT('Ctrl Pts',(132.278835326839,-32.4855959242417,18.4316394144455));
#24839=CARTESIAN_POINT('Ctrl Pts',(132.52336848855,-32.7288722685458,18.4133516375025));
#24840=CARTESIAN_POINT('Ctrl Pts',(132.64483913155,-32.8715684590044,18.403440393696));
#24841=CARTESIAN_POINT('Ctrl Pts',(132.774104580174,-33.0516804879517,18.3909148352169));
#24842=CARTESIAN_POINT('Ctrl Pts',(132.793869980971,-33.0801313903786,18.3889354357717));
#24843=CARTESIAN_POINT('Ctrl Pts',(132.823265630189,-33.123859791205,18.3858838012358));
#24844=CARTESIAN_POINT('Ctrl Pts',(132.833216113432,-33.138920387393,18.3848311294798));
#24845=CARTESIAN_POINT('Ctrl Pts',(132.851183733382,-33.166593413168,18.3828925184227));
#24846=CARTESIAN_POINT('Ctrl Pts',(132.859238425888,-33.1791804066967,18.3820090016143));
#24847=CARTESIAN_POINT('Ctrl Pts',(132.877759871358,-33.2085496471616,18.3799436211155));
#24848=CARTESIAN_POINT('Ctrl Pts',(132.888163230465,-33.2253706425049,18.378757909768));
#24849=CARTESIAN_POINT('Ctrl Pts',(132.921850351345,-33.2809195608662,18.3748356537938));
#24850=CARTESIAN_POINT('Ctrl Pts',(132.944506054018,-33.3200206216849,18.372064344113));
#24851=CARTESIAN_POINT('Ctrl Pts',(132.998623802116,-33.4178806216072,18.3651243598338));
#24852=CARTESIAN_POINT('Ctrl Pts',(133.029146924831,-33.4771361038905,18.3609187200448));
#24853=CARTESIAN_POINT('Ctrl Pts',(133.177026067828,-33.7862796863532,18.3390900475411));
#24854=CARTESIAN_POINT('Ctrl Pts',(133.265301156773,-34.0489725543816,18.3210233726508));
#24855=CARTESIAN_POINT('Ctrl Pts',(133.337659882871,-34.4020544940123,18.2986418583056));
#24856=CARTESIAN_POINT('Ctrl Pts',(133.351499164393,-34.4852500478249,18.2934898142347));
#24857=CARTESIAN_POINT('Ctrl Pts',(133.366429082766,-34.6016858558133,18.2864479223638));
#24858=CARTESIAN_POINT('Ctrl Pts',(133.370155257105,-34.6345515275437,18.2844786358201));
#24859=CARTESIAN_POINT('Ctrl Pts',(133.376058582061,-34.6944382097129,18.2809226455731));
#24860=CARTESIAN_POINT('Ctrl Pts',(133.378393736691,-34.7214405258275,18.279331207424));
#24861=CARTESIAN_POINT('Ctrl Pts',(133.382466923121,-34.7761812699939,18.2761281119568));
#24862=CARTESIAN_POINT('Ctrl Pts',(133.384188170422,-34.8039188838642,18.2745170891414));
#24863=CARTESIAN_POINT('Ctrl Pts',(133.387630316049,-34.873151788719,18.2705242603528));
#24864=CARTESIAN_POINT('Ctrl Pts',(133.388930157072,-34.9146640198602,18.268155480267));
#24865=CARTESIAN_POINT('Ctrl Pts',(133.391211033744,-35.0911335231722,18.258180995659));
#24866=CARTESIAN_POINT('Ctrl Pts',(133.384895344212,-35.2260670193766,18.2507971253351));
#24867=CARTESIAN_POINT('Ctrl Pts',(133.355835061997,-35.4979398308932,18.2360976861326));
#24868=CARTESIAN_POINT('Ctrl Pts',(133.332699803436,-35.6345753081353,18.2288024029005));
#24869=CARTESIAN_POINT('Ctrl Pts',(133.2630799492,-35.9332890870801,18.2125030741845));
#24870=CARTESIAN_POINT('Ctrl Pts',(133.212740722508,-36.094076702464,18.2034922062943));
#24871=CARTESIAN_POINT('Ctrl Pts',(133.140089794339,-36.2771317983322,18.1922827891402));
#24872=CARTESIAN_POINT('Ctrl Pts',(133.129159248019,-36.3036839463369,18.1906323372373));
#24873=CARTESIAN_POINT('Ctrl Pts',(133.111371119638,-36.3453813908292,18.1879967718016));
#24874=CARTESIAN_POINT('Ctrl Pts',(133.104736922516,-36.3606211623851,18.1870241875102));
#24875=CARTESIAN_POINT('Ctrl Pts',(133.091756207061,-36.3898505662743,18.1851396671487));
#24876=CARTESIAN_POINT('Ctrl Pts',(133.085426242942,-36.4038468240844,18.184228670821));
#24877=CARTESIAN_POINT('Ctrl Pts',(133.069542534958,-36.4383411049273,18.1819629060496));
#24878=CARTESIAN_POINT('Ctrl Pts',(133.059878442487,-36.4587872925124,18.1806018248118));
#24879=CARTESIAN_POINT('Ctrl Pts',(133.02177986218,-36.5373474708199,18.1753063967178));
#24880=CARTESIAN_POINT('Ctrl Pts',(132.991889921864,-36.5947364601631,18.1712981279529));
#24881=CARTESIAN_POINT('Ctrl Pts',(132.904597971617,-36.7512361804467,18.1600431191));
#24882=CARTESIAN_POINT('Ctrl Pts',(132.843788341487,-36.8483460157888,18.1526885743109));
#24883=CARTESIAN_POINT('Ctrl Pts',(132.631465179245,-37.1520617793127,18.1288196479806));
#24884=CARTESIAN_POINT('Ctrl Pts',(132.461411011713,-37.3446694078615,18.1123734838229));
#24885=CARTESIAN_POINT('Ctrl Pts',(132.233803173838,-37.5501127231479,18.0937499008354));
#24886=CARTESIAN_POINT('Ctrl Pts',(132.195591825298,-37.583085067533,18.090718049193));
#24887=CARTESIAN_POINT('Ctrl Pts',(132.133794364905,-37.6340472351923,18.0859601753148));
#24888=CARTESIAN_POINT('Ctrl Pts',(132.110685048688,-37.6526009759333,18.0842119226885));
#24889=CARTESIAN_POINT('Ctrl Pts',(132.066359731432,-37.6872423028046,18.0809157832972));
#24890=CARTESIAN_POINT('Ctrl Pts',(132.045191826167,-37.7033875392322,18.0793657187491));
#24891=CARTESIAN_POINT('Ctrl Pts',(131.996183847535,-37.7398619035306,18.0758304275401));
#24892=CARTESIAN_POINT('Ctrl Pts',(131.968219244793,-37.7600192630136,18.0738518384433));
#24893=CARTESIAN_POINT('Ctrl Pts',(131.877336565676,-37.8234451659866,18.0675397857226));
#24894=CARTESIAN_POINT('Ctrl Pts',(131.813260478001,-37.8650170688038,18.0632685564321));
#24895=CARTESIAN_POINT('Ctrl Pts',(131.653346132881,-37.9612517954993,18.0529807859348));
#24896=CARTESIAN_POINT('Ctrl Pts',(131.556138539751,-38.0134698723063,18.0470393456623));
#24897=CARTESIAN_POINT('Ctrl Pts',(131.26405781251,-38.152460730579,18.0297841027004));
#24898=CARTESIAN_POINT('Ctrl Pts',(131.063363848881,-38.2256931656923,18.0186901417195));
#24899=CARTESIAN_POINT('Ctrl Pts',(130.79039754933,-38.2970343272597,18.0031905499797));
#24900=CARTESIAN_POINT('Ctrl Pts',(130.723144287412,-38.3124348622644,17.9993373986244));
#24901=CARTESIAN_POINT('Ctrl Pts',(130.63214379847,-38.3303700489791,17.9940222027271));
#24902=CARTESIAN_POINT('Ctrl Pts',(130.608767773328,-38.3347222035616,17.9926479188277));
#24903=CARTESIAN_POINT('Ctrl Pts',(130.571542219136,-38.3412484237817,17.9904425171903));
#24904=CARTESIAN_POINT('Ctrl Pts',(130.557721218131,-38.3435831924806,17.9896200133399));
#24905=CARTESIAN_POINT('Ctrl Pts',(130.528418821226,-38.3483464844744,17.9878676412538));
#24906=CARTESIAN_POINT('Ctrl Pts',(130.512934484609,-38.3507534696772,17.9869365395897));
#24907=CARTESIAN_POINT('Ctrl Pts',(130.473101252477,-38.3566628375464,17.9845291745354));
#24908=CARTESIAN_POINT('Ctrl Pts',(130.44873021279,-38.3600076367347,17.9830446835731));
#24909=CARTESIAN_POINT('Ctrl Pts',(130.340283266068,-38.3736905512696,17.9763938969927));
#24910=CARTESIAN_POINT('Ctrl Pts',(130.255879136783,-38.3811394912298,17.9710980995961));
#24911=CARTESIAN_POINT('Ctrl Pts',(129.983389289538,-38.3949266414624,17.9537936223479));
#24912=CARTESIAN_POINT('Ctrl Pts',(129.795023440882,-38.388773793292,17.9415341060517));
#24913=CARTESIAN_POINT('Ctrl Pts',(129.437052341674,-38.3471125981063,17.9184678384327));
#24914=CARTESIAN_POINT('Ctrl Pts',(129.267712327729,-38.3141879324533,17.9076576356069));
#24915=CARTESIAN_POINT('Ctrl Pts',(129.058730850768,-38.2567457812821,17.8945556969853));
#24916=CARTESIAN_POINT('Ctrl Pts',(129.01610672144,-38.2441231472432,17.8918950544516));
#24917=CARTESIAN_POINT('Ctrl Pts',(128.946795296086,-38.2221055674022,17.8875859317341));
#24918=CARTESIAN_POINT('Ctrl Pts',(128.919956556696,-38.2132087808207,17.8859216547072));
#24919=CARTESIAN_POINT('Ctrl Pts',(128.867856397371,-38.1952115208429,17.882698338912));
#24920=CARTESIAN_POINT('Ctrl Pts',(128.842585664371,-38.1861446791763,17.8811383458599));
#24921=CARTESIAN_POINT('Ctrl Pts',(128.782739572441,-38.163866604405,17.8774508339721));
#24922=CARTESIAN_POINT('Ctrl Pts',(128.748267254708,-38.1503872978444,17.8753322919282));
#24923=CARTESIAN_POINT('Ctrl Pts',(128.626792755377,-38.1005797848743,17.867879709799));
#24924=CARTESIAN_POINT('Ctrl Pts',(128.541089620823,-38.0611886156602,17.8626467271575));
#24925=CARTESIAN_POINT('Ctrl Pts',(128.319971360017,-37.9481585207498,17.8490894622658));
#24926=CARTESIAN_POINT('Ctrl Pts',(128.187742043829,-37.8687731229112,17.8409305495564));
#24927=CARTESIAN_POINT('Ctrl Pts',(127.903132206333,-37.6703481708868,17.8225442555283));
#24928=CARTESIAN_POINT('Ctrl Pts',(127.754618625309,-37.5467352224207,17.8123493429224));
#24929=CARTESIAN_POINT('Ctrl Pts',(127.592876456827,-37.3869129949111,17.7995020696251));
#24930=CARTESIAN_POINT('Ctrl Pts',(127.568687843633,-37.3622697565442,17.7975289659534));
#24931=CARTESIAN_POINT('Ctrl Pts',(127.532474516033,-37.3242303670103,17.7944869797433));
#24932=CARTESIAN_POINT('Ctrl Pts',(127.520172400123,-37.3111001398097,17.7934376143206));
#24933=CARTESIAN_POINT('Ctrl Pts',(127.497835876034,-37.2868763629743,17.7915014614576));
#24934=CARTESIAN_POINT('Ctrl Pts',(127.487769518351,-37.2758134326629,17.7906170411775));
#24935=CARTESIAN_POINT('Ctrl Pts',(127.464521012875,-37.2499211180624,17.7885469536882));
#24936=CARTESIAN_POINT('Ctrl Pts',(127.451395444455,-37.2350421716924,17.7873573817174));
#24937=CARTESIAN_POINT('Ctrl Pts',(127.408718700198,-37.1857997149593,17.7834229196771));
#24938=CARTESIAN_POINT('Ctrl Pts',(127.379727158317,-37.1509600143214,17.7806431702724));
#24939=CARTESIAN_POINT('Ctrl Pts',(127.309722490491,-37.0633179667377,17.7736815097468));
#24940=CARTESIAN_POINT('Ctrl Pts',(127.269556988181,-37.0098642165119,17.7694625353038));
#24941=CARTESIAN_POINT('Ctrl Pts',(127.078705362645,-36.7395841170604,17.7483860149391));
#24942=CARTESIAN_POINT('Ctrl Pts',(126.952109567845,-36.5068195970155,17.731116821213));
#24943=CARTESIAN_POINT('Ctrl Pts',(126.81899010555,-36.1748767563502,17.7088108716309));
#24944=CARTESIAN_POINT('Ctrl Pts',(126.787772220534,-36.0866252862021,17.7030738942789));
#24945=CARTESIAN_POINT('Ctrl Pts',(126.74903620437,-35.960776209736,17.6951634063781));
#24946=CARTESIAN_POINT('Ctrl Pts',(126.738442944244,-35.9241765386893,17.692894075791));
#24947=CARTESIAN_POINT('Ctrl Pts',(126.721406087775,-35.8613679941586,17.6890512677439));
#24948=CARTESIAN_POINT('Ctrl Pts',(126.714654492358,-35.835247161283,17.6874681773312));
#24949=CARTESIAN_POINT('Ctrl Pts',(126.701459571084,-35.7815607998907,17.6842442175936));
#24950=CARTESIAN_POINT('Ctrl Pts',(126.695048248268,-35.7539895451384,17.6826044651235));
#24951=CARTESIAN_POINT('Ctrl Pts',(126.68281683795,-35.6982327706171,17.6793190421195));
#24952=CARTESIAN_POINT('Ctrl Pts',(126.677008842061,-35.6700469891726,17.6776738631822));
#24953=CARTESIAN_POINT('Ctrl Pts',(126.663698493986,-35.6010171084343,17.6736804751609));
#24954=CARTESIAN_POINT('Ctrl Pts',(126.656586298347,-35.5601020621826,17.6713440228477));
#24955=CARTESIAN_POINT('Ctrl Pts',(126.623479488232,-35.3464483074093,17.6592834070774));
#24956=CARTESIAN_POINT('Ctrl Pts',(126.610113414419,-35.1720170055958,17.6499289047321));
#24957=CARTESIAN_POINT('Ctrl Pts',(126.610251052174,-34.9973291930011,17.6406471279412));
#24958=CARTESIAN_POINT('Ctrl Pts',(126.610251067749,-34.9973094977347,17.6410178032139));
#24959=CARTESIAN_POINT('Ctrl Pts',(126.610355871654,-34.865267636549,17.6332712573477));
#24960=CARTESIAN_POINT('Ctrl Pts',(126.618179523068,-34.733553041647,17.6255247114816));
#24961=CARTESIAN_POINT('Ctrl Pts',(126.633585920167,-34.6029341293948,17.6177781656156));
#24962=CARTESIAN_POINT('Ctrl Pts',(126.649300610227,-34.4697014398218,17.6098766058579));
#24963=CARTESIAN_POINT('Ctrl Pts',(126.672904558712,-34.3376084643416,17.6019750461003));
#24964=CARTESIAN_POINT('Ctrl Pts',(126.704204838343,-34.2074475948576,17.5940734863427));
#24965=CARTESIAN_POINT('Ctrl Pts',(126.707948416483,-34.191880085832,17.5931284434636));
#24966=CARTESIAN_POINT('Ctrl Pts',(126.711802031722,-34.1763401910708,17.5921834005845));
#24967=CARTESIAN_POINT('Ctrl Pts',(126.715765308226,-34.1608292475032,17.5912383577054));
#24968=CARTESIAN_POINT('Ctrl Pts',(126.741359218008,-34.0606632131708,17.5851354925212));
#24969=CARTESIAN_POINT('Ctrl Pts',(126.77158242967,-33.9615021246093,17.579032627337));
#24970=CARTESIAN_POINT('Ctrl Pts',(126.806339696859,-33.863805064858,17.5729297621527));
#24971=CARTESIAN_POINT('Ctrl Pts',(126.811217984641,-33.8500929864498,17.5720732065293));
#24972=CARTESIAN_POINT('Ctrl Pts',(126.816185505764,-33.8364097348622,17.5712166509059));
#24973=CARTESIAN_POINT('Ctrl Pts',(126.821241915871,-33.8227565650715,17.5703600952825));
#24974=CARTESIAN_POINT('Ctrl Pts',(126.821241975899,-33.822756402985,17.9148966234937));
#24975=CARTESIAN_POINT('Ctrl Pts',(126.742546197666,-34.0352483945782,17.9271214157023));
#24976=CARTESIAN_POINT('Ctrl Pts',(126.685311296885,-34.2552138019534,17.9388788299414));
#24977=CARTESIAN_POINT('Ctrl Pts',(126.640195493197,-34.5454746126536,17.9547793874544));
#24978=CARTESIAN_POINT('Ctrl Pts',(126.631880958229,-34.611859722398,17.9584447972027));
#24979=CARTESIAN_POINT('Ctrl Pts',(126.621238169152,-34.7235468980125,17.9647214780077));
#24980=CARTESIAN_POINT('Ctrl Pts',(126.617845161582,-34.7687294485601,17.9672907212788));
#24981=CARTESIAN_POINT('Ctrl Pts',(126.614272276037,-34.8337326882671,17.9710471355269));
#24982=CARTESIAN_POINT('Ctrl Pts',(126.613358943449,-34.8535098883138,17.9721980028177));
#24983=CARTESIAN_POINT('Ctrl Pts',(126.612060270353,-34.8882286937041,17.9742340908642));
#24984=CARTESIAN_POINT('Ctrl Pts',(126.61160041897,-34.9031666160634,17.9751153082091));
#24985=CARTESIAN_POINT('Ctrl Pts',(126.610803622922,-34.9361385413936,17.9770722020195));
#24986=CARTESIAN_POINT('Ctrl Pts',(126.610511815254,-34.9541722615471,17.978150144148));
#24987=CARTESIAN_POINT('Ctrl Pts',(126.610071562035,-35.0078655716658,17.9813806106298));
#24988=CARTESIAN_POINT('Ctrl Pts',(126.610341899981,-35.0435250438162,17.983553654545));
#24989=CARTESIAN_POINT('Ctrl Pts',(126.615219413334,-35.2522987528171,17.9964123801132));
#24990=CARTESIAN_POINT('Ctrl Pts',(126.632524775447,-35.4248481566212,18.0075757552706));
#24991=CARTESIAN_POINT('Ctrl Pts',(126.692217547691,-35.7594643548647,18.0294869038277));
#24992=CARTESIAN_POINT('Ctrl Pts',(126.733577611508,-35.9212513033148,18.0402040886711));
#24993=CARTESIAN_POINT('Ctrl Pts',(126.818119506551,-36.1729406631513,18.05679038483));
#24994=CARTESIAN_POINT('Ctrl Pts',(126.853633743345,-36.2651227487906,18.062849467648));
#24995=CARTESIAN_POINT('Ctrl Pts',(126.908200264692,-36.3901799965359,18.0710431028602));
#24996=CARTESIAN_POINT('Ctrl Pts',(126.92385123098,-36.4244770791736,18.0732876594508));
#24997=CARTESIAN_POINT('Ctrl Pts',(126.951712606116,-36.4829298758816,18.0771100750361));
#24998=CARTESIAN_POINT('Ctrl Pts',(126.963645910807,-36.5072129779049,18.0786971296182));
#24999=CARTESIAN_POINT('Ctrl Pts',(126.988628986083,-36.5565498621974,18.0819207510702));
#25000=CARTESIAN_POINT('Ctrl Pts',(127.001703768039,-36.5815886420373,18.0835562987486));
#25001=CARTESIAN_POINT('Ctrl Pts',(127.035892859641,-36.6451141874476,18.0877064703405));
#25002=CARTESIAN_POINT('Ctrl Pts',(127.057444890778,-36.6833601834662,18.0902056770278));
#25003=CARTESIAN_POINT('Ctrl Pts',(127.158033880521,-36.8540261765712,18.1013763490971));
#25004=CARTESIAN_POINT('Ctrl Pts',(127.245311037512,-36.9813834030212,18.1097524451115));
#25005=CARTESIAN_POINT('Ctrl Pts',(127.361761917975,-37.1286684165079,18.1197877427296));
#25006=CARTESIAN_POINT('Ctrl Pts',(127.382947691325,-37.1546616099905,18.121573565333));
#25007=CARTESIAN_POINT('Ctrl Pts',(127.527383069498,-37.326598263652,18.1335087744686));
#25008=CARTESIAN_POINT('Ctrl Pts',(127.662385320098,-37.4622027197175,18.1435048935434));
#25009=CARTESIAN_POINT('Ctrl Pts',(127.860000073998,-37.6297221624873,18.1577444317777));
#25010=CARTESIAN_POINT('Ctrl Pts',(127.913233223272,-37.6721604618926,18.1615482296479));
#25011=CARTESIAN_POINT('Ctrl Pts',(127.986639249914,-37.7271492989601,18.1668050267503));
#25012=CARTESIAN_POINT('Ctrl Pts',(128.005721961065,-37.7411347731954,18.1681726127466));
#25013=CARTESIAN_POINT('Ctrl Pts',(128.036322262084,-37.7630726810373,18.1703699412898));
#25014=CARTESIAN_POINT('Ctrl Pts',(128.04774576274,-37.771155765516,18.1711911762168));
#25015=CARTESIAN_POINT('Ctrl Pts',(128.072168910665,-37.7882112267234,18.1729497030175));
#25016=CARTESIAN_POINT('Ctrl Pts',(128.085181804485,-37.797163886516,18.1738883093237));
#25017=CARTESIAN_POINT('Ctrl Pts',(128.118877158737,-37.8200004330194,18.176321943342));
#25018=CARTESIAN_POINT('Ctrl Pts',(128.139650614521,-37.833747637063,18.1778253925099));
#25019=CARTESIAN_POINT('Ctrl Pts',(128.233896834548,-37.894633817142,18.1846534521182));
#25020=CARTESIAN_POINT('Ctrl Pts',(128.309017618409,-37.9391497939088,18.1901145102757));
#25021=CARTESIAN_POINT('Ctrl Pts',(128.562564195531,-38.0764603716429,18.2084111320971));
#25022=CARTESIAN_POINT('Ctrl Pts',(128.747529951231,-38.1562876207681,18.2215191385987));
#25023=CARTESIAN_POINT('Ctrl Pts',(129.086265750315,-38.2679824174949,18.2442529740116));
#25024=CARTESIAN_POINT('Ctrl Pts',(129.237242419853,-38.3064831384604,18.2539759954902));
#25025=CARTESIAN_POINT('Ctrl Pts',(129.433612589681,-38.3423860922147,18.2660370087093));
#25026=CARTESIAN_POINT('Ctrl Pts',(129.477028794827,-38.3494538180393,18.2686686583663));
#25027=CARTESIAN_POINT('Ctrl Pts',(129.54856497468,-38.3596742537292,18.2729492882096));
#25028=CARTESIAN_POINT('Ctrl Pts',(129.576607664316,-38.3633233082362,18.2746134255675));
#25029=CARTESIAN_POINT('Ctrl Pts',(129.631578842907,-38.3697779908043,18.2778494120573));
#25030=CARTESIAN_POINT('Ctrl Pts',(129.65850170181,-38.3726127602939,18.2794220475535));
#25031=CARTESIAN_POINT('Ctrl Pts',(129.722985151813,-38.3786222768921,18.283160893169));
#25032=CARTESIAN_POINT('Ctrl Pts',(129.760570812204,-38.381493684856,18.2853176406677));
#25033=CARTESIAN_POINT('Ctrl Pts',(129.896601036891,-38.3896063762216,18.2930495096983));
#25034=CARTESIAN_POINT('Ctrl Pts',(129.995218555166,-38.3911800628745,18.2985135970312));
#25035=CARTESIAN_POINT('Ctrl Pts',(130.259982339619,-38.3838530728876,18.3129496554169));
#25036=CARTESIAN_POINT('Ctrl Pts',(130.425635436939,-38.3670298453148,18.3217256475646));
#25037=CARTESIAN_POINT('Ctrl Pts',(130.760502564446,-38.3079048222386,18.3397663067097));
#25038=CARTESIAN_POINT('Ctrl Pts',(130.929025161924,-38.264582429495,18.3490119741938));
#25039=CARTESIAN_POINT('Ctrl Pts',(131.127198495656,-38.1970453090688,18.3608337963474));
#25040=CARTESIAN_POINT('Ctrl Pts',(131.160746944978,-38.1850182850464,18.3628694341934));
#25041=CARTESIAN_POINT('Ctrl Pts',(131.210981919776,-38.1661101213727,18.3659782799465));
#25042=CARTESIAN_POINT('Ctrl Pts',(131.227814304606,-38.1596206279186,18.3670303620466));
#25043=CARTESIAN_POINT('Ctrl Pts',(131.258500617846,-38.1475077117334,18.3689688014109));
#25044=CARTESIAN_POINT('Ctrl Pts',(131.272370277748,-38.1419265507441,18.3698527520082));
#25045=CARTESIAN_POINT('Ctrl Pts',(131.304534209077,-38.1287358676301,18.3719206923424));
#25046=CARTESIAN_POINT('Ctrl Pts',(131.322799120678,-38.1210575253567,18.3731085551237));
#25047=CARTESIAN_POINT('Ctrl Pts',(131.382693801934,-38.0952583572703,18.3770460636406));
#25048=CARTESIAN_POINT('Ctrl Pts',(131.424025266718,-38.0764619393618,18.3798308321482));
#25049=CARTESIAN_POINT('Ctrl Pts',(131.525470725824,-38.0278451003667,18.3868131419406));
#25050=CARTESIAN_POINT('Ctrl Pts',(131.58509968408,-37.9970593870271,18.3910481812307));
#25051=CARTESIAN_POINT('Ctrl Pts',(131.890786374131,-37.8275620167856,18.4133166027036));
#25052=CARTESIAN_POINT('Ctrl Pts',(132.119756924759,-37.6602346346548,18.4318015867138));
#25053=CARTESIAN_POINT('Ctrl Pts',(132.382870797524,-37.4121750693482,18.4541959423932));
#25054=CARTESIAN_POINT('Ctrl Pts',(132.438511173619,-37.3559131115129,18.4590199506016));
#25055=CARTESIAN_POINT('Ctrl Pts',(132.514032687282,-37.2740026894461,18.4656968409419));
#25056=CARTESIAN_POINT('Ctrl Pts',(132.535589703829,-37.2499407873399,18.4676187016614));
#25057=CARTESIAN_POINT('Ctrl Pts',(132.57446485489,-37.2052799500275,18.4711152887041));
#25058=CARTESIAN_POINT('Ctrl Pts',(132.591887789899,-37.1847761198377,18.472694218555));
#25059=CARTESIAN_POINT('Ctrl Pts',(132.626961324399,-37.1424903891693,18.4758981838077));
#25060=CARTESIAN_POINT('Ctrl Pts',(132.644589549149,-37.1206925880053,18.4775222555223));
#25061=CARTESIAN_POINT('Ctrl Pts',(132.688436208715,-37.0650778526825,18.4815987891301));
#25062=CARTESIAN_POINT('Ctrl Pts',(132.714288903343,-37.0309780319581,18.4840369732826));
#25063=CARTESIAN_POINT('Ctrl Pts',(132.828873267993,-36.8737434000694,18.4950192977643));
#25064=CARTESIAN_POINT('Ctrl Pts',(132.909923400294,-36.7452194459429,18.5032763502417));
#25065=CARTESIAN_POINT('Ctrl Pts',(133.003058114906,-36.5728926723312,18.5137573189503));
#25066=CARTESIAN_POINT('Ctrl Pts',(133.023264564435,-36.5336951625509,18.5161050236613));
#25067=CARTESIAN_POINT('Ctrl Pts',(133.131185549468,-36.3139186180434,18.5291112895381));
#25068=CARTESIAN_POINT('Ctrl Pts',(133.203480922128,-36.1262336873626,18.5396166872158));
#25069=CARTESIAN_POINT('Ctrl Pts',(133.274168459502,-35.8794117713362,18.5538461856615));
#25070=CARTESIAN_POINT('Ctrl Pts',(133.288255491707,-35.8251783221317,18.5569988105232));
#25071=CARTESIAN_POINT('Ctrl Pts',(133.305997809209,-35.7491785622284,18.5614837708066));
#25072=CARTESIAN_POINT('Ctrl Pts',(133.310795041277,-35.7276854898212,18.5627595369943));
#25073=CARTESIAN_POINT('Ctrl Pts',(133.318524602358,-35.691394999471,18.5649283821967));
#25074=CARTESIAN_POINT('Ctrl Pts',(133.321568274232,-35.6766215898298,18.5658154125245));
#25075=CARTESIAN_POINT('Ctrl Pts',(133.327784335631,-35.6453969083609,18.5676996797267));
#25076=CARTESIAN_POINT('Ctrl Pts',(133.330933483938,-35.6289418519974,18.568698072102));
#25077=CARTESIAN_POINT('Ctrl Pts',(133.339268824645,-35.5835682907358,18.5714646538095));
#25078=CARTESIAN_POINT('Ctrl Pts',(133.344201108174,-35.5546053144903,18.5732457794629));
#25079=CARTESIAN_POINT('Ctrl Pts',(133.377084226314,-35.3450902651531,18.5862218493349));
#25080=CARTESIAN_POINT('Ctrl Pts',(133.390771218413,-35.1626177062943,18.5979964196479));
#25081=CARTESIAN_POINT('Ctrl Pts',(133.388291363512,-34.7433832583471,18.6250213381813));
#25082=CARTESIAN_POINT('Ctrl Pts',(133.362130793579,-34.5075786205291,18.6401649137118));
#25083=CARTESIAN_POINT('Ctrl Pts',(133.300529997481,-34.2256590417183,18.6577220000289));
#25084=CARTESIAN_POINT('Ctrl Pts',(133.288278822042,-34.175181826916,18.6608466664282));
#25085=CARTESIAN_POINT('Ctrl Pts',(133.267077481984,-34.0958309879908,18.6657306688188));
#25086=CARTESIAN_POINT('Ctrl Pts',(133.258893281555,-34.066762868622,18.6675138100103));
#25087=CARTESIAN_POINT('Ctrl Pts',(133.243557427608,-34.0149578041453,18.6706819713804));
#25088=CARTESIAN_POINT('Ctrl Pts',(133.23655242203,-33.9921798890356,18.6720715644554));
#25089=CARTESIAN_POINT('Ctrl Pts',(133.219549827643,-33.93889954081,18.6753148693733));
#25090=CARTESIAN_POINT('Ctrl Pts',(133.209357947523,-33.9084612040258,18.6771621894245));
#25091=CARTESIAN_POINT('Ctrl Pts',(133.177867064261,-33.8186694164423,18.6825986761169));
#25092=CARTESIAN_POINT('Ctrl Pts',(133.155342094371,-33.7597588996141,18.6861481439059));
#25093=CARTESIAN_POINT('Ctrl Pts',(133.071184427493,-33.5568209103673,18.6983564846071));
#25094=CARTESIAN_POINT('Ctrl Pts',(133.001223381791,-33.4164585476328,18.7067563143908));
#25095=CARTESIAN_POINT('Ctrl Pts',(132.822420502467,-33.112469274648,18.7254963833426));
#25096=CARTESIAN_POINT('Ctrl Pts',(132.708578115965,-32.9524592028829,18.7357545263718));
#25097=CARTESIAN_POINT('Ctrl Pts',(132.541560314946,-32.7561894822093,18.7499797088768));
#25098=CARTESIAN_POINT('Ctrl Pts',(132.500287046359,-32.7102886160496,18.7534410390833));
#25099=CARTESIAN_POINT('Ctrl Pts',(132.442054517504,-32.6489796613059,18.7582937228304));
#25100=CARTESIAN_POINT('Ctrl Pts',(132.426155886665,-32.6325764105409,18.759615607848));
#25101=CARTESIAN_POINT('Ctrl Pts',(132.399385536062,-32.6055092452614,18.761839030863));
#25102=CARTESIAN_POINT('Ctrl Pts',(132.388605223777,-32.5947553133353,18.7627337762472));
#25103=CARTESIAN_POINT('Ctrl Pts',(132.366029953173,-32.5725367422475,18.764607071456));
#25104=CARTESIAN_POINT('Ctrl Pts',(132.354223493009,-32.5610848052609,18.7655864510681));
#25105=CARTESIAN_POINT('Ctrl Pts',(132.32213319358,-32.5304082302105,18.7682463979172));
#25106=CARTESIAN_POINT('Ctrl Pts',(132.301694610797,-32.5113481788546,18.7699383749244));
#25107=CARTESIAN_POINT('Ctrl Pts',(132.176650579833,-32.3975961004797,18.7802643474275));
#25108=CARTESIAN_POINT('Ctrl Pts',(132.06646031676,-32.3092662225133,18.789251639162));
#25109=CARTESIAN_POINT('Ctrl Pts',(131.755785293099,-32.0905892657241,18.8136751399559));
#25110=CARTESIAN_POINT('Ctrl Pts',(131.546460729699,-31.9741220393048,18.8291495214459));
#25111=CARTESIAN_POINT('Ctrl Pts',(131.255407028713,-31.8503419047845,18.8487181809404));
#25112=CARTESIAN_POINT('Ctrl Pts',(131.183177960155,-31.8225034579676,18.853434021677));
#25113=CARTESIAN_POINT('Ctrl Pts',(131.07680873452,-31.7856375320606,18.8601782595072));
#25114=CARTESIAN_POINT('Ctrl Pts',(131.043384477365,-31.774633028868,18.8622694667274));
#25115=CARTESIAN_POINT('Ctrl Pts',(130.984242693153,-31.756176973093,18.8659218907131));
#25116=CARTESIAN_POINT('Ctrl Pts',(130.958597353015,-31.7485060841511,18.8674900448567));
#25117=CARTESIAN_POINT('Ctrl Pts',(130.905045337785,-31.7331765816433,18.8707332236701));
#25118=CARTESIAN_POINT('Ctrl Pts',(130.87712597474,-31.7255699106833,18.8724064802458));
#25119=CARTESIAN_POINT('Ctrl Pts',(130.803418281729,-31.7064985465092,18.8767799067361));
#25120=CARTESIAN_POINT('Ctrl Pts',(130.757481168686,-31.6956308704177,18.8794611586634));
#25121=CARTESIAN_POINT('Ctrl Pts',(130.500602450114,-31.640497941406,18.8942336851626));
#25122=CARTESIAN_POINT('Ctrl Pts',(130.286036047075,-31.6154686476948,18.9057081681737));
#25123=CARTESIAN_POINT('Ctrl Pts',(129.864530546271,-31.6066968560081,18.9280616241933));
#25124=CARTESIAN_POINT('Ctrl Pts',(129.658594487553,-31.6212011923239,18.9389118029072));
#25125=CARTESIAN_POINT('Ctrl Pts',(129.422296688807,-31.6596736027537,18.9524564735133));
#25126=CARTESIAN_POINT('Ctrl Pts',(129.389399459689,-31.6655302729447,18.9543677409905));
#25127=CARTESIAN_POINT('Ctrl Pts',(129.339121196669,-31.675250229995,18.9573354323215));
#25128=CARTESIAN_POINT('Ctrl Pts',(129.321674194063,-31.6787659076372,18.958373903616));
#25129=CARTESIAN_POINT('Ctrl Pts',(129.289596782035,-31.6854929963254,18.9603004959578));
#25130=CARTESIAN_POINT('Ctrl Pts',(129.274958829442,-31.6886642148989,18.9611864381891));
#25131=CARTESIAN_POINT('Ctrl Pts',(129.240679099206,-31.696328888878,18.9632768311574));
#25132=CARTESIAN_POINT('Ctrl Pts',(129.221055836689,-31.7009005793288,18.9644854538693));
#25133=CARTESIAN_POINT('Ctrl Pts',(129.155367778879,-31.7168228411771,18.9685688919492));
#25134=CARTESIAN_POINT('Ctrl Pts',(129.109502613729,-31.7289650303944,18.9714823328456));
#25135=CARTESIAN_POINT('Ctrl Pts',(128.99525996173,-31.7617899380875,18.978871068747));
#25136=CARTESIAN_POINT('Ctrl Pts',(128.927253994525,-31.7836788233089,18.9833891606425));
#25137=CARTESIAN_POINT('Ctrl Pts',(128.707117692007,-31.8622919144508,18.998309184041));
#25138=CARTESIAN_POINT('Ctrl Pts',(128.558360746719,-31.9277965724441,19.0088507860279));
#25139=CARTESIAN_POINT('Ctrl Pts',(128.263205566821,-32.0839428285042,19.0302111957088));
#25140=CARTESIAN_POINT('Ctrl Pts',(128.117837333673,-32.1755846957157,19.0409776975598));
#25141=CARTESIAN_POINT('Ctrl Pts',(127.943986652209,-32.3045914302407,19.054067765254));
#25142=CARTESIAN_POINT('Ctrl Pts',(127.908488116279,-32.33204262144,19.0567541039752));
#25143=CARTESIAN_POINT('Ctrl Pts',(127.851384171362,-32.3780418077401,19.0610995874499));
#25144=CARTESIAN_POINT('Ctrl Pts',(127.829449772376,-32.3961707958878,19.0627748092974));
#25145=CARTESIAN_POINT('Ctrl Pts',(127.787177295572,-32.432014802443,19.0660162626987));
#25146=CARTESIAN_POINT('Ctrl Pts',(127.76681729208,-32.4497005370415,19.0675834933851));
#25147=CARTESIAN_POINT('Ctrl Pts',(127.718951662944,-32.4922918481688,19.0712838446877));
#25148=CARTESIAN_POINT('Ctrl Pts',(127.691639343045,-32.5174100375277,19.0734080204768));
#25149=CARTESIAN_POINT('Ctrl Pts',(127.596497904265,-32.6078362071488,19.0808601780285));
#25150=CARTESIAN_POINT('Ctrl Pts',(127.530980377487,-32.6755185264377,19.0860879141772));
#25151=CARTESIAN_POINT('Ctrl Pts',(127.366309369364,-32.860460328479,19.0996118788348));
#25152=CARTESIAN_POINT('Ctrl Pts',(127.272154537069,-32.9818774315783,19.1077449333051));
#25153=CARTESIAN_POINT('Ctrl Pts',(127.078619855762,-33.2698600250653,19.1261397481423));
#25154=CARTESIAN_POINT('Ctrl Pts',(126.984651439986,-33.4393901057894,19.136367731128));
#25155=CARTESIAN_POINT('Ctrl Pts',(126.891515948642,-33.647619573974,19.1492555193022));
#25156=CARTESIAN_POINT('Ctrl Pts',(126.877853698947,-33.679466700531,19.1512355482606));
#25157=CARTESIAN_POINT('Ctrl Pts',(126.857818504125,-33.7282191195397,19.1542882232668));
#25158=CARTESIAN_POINT('Ctrl Pts',(126.851088120362,-33.7449760546561,19.1553413055566));
#25159=CARTESIAN_POINT('Ctrl Pts',(126.83903263467,-33.7756986652119,19.1572804176327));
#25160=CARTESIAN_POINT('Ctrl Pts',(126.833665552645,-33.7896469175918,19.1581640207011));
#25161=CARTESIAN_POINT('Ctrl Pts',(126.825988669521,-33.8099985449431,19.1594578654587));
#25162=CARTESIAN_POINT('Ctrl Pts',(126.823605668016,-33.8163740310795,19.1598638224713));
#25163=CARTESIAN_POINT('Ctrl Pts',(126.821241915874,-33.8227565650612,19.1602708352289));
#25164=CARTESIAN_POINT('Origin',(130.,-35.,23.));
#25165=CARTESIAN_POINT('',(126.821241916136,-33.8227565643555,20.4155868599104));
#25166=CARTESIAN_POINT('',(126.82124191022,-33.822756580328,20.0676573852273));
#25167=CARTESIAN_POINT('',(126.821241915871,-33.8227565650715,23.));
#25168=CARTESIAN_POINT('Ctrl Pts',(126.82124191022,-33.822756580328,20.0676573852273));
#25169=CARTESIAN_POINT('Ctrl Pts',(126.830737944534,-33.7971156675063,20.0659955135839));
#25170=CARTESIAN_POINT('Ctrl Pts',(126.840545002458,-33.7715875409957,20.0643431471796));
#25171=CARTESIAN_POINT('Ctrl Pts',(126.864662288883,-33.7110099642004,20.0604270690341));
#25172=CARTESIAN_POINT('Ctrl Pts',(126.879251901058,-33.6760780414383,20.0581728848126));
#25173=CARTESIAN_POINT('Ctrl Pts',(126.905283146217,-33.6165742766722,20.0543385598621));
#25174=CARTESIAN_POINT('Ctrl Pts',(126.916439715656,-33.5918824007403,20.0527490979748));
#25175=CARTESIAN_POINT('Ctrl Pts',(126.939819199682,-33.5417493389165,20.0495243248565));
#25176=CARTESIAN_POINT('Ctrl Pts',(126.952066224576,-33.5163217020307,20.0478899859034));
#25177=CARTESIAN_POINT('Ctrl Pts',(126.984094549459,-33.4518942595872,20.0437504203348));
#25178=CARTESIAN_POINT('Ctrl Pts',(127.004315838557,-33.413118239776,20.0412604214548));
#25179=CARTESIAN_POINT('Ctrl Pts',(127.097667401596,-33.2422563130808,20.0302795296636));
#25180=CARTESIAN_POINT('Ctrl Pts',(127.178825954979,-33.1147464245847,20.022070276748));
#25181=CARTESIAN_POINT('Ctrl Pts',(127.389761482984,-32.8276280513897,20.0030122806015));
#25182=CARTESIAN_POINT('Ctrl Pts',(127.526069272746,-32.6735855359763,19.9923253809962));
#25183=CARTESIAN_POINT('Ctrl Pts',(127.739579145407,-32.4724197106059,19.9763680460375));
#25184=CARTESIAN_POINT('Ctrl Pts',(127.806017957918,-32.4145397079635,19.971490269403));
#25185=CARTESIAN_POINT('Ctrl Pts',(127.894087136384,-32.3436566622624,19.965023333165));
#25186=CARTESIAN_POINT('Ctrl Pts',(127.913716667303,-32.3282120790643,19.9635818384173));
#25187=CARTESIAN_POINT('Ctrl Pts',(127.946046125913,-32.3033486556651,19.9612043081926));
#25188=CARTESIAN_POINT('Ctrl Pts',(127.958644812193,-32.2937989788841,19.9602769608721));
#25189=CARTESIAN_POINT('Ctrl Pts',(127.98251934731,-32.2759639021357,19.9585171207978));
#25190=CARTESIAN_POINT('Ctrl Pts',(127.993780636098,-32.2676594841001,19.9576859968555));
#25191=CARTESIAN_POINT('Ctrl Pts',(128.024187885427,-32.2455255723737,19.9554397952754));
#25192=CARTESIAN_POINT('Ctrl Pts',(128.043427149575,-32.231826324622,19.9540164323293));
#25193=CARTESIAN_POINT('Ctrl Pts',(128.118338628393,-32.1796569639005,19.9484709992904));
#25194=CARTESIAN_POINT('Ctrl Pts',(128.17501187875,-32.1426583185284,19.9442689008102));
#25195=CARTESIAN_POINT('Ctrl Pts',(128.395952137029,-32.0076744539395,19.9279694184905));
#25196=CARTESIAN_POINT('Ctrl Pts',(128.567295312653,-31.9219589279726,19.9155194535873));
#25197=CARTESIAN_POINT('Ctrl Pts',(128.904312611274,-31.7876323888814,19.8922542655064));
#25198=CARTESIAN_POINT('Ctrl Pts',(129.068284640661,-31.7362971708579,19.8814339471127));
#25199=CARTESIAN_POINT('Ctrl Pts',(129.28657457001,-31.6857606861343,19.8678024442814));
#25200=CARTESIAN_POINT('Ctrl Pts',(129.337961581155,-31.6751144883008,19.8646461456914));
#25201=CARTESIAN_POINT('Ctrl Pts',(129.419105452088,-31.6602593331375,19.8597423693043));
#25202=CARTESIAN_POINT('Ctrl Pts',(129.44870480714,-31.6552459141466,19.8579701826528));
#25203=CARTESIAN_POINT('Ctrl Pts',(129.504556779525,-31.6465475122618,19.8546563134145));
#25204=CARTESIAN_POINT('Ctrl Pts',(129.530793436295,-31.6427760230205,19.8531120542259));
#25205=CARTESIAN_POINT('Ctrl Pts',(129.590463085674,-31.6349117549119,19.849626977559));
#25206=CARTESIAN_POINT('Ctrl Pts',(129.623918525166,-31.6310087233696,19.8476921580684));
#25207=CARTESIAN_POINT('Ctrl Pts',(129.728894506189,-31.6203451188357,19.8416767545401));
#25208=CARTESIAN_POINT('Ctrl Pts',(129.800577317753,-31.6153586754793,19.8376502534484));
#25209=CARTESIAN_POINT('Ctrl Pts',(130.118771119807,-31.6033694477644,19.8200529042631));
#25210=CARTESIAN_POINT('Ctrl Pts',(130.365445416647,-31.6209973013003,19.8072052574937));
#25211=CARTESIAN_POINT('Ctrl Pts',(130.749659797129,-31.691051439037,19.7863666261384));
#25212=CARTESIAN_POINT('Ctrl Pts',(130.889485008773,-31.7258683162843,19.7785838720519));
#25213=CARTESIAN_POINT('Ctrl Pts',(131.053378387976,-31.7779532712119,19.7687876179265));
#25214=CARTESIAN_POINT('Ctrl Pts',(131.079991486189,-31.7867758508939,19.767174955232));
#25215=CARTESIAN_POINT('Ctrl Pts',(131.122056708702,-31.8013026110357,19.7645865013402));
#25216=CARTESIAN_POINT('Ctrl Pts',(131.137582527387,-31.8067912357063,19.7636225203716));
#25217=CARTESIAN_POINT('Ctrl Pts',(131.167377667414,-31.8175691641814,19.761754860786));
#25218=CARTESIAN_POINT('Ctrl Pts',(131.181652359512,-31.8228417868254,19.7608521132334));
#25219=CARTESIAN_POINT('Ctrl Pts',(131.217213496199,-31.836249746466,19.75858402694));
#25220=CARTESIAN_POINT('Ctrl Pts',(131.238454127222,-31.8445038940108,19.7572120807001));
#25221=CARTESIAN_POINT('Ctrl Pts',(131.316530189969,-31.8757541122032,19.7521095308907));
#25222=CARTESIAN_POINT('Ctrl Pts',(131.372819044646,-31.9000756410706,19.7483136772788));
#25223=CARTESIAN_POINT('Ctrl Pts',(131.628583592661,-32.0189197204648,19.7306183394088));
#25224=CARTESIAN_POINT('Ctrl Pts',(131.81918642865,-32.131257330255,19.7161940995058));
#25225=CARTESIAN_POINT('Ctrl Pts',(132.087586577362,-32.327021100415,19.6949713080096));
#25226=CARTESIAN_POINT('Ctrl Pts',(132.17436802999,-32.3971244801238,19.6879360963486));
#25227=CARTESIAN_POINT('Ctrl Pts',(132.314898987542,-32.5225901164289,19.6762947048432));
#25228=CARTESIAN_POINT('Ctrl Pts',(132.370499635818,-32.5757372370219,19.6716149100946));
#25229=CARTESIAN_POINT('Ctrl Pts',(132.448381408971,-32.6554263228917,19.6649479047418));
#25230=CARTESIAN_POINT('Ctrl Pts',(132.472136764199,-32.6804877231172,19.662898119216));
#25231=CARTESIAN_POINT('Ctrl Pts',(132.513504884782,-32.725487837064,19.659298127611));
#25232=CARTESIAN_POINT('Ctrl Pts',(132.531273345969,-32.7452787992734,19.6577414766571));
#25233=CARTESIAN_POINT('Ctrl Pts',(132.568276700126,-32.7874828822709,19.6544764942763));
#25234=CARTESIAN_POINT('Ctrl Pts',(132.58745537382,-32.8099424726989,19.6527705306142));
#25235=CARTESIAN_POINT('Ctrl Pts',(132.638367560109,-32.8711667396767,19.648201926184));
#25236=CARTESIAN_POINT('Ctrl Pts',(132.66953992508,-32.9103896575483,19.6453615107732));
#25237=CARTESIAN_POINT('Ctrl Pts',(132.857026551126,-33.1573429613659,19.6279691685409));
#25238=CARTESIAN_POINT('Ctrl Pts',(132.989880155607,-33.3817870484092,19.6143483000809));
#25239=CARTESIAN_POINT('Ctrl Pts',(133.141855624863,-33.7225250636265,19.5945156606457));
#25240=CARTESIAN_POINT('Ctrl Pts',(133.182727929545,-33.828061850002,19.5884643653526));
#25241=CARTESIAN_POINT('Ctrl Pts',(133.238412522682,-33.9964002044334,19.5786864551119));
#25242=CARTESIAN_POINT('Ctrl Pts',(133.256840896426,-34.0579200994591,19.5750872112681));
#25243=CARTESIAN_POINT('Ctrl Pts',(133.279358338388,-34.1416752618375,19.5701072568024));
#25244=CARTESIAN_POINT('Ctrl Pts',(133.284989508949,-34.1634856037982,19.568803220226));
#25245=CARTESIAN_POINT('Ctrl Pts',(133.294084892809,-34.2002222009744,19.5665921723164));
#25246=CARTESIAN_POINT('Ctrl Pts',(133.297666131027,-34.2151191869144,19.5656915539131));
#25247=CARTESIAN_POINT('Ctrl Pts',(133.304919839925,-34.2462189218737,19.5638021611607));
#25248=CARTESIAN_POINT('Ctrl Pts',(133.308574352005,-34.2624250588927,19.5628125136921));
#25249=CARTESIAN_POINT('Ctrl Pts',(133.318220657547,-34.3067169163491,19.56009516443));
#25250=CARTESIAN_POINT('Ctrl Pts',(133.323974765379,-34.3348523421205,19.5583552412008));
#25251=CARTESIAN_POINT('Ctrl Pts',(133.361079654356,-34.5288034717945,19.5462821732507));
#25252=CARTESIAN_POINT('Ctrl Pts',(133.380364637538,-34.6966727376086,19.5354488214455));
#25253=CARTESIAN_POINT('Ctrl Pts',(133.392591895672,-35.0040449210967,19.5156259006755));
#25254=CARTESIAN_POINT('Ctrl Pts',(133.389577918343,-35.143041951486,19.5066654864244));
#25255=CARTESIAN_POINT('Ctrl Pts',(133.366895798481,-35.4152632785626,19.4893684828256));
#25256=CARTESIAN_POINT('Ctrl Pts',(133.347807510332,-35.548290773347,19.4810359299813));
#25257=CARTESIAN_POINT('Ctrl Pts',(133.312559728758,-35.7204665599387,19.470442131707));
#25258=CARTESIAN_POINT('Ctrl Pts',(133.303499682309,-35.760929759087,19.4679658971067));
#25259=CARTESIAN_POINT('Ctrl Pts',(133.287135994972,-35.8281986772698,19.463870106073));
#25260=CARTESIAN_POINT('Ctrl Pts',(133.280241308915,-35.8550983114437,19.4622378884108));
#25261=CARTESIAN_POINT('Ctrl Pts',(133.265966828475,-35.9080748856431,19.4590335254165));
#25262=CARTESIAN_POINT('Ctrl Pts',(133.258603326212,-35.9341540276346,19.4574609998783));
#25263=CARTESIAN_POINT('Ctrl Pts',(133.239770931259,-35.997918256818,19.4536267231888));
#25264=CARTESIAN_POINT('Ctrl Pts',(133.227956235934,-36.0354975883954,19.4513761799896));
#25265=CARTESIAN_POINT('Ctrl Pts',(133.182620222873,-36.1713745490391,19.4432636047178));
#25266=CARTESIAN_POINT('Ctrl Pts',(133.145240293091,-36.2683280275595,19.4375247484902));
#25267=CARTESIAN_POINT('Ctrl Pts',(133.001654836658,-36.5951626352275,19.4181291648662));
#25268=CARTESIAN_POINT('Ctrl Pts',(132.874215616292,-36.8147592541918,19.4050653273042));
#25269=CARTESIAN_POINT('Ctrl Pts',(132.684973685579,-37.0701485437394,19.3878357314506));
#25270=CARTESIAN_POINT('Ctrl Pts',(132.64493808778,-37.1210611418539,19.384282300992));
#25271=CARTESIAN_POINT('Ctrl Pts',(132.575118169129,-37.2047974169777,19.3781773764767));
#25272=CARTESIAN_POINT('Ctrl Pts',(132.546103134713,-37.2382412021783,19.3756649896913));
#25273=CARTESIAN_POINT('Ctrl Pts',(132.503296749702,-37.2856717708358,19.3719771938113));
#25274=CARTESIAN_POINT('Ctrl Pts',(132.490024696034,-37.3001232649984,19.3708362956679));
#25275=CARTESIAN_POINT('Ctrl Pts',(132.466524232604,-37.325270363624,19.3688187753727));
#25276=CARTESIAN_POINT('Ctrl Pts',(132.456350086203,-37.3360154741698,19.3679460973316));
#25277=CARTESIAN_POINT('Ctrl Pts',(132.433566989721,-37.3597637180413,19.3659932756243));
#25278=CARTESIAN_POINT('Ctrl Pts',(132.420924136429,-37.3727324736671,19.3649106909307));
#25279=CARTESIAN_POINT('Ctrl Pts',(132.382829563148,-37.4111876060401,19.3616536556656));
#25280=CARTESIAN_POINT('Ctrl Pts',(132.357075676757,-37.4363695182129,19.3594582224381));
#25281=CARTESIAN_POINT('Ctrl Pts',(132.221050747283,-37.5651979253716,19.3479188110186));
#25282=CARTESIAN_POINT('Ctrl Pts',(132.104337796046,-37.6617779950932,19.338213299181));
#25283=CARTESIAN_POINT('Ctrl Pts',(131.873603281396,-37.8280250444343,19.3198917442089));
#25284=CARTESIAN_POINT('Ctrl Pts',(131.761140078117,-37.8993970237987,19.311300125933));
#25285=CARTESIAN_POINT('Ctrl Pts',(131.519302174393,-38.0335977579744,19.2937374923244));
#25286=CARTESIAN_POINT('Ctrl Pts',(131.389530159568,-38.0951912403951,19.2848084469085));
#25287=CARTESIAN_POINT('Ctrl Pts',(131.217036963647,-38.1640175037994,19.2736058749596));
#25288=CARTESIAN_POINT('Ctrl Pts',(131.177553856138,-38.1789232284152,19.2710841962039));
#25289=CARTESIAN_POINT('Ctrl Pts',(131.11150664511,-38.2024579999321,19.2669344698561));
#25290=CARTESIAN_POINT('Ctrl Pts',(131.085096661619,-38.2115026962444,19.2652930449604));
#25291=CARTESIAN_POINT('Ctrl Pts',(131.032940975786,-38.2286477430164,19.2620855692815));
#25292=CARTESIAN_POINT('Ctrl Pts',(131.00720434663,-38.2367688786307,19.2605189453443));
#25293=CARTESIAN_POINT('Ctrl Pts',(130.950131819949,-38.2540313280403,19.2570790482898));
#25294=CARTESIAN_POINT('Ctrl Pts',(130.918755139911,-38.2630291841523,19.255210457974));
#25295=CARTESIAN_POINT('Ctrl Pts',(130.808842249527,-38.2928376302635,19.2487384844376));
#25296=CARTESIAN_POINT('Ctrl Pts',(130.729689180986,-38.3112777789999,19.2442088981335));
#25297=CARTESIAN_POINT('Ctrl Pts',(130.375391617486,-38.3804944914267,19.2243845332523));
#25298=CARTESIAN_POINT('Ctrl Pts',(130.095274566259,-38.3999375058523,19.2100008401026));
#25299=CARTESIAN_POINT('Ctrl Pts',(129.749160724202,-38.3811181684098,19.1912382798433));
#25300=CARTESIAN_POINT('Ctrl Pts',(129.68248675719,-38.3755095696038,19.1875726372736));
#25301=CARTESIAN_POINT('Ctrl Pts',(129.57101034035,-38.3628002734263,19.1812957669168));
#25302=CARTESIAN_POINT('Ctrl Pts',(129.526104361182,-38.3567663490817,19.1787265817193));
#25303=CARTESIAN_POINT('Ctrl Pts',(129.461771722245,-38.346805534286,19.1749703479391));
#25304=CARTESIAN_POINT('Ctrl Pts',(129.442235769276,-38.3436052376457,19.1738196095493));
#25305=CARTESIAN_POINT('Ctrl Pts',(129.408000973724,-38.3376886648702,19.1717835957511));
#25306=CARTESIAN_POINT('Ctrl Pts',(129.393290319951,-38.3350460001238,19.1709023209343));
#25307=CARTESIAN_POINT('Ctrl Pts',(129.360859320256,-38.3289983217153,19.1689449474997));
#25308=CARTESIAN_POINT('Ctrl Pts',(129.343148608262,-38.3255491052591,19.1678665778649));
#25309=CARTESIAN_POINT('Ctrl Pts',(129.291571789138,-38.3150762837749,19.1647002700099));
#25310=CARTESIAN_POINT('Ctrl Pts',(129.257785559828,-38.3076757433622,19.1625934596495));
#25311=CARTESIAN_POINT('Ctrl Pts',(129.040876746305,-38.2566734787021,19.1488818486681));
#25312=CARTESIAN_POINT('Ctrl Pts',(128.861554201773,-38.198401280825,19.1367078875408));
#25313=CARTESIAN_POINT('Ctrl Pts',(128.543155738256,-38.0647495209478,19.1144548503293));
#25314=CARTESIAN_POINT('Ctrl Pts',(128.402693473605,-37.9939445685754,19.1043858766844));
#25315=CARTESIAN_POINT('Ctrl Pts',(128.185598444882,-37.8648669016545,19.0886317187811));
#25316=CARTESIAN_POINT('Ctrl Pts',(128.105648162496,-37.8126409525438,19.0827810643623));
#25317=CARTESIAN_POINT('Ctrl Pts',(127.99768399278,-37.7354204714346,19.0748136808338));
#25318=CARTESIAN_POINT('Ctrl Pts',(127.967724036539,-37.7132359136485,19.0725949619642));
#25319=CARTESIAN_POINT('Ctrl Pts',(127.916708654769,-37.6741411594073,19.0688019835447));
#25320=CARTESIAN_POINT('Ctrl Pts',(127.895478596384,-37.6574656148347,19.0672189120923));
#25321=CARTESIAN_POINT('Ctrl Pts',(127.852329832161,-37.6227322081549,19.0639908557788));
#25322=CARTESIAN_POINT('Ctrl Pts',(127.830434271734,-37.6046489221274,19.0623470507372));
#25323=CARTESIAN_POINT('Ctrl Pts',(127.774749822837,-37.5574703614813,19.0581497415298));
#25324=CARTESIAN_POINT('Ctrl Pts',(127.741302544589,-37.5279792455196,19.0556123537418));
#25325=CARTESIAN_POINT('Ctrl Pts',(127.579355106281,-37.3794060904274,19.0432269759379));
#25326=CARTESIAN_POINT('Ctrl Pts',(127.459633297536,-37.2511421956431,19.0337712314917));
#25327=CARTESIAN_POINT('Ctrl Pts',(127.251118128711,-36.9898163153125,19.0159729204797));
#25328=CARTESIAN_POINT('Ctrl Pts',(127.160765286253,-36.8586187859908,19.0076254218208));
#25329=CARTESIAN_POINT('Ctrl Pts',(127.043624510451,-36.6599302610241,18.9951758156346));
#25330=CARTESIAN_POINT('Ctrl Pts',(127.009248391523,-36.597162568518,18.991266872403));
#25331=CARTESIAN_POINT('Ctrl Pts',(126.955399758409,-36.4909964981786,18.9846197088263));
#25332=CARTESIAN_POINT('Ctrl Pts',(126.934807506673,-36.4481904925946,18.9819302521196));
#25333=CARTESIAN_POINT('Ctrl Pts',(126.906767803111,-36.3866239408624,18.9780295146676));
#25334=CARTESIAN_POINT('Ctrl Pts',(126.898577132215,-36.3682059528073,18.9768585037977));
#25335=CARTESIAN_POINT('Ctrl Pts',(126.884587547551,-36.335977041105,18.9748004777273));
#25336=CARTESIAN_POINT('Ctrl Pts',(126.878715131583,-36.3221989878863,18.9739177819017));
#25337=CARTESIAN_POINT('Ctrl Pts',(126.86606734434,-36.2919704569789,18.971974445059));
#25338=CARTESIAN_POINT('Ctrl Pts',(126.859330139233,-36.275505525923,18.9709117730339));
#25339=CARTESIAN_POINT('Ctrl Pts',(126.84032528591,-36.2279963339575,18.9678350794381));
#25340=CARTESIAN_POINT('Ctrl Pts',(126.828386516974,-36.1968237252505,18.9658036888101));
#25341=CARTESIAN_POINT('Ctrl Pts',(126.745804919668,-35.971282022719,18.9510410006886));
#25342=CARTESIAN_POINT('Ctrl Pts',(126.692625240065,-35.7709965558779,18.9376147101442));
#25343=CARTESIAN_POINT('Ctrl Pts',(126.626335021558,-35.3803631093282,18.9121058551246));
#25344=CARTESIAN_POINT('Ctrl Pts',(126.610349291643,-35.1912478961659,18.9000493839968));
#25345=CARTESIAN_POINT('Ctrl Pts',(126.6102214509,-34.9461491383693,18.8850413354147));
#25346=CARTESIAN_POINT('Ctrl Pts',(126.611561328262,-34.8905356796344,18.8816747745842));
#25347=CARTESIAN_POINT('Ctrl Pts',(126.615917247258,-34.8011660559186,18.8763257076945));
#25348=CARTESIAN_POINT('Ctrl Pts',(126.618071693678,-34.7673799872712,18.8743174906237));
#25349=CARTESIAN_POINT('Ctrl Pts',(126.62281608338,-34.7071907034308,18.8707636366067));
#25350=CARTESIAN_POINT('Ctrl Pts',(126.62521050149,-34.6807753285021,18.8692121256732));
#25351=CARTESIAN_POINT('Ctrl Pts',(126.63096475465,-34.6246315717396,18.8659308985182));
#25352=CARTESIAN_POINT('Ctrl Pts',(126.634408622081,-34.5949139585812,18.8642039126751));
#25353=CARTESIAN_POINT('Ctrl Pts',(126.644909082024,-34.5137188526947,18.8595098343058));
#25354=CARTESIAN_POINT('Ctrl Pts',(126.652756627622,-34.4623508299043,18.8565672043406));
#25355=CARTESIAN_POINT('Ctrl Pts',(126.690906854619,-34.2460638648988,18.8442656239512));
#25356=CARTESIAN_POINT('Ctrl Pts',(126.732242904627,-34.0833276277052,18.8352430382239));
#25357=CARTESIAN_POINT('Ctrl Pts',(126.796849932018,-33.8902596431973,18.8244142701401));
#25358=CARTESIAN_POINT('Ctrl Pts',(126.808780054898,-33.856405717364,18.8225099732079));
#25359=CARTESIAN_POINT('Ctrl Pts',(126.821241893434,-33.8227566256554,18.8206072661261));
#25360=CARTESIAN_POINT('',(126.610251372999,-34.9977875375927,19.2361966383981));
#25361=CARTESIAN_POINT('Ctrl Pts',(126.821241915874,-33.8227565650612,19.1602708352289));
#25362=CARTESIAN_POINT('Ctrl Pts',(126.816736953399,-33.8349207321845,19.1610465414327));
#25363=CARTESIAN_POINT('Ctrl Pts',(126.812301909871,-33.8471104990182,19.1618260822225));
#25364=CARTESIAN_POINT('Ctrl Pts',(126.792726924733,-33.901889116889,19.1653381032647));
#25365=CARTESIAN_POINT('Ctrl Pts',(126.778370469,-33.9447508173432,19.1681101177204));
#25366=CARTESIAN_POINT('Ctrl Pts',(126.744968324843,-34.0515173590052,19.1750527022559));
#25367=CARTESIAN_POINT('Ctrl Pts',(126.726943361646,-34.1157207046637,19.1792602750059));
#25368=CARTESIAN_POINT('Ctrl Pts',(126.644210410436,-34.4477444133355,19.2010559226414));
#25369=CARTESIAN_POINT('Ctrl Pts',(126.610430890917,-34.7222374851469,19.2190847940162));
#25370=CARTESIAN_POINT('Ctrl Pts',(126.610250724596,-34.9977836064225,19.2361975235207));
#25371=CARTESIAN_POINT('Ctrl Pts',(126.610250722074,-34.9977874673202,19.2361977633008));
#25372=CARTESIAN_POINT('Ctrl Pts',(126.610215475891,-35.0517869964763,19.2395513902642));
#25373=CARTESIAN_POINT('Ctrl Pts',(126.611470566682,-35.1057822568918,19.2428715249805));
#25374=CARTESIAN_POINT('Ctrl Pts',(126.615959723836,-35.2009458075462,19.2486631010251));
#25375=CARTESIAN_POINT('Ctrl Pts',(126.618656669346,-35.2421266443502,19.2511495142746));
#25376=CARTESIAN_POINT('Ctrl Pts',(126.624315591746,-35.3096122172126,19.2551925444575));
#25377=CARTESIAN_POINT('Ctrl Pts',(126.626834810277,-35.3359488228297,19.2567624477098));
#25378=CARTESIAN_POINT('Ctrl Pts',(126.63235118281,-35.3872720625358,19.259806964583));
#25379=CARTESIAN_POINT('Ctrl Pts',(126.635318754657,-35.4122600810101,19.2612823870852));
#25380=CARTESIAN_POINT('Ctrl Pts',(126.642207569199,-35.4652234956728,19.2643958356638));
#25381=CARTESIAN_POINT('Ctrl Pts',(126.646200829735,-35.4931876975554,19.2660315094045));
#25382=CARTESIAN_POINT('Ctrl Pts',(126.657283866026,-35.5644258418229,19.2701792150951));
#25383=CARTESIAN_POINT('Ctrl Pts',(126.664864716015,-35.607618769188,19.2726758952135));
#25384=CARTESIAN_POINT('Ctrl Pts',(126.703952801223,-35.8074716358138,19.2841596591186));
#25385=CARTESIAN_POINT('Ctrl Pts',(126.745674981425,-35.9619323369152,19.2928266039349));
#25386=CARTESIAN_POINT('Ctrl Pts',(126.868023081428,-36.3139368607722,19.3127242568782));
#25387=CARTESIAN_POINT('Ctrl Pts',(126.95667909956,-36.5079444781437,19.3237971593411));
#25388=CARTESIAN_POINT('Ctrl Pts',(127.099974271123,-36.7566333809814,19.3395269336545));
#25389=CARTESIAN_POINT('Ctrl Pts',(127.139114944674,-36.8196827234399,19.3436637006914));
#25390=CARTESIAN_POINT('Ctrl Pts',(127.193423675289,-36.9010771644574,19.3492720263093));
#25391=CARTESIAN_POINT('Ctrl Pts',(127.20676318801,-36.9206231010795,19.3506399324129));
#25392=CARTESIAN_POINT('Ctrl Pts',(127.22919845104,-36.9527686144097,19.352927674653));
#25393=CARTESIAN_POINT('Ctrl Pts',(127.238178441058,-36.9654485876958,19.3538400724683));
#25394=CARTESIAN_POINT('Ctrl Pts',(127.255549040383,-36.989622196841,19.3555996164857));
#25395=CARTESIAN_POINT('Ctrl Pts',(127.263925392552,-37.0011255038456,19.3564457149268));
#25396=CARTESIAN_POINT('Ctrl Pts',(127.287153991146,-37.0326070235525,19.3587847830008));
#25397=CARTESIAN_POINT('Ctrl Pts',(127.302153977148,-37.0524744913238,19.3602872315245));
#25398=CARTESIAN_POINT('Ctrl Pts',(127.366005101649,-37.1351359174747,19.3666433956339));
#25399=CARTESIAN_POINT('Ctrl Pts',(127.416837337539,-37.1963613758636,19.3716086362371));
#25400=CARTESIAN_POINT('Ctrl Pts',(127.604929047678,-37.4073411404047,19.3894983438435));
#25401=CARTESIAN_POINT('Ctrl Pts',(127.753436768156,-37.5464900332526,19.4027441967379));
#25402=CARTESIAN_POINT('Ctrl Pts',(127.998979629321,-37.7382629343204,19.4226268813693));
#25403=CARTESIAN_POINT('Ctrl Pts',(128.087609881186,-37.8008808645023,19.4294621294333));
#25404=CARTESIAN_POINT('Ctrl Pts',(128.242748668098,-37.8996840911201,19.4408189327648));
#25405=CARTESIAN_POINT('Ctrl Pts',(128.307740578387,-37.938087721698,19.4454093261073));
#25406=CARTESIAN_POINT('Ctrl Pts',(128.404055015417,-37.9907425050132,19.4519751671637));
#25407=CARTESIAN_POINT('Ctrl Pts',(128.434394333691,-38.0067357969035,19.4540105471248));
#25408=CARTESIAN_POINT('Ctrl Pts',(128.4886603915,-38.0342978672481,19.4575944719336));
#25409=CARTESIAN_POINT('Ctrl Pts',(128.512489906022,-38.046050679056,19.4591492635014));
#25410=CARTESIAN_POINT('Ctrl Pts',(128.563207636043,-38.0703277368329,19.4624194715049));
#25411=CARTESIAN_POINT('Ctrl Pts',(128.590127115723,-38.0827817372623,19.4641323985691));
#25412=CARTESIAN_POINT('Ctrl Pts',(128.663505249134,-38.1155670848793,19.4687425015449));
#25413=CARTESIAN_POINT('Ctrl Pts',(128.710263188707,-38.1352122435713,19.4716167221714));
#25414=CARTESIAN_POINT('Ctrl Pts',(128.994746451094,-38.24729468547,19.488759843582));
#25415=CARTESIAN_POINT('Ctrl Pts',(129.2418378593,-38.3137076845742,19.5021404355514));
#25416=CARTESIAN_POINT('Ctrl Pts',(129.608486885277,-38.3690525909381,19.5218420282797));
#25417=CARTESIAN_POINT('Ctrl Pts',(129.723721208312,-38.3804533564389,19.5280267362175));
#25418=CARTESIAN_POINT('Ctrl Pts',(129.904345972995,-38.3890256963134,19.5379927647802));
#25419=CARTESIAN_POINT('Ctrl Pts',(129.96945784759,-38.3902375944467,19.5416407478837));
#25420=CARTESIAN_POINT('Ctrl Pts',(130.057194919791,-38.3893430343751,19.546677926323));
#25421=CARTESIAN_POINT('Ctrl Pts',(130.079826484096,-38.3888855301423,19.5479881717945));
#25422=CARTESIAN_POINT('Ctrl Pts',(130.117785664961,-38.3877377353283,19.5502066176384));
#25423=CARTESIAN_POINT('Ctrl Pts',(130.133116700031,-38.3871699638146,19.5511083250721));
#25424=CARTESIAN_POINT('Ctrl Pts',(130.165000628942,-38.3857723676685,19.5529963594252));
#25425=CARTESIAN_POINT('Ctrl Pts',(130.181551997265,-38.384925195643,19.5539835157157));
#25426=CARTESIAN_POINT('Ctrl Pts',(130.226577344332,-38.3822894214789,19.5566869006675));
#25427=CARTESIAN_POINT('Ctrl Pts',(130.255035401087,-38.3802626896993,19.5584151511606));
#25428=CARTESIAN_POINT('Ctrl Pts',(130.447526910326,-38.3641092582399,19.5702227641813));
#25429=CARTESIAN_POINT('Ctrl Pts',(130.610355108811,-38.3384080562368,19.580779689856));
#25430=CARTESIAN_POINT('Ctrl Pts',(130.901331910001,-38.2704759623411,19.6000305194481));
#25431=CARTESIAN_POINT('Ctrl Pts',(131.03008708596,-38.2322338275067,19.6086933463872));
#25432=CARTESIAN_POINT('Ctrl Pts',(131.24561578217,-38.1540269935091,19.6232464342937));
#25433=CARTESIAN_POINT('Ctrl Pts',(131.33359304085,-38.1178481068058,19.6292040888516));
#25434=CARTESIAN_POINT('Ctrl Pts',(131.482487280298,-38.0491607839702,19.6392901065023));
#25435=CARTESIAN_POINT('Ctrl Pts',(131.544145142191,-38.0184046826063,19.6434682179105));
#25436=CARTESIAN_POINT('Ctrl Pts',(131.634037660264,-37.9700885165434,19.6495637788521));
#25437=CARTESIAN_POINT('Ctrl Pts',(131.663017663586,-37.953959586572,19.6515296541311));
#25438=CARTESIAN_POINT('Ctrl Pts',(131.714477138844,-37.9243222509504,19.6550229906314));
#25439=CARTESIAN_POINT('Ctrl Pts',(131.737045050106,-37.9109735550463,19.6565559228395));
#25440=CARTESIAN_POINT('Ctrl Pts',(131.785329582839,-37.8816522399491,19.6598386467291));
#25441=CARTESIAN_POINT('Ctrl Pts',(131.810991827585,-37.8655941857449,19.6615852008343));
#25442=CARTESIAN_POINT('Ctrl Pts',(131.880374477991,-37.820873889295,19.6663149917191));
#25443=CARTESIAN_POINT('Ctrl Pts',(131.923653335046,-37.7915400644277,19.6692736329023));
#25444=CARTESIAN_POINT('Ctrl Pts',(132.19678451895,-37.5970456909897,19.6880408864379));
#25445=CARTESIAN_POINT('Ctrl Pts',(132.405854894409,-37.4046571971606,19.7027322568091));
#25446=CARTESIAN_POINT('Ctrl Pts',(132.678034171645,-37.0827219615734,19.7252541804833));
#25447=CARTESIAN_POINT('Ctrl Pts',(132.760899595045,-36.9715535676053,19.732759928562));
#25448=CARTESIAN_POINT('Ctrl Pts',(132.851975043394,-36.8323262813569,19.7422393238943));
#25449=CARTESIAN_POINT('Ctrl Pts',(132.866937901877,-36.8088250910627,19.7438420925372));
#25450=CARTESIAN_POINT('Ctrl Pts',(132.890261159672,-36.7711762818887,19.7464183398467));
#25451=CARTESIAN_POINT('Ctrl Pts',(132.898811596143,-36.7571472044543,19.7473801985655));
#25452=CARTESIAN_POINT('Ctrl Pts',(132.915095311493,-36.7299874554653,19.7492470089152));
#25453=CARTESIAN_POINT('Ctrl Pts',(132.922842582926,-36.7168658870126,19.7501510729468));
#25454=CARTESIAN_POINT('Ctrl Pts',(132.942010626481,-36.6838951754522,19.7524273234342));
#25455=CARTESIAN_POINT('Ctrl Pts',(132.953319110528,-36.663981867943,19.7538062173939));
#25456=CARTESIAN_POINT('Ctrl Pts',(132.994555940667,-36.5896225385892,19.7589660681125));
#25457=CARTESIAN_POINT('Ctrl Pts',(133.023185928337,-36.5344741632048,19.7628140964044));
#25458=CARTESIAN_POINT('Ctrl Pts',(133.146196207625,-36.2807052601986,19.7805163880707));
#25459=CARTESIAN_POINT('Ctrl Pts',(133.222627618009,-36.0739774251647,19.7948847781485));
#25460=CARTESIAN_POINT('Ctrl Pts',(133.306791367939,-35.7536137909025,19.8160443970512));
#25461=CARTESIAN_POINT('Ctrl Pts',(133.329761767628,-35.6445873435912,19.8230704295038));
#25462=CARTESIAN_POINT('Ctrl Pts',(133.359441774787,-35.4587570945061,19.8346988025996));
#25463=CARTESIAN_POINT('Ctrl Pts',(133.368976469921,-35.3824997584737,19.8393745347971));
#25464=CARTESIAN_POINT('Ctrl Pts',(133.379027746316,-35.2716026918333,19.846036959189));
#25465=CARTESIAN_POINT('Ctrl Pts',(133.381618337571,-35.2371794337575,19.8480861046058));
#25466=CARTESIAN_POINT('Ctrl Pts',(133.385273222976,-35.1761747302857,19.8516853912278));
#25467=CARTESIAN_POINT('Ctrl Pts',(133.386551252857,-35.1496094964039,19.8532419683326));
#25468=CARTESIAN_POINT('Ctrl Pts',(133.38858862795,-35.0935129065476,19.8565072071534));
#25469=CARTESIAN_POINT('Ctrl Pts',(133.389274857872,-35.0639810186423,19.8582134956124));
#25470=CARTESIAN_POINT('Ctrl Pts',(133.390084291149,-34.9843243198225,19.862783990647));
#25471=CARTESIAN_POINT('Ctrl Pts',(133.389481931877,-34.934198598235,19.8656259392149));
#25472=CARTESIAN_POINT('Ctrl Pts',(133.378887229694,-34.6245070176078,19.8830073997862));
#25473=CARTESIAN_POINT('Ctrl Pts',(133.340200084402,-34.3667953565156,19.8966177603642));
#25474=CARTESIAN_POINT('Ctrl Pts',(133.242930759682,-34.0067102163326,19.9164445520153));
#25475=CARTESIAN_POINT('Ctrl Pts',(133.207947955851,-33.8989588864861,19.9225016021018));
#25476=CARTESIAN_POINT('Ctrl Pts',(133.144767409337,-33.7331254185884,19.9322876449867));
#25477=CARTESIAN_POINT('Ctrl Pts',(133.120191439165,-33.6737505543854,19.9358890130272));
#25478=CARTESIAN_POINT('Ctrl Pts',(133.0847400329,-33.5945493176286,19.940871467982));
#25479=CARTESIAN_POINT('Ctrl Pts',(133.075330590271,-33.5740777044597,19.9421757830238));
#25480=CARTESIAN_POINT('Ctrl Pts',(133.059180465775,-33.5398442833371,19.944387167526));
#25481=CARTESIAN_POINT('Ctrl Pts',(133.052549081894,-33.526031229869,19.9452878396822));
#25482=CARTESIAN_POINT('Ctrl Pts',(133.038533552067,-33.4973374092028,19.9471771878438));
#25483=CARTESIAN_POINT('Ctrl Pts',(133.031133375043,-33.4824653394593,19.9481667350843));
#25484=CARTESIAN_POINT('Ctrl Pts',(133.010645971728,-33.4420397476596,19.9508835030708));
#25485=CARTESIAN_POINT('Ctrl Pts',(132.997343219713,-33.4165977075638,19.9526229367354));
#25486=CARTESIAN_POINT('Ctrl Pts',(132.903711935006,-33.2429329749408,19.9646854283372));
#25487=CARTESIAN_POINT('Ctrl Pts',(132.812752087564,-33.1007256279803,19.975507785595));
#25488=CARTESIAN_POINT('Ctrl Pts',(132.628351199254,-32.8549073312108,19.9953099050514));
#25489=CARTESIAN_POINT('Ctrl Pts',(132.538360600551,-32.7491376420928,20.0042604378855));
#25490=CARTESIAN_POINT('Ctrl Pts',(132.348833986512,-32.552249048837,20.0215666835943));
#25491=CARTESIAN_POINT('Ctrl Pts',(132.249834291612,-32.4609532288098,20.0299172091076));
#25492=CARTESIAN_POINT('Ctrl Pts',(132.113543338317,-32.3495169244659,20.0405294674718));
#25493=CARTESIAN_POINT('Ctrl Pts',(132.080947640085,-32.32384919615,20.0430071540465));
#25494=CARTESIAN_POINT('Ctrl Pts',(132.025756807603,-32.2820070427779,20.047104668851));
#25495=CARTESIAN_POINT('Ctrl Pts',(132.003419919627,-32.2655009502264,20.0487371809818));
#25496=CARTESIAN_POINT('Ctrl Pts',(131.958896197835,-32.233438088688,20.0519416361506));
#25497=CARTESIAN_POINT('Ctrl Pts',(131.936720725371,-32.2178691588593,20.0535139656573));
#25498=CARTESIAN_POINT('Ctrl Pts',(131.881871312146,-32.1803341880507,20.0573468988262));
#25499=CARTESIAN_POINT('Ctrl Pts',(131.848996377523,-32.1586680052232,20.059596313516));
#25500=CARTESIAN_POINT('Ctrl Pts',(131.728203232173,-32.0820439890653,20.0676980424927));
#25501=CARTESIAN_POINT('Ctrl Pts',(131.638149869025,-32.0305520112295,20.0734276424108));
#25502=CARTESIAN_POINT('Ctrl Pts',(131.320431579276,-31.8677429578912,20.0928257013155));
#25503=CARTESIAN_POINT('Ctrl Pts',(131.082767847086,-31.7778611938597,20.1058991359685));
#25504=CARTESIAN_POINT('Ctrl Pts',(130.774551535498,-31.6992923746749,20.1231399609527));
#25505=CARTESIAN_POINT('Ctrl Pts',(130.711340740496,-31.685095110012,20.12669429097));
#25506=CARTESIAN_POINT('Ctrl Pts',(130.604299290924,-31.6642559542592,20.132800595864));
#25507=CARTESIAN_POINT('Ctrl Pts',(130.560673648247,-31.6566467957303,20.1353134399064));
#25508=CARTESIAN_POINT('Ctrl Pts',(130.497520420058,-31.6469023953297,20.1390017846809));
#25509=CARTESIAN_POINT('Ctrl Pts',(130.478102053031,-31.6440785912536,20.1401427597984));
#25510=CARTESIAN_POINT('Ctrl Pts',(130.443998655354,-31.6394212933619,20.1421603478744));
#25511=CARTESIAN_POINT('Ctrl Pts',(130.429324437796,-31.637515120602,20.1430330152535));
#25512=CARTESIAN_POINT('Ctrl Pts',(130.396663856719,-31.633489816429,20.1449857148189));
#25513=CARTESIAN_POINT('Ctrl Pts',(130.37867291998,-31.6314187231879,20.1460681865974));
#25514=CARTESIAN_POINT('Ctrl Pts',(130.324860217061,-31.6256604072789,20.1493246429877));
#25515=CARTESIAN_POINT('Ctrl Pts',(130.288996457512,-31.622399864992,20.1515196012223));
#25516=CARTESIAN_POINT('Ctrl Pts',(130.102285991814,-31.608420468476,20.163051833763));
#25517=CARTESIAN_POINT('Ctrl Pts',(129.95090766196,-31.6072346191829,20.1727501719458));
#25518=CARTESIAN_POINT('Ctrl Pts',(129.618366999672,-31.6268922275347,20.1942113124854));
#25519=CARTESIAN_POINT('Ctrl Pts',(129.437908711403,-31.6522301535943,20.2059498770714));
#25520=CARTESIAN_POINT('Ctrl Pts',(129.191875936219,-31.7072407972895,20.2217316454497));
#25521=CARTESIAN_POINT('Ctrl Pts',(129.123893920941,-31.7246730224662,20.2260710565437));
#25522=CARTESIAN_POINT('Ctrl Pts',(129.00347524158,-31.759569315421,20.233713825701));
#25523=CARTESIAN_POINT('Ctrl Pts',(128.95083325386,-31.7762285612515,20.2370397591887));
#25524=CARTESIAN_POINT('Ctrl Pts',(128.869706038507,-31.8041002413739,20.242143843824));
#25525=CARTESIAN_POINT('Ctrl Pts',(128.840927851766,-31.8144244549056,20.2439501682841));
#25526=CARTESIAN_POINT('Ctrl Pts',(128.787528839335,-31.8344008765015,20.2472949916082));
#25527=CARTESIAN_POINT('Ctrl Pts',(128.762873868321,-31.8439545125429,20.2488365679187));
#25528=CARTESIAN_POINT('Ctrl Pts',(128.70782595241,-31.8660294172508,20.2522734077765));
#25529=CARTESIAN_POINT('Ctrl Pts',(128.677498050859,-31.8787063441986,20.2541633595127));
#25530=CARTESIAN_POINT('Ctrl Pts',(128.585707950495,-31.9186522942257,20.2598765308522));
#25531=CARTESIAN_POINT('Ctrl Pts',(128.524866718545,-31.9473112970534,20.2636534655531));
#25532=CARTESIAN_POINT('Ctrl Pts',(128.196759698843,-32.1139666567642,20.284048415187));
#25533=CARTESIAN_POINT('Ctrl Pts',(127.947944877892,-32.2852396274746,20.2994742431764));
#25534=CARTESIAN_POINT('Ctrl Pts',(127.674358370537,-32.5329245619873,20.3194330101063));
#25535=CARTESIAN_POINT('Ctrl Pts',(127.625123851497,-32.5802825491507,20.3231721618661));
#25536=CARTESIAN_POINT('Ctrl Pts',(127.545198565302,-32.6619519237733,20.3295612709896));
#25537=CARTESIAN_POINT('Ctrl Pts',(127.513714554314,-32.6954603175193,20.3321672065368));
#25538=CARTESIAN_POINT('Ctrl Pts',(127.469589160205,-32.7443798235453,20.3359676562647));
#25539=CARTESIAN_POINT('Ctrl Pts',(127.456385795957,-32.7592795493614,20.3371246720448));
#25540=CARTESIAN_POINT('Ctrl Pts',(127.433494644613,-32.7855747906894,20.3391674752441));
#25541=CARTESIAN_POINT('Ctrl Pts',(127.423749829932,-32.7969194756355,20.340049163677));
#25542=CARTESIAN_POINT('Ctrl Pts',(127.402465624827,-32.8220323876268,20.3420020647311));
#25543=CARTESIAN_POINT('Ctrl Pts',(127.390960555121,-32.8358278963901,20.3430754724506));
#25544=CARTESIAN_POINT('Ctrl Pts',(127.357195558682,-32.8769754180763,20.3462771949156));
#25545=CARTESIAN_POINT('Ctrl Pts',(127.33525286723,-32.9045832876639,20.3484254983314));
#25546=CARTESIAN_POINT('Ctrl Pts',(127.202225284048,-33.0774251784764,20.3618501159945));
#25547=CARTESIAN_POINT('Ctrl Pts',(127.102619442563,-33.2310981983309,20.3736613701719));
#25548=CARTESIAN_POINT('Ctrl Pts',(126.941073417759,-33.5309001692829,20.3956112185553));
#25549=CARTESIAN_POINT('Ctrl Pts',(126.876029076999,-33.6748218847371,20.4057322719259));
#25550=CARTESIAN_POINT('Ctrl Pts',(126.821241916136,-33.8227565643555,20.4155868599104));
#25551=CARTESIAN_POINT('Origin',(130.,-35.,23.));
#25552=CARTESIAN_POINT('',(126.821241920569,-33.8227565523843,21.6644320182169));
#25553=CARTESIAN_POINT('',(126.821241906568,-33.8227565901911,21.3230638867798));
#25554=CARTESIAN_POINT('',(126.821241915871,-33.8227565650715,23.));
#25555=CARTESIAN_POINT('',(126.610249333224,-35.0010395456522,20.1438703980445));
#25556=CARTESIAN_POINT('Ctrl Pts',(126.821241906568,-33.8227565901911,21.3230638867798));
#25557=CARTESIAN_POINT('Ctrl Pts',(126.859773755242,-33.7187140236256,21.3161349444083));
#25558=CARTESIAN_POINT('Ctrl Pts',(126.903393986687,-33.6166164168015,21.3090328813153));
#25559=CARTESIAN_POINT('Ctrl Pts',(127.06846590041,-33.277377232492,21.2847520991139));
#25560=CARTESIAN_POINT('Ctrl Pts',(127.212817793153,-33.0524426550774,21.2675617727641));
#25561=CARTESIAN_POINT('Ctrl Pts',(127.416488571569,-32.8048198627095,21.2480209965305));
#25562=CARTESIAN_POINT('Ctrl Pts',(127.451946182574,-32.763759989001,21.2447532248313));
#25563=CARTESIAN_POINT('Ctrl Pts',(127.508984933493,-32.7008282369973,21.2396985833579));
#25564=CARTESIAN_POINT('Ctrl Pts',(127.529902661678,-32.6783699499337,21.237885059339));
#25565=CARTESIAN_POINT('Ctrl Pts',(127.569397916283,-32.6371040792032,21.2345334744583));
#25566=CARTESIAN_POINT('Ctrl Pts',(127.587895871424,-32.6182239078389,21.2329922324592));
#25567=CARTESIAN_POINT('Ctrl Pts',(127.629779312757,-32.576463503472,21.2295643934529));
#25568=CARTESIAN_POINT('Ctrl Pts',(127.653279184206,-32.5537014131698,21.2276829775776));
#25569=CARTESIAN_POINT('Ctrl Pts',(127.725452292415,-32.4857914491748,21.2220260037073));
#25570=CARTESIAN_POINT('Ctrl Pts',(127.775126953947,-32.4417285833791,21.2182953501243));
#25571=CARTESIAN_POINT('Ctrl Pts',(127.895317455162,-32.3412666949094,21.2096092682179));
#25572=CARTESIAN_POINT('Ctrl Pts',(127.966855911994,-32.2861691340578,21.2046998713434));
#25573=CARTESIAN_POINT('Ctrl Pts',(128.153666406531,-32.1538293958193,21.1923918187075));
#25574=CARTESIAN_POINT('Ctrl Pts',(128.271635314369,-32.0806865297782,21.1850855022926));
#25575=CARTESIAN_POINT('Ctrl Pts',(128.542146797576,-31.9351237791153,21.1687632961399));
#25576=CARTESIAN_POINT('Ctrl Pts',(128.696273499869,-31.8664577763994,21.159740764265));
#25577=CARTESIAN_POINT('Ctrl Pts',(128.881867984865,-31.7998421691392,21.148517695639));
#25578=CARTESIAN_POINT('Ctrl Pts',(128.909011560901,-31.790487037579,21.1468674532568));
#25579=CARTESIAN_POINT('Ctrl Pts',(128.952042324984,-31.7762652523802,21.1442326366521));
#25580=CARTESIAN_POINT('Ctrl Pts',(128.967852670224,-31.7711684968163,21.1432606068666));
#25581=CARTESIAN_POINT('Ctrl Pts',(128.998317355534,-31.7615942611086,21.1413789191015));
#25582=CARTESIAN_POINT('Ctrl Pts',(129.012965587288,-31.7570996186416,21.1404702201279));
#25583=CARTESIAN_POINT('Ctrl Pts',(129.049226690899,-31.746241744309,21.1382118162415));
#25584=CARTESIAN_POINT('Ctrl Pts',(129.070873310223,-31.7399944469147,21.1368558427123));
#25585=CARTESIAN_POINT('Ctrl Pts',(129.154482959024,-31.7167647389613,21.1315927905092));
#25586=CARTESIAN_POINT('Ctrl Pts',(129.216858517564,-31.701330392302,21.127612585129));
#25587=CARTESIAN_POINT('Ctrl Pts',(129.390256962549,-31.6636193953959,21.1164675636157));
#25588=CARTESIAN_POINT('Ctrl Pts',(129.502014204305,-31.645118503067,21.1091966671459));
#25589=CARTESIAN_POINT('Ctrl Pts',(129.872525306431,-31.6027048368204,21.085168803525));
#25590=CARTESIAN_POINT('Ctrl Pts',(130.133153666791,-31.6029165292737,21.06847297977));
#25591=CARTESIAN_POINT('Ctrl Pts',(130.44101147656,-31.638686877902,21.0496515724498));
#25592=CARTESIAN_POINT('Ctrl Pts',(130.490663489561,-31.6455750464352,21.0466407698371));
#25593=CARTESIAN_POINT('Ctrl Pts',(130.569306660171,-31.6582687938726,21.0419094301623));
#25594=CARTESIAN_POINT('Ctrl Pts',(130.598404659501,-31.6633565558373,21.0401670069435));
#25595=CARTESIAN_POINT('Ctrl Pts',(130.653568123068,-31.6737466964143,21.0368782908773));
#25596=CARTESIAN_POINT('Ctrl Pts',(130.679644788603,-31.6789767613357,21.0353298748655));
#25597=CARTESIAN_POINT('Ctrl Pts',(130.739419842849,-31.6916990958462,21.0317935427955));
#25598=CARTESIAN_POINT('Ctrl Pts',(130.773071029569,-31.69940037501,21.0298123358701));
#25599=CARTESIAN_POINT('Ctrl Pts',(130.881222139028,-31.7258962530373,21.0234712052757));
#25600=CARTESIAN_POINT('Ctrl Pts',(130.955204878489,-31.7467104886632,21.0191744895268));
#25601=CARTESIAN_POINT('Ctrl Pts',(131.134528011522,-31.8038067201689,21.0088040968927));
#25602=CARTESIAN_POINT('Ctrl Pts',(131.238910812551,-31.8428006836137,21.0028073761437));
#25603=CARTESIAN_POINT('Ctrl Pts',(131.543193959248,-31.9738907795177,20.9851390168922));
#25604=CARTESIAN_POINT('Ctrl Pts',(131.736232105777,-32.0803650125761,20.9737018556521));
#25605=CARTESIAN_POINT('Ctrl Pts',(131.96877421985,-32.2398936285405,20.9581398140606));
#25606=CARTESIAN_POINT('Ctrl Pts',(132.018989343203,-32.2764104219727,20.9546589659596));
#25607=CARTESIAN_POINT('Ctrl Pts',(132.086309201272,-32.3282509280813,20.9497831011088));
#25608=CARTESIAN_POINT('Ctrl Pts',(132.104305545333,-32.3424019684997,20.9484584067004));
#25609=CARTESIAN_POINT('Ctrl Pts',(132.134037985052,-32.3662727742873,20.9462315983099));
#25610=CARTESIAN_POINT('Ctrl Pts',(132.145854732596,-32.3758916409401,20.9453363219601));
#25611=CARTESIAN_POINT('Ctrl Pts',(132.170279451822,-32.3960487399837,20.9434635057661));
#25612=CARTESIAN_POINT('Ctrl Pts',(132.182876218778,-32.4065994423888,20.9424851545431));
#25613=CARTESIAN_POINT('Ctrl Pts',(132.216630748349,-32.4352914511176,20.9398309037964));
#25614=CARTESIAN_POINT('Ctrl Pts',(132.237641853639,-32.4536024188978,20.9381436735157));
#25615=CARTESIAN_POINT('Ctrl Pts',(132.361954231143,-32.5646660703355,20.9279617628552));
#25616=CARTESIAN_POINT('Ctrl Pts',(132.459695164844,-32.663427345246,20.9191248187912));
#25617=CARTESIAN_POINT('Ctrl Pts',(132.73710780747,-32.9804847354087,20.8920502522279));
#25618=CARTESIAN_POINT('Ctrl Pts',(132.895850796657,-33.2155391924482,20.8737600413138));
#25619=CARTESIAN_POINT('Ctrl Pts',(133.047270541718,-33.5143047745597,20.8533746700617));
#25620=CARTESIAN_POINT('Ctrl Pts',(133.069862239451,-33.5615653141194,20.850222740593));
#25621=CARTESIAN_POINT('Ctrl Pts',(133.103777922287,-33.6369573581211,20.8453061307776));
#25622=CARTESIAN_POINT('Ctrl Pts',(133.115834630705,-33.6647482343102,20.8435171145053));
#25623=CARTESIAN_POINT('Ctrl Pts',(133.137628115932,-33.7168857587398,20.8402030236323));
#25624=CARTESIAN_POINT('Ctrl Pts',(133.147457988454,-33.7411907936983,20.8386749405761));
#25625=CARTESIAN_POINT('Ctrl Pts',(133.169070401186,-33.7964653693545,20.8352365975405));
#25626=CARTESIAN_POINT('Ctrl Pts',(133.180682916066,-33.8274987790066,20.8333320435934));
#25627=CARTESIAN_POINT('Ctrl Pts',(133.214972881802,-33.9233963337106,20.8275217668704));
#25628=CARTESIAN_POINT('Ctrl Pts',(133.236135386097,-33.9887855175925,20.8236647656838));
#25629=CARTESIAN_POINT('Ctrl Pts',(133.281714492032,-34.145757323562,20.8146143503214));
#25630=CARTESIAN_POINT('Ctrl Pts',(133.304307540692,-34.2378098354776,20.8094728603572));
#25631=CARTESIAN_POINT('Ctrl Pts',(133.34959295557,-34.4626452836973,20.7971677094481));
#25632=CARTESIAN_POINT('Ctrl Pts',(133.368287519213,-34.5960659019881,20.7900769695353));
#25633=CARTESIAN_POINT('Ctrl Pts',(133.392115984737,-34.8945444133617,20.7741590735634));
#25634=CARTESIAN_POINT('Ctrl Pts',(133.393230285814,-35.0595655312461,20.7653209861682));
#25635=CARTESIAN_POINT('Ctrl Pts',(133.380455323631,-35.2524706642951,20.7543152395594));
#25636=CARTESIAN_POINT('Ctrl Pts',(133.378209849686,-35.2809229952767,20.7526744686298));
#25637=CARTESIAN_POINT('Ctrl Pts',(133.374092816968,-35.3258488454448,20.7500513369237));
#25638=CARTESIAN_POINT('Ctrl Pts',(133.372459156744,-35.3423434218908,20.7490813338481));
#25639=CARTESIAN_POINT('Ctrl Pts',(133.369080721447,-35.3740795281454,20.747200562248));
#25640=CARTESIAN_POINT('Ctrl Pts',(133.367353347112,-35.3893222344036,20.7462907117488));
#25641=CARTESIAN_POINT('Ctrl Pts',(133.362821873032,-35.427020157652,20.7440250845846));
#25642=CARTESIAN_POINT('Ctrl Pts',(133.359896273264,-35.4494598279762,20.742662950993));
#25643=CARTESIAN_POINT('Ctrl Pts',(133.347689641711,-35.5362946605122,20.7373437950091));
#25644=CARTESIAN_POINT('Ctrl Pts',(133.336780582456,-35.600443273135,20.7333117251082));
#25645=CARTESIAN_POINT('Ctrl Pts',(133.30138720749,-35.7775627861017,20.7219627776854));
#25646=CARTESIAN_POINT('Ctrl Pts',(133.272961033268,-35.889654426404,20.7145357285367));
#25647=CARTESIAN_POINT('Ctrl Pts',(133.163544255588,-36.2440162374779,20.6906368715027));
#25648=CARTESIAN_POINT('Ctrl Pts',(133.060888270915,-36.4787127307769,20.6742375603121));
#25649=CARTESIAN_POINT('Ctrl Pts',(132.907423420061,-36.7435199997241,20.6556429101796));
#25650=CARTESIAN_POINT('Ctrl Pts',(132.881033665064,-36.7867899621619,20.6525977792643));
#25651=CARTESIAN_POINT('Ctrl Pts',(132.837679534634,-36.8544161171508,20.6478257097789));
#25652=CARTESIAN_POINT('Ctrl Pts',(132.821349335328,-36.8791679777266,20.6460762313326));
#25653=CARTESIAN_POINT('Ctrl Pts',(132.789774194258,-36.9256871430759,20.6427817354166));
#25654=CARTESIAN_POINT('Ctrl Pts',(132.774594061156,-36.9474955411837,20.6412344855192));
#25655=CARTESIAN_POINT('Ctrl Pts',(132.739229954676,-36.9970481342958,20.6377112186631));
#25656=CARTESIAN_POINT('Ctrl Pts',(132.718877890896,-37.0246691414448,20.635741730824));
#25657=CARTESIAN_POINT('Ctrl Pts',(132.652379795883,-37.112106342507,20.6294842577165));
#25658=CARTESIAN_POINT('Ctrl Pts',(132.604650864281,-37.1706927015846,20.6252570643444));
#25659=CARTESIAN_POINT('Ctrl Pts',(132.483623205743,-37.3095060094869,20.6151012301935));
#25660=CARTESIAN_POINT('Ctrl Pts',(132.408348446616,-37.387899103388,20.6092450690748));
#25661=CARTESIAN_POINT('Ctrl Pts',(132.181212029347,-37.6027579474692,20.5925577769525));
#25662=CARTESIAN_POINT('Ctrl Pts',(132.020640756066,-37.7292923828891,20.5819272899538));
#25663=CARTESIAN_POINT('Ctrl Pts',(131.783848104023,-37.8834808987926,20.5664898418752));
#25664=CARTESIAN_POINT('Ctrl Pts',(131.716552258405,-37.9240421868466,20.5621233185625));
#25665=CARTESIAN_POINT('Ctrl Pts',(131.626240949896,-37.9742831916333,20.5562100665069));
#25666=CARTESIAN_POINT('Ctrl Pts',(131.60443729217,-37.9861013093735,20.554778459207));
#25667=CARTESIAN_POINT('Ctrl Pts',(131.569938356575,-38.0043136657504,20.5525039863005));
#25668=CARTESIAN_POINT('Ctrl Pts',(131.55732874817,-38.0108693428522,20.5516707183298));
#25669=CARTESIAN_POINT('Ctrl Pts',(131.530832264893,-38.0244337657655,20.5499149730549));
#25670=CARTESIAN_POINT('Ctrl Pts',(131.516937833453,-38.0314264966941,20.5489914849855));
#25671=CARTESIAN_POINT('Ctrl Pts',(131.481708786511,-38.0488535843119,20.5466438550995));
#25672=CARTESIAN_POINT('Ctrl Pts',(131.460311943731,-38.059159699008,20.5452123530944));
#25673=CARTESIAN_POINT('Ctrl Pts',(131.370888872964,-38.1010797669131,20.5392117878531));
#25674=CARTESIAN_POINT('Ctrl Pts',(131.301935019881,-38.1306541806046,20.5345422854971));
#25675=CARTESIAN_POINT('Ctrl Pts',(131.094226399504,-38.2116918228963,20.5204653533826));
#25676=CARTESIAN_POINT('Ctrl Pts',(130.953021865792,-38.2563848872775,20.5108880952779));
#25677=CARTESIAN_POINT('Ctrl Pts',(130.610081511397,-38.3407059093794,20.4881481229481));
#25678=CARTESIAN_POINT('Ctrl Pts',(130.40674676347,-38.3715121055298,20.4750991709274));
#25679=CARTESIAN_POINT('Ctrl Pts',(130.148966182982,-38.386889557602,20.4593751703967));
#25680=CARTESIAN_POINT('Ctrl Pts',(130.096012796522,-38.3888041866135,20.4561857195452));
#25681=CARTESIAN_POINT('Ctrl Pts',(130.012615779515,-38.3898630236812,20.4512243572008));
#25682=CARTESIAN_POINT('Ctrl Pts',(129.982193071018,-38.3898397426532,20.4494273683715));
#25683=CARTESIAN_POINT('Ctrl Pts',(129.925322634463,-38.3890305651922,20.4460912071455));
#25684=CARTESIAN_POINT('Ctrl Pts',(129.898876014868,-38.388344563187,20.4445490925656));
#25685=CARTESIAN_POINT('Ctrl Pts',(129.83938678588,-38.3861043241054,20.4411000398793));
#25686=CARTESIAN_POINT('Ctrl Pts',(129.806353198417,-38.3843758841064,20.4391985895675));
#25687=CARTESIAN_POINT('Ctrl Pts',(129.705107801927,-38.3775910757621,20.433409050608));
#25688=CARTESIAN_POINT('Ctrl Pts',(129.637017468586,-38.3709534906077,20.4295691577197));
#25689=CARTESIAN_POINT('Ctrl Pts',(129.475809481098,-38.350296836443,20.4205684371169));
#25690=CARTESIAN_POINT('Ctrl Pts',(129.382982726584,-38.3344498597171,20.4154587048134));
#25691=CARTESIAN_POINT('Ctrl Pts',(129.077947882023,-38.2691991019591,20.3987181821178));
#25692=CARTESIAN_POINT('Ctrl Pts',(128.869863147881,-38.2032210988882,20.3874080410901));
#25693=CARTESIAN_POINT('Ctrl Pts',(128.588471843518,-38.0831420843416,20.3707764216785));
#25694=CARTESIAN_POINT('Ctrl Pts',(128.50877501658,-38.0453936494679,20.3658989754533));
#25695=CARTESIAN_POINT('Ctrl Pts',(128.407858305335,-37.9926828868083,20.359392964211));
#25696=CARTESIAN_POINT('Ctrl Pts',(128.38520702745,-37.9805217006054,20.3579104618822));
#25697=CARTESIAN_POINT('Ctrl Pts',(128.348716749315,-37.9603924757447,20.3554824904944));
#25698=CARTESIAN_POINT('Ctrl Pts',(128.334791467079,-37.9525820062384,20.3545464262084));
#25699=CARTESIAN_POINT('Ctrl Pts',(128.307236798478,-37.9368701011722,20.3526741810172));
#25700=CARTESIAN_POINT('Ctrl Pts',(128.293606329227,-37.9289714682675,20.3517381721666));
#25701=CARTESIAN_POINT('Ctrl Pts',(128.258733684731,-37.9084373067436,20.3493189972118));
#25702=CARTESIAN_POINT('Ctrl Pts',(128.237574069281,-37.8956641222464,20.3478275881173));
#25703=CARTESIAN_POINT('Ctrl Pts',(128.144209710245,-37.8379015087755,20.3411481912208));
#25704=CARTESIAN_POINT('Ctrl Pts',(128.073578741764,-37.7904375032694,20.3358306400722));
#25705=CARTESIAN_POINT('Ctrl Pts',(127.85126862087,-37.6285798321187,20.3183957051997));
#25706=CARTESIAN_POINT('Ctrl Pts',(127.707392184788,-37.5040823930608,20.3060271150506));
#25707=CARTESIAN_POINT('Ctrl Pts',(127.457056991398,-37.2477101688592,20.2831229962828));
#25708=CARTESIAN_POINT('Ctrl Pts',(127.348543251883,-37.1186199206653,20.2725675785924));
#25709=CARTESIAN_POINT('Ctrl Pts',(127.224081370735,-36.9459330465488,20.2597014097012));
#25710=CARTESIAN_POINT('Ctrl Pts',(127.198809954639,-36.9093753609102,20.2570417276768));
#25711=CARTESIAN_POINT('Ctrl Pts',(127.158595581403,-36.8486834884419,20.2527279720168));
#25712=CARTESIAN_POINT('Ctrl Pts',(127.143224528853,-36.8248407303131,20.2510582692216));
#25713=CARTESIAN_POINT('Ctrl Pts',(127.113803744457,-36.7779217975867,20.2478198728546));
#25714=CARTESIAN_POINT('Ctrl Pts',(127.099727051058,-36.7548651308258,20.246250281829));
#25715=CARTESIAN_POINT('Ctrl Pts',(127.066833631517,-36.6995108419458,20.2425322135636));
#25716=CARTESIAN_POINT('Ctrl Pts',(127.048272330219,-36.6670650759384,20.2403929232357));
#25717=CARTESIAN_POINT('Ctrl Pts',(126.983872086,-36.550042217053,20.2328116610712));
#25718=CARTESIAN_POINT('Ctrl Pts',(126.941099300056,-36.4638262121703,20.2274748578003));
#25719=CARTESIAN_POINT('Ctrl Pts',(126.837415130847,-36.2303731777448,20.2135375041085));
#25720=CARTESIAN_POINT('Ctrl Pts',(126.783113675241,-36.0804660023441,20.2051145483497));
#25721=CARTESIAN_POINT('Ctrl Pts',(126.71186937848,-35.8299646754079,20.191305205481));
#25722=CARTESIAN_POINT('Ctrl Pts',(126.688561079136,-35.7314474332906,20.1859351981973));
#25723=CARTESIAN_POINT('Ctrl Pts',(126.651263933784,-35.5349233021026,20.1751127654718));
#25724=CARTESIAN_POINT('Ctrl Pts',(126.637091279735,-35.4370558995753,20.1696699745491));
#25725=CARTESIAN_POINT('Ctrl Pts',(126.624573230346,-35.3124074518496,20.1625185518193));
#25726=CARTESIAN_POINT('Ctrl Pts',(126.622238982669,-35.2860676689685,20.160995002182));
#25727=CARTESIAN_POINT('Ctrl Pts',(126.61897784093,-35.2436272081478,20.158516461183));
#25728=CARTESIAN_POINT('Ctrl Pts',(126.617857237862,-35.2275420176978,20.1575716104813));
#25729=CARTESIAN_POINT('Ctrl Pts',(126.615979816103,-35.1975036991971,20.1557959404069));
#25730=CARTESIAN_POINT('Ctrl Pts',(126.615194438922,-35.1835527391387,20.1549667072676));
#25731=CARTESIAN_POINT('Ctrl Pts',(126.613711948982,-35.1539593154366,20.1531986225364));
#25732=CARTESIAN_POINT('Ctrl Pts',(126.613036921538,-35.1383160148335,20.1522586297319));
#25733=CARTESIAN_POINT('Ctrl Pts',(126.611002640217,-35.0821388850985,20.1488650590904));
#25734=CARTESIAN_POINT('Ctrl Pts',(126.610262546074,-35.0415878496477,20.1463819526198));
#25735=CARTESIAN_POINT('Ctrl Pts',(126.610250158162,-35.0010354991548,20.1438715788674));
#25736=CARTESIAN_POINT('Ctrl Pts',(126.610250159373,-35.0010394571165,20.143871823883));
#25737=CARTESIAN_POINT('Ctrl Pts',(126.610149230195,-34.6719016210195,20.1234967188205));
#25738=CARTESIAN_POINT('Ctrl Pts',(126.657981717222,-34.3444712680937,20.1016491473991));
#25739=CARTESIAN_POINT('Ctrl Pts',(126.773063007837,-33.9595473749733,20.0765392240846));
#25740=CARTESIAN_POINT('Ctrl Pts',(126.796058758342,-33.8907553870495,20.072064610877));
#25741=CARTESIAN_POINT('Ctrl Pts',(126.82124191022,-33.822756580328,20.0676573852273));
#25742=CARTESIAN_POINT('Ctrl Pts',(126.821241916136,-33.8227565643555,20.4155868599104));
#25743=CARTESIAN_POINT('Ctrl Pts',(126.820287593857,-33.8253333972916,20.4157585142308));
#25744=CARTESIAN_POINT('Ctrl Pts',(126.819336383827,-33.8279114475735,20.4159300917818));
#25745=CARTESIAN_POINT('Ctrl Pts',(126.78505051154,-33.9211850399282,20.4221320307644));
#25746=CARTESIAN_POINT('Ctrl Pts',(126.755603743355,-34.0132692357797,20.4280574555847));
#25747=CARTESIAN_POINT('Ctrl Pts',(126.720262735379,-34.1426028844148,20.43610650087));
#25748=CARTESIAN_POINT('Ctrl Pts',(126.710994121633,-34.1788746506242,20.4383349228403));
#25749=CARTESIAN_POINT('Ctrl Pts',(126.696072440349,-34.2415819426616,20.4421392521894));
#25750=CARTESIAN_POINT('Ctrl Pts',(126.690131375848,-34.2679446585663,20.4437241091623));
#25751=CARTESIAN_POINT('Ctrl Pts',(126.67860493898,-34.3221035893835,20.4469513216356));
#25752=CARTESIAN_POINT('Ctrl Pts',(126.673051753885,-34.3499045196963,20.4485925544366));
#25753=CARTESIAN_POINT('Ctrl Pts',(126.659707166987,-34.4213674361841,20.4527739451933));
#25754=CARTESIAN_POINT('Ctrl Pts',(126.652422558014,-34.4651192841586,20.4552982355576));
#25755=CARTESIAN_POINT('Ctrl Pts',(126.622062488983,-34.6725089710146,20.4671127850266));
#25756=CARTESIAN_POINT('Ctrl Pts',(126.610113321141,-34.8375542996702,20.4760588099895));
#25757=CARTESIAN_POINT('Ctrl Pts',(126.610434020515,-35.2220294011891,20.4965625636002));
#25758=CARTESIAN_POINT('Ctrl Pts',(126.631878462955,-35.440678979504,20.5079616797009));
#25759=CARTESIAN_POINT('Ctrl Pts',(126.686426697232,-35.7173448321876,20.5235153390101));
#25760=CARTESIAN_POINT('Ctrl Pts',(126.700289207335,-35.7786265741539,20.5270362472441));
#25761=CARTESIAN_POINT('Ctrl Pts',(126.721539861997,-35.8617615159784,20.5319595795821));
#25762=CARTESIAN_POINT('Ctrl Pts',(126.727460774096,-35.8839800561133,20.5332898991135));
#25763=CARTESIAN_POINT('Ctrl Pts',(126.737685090256,-35.9208361511508,20.5355234339344));
#25764=CARTESIAN_POINT('Ctrl Pts',(126.741862229316,-35.9355084429598,20.5364197197017));
#25765=CARTESIAN_POINT('Ctrl Pts',(126.750734759437,-35.9658930418776,20.5382915112906));
#25766=CARTESIAN_POINT('Ctrl Pts',(126.755445330979,-35.9816001970923,20.5392677917796));
#25767=CARTESIAN_POINT('Ctrl Pts',(126.768423509854,-36.0237610047166,20.5419105051132));
#25768=CARTESIAN_POINT('Ctrl Pts',(126.776901727913,-36.0501479074717,20.5435881087229));
#25769=CARTESIAN_POINT('Ctrl Pts',(126.828423407328,-36.2039958022773,20.5534961823521));
#25770=CARTESIAN_POINT('Ctrl Pts',(126.878697446336,-36.3288971841403,20.5620484418298));
#25771=CARTESIAN_POINT('Ctrl Pts',(127.060272170925,-36.712427684662,20.5893018835114));
#25772=CARTESIAN_POINT('Ctrl Pts',(127.217403975416,-36.9574532626752,20.6080878925377));
#25773=CARTESIAN_POINT('Ctrl Pts',(127.436522120658,-37.218461883155,20.6288049802505));
#25774=CARTESIAN_POINT('Ctrl Pts',(127.470098427761,-37.25667685306,20.6318631997782));
#25775=CARTESIAN_POINT('Ctrl Pts',(127.52480459498,-37.316184532881,20.6366678748007));
#25776=CARTESIAN_POINT('Ctrl Pts',(127.545377853937,-37.33797632362,20.6384368539857));
#25777=CARTESIAN_POINT('Ctrl Pts',(127.584692667842,-37.3785286395582,20.6417479216268));
#25778=CARTESIAN_POINT('Ctrl Pts',(127.603370509505,-37.3973475221807,20.6432925386918));
#25779=CARTESIAN_POINT('Ctrl Pts',(127.646331585218,-37.4396290764838,20.6467826823124));
#25780=CARTESIAN_POINT('Ctrl Pts',(127.670748638937,-37.4629521415749,20.6487221399036));
#25781=CARTESIAN_POINT('Ctrl Pts',(127.748549328397,-37.5350750509929,20.6547694761412));
#25782=CARTESIAN_POINT('Ctrl Pts',(127.803150163531,-37.5825350826226,20.6588224105451));
#25783=CARTESIAN_POINT('Ctrl Pts',(127.938266990732,-37.6925923117058,20.6684504514533));
#25784=CARTESIAN_POINT('Ctrl Pts',(128.020170538602,-37.7533749370772,20.6739634071083));
#25785=CARTESIAN_POINT('Ctrl Pts',(128.144188316743,-37.8370120573627,20.6819655826703));
#25786=CARTESIAN_POINT('Ctrl Pts',(128.184241343463,-37.8628124305117,20.6845005365484));
#25787=CARTESIAN_POINT('Ctrl Pts',(128.402282279954,-37.9968473667998,20.6980904430487));
#25788=CARTESIAN_POINT('Ctrl Pts',(128.589400201139,-38.0893346173491,20.7089922971266));
#25789=CARTESIAN_POINT('Ctrl Pts',(128.827700399478,-38.180932354407,20.7232391805213));
#25790=CARTESIAN_POINT('Ctrl Pts',(128.87194446919,-38.1968902496851,20.7258999659437));
#25791=CARTESIAN_POINT('Ctrl Pts',(128.934236314361,-38.2179035177958,20.7296863015));
#25792=CARTESIAN_POINT('Ctrl Pts',(128.952017549844,-38.2237382079705,20.7307716347112));
#25793=CARTESIAN_POINT('Ctrl Pts',(128.984257072195,-38.2340222921873,20.7327491497458));
#25794=CARTESIAN_POINT('Ctrl Pts',(128.998698807387,-38.2385227801463,20.7336384855201));
#25795=CARTESIAN_POINT('Ctrl Pts',(129.02910307024,-38.2477748656496,20.7355189673773));
#25796=CARTESIAN_POINT('Ctrl Pts',(129.045071095319,-38.2525056783061,20.7365111641546));
#25797=CARTESIAN_POINT('Ctrl Pts',(129.088851164086,-38.2651261249449,20.7392427823008));
#25798=CARTESIAN_POINT('Ctrl Pts',(129.116729684759,-38.2727777563369,20.7409946300442));
#25799=CARTESIAN_POINT('Ctrl Pts',(129.323955843639,-38.3268132221219,20.7540907523586));
#25800=CARTESIAN_POINT('Ctrl Pts',(129.506725061284,-38.3587780848658,20.7660344910275));
#25801=CARTESIAN_POINT('Ctrl Pts',(129.924822853205,-38.3970285891289,20.7930980191956));
#25802=CARTESIAN_POINT('Ctrl Pts',(130.160096080795,-38.3940912060254,20.808111416691));
#25803=CARTESIAN_POINT('Ctrl Pts',(130.444922949057,-38.3608272616754,20.8255602516092));
#25804=CARTESIAN_POINT('Ctrl Pts',(130.49649707673,-38.3535961915296,20.8286933374334));
#25805=CARTESIAN_POINT('Ctrl Pts',(130.577715390762,-38.3402939434571,20.8335874604137));
#25806=CARTESIAN_POINT('Ctrl Pts',(130.607478426116,-38.3350095579873,20.8353724645112));
#25807=CARTESIAN_POINT('Ctrl Pts',(130.662924281831,-38.3243983165584,20.838682939486));
#25808=CARTESIAN_POINT('Ctrl Pts',(130.68862346733,-38.3191701595135,20.8402113598081));
#25809=CARTESIAN_POINT('Ctrl Pts',(130.746741669479,-38.3066427120293,20.8436553956946));
#25810=CARTESIAN_POINT('Ctrl Pts',(130.779119478534,-38.2991638480062,20.845565225006));
#25811=CARTESIAN_POINT('Ctrl Pts',(130.878617047122,-38.2746346837263,20.8514108523649));
#25812=CARTESIAN_POINT('Ctrl Pts',(130.9453302802,-38.2560024246874,20.8552970258375));
#25813=CARTESIAN_POINT('Ctrl Pts',(131.102856956312,-38.2067565479753,20.864432441114));
#25814=CARTESIAN_POINT('Ctrl Pts',(131.193035764187,-38.1743106875792,20.8696283227387));
#25815=CARTESIAN_POINT('Ctrl Pts',(131.405175393261,-38.0876641796424,20.8819172570561));
#25816=CARTESIAN_POINT('Ctrl Pts',(131.525545902882,-38.0299996908448,20.888942274422));
#25817=CARTESIAN_POINT('Ctrl Pts',(131.774703126616,-37.8920189123316,20.9040844365503));
#25818=CARTESIAN_POINT('Ctrl Pts',(131.902121670271,-37.8098521388453,20.9122038045981));
#25819=CARTESIAN_POINT('Ctrl Pts',(132.0525130592,-37.6979424448265,20.9227842417959));
#25820=CARTESIAN_POINT('Ctrl Pts',(132.081073188371,-37.6759741144796,20.9248416205529));
#25821=CARTESIAN_POINT('Ctrl Pts',(132.123456332016,-37.6422843108382,20.9279768837471));
#25822=CARTESIAN_POINT('Ctrl Pts',(132.137545233771,-37.6308997538443,20.9290330893307));
#25823=CARTESIAN_POINT('Ctrl Pts',(132.162976895045,-37.6100105352697,20.9309665950521));
#25824=CARTESIAN_POINT('Ctrl Pts',(132.174349628666,-37.6005437335457,20.9318413113802));
#25825=CARTESIAN_POINT('Ctrl Pts',(132.200655042083,-37.578353602582,20.9338879865361));
#25826=CARTESIAN_POINT('Ctrl Pts',(132.215539574857,-37.565574841197,20.9350637486538));
#25827=CARTESIAN_POINT('Ctrl Pts',(132.263636356245,-37.5235518172059,20.9389186129392));
#25828=CARTESIAN_POINT('Ctrl Pts',(132.296385770554,-37.4937873456795,20.9416309347357));
#25829=CARTESIAN_POINT('Ctrl Pts',(132.375570207479,-37.4189376058717,20.9483882534124));
#25830=CARTESIAN_POINT('Ctrl Pts',(132.421314034323,-37.3731477959729,20.9524679640954));
#25831=CARTESIAN_POINT('Ctrl Pts',(132.639045064265,-37.1423460921838,20.972660057934));
#25832=CARTESIAN_POINT('Ctrl Pts',(132.791314782899,-36.9397904969845,20.9891813928842));
#25833=CARTESIAN_POINT('Ctrl Pts',(132.972656275966,-36.6323598482052,21.0115501811179));
#25834=CARTESIAN_POINT('Ctrl Pts',(133.021477092835,-36.540118042203,21.0179694783276));
#25835=CARTESIAN_POINT('Ctrl Pts',(133.082792203004,-36.4100896863981,21.0266180496944));
#25836=CARTESIAN_POINT('Ctrl Pts',(133.098990987637,-36.3741236284215,21.0289699883953));
#25837=CARTESIAN_POINT('Ctrl Pts',(133.124285881217,-36.3152376850167,21.0327572776763));
#25838=CARTESIAN_POINT('Ctrl Pts',(133.133765804597,-36.2924876654957,21.0342053433743));
#25839=CARTESIAN_POINT('Ctrl Pts',(133.153224587626,-36.2443172414362,21.0372404632677));
#25840=CARTESIAN_POINT('Ctrl Pts',(133.163146112001,-36.2188754798109,21.0388255311379));
#25841=CARTESIAN_POINT('Ctrl Pts',(133.186503883485,-36.1567724118986,21.0426527227575));
#25842=CARTESIAN_POINT('Ctrl Pts',(133.199616413212,-36.1199930350217,21.044884154967));
#25843=CARTESIAN_POINT('Ctrl Pts',(133.247159301728,-35.9789838942373,21.0533150691245));
#25844=CARTESIAN_POINT('Ctrl Pts',(133.277156909894,-35.8733262245528,21.0593735941721));
#25845=CARTESIAN_POINT('Ctrl Pts',(133.348234777279,-35.5670892124865,21.0764258355136));
#25846=CARTESIAN_POINT('Ctrl Pts',(133.376353233746,-35.3640124893995,21.087105006235));
#25847=CARTESIAN_POINT('Ctrl Pts',(133.392305716176,-35.0256567040839,21.1052179492294));
#25848=CARTESIAN_POINT('Ctrl Pts',(133.390663907451,-34.8914297655106,21.1124954389765));
#25849=CARTESIAN_POINT('Ctrl Pts',(133.379068377582,-34.729646136544,21.1217343647834));
#25850=CARTESIAN_POINT('Ctrl Pts',(133.376711765118,-34.7016514480393,21.1233501728052));
#25851=CARTESIAN_POINT('Ctrl Pts',(133.372421166223,-34.6572871173794,21.1259425081241));
#25852=CARTESIAN_POINT('Ctrl Pts',(133.370715210553,-34.6408961335983,21.1269071644245));
#25853=CARTESIAN_POINT('Ctrl Pts',(133.367184962585,-34.6092220824792,21.1287857067231));
#25854=CARTESIAN_POINT('Ctrl Pts',(133.365375987353,-34.5939379569628,21.1296987844487));
#25855=CARTESIAN_POINT('Ctrl Pts',(133.360616237692,-34.5559412934743,21.1319843497481));
#25856=CARTESIAN_POINT('Ctrl Pts',(133.357539253476,-34.5332455351663,21.1333634378651));
#25857=CARTESIAN_POINT('Ctrl Pts',(133.344508280128,-34.4439373361143,21.1388404313999));
#25858=CARTESIAN_POINT('Ctrl Pts',(133.332800420255,-34.3776002467393,21.1430189259567));
#25859=CARTESIAN_POINT('Ctrl Pts',(133.294264914669,-34.1917846567766,21.1549567697375));
#25860=CARTESIAN_POINT('Ctrl Pts',(133.262929354052,-34.0733486064671,21.162838424998));
#25861=CARTESIAN_POINT('Ctrl Pts',(133.150438565884,-33.7255368893349,21.1864011314886));
#25862=CARTESIAN_POINT('Ctrl Pts',(133.050935071364,-33.5028864628366,21.2019842645644));
#25863=CARTESIAN_POINT('Ctrl Pts',(132.902563947965,-33.2483811352218,21.219900462612));
#25864=CARTESIAN_POINT('Ctrl Pts',(132.875673876993,-33.2045762881228,21.2229914967536));
#25865=CARTESIAN_POINT('Ctrl Pts',(132.831481069952,-33.1361263791028,21.2278353957712));
#25866=CARTESIAN_POINT('Ctrl Pts',(132.81482911876,-33.1110725149671,21.2296114125014));
#25867=CARTESIAN_POINT('Ctrl Pts',(132.784383061657,-33.0665614495388,21.2327732546111));
#25868=CARTESIAN_POINT('Ctrl Pts',(132.77071311444,-33.0470221345846,21.234163548169));
#25869=CARTESIAN_POINT('Ctrl Pts',(132.738068487334,-33.001393846203,21.237416552046));
#25870=CARTESIAN_POINT('Ctrl Pts',(132.718925151498,-32.9754280149584,21.2392727411446));
#25871=CARTESIAN_POINT('Ctrl Pts',(132.660760526403,-32.8988473454725,21.2447657551839));
#25872=CARTESIAN_POINT('Ctrl Pts',(132.620674489013,-32.8490571835975,21.2483615817674));
#25873=CARTESIAN_POINT('Ctrl Pts',(132.472469089335,-32.6752725775131,21.2610464877853));
#25874=CARTESIAN_POINT('Ctrl Pts',(132.356761512215,-32.5580453977352,21.269845693574));
#25875=CARTESIAN_POINT('Ctrl Pts',(132.073651224566,-32.3101616406124,21.2898223389195));
#25876=CARTESIAN_POINT('Ctrl Pts',(131.901600002336,-32.1858998320389,21.3009073687721));
#25877=CARTESIAN_POINT('Ctrl Pts',(131.680813906284,-32.055981768142,21.3152499794785));
#25878=CARTESIAN_POINT('Ctrl Pts',(131.64208752184,-32.0342072019635,21.3177707359521));
#25879=CARTESIAN_POINT('Ctrl Pts',(131.585817718685,-32.0040084913975,21.3214566269803));
#25880=CARTESIAN_POINT('Ctrl Pts',(131.56861074205,-31.9949636844864,21.322586812008));
#25881=CARTESIAN_POINT('Ctrl Pts',(131.538038788806,-31.9792277283836,21.3246018904176));
#25882=CARTESIAN_POINT('Ctrl Pts',(131.524705897415,-31.9724762020515,21.3254831165395));
#25883=CARTESIAN_POINT('Ctrl Pts',(131.495161865255,-31.9577603219726,21.3274414986867));
#25884=CARTESIAN_POINT('Ctrl Pts',(131.478931653073,-31.9498373166076,21.3285209416322));
#25885=CARTESIAN_POINT('Ctrl Pts',(131.430378892346,-31.9266142257537,21.3317590492175));
#25886=CARTESIAN_POINT('Ctrl Pts',(131.397877670878,-31.9116959846269,21.3339383548076));
#25887=CARTESIAN_POINT('Ctrl Pts',(131.233519125562,-31.8393804535754,21.3449957003125));
#25888=CARTESIAN_POINT('Ctrl Pts',(131.098348199541,-31.7899049800216,21.3542004646612));
#25889=CARTESIAN_POINT('Ctrl Pts',(130.699241030071,-31.6719890429284,21.3809974654698));
#25890=CARTESIAN_POINT('Ctrl Pts',(130.429625960381,-31.6265648421354,21.3985436677035));
#25891=CARTESIAN_POINT('Ctrl Pts',(130.109125059716,-31.6116615507698,21.4180011702165));
#25892=CARTESIAN_POINT('Ctrl Pts',(130.060752571116,-31.6104491134969,21.4209044068304));
#25893=CARTESIAN_POINT('Ctrl Pts',(129.983190022656,-31.6101660959475,21.4255079706179));
#25894=CARTESIAN_POINT('Ctrl Pts',(129.954010476047,-31.6104363826967,21.4272281844018));
#25895=CARTESIAN_POINT('Ctrl Pts',(129.898156769915,-31.6116751597812,21.4304995703979));
#25896=CARTESIAN_POINT('Ctrl Pts',(129.871483563404,-31.6125819785923,21.4320525129762));
#25897=CARTESIAN_POINT('Ctrl Pts',(129.809612709081,-31.6154172887375,21.4356343324276));
#25898=CARTESIAN_POINT('Ctrl Pts',(129.774428565088,-31.6175799920439,21.4376558776803));
#25899=CARTESIAN_POINT('Ctrl Pts',(129.658128238933,-31.626551594448,21.4442926742673));
#25900=CARTESIAN_POINT('Ctrl Pts',(129.57722098049,-31.6357334005355,21.4488357700602));
#25901=CARTESIAN_POINT('Ctrl Pts',(129.376603024897,-31.6658533143611,21.4599866375184));
#25902=CARTESIAN_POINT('Ctrl Pts',(129.257539108534,-31.6903304809292,21.4664997638447));
#25903=CARTESIAN_POINT('Ctrl Pts',(128.962595429627,-31.7676866294816,21.4827179892139));
#25904=CARTESIAN_POINT('Ctrl Pts',(128.789230696818,-31.8285510376674,21.4923211826765));
#25905=CARTESIAN_POINT('Ctrl Pts',(128.55041494736,-31.9348428776452,21.5066067726672));
#25906=CARTESIAN_POINT('Ctrl Pts',(128.480298371473,-31.9689951799723,21.5109421688899));
#25907=CARTESIAN_POINT('Ctrl Pts',(128.389567187416,-32.0171283052853,21.5168194241486));
#25908=CARTESIAN_POINT('Ctrl Pts',(128.3678358013,-32.0289635910794,21.5182479330366));
#25909=CARTESIAN_POINT('Ctrl Pts',(128.333839870898,-32.0479638940704,21.5205186715805));
#25910=CARTESIAN_POINT('Ctrl Pts',(128.321487030528,-32.0549701288763,21.5213513578358));
#25911=CARTESIAN_POINT('Ctrl Pts',(128.295687957207,-32.0698177857296,21.5231071599524));
#25912=CARTESIAN_POINT('Ctrl Pts',(128.282251179972,-32.0776745033739,21.52403130068));
#25913=CARTESIAN_POINT('Ctrl Pts',(128.248406194686,-32.097778317842,21.5263827223055));
#25914=CARTESIAN_POINT('Ctrl Pts',(128.228072201531,-32.1101482117179,21.5278174099003));
#25915=CARTESIAN_POINT('Ctrl Pts',(128.143777184807,-32.1626520101382,21.5338517000191));
#25916=CARTESIAN_POINT('Ctrl Pts',(128.081039854025,-32.2047009002592,21.5385530978229));
#25917=CARTESIAN_POINT('Ctrl Pts',(127.898206825027,-32.3362992590072,21.5527791308458));
#25918=CARTESIAN_POINT('Ctrl Pts',(127.782586113114,-32.431749755275,21.5624770742481));
#25919=CARTESIAN_POINT('Ctrl Pts',(127.526206777901,-32.6736612024014,21.5851702616093));
#25920=CARTESIAN_POINT('Ctrl Pts',(127.391514919853,-32.8257572873833,21.5980547467719));
#25921=CARTESIAN_POINT('Ctrl Pts',(127.239764229064,-33.0316724069148,21.6136300876327));
#25922=CARTESIAN_POINT('Ctrl Pts',(127.209320179376,-33.0750787970273,21.6168214262843));
#25923=CARTESIAN_POINT('Ctrl Pts',(127.16302275823,-33.1444971020334,21.6217850418477));
#25924=CARTESIAN_POINT('Ctrl Pts',(127.146481326923,-33.170037664999,21.6235824336054));
#25925=CARTESIAN_POINT('Ctrl Pts',(127.116205688537,-33.2181932713178,21.6269189698705));
#25926=CARTESIAN_POINT('Ctrl Pts',(127.102388120413,-33.2407529158776,21.6284610623735));
#25927=CARTESIAN_POINT('Ctrl Pts',(127.071895827569,-33.2918710649817,21.6319095880549));
#25928=CARTESIAN_POINT('Ctrl Pts',(127.055371941876,-33.3205166827609,21.6338105410874));
#25929=CARTESIAN_POINT('Ctrl Pts',(127.005990138883,-33.4090943123837,21.6395967470595));
#25930=CARTESIAN_POINT('Ctrl Pts',(126.974522390244,-33.4697836568545,21.6434338885759));
#25931=CARTESIAN_POINT('Ctrl Pts',(126.904172418033,-33.6161294763308,21.6524266251195));
#25932=CARTESIAN_POINT('Ctrl Pts',(126.866977252481,-33.7025347427677,21.6575312572186));
#25933=CARTESIAN_POINT('Ctrl Pts',(126.829305917559,-33.8011517640883,21.6631969367738));
#25934=CARTESIAN_POINT('Ctrl Pts',(126.825246120578,-33.8119445294727,21.6638149053911));
#25935=CARTESIAN_POINT('Ctrl Pts',(126.821241920569,-33.8227565523843,21.6644320182169));
#25936=CARTESIAN_POINT('Origin',(130.,-35.,23.));
#25937=CARTESIAN_POINT('',(126.821241915871,-33.8227565650708,22.910437866903));
#25938=CARTESIAN_POINT('',(126.82124189288,-33.8227566271494,22.5700841492926));
#25939=CARTESIAN_POINT('',(126.821241915871,-33.8227565650715,23.));
#25940=CARTESIAN_POINT('Ctrl Pts',(126.82124189288,-33.8227566271494,22.5700841492926));
#25941=CARTESIAN_POINT('Ctrl Pts',(126.875221356717,-33.6770028584336,22.5618222215772));
#25942=CARTESIAN_POINT('Ctrl Pts',(126.939173664941,-33.5351017100661,22.5536556010467));
#25943=CARTESIAN_POINT('Ctrl Pts',(127.044327726873,-33.3390072460445,22.5416122053039));
#25944=CARTESIAN_POINT('Ctrl Pts',(127.077738565226,-33.2809064246452,22.5379406552031));
#25945=CARTESIAN_POINT('Ctrl Pts',(127.136615781811,-33.1852015218415,22.5316547567207));
#25946=CARTESIAN_POINT('Ctrl Pts',(127.161156104269,-33.147048941982,22.5290826089747));
#25947=CARTESIAN_POINT('Ctrl Pts',(127.197499573133,-33.092963378713,22.5253228145811));
#25948=CARTESIAN_POINT('Ctrl Pts',(127.208689415927,-33.0766221120918,22.5241715736982));
#25949=CARTESIAN_POINT('Ctrl Pts',(127.228574699369,-33.0481213398838,22.5221350008219));
#25950=CARTESIAN_POINT('Ctrl Pts',(127.237208371548,-33.0359198319151,22.5212536770162));
#25951=CARTESIAN_POINT('Ctrl Pts',(127.25643899417,-33.0091199319431,22.519296588666));
#25952=CARTESIAN_POINT('Ctrl Pts',(127.267071805655,-32.9945489558439,22.5182185586158));
#25953=CARTESIAN_POINT('Ctrl Pts',(127.299060536642,-32.9514391369945,22.5149889810653));
#25954=CARTESIAN_POINT('Ctrl Pts',(127.320750228251,-32.9231523797288,22.5128169463551));
#25955=CARTESIAN_POINT('Ctrl Pts',(127.432642462585,-32.7818976367237,22.5017215039121));
#25956=CARTESIAN_POINT('Ctrl Pts',(127.529554033828,-32.6744478246296,22.4924672381036));
#25957=CARTESIAN_POINT('Ctrl Pts',(127.721678552639,-32.4870342214296,22.4751843327712));
#25958=CARTESIAN_POINT('Ctrl Pts',(127.815015076258,-32.4054695775771,22.4671815930314));
#25959=CARTESIAN_POINT('Ctrl Pts',(127.995772758507,-32.2641967550436,22.4525565229874));
#25960=CARTESIAN_POINT('Ctrl Pts',(128.081933114347,-32.2031144807136,22.4459119587034));
#25961=CARTESIAN_POINT('Ctrl Pts',(128.233179187261,-32.1061725446786,22.4348282356796));
#25962=CARTESIAN_POINT('Ctrl Pts',(128.296845796887,-32.0682496432615,22.4303246455869));
#25963=CARTESIAN_POINT('Ctrl Pts',(128.391527846991,-32.0159787804679,22.4238573207223));
#25964=CARTESIAN_POINT('Ctrl Pts',(128.421594965392,-31.9999661702924,22.4218361685239));
#25965=CARTESIAN_POINT('Ctrl Pts',(128.475512611406,-31.9722867029102,22.4182680576704));
#25966=CARTESIAN_POINT('Ctrl Pts',(128.499268091112,-31.9604419063832,22.4167150472767));
#25967=CARTESIAN_POINT('Ctrl Pts',(128.549973947418,-31.9358986805628,22.4134393429106));
#25968=CARTESIAN_POINT('Ctrl Pts',(128.576957639627,-31.9232739850169,22.4117192621436));
#25969=CARTESIAN_POINT('Ctrl Pts',(128.650893790988,-31.8898627437939,22.4070663652008));
#25970=CARTESIAN_POINT('Ctrl Pts',(128.698158637001,-31.8697842294994,22.4041572684698));
#25971=CARTESIAN_POINT('Ctrl Pts',(128.977721208215,-31.7584517649315,22.3872945684435));
#25972=CARTESIAN_POINT('Ctrl Pts',(129.219065434033,-31.6920034490645,22.3741831590362));
#25973=CARTESIAN_POINT('Ctrl Pts',(129.582798735268,-31.6339266193383,22.3546218455725));
#25974=CARTESIAN_POINT('Ctrl Pts',(129.700961062595,-31.6213790619869,22.3482831836327));
#25975=CARTESIAN_POINT('Ctrl Pts',(129.885572754549,-31.61153641757,22.3381009691775));
#25976=CARTESIAN_POINT('Ctrl Pts',(129.951699729036,-31.6099491172216,22.3343977877195));
#25977=CARTESIAN_POINT('Ctrl Pts',(130.040585416341,-31.6104165625916,22.3292958785399));
#25978=CARTESIAN_POINT('Ctrl Pts',(130.063342108821,-31.6107654592859,22.3279787206335));
#25979=CARTESIAN_POINT('Ctrl Pts',(130.101451985475,-31.6117336865038,22.325752033465));
#25980=CARTESIAN_POINT('Ctrl Pts',(130.116808051709,-31.6122283151603,22.3248491091045));
#25981=CARTESIAN_POINT('Ctrl Pts',(130.148676924486,-31.6134717700329,22.3229625404597));
#25982=CARTESIAN_POINT('Ctrl Pts',(130.165188343072,-31.6142370038163,22.3219781148505));
#25983=CARTESIAN_POINT('Ctrl Pts',(130.209977563612,-31.6166411954713,22.3192899832394));
#25984=CARTESIAN_POINT('Ctrl Pts',(130.238240876734,-31.6185138551292,22.3175744716415));
#25985=CARTESIAN_POINT('Ctrl Pts',(130.418759564762,-31.6327489157916,22.3065084140503));
#25986=CARTESIAN_POINT('Ctrl Pts',(130.570043585579,-31.6550364373433,22.2967454988852));
#25987=CARTESIAN_POINT('Ctrl Pts',(130.905315344659,-31.7278378878598,22.2746608816278));
#25988=CARTESIAN_POINT('Ctrl Pts',(131.087619518073,-31.7838322343053,22.2623521568806));
#25989=CARTESIAN_POINT('Ctrl Pts',(131.362576995636,-31.8943574607892,22.2437822505309));
#25990=CARTESIAN_POINT('Ctrl Pts',(131.458987260906,-31.9384658433892,22.2372640026014));
#25991=CARTESIAN_POINT('Ctrl Pts',(131.58749118131,-32.0047092228763,22.2285739755291));
#25992=CARTESIAN_POINT('Ctrl Pts',(131.621497940462,-32.0229814068246,22.2262737573928));
#25993=CARTESIAN_POINT('Ctrl Pts',(131.678945818758,-32.0551252569402,22.2223856046329));
#25994=CARTESIAN_POINT('Ctrl Pts',(131.702544840901,-32.0687055003295,22.2207876772764));
#25995=CARTESIAN_POINT('Ctrl Pts',(131.750090236053,-32.0968337793337,22.2175658640644));
#25996=CARTESIAN_POINT('Ctrl Pts',(131.774024992314,-32.1113973387821,22.215942694943));
#25997=CARTESIAN_POINT('Ctrl Pts',(131.833983331831,-32.1489065021916,22.2118715301933));
#25998=CARTESIAN_POINT('Ctrl Pts',(131.869759457529,-32.1722396148944,22.2094377336443));
#25999=CARTESIAN_POINT('Ctrl Pts',(132.017878554505,-32.2728830341861,22.1993285089663));
#26000=CARTESIAN_POINT('Ctrl Pts',(132.125949432966,-32.3562630461693,22.1918781044542));
#26001=CARTESIAN_POINT('Ctrl Pts',(132.39383308219,-32.5900218777712,22.1727849839951));
#26002=CARTESIAN_POINT('Ctrl Pts',(132.544583463436,-32.7497737115449,22.1614079093625));
#26003=CARTESIAN_POINT('Ctrl Pts',(132.716442449432,-32.9714269845317,22.1461691520912));
#26004=CARTESIAN_POINT('Ctrl Pts',(132.75270557425,-33.0209145157086,22.1427952045048));
#26005=CARTESIAN_POINT('Ctrl Pts',(132.811836850997,-33.1063810954357,22.1369668667414));
#26006=CARTESIAN_POINT('Ctrl Pts',(132.835406014853,-33.1418580735475,22.1345471040134));
#26007=CARTESIAN_POINT('Ctrl Pts',(132.868690455659,-33.1940670644545,22.1309711652016));
#26008=CARTESIAN_POINT('Ctrl Pts',(132.87894164973,-33.2104543489647,22.1298466606475));
#26009=CARTESIAN_POINT('Ctrl Pts',(132.896855656515,-33.2396435157445,22.127838350852));
#26010=CARTESIAN_POINT('Ctrl Pts',(132.904574953705,-33.2524096677341,22.1269581315384));
#26011=CARTESIAN_POINT('Ctrl Pts',(132.92163476998,-33.2810484332341,22.1249790993513));
#26012=CARTESIAN_POINT('Ctrl Pts',(132.930930293566,-33.2969463313673,22.1238776689857));
#26013=CARTESIAN_POINT('Ctrl Pts',(132.958808882547,-33.3455306645392,22.1205049494262));
#26014=CARTESIAN_POINT('Ctrl Pts',(132.976977472753,-33.3784502287916,22.1182105201633));
#26015=CARTESIAN_POINT('Ctrl Pts',(133.096987633331,-33.604713198634,22.1024129100212));
#26016=CARTESIAN_POINT('Ctrl Pts',(133.180468150924,-33.8072004344837,22.0881766317165));
#26017=CARTESIAN_POINT('Ctrl Pts',(133.302260934746,-34.2088278577358,22.0612052177804));
#26018=CARTESIAN_POINT('Ctrl Pts',(133.343396063065,-34.4061945576884,22.0484936598183));
#26019=CARTESIAN_POINT('Ctrl Pts',(133.372016960801,-34.6508073356001,22.0335998169214));
#26020=CARTESIAN_POINT('Ctrl Pts',(133.376359421202,-34.6956461724549,22.0309027334509));
#26021=CARTESIAN_POINT('Ctrl Pts',(133.381987648654,-34.7689668518173,22.0265444658337));
#26022=CARTESIAN_POINT('Ctrl Pts',(133.383810041427,-34.7974007679625,22.0248670226781));
#26023=CARTESIAN_POINT('Ctrl Pts',(133.386658289675,-34.8527689791085,22.0216243055483));
#26024=CARTESIAN_POINT('Ctrl Pts',(133.387721816002,-34.8796991129522,22.0200579919012));
#26025=CARTESIAN_POINT('Ctrl Pts',(133.389483026834,-34.9436213208268,22.0163645832592));
#26026=CARTESIAN_POINT('Ctrl Pts',(133.389896494211,-34.9806181651762,22.0142463385183));
#26027=CARTESIAN_POINT('Ctrl Pts',(133.389250312565,-35.1049616979434,22.0071858335102));
#26028=CARTESIAN_POINT('Ctrl Pts',(133.385420458441,-35.1922619273485,22.0023271882629));
#26029=CARTESIAN_POINT('Ctrl Pts',(133.355756761783,-35.5510255332498,21.9826167083828));
#26030=CARTESIAN_POINT('Ctrl Pts',(133.300598417627,-35.8190074566996,21.9685856390136));
#26031=CARTESIAN_POINT('Ctrl Pts',(133.192848217436,-36.1404078295949,21.9502306191092));
#26032=CARTESIAN_POINT('Ctrl Pts',(133.169909743399,-36.2026974248961,21.9465927620871));
#26033=CARTESIAN_POINT('Ctrl Pts',(133.128355873861,-36.3060720986387,21.9403584028179));
#26034=CARTESIAN_POINT('Ctrl Pts',(133.110721785273,-36.3475326983147,21.9378032073753));
#26035=CARTESIAN_POINT('Ctrl Pts',(133.084175471041,-36.4066474069874,21.9340638251363));
#26036=CARTESIAN_POINT('Ctrl Pts',(133.075926200067,-36.4245958145135,21.9329155017651));
#26037=CARTESIAN_POINT('Ctrl Pts',(133.061161509957,-36.4559940228749,21.9308820597518));
#26038=CARTESIAN_POINT('Ctrl Pts',(133.054713288279,-36.4694744294754,21.9300009033708));
#26039=CARTESIAN_POINT('Ctrl Pts',(133.040267886372,-36.4991674397782,21.928041626554));
#26040=CARTESIAN_POINT('Ctrl Pts',(133.032230127418,-36.5153587876941,21.92696120431));
#26041=CARTESIAN_POINT('Ctrl Pts',(133.00787023519,-36.5634597327342,21.9237171615184));
#26042=CARTESIAN_POINT('Ctrl Pts',(132.991171580083,-36.5951746129659,21.9215327926247));
#26043=CARTESIAN_POINT('Ctrl Pts',(132.902689659023,-36.7569477101237,21.910177445218));
#26044=CARTESIAN_POINT('Ctrl Pts',(132.822920521991,-36.8824413110184,21.9006575252438));
#26045=CARTESIAN_POINT('Ctrl Pts',(132.660089189368,-37.10487387355,21.8829012027134));
#26046=CARTESIAN_POINT('Ctrl Pts',(132.579277157378,-37.203156791653,21.8746901900265));
#26047=CARTESIAN_POINT('Ctrl Pts',(132.424599185356,-37.3710663485271,21.8601615846144));
#26048=CARTESIAN_POINT('Ctrl Pts',(132.35276543755,-37.4423624399458,21.8538059980752));
#26049=CARTESIAN_POINT('Ctrl Pts',(132.224571909779,-37.5586831918333,21.8431392994375));
#26050=CARTESIAN_POINT('Ctrl Pts',(132.169770335166,-37.6053172003812,21.8387701607497));
#26051=CARTESIAN_POINT('Ctrl Pts',(132.087177910723,-37.6711849288741,21.8324559468023));
#26052=CARTESIAN_POINT('Ctrl Pts',(132.060520357714,-37.691801726297,21.8304572525341));
#26053=CARTESIAN_POINT('Ctrl Pts',(132.012352182321,-37.7279197844041,21.8269139170658));
#26054=CARTESIAN_POINT('Ctrl Pts',(131.990959078749,-37.743572426924,21.8253635315419));
#26055=CARTESIAN_POINT('Ctrl Pts',(131.944960207124,-37.7764069097351,21.8220782134291));
#26056=CARTESIAN_POINT('Ctrl Pts',(131.920305332038,-37.7935162521357,21.8203460988291));
#26057=CARTESIAN_POINT('Ctrl Pts',(131.853100999014,-37.8388427298664,21.8156992605478));
#26058=CARTESIAN_POINT('Ctrl Pts',(131.81013515642,-37.8664302633139,21.8128076563953));
#26059=CARTESIAN_POINT('Ctrl Pts',(131.556047448402,-38.0215825434769,21.796128483962));
#26060=CARTESIAN_POINT('Ctrl Pts',(131.332133877025,-38.1267675299052,21.7831600961581));
#26061=CARTESIAN_POINT('Ctrl Pts',(130.984873325064,-38.2457550638413,21.7636703318022));
#26062=CARTESIAN_POINT('Ctrl Pts',(130.868981081366,-38.2786841910303,21.7572477596199));
#26063=CARTESIAN_POINT('Ctrl Pts',(130.686565101661,-38.320162695996,21.7469481127064));
#26064=CARTESIAN_POINT('Ctrl Pts',(130.62112184417,-38.3330254208299,21.7432153061226));
#26065=CARTESIAN_POINT('Ctrl Pts',(130.532829948524,-38.3476884982262,21.738078679639));
#26066=CARTESIAN_POINT('Ctrl Pts',(130.510276984202,-38.3512002885019,21.7367578531742));
#26067=CARTESIAN_POINT('Ctrl Pts',(130.472474772301,-38.3566961551044,21.7345267823099));
#26068=CARTESIAN_POINT('Ctrl Pts',(130.457243920226,-38.358804769317,21.7336232023414));
#26069=CARTESIAN_POINT('Ctrl Pts',(130.425633665275,-38.3629620146003,21.7317373686895));
#26070=CARTESIAN_POINT('Ctrl Pts',(130.409252914079,-38.3649947334059,21.730754358794));
#26071=CARTESIAN_POINT('Ctrl Pts',(130.364829497876,-38.3701781574071,21.7280741321064));
#26072=CARTESIAN_POINT('Ctrl Pts',(130.336761875379,-38.3730983830254,21.7263652211955));
#26073=CARTESIAN_POINT('Ctrl Pts',(130.169925087337,-38.3883534954738,21.7161282559049));
#26074=CARTESIAN_POINT('Ctrl Pts',(130.03054997845,-38.3924730763807,21.707257317377));
#26075=CARTESIAN_POINT('Ctrl Pts',(129.690938800354,-38.3815802011859,21.6854173459184));
#26076=CARTESIAN_POINT('Ctrl Pts',(129.491494345156,-38.3573854308202,21.6724217762087));
#26077=CARTESIAN_POINT('Ctrl Pts',(129.189017913185,-38.2931034686713,21.6530219697648));
#26078=CARTESIAN_POINT('Ctrl Pts',(129.083826055173,-38.2654022024886,21.6463283351088));
#26079=CARTESIAN_POINT('Ctrl Pts',(128.943019507733,-38.2209800141382,21.6374505728627));
#26080=CARTESIAN_POINT('Ctrl Pts',(128.906103917149,-38.2086307923856,21.6351305758812));
#26081=CARTESIAN_POINT('Ctrl Pts',(128.843686141581,-38.1865479364285,21.6312192195372));
#26082=CARTESIAN_POINT('Ctrl Pts',(128.818074539928,-38.1771373533466,21.6296175757162));
#26083=CARTESIAN_POINT('Ctrl Pts',(128.769531062382,-38.1586325591241,21.6265872255135));
#26084=CARTESIAN_POINT('Ctrl Pts',(128.746579498941,-38.1495952985207,21.625156771354));
#26085=CARTESIAN_POINT('Ctrl Pts',(128.692955588167,-38.1278016771449,21.6218190166652));
#26086=CARTESIAN_POINT('Ctrl Pts',(128.66236777198,-38.1148432638927,21.6199185044834));
#26087=CARTESIAN_POINT('Ctrl Pts',(128.553199733295,-38.066689891399,21.613142722471));
#26088=CARTESIAN_POINT('Ctrl Pts',(128.475773598282,-38.0289525256209,21.6083515493266));
#26089=CARTESIAN_POINT('Ctrl Pts',(128.158332900447,-37.8589738130607,21.5886247714017));
#26090=CARTESIAN_POINT('Ctrl Pts',(127.933388876429,-37.7008476361053,21.5745269229572));
#26091=CARTESIAN_POINT('Ctrl Pts',(127.680569480258,-37.4728658379607,21.556094613114));
#26092=CARTESIAN_POINT('Ctrl Pts',(127.632527933754,-37.4269113128627,21.5524513776684));
#26093=CARTESIAN_POINT('Ctrl Pts',(127.554209658539,-37.3474558258223,21.5462087867545));
#26094=CARTESIAN_POINT('Ctrl Pts',(127.523194235355,-37.3147077676494,21.5436508801519));
#26095=CARTESIAN_POINT('Ctrl Pts',(127.47954294819,-37.2667359445908,21.5399082327382));
#26096=CARTESIAN_POINT('Ctrl Pts',(127.466371359267,-37.2520038771194,21.5387594418239));
#26097=CARTESIAN_POINT('Ctrl Pts',(127.443466599012,-37.225930226349,21.5367254987961));
#26098=CARTESIAN_POINT('Ctrl Pts',(127.433678447333,-37.2146381372794,21.5358443163057));
#26099=CARTESIAN_POINT('Ctrl Pts',(127.412219409588,-37.1895486347702,21.5338853933744));
#26100=CARTESIAN_POINT('Ctrl Pts',(127.400584124366,-37.1757225653415,21.5328053569752));
#26101=CARTESIAN_POINT('Ctrl Pts',(127.366922352102,-37.1350672420323,21.5296296648581));
#26102=CARTESIAN_POINT('Ctrl Pts',(127.345197386002,-37.1079926251747,21.5275149789163));
#26103=CARTESIAN_POINT('Ctrl Pts',(127.209833924155,-36.9338847728349,21.5139424984479));
#26104=CARTESIAN_POINT('Ctrl Pts',(127.108039954802,-36.7780591445625,21.5019308223391));
#26105=CARTESIAN_POINT('Ctrl Pts',(126.94398907362,-36.4752471499145,21.479735322859));
#26106=CARTESIAN_POINT('Ctrl Pts',(126.878317469425,-36.3306624840133,21.4695661429436));
#26107=CARTESIAN_POINT('Ctrl Pts',(126.78954259032,-36.0920526132474,21.4536822123608));
#26108=CARTESIAN_POINT('Ctrl Pts',(126.75991016541,-36.000717862271,21.4477983459049));
#26109=CARTESIAN_POINT('Ctrl Pts',(126.724185279051,-35.8722601470201,21.439794623547));
#26110=CARTESIAN_POINT('Ctrl Pts',(126.71477369126,-35.8361148951158,21.4375715375384));
#26111=CARTESIAN_POINT('Ctrl Pts',(126.699588536887,-35.7735752404079,21.4337734125112));
#26112=CARTESIAN_POINT('Ctrl Pts',(126.693529755223,-35.7472543487111,21.4321895004332));
#26113=CARTESIAN_POINT('Ctrl Pts',(126.681751699707,-35.6931366803916,21.4289617190237));
#26114=CARTESIAN_POINT('Ctrl Pts',(126.676065601144,-35.6653348204779,21.4273190042138));
#26115=CARTESIAN_POINT('Ctrl Pts',(126.662364005628,-35.5937757870995,21.4231286326974));
#26116=CARTESIAN_POINT('Ctrl Pts',(126.654859375633,-35.549925611132,21.4205969821994));
#26117=CARTESIAN_POINT('Ctrl Pts',(126.622801563957,-35.3375467408126,21.4084916433636));
#26118=CARTESIAN_POINT('Ctrl Pts',(126.610107772386,-35.1674705458382,21.3992861357667));
#26119=CARTESIAN_POINT('Ctrl Pts',(126.610452580932,-34.758004344421,21.377469519136));
#26120=CARTESIAN_POINT('Ctrl Pts',(126.63595943991,-34.5195817834189,21.3650620872863));
#26121=CARTESIAN_POINT('Ctrl Pts',(126.695861222004,-34.2416344671744,21.3491545163103));
#26122=CARTESIAN_POINT('Ctrl Pts',(126.706275168305,-34.1976112711154,21.3465892521772));
#26123=CARTESIAN_POINT('Ctrl Pts',(126.722452827094,-34.1348567950213,21.3428498373894));
#26124=CARTESIAN_POINT('Ctrl Pts',(126.727503287372,-34.1159448761843,21.3417120500325));
#26125=CARTESIAN_POINT('Ctrl Pts',(126.73670109481,-34.0826619933657,21.3396887658171));
#26126=CARTESIAN_POINT('Ctrl Pts',(126.740780196718,-34.0682730948824,21.3388070536722));
#26127=CARTESIAN_POINT('Ctrl Pts',(126.74996678249,-34.0366663850937,21.3368544382099));
#26128=CARTESIAN_POINT('Ctrl Pts',(126.755115877096,-34.0194621038904,21.3357813445513));
#26129=CARTESIAN_POINT('Ctrl Pts',(126.770773309181,-33.968621374732,21.3325815004086));
#26130=CARTESIAN_POINT('Ctrl Pts',(126.781669436654,-33.9351079565262,21.3304347946027));
#26131=CARTESIAN_POINT('Ctrl Pts',(126.802146273574,-33.87531394158,21.3265447011104));
#26132=CARTESIAN_POINT('Ctrl Pts',(126.811532548339,-33.8489735142301,21.3248098602003));
#26133=CARTESIAN_POINT('Ctrl Pts',(126.821241906568,-33.8227565901911,21.3230638867798));
#26134=CARTESIAN_POINT('',(126.610250132114,-34.9990536039932,21.7310836956603));
#26135=CARTESIAN_POINT('Ctrl Pts',(126.821241920569,-33.8227565523843,21.6644320182169));
#26136=CARTESIAN_POINT('Ctrl Pts',(126.752438318367,-34.0085380123179,21.6750357805896));
#26137=CARTESIAN_POINT('Ctrl Pts',(126.700049022576,-34.2000063967079,21.6853623555409));
#26138=CARTESIAN_POINT('Ctrl Pts',(126.647643744624,-34.4888977139629,21.7012706745202));
#26139=CARTESIAN_POINT('Ctrl Pts',(126.634581709237,-34.5834969871236,21.7065349591291));
#26140=CARTESIAN_POINT('Ctrl Pts',(126.623044381903,-34.7045978728204,21.7134816678112));
#26141=CARTESIAN_POINT('Ctrl Pts',(126.62086188101,-34.7307099210969,21.7149917963618));
#26142=CARTESIAN_POINT('Ctrl Pts',(126.617829448334,-34.7728750299003,21.7174537985805));
#26143=CARTESIAN_POINT('Ctrl Pts',(126.616790572028,-34.7889139135047,21.7183957745052));
#26144=CARTESIAN_POINT('Ctrl Pts',(126.615063215451,-34.8188851141068,21.7201672184858));
#26145=CARTESIAN_POINT('Ctrl Pts',(126.614346600264,-34.8328154512365,21.7209951189075));
#26146=CARTESIAN_POINT('Ctrl Pts',(126.613006262979,-34.8624320673733,21.7227643873754));
#26147=CARTESIAN_POINT('Ctrl Pts',(126.612405494094,-34.878119100501,21.7237069409951));
#26148=CARTESIAN_POINT('Ctrl Pts',(126.610814475245,-34.9288816874263,21.7267733351668));
#26149=CARTESIAN_POINT('Ctrl Pts',(126.610259927971,-34.9639673342148,21.7289179407535));
#26150=CARTESIAN_POINT('Ctrl Pts',(126.610250132114,-34.9990536039932,21.7310836956603));
#26151=CARTESIAN_POINT('Ctrl Pts',(126.610250133167,-34.9990498377178,21.7310834631812));
#26152=CARTESIAN_POINT('Ctrl Pts',(126.610184089431,-35.2346640589123,21.7456271095323));
#26153=CARTESIAN_POINT('Ctrl Pts',(126.634683158631,-35.4696432505531,21.7610327902304));
#26154=CARTESIAN_POINT('Ctrl Pts',(126.718321766228,-35.8658252201045,21.7869870984347));
#26155=CARTESIAN_POINT('Ctrl Pts',(126.765653934861,-36.0286318897158,21.7976574643732));
#26156=CARTESIAN_POINT('Ctrl Pts',(126.84323383648,-36.2361045111181,21.8111301719299));
#26157=CARTESIAN_POINT('Ctrl Pts',(126.862633153511,-36.284545326814,21.8142680560725));
#26158=CARTESIAN_POINT('Ctrl Pts',(126.894920506843,-36.3600676098888,21.8191500380044));
#26159=CARTESIAN_POINT('Ctrl Pts',(126.907062139507,-36.3874574010428,21.8209184799051));
#26160=CARTESIAN_POINT('Ctrl Pts',(126.930631104539,-36.438778181232,21.8242290802648));
#26161=CARTESIAN_POINT('Ctrl Pts',(126.941979169833,-36.4627428797727,21.8257737592733));
#26162=CARTESIAN_POINT('Ctrl Pts',(126.9684206794,-36.5169287455225,21.8292647617316));
#26163=CARTESIAN_POINT('Ctrl Pts',(126.983687137532,-36.5470626454893,21.8312050042061));
#26164=CARTESIAN_POINT('Ctrl Pts',(127.033086036067,-36.6410573286293,21.8372577575565));
#26165=CARTESIAN_POINT('Ctrl Pts',(127.068816559942,-36.7040575944839,21.8413151773829));
#26166=CARTESIAN_POINT('Ctrl Pts',(127.259517253358,-37.0165298934346,21.86153893919));
#26167=CARTESIAN_POINT('Ctrl Pts',(127.444403973806,-37.2462318720692,21.876612247925));
#26168=CARTESIAN_POINT('Ctrl Pts',(127.705596352677,-37.4961412204957,21.8961677318682));
#26169=CARTESIAN_POINT('Ctrl Pts',(127.756017916026,-37.5415649840546,21.8998833870045));
#26170=CARTESIAN_POINT('Ctrl Pts',(127.842670409812,-37.6150388843688,21.9062366530857));
#26171=CARTESIAN_POINT('Ctrl Pts',(127.878169076405,-37.6439236826234,21.9088308794442));
#26172=CARTESIAN_POINT('Ctrl Pts',(127.929905028485,-37.6843075076711,21.9126172452596));
#26173=CARTESIAN_POINT('Ctrl Pts',(127.945677144192,-37.6963971423887,21.9137722667569));
#26174=CARTESIAN_POINT('Ctrl Pts',(127.973501542113,-37.7173392611635,21.9158129146997));
#26175=CARTESIAN_POINT('Ctrl Pts',(127.985507525298,-37.7262517708347,21.9166944735153));
#26176=CARTESIAN_POINT('Ctrl Pts',(128.012087314788,-37.7457115335876,21.9186488036377));
#26177=CARTESIAN_POINT('Ctrl Pts',(128.026686161449,-37.7562222574362,21.919723794173));
#26178=CARTESIAN_POINT('Ctrl Pts',(128.07025576623,-37.7870674627045,21.922935036427));
#26179=CARTESIAN_POINT('Ctrl Pts',(128.09946126998,-37.8070643334998,21.9250914465276));
#26180=CARTESIAN_POINT('Ctrl Pts',(128.277547850465,-37.9249461814373,21.9382382221361));
#26181=CARTESIAN_POINT('Ctrl Pts',(128.433634347324,-38.0114184188415,21.9497358629018));
#26182=CARTESIAN_POINT('Ctrl Pts',(128.744644839366,-38.1529732583397,21.9717619954101));
#26183=CARTESIAN_POINT('Ctrl Pts',(128.898230702646,-38.2098706163406,21.982264450798));
#26184=CARTESIAN_POINT('Ctrl Pts',(129.149140857578,-38.2826794501964,21.9985772580142));
#26185=CARTESIAN_POINT('Ctrl Pts',(129.244086022803,-38.3058346205192,22.0045691858803));
#26186=CARTESIAN_POINT('Ctrl Pts',(129.376758062242,-38.332174384776,22.0126906453767));
#26187=CARTESIAN_POINT('Ctrl Pts',(129.413729974842,-38.338877696407,22.0149275165718));
#26188=CARTESIAN_POINT('Ctrl Pts',(129.477495112424,-38.349346976491,22.0187416739526));
#26189=CARTESIAN_POINT('Ctrl Pts',(129.504235419351,-38.3534093204029,22.0203280312455));
#26190=CARTESIAN_POINT('Ctrl Pts',(129.559055753787,-38.3610674581038,22.0235543816657));
#26191=CARTESIAN_POINT('Ctrl Pts',(129.587137979988,-38.3646324181504,22.0251933020372));
#26192=CARTESIAN_POINT('Ctrl Pts',(129.659117206343,-38.3728552213844,22.0293606838535));
#26193=CARTESIAN_POINT('Ctrl Pts',(129.703067210523,-38.3770082313533,22.0318734930034));
#26194=CARTESIAN_POINT('Ctrl Pts',(129.905948185439,-38.3921876985808,22.0433434210747));
#26195=CARTESIAN_POINT('Ctrl Pts',(130.065457276097,-38.3928610287155,22.0519832784894));
#26196=CARTESIAN_POINT('Ctrl Pts',(130.421778521114,-38.3692170374748,22.0710499266387));
#26197=CARTESIAN_POINT('Ctrl Pts',(130.617585439835,-38.3388772972301,22.0813628826014));
#26198=CARTESIAN_POINT('Ctrl Pts',(130.893765739832,-38.2709473694263,22.0968450230371));
#26199=CARTESIAN_POINT('Ctrl Pts',(130.97708041638,-38.2470333255409,22.1016466470498));
#26200=CARTESIAN_POINT('Ctrl Pts',(131.082990115519,-38.2121885400554,22.1080256693629));
#26201=CARTESIAN_POINT('Ctrl Pts',(131.106512734401,-38.2041617154124,22.1094602958369));
#26202=CARTESIAN_POINT('Ctrl Pts',(131.144824577782,-38.1906160617389,22.1118293987248));
#26203=CARTESIAN_POINT('Ctrl Pts',(131.159667724175,-38.1852511545534,22.1127553058751));
#26204=CARTESIAN_POINT('Ctrl Pts',(131.189419802427,-38.1742620395046,22.1146284459386));
#26205=CARTESIAN_POINT('Ctrl Pts',(131.204327580887,-38.168635986816,22.1155757562416));
#26206=CARTESIAN_POINT('Ctrl Pts',(131.243044621624,-38.1537118546385,22.118057807387));
#26207=CARTESIAN_POINT('Ctrl Pts',(131.266788925926,-38.1442493738683,22.1196015817096));
#26208=CARTESIAN_POINT('Ctrl Pts',(131.370984535479,-38.1013539880753,22.1264645161839));
#26209=CARTESIAN_POINT('Ctrl Pts',(131.450231376754,-38.0650973466966,22.1319178141608));
#26210=CARTESIAN_POINT('Ctrl Pts',(131.723347585185,-37.9271788971476,22.1513397242616));
#26211=CARTESIAN_POINT('Ctrl Pts',(131.908696543025,-37.8098375472863,22.1656310211412));
#26212=CARTESIAN_POINT('Ctrl Pts',(132.155851447953,-37.6175554713786,22.1854998369281));
#26213=CARTESIAN_POINT('Ctrl Pts',(132.227814251974,-37.5565871750673,22.1914047018569));
#26214=CARTESIAN_POINT('Ctrl Pts',(132.347496579117,-37.4462937303417,22.2014131162497));
#26215=CARTESIAN_POINT('Ctrl Pts',(132.396431872003,-37.3983762203588,22.2055653630469));
#26216=CARTESIAN_POINT('Ctrl Pts',(132.466815181706,-37.3251500712227,22.2116312171359));
#26217=CARTESIAN_POINT('Ctrl Pts',(132.489395533275,-37.3009584937079,22.2135925654058));
#26218=CARTESIAN_POINT('Ctrl Pts',(132.529385012088,-37.256837698431,22.2170952399564));
#26219=CARTESIAN_POINT('Ctrl Pts',(132.546921646025,-37.2370281903119,22.2186418000029));
#26220=CARTESIAN_POINT('Ctrl Pts',(132.584114913181,-37.1940100310811,22.221945859541));
#26221=CARTESIAN_POINT('Ctrl Pts',(132.603694834624,-37.1707379380984,22.2237001723004));
#26222=CARTESIAN_POINT('Ctrl Pts',(132.656489993688,-37.1062449985358,22.2284746855898));
#26223=CARTESIAN_POINT('Ctrl Pts',(132.689057713821,-37.0645038422921,22.231469478068));
#26224=CARTESIAN_POINT('Ctrl Pts',(132.844899887195,-36.8548171161176,22.2460848468508));
#26225=CARTESIAN_POINT('Ctrl Pts',(132.95349031581,-36.6765163826288,22.2571554977244));
#26226=CARTESIAN_POINT('Ctrl Pts',(133.109050969757,-36.3584690494355,22.2759260114666));
#26227=CARTESIAN_POINT('Ctrl Pts',(133.164561654783,-36.2235934840538,22.2836297957879));
#26228=CARTESIAN_POINT('Ctrl Pts',(133.235043387952,-36.015102509684,22.2956898279514));
#26229=CARTESIAN_POINT('Ctrl Pts',(133.256538817358,-35.9438708586632,22.2998369770416));
#26230=CARTESIAN_POINT('Ctrl Pts',(133.281765082318,-35.8491077454208,22.3054573913496));
#26231=CARTESIAN_POINT('Ctrl Pts',(133.287617573049,-35.8261577601654,22.3068264433262));
#26232=CARTESIAN_POINT('Ctrl Pts',(133.296911331859,-35.7880496705314,22.3091155769322));
#26233=CARTESIAN_POINT('Ctrl Pts',(133.30048980961,-35.772925364493,22.3100282012526));
#26234=CARTESIAN_POINT('Ctrl Pts',(133.30714427166,-35.7439114195566,22.3117877077815));
#26235=CARTESIAN_POINT('Ctrl Pts',(133.310237046073,-35.7300261065887,22.3126335368375));
#26236=CARTESIAN_POINT('Ctrl Pts',(133.318496705012,-35.6918115979305,22.3149709715902));
#26237=CARTESIAN_POINT('Ctrl Pts',(133.32348325711,-35.6674448506925,22.31647203487));
#26238=CARTESIAN_POINT('Ctrl Pts',(133.343247215751,-35.5651497581732,22.3228119759294));
#26239=CARTESIAN_POINT('Ctrl Pts',(133.355554311687,-35.4867746852462,22.3277616891127));
#26240=CARTESIAN_POINT('Ctrl Pts',(133.389576254935,-35.2062005783271,22.3456483341834));
#26241=CARTESIAN_POINT('Ctrl Pts',(133.395841705234,-35.0025635363479,22.3589089253334));
#26242=CARTESIAN_POINT('Ctrl Pts',(133.377406421914,-34.6912917783067,22.3788084560034));
#26243=CARTESIAN_POINT('Ctrl Pts',(133.365796517691,-34.5833564213881,22.3856462795732));
#26244=CARTESIAN_POINT('Ctrl Pts',(133.337363583791,-34.4015794389906,22.3970067562618));
#26245=CARTESIAN_POINT('Ctrl Pts',(133.323210122675,-34.3274089813116,22.4015983082196));
#26246=CARTESIAN_POINT('Ctrl Pts',(133.299040697024,-34.2203130049996,22.4081654582626));
#26247=CARTESIAN_POINT('Ctrl Pts',(133.290982980952,-34.1869732602412,22.4102010227236));
#26248=CARTESIAN_POINT('Ctrl Pts',(133.27578758345,-34.1280328666723,22.4137851487468));
#26249=CARTESIAN_POINT('Ctrl Pts',(133.268852340374,-34.102383483895,22.415339959633));
#26250=CARTESIAN_POINT('Ctrl Pts',(133.253539150372,-34.0482817653181,22.4186100854218));
#26251=CARTESIAN_POINT('Ctrl Pts',(133.245087880979,-34.0198523954727,22.4203229126016));
#26252=CARTESIAN_POINT('Ctrl Pts',(133.22118078816,-33.9431320120994,22.4249324364401));
#26253=CARTESIAN_POINT('Ctrl Pts',(133.205012576533,-33.8950699691313,22.4278061878758));
#26254=CARTESIAN_POINT('Ctrl Pts',(133.101021658256,-33.6074632293198,22.4449529549382));
#26255=CARTESIAN_POINT('Ctrl Pts',(132.987465500873,-33.3781014703135,22.4583370456428));
#26256=CARTESIAN_POINT('Ctrl Pts',(132.786568812553,-33.0663962690906,22.4780405459557));
#26257=CARTESIAN_POINT('Ctrl Pts',(132.718961467793,-32.9724313426805,22.484223325471));
#26258=CARTESIAN_POINT('Ctrl Pts',(132.606013255887,-32.8312819245049,22.4941866409162));
#26259=CARTESIAN_POINT('Ctrl Pts',(132.56388549353,-32.7816372559472,22.4978339253717));
#26260=CARTESIAN_POINT('Ctrl Pts',(132.505221491868,-32.7164101360827,22.5028702813325));
#26261=CARTESIAN_POINT('Ctrl Pts',(132.48991772378,-32.6997332634724,22.504180435362));
#26262=CARTESIAN_POINT('Ctrl Pts',(132.463963288543,-32.6720126012728,22.5063987698874));
#26263=CARTESIAN_POINT('Ctrl Pts',(132.453402267455,-32.6608852693096,22.5073004588663));
#26264=CARTESIAN_POINT('Ctrl Pts',(132.43127524936,-32.6378864522204,22.5091885071081));
#26265=CARTESIAN_POINT('Ctrl Pts',(132.419697236351,-32.6260275886735,22.5101756963591));
#26266=CARTESIAN_POINT('Ctrl Pts',(132.387951484392,-32.593985271296,22.5128792674677));
#26267=CARTESIAN_POINT('Ctrl Pts',(132.367615562871,-32.573971229243,22.5146076738232));
#26268=CARTESIAN_POINT('Ctrl Pts',(132.228191839359,-32.440176985522,22.5264194278298));
#26269=CARTESIAN_POINT('Ctrl Pts',(132.101210164485,-32.3349598785437,22.5369806949257));
#26270=CARTESIAN_POINT('Ctrl Pts',(131.857699811985,-32.1614437715059,22.5562448387764));
#26271=CARTESIAN_POINT('Ctrl Pts',(131.743758974418,-32.0900588672015,22.564916675378));
#26272=CARTESIAN_POINT('Ctrl Pts',(131.501385953946,-31.9575708947373,22.5824483428808));
#26273=CARTESIAN_POINT('Ctrl Pts',(131.372732145685,-31.8973963736867,22.5912730949246));
#26274=CARTESIAN_POINT('Ctrl Pts',(131.20151557434,-31.8300574594483,22.6023697703212));
#26275=CARTESIAN_POINT('Ctrl Pts',(131.162075298258,-31.8153875234316,22.6048838840267));
#26276=CARTESIAN_POINT('Ctrl Pts',(131.096054612181,-31.7922208365859,22.6090246050085));
#26277=CARTESIAN_POINT('Ctrl Pts',(131.069624960091,-31.7833114250413,22.6106644701131));
#26278=CARTESIAN_POINT('Ctrl Pts',(131.017394951661,-31.7664196716079,22.6138713167247));
#26279=CARTESIAN_POINT('Ctrl Pts',(130.991603251331,-31.7584174726705,22.6154388399871));
#26280=CARTESIAN_POINT('Ctrl Pts',(130.934363486134,-31.7414052271095,22.6188836228549));
#26281=CARTESIAN_POINT('Ctrl Pts',(130.902874869762,-31.7325404221423,22.6207561490613));
#26282=CARTESIAN_POINT('Ctrl Pts',(130.792298283057,-31.7031310555451,22.6272580668999));
#26283=CARTESIAN_POINT('Ctrl Pts',(130.712597352665,-31.6849905237577,22.6318127169709));
#26284=CARTESIAN_POINT('Ctrl Pts',(130.402046100968,-31.626026246427,22.6491671950613));
#26285=CARTESIAN_POINT('Ctrl Pts',(130.16787032721,-31.6063056199236,22.6613775133596));
#26286=CARTESIAN_POINT('Ctrl Pts',(129.794148306511,-31.6136354855097,22.6813427723163));
#26287=CARTESIAN_POINT('Ctrl Pts',(129.655082326422,-31.6249646710824,22.6888930026413));
#26288=CARTESIAN_POINT('Ctrl Pts',(129.489518815417,-31.6487924752175,22.6984232724398));
#26289=CARTESIAN_POINT('Ctrl Pts',(129.461964281328,-31.6531058617174,22.7000277088801));
#26290=CARTESIAN_POINT('Ctrl Pts',(129.418261448175,-31.6605007170222,22.7026060143201));
#26291=CARTESIAN_POINT('Ctrl Pts',(129.402076358949,-31.6633605980633,22.7035682313963));
#26292=CARTESIAN_POINT('Ctrl Pts',(129.370930258535,-31.6690979562435,22.7054351844467));
#26293=CARTESIAN_POINT('Ctrl Pts',(129.355966803847,-31.6719587781506,22.7063390254833));
#26294=CARTESIAN_POINT('Ctrl Pts',(129.318578828497,-31.6793684630758,22.7086138914072));
#26295=CARTESIAN_POINT('Ctrl Pts',(129.296180327208,-31.6840436639568,22.7099916068013));
#26296=CARTESIAN_POINT('Ctrl Pts',(129.213281287075,-31.7022247781861,22.7151416750835));
#26297=CARTESIAN_POINT('Ctrl Pts',(129.153110397447,-31.7171620856801,22.7189807864738));
#26298=CARTESIAN_POINT('Ctrl Pts',(128.88137091605,-31.79258857924,22.7366818667814));
#26299=CARTESIAN_POINT('Ctrl Pts',(128.675592610951,-31.8719392858899,22.7510597656125));
#26300=CARTESIAN_POINT('Ctrl Pts',(128.379428962843,-32.0206447529596,22.7722301399837));
#26301=CARTESIAN_POINT('Ctrl Pts',(128.282418347726,-32.075495799312,22.7792577344384));
#26302=CARTESIAN_POINT('Ctrl Pts',(128.123337052652,-32.1760940192633,22.7908883247868));
#26303=CARTESIAN_POINT('Ctrl Pts',(128.059807978172,-32.2193588625678,22.7955647500366));
#26304=CARTESIAN_POINT('Ctrl Pts',(127.96994591637,-32.2851377427901,22.8022279586107));
#26305=CARTESIAN_POINT('Ctrl Pts',(127.942403843196,-32.3059519592587,22.8042772157689));
#26306=CARTESIAN_POINT('Ctrl Pts',(127.894213799616,-32.3435405479725,22.8078766282606));
#26307=CARTESIAN_POINT('Ctrl Pts',(127.873436663713,-32.3601437958476,22.809433221016));
#26308=CARTESIAN_POINT('Ctrl Pts',(127.830000691357,-32.3956996143193,22.8126984237339));
#26309=CARTESIAN_POINT('Ctrl Pts',(127.807389772795,-32.4147073725196,22.8144046613531));
#26310=CARTESIAN_POINT('Ctrl Pts',(127.74709185758,-32.4667566890721,22.8189748495515));
#26311=CARTESIAN_POINT('Ctrl Pts',(127.709883722034,-32.5003431101859,22.8218165475283));
#26312=CARTESIAN_POINT('Ctrl Pts',(127.484500773233,-32.713046583648,22.839199802642));
#26313=CARTESIAN_POINT('Ctrl Pts',(127.316692922024,-32.9124736538238,22.852811895961));
#26314=CARTESIAN_POINT('Ctrl Pts',(127.110821566848,-33.2235236397755,22.8726396482673));
#26315=CARTESIAN_POINT('Ctrl Pts',(127.053113162414,-33.3209897680172,22.8786957461462));
#26316=CARTESIAN_POINT('Ctrl Pts',(126.970468588516,-33.4780039889782,22.8884804441466));
#26317=CARTESIAN_POINT('Ctrl Pts',(126.942169452699,-33.535690019088,22.8920814618493));
#26318=CARTESIAN_POINT('Ctrl Pts',(126.906184193166,-33.6146421368958,22.8970635057497));
#26319=CARTESIAN_POINT('Ctrl Pts',(126.897045104032,-33.6352349981405,22.8983677763938));
#26320=CARTESIAN_POINT('Ctrl Pts',(126.88203673246,-33.6699831214862,22.9005791083759));
#26321=CARTESIAN_POINT('Ctrl Pts',(126.876056756953,-33.6840902604301,22.9014797731322));
#26322=CARTESIAN_POINT('Ctrl Pts',(126.863793172486,-33.7135755935075,22.9033691318452));
#26323=CARTESIAN_POINT('Ctrl Pts',(126.857526693039,-33.7289600682777,22.9043586973535));
#26324=CARTESIAN_POINT('Ctrl Pts',(126.841006257433,-33.7703874720365,22.9070322637399));
#26325=CARTESIAN_POINT('Ctrl Pts',(126.83096158199,-33.7965118086049,22.9087275643847));
#26326=CARTESIAN_POINT('Ctrl Pts',(126.821241915871,-33.8227565650702,22.910437866903));
#26327=CARTESIAN_POINT('Origin',(130.,-35.,23.));
#26328=CARTESIAN_POINT('',(126.821241975209,-33.8227564048483,24.1659080048185));
#26329=CARTESIAN_POINT('',(126.821241884814,-33.8227566489294,23.8178897147876));
#26330=CARTESIAN_POINT('',(126.821241915871,-33.8227565650715,23.));
#26331=CARTESIAN_POINT('',(126.610250686307,-35.0021570388984,22.6387449561209));
#26332=CARTESIAN_POINT('Ctrl Pts',(126.821241884814,-33.8227566489294,23.8178897147877));
#26333=CARTESIAN_POINT('Ctrl Pts',(126.830547911808,-33.7976287866224,23.8162401981369));
#26334=CARTESIAN_POINT('Ctrl Pts',(126.840153848162,-33.772605981515,23.8145990229724));
#26335=CARTESIAN_POINT('Ctrl Pts',(126.869647419057,-33.6984204307351,23.8097378524965));
#26336=CARTESIAN_POINT('Ctrl Pts',(126.890390936526,-33.6496116843828,23.8065455595275));
#26337=CARTESIAN_POINT('Ctrl Pts',(126.924828262693,-33.573588468545,23.8015808094579));
#26338=CARTESIAN_POINT('Ctrl Pts',(126.937757555136,-33.5460390753756,23.7997832184751));
#26339=CARTESIAN_POINT('Ctrl Pts',(126.962616483277,-33.4948733609272,23.7964465035576));
#26340=CARTESIAN_POINT('Ctrl Pts',(126.974454927409,-33.4712155483715,23.7949044286691));
#26341=CARTESIAN_POINT('Ctrl Pts',(127.001709970506,-33.4183062597122,23.7914561874206));
#26342=CARTESIAN_POINT('Ctrl Pts',(127.01728016263,-33.3891366690291,23.7895554972374));
#26343=CARTESIAN_POINT('Ctrl Pts',(127.066323880393,-33.3004068760858,23.7837710257596));
#26344=CARTESIAN_POINT('Ctrl Pts',(127.101174120129,-33.2416252539697,23.779935312226));
#26345=CARTESIAN_POINT('Ctrl Pts',(127.272238238132,-32.9720186516412,23.7622517386775));
#26346=CARTESIAN_POINT('Ctrl Pts',(127.429811750342,-32.7756957429772,23.7491758103101));
#26347=CARTESIAN_POINT('Ctrl Pts',(127.709944854719,-32.4966192310434,23.7280812087678));
#26348=CARTESIAN_POINT('Ctrl Pts',(127.818672898893,-32.4013327739757,23.7202756841766));
#26349=CARTESIAN_POINT('Ctrl Pts',(127.955551913448,-32.2960330648351,23.71044126171));
#26350=CARTESIAN_POINT('Ctrl Pts',(127.978185726328,-32.2790677889654,23.708814703716));
#26351=CARTESIAN_POINT('Ctrl Pts',(128.014370942396,-32.2526457729037,23.7062091070921));
#26352=CARTESIAN_POINT('Ctrl Pts',(128.027784226679,-32.2430011022744,23.7052421480911));
#26353=CARTESIAN_POINT('Ctrl Pts',(128.053810504954,-32.2245743181905,23.7033626815613));
#26354=CARTESIAN_POINT('Ctrl Pts',(128.066413574875,-32.2157793248051,23.7024510298915));
#26355=CARTESIAN_POINT('Ctrl Pts',(128.097847635245,-32.194159568455,23.7001742193603));
#26356=CARTESIAN_POINT('Ctrl Pts',(128.116748788784,-32.1814384946211,23.6988025668957));
#26357=CARTESIAN_POINT('Ctrl Pts',(128.191179995932,-32.1324268431552,23.6933954198613));
#26358=CARTESIAN_POINT('Ctrl Pts',(128.247639251099,-32.0975809670038,23.6892818135176));
#26359=CARTESIAN_POINT('Ctrl Pts',(128.408439617249,-32.0047395670314,23.6776073996966));
#26360=CARTESIAN_POINT('Ctrl Pts',(128.514874052137,-31.9505659714966,23.6699297714933));
#26361=CARTESIAN_POINT('Ctrl Pts',(128.851013931739,-31.8012543832227,23.646223659805));
#26362=CARTESIAN_POINT('Ctrl Pts',(129.088528188507,-31.7256453661697,23.630283015533));
#26363=CARTESIAN_POINT('Ctrl Pts',(129.382064835819,-31.6666611377677,23.6120818757022));
#26364=CARTESIAN_POINT('Ctrl Pts',(129.432149513526,-31.6577645082902,23.609023733643));
#26365=CARTESIAN_POINT('Ctrl Pts',(129.512032838721,-31.645422364358,23.6042191544235));
#26366=CARTESIAN_POINT('Ctrl Pts',(129.541708179297,-31.6412395504485,23.6024501949986));
#26367=CARTESIAN_POINT('Ctrl Pts',(129.597735958085,-31.6340986888464,23.5991391497192));
#26368=CARTESIAN_POINT('Ctrl Pts',(129.624075048423,-31.6310552860772,23.5975945354879));
#26369=CARTESIAN_POINT('Ctrl Pts',(129.684031498166,-31.6248394167985,23.5941043790031));
#26370=CARTESIAN_POINT('Ctrl Pts',(129.717666261645,-31.6218595597769,23.5921649060012));
#26371=CARTESIAN_POINT('Ctrl Pts',(129.823470678403,-31.614077182643,23.5861174438135));
#26372=CARTESIAN_POINT('Ctrl Pts',(129.895754954031,-31.6110813062142,23.5820644024377));
#26373=CARTESIAN_POINT('Ctrl Pts',(130.070020760732,-31.6094404171182,23.5724360378762));
#26374=CARTESIAN_POINT('Ctrl Pts',(130.171953638521,-31.6130794192745,23.5669228717045));
#26375=CARTESIAN_POINT('Ctrl Pts',(130.321071319966,-31.6251534497163,23.5589195841914));
#26376=CARTESIAN_POINT('Ctrl Pts',(130.368484631765,-31.6300007121009,23.5563837374015));
#26377=CARTESIAN_POINT('Ctrl Pts',(130.622554238047,-31.6614015264397,23.5427907337562));
#26378=CARTESIAN_POINT('Ctrl Pts',(130.826512211952,-31.7059636903256,23.5318866740389));
#26379=CARTESIAN_POINT('Ctrl Pts',(131.069853690381,-31.7831652559476,23.5176394498414));
#26380=CARTESIAN_POINT('Ctrl Pts',(131.114336748879,-31.7983026606069,23.5149811738008));
#26381=CARTESIAN_POINT('Ctrl Pts',(131.176068908901,-31.8207521442701,23.5111978460947));
#26382=CARTESIAN_POINT('Ctrl Pts',(131.193595648791,-31.827290684641,23.5101129280441));
#26383=CARTESIAN_POINT('Ctrl Pts',(131.225193703566,-31.8393775585697,23.5081359280701));
#26384=CARTESIAN_POINT('Ctrl Pts',(131.2392839456,-31.8448757354378,23.5072466869939));
#26385=CARTESIAN_POINT('Ctrl Pts',(131.268814488704,-31.85662723395,23.5053660668784));
#26386=CARTESIAN_POINT('Ctrl Pts',(131.284246079543,-31.8629002989227,23.5043736330825));
#26387=CARTESIAN_POINT('Ctrl Pts',(131.326347231351,-31.8803774465944,23.5016406775824));
#26388=CARTESIAN_POINT('Ctrl Pts',(131.352920002706,-31.891809336757,23.4998877101594));
#26389=CARTESIAN_POINT('Ctrl Pts',(131.547656144271,-31.9785571740614,23.4868507326663));
#26390=CARTESIAN_POINT('Ctrl Pts',(131.709562378444,-32.0671274624447,23.4749736608001));
#26391=CARTESIAN_POINT('Ctrl Pts',(132.060360576384,-32.2979854492503,23.4479034754087));
#26392=CARTESIAN_POINT('Ctrl Pts',(132.243241443606,-32.4477720307668,23.4328169775543));
#26393=CARTESIAN_POINT('Ctrl Pts',(132.445692207619,-32.6522993780657,23.4153071852525));
#26394=CARTESIAN_POINT('Ctrl Pts',(132.481416759889,-32.6900909333667,23.4121787034557));
#26395=CARTESIAN_POINT('Ctrl Pts',(132.536501879554,-32.7511167322913,23.4072900800265));
#26396=CARTESIAN_POINT('Ctrl Pts',(132.556444254683,-32.7738125420433,23.4055060611986));
#26397=CARTESIAN_POINT('Ctrl Pts',(132.591569510411,-32.8148820662251,23.4023370114084));
#26398=CARTESIAN_POINT('Ctrl Pts',(132.606866858328,-32.8331547961255,23.400947396156));
#26399=CARTESIAN_POINT('Ctrl Pts',(132.642304240279,-32.8764033710224,23.3977048811682));
#26400=CARTESIAN_POINT('Ctrl Pts',(132.662285086708,-32.9015070743428,23.3958583601764));
#26401=CARTESIAN_POINT('Ctrl Pts',(132.720419446321,-32.9767134287119,23.3904273342128));
#26402=CARTESIAN_POINT('Ctrl Pts',(132.75753757047,-33.0276010159845,23.3868823979259));
#26403=CARTESIAN_POINT('Ctrl Pts',(132.881115753394,-33.2073354686621,23.374760947598));
#26404=CARTESIAN_POINT('Ctrl Pts',(132.960137982987,-33.3410657717112,23.3664375811743));
#26405=CARTESIAN_POINT('Ctrl Pts',(133.11643160582,-33.6525444661945,23.3479161257107));
#26406=CARTESIAN_POINT('Ctrl Pts',(133.188190100291,-33.832431516262,23.3377982930934));
#26407=CARTESIAN_POINT('Ctrl Pts',(133.263078529485,-34.0796982057225,23.3235692996567));
#26408=CARTESIAN_POINT('Ctrl Pts',(133.280137473007,-34.1424838427764,23.3199279111274));
#26409=CARTESIAN_POINT('Ctrl Pts',(133.300835350781,-34.2283567038766,23.3148621135368));
#26410=CARTESIAN_POINT('Ctrl Pts',(133.306058540883,-34.2510512372541,23.3135153055207));
#26411=CARTESIAN_POINT('Ctrl Pts',(133.314032361246,-34.2874070501608,23.3113423995842));
#26412=CARTESIAN_POINT('Ctrl Pts',(133.316933395637,-34.3010350235389,23.3105244510493));
#26413=CARTESIAN_POINT('Ctrl Pts',(133.322963780649,-34.330246748709,23.3087630818801));
#26414=CARTESIAN_POINT('Ctrl Pts',(133.326067685264,-34.3458353146965,23.3078182419956));
#26415=CARTESIAN_POINT('Ctrl Pts',(133.333842216942,-34.386367277142,23.3053498720477));
#26416=CARTESIAN_POINT('Ctrl Pts',(133.338342488312,-34.4113418708958,23.3038174829395));
#26417=CARTESIAN_POINT('Ctrl Pts',(133.358026144364,-34.5280729063963,23.296609143737));
#26418=CARTESIAN_POINT('Ctrl Pts',(133.369708432472,-34.6203725044751,23.2907782567168));
#26419=CARTESIAN_POINT('Ctrl Pts',(133.397431156424,-34.9466605214832,23.2699568352102));
#26420=CARTESIAN_POINT('Ctrl Pts',(133.392988439629,-35.1817277983134,23.2546334935683));
#26421=CARTESIAN_POINT('Ctrl Pts',(133.349461587637,-35.5350428979376,23.2321773893474));
#26422=CARTESIAN_POINT('Ctrl Pts',(133.328135175159,-35.6547406614057,23.2246606915477));
#26423=CARTESIAN_POINT('Ctrl Pts',(133.291035715214,-35.8131322441544,23.2148573409886));
#26424=CARTESIAN_POINT('Ctrl Pts',(133.280916644145,-35.8530453232092,23.2123989176489));
#26425=CARTESIAN_POINT('Ctrl Pts',(133.263503255684,-35.9168280787533,23.208487940403));
#26426=CARTESIAN_POINT('Ctrl Pts',(133.256668392898,-35.940817864531,23.2070210011448));
#26427=CARTESIAN_POINT('Ctrl Pts',(133.241875138925,-35.9906470159029,23.2039817436943));
#26428=CARTESIAN_POINT('Ctrl Pts',(133.233871138667,-36.0164710753585,23.2024110098273));
#26429=CARTESIAN_POINT('Ctrl Pts',(133.214027460683,-36.0778864706726,23.1986845092971));
#26430=CARTESIAN_POINT('Ctrl Pts',(133.201904200699,-36.1133828675132,23.1965380448515));
#26431=CARTESIAN_POINT('Ctrl Pts',(133.156263131924,-36.2401015902052,23.1888946129706));
#26432=CARTESIAN_POINT('Ctrl Pts',(133.119414173454,-36.3300775879569,23.1835052320613));
#26433=CARTESIAN_POINT('Ctrl Pts',(133.010920902795,-36.5655786732497,23.1693643398103));
#26434=CARTESIAN_POINT('Ctrl Pts',(132.932619025583,-36.7077558594452,23.160797815657));
#26435=CARTESIAN_POINT('Ctrl Pts',(132.746190528454,-36.9953624870278,23.1426212160717));
#26436=CARTESIAN_POINT('Ctrl Pts',(132.635989208321,-37.1388270564738,23.1330308783856));
#26437=CARTESIAN_POINT('Ctrl Pts',(132.491583098022,-37.2986143742496,23.1208643112932));
#26438=CARTESIAN_POINT('Ctrl Pts',(132.4678717687,-37.3240531648718,23.1188775247553));
#26439=CARTESIAN_POINT('Ctrl Pts',(132.431242187615,-37.3621586535904,23.1158165038008));
#26440=CARTESIAN_POINT('Ctrl Pts',(132.418606292562,-37.3750948716228,23.1147619946361));
#26441=CARTESIAN_POINT('Ctrl Pts',(132.395340799283,-37.3985351414718,23.1128216177442));
#26442=CARTESIAN_POINT('Ctrl Pts',(132.384744390141,-37.4090708866835,23.1119382005952));
#26443=CARTESIAN_POINT('Ctrl Pts',(132.359985474236,-37.4333646391614,23.1098749922807));
#26444=CARTESIAN_POINT('Ctrl Pts',(132.345772098309,-37.4470692934874,23.1086913862744));
#26445=CARTESIAN_POINT('Ctrl Pts',(132.298775093558,-37.4915984898068,23.1047828808652));
#26446=CARTESIAN_POINT('Ctrl Pts',(132.265498565563,-37.5218932969624,23.1020235296191));
#26447=CARTESIAN_POINT('Ctrl Pts',(132.181758654428,-37.5951347013873,23.095120398463));
#26448=CARTESIAN_POINT('Ctrl Pts',(132.130620880852,-37.6372805544383,23.0909401093218));
#26449=CARTESIAN_POINT('Ctrl Pts',(131.864087685929,-37.8441336498446,23.069453858277));
#26450=CARTESIAN_POINT('Ctrl Pts',(131.630684552988,-37.9840940142984,23.0517111109592));
#26451=CARTESIAN_POINT('Ctrl Pts',(131.302187293109,-38.1309051340909,23.0293243240089));
#26452=CARTESIAN_POINT('Ctrl Pts',(131.219887275039,-38.1638798759714,23.0239010450524));
#26453=CARTESIAN_POINT('Ctrl Pts',(131.101390762603,-38.2060447563607,23.0163527060142));
#26454=CARTESIAN_POINT('Ctrl Pts',(131.066194793751,-38.2179206668567,23.0141422165452));
#26455=CARTESIAN_POINT('Ctrl Pts',(131.005113457647,-38.2374186595166,23.0103587117697));
#26456=CARTESIAN_POINT('Ctrl Pts',(130.979319730512,-38.2453144019889,23.0087770036859));
#26457=CARTESIAN_POINT('Ctrl Pts',(130.926140346136,-38.2609014181675,23.0055477475181));
#26458=CARTESIAN_POINT('Ctrl Pts',(130.89874657401,-38.2685575820333,23.0039014302249));
#26459=CARTESIAN_POINT('Ctrl Pts',(130.827959044338,-38.2873844311032,22.9996893054904));
#26460=CARTESIAN_POINT('Ctrl Pts',(130.784433627119,-38.2980413468147,22.9971398414552));
#26461=CARTESIAN_POINT('Ctrl Pts',(130.552377577873,-38.3500046256461,22.9837410651453));
#26462=CARTESIAN_POINT('Ctrl Pts',(130.36078205061,-38.3760182465848,22.9733791174867));
#26463=CARTESIAN_POINT('Ctrl Pts',(129.965421590042,-38.3956364624001,22.9523541217555));
#26464=CARTESIAN_POINT('Ctrl Pts',(129.762370688194,-38.3874859997452,22.9417399257189));
#26465=CARTESIAN_POINT('Ctrl Pts',(129.508132125618,-38.3543023849092,22.9275033880633));
#26466=CARTESIAN_POINT('Ctrl Pts',(129.455153527463,-38.3461052247901,22.9244825521568));
#26467=CARTESIAN_POINT('Ctrl Pts',(129.381102230195,-38.3328424087904,22.9201564105175));
#26468=CARTESIAN_POINT('Ctrl Pts',(129.359847429409,-38.3288252590359,22.9189025926186));
#26469=CARTESIAN_POINT('Ctrl Pts',(129.323754363032,-38.3216452308235,22.916750648339));
#26470=CARTESIAN_POINT('Ctrl Pts',(129.308895902455,-38.3185855905414,22.9158581143804));
#26471=CARTESIAN_POINT('Ctrl Pts',(129.277451050542,-38.3118901530993,22.9139544251808));
#26472=CARTESIAN_POINT('Ctrl Pts',(129.260870901783,-38.3082293632031,22.912942011824));
#26473=CARTESIAN_POINT('Ctrl Pts',(129.214640505371,-38.2976571116272,22.9100962666));
#26474=CARTESIAN_POINT('Ctrl Pts',(129.185055544493,-38.2904706891914,22.9082488171383));
#26475=CARTESIAN_POINT('Ctrl Pts',(128.983414280014,-38.2386043229692,22.8954950754344));
#26476=CARTESIAN_POINT('Ctrl Pts',(128.815020202468,-38.1808515946106,22.8840477355071));
#26477=CARTESIAN_POINT('Ctrl Pts',(128.431649475386,-38.0146856757006,22.8571141772499));
#26478=CARTESIAN_POINT('Ctrl Pts',(128.222087469648,-37.896051324041,22.8417341823877));
#26479=CARTESIAN_POINT('Ctrl Pts',(127.984789883333,-37.7261700232894,22.8239819014037));
#26480=CARTESIAN_POINT('Ctrl Pts',(127.943468278206,-37.6951349737892,22.8208736145039));
#26481=CARTESIAN_POINT('Ctrl Pts',(127.879190504197,-37.6445189738938,22.8160091072229));
#26482=CARTESIAN_POINT('Ctrl Pts',(127.855759641064,-37.6255564918252,22.8142294019036));
#26483=CARTESIAN_POINT('Ctrl Pts',(127.814256013385,-37.5910415913594,22.8110642528796));
#26484=CARTESIAN_POINT('Ctrl Pts',(127.79608875507,-37.5756064471289,22.8096742873531));
#26485=CARTESIAN_POINT('Ctrl Pts',(127.753786027696,-37.5388901366872,22.8064261919594));
#26486=CARTESIAN_POINT('Ctrl Pts',(127.729787526294,-37.5174542223757,22.8045745168159));
#26487=CARTESIAN_POINT('Ctrl Pts',(127.659368595675,-37.4527286879265,22.7991104899942));
#26488=CARTESIAN_POINT('Ctrl Pts',(127.61385359762,-37.4084724288458,22.7955384650104));
#26489=CARTESIAN_POINT('Ctrl Pts',(127.45639460684,-37.2465200337467,22.7829898299827));
#26490=CARTESIAN_POINT('Ctrl Pts',(127.351691651454,-37.122086135163,22.7742953230129));
#26491=CARTESIAN_POINT('Ctrl Pts',(127.134824245472,-36.8231754321495,22.7546852202155));
#26492=CARTESIAN_POINT('Ctrl Pts',(127.028934115131,-36.6449781200022,22.7438586818861));
#26493=CARTESIAN_POINT('Ctrl Pts',(126.919040066319,-36.4143742294821,22.7296222409634));
#26494=CARTESIAN_POINT('Ctrl Pts',(126.899073250631,-36.3700442982055,22.7268747045796));
#26495=CARTESIAN_POINT('Ctrl Pts',(126.872653691574,-36.3078492724187,22.7229847289986));
#26496=CARTESIAN_POINT('Ctrl Pts',(126.865386487054,-36.2903343525093,22.7218854437274));
#26497=CARTESIAN_POINT('Ctrl Pts',(126.852564786459,-36.2586847341258,22.7198905983247));
#26498=CARTESIAN_POINT('Ctrl Pts',(126.846957496691,-36.2445716729039,22.7189980600518));
#26499=CARTESIAN_POINT('Ctrl Pts',(126.835445788105,-36.2150205281709,22.7171220809651));
#26500=CARTESIAN_POINT('Ctrl Pts',(126.829559191831,-36.1995763004391,22.71613772376));
#26501=CARTESIAN_POINT('Ctrl Pts',(126.813893304726,-36.1575539784773,22.7134499742199));
#26502=CARTESIAN_POINT('Ctrl Pts',(126.804333979025,-36.1308959523763,22.7117347816865));
#26503=CARTESIAN_POINT('Ctrl Pts',(126.744820610243,-35.9581489655936,22.7005690518424));
#26504=CARTESIAN_POINT('Ctrl Pts',(126.704567254605,-35.8089231302589,22.6906971957163));
#26505=CARTESIAN_POINT('Ctrl Pts',(126.63195401171,-35.4416684464721,22.6665957114359));
#26506=CARTESIAN_POINT('Ctrl Pts',(126.61039070071,-35.2221872513799,22.6523831461664));
#26507=CARTESIAN_POINT('Ctrl Pts',(126.610250686307,-35.0021570388984,22.6387449561209));
#26508=CARTESIAN_POINT('Ctrl Pts',(126.610250683868,-35.0021532034418,22.6387447183869));
#26509=CARTESIAN_POINT('Ctrl Pts',(126.610218691316,-34.9517879050375,22.6356229144437));
#26510=CARTESIAN_POINT('Ctrl Pts',(126.61130919799,-34.901425866968,22.6325306774218));
#26511=CARTESIAN_POINT('Ctrl Pts',(126.615250248782,-34.8117907148621,22.6270802631384));
#26512=CARTESIAN_POINT('Ctrl Pts',(126.617663286356,-34.7725089830984,22.624709880538));
#26513=CARTESIAN_POINT('Ctrl Pts',(126.622844410456,-34.706866888933,22.6207784648604));
#26514=CARTESIAN_POINT('Ctrl Pts',(126.625238527359,-34.6804816760169,22.6192062325317));
#26515=CARTESIAN_POINT('Ctrl Pts',(126.630507076093,-34.6291164756261,22.6161605211917));
#26516=CARTESIAN_POINT('Ctrl Pts',(126.63335059779,-34.6041351162239,22.6146861925193));
#26517=CARTESIAN_POINT('Ctrl Pts',(126.63997234392,-34.5512079497467,22.6115765120531));
#26518=CARTESIAN_POINT('Ctrl Pts',(126.643821893556,-34.5232728855082,22.6099434891408));
#26519=CARTESIAN_POINT('Ctrl Pts',(126.654511184851,-34.4522671855163,22.6058119415004));
#26520=CARTESIAN_POINT('Ctrl Pts',(126.661834404157,-34.4092738814656,22.6033285227861));
#26521=CARTESIAN_POINT('Ctrl Pts',(126.699004926034,-34.2139065936132,22.5921111504173));
#26522=CARTESIAN_POINT('Ctrl Pts',(126.738470590289,-34.0635469347733,22.5836776502972));
#26523=CARTESIAN_POINT('Ctrl Pts',(126.798698643084,-33.8850238155912,22.5736077440637));
#26524=CARTESIAN_POINT('Ctrl Pts',(126.80974403253,-33.8538028132203,22.571843975796));
#26525=CARTESIAN_POINT('Ctrl Pts',(126.82124189288,-33.8227566271494,22.5700841492926));
#26526=CARTESIAN_POINT('Ctrl Pts',(126.821241915871,-33.8227565650702,22.910437866903));
#26527=CARTESIAN_POINT('Ctrl Pts',(126.82099104874,-33.8234339491151,22.9104820102593));
#26528=CARTESIAN_POINT('Ctrl Pts',(126.820740398121,-33.8241114133797,22.9105261636133));
#26529=CARTESIAN_POINT('Ctrl Pts',(126.762030822358,-33.982948999682,22.9208794240525));
#26530=CARTESIAN_POINT('Ctrl Pts',(126.715459369069,-34.1452369403566,22.9317036970583));
#26531=CARTESIAN_POINT('Ctrl Pts',(126.652004459477,-34.4505819230391,22.9518005612867));
#26532=CARTESIAN_POINT('Ctrl Pts',(126.631773965391,-34.592579412559,22.9610437876921));
#26533=CARTESIAN_POINT('Ctrl Pts',(126.61374749444,-34.8228406799421,22.9756516692902));
#26534=CARTESIAN_POINT('Ctrl Pts',(126.610297960021,-34.9104825912722,22.981125822323));
#26535=CARTESIAN_POINT('Ctrl Pts',(126.610215302828,-35.0631810994019,22.9904959503338));
#26536=CARTESIAN_POINT('Ctrl Pts',(126.612050631295,-35.1281876952586,22.9944324614789));
#26537=CARTESIAN_POINT('Ctrl Pts',(126.617604134591,-35.2255152586737,23.0002495803037));
#26538=CARTESIAN_POINT('Ctrl Pts',(126.619919010954,-35.2578983126503,23.002172388253));
#26539=CARTESIAN_POINT('Ctrl Pts',(126.624960736115,-35.3165642123053,23.0056339323517));
#26540=CARTESIAN_POINT('Ctrl Pts',(126.627530335416,-35.3428576282269,23.0071773747259));
#26541=CARTESIAN_POINT('Ctrl Pts',(126.63377052809,-35.3998227684592,23.0105049966958));
#26542=CARTESIAN_POINT('Ctrl Pts',(126.637553537661,-35.4304799441682,23.0122855648604));
#26543=CARTESIAN_POINT('Ctrl Pts',(126.649479605335,-35.5173422938289,23.0173041973384));
#26544=CARTESIAN_POINT('Ctrl Pts',(126.658616919227,-35.573401768844,23.020511566431));
#26545=CARTESIAN_POINT('Ctrl Pts',(126.682685868905,-35.7008157627025,23.0277482778569));
#26546=CARTESIAN_POINT('Ctrl Pts',(126.698519070877,-35.7719717129499,23.0317510149133));
#26547=CARTESIAN_POINT('Ctrl Pts',(126.765572759789,-36.0332711437679,23.0463955384083));
#26548=CARTESIAN_POINT('Ctrl Pts',(126.83103182175,-36.2193483948337,23.056693662574));
#26549=CARTESIAN_POINT('Ctrl Pts',(126.971707682056,-36.5299015523981,23.0748827619362));
#26550=CARTESIAN_POINT('Ctrl Pts',(127.039439883645,-36.657174828069,23.0826679670223));
#26551=CARTESIAN_POINT('Ctrl Pts',(127.129901141975,-36.8038119459335,23.0924796146608));
#26552=CARTESIAN_POINT('Ctrl Pts',(127.145050909777,-36.8276954266485,23.0941060009977));
#26553=CARTESIAN_POINT('Ctrl Pts',(127.16952014108,-36.8652243165318,23.0967113875397));
#26554=CARTESIAN_POINT('Ctrl Pts',(127.178643900167,-36.8789964650642,23.0976783114826));
#26555=CARTESIAN_POINT('Ctrl Pts',(127.196449364859,-36.9054514201454,23.0995577678874));
#26556=CARTESIAN_POINT('Ctrl Pts',(127.205117237884,-36.9181427449747,23.1004694452645));
#26557=CARTESIAN_POINT('Ctrl Pts',(127.226849237619,-36.9495022665738,23.1027464050047));
#26558=CARTESIAN_POINT('Ctrl Pts',(127.240015752354,-36.968098353516,23.1041181827489));
#26559=CARTESIAN_POINT('Ctrl Pts',(127.292254643203,-37.0403242169623,23.1095264794334));
#26560=CARTESIAN_POINT('Ctrl Pts',(127.332708699814,-37.092931859177,23.1136411504478));
#26561=CARTESIAN_POINT('Ctrl Pts',(127.450208391119,-37.2367888088423,23.125319848251));
#26562=CARTESIAN_POINT('Ctrl Pts',(127.530569280683,-37.325203390577,23.133000784026));
#26563=CARTESIAN_POINT('Ctrl Pts',(127.791954538115,-37.5839183108784,23.1567044608626));
#26564=CARTESIAN_POINT('Ctrl Pts',(127.987184666386,-37.7387423425457,23.1726391825686));
#26565=CARTESIAN_POINT('Ctrl Pts',(128.24068951947,-37.8978991404231,23.1908356517705));
#26566=CARTESIAN_POINT('Ctrl Pts',(128.284377223569,-37.9239753254123,23.1938943767824));
#26567=CARTESIAN_POINT('Ctrl Pts',(128.354709767108,-37.9638358993376,23.1986996561776));
#26568=CARTESIAN_POINT('Ctrl Pts',(128.380977789022,-37.9782663338575,23.2004687438768));
#26569=CARTESIAN_POINT('Ctrl Pts',(128.430838771203,-38.0048029920779,23.2037799058657));
#26570=CARTESIAN_POINT('Ctrl Pts',(128.454388967973,-38.0169843519115,23.2053245103925));
#26571=CARTESIAN_POINT('Ctrl Pts',(128.508246765071,-38.0440461773995,23.2088144805509));
#26572=CARTESIAN_POINT('Ctrl Pts',(128.53863886894,-38.0587527859887,23.2107537796421));
#26573=CARTESIAN_POINT('Ctrl Pts',(128.634795987094,-38.1035223903969,23.2168000227788));
#26574=CARTESIAN_POINT('Ctrl Pts',(128.701308082851,-38.1319376661058,23.2208520521741));
#26575=CARTESIAN_POINT('Ctrl Pts',(128.863624578295,-38.1952214841995,23.2304773877655));
#26576=CARTESIAN_POINT('Ctrl Pts',(128.96019232814,-38.2279391751071,23.2359885935928));
#26577=CARTESIAN_POINT('Ctrl Pts',(129.10371966805,-38.2694560289283,23.2439815973126));
#26578=CARTESIAN_POINT('Ctrl Pts',(129.149620329422,-38.2816940240597,23.2465091996543));
#26579=CARTESIAN_POINT('Ctrl Pts',(129.397783530491,-38.342302626394,23.2600735243816));
#26580=CARTESIAN_POINT('Ctrl Pts',(129.603896497924,-38.3729420110107,23.2709571366214));
#26581=CARTESIAN_POINT('Ctrl Pts',(129.858832844804,-38.3871410868485,23.2852012808286));
#26582=CARTESIAN_POINT('Ctrl Pts',(129.906218652212,-38.3887840753286,23.2878828898149));
#26583=CARTESIAN_POINT('Ctrl Pts',(129.972394059845,-38.3896895837878,23.2916941549857));
#26584=CARTESIAN_POINT('Ctrl Pts',(129.991168634878,-38.3897904854055,23.292782899158));
#26585=CARTESIAN_POINT('Ctrl Pts',(130.025083617667,-38.3896910075231,23.2947646364064));
#26586=CARTESIAN_POINT('Ctrl Pts',(130.040223947393,-38.3895451527241,23.295654740488));
#26587=CARTESIAN_POINT('Ctrl Pts',(130.071983152491,-38.389026379111,23.2975340552605));
#26588=CARTESIAN_POINT('Ctrl Pts',(130.088600907703,-38.3886326484421,23.2985242831775));
#26589=CARTESIAN_POINT('Ctrl Pts',(130.133961883737,-38.3872240069773,23.3012448645861));
#26590=CARTESIAN_POINT('Ctrl Pts',(130.162695517743,-38.385965491429,23.3029874856713));
#26591=CARTESIAN_POINT('Ctrl Pts',(130.376393709729,-38.373879337996,23.3160743407193));
#26592=CARTESIAN_POINT('Ctrl Pts',(130.560194154702,-38.3482689477335,23.3280194918785));
#26593=CARTESIAN_POINT('Ctrl Pts',(130.970179870068,-38.2564294129084,23.3551025273855));
#26594=CARTESIAN_POINT('Ctrl Pts',(131.193471606607,-38.1813893440609,23.3701339875679));
#26595=CARTESIAN_POINT('Ctrl Pts',(131.454584943649,-38.0622372677699,23.3875979139282));
#26596=CARTESIAN_POINT('Ctrl Pts',(131.501437119071,-38.0395396804537,23.390729885767));
#26597=CARTESIAN_POINT('Ctrl Pts',(131.574638243906,-38.0019714971347,23.3956226789002));
#26598=CARTESIAN_POINT('Ctrl Pts',(131.601341372054,-37.9878126392964,23.3974074453966));
#26599=CARTESIAN_POINT('Ctrl Pts',(131.650855045311,-37.9607043782557,23.4007177068324));
#26600=CARTESIAN_POINT('Ctrl Pts',(131.673711392157,-37.9478437931481,23.4022461477179));
#26601=CARTESIAN_POINT('Ctrl Pts',(131.725188957321,-37.9180871450768,23.4056905240933));
#26602=CARTESIAN_POINT('Ctrl Pts',(131.753715784527,-37.9010326754021,23.4076006685354));
#26603=CARTESIAN_POINT('Ctrl Pts',(131.840921846817,-37.8471409244757,23.4134484137288));
#26604=CARTESIAN_POINT('Ctrl Pts',(131.898727851236,-37.8089211699321,23.4173363355261));
#26605=CARTESIAN_POINT('Ctrl Pts',(132.033624581195,-37.7136625089983,23.4264768559567));
#26606=CARTESIAN_POINT('Ctrl Pts',(132.109547061533,-37.6550717503198,23.4316760074138));
#26607=CARTESIAN_POINT('Ctrl Pts',(132.284852332273,-37.5075123022938,23.4439640120745));
#26608=CARTESIAN_POINT('Ctrl Pts',(132.381667757404,-37.4157456970804,23.450985117923));
#26609=CARTESIAN_POINT('Ctrl Pts',(132.576399169963,-37.2080538013853,23.4661215911864));
#26610=CARTESIAN_POINT('Ctrl Pts',(132.672442355327,-37.0907839315999,23.4742392434749));
#26611=CARTESIAN_POINT('Ctrl Pts',(132.781228110879,-36.9381623548048,23.4848176505006));
#26612=CARTESIAN_POINT('Ctrl Pts',(132.801670091542,-36.9084935418959,23.4868748943246));
#26613=CARTESIAN_POINT('Ctrl Pts',(132.831672365347,-36.8634282308166,23.4900099925321));
#26614=CARTESIAN_POINT('Ctrl Pts',(132.841589026969,-36.8482707934181,23.4910661714537));
#26615=CARTESIAN_POINT('Ctrl Pts',(132.859385644309,-36.8205872077836,23.4929996534261));
#26616=CARTESIAN_POINT('Ctrl Pts',(132.867305736671,-36.8080878937493,23.4938743731124));
#26617=CARTESIAN_POINT('Ctrl Pts',(132.885535456707,-36.7788971489478,23.4959210893217));
#26618=CARTESIAN_POINT('Ctrl Pts',(132.895782244796,-36.7621677242874,23.4970968896798));
#26619=CARTESIAN_POINT('Ctrl Pts',(132.928669921785,-36.7074121168421,23.5009520140095));
#26620=CARTESIAN_POINT('Ctrl Pts',(132.950710589783,-36.6690327342506,23.5036645635286));
#26621=CARTESIAN_POINT('Ctrl Pts',(133.003118944002,-36.5734899177844,23.5104225855791));
#26622=CARTESIAN_POINT('Ctrl Pts',(133.032612369083,-36.5158678354111,23.5145027804693));
#26623=CARTESIAN_POINT('Ctrl Pts',(133.16907408796,-36.2293157499042,23.5347007294079));
#26624=CARTESIAN_POINT('Ctrl Pts',(133.251876674452,-35.9897301058736,23.5512275691034));
#26625=CARTESIAN_POINT('Ctrl Pts',(133.330131363948,-35.6414774120627,23.5735961284351));
#26626=CARTESIAN_POINT('Ctrl Pts',(133.348281278378,-35.5387801430027,23.5800105924801));
#26627=CARTESIAN_POINT('Ctrl Pts',(133.366735839005,-35.3962950804308,23.5886539906304));
#26628=CARTESIAN_POINT('Ctrl Pts',(133.371118217657,-35.3571024501742,23.5910053908385));
#26629=CARTESIAN_POINT('Ctrl Pts',(133.377126574664,-35.2933060891642,23.5947920565171));
#26630=CARTESIAN_POINT('Ctrl Pts',(133.379169700171,-35.2687462530776,23.5962400288211));
#26631=CARTESIAN_POINT('Ctrl Pts',(133.382911860536,-35.2169288547645,23.5992751419442));
#26632=CARTESIAN_POINT('Ctrl Pts',(133.384549702556,-35.1896685501678,23.600860294272));
#26633=CARTESIAN_POINT('Ctrl Pts',(133.387728805286,-35.1233840794671,23.6046880573141));
#26634=CARTESIAN_POINT('Ctrl Pts',(133.388925475389,-35.0843468399124,23.6069199685269));
#26635=CARTESIAN_POINT('Ctrl Pts',(133.390915102305,-34.9354668633698,23.6153556218887));
#26636=CARTESIAN_POINT('Ctrl Pts',(133.38704388264,-34.8256250878844,23.6214181905919));
#26637=CARTESIAN_POINT('Ctrl Pts',(133.360687703521,-34.5119756760426,23.6384903743963));
#26638=CARTESIAN_POINT('Ctrl Pts',(133.32505315594,-34.309774675517,23.6491843918476));
#26639=CARTESIAN_POINT('Ctrl Pts',(133.236339528424,-33.9829444446467,23.6672950312395));
#26640=CARTESIAN_POINT('Ctrl Pts',(133.193694996535,-33.856059111773,23.6745531928376));
#26641=CARTESIAN_POINT('Ctrl Pts',(133.133168268083,-33.7059944809986,23.6837701862437));
#26642=CARTESIAN_POINT('Ctrl Pts',(133.122340989274,-33.6800832157172,23.6853853654109));
#26643=CARTESIAN_POINT('Ctrl Pts',(133.104652142154,-33.6391871403826,23.6879769248676));
#26644=CARTESIAN_POINT('Ctrl Pts',(133.098000835993,-33.624112156426,23.6889414463183));
#26645=CARTESIAN_POINT('Ctrl Pts',(133.08492401723,-33.5950495375422,23.6908199358509));
#26646=CARTESIAN_POINT('Ctrl Pts',(133.078512709476,-33.5810562175969,23.6917330984575));
#26647=CARTESIAN_POINT('Ctrl Pts',(133.062321912723,-33.5463444490477,23.6940191830544));
#26648=CARTESIAN_POINT('Ctrl Pts',(133.052427333971,-33.5256807449137,23.6953987119341));
#26649=CARTESIAN_POINT('Ctrl Pts',(133.012595449593,-33.4446163945177,23.7008798788137));
#26650=CARTESIAN_POINT('Ctrl Pts',(132.981070231003,-33.3850174768372,23.7050622552517));
#26651=CARTESIAN_POINT('Ctrl Pts',(132.887254895,-33.219775821444,23.717015986941));
#26652=CARTESIAN_POINT('Ctrl Pts',(132.820980027847,-33.1165170455659,23.7249099819555));
#26653=CARTESIAN_POINT('Ctrl Pts',(132.607218004869,-32.8201421700877,23.7484644145453));
#26654=CARTESIAN_POINT('Ctrl Pts',(132.444403485207,-32.6390061985273,23.7640263896184));
#26655=CARTESIAN_POINT('Ctrl Pts',(132.22533177626,-32.4424723667827,23.7819255359141));
#26656=CARTESIAN_POINT('Ctrl Pts',(132.186278816788,-32.4090089777049,23.7850183720514));
#26657=CARTESIAN_POINT('Ctrl Pts',(132.123191479038,-32.3573936646943,23.7898644242251));
#26658=CARTESIAN_POINT('Ctrl Pts',(132.099651846995,-32.3386521255418,23.7916408268109));
#26659=CARTESIAN_POINT('Ctrl Pts',(132.057014879181,-32.3056237435785,23.7948030142445));
#26660=CARTESIAN_POINT('Ctrl Pts',(132.038010638914,-32.2912205141639,23.7961932728847));
#26661=CARTESIAN_POINT('Ctrl Pts',(131.992950259457,-32.2578121311745,23.7994457596723));
#26662=CARTESIAN_POINT('Ctrl Pts',(131.966771507508,-32.2389757363414,23.8013014736034));
#26663=CARTESIAN_POINT('Ctrl Pts',(131.887964141413,-32.1839611926456,23.8067914299035));
#26664=CARTESIAN_POINT('Ctrl Pts',(131.834576422565,-32.1488926305017,23.8103847450437));
#26665=CARTESIAN_POINT('Ctrl Pts',(131.640206361493,-32.0289393970981,23.823070345762));
#26666=CARTESIAN_POINT('Ctrl Pts',(131.494072041906,-31.9528319911576,23.8318724069918));
#26667=CARTESIAN_POINT('Ctrl Pts',(131.148558022859,-31.8037431645573,23.8518497691372));
#26668=CARTESIAN_POINT('Ctrl Pts',(130.94672145762,-31.7382605386934,23.862932748559));
#26669=CARTESIAN_POINT('Ctrl Pts',(130.69672555456,-31.6823267289896,23.8772749766537));
#26670=CARTESIAN_POINT('Ctrl Pts',(130.653146080762,-31.6734729460076,23.8797980181451));
#26671=CARTESIAN_POINT('Ctrl Pts',(130.59027762137,-31.6619832897281,23.8834866588573));
#26672=CARTESIAN_POINT('Ctrl Pts',(130.571118738339,-31.658651982187,23.8846172366288));
#26673=CARTESIAN_POINT('Ctrl Pts',(130.537186083,-31.6530522021898,23.8866327371998));
#26674=CARTESIAN_POINT('Ctrl Pts',(130.522424344964,-31.6507163093001,23.8875139866667));
#26675=CARTESIAN_POINT('Ctrl Pts',(130.489795206329,-31.6457740501232,23.8894720630821));
#26676=CARTESIAN_POINT('Ctrl Pts',(130.471922353268,-31.6432127968506,23.8905511718802));
#26677=CARTESIAN_POINT('Ctrl Pts',(130.418619126482,-31.6360083307154,23.8937872588269));
#26678=CARTESIAN_POINT('Ctrl Pts',(130.383135930791,-31.6317825835941,23.8959648414437));
#26679=CARTESIAN_POINT('Ctrl Pts',(130.204804610918,-31.6133991009827,23.9070041884261));
#26680=CARTESIAN_POINT('Ctrl Pts',(130.061235112937,-31.6077655870104,23.9161915897613));
#26681=CARTESIAN_POINT('Ctrl Pts',(129.645035363894,-31.6178668901878,23.9429982833793));
#26682=CARTESIAN_POINT('Ctrl Pts',(129.374061635519,-31.6573851642018,23.9605728054815));
#26683=CARTESIAN_POINT('Ctrl Pts',(129.064104621089,-31.7416507753097,23.9800511756094));
#26684=CARTESIAN_POINT('Ctrl Pts',(129.01775224568,-31.7553228912587,23.9829506436435));
#26685=CARTESIAN_POINT('Ctrl Pts',(128.94391420433,-31.778829633505,23.9875497270389));
#26686=CARTESIAN_POINT('Ctrl Pts',(128.916236970659,-31.7880358791561,23.9892691602955));
#26687=CARTESIAN_POINT('Ctrl Pts',(128.863465654284,-31.8063489317281,23.992539963171));
#26688=CARTESIAN_POINT('Ctrl Pts',(128.838353690229,-31.8153971400255,23.9940930904858));
#26689=CARTESIAN_POINT('Ctrl Pts',(128.780307724944,-31.8370899247414,23.9976766400935));
#26690=CARTESIAN_POINT('Ctrl Pts',(128.747458711238,-31.8499539935427,23.9996997071762));
#26691=CARTESIAN_POINT('Ctrl Pts',(128.639332609322,-31.8942563683168,24.0063479059001));
#26692=CARTESIAN_POINT('Ctrl Pts',(128.564987141215,-31.9278999425594,24.0109005240269));
#26693=CARTESIAN_POINT('Ctrl Pts',(128.382783596397,-32.0184119673033,24.0220822268754));
#26694=CARTESIAN_POINT('Ctrl Pts',(128.276642139766,-32.0784770439541,24.0286159209385));
#26695=CARTESIAN_POINT('Ctrl Pts',(128.018536703292,-32.2435092327085,24.0449091424842));
#26696=CARTESIAN_POINT('Ctrl Pts',(127.871492782923,-32.3554040474251,24.0545660389377));
#26697=CARTESIAN_POINT('Ctrl Pts',(127.677338622234,-32.5298761191181,24.0688423294303));
#26698=CARTESIAN_POINT('Ctrl Pts',(127.622140874676,-32.5829662446655,24.0731025600854));
#26699=CARTESIAN_POINT('Ctrl Pts',(127.551643713595,-32.655525190657,24.0788927647717));
#26700=CARTESIAN_POINT('Ctrl Pts',(127.534688736915,-32.6733605913742,24.0803136059769));
#26701=CARTESIAN_POINT('Ctrl Pts',(127.508275595749,-32.7017581716639,24.0825751061112));
#26702=CARTESIAN_POINT('Ctrl Pts',(127.498686610119,-32.712198147149,24.0834063553604));
#26703=CARTESIAN_POINT('Ctrl Pts',(127.478688857615,-32.7342466413048,24.0851623302159));
#26704=CARTESIAN_POINT('Ctrl Pts',(127.468294282524,-32.7458672867926,24.0860881158017));
#26705=CARTESIAN_POINT('Ctrl Pts',(127.442149843759,-32.7755044848018,24.0884490725075));
#26706=CARTESIAN_POINT('Ctrl Pts',(127.426510093778,-32.7936166809816,24.0898917674628));
#26707=CARTESIAN_POINT('Ctrl Pts',(127.361504641657,-32.8705301557401,24.0960119500959));
#26708=CARTESIAN_POINT('Ctrl Pts',(127.313955328994,-32.9308306329129,24.1007947299246));
#26709=CARTESIAN_POINT('Ctrl Pts',(127.177005913177,-33.1171881710146,24.1154076957921));
#26710=CARTESIAN_POINT('Ctrl Pts',(127.094135743321,-33.2477938054022,24.1254203025004));
#26711=CARTESIAN_POINT('Ctrl Pts',(126.943698634776,-33.5250954934791,24.145719522381));
#26712=CARTESIAN_POINT('Ctrl Pts',(126.87712746268,-33.6718560792905,24.1559689145811));
#26713=CARTESIAN_POINT('Ctrl Pts',(126.821241975209,-33.8227564048483,24.1659080048185));
#26714=CARTESIAN_POINT('Origin',(130.,-35.,23.));
#26715=CARTESIAN_POINT('',(126.82124193643,-33.8227565095591,25.4139334024237));
#26716=CARTESIAN_POINT('',(126.821241914321,-33.8227565692546,25.0733699431874));
#26717=CARTESIAN_POINT('',(126.821241915871,-33.8227565650715,23.));
#26718=CARTESIAN_POINT('Ctrl Pts',(126.821241914321,-33.8227565692547,25.0733699431874));
#26719=CARTESIAN_POINT('Ctrl Pts',(126.875893823826,-33.6751870906752,25.0637024941563));
#26720=CARTESIAN_POINT('Ctrl Pts',(126.940754520208,-33.5316051062762,25.0536068363797));
#26721=CARTESIAN_POINT('Ctrl Pts',(127.101016925518,-33.2339431825994,25.0318253550778));
#26722=CARTESIAN_POINT('Ctrl Pts',(127.199275152069,-33.0819255671996,25.0201687247304));
#26723=CARTESIAN_POINT('Ctrl Pts',(127.351719310163,-32.8829491129561,25.004479979221));
#26724=CARTESIAN_POINT('Ctrl Pts',(127.395957199737,-32.8287659827226,25.0001555604634));
#26725=CARTESIAN_POINT('Ctrl Pts',(127.477971830063,-32.7344291177899,24.9925360805312));
#26726=CARTESIAN_POINT('Ctrl Pts',(127.515110482934,-32.6937558387858,24.9892186467732));
#26727=CARTESIAN_POINT('Ctrl Pts',(127.5743647106,-32.6319561938971,24.9841245811721));
#26728=CARTESIAN_POINT('Ctrl Pts',(127.595801592221,-32.6101949593467,24.9823199540119));
#26729=CARTESIAN_POINT('Ctrl Pts',(127.636339655425,-32.5701411510711,24.9789767193885));
#26730=CARTESIAN_POINT('Ctrl Pts',(127.655366285614,-32.5517767556746,24.9774350589407));
#26731=CARTESIAN_POINT('Ctrl Pts',(127.698547872695,-32.5110632957582,24.9739960620206));
#26732=CARTESIAN_POINT('Ctrl Pts',(127.722817473349,-32.488839379671,24.9721040686612));
#26733=CARTESIAN_POINT('Ctrl Pts',(127.797803243295,-32.4221554057985,24.9663773758941));
#26734=CARTESIAN_POINT('Ctrl Pts',(127.849527337279,-32.3788511162025,24.962589296921));
#26735=CARTESIAN_POINT('Ctrl Pts',(128.138556389407,-32.1511899503183,24.9422015487431));
#26736=CARTESIAN_POINT('Ctrl Pts',(128.398253180408,-31.9974863518289,24.9267899944319));
#26737=CARTESIAN_POINT('Ctrl Pts',(128.73765046983,-31.853328512598,24.9068475310897));
#26738=CARTESIAN_POINT('Ctrl Pts',(128.801289414047,-31.8285398040028,24.90310930642));
#26739=CARTESIAN_POINT('Ctrl Pts',(128.908947636574,-31.7903079811134,24.8967216121689));
#26740=CARTESIAN_POINT('Ctrl Pts',(128.952571523532,-31.7758084303568,24.8941161392245));
#26741=CARTESIAN_POINT('Ctrl Pts',(129.015488887375,-31.7563077811375,24.8903162476382));
#26742=CARTESIAN_POINT('Ctrl Pts',(129.034554340259,-31.7505822093758,24.8891593123638));
#26743=CARTESIAN_POINT('Ctrl Pts',(129.068029895214,-31.7408497325236,24.8871165984788));
#26744=CARTESIAN_POINT('Ctrl Pts',(129.082417819552,-31.7367697486889,24.8862349176171));
#26745=CARTESIAN_POINT('Ctrl Pts',(129.114147808661,-31.7279985209001,24.8842819674329));
#26746=CARTESIAN_POINT('Ctrl Pts',(129.131500225542,-31.7233498975141,24.8832085020978));
#26747=CARTESIAN_POINT('Ctrl Pts',(129.183028443219,-31.7099838133465,24.8800064246755));
#26748=CARTESIAN_POINT('Ctrl Pts',(129.217303265452,-31.7016618359966,24.8778578175446));
#26749=CARTESIAN_POINT('Ctrl Pts',(129.429346921317,-31.6536683997751,24.8644762127533));
#26750=CARTESIAN_POINT('Ctrl Pts',(129.60993242284,-31.6278467096305,24.8527123825411));
#26751=CARTESIAN_POINT('Ctrl Pts',(129.952361894427,-31.6067648088782,24.830599611446));
#26752=CARTESIAN_POINT('Ctrl Pts',(130.113534106895,-31.6083289931502,24.8202714235265));
#26753=CARTESIAN_POINT('Ctrl Pts',(130.37047077841,-31.6291655068897,24.8041823743001));
#26754=CARTESIAN_POINT('Ctrl Pts',(130.466573076162,-31.6411183266721,24.7982465083586));
#26755=CARTESIAN_POINT('Ctrl Pts',(130.598976278609,-31.6633796476745,24.7901860889087));
#26756=CARTESIAN_POINT('Ctrl Pts',(130.635808668836,-31.6702018884951,24.7879563372232));
#26757=CARTESIAN_POINT('Ctrl Pts',(130.69901025272,-31.6829953075673,24.7841504652557));
#26758=CARTESIAN_POINT('Ctrl Pts',(130.725434415827,-31.6886739160363,24.7825653762343));
#26759=CARTESIAN_POINT('Ctrl Pts',(130.779424149527,-31.7009537286371,24.7793383136194));
#26760=CARTESIAN_POINT('Ctrl Pts',(130.806980541334,-31.7075858732133,24.7776974547774));
#26761=CARTESIAN_POINT('Ctrl Pts',(130.877402580308,-31.7254720023353,24.7735183119634));
#26762=CARTESIAN_POINT('Ctrl Pts',(130.920137270263,-31.7372225704428,24.7709958610612));
#26763=CARTESIAN_POINT('Ctrl Pts',(131.120039856985,-31.7964290345649,24.7592437544084));
#26764=CARTESIAN_POINT('Ctrl Pts',(131.273862044502,-31.8544253801053,24.7503533319201));
#26765=CARTESIAN_POINT('Ctrl Pts',(131.598557818831,-32.0045904945581,24.7312714924699));
#26766=CARTESIAN_POINT('Ctrl Pts',(131.766936535618,-32.1007253521701,24.7211695281631));
#26767=CARTESIAN_POINT('Ctrl Pts',(131.97405619726,-32.2437540348335,24.707461954135));
#26768=CARTESIAN_POINT('Ctrl Pts',(132.021067230905,-32.27803815241,24.7042548591645));
#26769=CARTESIAN_POINT('Ctrl Pts',(132.099657977262,-32.3385113590126,24.6986854124545));
#26770=CARTESIAN_POINT('Ctrl Pts',(132.131687867204,-32.3640956135696,24.696353762319));
#26771=CARTESIAN_POINT('Ctrl Pts',(132.177907122695,-32.4024072023963,24.6928845204022));
#26772=CARTESIAN_POINT('Ctrl Pts',(132.192466739078,-32.4146842865059,24.6917760069932));
#26773=CARTESIAN_POINT('Ctrl Pts',(132.218239271372,-32.4367906989044,24.6897840875354));
#26774=CARTESIAN_POINT('Ctrl Pts',(132.229491936485,-32.4465722892715,24.6889040128183));
#26775=CARTESIAN_POINT('Ctrl Pts',(132.254690087242,-32.4687698094187,24.6869095918574));
#26776=CARTESIAN_POINT('Ctrl Pts',(132.268597683253,-32.4812268495621,24.6857923943984));
#26777=CARTESIAN_POINT('Ctrl Pts',(132.311200168924,-32.5200249839481,24.6823210563346));
#26778=CARTESIAN_POINT('Ctrl Pts',(132.33954353939,-32.5467454166296,24.6799418583471));
#26779=CARTESIAN_POINT('Ctrl Pts',(132.522818156495,-32.7255905571389,24.6641284709953));
#26780=CARTESIAN_POINT('Ctrl Pts',(132.663279390932,-32.8918055326581,24.6499832656876));
#26781=CARTESIAN_POINT('Ctrl Pts',(132.901022739427,-33.2351546624578,24.6231467391655));
#26782=CARTESIAN_POINT('Ctrl Pts',(133.000333295119,-33.4098322665787,24.6104795577287));
#26783=CARTESIAN_POINT('Ctrl Pts',(133.102325110033,-33.6332479227907,24.595627456806));
#26784=CARTESIAN_POINT('Ctrl Pts',(133.120206079079,-33.6745768051963,24.592931450274));
#26785=CARTESIAN_POINT('Ctrl Pts',(133.148047433661,-33.7426162389387,24.5885744644279));
#26786=CARTESIAN_POINT('Ctrl Pts',(133.158503311044,-33.7691167905398,24.5868972443618));
#26787=CARTESIAN_POINT('Ctrl Pts',(133.178198952359,-33.8209398414679,24.5836546561143));
#26788=CARTESIAN_POINT('Ctrl Pts',(133.187473171261,-33.8462468711979,24.5820882523075));
#26789=CARTESIAN_POINT('Ctrl Pts',(133.208762993143,-33.9065583755539,24.5783941555274));
#26790=CARTESIAN_POINT('Ctrl Pts',(133.22050925611,-33.9416546801746,24.5762753221904));
#26791=CARTESIAN_POINT('Ctrl Pts',(133.258073864831,-34.0603148072602,24.5692081477171));
#26792=CARTESIAN_POINT('Ctrl Pts',(133.281233625542,-34.1446865133921,24.5643436643755));
#26793=CARTESIAN_POINT('Ctrl Pts',(133.363018642583,-34.4952495192453,24.5446347664032));
#26794=CARTESIAN_POINT('Ctrl Pts',(133.392701213385,-34.7671127671767,24.5306096205587));
#26795=CARTESIAN_POINT('Ctrl Pts',(133.388743834586,-35.1059422768452,24.512261459041));
#26796=CARTESIAN_POINT('Ctrl Pts',(133.386020594541,-35.1722561925368,24.5086240818133));
#26797=CARTESIAN_POINT('Ctrl Pts',(133.378184404678,-35.2833805420892,24.5023904569481));
#26798=CARTESIAN_POINT('Ctrl Pts',(133.374120284345,-35.328247328336,24.4998355034537));
#26799=CARTESIAN_POINT('Ctrl Pts',(133.366989895216,-35.3926503278033,24.4960964126159));
#26800=CARTESIAN_POINT('Ctrl Pts',(133.364644737093,-35.4122632493966,24.4949481309856));
#26801=CARTESIAN_POINT('Ctrl Pts',(133.360224512184,-35.4466761811227,24.4929147336864));
#26802=CARTESIAN_POINT('Ctrl Pts',(133.358222779718,-35.4614847046468,24.4920335796212));
#26803=CARTESIAN_POINT('Ctrl Pts',(133.353583152089,-35.4941779998795,24.4900742711456));
#26804=CARTESIAN_POINT('Ctrl Pts',(133.350900104469,-35.5120549883257,24.4889938144035));
#26805=CARTESIAN_POINT('Ctrl Pts',(133.342470802727,-35.5653130324419,24.4857495627475));
#26806=CARTESIAN_POINT('Ctrl Pts',(133.336306366831,-35.600624256997,24.4835650157044));
#26807=CARTESIAN_POINT('Ctrl Pts',(133.298062712453,-35.8008908889849,24.4710090214047));
#26808=CARTESIAN_POINT('Ctrl Pts',(133.254313802097,-35.9633675392982,24.4601891807129));
#26809=CARTESIAN_POINT('Ctrl Pts',(133.143508726153,-36.2792846214322,24.4386090022506));
#26810=CARTESIAN_POINT('Ctrl Pts',(133.076771357625,-36.4323764362759,24.4278799010688));
#26811=CARTESIAN_POINT('Ctrl Pts',(132.966652538034,-36.6414029314021,24.4130971627072));
#26812=CARTESIAN_POINT('Ctrl Pts',(132.932390765654,-36.7018567028678,24.408802411961));
#26813=CARTESIAN_POINT('Ctrl Pts',(132.867823011802,-36.8080372920871,24.4012290523111));
#26814=CARTESIAN_POINT('Ctrl Pts',(132.83822028184,-36.854161220482,24.3979284696695));
#26815=CARTESIAN_POINT('Ctrl Pts',(132.790425001181,-36.9248020701622,24.3928542677881));
#26816=CARTESIAN_POINT('Ctrl Pts',(132.77299872563,-36.9498238010583,24.3910530048198));
#26817=CARTESIAN_POINT('Ctrl Pts',(132.739830679199,-36.9961042974664,24.3877128970109));
#26818=CARTESIAN_POINT('Ctrl Pts',(132.724173212354,-37.0174203539709,24.3861710478909));
#26819=CARTESIAN_POINT('Ctrl Pts',(132.688433988152,-37.0649008242302,24.3827276787155));
#26820=CARTESIAN_POINT('Ctrl Pts',(132.668216474972,-37.0909599887926,24.3808315648287));
#26821=CARTESIAN_POINT('Ctrl Pts',(132.60524933025,-37.169720102317,24.3750775487913));
#26822=CARTESIAN_POINT('Ctrl Pts',(132.561293723805,-37.2214375316467,24.3712669486538));
#26823=CARTESIAN_POINT('Ctrl Pts',(132.347635325388,-37.4580445608414,24.3536058901353));
#26824=CARTESIAN_POINT('Ctrl Pts',(132.159302421337,-37.6250318853284,24.3405293951551));
#26825=CARTESIAN_POINT('Ctrl Pts',(131.835327009499,-37.853623356693,24.319380312681));
#26826=CARTESIAN_POINT('Ctrl Pts',(131.711126149247,-37.9297832738017,24.3115164386881));
#26827=CARTESIAN_POINT('Ctrl Pts',(131.557593852507,-38.010829658664,24.3016273679988));
#26828=CARTESIAN_POINT('Ctrl Pts',(131.532595599175,-38.0236310065254,24.3000120262671));
#26829=CARTESIAN_POINT('Ctrl Pts',(131.492683211789,-38.0434476193215,24.2974202679454));
#26830=CARTESIAN_POINT('Ctrl Pts',(131.477871480686,-38.0506675407377,24.2964557133605));
#26831=CARTESIAN_POINT('Ctrl Pts',(131.449285421754,-38.0643446684004,24.2945878106088));
#26832=CARTESIAN_POINT('Ctrl Pts',(131.435519313781,-38.0708176024146,24.293685405137));
#26833=CARTESIAN_POINT('Ctrl Pts',(131.401050533551,-38.0867426863635,24.2914194736652));
#26834=CARTESIAN_POINT('Ctrl Pts',(131.380295537576,-38.096079323376,24.290049366698));
#26835=CARTESIAN_POINT('Ctrl Pts',(131.303481589911,-38.1297082112448,24.2849619131463));
#26836=CARTESIAN_POINT('Ctrl Pts',(131.246865642598,-38.1526913697427,24.2811797928546));
#26837=CARTESIAN_POINT('Ctrl Pts',(131.005648120923,-38.2430996373723,24.2650188323532));
#26838=CARTESIAN_POINT('Ctrl Pts',(130.815989725741,-38.295934006517,24.2522227774963));
#26839=CARTESIAN_POINT('Ctrl Pts',(130.436596013824,-38.3668506153915,24.22746015288));
#26840=CARTESIAN_POINT('Ctrl Pts',(130.247752227897,-38.3859911698679,24.2155250057647));
#26841=CARTESIAN_POINT('Ctrl Pts',(130.013594167302,-38.3900172877107,24.2013666171102));
#26842=CARTESIAN_POINT('Ctrl Pts',(129.968901205641,-38.3899019400603,24.1986914613154));
#26843=CARTESIAN_POINT('Ctrl Pts',(129.895811383336,-38.3882676041646,24.194359290837));
#26844=CARTESIAN_POINT('Ctrl Pts',(129.867409328543,-38.3872750718854,24.19268638746));
#26845=CARTESIAN_POINT('Ctrl Pts',(129.812067007864,-38.3846439238437,24.1894462423995));
#26846=CARTESIAN_POINT('Ctrl Pts',(129.78512728165,-38.383040507796,24.1878780440071));
#26847=CARTESIAN_POINT('Ctrl Pts',(129.721087736956,-38.3784608990628,24.1841703699146));
#26848=CARTESIAN_POINT('Ctrl Pts',(129.684011738647,-38.3751950566755,24.1820399390979));
#26849=CARTESIAN_POINT('Ctrl Pts',(129.558351692207,-38.3620374467854,24.1748675314108));
#26850=CARTESIAN_POINT('Ctrl Pts',(129.470103729425,-38.3492627171622,24.1699131452475));
#26851=CARTESIAN_POINT('Ctrl Pts',(129.116415008417,-38.2837311780441,24.1502346186156));
#26852=CARTESIAN_POINT('Ctrl Pts',(128.857250454102,-38.2027686380154,24.136305727162));
#26853=CARTESIAN_POINT('Ctrl Pts',(128.550083629725,-38.0647236722473,24.1180690686392));
#26854=CARTESIAN_POINT('Ctrl Pts',(128.490504203096,-38.035821179182,24.114439550148));
#26855=CARTESIAN_POINT('Ctrl Pts',(128.391938754509,-37.9843871964846,24.1082179562922));
#26856=CARTESIAN_POINT('Ctrl Pts',(128.352485094035,-37.9627895879264,24.105666967951));
#26857=CARTESIAN_POINT('Ctrl Pts',(128.296350961136,-37.9305928932128,24.101932653028));
#26858=CARTESIAN_POINT('Ctrl Pts',(128.279313696641,-37.9206220840956,24.1007850558861));
#26859=CARTESIAN_POINT('Ctrl Pts',(128.249534572845,-37.9028432863217,24.0987523915376));
#26860=CARTESIAN_POINT('Ctrl Pts',(128.236755746736,-37.8950989702657,24.0978712751555));
#26861=CARTESIAN_POINT('Ctrl Pts',(128.208622689531,-37.8777942101719,24.0959114462088));
#26862=CARTESIAN_POINT('Ctrl Pts',(128.193293694891,-37.8681953349207,24.094830422724));
#26863=CARTESIAN_POINT('Ctrl Pts',(128.148705998996,-37.8397756721785,24.0916490542294));
#26864=CARTESIAN_POINT('Ctrl Pts',(128.119660164121,-37.8206271015588,24.0895295815972));
#26865=CARTESIAN_POINT('Ctrl Pts',(127.938696991767,-37.6972891528411,24.0760509020725));
#26866=CARTESIAN_POINT('Ctrl Pts',(127.795199817523,-37.5813146465733,24.064147854628));
#26867=CARTESIAN_POINT('Ctrl Pts',(127.546280292757,-37.344171767919,24.0419897502178));
#26868=CARTESIAN_POINT('Ctrl Pts',(127.438627527818,-37.2260414121756,24.0317521288504));
#26869=CARTESIAN_POINT('Ctrl Pts',(127.279996660215,-37.0251581944908,24.0157797971023));
#26870=CARTESIAN_POINT('Ctrl Pts',(127.223545049045,-36.9470450692669,24.0098734487436));
#26871=CARTESIAN_POINT('Ctrl Pts',(127.149901694267,-36.835413580024,24.0018452035483));
#26872=CARTESIAN_POINT('Ctrl Pts',(127.129827417018,-36.8038605472737,23.9996192278667));
#26873=CARTESIAN_POINT('Ctrl Pts',(127.096156422575,-36.7489503658316,23.9958177452791));
#26874=CARTESIAN_POINT('Ctrl Pts',(127.082309647367,-36.7257514228154,23.9942333238592));
#26875=CARTESIAN_POINT('Ctrl Pts',(127.054498125793,-36.6778641500091,23.9910058591832));
#26876=CARTESIAN_POINT('Ctrl Pts',(127.040562909077,-36.6531610849346,23.9893639531585));
#26877=CARTESIAN_POINT('Ctrl Pts',(127.005606757017,-36.5893351944016,23.9851784729584));
#26878=CARTESIAN_POINT('Ctrl Pts',(126.985041316327,-36.5499682727796,23.9826508294941));
#26879=CARTESIAN_POINT('Ctrl Pts',(126.890676103926,-36.3603423899407,23.9707124635746));
#26880=CARTESIAN_POINT('Ctrl Pts',(126.827297129446,-36.2051519913493,23.9616560414043));
#26881=CARTESIAN_POINT('Ctrl Pts',(126.716772248405,-35.8644194912719,23.9425605862669));
#26882=CARTESIAN_POINT('Ctrl Pts',(126.673334495947,-35.678303230035,23.9325962202296));
#26883=CARTESIAN_POINT('Ctrl Pts',(126.633472967456,-35.4051767320333,23.9175602303984));
#26884=CARTESIAN_POINT('Ctrl Pts',(126.624349200229,-35.3203933316099,23.9128332486971));
#26885=CARTESIAN_POINT('Ctrl Pts',(126.616713742662,-35.2106912823588,23.906540464242));
#26886=CARTESIAN_POINT('Ctrl Pts',(126.6152666468,-35.1860020620336,23.9051127202299));
#26887=CARTESIAN_POINT('Ctrl Pts',(126.613340081839,-35.1455607975624,23.902752056321));
#26888=CARTESIAN_POINT('Ctrl Pts',(126.612700055594,-35.1298168536005,23.9018275870525));
#26889=CARTESIAN_POINT('Ctrl Pts',(126.61169766522,-35.1000461078001,23.9000682245249));
#26890=CARTESIAN_POINT('Ctrl Pts',(126.611312582627,-35.0860203886457,23.8992346436669));
#26891=CARTESIAN_POINT('Ctrl Pts',(126.610508419963,-35.0481653627905,23.8969728779139));
#26892=CARTESIAN_POINT('Ctrl Pts',(126.610253568687,-35.0243338132724,23.8955362101897));
#26893=CARTESIAN_POINT('Ctrl Pts',(126.610238801731,-34.924681597953,23.8894808002329));
#26894=CARTESIAN_POINT('Ctrl Pts',(126.612771476117,-34.8488871420349,23.8847594083724));
#26895=CARTESIAN_POINT('Ctrl Pts',(126.627938209812,-34.6226659146988,23.870439178431));
#26896=CARTESIAN_POINT('Ctrl Pts',(126.64807845332,-34.4729315193651,23.8606648240289));
#26897=CARTESIAN_POINT('Ctrl Pts',(126.712848075336,-34.154161297163,23.8397259590213));
#26898=CARTESIAN_POINT('Ctrl Pts',(126.760697730583,-33.9862362059936,23.8286213181425));
#26899=CARTESIAN_POINT('Ctrl Pts',(126.821241884814,-33.8227566489294,23.8178897147877));
#26900=CARTESIAN_POINT('',(126.610251398414,-35.0029526077136,24.2343658980132));
#26901=CARTESIAN_POINT('Ctrl Pts',(126.821241975209,-33.8227564048483,24.1659080048185));
#26902=CARTESIAN_POINT('Ctrl Pts',(126.807344274267,-33.8602825622005,24.168379675193));
#26903=CARTESIAN_POINT('Ctrl Pts',(126.794107430046,-33.8980646848755,24.1708330162916));
#26904=CARTESIAN_POINT('Ctrl Pts',(126.765504500368,-33.984591761951,24.1763714619477));
#26905=CARTESIAN_POINT('Ctrl Pts',(126.750567979835,-34.0334561579263,24.1794422012933));
#26906=CARTESIAN_POINT('Ctrl Pts',(126.728693599679,-34.1112684560801,24.1842446403351));
#26907=CARTESIAN_POINT('Ctrl Pts',(126.721022952137,-34.1400006244833,24.1859993724584));
#26908=CARTESIAN_POINT('Ctrl Pts',(126.707220319802,-34.1945733341013,24.18929825462));
#26909=CARTESIAN_POINT('Ctrl Pts',(126.701012019139,-34.2203920872161,24.1908447176221));
#26910=CARTESIAN_POINT('Ctrl Pts',(126.687513281788,-34.2795811411885,24.1943586620257));
#26911=CARTESIAN_POINT('Ctrl Pts',(126.68042248472,-34.3129943001812,24.1963197433085));
#26912=CARTESIAN_POINT('Ctrl Pts',(126.666629190672,-34.3831999981619,24.200396128665));
#26913=CARTESIAN_POINT('Ctrl Pts',(126.660028074952,-34.4200078597816,24.2025081495119));
#26914=CARTESIAN_POINT('Ctrl Pts',(126.624735767856,-34.6374461818767,24.2148510598649));
#26915=CARTESIAN_POINT('Ctrl Pts',(126.610091916046,-34.8200503077089,24.2246539376064));
#26916=CARTESIAN_POINT('Ctrl Pts',(126.610251286801,-35.0029536196393,24.2343661467437));
#26917=CARTESIAN_POINT('Ctrl Pts',(126.610251285911,-35.0029525974854,24.2343660924671));
#26918=CARTESIAN_POINT('Ctrl Pts',(126.610436908779,-35.2160581364856,24.2456820473744));
#26919=CARTESIAN_POINT('Ctrl Pts',(126.630718128161,-35.4286581131638,24.256828764692));
#26920=CARTESIAN_POINT('Ctrl Pts',(126.679338029607,-35.6823917574262,24.2712824344637));
#26921=CARTESIAN_POINT('Ctrl Pts',(126.688746957028,-35.7266755192801,24.2738495722609));
#26922=CARTESIAN_POINT('Ctrl Pts',(126.703539186111,-35.790027097529,24.2776033371392));
#26923=CARTESIAN_POINT('Ctrl Pts',(126.70820759982,-35.809258589989,24.2787537191822));
#26924=CARTESIAN_POINT('Ctrl Pts',(126.716696964117,-35.8429410666196,24.2807893716379));
#26925=CARTESIAN_POINT('Ctrl Pts',(126.720445514594,-35.8574093727653,24.2816706474096));
#26926=CARTESIAN_POINT('Ctrl Pts',(126.728932152827,-35.8892952204943,24.283628383695));
#26927=CARTESIAN_POINT('Ctrl Pts',(126.733713681397,-35.9066997864303,24.2847071204101));
#26928=CARTESIAN_POINT('Ctrl Pts',(126.748366571423,-35.9584152443109,24.2879409581653));
#26929=CARTESIAN_POINT('Ctrl Pts',(126.758640964347,-35.9926082401722,24.2901166231013));
#26930=CARTESIAN_POINT('Ctrl Pts',(126.813623987023,-36.1656258332153,24.3012952896008));
#26931=CARTESIAN_POINT('Ctrl Pts',(126.866715971581,-36.3016144375825,24.310634954532));
#26932=CARTESIAN_POINT('Ctrl Pts',(127.007142546088,-36.6024585349234,24.33201609475));
#26933=CARTESIAN_POINT('Ctrl Pts',(127.09966384379,-36.7644062583769,24.3440425930186));
#26934=CARTESIAN_POINT('Ctrl Pts',(127.245174344422,-36.9764555324361,24.3601500718101));
#26935=CARTESIAN_POINT('Ctrl Pts',(127.287155274596,-37.0336950100936,24.3645411782755));
#26936=CARTESIAN_POINT('Ctrl Pts',(127.365224917559,-37.1334162901762,24.3722641494602));
#26937=CARTESIAN_POINT('Ctrl Pts',(127.400621643439,-37.1764047211051,24.3756192960652));
#26938=CARTESIAN_POINT('Ctrl Pts',(127.4571331044,-37.2416898593376,24.3807577874005));
#26939=CARTESIAN_POINT('Ctrl Pts',(127.477517480785,-37.2646031676762,24.3825699209641));
#26940=CARTESIAN_POINT('Ctrl Pts',(127.516045575909,-37.3067453557586,24.3859201979737));
#26941=CARTESIAN_POINT('Ctrl Pts',(127.5341085714,-37.3260445477324,24.3874615025292));
#26942=CARTESIAN_POINT('Ctrl Pts',(127.575048705052,-37.368773608732,24.3908910641822));
#26943=CARTESIAN_POINT('Ctrl Pts',(127.598043483406,-37.3920874131044,24.3927741151482));
#26944=CARTESIAN_POINT('Ctrl Pts',(127.668784765945,-37.4617613650883,24.3984418093849));
#26945=CARTESIAN_POINT('Ctrl Pts',(127.717563220923,-37.5070533783992,24.4021812866695));
#26946=CARTESIAN_POINT('Ctrl Pts',(127.994709762611,-37.7495927033872,24.4226007048005));
#26947=CARTESIAN_POINT('Ctrl Pts',(128.247267861713,-37.9170822870038,24.438074685957));
#26948=CARTESIAN_POINT('Ctrl Pts',(128.580138633457,-38.0788101621423,24.4580884341411));
#26949=CARTESIAN_POINT('Ctrl Pts',(128.642513248589,-38.1068162304265,24.4618306913904));
#26950=CARTESIAN_POINT('Ctrl Pts',(128.748207332888,-38.1504819626931,24.4682245354235));
#26951=CARTESIAN_POINT('Ctrl Pts',(128.791077272663,-38.1671796432037,24.4708320158464));
#26952=CARTESIAN_POINT('Ctrl Pts',(128.852969817343,-38.1898469155771,24.4746343234939));
#26953=CARTESIAN_POINT('Ctrl Pts',(128.871727626187,-38.1965298361735,24.4757916019916));
#26954=CARTESIAN_POINT('Ctrl Pts',(128.904675415796,-38.2079421462605,24.4778346895675));
#26955=CARTESIAN_POINT('Ctrl Pts',(128.918839524934,-38.2127434965227,24.4787163955311));
#26956=CARTESIAN_POINT('Ctrl Pts',(128.950082689076,-38.2231042910342,24.4806691102535));
#26957=CARTESIAN_POINT('Ctrl Pts',(128.967174210528,-38.2286217628435,24.4817423109499));
#26958=CARTESIAN_POINT('Ctrl Pts',(129.017936985997,-38.2445646445416,24.4849427891844));
#26959=CARTESIAN_POINT('Ctrl Pts',(129.051726924969,-38.2546006607534,24.4870900332582));
#26960=CARTESIAN_POINT('Ctrl Pts',(129.260748089142,-38.3131511867445,24.5004504183648));
#26961=CARTESIAN_POINT('Ctrl Pts',(129.439479775454,-38.3480250414412,24.5121927155569));
#26962=CARTESIAN_POINT('Ctrl Pts',(129.780321718107,-38.3864633883233,24.5343008154518));
#26963=CARTESIAN_POINT('Ctrl Pts',(129.941610093308,-38.393079903419,24.5446453280976));
#26964=CARTESIAN_POINT('Ctrl Pts',(130.199598421458,-38.3852548527202,24.5607553870761));
#26965=CARTESIAN_POINT('Ctrl Pts',(130.296265384888,-38.3781680730078,24.5666965482075));
#26966=CARTESIAN_POINT('Ctrl Pts',(130.429717795511,-38.3626108013519,24.5747627404839));
#26967=CARTESIAN_POINT('Ctrl Pts',(130.466858644995,-38.3576557238271,24.5769931711046));
#26968=CARTESIAN_POINT('Ctrl Pts',(130.530638399757,-38.3480678690337,24.5807998359523));
#26969=CARTESIAN_POINT('Ctrl Pts',(130.557317476455,-38.3437303809341,24.582385048631));
#26970=CARTESIAN_POINT('Ctrl Pts',(130.611856980228,-38.3341924288818,24.5856120503617));
#26971=CARTESIAN_POINT('Ctrl Pts',(130.639709824671,-38.328960727939,24.5872527286439));
#26972=CARTESIAN_POINT('Ctrl Pts',(130.710925686642,-38.3146571614297,24.5914307620992));
#26973=CARTESIAN_POINT('Ctrl Pts',(130.754183103735,-38.3050832865524,24.5939523013676));
#26974=CARTESIAN_POINT('Ctrl Pts',(130.956302146785,-38.2561745746636,24.60567449531));
#26975=CARTESIAN_POINT('Ctrl Pts',(131.112374188894,-38.2062155656347,24.6145382953326));
#26976=CARTESIAN_POINT('Ctrl Pts',(131.444234180228,-38.0728204255457,24.6336181954355));
#26977=CARTESIAN_POINT('Ctrl Pts',(131.617675828643,-37.9851558799842,24.643742371876));
#26978=CARTESIAN_POINT('Ctrl Pts',(131.855722522548,-37.837970750278,24.6589832866789));
#26979=CARTESIAN_POINT('Ctrl Pts',(131.927036456209,-37.7900380419107,24.6637449353574));
#26980=CARTESIAN_POINT('Ctrl Pts',(132.01648080816,-37.724853153555,24.6700777814639));
#26981=CARTESIAN_POINT('Ctrl Pts',(132.036352872599,-37.7100344019353,24.6715087414383));
#26982=CARTESIAN_POINT('Ctrl Pts',(132.068597202239,-37.6854346659395,24.6738733484276));
#26983=CARTESIAN_POINT('Ctrl Pts',(132.081067271454,-37.6757826374976,24.6747984894508));
#26984=CARTESIAN_POINT('Ctrl Pts',(132.104497549176,-37.6573843796994,24.6765579523125));
#26985=CARTESIAN_POINT('Ctrl Pts',(132.115471735024,-37.6486564516115,24.6773909484308));
#26986=CARTESIAN_POINT('Ctrl Pts',(132.144912126016,-37.624942402806,24.6796490180205));
#26987=CARTESIAN_POINT('Ctrl Pts',(132.163274940736,-37.6098299000797,24.6810825273098));
#26988=CARTESIAN_POINT('Ctrl Pts',(132.23430205968,-37.5501103188006,24.6867209725807));
#26989=CARTESIAN_POINT('Ctrl Pts',(132.285755218997,-37.5040946695482,24.6910092465469));
#26990=CARTESIAN_POINT('Ctrl Pts',(132.490152603477,-37.3097467928741,24.7087768763713));
#26991=CARTESIAN_POINT('Ctrl Pts',(132.630356267499,-37.1487244476289,24.7226868440036));
#26992=CARTESIAN_POINT('Ctrl Pts',(132.818737611109,-36.886071096317,24.7433266411604));
#26993=CARTESIAN_POINT('Ctrl Pts',(132.878555831865,-36.7934507277802,24.7502762127446));
#26994=CARTESIAN_POINT('Ctrl Pts',(132.971973488392,-36.6320532235835,24.761795943397));
#26995=CARTESIAN_POINT('Ctrl Pts',(133.007949488169,-36.5647572969367,24.7664376519188));
#26996=CARTESIAN_POINT('Ctrl Pts',(133.056823734463,-36.4654074726031,24.7730615990404));
#26997=CARTESIAN_POINT('Ctrl Pts',(133.071550122843,-36.4342839253048,24.7751052801298));
#26998=CARTESIAN_POINT('Ctrl Pts',(133.096802757864,-36.3787401695698,24.7786984590859));
#26999=CARTESIAN_POINT('Ctrl Pts',(133.10752046497,-36.354410719046,24.7802543177324));
#27000=CARTESIAN_POINT('Ctrl Pts',(133.129558762794,-36.302744142241,24.7835214811389));
#27001=CARTESIAN_POINT('Ctrl Pts',(133.140809930037,-36.2753797134425,24.785230367012));
#27002=CARTESIAN_POINT('Ctrl Pts',(133.170237565398,-36.201055413356,24.789816358468));
#27003=CARTESIAN_POINT('Ctrl Pts',(133.187728689355,-36.1538312258618,24.7926709342583));
#27004=CARTESIAN_POINT('Ctrl Pts',(133.288341765249,-35.8624092958261,24.809961079061));
#27005=CARTESIAN_POINT('Ctrl Pts',(133.344416872628,-35.6097770377765,24.8234833202264));
#27006=CARTESIAN_POINT('Ctrl Pts',(133.383194451374,-35.2396592722044,24.843261552494));
#27007=CARTESIAN_POINT('Ctrl Pts',(133.389346167686,-35.1255821806748,24.8493672058927));
#27008=CARTESIAN_POINT('Ctrl Pts',(133.389948327781,-34.9468387208198,24.8592218536625));
#27009=CARTESIAN_POINT('Ctrl Pts',(133.38832025085,-34.8822689723597,24.8628410605483));
#27010=CARTESIAN_POINT('Ctrl Pts',(133.383635962622,-34.7952509000251,24.8678444621272));
#27011=CARTESIAN_POINT('Ctrl Pts',(133.382197634648,-34.7727256666619,24.8691510549399));
#27012=CARTESIAN_POINT('Ctrl Pts',(133.379404898653,-34.7349290769522,24.8713651491035));
#27013=CARTESIAN_POINT('Ctrl Pts',(133.378171607038,-34.719649058839,24.8722662164328));
#27014=CARTESIAN_POINT('Ctrl Pts',(133.37538729903,-34.6878444364612,24.8741550497788));
#27015=CARTESIAN_POINT('Ctrl Pts',(133.373818514529,-34.6713221640996,24.8751436708627));
#27016=CARTESIAN_POINT('Ctrl Pts',(133.369211997512,-34.6263212130996,24.8778552538438));
#27017=CARTESIAN_POINT('Ctrl Pts',(133.365934628095,-34.5978690739955,24.8795903544918));
#27018=CARTESIAN_POINT('Ctrl Pts',(133.341066605702,-34.4036612151039,24.8915599551861));
#27019=CARTESIAN_POINT('Ctrl Pts',(133.307602806705,-34.2396713050136,24.9022858505088));
#27020=CARTESIAN_POINT('Ctrl Pts',(133.225082045367,-33.94743475074,24.921852633121));
#27021=CARTESIAN_POINT('Ctrl Pts',(133.180070812314,-33.8183907355127,24.9306636078335));
#27022=CARTESIAN_POINT('Ctrl Pts',(133.074268950022,-33.5653417371081,24.9480500195027));
#27023=CARTESIAN_POINT('Ctrl Pts',(133.013441517617,-33.4416189047824,24.9566063656474));
#27024=CARTESIAN_POINT('Ctrl Pts',(132.924580152183,-33.2856549758569,24.9674294865618));
#27025=CARTESIAN_POINT('Ctrl Pts',(132.903244286699,-33.2497655089816,24.9699234195639));
#27026=CARTESIAN_POINT('Ctrl Pts',(132.866592293773,-33.1906277679722,24.9740401973353));
#27027=CARTESIAN_POINT('Ctrl Pts',(132.851643500477,-33.1671583080248,24.9756759810408));
#27028=CARTESIAN_POINT('Ctrl Pts',(132.821594120495,-33.1212388382192,24.9788814389872));
#27029=CARTESIAN_POINT('Ctrl Pts',(132.806510407494,-33.0987803181955,24.9804515695561));
#27030=CARTESIAN_POINT('Ctrl Pts',(132.772485110212,-33.0494066604086,24.9839100793754));
#27031=CARTESIAN_POINT('Ctrl Pts',(132.753417030398,-33.0225817775156,24.9857935849184));
#27032=CARTESIAN_POINT('Ctrl Pts',(132.684874284082,-32.9290704242584,24.9923802708236));
#27033=CARTESIAN_POINT('Ctrl Pts',(132.633341511965,-32.8639257547196,24.9970059992321));
#27034=CARTESIAN_POINT('Ctrl Pts',(132.399444397277,-32.5895933458376,25.016784667415));
#27035=CARTESIAN_POINT('Ctrl Pts',(132.194194887457,-32.4013671084972,25.0310555234053));
#27036=CARTESIAN_POINT('Ctrl Pts',(131.913981377329,-32.2015122943597,25.0496878314616));
#27037=CARTESIAN_POINT('Ctrl Pts',(131.858522721635,-32.1643782775739,25.0533447439061));
#27038=CARTESIAN_POINT('Ctrl Pts',(131.763700145047,-32.1048640154398,25.0596082609953));
#27039=CARTESIAN_POINT('Ctrl Pts',(131.72491749436,-32.0815912208658,25.0621730545131));
#27040=CARTESIAN_POINT('Ctrl Pts',(131.668519435158,-32.0492646132009,25.0659239968495));
#27041=CARTESIAN_POINT('Ctrl Pts',(131.651270674401,-32.0395774714856,25.0670739757018));
#27042=CARTESIAN_POINT('Ctrl Pts',(131.620843336266,-32.0228377050667,25.0691091952802));
#27043=CARTESIAN_POINT('Ctrl Pts',(131.607701369389,-32.0157203974954,25.0699904477118));
#27044=CARTESIAN_POINT('Ctrl Pts',(131.578579657438,-32.0001971218945,25.0719484855451));
#27045=CARTESIAN_POINT('Ctrl Pts',(131.562579757073,-31.9918318675765,25.0730275521562));
#27046=CARTESIAN_POINT('Ctrl Pts',(131.515691762351,-31.9677923402809,25.0761976641346));
#27047=CARTESIAN_POINT('Ctrl Pts',(131.484630182155,-31.9524636453704,25.0783076441454));
#27048=CARTESIAN_POINT('Ctrl Pts',(131.284132859435,-31.8573120526994,25.0919648560047));
#27049=CARTESIAN_POINT('Ctrl Pts',(131.108573072493,-31.7911776983037,25.1040752045084));
#27050=CARTESIAN_POINT('Ctrl Pts',(130.776820086821,-31.6966960226035,25.1263051174737));
#27051=CARTESIAN_POINT('Ctrl Pts',(130.622334867936,-31.6641382866081,25.1364127535991));
#27052=CARTESIAN_POINT('Ctrl Pts',(130.371391545657,-31.6292994034178,25.152217049404));
#27053=CARTESIAN_POINT('Ctrl Pts',(130.276128787727,-31.6201612841146,25.1580805728196));
#27054=CARTESIAN_POINT('Ctrl Pts',(130.143348421782,-31.6130769276361,25.1660620960981));
#27055=CARTESIAN_POINT('Ctrl Pts',(130.106065846671,-31.6117044297849,25.1682825608067));
#27056=CARTESIAN_POINT('Ctrl Pts',(130.041771982493,-31.6103998468723,25.1720776447012));
#27057=CARTESIAN_POINT('Ctrl Pts',(130.01477076835,-31.610174638156,25.1736610993292));
#27058=CARTESIAN_POINT('Ctrl Pts',(129.959379982093,-31.610374499745,25.1768891850223));
#27059=CARTESIAN_POINT('Ctrl Pts',(129.930992620713,-31.610833572886,25.1785326457682));
#27060=CARTESIAN_POINT('Ctrl Pts',(129.858083340608,-31.6129290946049,25.1827275098656));
#27061=CARTESIAN_POINT('Ctrl Pts',(129.813581149839,-31.6150867177881,25.1852628376556));
#27062=CARTESIAN_POINT('Ctrl Pts',(129.596223322366,-31.629924850698,25.1975409740153));
#27063=CARTESIAN_POINT('Ctrl Pts',(129.424465534204,-31.6549721786094,25.2069008791239));
#27064=CARTESIAN_POINT('Ctrl Pts',(129.098110558649,-31.7284587366632,25.2247156401648));
#27065=CARTESIAN_POINT('Ctrl Pts',(128.943590608699,-31.7750375258261,25.2331693424943));
#27066=CARTESIAN_POINT('Ctrl Pts',(128.726189794318,-31.8578795882111,25.2457275605851));
#27067=CARTESIAN_POINT('Ctrl Pts',(128.660228530845,-31.8854335000244,25.2496323604552));
#27068=CARTESIAN_POINT('Ctrl Pts',(128.551996450094,-31.9347196780033,25.2562732651985));
#27069=CARTESIAN_POINT('Ctrl Pts',(128.509221941368,-31.9552934379189,25.2589607293781));
#27070=CARTESIAN_POINT('Ctrl Pts',(128.448922566152,-31.9858716083388,25.2628591117792));
#27071=CARTESIAN_POINT('Ctrl Pts',(128.431031519794,-31.995145755242,25.2640298306471));
#27072=CARTESIAN_POINT('Ctrl Pts',(128.399989054328,-32.0115899916525,25.2660875674119));
#27073=CARTESIAN_POINT('Ctrl Pts',(128.386800772914,-32.018688602625,25.2669702711297));
#27074=CARTESIAN_POINT('Ctrl Pts',(128.35804650642,-32.0344122935125,25.2689139020258));
#27075=CARTESIAN_POINT('Ctrl Pts',(128.342501352489,-32.0430725537307,25.2699768640977));
#27076=CARTESIAN_POINT('Ctrl Pts',(128.297975204728,-32.0683396623369,25.273055167941));
#27077=CARTESIAN_POINT('Ctrl Pts',(128.269171318839,-32.0852525606394,25.275087904618));
#27078=CARTESIAN_POINT('Ctrl Pts',(128.024560012043,-32.2337862826416,25.2926777341158));
#27079=CARTESIAN_POINT('Ctrl Pts',(127.823859975425,-32.388734247844,25.3092496628992));
#27080=CARTESIAN_POINT('Ctrl Pts',(127.558345411499,-32.6457766427049,25.3328979198023));
#27081=CARTESIAN_POINT('Ctrl Pts',(127.478684074648,-32.731296726382,25.3402832421547));
#27082=CARTESIAN_POINT('Ctrl Pts',(127.352597774039,-32.8815198785215,25.3524186652358));
#27083=CARTESIAN_POINT('Ctrl Pts',(127.30374974135,-32.9440494506282,25.357251122086));
#27084=CARTESIAN_POINT('Ctrl Pts',(127.23661886655,-33.0364956829248,25.3640902712282));
#27085=CARTESIAN_POINT('Ctrl Pts',(127.216537573947,-33.0650680757396,25.3661641698332));
#27086=CARTESIAN_POINT('Ctrl Pts',(127.181918826337,-33.1159794398359,25.3697912596576));
#27087=CARTESIAN_POINT('Ctrl Pts',(127.167196842172,-33.1381887040619,25.3713512277966));
#27088=CARTESIAN_POINT('Ctrl Pts',(127.136820122179,-33.1852089601518,25.3746084524684));
#27089=CARTESIAN_POINT('Ctrl Pts',(127.121222471287,-33.2100543166143,25.3763035354955));
#27090=CARTESIAN_POINT('Ctrl Pts',(127.080368775087,-33.277045452513,25.3808072147052));
#27091=CARTESIAN_POINT('Ctrl Pts',(127.05570273539,-33.3195438646867,25.3835947092113));
#27092=CARTESIAN_POINT('Ctrl Pts',(126.95028996597,-33.5106161476536,25.3958450224807));
#27093=CARTESIAN_POINT('Ctrl Pts',(126.879871394148,-33.6644469814127,25.4049493855538));
#27094=CARTESIAN_POINT('Ctrl Pts',(126.82124193643,-33.822756509559,25.4139334024237));
#27095=CARTESIAN_POINT('Origin',(130.,-35.,23.));
#27096=CARTESIAN_POINT('',(126.821241917671,-33.8227565602112,26.6607167036746));
#27097=CARTESIAN_POINT('',(126.821241846765,-33.8227567516686,26.3195780637354));
#27098=CARTESIAN_POINT('',(126.821241915871,-33.8227565650715,23.));
#27099=CARTESIAN_POINT('',(126.61025105039,-34.9973314581693,25.1397298775655));
#27100=CARTESIAN_POINT('Ctrl Pts',(126.821241846765,-33.8227567516686,26.3195780637354));
#27101=CARTESIAN_POINT('Ctrl Pts',(126.872641896856,-33.6839678237783,26.3116709482775));
#27102=CARTESIAN_POINT('Ctrl Pts',(126.933097475216,-33.5486368529399,26.3038949810359));
#27103=CARTESIAN_POINT('Ctrl Pts',(127.064470118871,-33.2997532174182,26.2888430489513));
#27104=CARTESIAN_POINT('Ctrl Pts',(127.13359097118,-33.1856496796866,26.2816081180484));
#27105=CARTESIAN_POINT('Ctrl Pts',(127.225173164613,-33.0528151267007,26.2724174983671));
#27106=CARTESIAN_POINT('Ctrl Pts',(127.241391093988,-33.0299061716714,26.2708030971816));
#27107=CARTESIAN_POINT('Ctrl Pts',(127.26757610129,-32.9938753525737,26.2682124992475));
#27108=CARTESIAN_POINT('Ctrl Pts',(127.277357937171,-32.9806197395715,26.2672481463267));
#27109=CARTESIAN_POINT('Ctrl Pts',(127.296466445943,-32.9551165399456,26.2653697269105));
#27110=CARTESIAN_POINT('Ctrl Pts',(127.305780551951,-32.9428603414275,26.2644564624457));
#27111=CARTESIAN_POINT('Ctrl Pts',(127.329168992009,-32.9125153694444,26.2621697457715));
#27112=CARTESIAN_POINT('Ctrl Pts',(127.343343799958,-32.8945052534146,26.2607896789041));
#27113=CARTESIAN_POINT('Ctrl Pts',(127.399973941049,-32.8240349162805,26.2553033936031));
#27114=CARTESIAN_POINT('Ctrl Pts',(127.443806997026,-32.7727066538227,26.2511162532689));
#27115=CARTESIAN_POINT('Ctrl Pts',(127.571665839718,-32.6317330599146,26.2391429971847));
#27116=CARTESIAN_POINT('Ctrl Pts',(127.659073905266,-32.5452988957365,26.2312338308905));
#27117=CARTESIAN_POINT('Ctrl Pts',(127.932361624292,-32.3029553962049,26.2076894962586));
#27118=CARTESIAN_POINT('Ctrl Pts',(128.130507823779,-32.1620057896263,26.1921534497731));
#27119=CARTESIAN_POINT('Ctrl Pts',(128.386902966921,-32.0182269213214,26.1742752335936));
#27120=CARTESIAN_POINT('Ctrl Pts',(128.43235239155,-31.994083477423,26.1711802157235));
#27121=CARTESIAN_POINT('Ctrl Pts',(128.505227863689,-31.9574735806384,26.166331559897));
#27122=CARTESIAN_POINT('Ctrl Pts',(128.532299237725,-31.9443224463463,26.1645546933086));
#27123=CARTESIAN_POINT('Ctrl Pts',(128.581126425488,-31.9214010727991,26.1613920947902));
#27124=CARTESIAN_POINT('Ctrl Pts',(128.602816715877,-31.9114967235814,26.1600018822684));
#27125=CARTESIAN_POINT('Ctrl Pts',(128.654075351643,-31.8887412183173,26.1567500320226));
#27126=CARTESIAN_POINT('Ctrl Pts',(128.683726379171,-31.876081271332,26.1548948999792));
#27127=CARTESIAN_POINT('Ctrl Pts',(128.772584788656,-31.8396316836202,26.1494086693622));
#27128=CARTESIAN_POINT('Ctrl Pts',(128.832289555741,-31.8170879635669,26.1458184115659));
#27129=CARTESIAN_POINT('Ctrl Pts',(129.048072915008,-31.7425008865129,26.133137551249));
#27130=CARTESIAN_POINT('Ctrl Pts',(129.207262065151,-31.7001457085345,26.1243371640464));
#27131=CARTESIAN_POINT('Ctrl Pts',(129.576727174316,-31.6301356227021,26.1043737983293));
#27132=CARTESIAN_POINT('Ctrl Pts',(129.787758316995,-31.6102976643573,26.0933029327255));
#27133=CARTESIAN_POINT('Ctrl Pts',(130.043951014271,-31.6102400261106,26.0789629364333));
#27134=CARTESIAN_POINT('Ctrl Pts',(130.088658298929,-31.6111146840661,26.0764263702882));
#27135=CARTESIAN_POINT('Ctrl Pts',(130.152805593533,-31.613639817594,26.0727214602308));
#27136=CARTESIAN_POINT('Ctrl Pts',(130.172270775874,-31.6145742402129,26.0715885649613));
#27137=CARTESIAN_POINT('Ctrl Pts',(130.206651730642,-31.6165219658253,26.0695705714045));
#27138=CARTESIAN_POINT('Ctrl Pts',(130.221570520848,-31.6174661807976,26.0686891822981));
#27139=CARTESIAN_POINT('Ctrl Pts',(130.254463019463,-31.6197665029575,26.0667328999854));
#27140=CARTESIAN_POINT('Ctrl Pts',(130.272432231053,-31.6211672769704,26.0656557547198));
#27141=CARTESIAN_POINT('Ctrl Pts',(130.325829951156,-31.625758566004,26.0624315179375));
#27142=CARTESIAN_POINT('Ctrl Pts',(130.361219290762,-31.6293634399044,26.0602640352331));
#27143=CARTESIAN_POINT('Ctrl Pts',(130.537598092024,-31.6501394461733,26.0493296501669));
#27144=CARTESIAN_POINT('Ctrl Pts',(130.677457965805,-31.6756020497781,26.0402434210629));
#27145=CARTESIAN_POINT('Ctrl Pts',(131.082481233426,-31.7759636241809,26.013379422321));
#27146=CARTESIAN_POINT('Ctrl Pts',(131.340658093015,-31.8744821345834,25.9956387661412));
#27147=CARTESIAN_POINT('Ctrl Pts',(131.626496728509,-32.0255734220944,25.976038353868));
#27148=CARTESIAN_POINT('Ctrl Pts',(131.668417347394,-32.048883434574,25.973161199341));
#27149=CARTESIAN_POINT('Ctrl Pts',(131.73495049132,-32.0877503226696,25.9685886514542));
#27150=CARTESIAN_POINT('Ctrl Pts',(131.759880726629,-32.1027476296637,25.966873845163));
#27151=CARTESIAN_POINT('Ctrl Pts',(131.807327002476,-32.1321283534849,25.9636064649977));
#27152=CARTESIAN_POINT('Ctrl Pts',(131.829872018882,-32.1464605961522,25.9620522088917));
#27153=CARTESIAN_POINT('Ctrl Pts',(131.881927614971,-32.1804238689389,25.9584582225732));
#27154=CARTESIAN_POINT('Ctrl Pts',(131.9113047065,-32.2002543757691,25.9564259898748));
#27155=CARTESIAN_POINT('Ctrl Pts',(132.008132127398,-32.2678505364383,25.9497086975587));
#27156=CARTESIAN_POINT('Ctrl Pts',(132.074148411893,-32.3176232250213,25.9450983415721));
#27157=CARTESIAN_POINT('Ctrl Pts',(132.23475817385,-32.4481928430184,25.9337285281904));
#27158=CARTESIAN_POINT('Ctrl Pts',(132.326848966293,-32.5318751176796,25.9270690867836));
#27159=CARTESIAN_POINT('Ctrl Pts',(132.548147210143,-32.7563882352958,25.91031167277));
#27160=CARTESIAN_POINT('Ctrl Pts',(132.670423627442,-32.9034131784751,25.9003206459875));
#27161=CARTESIAN_POINT('Ctrl Pts',(132.818660588792,-33.1158027922413,25.8860841678037));
#27162=CARTESIAN_POINT('Ctrl Pts',(132.855957423047,-33.1728293435759,25.8822769506339));
#27163=CARTESIAN_POINT('Ctrl Pts',(132.903863713192,-33.2511314865916,25.877015743733));
#27164=CARTESIAN_POINT('Ctrl Pts',(132.916006803609,-33.2714544276159,25.8756472564802));
#27165=CARTESIAN_POINT('Ctrl Pts',(132.934991466135,-33.3039969862346,25.8734485363741));
#27166=CARTESIAN_POINT('Ctrl Pts',(132.941972125748,-33.3161350633563,25.8726268169666));
#27167=CARTESIAN_POINT('Ctrl Pts',(132.956666799108,-33.342056698505,25.8708678041221));
#27168=CARTESIAN_POINT('Ctrl Pts',(132.964360024048,-33.3558515349639,25.8699291995874));
#27169=CARTESIAN_POINT('Ctrl Pts',(132.983937628066,-33.391540524465,25.8674954835977));
#27170=CARTESIAN_POINT('Ctrl Pts',(132.995677373985,-33.413512482222,25.8659919482933));
#27171=CARTESIAN_POINT('Ctrl Pts',(133.047471513738,-33.5130746602782,25.8591622912028));
#27172=CARTESIAN_POINT('Ctrl Pts',(133.084758293183,-33.5920605612015,25.8536996380028));
#27173=CARTESIAN_POINT('Ctrl Pts',(133.197750322388,-33.8575126747524,25.8353926787601));
#27174=CARTESIAN_POINT('Ctrl Pts',(133.259911396775,-34.0492819644057,25.8222756581342));
#27175=CARTESIAN_POINT('Ctrl Pts',(133.339300697521,-34.3969760994267,25.799544777836));
#27176=CARTESIAN_POINT('Ctrl Pts',(133.363441043687,-34.5507319297071,25.7898326576385));
#27177=CARTESIAN_POINT('Ctrl Pts',(133.380761554616,-34.7494214907845,25.7777827414339));
#27178=CARTESIAN_POINT('Ctrl Pts',(133.383727489832,-34.7932953183525,25.7751519298529));
#27179=CARTESIAN_POINT('Ctrl Pts',(133.387196737493,-34.8654542344397,25.7708725235286));
#27180=CARTESIAN_POINT('Ctrl Pts',(133.388201083338,-34.893708924528,25.7692087800152));
#27181=CARTESIAN_POINT('Ctrl Pts',(133.389474857267,-34.9490315743568,25.7659734802388));
#27182=CARTESIAN_POINT('Ctrl Pts',(133.389773780234,-34.9760966626119,25.764401138764));
#27183=CARTESIAN_POINT('Ctrl Pts',(133.389713358641,-35.0408493910121,25.7606628942086));
#27184=CARTESIAN_POINT('Ctrl Pts',(133.389049714405,-35.0785335624023,25.75850645419));
#27185=CARTESIAN_POINT('Ctrl Pts',(133.384378890436,-35.2147093735066,25.7507755481));
#27186=CARTESIAN_POINT('Ctrl Pts',(133.376704821279,-35.3130295338046,25.7453121235378));
#27187=CARTESIAN_POINT('Ctrl Pts',(133.344606796192,-35.5758836534239,25.7308795366582));
#27188=CARTESIAN_POINT('Ctrl Pts',(133.31234735193,-35.7391851584835,25.7221063009621));
#27189=CARTESIAN_POINT('Ctrl Pts',(133.222074825556,-36.0671943225409,25.7040584589812));
#27190=CARTESIAN_POINT('Ctrl Pts',(133.163073370296,-36.2311069985198,25.6948028366459));
#27191=CARTESIAN_POINT('Ctrl Pts',(133.077155047246,-36.422248743592,25.6829698820208));
#27192=CARTESIAN_POINT('Ctrl Pts',(133.062035677305,-36.4545143429691,25.6809346394649));
#27193=CARTESIAN_POINT('Ctrl Pts',(133.038501848042,-36.5027431138328,25.6778264552161));
#27194=CARTESIAN_POINT('Ctrl Pts',(133.030463491483,-36.5188881926641,25.6767746393246));
#27195=CARTESIAN_POINT('Ctrl Pts',(133.015527904107,-36.5482958286826,25.6748366393828));
#27196=CARTESIAN_POINT('Ctrl Pts',(133.008671241512,-36.5615779991443,25.6739528607498));
#27197=CARTESIAN_POINT('Ctrl Pts',(132.992524138716,-36.5923557180179,25.6718853637653));
#27198=CARTESIAN_POINT('Ctrl Pts',(132.983167970902,-36.6098156009669,25.670697773503));
#27199=CARTESIAN_POINT('Ctrl Pts',(132.951874885448,-36.66700306412,25.6667618066143));
#27200=CARTESIAN_POINT('Ctrl Pts',(132.929294007879,-36.7063706360173,25.6639783386855));
#27201=CARTESIAN_POINT('Ctrl Pts',(132.871407254879,-36.8027538960762,25.6570000068675));
#27202=CARTESIAN_POINT('Ctrl Pts',(132.835187255167,-36.8591970183983,25.6527676909545));
#27203=CARTESIAN_POINT('Ctrl Pts',(132.638126155383,-37.1471235644097,25.6305395744156));
#27204=CARTESIAN_POINT('Ctrl Pts',(132.450512860566,-37.3589983418362,25.6120928473726));
#27205=CARTESIAN_POINT('Ctrl Pts',(132.178893386909,-37.5979223458838,25.5896843228841));
#27206=CARTESIAN_POINT('Ctrl Pts',(132.11711062319,-37.6485129955901,25.5848154736091));
#27207=CARTESIAN_POINT('Ctrl Pts',(132.02790930571,-37.7164372301631,25.5780964472045));
#27208=CARTESIAN_POINT('Ctrl Pts',(132.001944748504,-37.7356287594849,25.5761757371733));
#27209=CARTESIAN_POINT('Ctrl Pts',(131.95385080078,-37.7701255791025,25.57268060927));
#27210=CARTESIAN_POINT('Ctrl Pts',(131.931806011754,-37.7855438016303,25.5711020002461));
#27211=CARTESIAN_POINT('Ctrl Pts',(131.886414002077,-37.8164931018334,25.5678980516255));
#27212=CARTESIAN_POINT('Ctrl Pts',(131.86305290564,-37.8320001976431,25.566273683678));
#27213=CARTESIAN_POINT('Ctrl Pts',(131.803536961595,-37.8704516787979,25.5621951352898));
#27214=CARTESIAN_POINT('Ctrl Pts',(131.767134263767,-37.8930045173811,25.5597552639241));
#27215=CARTESIAN_POINT('Ctrl Pts',(131.599397881863,-37.9925757431818,25.5487446477152));
#27216=CARTESIAN_POINT('Ctrl Pts',(131.463389495656,-38.0613855047465,25.5404629722138));
#27217=CARTESIAN_POINT('Ctrl Pts',(131.280208020721,-38.139052949277,25.5298183173276));
#27218=CARTESIAN_POINT('Ctrl Pts',(131.236840002805,-38.156392385583,25.5273328398893));
#27219=CARTESIAN_POINT('Ctrl Pts',(131.000206013559,-38.2453774246887,25.5139075857791));
#27220=CARTESIAN_POINT('Ctrl Pts',(130.801087671491,-38.3001712553871,25.5031209759358));
#27221=CARTESIAN_POINT('Ctrl Pts',(130.549510224445,-38.3452795554704,25.4888867510208));
#27222=CARTESIAN_POINT('Ctrl Pts',(130.500589435965,-38.3529489248003,25.4860899342451));
#27223=CARTESIAN_POINT('Ctrl Pts',(130.432615073598,-38.3620846430312,25.4821425964938));
#27224=CARTESIAN_POINT('Ctrl Pts',(130.413688609792,-38.364465878408,25.4810369740353));
#27225=CARTESIAN_POINT('Ctrl Pts',(130.379632988619,-38.3684588944788,25.4790342045704));
#27226=CARTESIAN_POINT('Ctrl Pts',(130.364510881969,-38.3701288313052,25.4781401594019));
#27227=CARTESIAN_POINT('Ctrl Pts',(130.332991860657,-38.373394859023,25.4762659897216));
#27228=CARTESIAN_POINT('Ctrl Pts',(130.316593843099,-38.3749732988077,25.4752850075943));
#27229=CARTESIAN_POINT('Ctrl Pts',(130.272228509807,-38.3789176468158,25.4726160941092));
#27230=CARTESIAN_POINT('Ctrl Pts',(130.244242845664,-38.3810557739627,25.4709166274426));
#27231=CARTESIAN_POINT('Ctrl Pts',(130.071585019871,-38.3920922331794,25.4603468307246));
#27232=CARTESIAN_POINT('Ctrl Pts',(129.926503670802,-38.3920502235697,25.4511040990249));
#27233=CARTESIAN_POINT('Ctrl Pts',(129.533170004118,-38.3666884914843,25.4257534726648));
#27234=CARTESIAN_POINT('Ctrl Pts',(129.286944170252,-38.3232671306737,25.4096260701744));
#27235=CARTESIAN_POINT('Ctrl Pts',(128.981116253666,-38.2337428355661,25.3900195338736));
#27236=CARTESIAN_POINT('Ctrl Pts',(128.915153730744,-38.2122151910756,25.3858112077257));
#27237=CARTESIAN_POINT('Ctrl Pts',(128.818617880988,-38.1773962360449,25.3796809771827));
#27238=CARTESIAN_POINT('Ctrl Pts',(128.787508108005,-38.165655395324,25.3777098414903));
#27239=CARTESIAN_POINT('Ctrl Pts',(128.731952973321,-38.1437497222584,25.374196584072));
#27240=CARTESIAN_POINT('Ctrl Pts',(128.70744474499,-38.1337527901405,25.3726490947544));
#27241=CARTESIAN_POINT('Ctrl Pts',(128.655135577234,-38.1116977441667,25.3693503150698));
#27242=CARTESIAN_POINT('Ctrl Pts',(128.62737403661,-38.0995517768112,25.367602111026));
#27243=CARTESIAN_POINT('Ctrl Pts',(128.550732498311,-38.0647886014754,25.3627802649627));
#27244=CARTESIAN_POINT('Ctrl Pts',(128.502221982979,-38.041375826811,25.3597334638496));
#27245=CARTESIAN_POINT('Ctrl Pts',(128.291878573805,-37.933603155817,25.346514604831));
#27246=CARTESIAN_POINT('Ctrl Pts',(128.136447880491,-37.8374087380429,25.3367462433169));
#27247=CARTESIAN_POINT('Ctrl Pts',(127.817084479054,-37.6021428356282,25.3156905409571));
#27248=CARTESIAN_POINT('Ctrl Pts',(127.65710613106,-37.4590846297011,25.3044810377785));
#27249=CARTESIAN_POINT('Ctrl Pts',(127.483221020712,-37.271120485721,25.2901125714594));
#27250=CARTESIAN_POINT('Ctrl Pts',(127.455310362949,-37.2398033422622,25.2877282205396));
#27251=CARTESIAN_POINT('Ctrl Pts',(127.415472560754,-37.1933974190403,25.2841951278275));
#27252=CARTESIAN_POINT('Ctrl Pts',(127.403080300457,-37.1787111691146,25.2830770027148));
#27253=CARTESIAN_POINT('Ctrl Pts',(127.381292617278,-37.1524402806168,25.2810752821355));
#27254=CARTESIAN_POINT('Ctrl Pts',(127.371847779662,-37.1408978043242,25.2801951712567));
#27255=CARTESIAN_POINT('Ctrl Pts',(127.350848889111,-37.1148868195185,25.2782102224457));
#27256=CARTESIAN_POINT('Ctrl Pts',(127.339337091931,-37.1003858509212,25.2771026760653));
#27257=CARTESIAN_POINT('Ctrl Pts',(127.304488491964,-37.0557421895858,25.2736919179755));
#27258=CARTESIAN_POINT('Ctrl Pts',(127.281541624904,-37.0253004817645,25.2713648353679));
#27259=CARTESIAN_POINT('Ctrl Pts',(127.22812133883,-36.9518883980091,25.2657622338185));
#27260=CARTESIAN_POINT('Ctrl Pts',(127.198126974572,-36.908582371011,25.2624646658873));
#27261=CARTESIAN_POINT('Ctrl Pts',(127.105441547351,-36.7678666961246,25.25181438779));
#27262=CARTESIAN_POINT('Ctrl Pts',(127.04672991839,-36.6679374232611,25.2443498360029));
#27263=CARTESIAN_POINT('Ctrl Pts',(126.889102808978,-36.365136342913,25.2223446256813));
#27264=CARTESIAN_POINT('Ctrl Pts',(126.805169692314,-36.1551469310553,25.2078959013107));
#27265=CARTESIAN_POINT('Ctrl Pts',(126.728060203813,-35.8874784752449,25.190873112828));
#27266=CARTESIAN_POINT('Ctrl Pts',(126.714597682359,-35.8362656003739,25.1876734303632));
#27267=CARTESIAN_POINT('Ctrl Pts',(126.694675858038,-35.7525511772749,25.1825340661964));
#27268=CARTESIAN_POINT('Ctrl Pts',(126.687483913848,-35.7202348599203,25.1805718226491));
#27269=CARTESIAN_POINT('Ctrl Pts',(126.675398087947,-35.6619117131779,25.177068185866));
#27270=CARTESIAN_POINT('Ctrl Pts',(126.670333204605,-35.6359434567092,25.1755215465766));
#27271=CARTESIAN_POINT('Ctrl Pts',(126.661092781109,-35.585425978005,25.1725376881475));
#27272=CARTESIAN_POINT('Ctrl Pts',(126.656882713319,-35.5608848788984,25.1710994834994));
#27273=CARTESIAN_POINT('Ctrl Pts',(126.648205463771,-35.5067299420334,25.1679495856491));
#27274=CARTESIAN_POINT('Ctrl Pts',(126.643859535123,-35.4770986343486,25.1662416958792));
#27275=CARTESIAN_POINT('Ctrl Pts',(126.632370063276,-35.39081213588,25.1613104073976));
#27276=CARTESIAN_POINT('Ctrl Pts',(126.626264485296,-35.3340279736208,25.1581178992765));
#27277=CARTESIAN_POINT('Ctrl Pts',(126.613962667415,-35.18405197675,25.1497989695217));
#27278=CARTESIAN_POINT('Ctrl Pts',(126.610177537892,-35.0907116357337,25.1447368543743));
#27279=CARTESIAN_POINT('Ctrl Pts',(126.61025105039,-34.9973314581693,25.1397298775655));
#27280=CARTESIAN_POINT('Ctrl Pts',(126.610251047991,-34.9973345073913,25.1397300410625));
#27281=CARTESIAN_POINT('Ctrl Pts',(126.610442852642,-34.7534135092292,25.1266511724115));
#27282=CARTESIAN_POINT('Ctrl Pts',(126.636961587853,-34.5102363678044,25.1140470393936));
#27283=CARTESIAN_POINT('Ctrl Pts',(126.703286733997,-34.2086073460077,25.0970240520163));
#27284=CARTESIAN_POINT('Ctrl Pts',(126.719048765736,-34.1456121463358,25.0933861108642));
#27285=CARTESIAN_POINT('Ctrl Pts',(126.742725428392,-34.0613420215835,25.0883607212718));
#27286=CARTESIAN_POINT('Ctrl Pts',(126.749059650024,-34.0396338110871,25.0870517513496));
#27287=CARTESIAN_POINT('Ctrl Pts',(126.76005363156,-34.0033115697369,25.0848348292149));
#27288=CARTESIAN_POINT('Ctrl Pts',(126.764596378906,-33.9886624206434,25.0839333494163));
#27289=CARTESIAN_POINT('Ctrl Pts',(126.774256935561,-33.9582410629125,25.0820450494289));
#27290=CARTESIAN_POINT('Ctrl Pts',(126.779391261301,-33.9424749045304,25.0810573909748));
#27291=CARTESIAN_POINT('Ctrl Pts',(126.793686010773,-33.8996492424574,25.0783511872542));
#27292=CARTESIAN_POINT('Ctrl Pts',(126.803072976973,-33.87266744937,25.0766205799485));
#27293=CARTESIAN_POINT('Ctrl Pts',(126.815585988529,-33.8381138444426,25.0743741277453));
#27294=CARTESIAN_POINT('Ctrl Pts',(126.818400150778,-33.8304298155902,25.0738726265239));
#27295=CARTESIAN_POINT('Ctrl Pts',(126.821241914321,-33.8227565692546,25.0733699431874));
#27296=CARTESIAN_POINT('Ctrl Pts',(126.82124193643,-33.822756509559,25.4139334024237));
#27297=CARTESIAN_POINT('Ctrl Pts',(126.787245704209,-33.9145521305829,25.4191427755899));
#27298=CARTESIAN_POINT('Ctrl Pts',(126.757213458934,-34.007853458936,25.4243154379788));
#27299=CARTESIAN_POINT('Ctrl Pts',(126.688840402644,-34.2568461875151,25.4380514877741));
#27300=CARTESIAN_POINT('Ctrl Pts',(126.657434412747,-34.4140822036232,25.4466549067327));
#27301=CARTESIAN_POINT('Ctrl Pts',(126.633676902108,-34.6011478868738,25.4573910116902));
#27302=CARTESIAN_POINT('Ctrl Pts',(126.630448555809,-34.6294097141762,25.4590264691335));
#27303=CARTESIAN_POINT('Ctrl Pts',(126.625904661282,-34.6741783018617,25.4616430471889));
#27304=CARTESIAN_POINT('Ctrl Pts',(126.624353671105,-34.6906604279019,25.4626119143837));
#27305=CARTESIAN_POINT('Ctrl Pts',(126.62161264791,-34.7222695651522,25.4644817185376));
#27306=CARTESIAN_POINT('Ctrl Pts',(126.620403354746,-34.7373942550521,25.4653816259913));
#27307=CARTESIAN_POINT('Ctrl Pts',(126.617650048824,-34.775006758323,25.4676317779128));
#27308=CARTESIAN_POINT('Ctrl Pts',(126.616228745331,-34.7975026245944,25.4689884097207));
#27309=CARTESIAN_POINT('Ctrl Pts',(126.611870212197,-34.8794711854176,25.4739669495039));
#27310=CARTESIAN_POINT('Ctrl Pts',(126.610275975973,-34.9390014906017,25.4776502533167));
#27311=CARTESIAN_POINT('Ctrl Pts',(126.610205881268,-35.1016313215704,25.4878440348002));
#27312=CARTESIAN_POINT('Ctrl Pts',(126.614864498925,-35.2046670969959,25.4944453108071));
#27313=CARTESIAN_POINT('Ctrl Pts',(126.648420621211,-35.573262356808,25.5182665406884));
#27314=CARTESIAN_POINT('Ctrl Pts',(126.703976296854,-35.8354551113146,25.5355024212253));
#27315=CARTESIAN_POINT('Ctrl Pts',(126.806981263004,-36.139261775208,25.5550454646257));
#27316=CARTESIAN_POINT('Ctrl Pts',(126.825421536744,-36.1896798391686,25.5582781045745));
#27317=CARTESIAN_POINT('Ctrl Pts',(126.856231318259,-36.2680922630069,25.5632909305051));
#27318=CARTESIAN_POINT('Ctrl Pts',(126.867795010541,-36.2963917261077,25.5650970584487));
#27319=CARTESIAN_POINT('Ctrl Pts',(126.890071584234,-36.3488696711284,25.5684416982363));
#27320=CARTESIAN_POINT('Ctrl Pts',(126.900687555886,-36.3730865133278,25.5699832846886));
#27321=CARTESIAN_POINT('Ctrl Pts',(126.925135306658,-36.4271274583494,25.5734203754036));
#27322=CARTESIAN_POINT('Ctrl Pts',(126.939119878457,-36.4568797667438,25.5753105642273));
#27323=CARTESIAN_POINT('Ctrl Pts',(126.983028987265,-36.5468725830967,25.581025302252));
#27324=CARTESIAN_POINT('Ctrl Pts',(127.014316359812,-36.6064317326092,25.5848035277591));
#27325=CARTESIAN_POINT('Ctrl Pts',(127.169687276383,-36.8819563252734,25.602333395267));
#27326=CARTESIAN_POINT('Ctrl Pts',(127.315548276213,-37.0847431046058,25.615321886196));
#27327=CARTESIAN_POINT('Ctrl Pts',(127.581383177703,-37.3796194675264,25.6364866707286));
#27328=CARTESIAN_POINT('Ctrl Pts',(127.687531428811,-37.4828967243146,25.6444716831675));
#27329=CARTESIAN_POINT('Ctrl Pts',(127.821605610217,-37.5972685753959,25.6545070952492));
#27330=CARTESIAN_POINT('Ctrl Pts',(127.843367470255,-37.6153665499935,25.6561346450307));
#27331=CARTESIAN_POINT('Ctrl Pts',(127.878189225958,-37.6435955003439,25.6587414669841));
#27332=CARTESIAN_POINT('Ctrl Pts',(127.891101444329,-37.6539074940926,25.6597086402304));
#27333=CARTESIAN_POINT('Ctrl Pts',(127.916165677873,-37.6736259505897,25.6615882001489));
#27334=CARTESIAN_POINT('Ctrl Pts',(127.928307079374,-37.6830448401183,25.6624997266158));
#27335=CARTESIAN_POINT('Ctrl Pts',(127.958599366436,-37.7062163824547,25.6647757545627));
#27336=CARTESIAN_POINT('Ctrl Pts',(127.976825445937,-37.7198691728403,25.6661467400372));
#27337=CARTESIAN_POINT('Ctrl Pts',(128.048604903044,-37.7725170478575,25.6715476500428));
#27338=CARTESIAN_POINT('Ctrl Pts',(128.103156292401,-37.8101203495046,25.6756554669053));
#27339=CARTESIAN_POINT('Ctrl Pts',(128.258750879866,-37.9107793199093,25.6873065634296));
#27340=CARTESIAN_POINT('Ctrl Pts',(128.362065870056,-37.9701437677219,25.6949661824686));
#27341=CARTESIAN_POINT('Ctrl Pts',(128.69037029607,-38.1364393504687,25.7186855316003));
#27342=CARTESIAN_POINT('Ctrl Pts',(128.924208465432,-38.2241419275337,25.7346584128665));
#27343=CARTESIAN_POINT('Ctrl Pts',(129.215397390698,-38.2980974281019,25.7529214078871));
#27344=CARTESIAN_POINT('Ctrl Pts',(129.265507339742,-38.3096176312419,25.7560120066338));
#27345=CARTESIAN_POINT('Ctrl Pts',(129.345051031264,-38.3260088820693,25.7608379839455));
#27346=CARTESIAN_POINT('Ctrl Pts',(129.374318694114,-38.3316386694311,25.7625967798613));
#27347=CARTESIAN_POINT('Ctrl Pts',(129.429784510833,-38.3415511038982,25.7658990934757));
#27348=CARTESIAN_POINT('Ctrl Pts',(129.455965969773,-38.3459134054856,25.7674449860698));
#27349=CARTESIAN_POINT('Ctrl Pts',(129.515836818474,-38.3551676237021,25.7709519192941));
#27350=CARTESIAN_POINT('Ctrl Pts',(129.549554353529,-38.3598605043914,25.7729066570245));
#27351=CARTESIAN_POINT('Ctrl Pts',(129.656724560794,-38.3731343402817,25.7790601601875));
#27352=CARTESIAN_POINT('Ctrl Pts',(129.730392340303,-38.3798204234853,25.7832010664015));
#27353=CARTESIAN_POINT('Ctrl Pts',(129.909322663475,-38.3901718880995,25.793093815337));
#27354=CARTESIAN_POINT('Ctrl Pts',(130.014652084743,-38.3913529945894,25.7987784469583));
#27355=CARTESIAN_POINT('Ctrl Pts',(130.243976267176,-38.3832384183336,25.8110392872419));
#27356=CARTESIAN_POINT('Ctrl Pts',(130.367746534448,-38.3720304194298,25.8175820577195));
#27357=CARTESIAN_POINT('Ctrl Pts',(130.633803881423,-38.3331122438844,25.8318931334268));
#27358=CARTESIAN_POINT('Ctrl Pts',(130.775484373895,-38.30302297775,25.839670564831));
#27359=CARTESIAN_POINT('Ctrl Pts',(130.949123615791,-38.2543571550464,25.849852613178));
#27360=CARTESIAN_POINT('Ctrl Pts',(130.983297503208,-38.2441951143609,25.8518889890201));
#27361=CARTESIAN_POINT('Ctrl Pts',(131.034511437505,-38.2280824924763,25.8549985616961));
#27362=CARTESIAN_POINT('Ctrl Pts',(131.051675651107,-38.2225314250919,25.8560506046008));
#27363=CARTESIAN_POINT('Ctrl Pts',(131.082979757373,-38.2121306554416,25.8579888070591));
#27364=CARTESIAN_POINT('Ctrl Pts',(131.097133038533,-38.2073240515501,25.8588725574213));
#27365=CARTESIAN_POINT('Ctrl Pts',(131.129963181995,-38.1959318593251,25.8609397007394));
#27366=CARTESIAN_POINT('Ctrl Pts',(131.148614570608,-38.1892760571265,25.8621269608499));
#27367=CARTESIAN_POINT('Ctrl Pts',(131.20978244548,-38.1668419737231,25.8660606346946));
#27368=CARTESIAN_POINT('Ctrl Pts',(131.252039042161,-38.150374496244,25.8688420860223));
#27369=CARTESIAN_POINT('Ctrl Pts',(131.355864450288,-38.1074947884238,25.8758141153587));
#27370=CARTESIAN_POINT('Ctrl Pts',(131.417004005171,-38.0800959418345,25.8800420658591));
#27371=CARTESIAN_POINT('Ctrl Pts',(131.730130198394,-37.9284761305506,25.902205670715));
#27372=CARTESIAN_POINT('Ctrl Pts',(131.966816192955,-37.775066412917,25.9205910798073));
#27373=CARTESIAN_POINT('Ctrl Pts',(132.243504116812,-37.5423576745732,25.9429952833657));
#27374=CARTESIAN_POINT('Ctrl Pts',(132.303285096733,-37.488327278408,25.9479098378704));
#27375=CARTESIAN_POINT('Ctrl Pts',(132.384333435747,-37.4096490778797,25.9546800258246));
#27376=CARTESIAN_POINT('Ctrl Pts',(132.407254642719,-37.3867508889208,25.9566076214498));
#27377=CARTESIAN_POINT('Ctrl Pts',(132.448619636211,-37.344225244498,25.9601112747249));
#27378=CARTESIAN_POINT('Ctrl Pts',(132.467164330396,-37.3247000556938,25.9616916011689));
#27379=CARTESIAN_POINT('Ctrl Pts',(132.504512491792,-37.2844268648241,25.9648950353677));
#27380=CARTESIAN_POINT('Ctrl Pts',(132.523295508523,-37.2636626885251,25.9665172218916));
#27381=CARTESIAN_POINT('Ctrl Pts',(132.57001493324,-37.2107113104227,25.9705823091845));
#27382=CARTESIAN_POINT('Ctrl Pts',(132.597606007651,-37.178225083099,25.9730111013198));
#27383=CARTESIAN_POINT('Ctrl Pts',(132.719058181566,-37.0296343572002,25.983845785645));
#27384=CARTESIAN_POINT('Ctrl Pts',(132.805803945586,-36.9079213311702,25.991974752014));
#27385=CARTESIAN_POINT('Ctrl Pts',(132.95191839456,-36.6712789097517,26.0068650138268));
#27386=CARTESIAN_POINT('Ctrl Pts',(133.013286259049,-36.557915786643,26.0136509503787));
#27387=CARTESIAN_POINT('Ctrl Pts',(133.131480819086,-36.3063245018191,26.0284346286501));
#27388=CARTESIAN_POINT('Ctrl Pts',(133.185920499401,-36.1672866050858,26.0364382882537));
#27389=CARTESIAN_POINT('Ctrl Pts',(133.241874119128,-35.990931202135,26.0468825855411));
#27390=CARTESIAN_POINT('Ctrl Pts',(133.252180903041,-35.9565623926181,26.0489316085174));
#27391=CARTESIAN_POINT('Ctrl Pts',(133.266858868967,-35.9046354168717,26.0520566529567));
#27392=CARTESIAN_POINT('Ctrl Pts',(133.271638495118,-35.8871942473503,26.0531112051102));
#27393=CARTESIAN_POINT('Ctrl Pts',(133.280112292474,-35.8552728907168,26.0550516230709));
#27394=CARTESIAN_POINT('Ctrl Pts',(133.28385059507,-35.8408053353152,26.0559350376184));
#27395=CARTESIAN_POINT('Ctrl Pts',(133.292305973281,-35.8071655649761,26.0579981896492));
#27396=CARTESIAN_POINT('Ctrl Pts',(133.296951319751,-35.7879764113146,26.0591817411637));
#27397=CARTESIAN_POINT('Ctrl Pts',(133.311632555241,-35.7249270985144,26.063089860786));
#27398=CARTESIAN_POINT('Ctrl Pts',(133.320962456073,-35.6809092679978,26.0658488717137));
#27399=CARTESIAN_POINT('Ctrl Pts',(133.341856309441,-35.5716553671269,26.0727509408532));
#27400=CARTESIAN_POINT('Ctrl Pts',(133.352388946846,-35.5062419553376,26.0769304949928));
#27401=CARTESIAN_POINT('Ctrl Pts',(133.396218345873,-35.1718750901233,26.0984066332734));
#27402=CARTESIAN_POINT('Ctrl Pts',(133.399095101174,-34.8998871634906,26.1161397992864));
#27403=CARTESIAN_POINT('Ctrl Pts',(133.3598719393,-34.5422434304771,26.1385264779311));
#27404=CARTESIAN_POINT('Ctrl Pts',(133.346736299976,-34.4544371706386,26.1439575261338));
#27405=CARTESIAN_POINT('Ctrl Pts',(133.323232021166,-34.3307356436352,26.1515144021166));
#27406=CARTESIAN_POINT('Ctrl Pts',(133.315695641226,-34.294345392661,26.1537259288782));
#27407=CARTESIAN_POINT('Ctrl Pts',(133.301657845245,-34.2317628841904,26.1575106399686));
#27408=CARTESIAN_POINT('Ctrl Pts',(133.295439369463,-34.2055113481075,26.1590925318514));
#27409=CARTESIAN_POINT('Ctrl Pts',(133.282023542729,-34.1517458184858,26.1623216706012));
#27410=CARTESIAN_POINT('Ctrl Pts',(133.274791990878,-34.1242425110012,26.1639676929666));
#27411=CARTESIAN_POINT('Ctrl Pts',(133.255284206633,-34.0536729326261,26.1681780231017));
#27412=CARTESIAN_POINT('Ctrl Pts',(133.242498966873,-34.010752357864,26.1707260154638));
#27413=CARTESIAN_POINT('Ctrl Pts',(133.170367075123,-33.7850488893111,26.1840770287661));
#27414=CARTESIAN_POINT('Ctrl Pts',(133.096406190468,-33.607300057701,26.194397302453));
#27415=CARTESIAN_POINT('Ctrl Pts',(132.914920076432,-33.2581089971184,26.2153015438782));
#27416=CARTESIAN_POINT('Ctrl Pts',(132.806343645562,-33.0880989341488,26.225838038678));
#27417=CARTESIAN_POINT('Ctrl Pts',(132.649533434162,-32.8849496238822,26.2400688177508));
#27418=CARTESIAN_POINT('Ctrl Pts',(132.614665041127,-32.841993619884,26.2431830582179));
#27419=CARTESIAN_POINT('Ctrl Pts',(132.5645435767,-32.7832453219295,26.2476217727078));
#27420=CARTESIAN_POINT('Ctrl Pts',(132.550162989169,-32.7667168263191,26.2488911814358));
#27421=CARTESIAN_POINT('Ctrl Pts',(132.525525832908,-32.7389480703399,26.2510613402408));
#27422=CARTESIAN_POINT('Ctrl Pts',(132.515351710289,-32.7276350800774,26.2519562511849));
#27423=CARTESIAN_POINT('Ctrl Pts',(132.493744968918,-32.7039326497257,26.2538548752673));
#27424=CARTESIAN_POINT('Ctrl Pts',(132.482295699705,-32.691559556845,26.2548597208605));
#27425=CARTESIAN_POINT('Ctrl Pts',(132.450306886043,-32.6575027692292,26.2576625587953));
#27426=CARTESIAN_POINT('Ctrl Pts',(132.429572798851,-32.6360048657712,26.2594740222598));
#27427=CARTESIAN_POINT('Ctrl Pts',(132.381780701611,-32.5877450553072,26.263631896904));
#27428=CARTESIAN_POINT('Ctrl Pts',(132.354550832211,-32.5611594183934,26.2659884990843));
#27429=CARTESIAN_POINT('Ctrl Pts',(132.261969026402,-32.4737638090419,26.2739434100994));
#27430=CARTESIAN_POINT('Ctrl Pts',(132.19466592247,-32.4150796904743,26.2796323149203));
#27431=CARTESIAN_POINT('Ctrl Pts',(131.895107286787,-32.1740230585245,26.304315104801));
#27432=CARTESIAN_POINT('Ctrl Pts',(131.641836126465,-32.0197297813164,26.3234667522904));
#27433=CARTESIAN_POINT('Ctrl Pts',(131.325760037249,-31.8798566150797,26.3444598076618));
#27434=CARTESIAN_POINT('Ctrl Pts',(131.279320405142,-31.8605296424742,26.3474813287574));
#27435=CARTESIAN_POINT('Ctrl Pts',(131.20491671409,-31.8314900428239,26.3522253915821));
#27436=CARTESIAN_POINT('Ctrl Pts',(131.177227330573,-31.821098376524,26.3539700227239));
#27437=CARTESIAN_POINT('Ctrl Pts',(131.124393203832,-31.8020550600788,26.3572605397195));
#27438=CARTESIAN_POINT('Ctrl Pts',(131.099275881102,-31.7933343622869,26.3588085829967));
#27439=CARTESIAN_POINT('Ctrl Pts',(131.041381834062,-31.7739938264764,26.3623407796383));
#27440=CARTESIAN_POINT('Ctrl Pts',(131.00854032239,-31.7635762795696,26.3643182808736));
#27441=CARTESIAN_POINT('Ctrl Pts',(130.902357678865,-31.7316677434358,26.3706328335647));
#27442=CARTESIAN_POINT('Ctrl Pts',(130.828444487925,-31.712154803958,26.3749074503057));
#27443=CARTESIAN_POINT('Ctrl Pts',(130.646218320187,-31.6705837248991,26.3852093804827));
#27444=CARTESIAN_POINT('Ctrl Pts',(130.53736446586,-31.6512909229631,26.3911611840199));
#27445=CARTESIAN_POINT('Ctrl Pts',(130.214716711872,-31.6102473811741,26.4085103118073));
#27446=CARTESIAN_POINT('Ctrl Pts',(129.999598238162,-31.6034556349267,26.4196843782863));
#27447=CARTESIAN_POINT('Ctrl Pts',(129.71816053168,-31.6213172038474,26.4351933914901));
#27448=CARTESIAN_POINT('Ctrl Pts',(129.651167112662,-31.62757574472,26.4389545883871));
#27449=CARTESIAN_POINT('Ctrl Pts',(129.561017366068,-31.6387123269632,26.4441616456333));
#27450=CARTESIAN_POINT('Ctrl Pts',(129.537657362573,-31.6418457759108,26.4455242355563));
#27451=CARTESIAN_POINT('Ctrl Pts',(129.500493436248,-31.6472259555943,26.4477159235646));
#27452=CARTESIAN_POINT('Ctrl Pts',(129.48666703266,-31.6493150178924,26.4485366073992));
#27453=CARTESIAN_POINT('Ctrl Pts',(129.457225277952,-31.6539499434106,26.4502961979962));
#27454=CARTESIAN_POINT('Ctrl Pts',(129.441614118659,-31.6565196929192,26.4512364455543));
#27455=CARTESIAN_POINT('Ctrl Pts',(129.401348776475,-31.6634376212321,26.4536793171709));
#27456=CARTESIAN_POINT('Ctrl Pts',(129.376724159326,-31.6679497391838,26.4551904792097));
#27457=CARTESIAN_POINT('Ctrl Pts',(129.265017159348,-31.6897000566389,26.4621171818812));
#27458=CARTESIAN_POINT('Ctrl Pts',(129.178588425886,-31.7100811540554,26.4676738549862));
#27459=CARTESIAN_POINT('Ctrl Pts',(128.891699580637,-31.7897429491614,26.486577467915));
#27460=CARTESIAN_POINT('Ctrl Pts',(128.695934086685,-31.8641593476491,26.5002117283727));
#27461=CARTESIAN_POINT('Ctrl Pts',(128.376302451349,-32.0208042372218,26.5228489240746));
#27462=CARTESIAN_POINT('Ctrl Pts',(128.248674742486,-32.093994163338,26.5320101448521));
#27463=CARTESIAN_POINT('Ctrl Pts',(128.08995362208,-32.1992824965346,26.5435127862868));
#27464=CARTESIAN_POINT('Ctrl Pts',(128.05418420511,-32.224014255096,26.5461135739441));
#27465=CARTESIAN_POINT('Ctrl Pts',(127.996039462624,-32.2658930370188,26.550357273483));
#27466=CARTESIAN_POINT('Ctrl Pts',(127.973385336374,-32.2826424973632,26.5520148398546));
#27467=CARTESIAN_POINT('Ctrl Pts',(127.929334782069,-32.3160688672133,26.5552471647612));
#27468=CARTESIAN_POINT('Ctrl Pts',(127.907924570049,-32.3327240059741,26.556822589318));
#27469=CARTESIAN_POINT('Ctrl Pts',(127.856984947556,-32.3733410045625,26.5605829652382));
#27470=CARTESIAN_POINT('Ctrl Pts',(127.827653992501,-32.3975465456926,26.5627581497772));
#27471=CARTESIAN_POINT('Ctrl Pts',(127.721750973548,-32.4879819031902,26.570656733372));
#27472=CARTESIAN_POINT('Ctrl Pts',(127.647745972011,-32.5571416221869,26.576262294808));
#27473=CARTESIAN_POINT('Ctrl Pts',(127.399746765793,-32.8106409177155,26.5955676588138));
#27474=CARTESIAN_POINT('Ctrl Pts',(127.243428179312,-33.011051966476,26.608651887737));
#27475=CARTESIAN_POINT('Ctrl Pts',(127.058954235618,-33.3116519519306,26.6277292490004));
#27476=CARTESIAN_POINT('Ctrl Pts',(127.010755401214,-33.3985373091709,26.6331964845641));
#27477=CARTESIAN_POINT('Ctrl Pts',(126.954607499484,-33.5111436573751,26.6403786564727));
#27478=CARTESIAN_POINT('Ctrl Pts',(126.943050346605,-33.5350196536688,26.6419068503812));
#27479=CARTESIAN_POINT('Ctrl Pts',(126.924912940587,-33.5736391716766,26.6443911186429));
#27480=CARTESIAN_POINT('Ctrl Pts',(126.91815552176,-33.5882988191386,26.645336967813));
#27481=CARTESIAN_POINT('Ctrl Pts',(126.905070274942,-33.6172278897419,26.6472101219333));
#27482=CARTESIAN_POINT('Ctrl Pts',(126.898735850074,-33.6314937507399,26.6481370260561));
#27483=CARTESIAN_POINT('Ctrl Pts',(126.88290537347,-33.6678202079074,26.6505044378755));
#27484=CARTESIAN_POINT('Ctrl Pts',(126.8735449547,-33.6899386704676,26.6519525488066));
#27485=CARTESIAN_POINT('Ctrl Pts',(126.849381463222,-33.748770663097,26.6558182816861));
#27486=CARTESIAN_POINT('Ctrl Pts',(126.834986479187,-33.7856438997939,26.6582553902751));
#27487=CARTESIAN_POINT('Ctrl Pts',(126.821241917671,-33.8227565602112,26.6607167036746));
#27488=CARTESIAN_POINT('Origin',(130.,-35.,23.));
#27489=CARTESIAN_POINT('',(126.821241915871,-33.8227565650715,27.9134201656876));
#27490=CARTESIAN_POINT('',(126.821241909639,-33.8227565818973,27.5681924492054));
#27491=CARTESIAN_POINT('',(126.821241915871,-33.8227565650715,23.));
#27492=CARTESIAN_POINT('Ctrl Pts',(126.821241909639,-33.8227565818973,27.5681924492054));
#27493=CARTESIAN_POINT('Ctrl Pts',(126.830994690413,-33.796422409788,27.5664434765392));
#27494=CARTESIAN_POINT('Ctrl Pts',(126.841075512034,-33.770207282694,27.5647030610561));
#27495=CARTESIAN_POINT('Ctrl Pts',(126.878262909731,-33.676977887363,27.5585167549009));
#27496=CARTESIAN_POINT('Ctrl Pts',(126.907185575693,-33.6107087819299,27.5541258504753));
#27497=CARTESIAN_POINT('Ctrl Pts',(126.952692476912,-33.5149203903061,27.5477868022147));
#27498=CARTESIAN_POINT('Ctrl Pts',(126.967633039461,-33.4846467977137,27.5457844326971));
#27499=CARTESIAN_POINT('Ctrl Pts',(126.995110796069,-33.4310038762966,27.5422370537086));
#27500=CARTESIAN_POINT('Ctrl Pts',(127.007474510898,-33.407549303618,27.5406862497125));
#27501=CARTESIAN_POINT('Ctrl Pts',(127.03439841979,-33.3578944622786,27.5374025701998));
#27502=CARTESIAN_POINT('Ctrl Pts',(127.049033564782,-33.3317372775957,27.5356724784264));
#27503=CARTESIAN_POINT('Ctrl Pts',(127.089444626059,-33.2617073529145,27.5310372553567));
#27504=CARTESIAN_POINT('Ctrl Pts',(127.115865074307,-33.2182143731757,27.528155039862));
#27505=CARTESIAN_POINT('Ctrl Pts',(127.276916839641,-32.9660679721129,27.5113907461457));
#27506=CARTESIAN_POINT('Ctrl Pts',(127.433164698986,-32.7721245466826,27.4983412475447));
#27507=CARTESIAN_POINT('Ctrl Pts',(127.6938938942,-32.5127222757983,27.4788112128993));
#27508=CARTESIAN_POINT('Ctrl Pts',(127.782970553315,-32.4330069977381,27.4724364634655));
#27509=CARTESIAN_POINT('Ctrl Pts',(127.927791128568,-32.3165766608859,27.4622037115341));
#27510=CARTESIAN_POINT('Ctrl Pts',(127.980726504992,-32.2765199054924,27.4584877494638));
#27511=CARTESIAN_POINT('Ctrl Pts',(128.053367195339,-32.224834226741,27.4533708578985));
#27512=CARTESIAN_POINT('Ctrl Pts',(128.072066789466,-32.2118110142414,27.4520521103479));
#27513=CARTESIAN_POINT('Ctrl Pts',(128.103595706058,-32.1903217208418,27.4498235219002));
#27514=CARTESIAN_POINT('Ctrl Pts',(128.116354260353,-32.1817523176812,27.4489203116299));
#27515=CARTESIAN_POINT('Ctrl Pts',(128.142946284133,-32.1641527806685,27.4470340585967));
#27516=CARTESIAN_POINT('Ctrl Pts',(128.156788093335,-32.1551365943247,27.4460502453972));
#27517=CARTESIAN_POINT('Ctrl Pts',(128.194502751086,-32.1309610563538,27.443365535753));
#27518=CARTESIAN_POINT('Ctrl Pts',(128.218499785379,-32.1159990208538,27.4416528820377));
#27519=CARTESIAN_POINT('Ctrl Pts',(128.366369978479,-32.0263523719625,27.4310858609728));
#27520=CARTESIAN_POINT('Ctrl Pts',(128.494721781097,-31.9593656735746,27.4218618191689));
#27521=CARTESIAN_POINT('Ctrl Pts',(128.856277882206,-31.7991842829979,27.3964273346959));
#27522=CARTESIAN_POINT('Ctrl Pts',(129.096214989827,-31.7233360766284,27.3801975822387));
#27523=CARTESIAN_POINT('Ctrl Pts',(129.409307172233,-31.6614154860398,27.3605736877328));
#27524=CARTESIAN_POINT('Ctrl Pts',(129.476658769481,-31.6501970910915,27.3564345310392));
#27525=CARTESIAN_POINT('Ctrl Pts',(129.577059300003,-31.6365763450943,27.3503837246341));
#27526=CARTESIAN_POINT('Ctrl Pts',(129.609875655481,-31.6326121948958,27.3484246787697));
#27527=CARTESIAN_POINT('Ctrl Pts',(129.669050647453,-31.6263406641625,27.3449244911459));
#27528=CARTESIAN_POINT('Ctrl Pts',(129.695387918909,-31.6238607364222,27.343378147041));
#27529=CARTESIAN_POINT('Ctrl Pts',(129.752086981207,-31.6191908297352,27.3400728226625));
#27530=CARTESIAN_POINT('Ctrl Pts',(129.782454829864,-31.6171009922646,27.3383170530493));
#27531=CARTESIAN_POINT('Ctrl Pts',(129.86582498547,-31.6124909845331,27.3335341136556));
#27532=CARTESIAN_POINT('Ctrl Pts',(129.9188658456,-31.6108057094804,27.3305325064398));
#27533=CARTESIAN_POINT('Ctrl Pts',(130.164975732085,-31.6087673880729,27.3167653520169));
#27534=CARTESIAN_POINT('Ctrl Pts',(130.35781472556,-31.6236626908488,27.3064610251735));
#27535=CARTESIAN_POINT('Ctrl Pts',(130.70331540003,-31.6802994820465,27.287889929921));
#27536=CARTESIAN_POINT('Ctrl Pts',(130.856318214848,-31.7164382169579,27.2796161127852));
#27537=CARTESIAN_POINT('Ctrl Pts',(131.080200314196,-31.7860353878578,27.2667911049631));
#27538=CARTESIAN_POINT('Ctrl Pts',(131.153330248597,-31.8115475777353,27.2624808425103));
#27539=CARTESIAN_POINT('Ctrl Pts',(131.24789027011,-31.8482146700501,27.2566707961217));
#27540=CARTESIAN_POINT('Ctrl Pts',(131.27017012622,-31.8571273215863,27.2552842540382));
#27541=CARTESIAN_POINT('Ctrl Pts',(131.306778848797,-31.8722248149294,27.2529738928787));
#27542=CARTESIAN_POINT('Ctrl Pts',(131.321163441263,-31.8782735999672,27.2520578237541));
#27543=CARTESIAN_POINT('Ctrl Pts',(131.348522531862,-31.890001186762,27.2502987669395));
#27544=CARTESIAN_POINT('Ctrl Pts',(131.361504125982,-31.8956623675598,27.2494569130484));
#27545=CARTESIAN_POINT('Ctrl Pts',(131.39688129249,-31.9113546817793,27.2471437447665));
#27546=CARTESIAN_POINT('Ctrl Pts',(131.419203573381,-31.9215477284648,27.2456632882036));
#27547=CARTESIAN_POINT('Ctrl Pts',(131.51009030064,-31.9642480191422,27.2395554289301));
#27548=CARTESIAN_POINT('Ctrl Pts',(131.57766057147,-31.9988088587972,27.2348267945692));
#27549=CARTESIAN_POINT('Ctrl Pts',(131.824595584461,-32.1357553206266,27.2169825853644));
#27550=CARTESIAN_POINT('Ctrl Pts',(131.995651137573,-32.2521964279902,27.2035098746665));
#27551=CARTESIAN_POINT('Ctrl Pts',(132.239222285499,-32.4528093100334,27.1833680636472));
#27552=CARTESIAN_POINT('Ctrl Pts',(132.320007305528,-32.5261636749289,27.1764933248361));
#27553=CARTESIAN_POINT('Ctrl Pts',(132.450678501914,-32.6568572817911,27.1650801803098));
#27554=CARTESIAN_POINT('Ctrl Pts',(132.502428549926,-32.7122072594907,27.160472005428));
#27555=CARTESIAN_POINT('Ctrl Pts',(132.574882752124,-32.7951047301561,27.1538860261557));
#27556=CARTESIAN_POINT('Ctrl Pts',(132.59708822907,-32.821303784652,27.1518477678726));
#27557=CARTESIAN_POINT('Ctrl Pts',(132.635764219446,-32.8683672425936,27.14826064464));
#27558=CARTESIAN_POINT('Ctrl Pts',(132.652394390311,-32.8890960962418,27.1467054933274));
#27559=CARTESIAN_POINT('Ctrl Pts',(132.687049828737,-32.933348993048,27.1434363795027));
#27560=CARTESIAN_POINT('Ctrl Pts',(132.705013905189,-32.9569182542266,27.141724881642));
#27561=CARTESIAN_POINT('Ctrl Pts',(132.752799486374,-33.0213492718809,27.1371232775701));
#27562=CARTESIAN_POINT('Ctrl Pts',(132.782019764605,-33.062648684945,27.1342559765518));
#27563=CARTESIAN_POINT('Ctrl Pts',(132.974684132486,-33.3483099866243,27.1149359097818));
#27564=CARTESIAN_POINT('Ctrl Pts',(133.10665403177,-33.6123652264817,27.0997163155911));
#27565=CARTESIAN_POINT('Ctrl Pts',(133.232303184815,-33.9749724160016,27.0791816976117));
#27566=CARTESIAN_POINT('Ctrl Pts',(133.25831508641,-34.060933199699,27.0743268618067));
#27567=CARTESIAN_POINT('Ctrl Pts',(133.290484324365,-34.1847843619575,27.0672264698843));
#27568=CARTESIAN_POINT('Ctrl Pts',(133.299459800818,-34.2219071846226,27.0650848523721));
#27569=CARTESIAN_POINT('Ctrl Pts',(133.314351099898,-34.2883970378607,27.0612127434705));
#27570=CARTESIAN_POINT('Ctrl Pts',(133.320508548394,-34.3177061928561,27.0594934216268));
#27571=CARTESIAN_POINT('Ctrl Pts',(133.3295269608,-34.3636510038532,27.0567734091824));
#27572=CARTESIAN_POINT('Ctrl Pts',(133.332653519902,-34.3802336589864,27.05578665987));
#27573=CARTESIAN_POINT('Ctrl Pts',(133.338362279986,-34.4118047435323,27.0538973080747));
#27574=CARTESIAN_POINT('Ctrl Pts',(133.340967615793,-34.4267882348552,27.0529959536205));
#27575=CARTESIAN_POINT('Ctrl Pts',(133.34650445416,-34.4599517555191,27.0509911964642));
#27576=CARTESIAN_POINT('Ctrl Pts',(133.349388806334,-34.4781391383884,27.0498853343631));
#27577=CARTESIAN_POINT('Ctrl Pts',(133.358842373799,-34.5410587327454,27.0460395179882));
#27578=CARTESIAN_POINT('Ctrl Pts',(133.364664480301,-34.5858965116578,27.0432639821675));
#27579=CARTESIAN_POINT('Ctrl Pts',(133.392456374922,-34.8395695690365,27.0274133846477));
#27580=CARTESIAN_POINT('Ctrl Pts',(133.395879099278,-35.0499676985824,27.0137349000843));
#27581=CARTESIAN_POINT('Ctrl Pts',(133.364753837455,-35.4556344683181,26.9876028523466));
#27582=CARTESIAN_POINT('Ctrl Pts',(133.332614428017,-35.6502864669629,26.9751760355249));
#27583=CARTESIAN_POINT('Ctrl Pts',(133.272601936296,-35.8845902202759,26.9605506438904));
#27584=CARTESIAN_POINT('Ctrl Pts',(133.260590714406,-35.9278856474808,26.9578608371576));
#27585=CARTESIAN_POINT('Ctrl Pts',(133.239568290055,-35.9982047324122,26.953511229768));
#27586=CARTESIAN_POINT('Ctrl Pts',(133.231071230352,-36.025375137211,26.9518352933306));
#27587=CARTESIAN_POINT('Ctrl Pts',(133.213861833918,-36.0780649773579,26.9485934408178));
#27588=CARTESIAN_POINT('Ctrl Pts',(133.205185302647,-36.1035937749889,26.9470265124761));
#27589=CARTESIAN_POINT('Ctrl Pts',(133.183858764982,-36.1639684117867,26.9433284271286));
#27590=CARTESIAN_POINT('Ctrl Pts',(133.170939802831,-36.1987159876285,26.9412061841352));
#27591=CARTESIAN_POINT('Ctrl Pts',(133.125426933817,-36.3152416350341,26.9341034775999));
#27592=CARTESIAN_POINT('Ctrl Pts',(133.09021738324,-36.3959628675105,26.9292081541935));
#27593=CARTESIAN_POINT('Ctrl Pts',(132.933585480935,-36.7199980722284,26.9095083337712));
#27594=CARTESIAN_POINT('Ctrl Pts',(132.786260944704,-36.9496301319206,26.8955150832843));
#27595=CARTESIAN_POINT('Ctrl Pts',(132.570860801857,-37.210311453422,26.8772038588778));
#27596=CARTESIAN_POINT('Ctrl Pts',(132.52713451787,-37.2601752661838,26.873569072913));
#27597=CARTESIAN_POINT('Ctrl Pts',(132.45131084207,-37.3416890094502,26.8673394145487));
#27598=CARTESIAN_POINT('Ctrl Pts',(132.419992910924,-37.3740400525759,26.8647857679079));
#27599=CARTESIAN_POINT('Ctrl Pts',(132.374025576047,-37.4196689113159,26.8610482507724));
#27600=CARTESIAN_POINT('Ctrl Pts',(132.359888633793,-37.4334585822378,26.859900194323));
#27601=CARTESIAN_POINT('Ctrl Pts',(132.334844298097,-37.4574642374002,26.8578670379586));
#27602=CARTESIAN_POINT('Ctrl Pts',(132.323988590493,-37.467732844832,26.8569858960968));
#27603=CARTESIAN_POINT('Ctrl Pts',(132.2998481233,-37.4902671688812,26.8550264158087));
#27604=CARTESIAN_POINT('Ctrl Pts',(132.286533072077,-37.5024984396797,26.8539457722239));
#27605=CARTESIAN_POINT('Ctrl Pts',(132.246519125892,-37.5386694969125,26.8507003892999));
#27606=CARTESIAN_POINT('Ctrl Pts',(132.219538308561,-37.562292035229,26.8485148773444));
#27607=CARTESIAN_POINT('Ctrl Pts',(132.078641501372,-37.6817562380133,26.8371386478315));
#27608=CARTESIAN_POINT('Ctrl Pts',(131.958883665927,-37.7704394633191,26.8275975467818));
#27609=CARTESIAN_POINT('Ctrl Pts',(131.726035903215,-37.9202039314815,26.8097642153179));
#27610=CARTESIAN_POINT('Ctrl Pts',(131.614535293586,-37.98329830662,26.8014972020417));
#27611=CARTESIAN_POINT('Ctrl Pts',(131.364972910286,-38.1064181195044,26.7837926976329));
#27612=CARTESIAN_POINT('Ctrl Pts',(131.225931158269,-38.1638721465648,26.7744242765136));
#27613=CARTESIAN_POINT('Ctrl Pts',(131.043074643412,-38.2255576705999,26.7627783238998));
#27614=CARTESIAN_POINT('Ctrl Pts',(131.002374441645,-38.2384367719991,26.7602266865295));
#27615=CARTESIAN_POINT('Ctrl Pts',(130.934579756203,-38.2584889681723,26.7560414116201));
#27616=CARTESIAN_POINT('Ctrl Pts',(130.907621091163,-38.2661006876111,26.7543939169789));
#27617=CARTESIAN_POINT('Ctrl Pts',(130.854576924671,-38.2803700868507,26.7511841091669));
#27618=CARTESIAN_POINT('Ctrl Pts',(130.828500400175,-38.28705290115,26.7496210990796));
#27619=CARTESIAN_POINT('Ctrl Pts',(130.770907154633,-38.3010838094103,26.7462004809165));
#27620=CARTESIAN_POINT('Ctrl Pts',(130.739359042992,-38.3082926813406,26.7443473595146));
#27621=CARTESIAN_POINT('Ctrl Pts',(130.629177908061,-38.3318146524044,26.7379423714849));
#27622=CARTESIAN_POINT('Ctrl Pts',(130.550069534292,-38.3457851949272,26.7334625747005));
#27623=CARTESIAN_POINT('Ctrl Pts',(130.191966373627,-38.3959798531437,26.7135917969621));
#27624=CARTESIAN_POINT('Ctrl Pts',(129.90964159175,-38.4001994052375,26.6991313994537));
#27625=CARTESIAN_POINT('Ctrl Pts',(129.563437805498,-38.3621880918611,26.6802803767095));
#27626=CARTESIAN_POINT('Ctrl Pts',(129.497063482505,-38.3529016199872,26.6766089048678));
#27627=CARTESIAN_POINT('Ctrl Pts',(129.386294668133,-38.3340408512872,26.670323126022));
#27628=CARTESIAN_POINT('Ctrl Pts',(129.341737353693,-38.3255304105277,26.6677510175765));
#27629=CARTESIAN_POINT('Ctrl Pts',(129.277991335347,-38.3120236715448,26.6639912705699));
#27630=CARTESIAN_POINT('Ctrl Pts',(129.258653031287,-38.3077487727487,26.6628400365185));
#27631=CARTESIAN_POINT('Ctrl Pts',(129.224787165396,-38.2999505392557,26.6608034710753));
#27632=CARTESIAN_POINT('Ctrl Pts',(129.210243718083,-38.2965001901647,26.6599221477652));
#27633=CARTESIAN_POINT('Ctrl Pts',(129.178199944245,-38.2886737614959,26.6579650546773));
#27634=CARTESIAN_POINT('Ctrl Pts',(129.160711652075,-38.2842541737943,26.6568870193113));
#27635=CARTESIAN_POINT('Ctrl Pts',(129.108772226055,-38.2706862705814,26.6536574094168));
#27636=CARTESIAN_POINT('Ctrl Pts',(129.074430239311,-38.2611341626483,26.6514853470934));
#27637=CARTESIAN_POINT('Ctrl Pts',(128.901591868381,-38.2101098613569,26.6403892496618));
#27638=CARTESIAN_POINT('Ctrl Pts',(128.765708177188,-38.1603516915279,26.631134310759));
#27639=CARTESIAN_POINT('Ctrl Pts',(128.520061010398,-38.0521356138726,26.6138492845831));
#27640=CARTESIAN_POINT('Ctrl Pts',(128.409514105401,-37.9960152615364,26.6058450916093));
#27641=CARTESIAN_POINT('Ctrl Pts',(128.210943111251,-37.8811139433955,26.5912199342369));
#27642=CARTESIAN_POINT('Ctrl Pts',(128.12211323902,-37.8240195418498,26.5845766547595));
#27643=CARTESIAN_POINT('Ctrl Pts',(127.975712549297,-37.7199544202773,26.5734947773514));
#27644=CARTESIAN_POINT('Ctrl Pts',(127.91675866483,-37.6750698194147,26.5689917772688));
#27645=CARTESIAN_POINT('Ctrl Pts',(127.832909850094,-37.6067768373599,26.5625251229662));
#27646=CARTESIAN_POINT('Ctrl Pts',(127.806825414567,-37.5848695445709,26.5605040682418));
#27647=CARTESIAN_POINT('Ctrl Pts',(127.761008902725,-37.5451971367022,26.5569360654727));
#27648=CARTESIAN_POINT('Ctrl Pts',(127.741147306139,-37.5275866286352,26.5553830670236));
#27649=CARTESIAN_POINT('Ctrl Pts',(127.699437937586,-37.4897202052171,26.5521073236154));
#27650=CARTESIAN_POINT('Ctrl Pts',(127.67764613392,-37.469405820383,26.5503871927245));
#27651=CARTESIAN_POINT('Ctrl Pts',(127.619029212581,-37.4133006200849,26.5457339955877));
#27652=CARTESIAN_POINT('Ctrl Pts',(127.582744288737,-37.3769554031527,26.5428246541864));
#27653=CARTESIAN_POINT('Ctrl Pts',(127.37506018272,-37.159249778047,26.5259640357805));
#27654=CARTESIAN_POINT('Ctrl Pts',(127.223284317831,-36.9602371688749,26.5128546183194));
#27655=CARTESIAN_POINT('Ctrl Pts',(127.033529265057,-36.6445557707527,26.4932943162819));
#27656=CARTESIAN_POINT('Ctrl Pts',(126.97773452637,-36.539617010713,26.486954496472));
#27657=CARTESIAN_POINT('Ctrl Pts',(126.899623154708,-36.3720216719875,26.4767706597061));
#27658=CARTESIAN_POINT('Ctrl Pts',(126.873443784974,-36.3112685252105,26.473067067287));
#27659=CARTESIAN_POINT('Ctrl Pts',(126.840668249408,-36.2286358233001,26.4679646764145));
#27660=CARTESIAN_POINT('Ctrl Pts',(126.832490101244,-36.2073955761962,26.4666474674454));
#27661=CARTESIAN_POINT('Ctrl Pts',(126.819150756607,-36.1716822147994,26.4644207193171));
#27662=CARTESIAN_POINT('Ctrl Pts',(126.81387279523,-36.1572530188819,26.4635177858885));
#27663=CARTESIAN_POINT('Ctrl Pts',(126.803120698791,-36.1272271302625,26.4616312276648));
#27664=CARTESIAN_POINT('Ctrl Pts',(126.797662295291,-36.1116255977065,26.460646821896));
#27665=CARTESIAN_POINT('Ctrl Pts',(126.783160633895,-36.0691827653424,26.457958801183));
#27666=CARTESIAN_POINT('Ctrl Pts',(126.774339539014,-36.0422676092873,26.4562433822108));
#27667=CARTESIAN_POINT('Ctrl Pts',(126.72019381854,-35.8697823310236,26.4451953637472));
#27668=CARTESIAN_POINT('Ctrl Pts',(126.684400509325,-35.721416265381,26.4354519754617));
#27669=CARTESIAN_POINT('Ctrl Pts',(126.62660463481,-35.3833111756366,26.413372798666));
#27670=CARTESIAN_POINT('Ctrl Pts',(126.610389780889,-35.1930722355296,26.4010493342579));
#27671=CARTESIAN_POINT('Ctrl Pts',(126.610175022661,-34.8983352556159,26.3825794060772));
#27672=CARTESIAN_POINT('Ctrl Pts',(126.614897717059,-34.7942452572275,26.3761707671459));
#27673=CARTESIAN_POINT('Ctrl Pts',(126.628005360703,-34.6512718640806,26.3675336110191));
#27674=CARTESIAN_POINT('Ctrl Pts',(126.632289101672,-34.6120790515124,26.3651828664172));
#27675=CARTESIAN_POINT('Ctrl Pts',(126.640359982631,-34.5485232826407,26.3613969628748));
#27676=CARTESIAN_POINT('Ctrl Pts',(126.643730790616,-34.5241120776792,26.3599491071496));
#27677=CARTESIAN_POINT('Ctrl Pts',(126.651397939722,-34.4727286025183,26.3569140105945));
#27678=CARTESIAN_POINT('Ctrl Pts',(126.655754678625,-34.4457670354514,26.3553287608552));
#27679=CARTESIAN_POINT('Ctrl Pts',(126.6671336537,-34.3803768772537,26.351500319755));
#27680=CARTESIAN_POINT('Ctrl Pts',(126.674495322243,-34.3420108566249,26.3492678374341));
#27681=CARTESIAN_POINT('Ctrl Pts',(126.705097450401,-34.1961921307263,26.3408264962036));
#27682=CARTESIAN_POINT('Ctrl Pts',(126.7328975702,-34.0897611642596,26.3347590711471));
#27683=CARTESIAN_POINT('Ctrl Pts',(126.782934654739,-33.9303456417629,26.3256968410527));
#27684=CARTESIAN_POINT('Ctrl Pts',(126.801414529506,-33.8762938999873,26.3226281947471));
#27685=CARTESIAN_POINT('Ctrl Pts',(126.821241846765,-33.8227567516686,26.3195780637354));
#27686=CARTESIAN_POINT('',(126.610250231881,-34.9987461903623,26.7339821967504));
#27687=CARTESIAN_POINT('Ctrl Pts',(126.821241917671,-33.8227565602112,26.6607167036746));
#27688=CARTESIAN_POINT('Ctrl Pts',(126.808026128393,-33.8584414453932,26.6630833269527));
#27689=CARTESIAN_POINT('Ctrl Pts',(126.795411679185,-33.8943476869306,26.6654723265988));
#27690=CARTESIAN_POINT('Ctrl Pts',(126.733599981728,-34.080243728041,26.6778554664346));
#27691=CARTESIAN_POINT('Ctrl Pts',(126.694320202069,-34.2333191535549,26.6880905081309));
#27692=CARTESIAN_POINT('Ctrl Pts',(126.628948778195,-34.5897919147975,26.7113996454761));
#27693=CARTESIAN_POINT('Ctrl Pts',(126.610336083526,-34.7939598524325,26.7243514856095));
#27694=CARTESIAN_POINT('Ctrl Pts',(126.610250297903,-34.9985788622999,26.7367448338284));
#27695=CARTESIAN_POINT('Ctrl Pts',(126.610250231881,-34.9987461903623,26.7339821967504));
#27696=CARTESIAN_POINT('Ctrl Pts',(126.610210918892,-35.1050312211208,26.7401898652714));
#27697=CARTESIAN_POINT('Ctrl Pts',(126.615174777716,-35.2112871242203,26.7463975337923));
#27698=CARTESIAN_POINT('Ctrl Pts',(126.625107297085,-35.3170241415319,26.7526052023133));
#27699=CARTESIAN_POINT('Ctrl Pts',(126.63504515388,-35.4228179786101,26.7588162066412));
#27700=CARTESIAN_POINT('Ctrl Pts',(126.649956949814,-35.5280919745356,26.7650272109691));
#27701=CARTESIAN_POINT('Ctrl Pts',(126.669756487617,-35.6323631952676,26.771238215297));
#27702=CARTESIAN_POINT('Ctrl Pts',(126.689810649996,-35.7379753571683,26.777529093931));
#27703=CARTESIAN_POINT('Ctrl Pts',(126.714879066237,-35.8425583544692,26.783819972565));
#27704=CARTESIAN_POINT('Ctrl Pts',(126.744819612008,-35.9456245048278,26.790110851199));
#27705=CARTESIAN_POINT('Ctrl Pts',(126.774450142078,-36.0476234694036,26.7963365917036));
#27706=CARTESIAN_POINT('Ctrl Pts',(126.808852175912,-36.1481364947945,26.8025623322082));
#27707=CARTESIAN_POINT('Ctrl Pts',(126.847839093249,-36.2467103434447,26.8087880727127));
#27708=CARTESIAN_POINT('Ctrl Pts',(126.887437873914,-36.3468312167672,26.8151115204114));
#27709=CARTESIAN_POINT('Ctrl Pts',(126.931766482523,-36.4449511376652,26.8214349681101));
#27710=CARTESIAN_POINT('Ctrl Pts',(126.980581021134,-36.540621333283,26.8277584158088));
#27711=CARTESIAN_POINT('Ctrl Pts',(127.029395559746,-36.6362915289008,26.8340818635075));
#27712=CARTESIAN_POINT('Ctrl Pts',(127.082695759616,-36.7295116605695,26.8404053112062));
#27713=CARTESIAN_POINT('Ctrl Pts',(127.140192688407,-36.8198646111885,26.8467287589049));
#27714=CARTESIAN_POINT('Ctrl Pts',(127.195672875856,-36.9070483746075,26.8528304076544));
#27715=CARTESIAN_POINT('Ctrl Pts',(127.255237266505,-36.991840115881,26.8589320564039));
#27716=CARTESIAN_POINT('Ctrl Pts',(127.318653174035,-37.0738332289239,26.8650337051533));
#27717=CARTESIAN_POINT('Ctrl Pts',(127.381985666394,-37.1557184909589,26.8711273279974));
#27718=CARTESIAN_POINT('Ctrl Pts',(127.449159344426,-37.2348121076691,26.8772209508415));
#27719=CARTESIAN_POINT('Ctrl Pts',(127.519897363522,-37.3107349426182,26.8833145736856));
#27720=CARTESIAN_POINT('Ctrl Pts',(127.590562576443,-37.3865796349879,26.8894019247485));
#27721=CARTESIAN_POINT('Ctrl Pts',(127.664784545446,-37.4592597237484,26.8954892758114));
#27722=CARTESIAN_POINT('Ctrl Pts',(127.742245693181,-37.5284284748709,26.9015766268743));
#27723=CARTESIAN_POINT('Ctrl Pts',(127.819651737321,-37.5975480213678,26.9076596475738));
#27724=CARTESIAN_POINT('Ctrl Pts',(127.900292059853,-37.6631609133593,26.9137426682733));
#27725=CARTESIAN_POINT('Ctrl Pts',(127.983812297837,-37.7249572862979,26.9198256889727));
#27726=CARTESIAN_POINT('Ctrl Pts',(128.067301613337,-37.7867307797833,26.9259064574982));
#27727=CARTESIAN_POINT('Ctrl Pts',(128.153668381677,-37.8446903083731,26.9319872260236));
#27728=CARTESIAN_POINT('Ctrl Pts',(128.242525864358,-37.8985668398449,26.938067994549));
#27729=CARTESIAN_POINT('Ctrl Pts',(128.33137346955,-37.9524373823466,26.9441480871301));
#27730=CARTESIAN_POINT('Ctrl Pts',(128.422710872761,-38.0022256084781,26.9502281797111));
#27731=CARTESIAN_POINT('Ctrl Pts',(128.516123897908,-38.0477068061314,26.9563082722921));
#27732=CARTESIAN_POINT('Ctrl Pts',(128.609550740135,-38.0931947310841,26.9623892642031));
#27733=CARTESIAN_POINT('Ctrl Pts',(128.705053429628,-38.1343741745972,26.9684702561141));
#27734=CARTESIAN_POINT('Ctrl Pts',(128.802195670963,-38.1710676201936,26.974551248025));
#27735=CARTESIAN_POINT('Ctrl Pts',(128.89943874179,-38.2077991520172,26.9806385517455));
#27736=CARTESIAN_POINT('Ctrl Pts',(128.998324362134,-38.2400352355096,26.986725855466));
#27737=CARTESIAN_POINT('Ctrl Pts',(129.098398877858,-38.2676475451083,26.9928131591865));
#27738=CARTESIAN_POINT('Ctrl Pts',(129.198527160484,-38.2952746899358,26.9989037334245));
#27739=CARTESIAN_POINT('Ctrl Pts',(129.299845193629,-38.3182730178205,27.0049943076626));
#27740=CARTESIAN_POINT('Ctrl Pts',(129.401888827044,-38.3365653129057,27.0110848819006));
#27741=CARTESIAN_POINT('Ctrl Pts',(129.504099053358,-38.3548874713577,27.0171853993991));
#27742=CARTESIAN_POINT('Ctrl Pts',(129.60703682202,-38.3684881927925,27.0232859168975));
#27743=CARTESIAN_POINT('Ctrl Pts',(129.710232315234,-38.3773421134622,27.0293864343959));
#27744=CARTESIAN_POINT('Ctrl Pts',(129.791551230606,-38.3843190773123,27.0341936934217));
#27745=CARTESIAN_POINT('Ctrl Pts',(129.873030044153,-38.3883495206598,27.0390009524475));
#27746=CARTESIAN_POINT('Ctrl Pts',(129.954440018181,-38.389443811388,27.0438082114734));
#27747=CARTESIAN_POINT('Ctrl Pts',(130.057770259678,-38.3908327483895,27.0499098623092));
#27748=CARTESIAN_POINT('Ctrl Pts',(130.16133869337,-38.3874945526483,27.0560115131451));
#27749=CARTESIAN_POINT('Ctrl Pts',(130.264677695181,-38.3794009498983,27.062113163981));
#27750=CARTESIAN_POINT('Ctrl Pts',(130.367880768739,-38.3713179931702,27.0682067889339));
#27751=CARTESIAN_POINT('Ctrl Pts',(130.470854587525,-38.358492097902,27.0743004138869));
#27752=CARTESIAN_POINT('Ctrl Pts',(130.573130296352,-38.340946980409,27.0803940388398));
#27753=CARTESIAN_POINT('Ctrl Pts',(130.675300739611,-38.3234199209353,27.0864813920309));
#27754=CARTESIAN_POINT('Ctrl Pts',(130.776774082327,-38.3011833697077,27.092568745222));
#27755=CARTESIAN_POINT('Ctrl Pts',(130.877086241575,-38.274312872549,27.0986560984131));
#27756=CARTESIAN_POINT('Ctrl Pts',(130.977327042043,-38.2474614901803,27.1047391212609));
#27757=CARTESIAN_POINT('Ctrl Pts',(131.076407889687,-38.2159828274786,27.1108221441086));
#27758=CARTESIAN_POINT('Ctrl Pts',(131.173875373655,-38.1800034071721,27.1169051669564));
#27759=CARTESIAN_POINT('Ctrl Pts',(131.271306771517,-38.1440373077922,27.1229859376417));
#27760=CARTESIAN_POINT('Ctrl Pts',(131.367125592008,-38.1035739105461,27.129066708327));
#27761=CARTESIAN_POINT('Ctrl Pts',(131.460894828175,-38.0587891989333,27.1351474790123));
#27762=CARTESIAN_POINT('Ctrl Pts',(131.554653641,-38.0140094655672,27.141227573762));
#27763=CARTESIAN_POINT('Ctrl Pts',(131.646362936558,-37.9649095573695,27.1473076685118));
#27764=CARTESIAN_POINT('Ctrl Pts',(131.735607735692,-37.911712700509,27.1533877632616));
#27765=CARTESIAN_POINT('Ctrl Pts',(131.824865735456,-37.8585079750444,27.1594687573475));
#27766=CARTESIAN_POINT('Ctrl Pts',(131.911658147093,-37.8012053159886,27.1655497514335));
#27767=CARTESIAN_POINT('Ctrl Pts',(131.995597339505,-37.7400723204073,27.1716307455195));
#27768=CARTESIAN_POINT('Ctrl Pts',(132.079623657122,-37.6788758714532,27.177718051411));
#27769=CARTESIAN_POINT('Ctrl Pts',(132.160790494676,-37.6138413984369,27.1838053573026));
#27770=CARTESIAN_POINT('Ctrl Pts',(132.238741847519,-37.5452779814131,27.1898926631942));
#27771=CARTESIAN_POINT('Ctrl Pts',(132.316735081181,-37.4766777274143,27.1959832396044));
#27772=CARTESIAN_POINT('Ctrl Pts',(132.391509081025,-37.4045450497778,27.2020738160146));
#27773=CARTESIAN_POINT('Ctrl Pts',(132.462744835503,-37.3292258236812,27.2081643924249));
#27774=CARTESIAN_POINT('Ctrl Pts',(132.534096886719,-37.2537836343285,27.2142649120746));
#27775=CARTESIAN_POINT('Ctrl Pts',(132.601898873521,-37.1751448282075,27.2203654317244));
#27776=CARTESIAN_POINT('Ctrl Pts',(132.665872045227,-37.0936884441047,27.2264659513742));
#27777=CARTESIAN_POINT('Ctrl Pts',(132.716283198907,-37.0295004386057,27.2312731889301));
#27778=CARTESIAN_POINT('Ctrl Pts',(132.7643176392,-36.963563539714,27.236080426486));
#27779=CARTESIAN_POINT('Ctrl Pts',(132.80985865339,-36.8960747375742,27.2408876640418));
#27780=CARTESIAN_POINT('Ctrl Pts',(132.867662092612,-36.8104138241755,27.2469893038236));
#27781=CARTESIAN_POINT('Ctrl Pts',(132.921642478689,-36.7219624582929,27.2530909436055));
#27782=CARTESIAN_POINT('Ctrl Pts',(132.971519829462,-36.6310962465826,27.2591925833873));
#27783=CARTESIAN_POINT('Ctrl Pts',(133.021331573161,-36.5403495573827,27.2652861972671));
#27784=CARTESIAN_POINT('Ctrl Pts',(133.067050806911,-36.4471947089995,27.271379811147));
#27785=CARTESIAN_POINT('Ctrl Pts',(133.108440357057,-36.3520368371902,27.2774734250269));
#27786=CARTESIAN_POINT('Ctrl Pts',(133.149787307592,-36.25697690528,27.2835607671405));
#27787=CARTESIAN_POINT('Ctrl Pts',(133.186813266121,-36.1599184395919,27.2896481092541));
#27788=CARTESIAN_POINT('Ctrl Pts',(133.219327023633,-36.0612909956297,27.2957354513678));
#27789=CARTESIAN_POINT('Ctrl Pts',(133.25181765209,-35.9627337114954,27.3018184631768));
#27790=CARTESIAN_POINT('Ctrl Pts',(133.279802328967,-35.8626100736336,27.3079014749858));
#27791=CARTESIAN_POINT('Ctrl Pts',(133.303138330882,-35.7613686554859,27.3139844867949));
#27792=CARTESIAN_POINT('Ctrl Pts',(133.326465693026,-35.6601647203073,27.3200652464689));
#27793=CARTESIAN_POINT('Ctrl Pts',(133.345147704808,-35.5578442436962,27.3261460061429));
#27794=CARTESIAN_POINT('Ctrl Pts',(133.359092002414,-35.4548691919879,27.3322267658169));
#27795=CARTESIAN_POINT('Ctrl Pts',(133.373034750068,-35.3519055862728,27.3383068495957));
#27796=CARTESIAN_POINT('Ctrl Pts',(133.382240773313,-35.2482879740206,27.3443869333746));
#27797=CARTESIAN_POINT('Ctrl Pts',(133.386669295573,-35.1444857948878,27.3504670171535));
#27798=CARTESIAN_POINT('Ctrl Pts',(133.391098472917,-35.0406682609339,27.356548000322));
#27799=CARTESIAN_POINT('Ctrl Pts',(133.390748726998,-34.9366665332639,27.3626289834905));
#27800=CARTESIAN_POINT('Ctrl Pts',(133.385631382985,-34.8329515009179,27.368709966659));
#27801=CARTESIAN_POINT('Ctrl Pts',(133.380508727258,-34.7291288141581,27.374797261783));
#27802=CARTESIAN_POINT('Ctrl Pts',(133.370608611621,-34.6255938450878,27.3808845569071));
#27803=CARTESIAN_POINT('Ctrl Pts',(133.355994392891,-34.5228137707522,27.3869718520312));
#27804=CARTESIAN_POINT('Ctrl Pts',(133.341372322225,-34.4199784746777,27.3930624177408));
#27805=CARTESIAN_POINT('Ctrl Pts',(133.322031182985,-34.3178993015912,27.3991529834504));
#27806=CARTESIAN_POINT('Ctrl Pts',(133.298085384627,-34.2170326582749,27.40524354916));
#27807=CARTESIAN_POINT('Ctrl Pts',(133.27410049235,-34.1160013400358,27.4113440583296));
#27808=CARTESIAN_POINT('Ctrl Pts',(133.245496041031,-34.0161869176726,27.4174445674992));
#27809=CARTESIAN_POINT('Ctrl Pts',(133.212436246745,-33.9180303039832,27.4235450766689));
#27810=CARTESIAN_POINT('Ctrl Pts',(133.186384340782,-33.8406805525787,27.428352423316));
#27811=CARTESIAN_POINT('Ctrl Pts',(133.157566757318,-33.7643599812258,27.4331597699631));
#27812=CARTESIAN_POINT('Ctrl Pts',(133.126084283109,-33.6892742020556,27.4379671166102));
#27813=CARTESIAN_POINT('Ctrl Pts',(133.08612560333,-33.5939726515496,27.4440687725343));
#27814=CARTESIAN_POINT('Ctrl Pts',(133.041737391341,-33.5003389802669,27.4501704284584));
#27815=CARTESIAN_POINT('Ctrl Pts',(132.993080319246,-33.4088132526192,27.4562720843826));
#27816=CARTESIAN_POINT('Ctrl Pts',(132.944487249362,-33.317407915463,27.4623657143518));
#27817=CARTESIAN_POINT('Ctrl Pts',(132.891636681597,-33.2281053841537,27.4684593443211));
#27818=CARTESIAN_POINT('Ctrl Pts',(132.834737451366,-33.1413261059775,27.4745529742904));
#27819=CARTESIAN_POINT('Ctrl Pts',(132.777896784393,-33.054636144953,27.4806403324205));
#27820=CARTESIAN_POINT('Ctrl Pts',(132.717015974492,-32.9704646286416,27.4867276905507));
#27821=CARTESIAN_POINT('Ctrl Pts',(132.652349477154,-32.8892069467753,27.4928150486808));
#27822=CARTESIAN_POINT('Ctrl Pts',(132.587728982838,-32.8080070707148,27.4988980763325));
#27823=CARTESIAN_POINT('Ctrl Pts',(132.519328422117,-32.72971724075,27.5049811039842));
#27824=CARTESIAN_POINT('Ctrl Pts',(132.447444734549,-32.6547027195202,27.5110641316358));
#27825=CARTESIAN_POINT('Ctrl Pts',(132.375587661986,-32.579715972488,27.5171449070407));
#27826=CARTESIAN_POINT('Ctrl Pts',(132.300250321271,-32.5080024325567,27.5232256824457));
#27827=CARTESIAN_POINT('Ctrl Pts',(132.221768458665,-32.4398925845622,27.5293064578506));
#27828=CARTESIAN_POINT('Ctrl Pts',(132.143295321211,-32.3717903086199,27.5353865572307));
#27829=CARTESIAN_POINT('Ctrl Pts',(132.06167868008,-32.3072912083081,27.5414666566108));
#27830=CARTESIAN_POINT('Ctrl Pts',(131.977288810259,-32.2466867190011,27.5475467559908));
#27831=CARTESIAN_POINT('Ctrl Pts',(131.892886459244,-32.1860732663394,27.5536277546127));
#27832=CARTESIAN_POINT('Ctrl Pts',(131.805710412133,-32.1293558186036,27.5597087532345));
#27833=CARTESIAN_POINT('Ctrl Pts',(131.716160716455,-32.0767830292987,27.5657897518564));
#27834=CARTESIAN_POINT('Ctrl Pts',(131.626518074739,-32.0241556732814,27.5718770621103));
#27835=CARTESIAN_POINT('Ctrl Pts',(131.534497233888,-31.9756817838379,27.5779643723642));
#27836=CARTESIAN_POINT('Ctrl Pts',(131.440523658722,-31.9315644619509,27.5840516826181));
#27837=CARTESIAN_POINT('Ctrl Pts',(131.346499595917,-31.8874234378751,27.5901422633012));
#27838=CARTESIAN_POINT('Ctrl Pts',(131.25052110427,-31.8476438074137,27.5962328439843));
#27839=CARTESIAN_POINT('Ctrl Pts',(131.153032625976,-31.8123800687763,27.6023234246674));
#27840=CARTESIAN_POINT('Ctrl Pts',(131.055384994923,-31.7770587610663,27.6084239483995));
#27841=CARTESIAN_POINT('Ctrl Pts',(130.956222861508,-31.7462681998162,27.6145244721317));
#27842=CARTESIAN_POINT('Ctrl Pts',(130.856005011475,-31.7201127332132,27.6206249958638));
#27843=CARTESIAN_POINT('Ctrl Pts',(130.777033700421,-31.6995023181207,27.6254321869687));
#27844=CARTESIAN_POINT('Ctrl Pts',(130.697407165734,-31.6817690097786,27.6302393780737));
#27845=CARTESIAN_POINT('Ctrl Pts',(130.617352600343,-31.6669412202377,27.6350465691787));
#27846=CARTESIAN_POINT('Ctrl Pts',(130.515741023193,-31.6481206186452,27.6411482358038));
#27847=CARTESIAN_POINT('Ctrl Pts',(130.413096306608,-31.633919041833,27.6472499024289));
#27848=CARTESIAN_POINT('Ctrl Pts',(130.309874584419,-31.6244433341401,27.653351569054));
#27849=CARTESIAN_POINT('Ctrl Pts',(130.206788633678,-31.6149800902052,27.6594452099254));
#27850=CARTESIAN_POINT('Ctrl Pts',(130.103127608539,-31.6102303962829,27.6655388507969));
#27851=CARTESIAN_POINT('Ctrl Pts',(129.999357636771,-31.6102500608644,27.6716324916684));
#27852=CARTESIAN_POINT('Ctrl Pts',(129.895694466417,-31.6102697052069,27.6777198608849));
#27853=CARTESIAN_POINT('Ctrl Pts',(129.79192299789,-31.6150489470218,27.6838072301015));
#27854=CARTESIAN_POINT('Ctrl Pts',(129.688513408595,-31.6245917038268,27.689894599318));
#27855=CARTESIAN_POINT('Ctrl Pts',(129.585177379706,-31.6341276723923,27.6959776382848));
#27856=CARTESIAN_POINT('Ctrl Pts',(129.482203142843,-31.6484203783877,27.7020606772516));
#27857=CARTESIAN_POINT('Ctrl Pts',(129.380058966024,-31.667421692309,27.7081437162183));
#27858=CARTESIAN_POINT('Ctrl Pts',(129.277952605832,-31.6864159714132,27.7142245030741));
#27859=CARTESIAN_POINT('Ctrl Pts',(129.176676115,-31.7101153156768,27.72030528993));
#27860=CARTESIAN_POINT('Ctrl Pts',(129.076689946649,-31.7384200748898,27.7263860767858));
#27861=CARTESIAN_POINT('Ctrl Pts',(128.976714892158,-31.7667216879166,27.7324661877381));
#27862=CARTESIAN_POINT('Ctrl Pts',(128.878030286519,-31.7996275814483,27.7385462986903));
#27863=CARTESIAN_POINT('Ctrl Pts',(128.781082850265,-31.8369878209873,27.7446264096426));
#27864=CARTESIAN_POINT('Ctrl Pts',(128.684121073889,-31.8743535867208,27.7507074199434));
#27865=CARTESIAN_POINT('Ctrl Pts',(128.58889737658,-31.9161748536409,27.7567884302442));
#27866=CARTESIAN_POINT('Ctrl Pts',(128.495839017465,-31.962253334934,27.762869440545));
#27867=CARTESIAN_POINT('Ctrl Pts',(128.402684069356,-32.0083796429266,27.7689567625697));
#27868=CARTESIAN_POINT('Ctrl Pts',(128.311699331944,-32.0587717996961,27.7750440845944));
#27869=CARTESIAN_POINT('Ctrl Pts',(128.223287898296,-32.1131852899503,27.7811314066191));
#27870=CARTESIAN_POINT('Ctrl Pts',(128.134828964388,-32.1676280146015,27.7872219991414));
#27871=CARTESIAN_POINT('Ctrl Pts',(128.048946441808,-32.2260961355533,27.7933125916637));
#27872=CARTESIAN_POINT('Ctrl Pts',(127.966013176318,-32.2883026231553,27.7994031841859));
#27873=CARTESIAN_POINT('Ctrl Pts',(127.882944520295,-32.3506106643308,27.8055037197457));
#27874=CARTESIAN_POINT('Ctrl Pts',(127.802835070017,-32.4166689917352,27.8116042553054));
#27875=CARTESIAN_POINT('Ctrl Pts',(127.726023589787,-32.4861510888093,27.8177047908651));
#27876=CARTESIAN_POINT('Ctrl Pts',(127.665497969812,-32.5409013291376,27.8225118678258));
#27877=CARTESIAN_POINT('Ctrl Pts',(127.607019413902,-32.5977766009208,27.8273189447864));
#27878=CARTESIAN_POINT('Ctrl Pts',(127.550736213157,-32.6566024739796,27.8321260217471));
#27879=CARTESIAN_POINT('Ctrl Pts',(127.480210872341,-32.7303138957067,27.8381495018707));
#27880=CARTESIAN_POINT('Ctrl Pts',(127.412881597948,-32.8073526954095,27.8441729819944));
#27881=CARTESIAN_POINT('Ctrl Pts',(127.349084152318,-32.8874067521153,27.850196462118));
#27882=CARTESIAN_POINT('Ctrl Pts',(127.285385722298,-32.9673365624479,27.856210593614));
#27883=CARTESIAN_POINT('Ctrl Pts',(127.225208491823,-33.0502719824567,27.8622247251101));
#27884=CARTESIAN_POINT('Ctrl Pts',(127.168851233696,-33.1358643489396,27.8682388566061));
#27885=CARTESIAN_POINT('Ctrl Pts',(127.112544514999,-33.2213799588598,27.8742475948168));
#27886=CARTESIAN_POINT('Ctrl Pts',(127.060051206712,-33.3095474187509,27.8802563330275));
#27887=CARTESIAN_POINT('Ctrl Pts',(127.011629294196,-33.3999857540655,27.8862650712381));
#27888=CARTESIAN_POINT('Ctrl Pts',(126.96323952536,-33.4903640541445,27.8922698206976));
#27889=CARTESIAN_POINT('Ctrl Pts',(126.918915988411,-33.58300984726,27.8982745701571));
#27890=CARTESIAN_POINT('Ctrl Pts',(126.878872257577,-33.6775149611506,27.9042793196166));
#27891=CARTESIAN_POINT('Ctrl Pts',(126.858553142843,-33.7254690406571,27.9073262683069));
#27892=CARTESIAN_POINT('Ctrl Pts',(126.839335262333,-33.7739014433273,27.9103732169973));
#27893=CARTESIAN_POINT('Ctrl Pts',(126.821241915871,-33.8227565650715,27.9134201656876));
#27894=CARTESIAN_POINT('Origin',(130.,-35.,23.));
#27895=CARTESIAN_POINT('',(126.821241931958,-33.822756521634,29.1634528404117));
#27896=CARTESIAN_POINT('',(126.821241915871,-33.8227565650717,28.8235739384178));
#27897=CARTESIAN_POINT('',(126.821241915871,-33.8227565650715,23.));
#27898=CARTESIAN_POINT('',(132.573234427015,-32.7934484719078,30.));
#27899=CARTESIAN_POINT('Ctrl Pts',(132.573234427015,-32.7934484719079,29.9999999999999));
#27900=CARTESIAN_POINT('Ctrl Pts',(132.579611511435,-32.8008852949168,29.9994250391984));
#27901=CARTESIAN_POINT('Ctrl Pts',(132.585956399471,-32.8083498133881,29.9988519729851));
#27902=CARTESIAN_POINT('Ctrl Pts',(132.600007252001,-32.825026072687,29.9975804179708));
#27903=CARTESIAN_POINT('Ctrl Pts',(132.607696829063,-32.8342515035189,29.9968828466264));
#27904=CARTESIAN_POINT('Ctrl Pts',(132.637470118023,-32.8703599354667,29.9941745295691));
#27905=CARTESIAN_POINT('Ctrl Pts',(132.659189092145,-32.8975421629648,29.9921828548663));
#27906=CARTESIAN_POINT('Ctrl Pts',(132.802145611422,-33.0822183703115,29.9789321000128));
#27907=CARTESIAN_POINT('Ctrl Pts',(132.909756478062,-33.2497897358446,29.9682440386));
#27908=CARTESIAN_POINT('Ctrl Pts',(133.073150607209,-33.5613965661057,29.9491490506503));
#27909=CARTESIAN_POINT('Ctrl Pts',(133.134966297491,-33.7016099934545,29.9408058913643));
#27910=CARTESIAN_POINT('Ctrl Pts',(133.20739195755,-33.9015492648347,29.9288672165697));
#27911=CARTESIAN_POINT('Ctrl Pts',(133.226208331665,-33.9581091836126,29.9254867018423));
#27912=CARTESIAN_POINT('Ctrl Pts',(133.253211617292,-34.0470408397768,29.9201490433486));
#27913=CARTESIAN_POINT('Ctrl Pts',(133.262428340742,-34.0790883825275,29.9182211637458));
#27914=CARTESIAN_POINT('Ctrl Pts',(133.278849847665,-34.1395311560066,29.9145740152084));
#27915=CARTESIAN_POINT('Ctrl Pts',(133.286162290575,-34.1678940680356,29.9128580448567));
#27916=CARTESIAN_POINT('Ctrl Pts',(133.30192669742,-34.2324914783355,29.9089376781382));
#27917=CARTESIAN_POINT('Ctrl Pts',(133.310151375338,-34.2687770764245,29.9067268805151));
#27918=CARTESIAN_POINT('Ctrl Pts',(133.333562014955,-34.3805648282459,29.8998854252298));
#27919=CARTESIAN_POINT('Ctrl Pts',(133.346772919315,-34.4564511986565,29.8951981720216));
#27920=CARTESIAN_POINT('Ctrl Pts',(133.393620096028,-34.7930443915162,29.8741973720993));
#27921=CARTESIAN_POINT('Ctrl Pts',(133.399446949911,-35.0566731102899,29.8571068577239));
#27922=CARTESIAN_POINT('Ctrl Pts',(133.364491187454,-35.4273159581913,29.8329885651439));
#27923=CARTESIAN_POINT('Ctrl Pts',(133.348928839309,-35.5357967083164,29.8259326655496));
#27924=CARTESIAN_POINT('Ctrl Pts',(133.316043062173,-35.7059224879963,29.8150225986625));
#27925=CARTESIAN_POINT('Ctrl Pts',(133.302181718188,-35.7681569793268,29.8110656306506));
#27926=CARTESIAN_POINT('Ctrl Pts',(133.281035730172,-35.851892579397,29.8058180836199));
#27927=CARTESIAN_POINT('Ctrl Pts',(133.275279491917,-35.8737624051622,29.8044547156108));
#27928=CARTESIAN_POINT('Ctrl Pts',(133.265241320972,-35.9104068951055,29.8021841213498));
#27929=CARTESIAN_POINT('Ctrl Pts',(133.261076992772,-35.9252126603911,29.801270532542));
#27930=CARTESIAN_POINT('Ctrl Pts',(133.252324285727,-35.9555384341778,29.7994078136172));
#27931=CARTESIAN_POINT('Ctrl Pts',(133.247725271621,-35.9710548565745,29.7984593973338));
#27932=CARTESIAN_POINT('Ctrl Pts',(133.234926992402,-36.0131262363495,29.7958990232918));
#27933=CARTESIAN_POINT('Ctrl Pts',(133.226511783729,-36.039614945532,29.7942991173387));
#27934=CARTESIAN_POINT('Ctrl Pts',(133.171831395826,-36.2046705821193,29.784388228408));
#27935=CARTESIAN_POINT('Ctrl Pts',(133.116969803896,-36.3402439961798,29.7765025398196));
#27936=CARTESIAN_POINT('Ctrl Pts',(132.944943736513,-36.6971282521409,29.7553920149646));
#27937=CARTESIAN_POINT('Ctrl Pts',(132.811778273929,-36.9096690530237,29.7423700365931));
#27938=CARTESIAN_POINT('Ctrl Pts',(132.617151624161,-37.1552087535418,29.7249890956176));
#27939=CARTESIAN_POINT('Ctrl Pts',(132.576475272214,-37.2036746248411,29.7214333632558));
#27940=CARTESIAN_POINT('Ctrl Pts',(132.513621493501,-37.274444459706,29.7160308332342));
#27941=CARTESIAN_POINT('Ctrl Pts',(132.492450045524,-37.2976255756651,29.7142257692305));
#27942=CARTESIAN_POINT('Ctrl Pts',(132.453564677613,-37.339032097701,29.7109345050955));
#27943=CARTESIAN_POINT('Ctrl Pts',(132.43596180134,-37.3573588674686,29.7094531893193));
#27944=CARTESIAN_POINT('Ctrl Pts',(132.39747363265,-37.39653837362,29.7062316254048));
#27945=CARTESIAN_POINT('Ctrl Pts',(132.376518849585,-37.41731960388,29.7044883149132));
#27946=CARTESIAN_POINT('Ctrl Pts',(132.317915794874,-37.4739387567862,29.6996403548318));
#27947=CARTESIAN_POINT('Ctrl Pts',(132.279711736574,-37.5091872258359,29.696510251551));
#27948=CARTESIAN_POINT('Ctrl Pts',(132.016349635554,-37.7411940681912,29.6751226057618));
#27949=CARTESIAN_POINT('Ctrl Pts',(131.766850229018,-37.9082615466856,29.6556005379831));
#27950=CARTESIAN_POINT('Ctrl Pts',(131.382386418046,-38.0977806878159,29.6278685445383));
#27951=CARTESIAN_POINT('Ctrl Pts',(131.262808845141,-38.1484213961159,29.6195585485893));
#27952=CARTESIAN_POINT('Ctrl Pts',(131.108989185093,-38.2033850515808,29.6094929774765));
#27953=CARTESIAN_POINT('Ctrl Pts',(131.077198029626,-38.2142148967209,29.6074453913095));
#27954=CARTESIAN_POINT('Ctrl Pts',(131.029016338119,-38.2298330691815,29.6043969062004));
#27955=CARTESIAN_POINT('Ctrl Pts',(131.012742925569,-38.2349726543789,29.6033766106406));
#27956=CARTESIAN_POINT('Ctrl Pts',(130.982363649703,-38.2443155409405,29.6014901961562));
#27957=CARTESIAN_POINT('Ctrl Pts',(130.968267981001,-38.2485502620121,29.6006222024175));
#27958=CARTESIAN_POINT('Ctrl Pts',(130.935691366313,-38.2581062849303,29.5986319947837));
#27959=CARTESIAN_POINT('Ctrl Pts',(130.917191647699,-38.2633624402099,29.5975134750781));
#27960=CARTESIAN_POINT('Ctrl Pts',(130.856787385743,-38.2799703032837,29.5938963385894));
#27961=CARTESIAN_POINT('Ctrl Pts',(130.81470775166,-38.2906749245336,29.5914311190113));
#27962=CARTESIAN_POINT('Ctrl Pts',(130.564644581916,-38.3491972090907,29.577040756179));
#27963=CARTESIAN_POINT('Ctrl Pts',(130.352708317561,-38.3781001377415,29.5658758599012));
#27964=CARTESIAN_POINT('Ctrl Pts',(129.973222249421,-38.3937242997488,29.5457251332386));
#27965=CARTESIAN_POINT('Ctrl Pts',(129.806731897867,-38.3883215358424,29.5368323424307));
#27966=CARTESIAN_POINT('Ctrl Pts',(129.577289571825,-38.3639065831947,29.5240203610878));
#27967=CARTESIAN_POINT('Ctrl Pts',(129.513467688545,-38.3552700610506,29.520397961575));
#27968=CARTESIAN_POINT('Ctrl Pts',(129.417831613124,-38.3395423952033,29.514862402352));
#27969=CARTESIAN_POINT('Ctrl Pts',(129.385808589249,-38.3338014707419,29.5129906272664));
#27970=CARTESIAN_POINT('Ctrl Pts',(129.330243225254,-38.3230122462417,29.5097089245382));
#27971=CARTESIAN_POINT('Ctrl Pts',(129.306662534691,-38.3181723345035,29.5083055660848));
#27972=CARTESIAN_POINT('Ctrl Pts',(129.253411948365,-38.3066503015099,29.5051114039644));
#27973=CARTESIAN_POINT('Ctrl Pts',(129.223776715518,-38.2998192766703,29.503316056454));
#27974=CARTESIAN_POINT('Ctrl Pts',(129.143583372027,-38.2801943828873,29.4984081103108));
#27975=CARTESIAN_POINT('Ctrl Pts',(129.093223673764,-38.2666314269643,29.4952718898123));
#27976=CARTESIAN_POINT('Ctrl Pts',(128.832934569379,-38.1900472948139,29.4787729263559));
#27977=CARTESIAN_POINT('Ctrl Pts',(128.629193782588,-38.107942874097,29.4648218878101));
#27978=CARTESIAN_POINT('Ctrl Pts',(128.31810376963,-37.9460053142572,29.4422925904713));
#27979=CARTESIAN_POINT('Ctrl Pts',(128.205010172565,-37.8784954791242,29.4338250411977));
#27980=CARTESIAN_POINT('Ctrl Pts',(128.038064456554,-37.7651651766539,29.4211369636581));
#27981=CARTESIAN_POINT('Ctrl Pts',(127.981237953753,-37.7239549659096,29.4167829297808));
#27982=CARTESIAN_POINT('Ctrl Pts',(127.907174969473,-37.6666530958381,29.4111019366394));
#27983=CARTESIAN_POINT('Ctrl Pts',(127.888770577908,-37.6521059056849,29.4096897189001));
#27984=CARTESIAN_POINT('Ctrl Pts',(127.858314424734,-37.6275147922911,29.4073539528856));
#27985=CARTESIAN_POINT('Ctrl Pts',(127.846178886392,-37.6175763077851,29.40642357703));
#27986=CARTESIAN_POINT('Ctrl Pts',(127.821322530603,-37.5969301082211,29.4045194048611));
#27987=CARTESIAN_POINT('Ctrl Pts',(127.808610703635,-37.586212380994,29.4035463339465));
#27988=CARTESIAN_POINT('Ctrl Pts',(127.774414690168,-37.556947517734,29.4009291241242));
#27989=CARTESIAN_POINT('Ctrl Pts',(127.753083287517,-37.5382229960679,29.3992969924296));
#27990=CARTESIAN_POINT('Ctrl Pts',(127.627017702105,-37.4247288287836,29.3896368417002));
#27991=CARTESIAN_POINT('Ctrl Pts',(127.528044719206,-37.3237469682956,29.3819890242514));
#27992=CARTESIAN_POINT('Ctrl Pts',(127.306050963309,-37.0669580246055,29.3638540851373));
#27993=CARTESIAN_POINT('Ctrl Pts',(127.189847421728,-36.9059691949673,29.3534822868552));
#27994=CARTESIAN_POINT('Ctrl Pts',(127.050931797165,-36.6729459682225,29.3387476980586));
#27995=CARTESIAN_POINT('Ctrl Pts',(127.015534118904,-36.6089481059611,29.3347302355318));
#27996=CARTESIAN_POINT('Ctrl Pts',(126.956287445656,-36.4931391872167,29.3274678062916));
#27997=CARTESIAN_POINT('Ctrl Pts',(126.931623991883,-36.4417763002849,29.3242494566258));
#27998=CARTESIAN_POINT('Ctrl Pts',(126.895546432862,-36.3615196467383,29.3192115070047));
#27999=CARTESIAN_POINT('Ctrl Pts',(126.8832148667,-36.3330484013627,29.3174225937205));
#28000=CARTESIAN_POINT('Ctrl Pts',(126.861053491503,-36.2798928078993,29.3140776791192));
#28001=CARTESIAN_POINT('Ctrl Pts',(126.851119654777,-36.2552542751105,29.3125252832496));
#28002=CARTESIAN_POINT('Ctrl Pts',(126.829609979132,-36.2000420030781,29.309041039671));
#28003=CARTESIAN_POINT('Ctrl Pts',(126.818184886186,-36.1694127429295,29.3071044184487));
#28004=CARTESIAN_POINT('Ctrl Pts',(126.785147905498,-36.0767743224212,29.3012339886558));
#28005=CARTESIAN_POINT('Ctrl Pts',(126.764894028021,-36.0143004454116,29.2972572611331));
#28006=CARTESIAN_POINT('Ctrl Pts',(126.661228634267,-35.6597483103477,29.2745808361231));
#28007=CARTESIAN_POINT('Ctrl Pts',(126.615569562297,-35.3581038595991,29.2547105263846));
#28008=CARTESIAN_POINT('Ctrl Pts',(126.609585600672,-34.9859259006388,29.2309812864319));
#28009=CARTESIAN_POINT('Ctrl Pts',(126.610564123725,-34.9173363804271,29.2266491728853));
#28010=CARTESIAN_POINT('Ctrl Pts',(126.615680876302,-34.8027225403464,29.2195243435344));
#28011=CARTESIAN_POINT('Ctrl Pts',(126.61868003125,-34.7566688717514,29.2166924944106));
#28012=CARTESIAN_POINT('Ctrl Pts',(126.624323906089,-34.6907830767939,29.2126987695243));
#28013=CARTESIAN_POINT('Ctrl Pts',(126.62620502512,-34.670892560446,29.2115006421746));
#28014=CARTESIAN_POINT('Ctrl Pts',(126.629803079382,-34.636129328525,29.2094212137074));
#28015=CARTESIAN_POINT('Ctrl Pts',(126.631442851152,-34.6212495352094,29.2085358866884));
#28016=CARTESIAN_POINT('Ctrl Pts',(126.635258901757,-34.5886090202942,29.2066045306057));
#28017=CARTESIAN_POINT('Ctrl Pts',(126.63747728662,-34.5708540696618,29.2055607737064));
#28018=CARTESIAN_POINT('Ctrl Pts',(126.644464713786,-34.5183148045883,29.2024901713332));
#28019=CARTESIAN_POINT('Ctrl Pts',(126.649633822217,-34.4835850871588,29.2004838618329));
#28020=CARTESIAN_POINT('Ctrl Pts',(126.685445527855,-34.2662257532156,29.1880396855573));
#28021=CARTESIAN_POINT('Ctrl Pts',(126.730474293754,-34.0862647071683,29.1782250990549));
#28022=CARTESIAN_POINT('Ctrl Pts',(126.800000382245,-33.8813493953562,29.1667560690774));
#28023=CARTESIAN_POINT('Ctrl Pts',(126.810420543352,-33.851976115516,29.1651051327837));
#28024=CARTESIAN_POINT('Ctrl Pts',(126.821241931958,-33.822756521634,29.1634528404117));
#28025=CARTESIAN_POINT('',(127.462899484434,-32.7519950986681,30.));
#28026=CARTESIAN_POINT('Origin',(130.,-35.,30.));
#28027=CARTESIAN_POINT('Ctrl Pts',(127.462899484433,-32.7519950986684,30.));
#28028=CARTESIAN_POINT('Ctrl Pts',(127.478841211814,-32.7340032496596,29.9985247980324));
#28029=CARTESIAN_POINT('Ctrl Pts',(127.494973853206,-32.7161815072181,29.9970389843388));
#28030=CARTESIAN_POINT('Ctrl Pts',(127.655532556121,-32.54256038369,29.982332718974));
#28031=CARTESIAN_POINT('Ctrl Pts',(127.814107040654,-32.4004994717988,29.968479649082));
#28032=CARTESIAN_POINT('Ctrl Pts',(128.115334933663,-32.1778123164891,29.9444203697092));
#28033=CARTESIAN_POINT('Ctrl Pts',(128.25250588551,-32.0908797629625,29.9341499832904));
#28034=CARTESIAN_POINT('Ctrl Pts',(128.45155791788,-31.9839100841736,29.920297256416));
#28035=CARTESIAN_POINT('Ctrl Pts',(128.508570815153,-31.9553142916071,29.9164394224824));
#28036=CARTESIAN_POINT('Ctrl Pts',(128.595733202631,-31.9146328270807,29.9107021911106));
#28037=CARTESIAN_POINT('Ctrl Pts',(128.625302752653,-31.9013449019518,29.9087829390122));
#28038=CARTESIAN_POINT('Ctrl Pts',(128.677145548552,-31.8789360607914,29.9054637086128));
#28039=CARTESIAN_POINT('Ctrl Pts',(128.699333377025,-31.8696245605349,29.9040574879752));
#28040=CARTESIAN_POINT('Ctrl Pts',(128.749864592398,-31.8490482974775,29.9008864454266));
#28041=CARTESIAN_POINT('Ctrl Pts',(128.778264846292,-31.8379281365532,29.8991264565951));
#28042=CARTESIAN_POINT('Ctrl Pts',(128.856001255967,-31.8086940426138,29.8943666083622));
#28043=CARTESIAN_POINT('Ctrl Pts',(128.90561572349,-31.7913413546243,29.8913912147908));
#28044=CARTESIAN_POINT('Ctrl Pts',(129.145569309334,-31.7136311688059,29.877266612353));
#28045=CARTESIAN_POINT('Ctrl Pts',(129.340591592957,-31.6690148984837,29.8666083712587));
#28046=CARTESIAN_POINT('Ctrl Pts',(129.682440454129,-31.6220280860358,29.8482471185181));
#28047=CARTESIAN_POINT('Ctrl Pts',(129.827576050535,-31.6115189341251,29.8405386994585));
#28048=CARTESIAN_POINT('Ctrl Pts',(130.047103311534,-31.6097657177983,29.8284892634394));
#28049=CARTESIAN_POINT('Ctrl Pts',(130.121271913425,-31.6116082245879,29.824349898015));
#28050=CARTESIAN_POINT('Ctrl Pts',(130.219171643299,-31.6172585246066,29.8187278936532));
#28051=CARTESIAN_POINT('Ctrl Pts',(130.243012368907,-31.6188876062566,29.8173463537531));
#28052=CARTESIAN_POINT('Ctrl Pts',(130.282558175012,-31.6220102489604,29.815031123508));
#28053=CARTESIAN_POINT('Ctrl Pts',(130.298274058582,-31.6233616644061,29.8141048272922));
#28054=CARTESIAN_POINT('Ctrl Pts',(130.328354383573,-31.6261599205397,29.8123190440699));
#28055=CARTESIAN_POINT('Ctrl Pts',(130.342720117328,-31.6275889355883,29.8114605922281));
#28056=CARTESIAN_POINT('Ctrl Pts',(130.382474769113,-31.6318001172697,29.8090702732338));
#28057=CARTESIAN_POINT('Ctrl Pts',(130.407841512791,-31.6347774791618,29.8075284235628));
#28058=CARTESIAN_POINT('Ctrl Pts',(130.518019607285,-31.6489733676891,29.8007660386851));
#28059=CARTESIAN_POINT('Ctrl Pts',(130.602417394555,-31.6631130007462,29.7954173465248));
#28060=CARTESIAN_POINT('Ctrl Pts',(130.879267284407,-31.7203401710726,29.7774942745521));
#28061=CARTESIAN_POINT('Ctrl Pts',(131.068500370582,-31.7770218056226,29.764655914404));
#28062=CARTESIAN_POINT('Ctrl Pts',(131.351308686713,-31.8893971444937,29.7452544606234));
#28063=CARTESIAN_POINT('Ctrl Pts',(131.448955684109,-31.9336641162856,29.7385073746334));
#28064=CARTESIAN_POINT('Ctrl Pts',(131.611006246129,-32.0166007508257,29.7272730573135));
#28065=CARTESIAN_POINT('Ctrl Pts',(131.676519041654,-32.0529171360565,29.7227196617578));
#28066=CARTESIAN_POINT('Ctrl Pts',(131.770213909791,-32.1089924726446,29.7161887391315));
#28067=CARTESIAN_POINT('Ctrl Pts',(131.799380394573,-32.1270551459805,29.7141528423898));
#28068=CARTESIAN_POINT('Ctrl Pts',(131.850747165765,-32.1599555334545,29.7105609147107));
#28069=CARTESIAN_POINT('Ctrl Pts',(131.873055440775,-32.1746184294003,29.7089987569814));
#28070=CARTESIAN_POINT('Ctrl Pts',(131.92000067502,-32.2062752367217,29.705705628646));
#28071=CARTESIAN_POINT('Ctrl Pts',(131.944590573733,-32.2233350529725,29.7039772620414));
#28072=CARTESIAN_POINT('Ctrl Pts',(132.010884456967,-32.2706406563581,29.699305790333));
#28073=CARTESIAN_POINT('Ctrl Pts',(132.052130896932,-32.3015156293555,29.6963864161049));
#28074=CARTESIAN_POINT('Ctrl Pts',(132.289390947357,-32.487703850879,29.6794814776684));
#28075=CARTESIAN_POINT('Ctrl Pts',(132.468434798278,-32.6633820086602,29.6663382243855));
#28076=CARTESIAN_POINT('Ctrl Pts',(132.701678574942,-32.949276153876,29.6467361058599));
#28077=CARTESIAN_POINT('Ctrl Pts',(132.771921928922,-33.045267008513,29.6403887243119));
#28078=CARTESIAN_POINT('Ctrl Pts',(132.873229397983,-33.2001817236004,29.6301914059989));
#28079=CARTESIAN_POINT('Ctrl Pts',(132.907849138409,-33.2566683480162,29.6264815140026));
#28080=CARTESIAN_POINT('Ctrl Pts',(132.95214015839,-33.3339284522975,29.6213691645074));
#28081=CARTESIAN_POINT('Ctrl Pts',(132.963290077767,-33.3538415109323,29.6200481865427));
#28082=CARTESIAN_POINT('Ctrl Pts',(132.981626424686,-33.3873791058198,29.6178153262414));
#28083=CARTESIAN_POINT('Ctrl Pts',(132.98892281339,-33.4009431872959,29.6169100707665));
#28084=CARTESIAN_POINT('Ctrl Pts',(133.003830534246,-33.4291153764499,29.6150244439665));
#28085=CARTESIAN_POINT('Ctrl Pts',(133.011428224115,-33.4437299704328,29.61404333391));
#28086=CARTESIAN_POINT('Ctrl Pts',(133.031760495018,-33.4835466791367,29.6113636421677));
#28087=CARTESIAN_POINT('Ctrl Pts',(133.044286894435,-33.5088529366953,29.6096532817275));
#28088=CARTESIAN_POINT('Ctrl Pts',(133.120046781933,-33.6668399736745,29.5989443660502));
#28089=CARTESIAN_POINT('Ctrl Pts',(133.174905914532,-33.8033496357441,29.5895625758721));
#28090=CARTESIAN_POINT('Ctrl Pts',(133.281471636943,-34.1280523134781,29.5675694911915));
#28091=CARTESIAN_POINT('Ctrl Pts',(133.326152205909,-34.3180385577463,29.5549564921927));
#28092=CARTESIAN_POINT('Ctrl Pts',(133.36972174774,-34.6167908719486,29.536024700485));
#28093=CARTESIAN_POINT('Ctrl Pts',(133.380146996494,-34.7234428212229,29.5294332539337));
#28094=CARTESIAN_POINT('Ctrl Pts',(133.387437586222,-34.8689913901223,29.5206724233102));
#28095=CARTESIAN_POINT('Ctrl Pts',(133.388710411931,-34.9075955279075,29.5183707767972));
#28096=CARTESIAN_POINT('Ctrl Pts',(133.389753696899,-34.9733383841115,29.5144870565039));
#28097=CARTESIAN_POINT('Ctrl Pts',(133.389858524057,-35.0004672928326,29.5128948430668));
#28098=CARTESIAN_POINT('Ctrl Pts',(133.389411253268,-35.0554076119964,29.5096904800148));
#28099=CARTESIAN_POINT('Ctrl Pts',(133.388842527335,-35.0832168233847,29.508078967019));
#28100=CARTESIAN_POINT('Ctrl Pts',(133.386550082098,-35.1531762175458,29.504049492468));
#28101=CARTESIAN_POINT('Ctrl Pts',(133.384381706613,-35.1953077040938,29.5016453560981));
#28102=CARTESIAN_POINT('Ctrl Pts',(133.372460687514,-35.3651135568099,29.4920344302891));
#28103=CARTESIAN_POINT('Ctrl Pts',(133.356264153654,-35.4922341728441,29.4850242839034));
#28104=CARTESIAN_POINT('Ctrl Pts',(133.291253845684,-35.8427573564131,29.4658457972842));
#28105=CARTESIAN_POINT('Ctrl Pts',(133.226999465458,-36.0625712985417,29.4540203849703));
#28106=CARTESIAN_POINT('Ctrl Pts',(133.106509735553,-36.3595900471022,29.4366288513963));
#28107=CARTESIAN_POINT('Ctrl Pts',(133.06842631856,-36.4434836341209,29.4315405041469));
#28108=CARTESIAN_POINT('Ctrl Pts',(133.015626832986,-36.5482363884655,29.4248343268036));
#28109=CARTESIAN_POINT('Ctrl Pts',(133.004024775013,-36.5706292307663,29.4233795411865));
#28110=CARTESIAN_POINT('Ctrl Pts',(132.984749678343,-36.6068366625051,29.4209892164612));
#28111=CARTESIAN_POINT('Ctrl Pts',(132.977227754632,-36.6207311875072,29.4200626952523));
#28112=CARTESIAN_POINT('Ctrl Pts',(132.96289661719,-36.646767279017,29.4183081511374));
#28113=CARTESIAN_POINT('Ctrl Pts',(132.956109213911,-36.6589204729349,29.4174815623257));
#28114=CARTESIAN_POINT('Ctrl Pts',(132.937785525292,-36.6912604355233,29.4152623393041));
#28115=CARTESIAN_POINT('Ctrl Pts',(132.926116282433,-36.7113705295886,29.4138617507756));
#28116=CARTESIAN_POINT('Ctrl Pts',(132.881161450912,-36.7870389964753,29.4085179058602));
#28117=CARTESIAN_POINT('Ctrl Pts',(132.846494536307,-36.8417566178106,29.404501548168));
#28118=CARTESIAN_POINT('Ctrl Pts',(132.702015419951,-37.0559688978315,29.3882595657944));
#28119=CARTESIAN_POINT('Ctrl Pts',(132.58019513135,-37.2069177437768,29.3756533520406));
#28120=CARTESIAN_POINT('Ctrl Pts',(132.326516778446,-37.4713544647548,29.3521492712588));
#28121=CARTESIAN_POINT('Ctrl Pts',(132.197500432843,-37.5867505596752,29.3412452219469));
#28122=CARTESIAN_POINT('Ctrl Pts',(132.018403373966,-37.7238258186841,29.3275226926755));
#28123=CARTESIAN_POINT('Ctrl Pts',(131.975835265241,-37.7548602033877,29.3243539909629));
#28124=CARTESIAN_POINT('Ctrl Pts',(131.907841428439,-37.8020441361666,29.319433933198));
#28125=CARTESIAN_POINT('Ctrl Pts',(131.882895689877,-37.8188675324368,29.3176576704253));
#28126=CARTESIAN_POINT('Ctrl Pts',(131.835529955723,-37.8499016074708,29.3143376830527));
#28127=CARTESIAN_POINT('Ctrl Pts',(131.81316076269,-37.8641853114283,29.312791355883));
#28128=CARTESIAN_POINT('Ctrl Pts',(131.762018393016,-37.8960026539388,29.3093034313769));
#28129=CARTESIAN_POINT('Ctrl Pts',(131.733146691286,-37.9133731054648,29.3073678090876));
#28130=CARTESIAN_POINT('Ctrl Pts',(131.641991147098,-37.9663814352736,29.3013558756328));
#28131=CARTESIAN_POINT('Ctrl Pts',(131.578829922599,-38.0004750980198,29.2973333744503));
#28132=CARTESIAN_POINT('Ctrl Pts',(131.252019648092,-38.1637035901683,29.2771411035599));
#28133=CARTESIAN_POINT('Ctrl Pts',(130.97350536681,-38.2601919036173,29.2620646190058));
#28134=CARTESIAN_POINT('Ctrl Pts',(130.619652660696,-38.3333215818098,29.2425120947366));
#28135=CARTESIAN_POINT('Ctrl Pts',(130.552860181364,-38.3450481139434,29.2387983813863));
#28136=CARTESIAN_POINT('Ctrl Pts',(130.440488133104,-38.3613194147462,29.2324478714702));
#28137=CARTESIAN_POINT('Ctrl Pts',(130.395085801481,-38.366957795219,29.2298542281665));
#28138=CARTESIAN_POINT('Ctrl Pts',(130.32979457595,-38.3737273891108,29.2260671405981));
#28139=CARTESIAN_POINT('Ctrl Pts',(130.309986372578,-38.3756050369781,29.2249106671137));
#28140=CARTESIAN_POINT('Ctrl Pts',(130.275239074104,-38.3785903704842,29.222867023552));
#28141=CARTESIAN_POINT('Ctrl Pts',(130.260307365872,-38.379773587641,29.2219839179486));
#28142=CARTESIAN_POINT('Ctrl Pts',(130.227384564231,-38.3821629799518,29.2200255469682));
#28143=CARTESIAN_POINT('Ctrl Pts',(130.209391632011,-38.3833245891236,29.218948049829));
#28144=CARTESIAN_POINT('Ctrl Pts',(130.156968008969,-38.3862892405329,29.2157893696504));
#28145=CARTESIAN_POINT('Ctrl Pts',(130.122518980383,-38.3877105364792,29.2136894750293));
#28146=CARTESIAN_POINT('Ctrl Pts',(129.895417175012,-38.3936119651958,29.1997121813691));
#28147=CARTESIAN_POINT('Ctrl Pts',(129.70271627876,-38.3821815352064,29.187238437771));
#28148=CARTESIAN_POINT('Ctrl Pts',(129.35955108603,-38.3322630414233,29.1648971983666));
#28149=CARTESIAN_POINT('Ctrl Pts',(129.208735357683,-38.2997059179865,29.1550296461056));
#28150=CARTESIAN_POINT('Ctrl Pts',(128.969964921749,-38.2308420517709,29.139537255849));
#28151=CARTESIAN_POINT('Ctrl Pts',(128.880407351219,-38.2009104150179,29.1337543321659));
#28152=CARTESIAN_POINT('Ctrl Pts',(128.757504127495,-38.1540432216105,29.1258602729314));
#28153=CARTESIAN_POINT('Ctrl Pts',(128.723018091405,-38.1402391639313,29.1236497478761));
#28154=CARTESIAN_POINT('Ctrl Pts',(128.663882468747,-38.1154330487683,29.119865646685));
#28155=CARTESIAN_POINT('Ctrl Pts',(128.639125098898,-38.1046984885592,29.1182833885195));
#28156=CARTESIAN_POINT('Ctrl Pts',(128.588523932318,-38.0820367194559,29.115052520482));
#28157=CARTESIAN_POINT('Ctrl Pts',(128.562696843926,-38.0700773180777,29.113405148314));
#28158=CARTESIAN_POINT('Ctrl Pts',(128.496562655612,-38.0384359410375,29.1091892517985));
#28159=CARTESIAN_POINT('Ctrl Pts',(128.456489418936,-38.0182763569392,29.1066371084714));
#28160=CARTESIAN_POINT('Ctrl Pts',(128.254323285386,-37.9114931952036,29.0937550470773));
#28161=CARTESIAN_POINT('Ctrl Pts',(128.099061997621,-37.8125832459622,29.0838613236284));
#28162=CARTESIAN_POINT('Ctrl Pts',(127.811353882473,-37.5945385142546,29.0646668353547));
#28163=CARTESIAN_POINT('Ctrl Pts',(127.67875235352,-37.4766116070571,29.0553819285376));
#28164=CARTESIAN_POINT('Ctrl Pts',(127.498935781337,-37.2895109809737,29.0412241209243));
#28165=CARTESIAN_POINT('Ctrl Pts',(127.444074416775,-37.2280989948424,29.0366526011648));
#28166=CARTESIAN_POINT('Ctrl Pts',(127.375879868763,-37.1459257648364,29.0305394849632));
#28167=CARTESIAN_POINT('Ctrl Pts',(127.360457617432,-37.1269273114062,29.0291263665175));
#28168=CARTESIAN_POINT('Ctrl Pts',(127.33547836026,-37.0954656031604,29.0267835195185));
#28169=CARTESIAN_POINT('Ctrl Pts',(127.325799585962,-37.0830995635218,29.0258619889336));
#28170=CARTESIAN_POINT('Ctrl Pts',(127.307612767747,-37.0595276165547,29.0241031751704));
#28171=CARTESIAN_POINT('Ctrl Pts',(127.299087894945,-37.0483351280391,29.0232671443138));
#28172=CARTESIAN_POINT('Ctrl Pts',(127.276172238462,-37.0178568884208,29.0209888472522));
#28173=CARTESIAN_POINT('Ctrl Pts',(127.26191701453,-36.9984708126906,29.0195378792274));
#28174=CARTESIAN_POINT('Ctrl Pts',(127.206137943803,-36.9208981563015,29.0137300273212));
#28175=CARTESIAN_POINT('Ctrl Pts',(127.166255116018,-36.8615594071029,29.0092835258124));
#28176=CARTESIAN_POINT('Ctrl Pts',(127.028235051219,-36.6414855896818,28.992899063843));
#28177=CARTESIAN_POINT('Ctrl Pts',(126.941657674828,-36.4739072011151,28.9806426900215));
#28178=CARTESIAN_POINT('Ctrl Pts',(126.798564021562,-36.1293230860652,28.9567220587969));
#28179=CARTESIAN_POINT('Ctrl Pts',(126.741753860513,-35.9531065428809,28.9450926735559));
#28180=CARTESIAN_POINT('Ctrl Pts',(126.689441068281,-35.7297843032429,28.9312280638086));
#28181=CARTESIAN_POINT('Ctrl Pts',(126.680145050042,-35.6862572137455,28.9285642615742));
#28182=CARTESIAN_POINT('Ctrl Pts',(126.666330870643,-35.6147031903601,28.9242462511849));
#28183=CARTESIAN_POINT('Ctrl Pts',(126.661302997939,-35.5867812862212,28.9225763278949));
#28184=CARTESIAN_POINT('Ctrl Pts',(126.652177311346,-35.5321809962047,28.9193391717641));
#28185=CARTESIAN_POINT('Ctrl Pts',(126.648046435952,-35.5055103694541,28.9177710196791));
#28186=CARTESIAN_POINT('Ctrl Pts',(126.638966803628,-35.4418729764437,28.9140590905716));
#28187=CARTESIAN_POINT('Ctrl Pts',(126.634308685247,-35.4048678848587,28.9119244408266));
#28188=CARTESIAN_POINT('Ctrl Pts',(126.620540237047,-35.2787204598076,28.9047217289337));
#28189=CARTESIAN_POINT('Ctrl Pts',(126.6143533784,-35.1892938167239,28.8997423539257));
#28190=CARTESIAN_POINT('Ctrl Pts',(126.603771012355,-34.8297322796127,28.8800693369051));
#28191=CARTESIAN_POINT('Ctrl Pts',(126.628122280371,-34.5597800057159,28.8661652196633));
#28192=CARTESIAN_POINT('Ctrl Pts',(126.697999995049,-34.23085757422,28.8479563580422));
#28193=CARTESIAN_POINT('Ctrl Pts',(126.713643320526,-34.1665475392923,28.8443288430707));
#28194=CARTESIAN_POINT('Ctrl Pts',(126.743057430617,-34.0593878775331,28.838110459357));
#28195=CARTESIAN_POINT('Ctrl Pts',(126.75581773537,-34.0162789525637,28.8355606692214));
#28196=CARTESIAN_POINT('Ctrl Pts',(126.775405901636,-33.9546353599272,28.8318281892463));
#28197=CARTESIAN_POINT('Ctrl Pts',(126.781544843671,-33.9358850175106,28.8306812242449));
#28198=CARTESIAN_POINT('Ctrl Pts',(126.79261855824,-33.9030348773328,28.8286495218307));
#28199=CARTESIAN_POINT('Ctrl Pts',(126.797483389167,-33.8889124525811,28.8277687306515));
#28200=CARTESIAN_POINT('Ctrl Pts',(126.808444380887,-33.8577632314348,28.8258093683885));
#28201=CARTESIAN_POINT('Ctrl Pts',(126.814583478882,-33.8407529771556,28.8247284833112));
#28202=CARTESIAN_POINT('Ctrl Pts',(126.820986072869,-33.8234475577599,28.8236182809077));
#28203=CARTESIAN_POINT('Ctrl Pts',(126.821113966276,-33.8231020508019,28.8235961111341));
#28204=CARTESIAN_POINT('Ctrl Pts',(126.821241915871,-33.8227565650717,28.8235739384178));
#28205=CARTESIAN_POINT('Origin',(-10.,-35.,32.7603849714045));
#28206=CARTESIAN_POINT('',(-7.51282745730981,-31.7594448403263,18.0469656703996));
#28207=CARTESIAN_POINT('',(-7.51282745730979,-31.7594448403263,17.9425398458891));
#28208=CARTESIAN_POINT('',(-7.5128274573098,-31.7594448403263,32.7603849714045));
#28209=CARTESIAN_POINT('',(-14.0827617124838,-35.0055111943466,17.1353849829093));
#28210=CARTESIAN_POINT('Ctrl Pts',(-7.51282745730979,-31.7594448403263,
17.9425398458891));
#28211=CARTESIAN_POINT('Ctrl Pts',(-7.41830337030683,-31.8319934322288,
17.9367380944228));
#28212=CARTESIAN_POINT('Ctrl Pts',(-7.32686995564933,-31.9087474254191,
17.9309363429564));
#28213=CARTESIAN_POINT('Ctrl Pts',(-7.23891895494735,-31.9894092834377,
17.9251345914901));
#28214=CARTESIAN_POINT('Ctrl Pts',(-7.15101699404093,-32.0700261659473,
17.9193360749695));
#28215=CARTESIAN_POINT('Ctrl Pts',(-7.06659388623147,-32.1545463036953,
17.9135375584488));
#28216=CARTESIAN_POINT('Ctrl Pts',(-6.98600812104434,-32.242632060535,17.9077390419282));
#28217=CARTESIAN_POINT('Ctrl Pts',(-6.90544513829122,-32.3306929146151,
17.9019421647084));
#28218=CARTESIAN_POINT('Ctrl Pts',(-6.82871761722978,-32.422317081744,17.8961452874887));
#28219=CARTESIAN_POINT('Ctrl Pts',(-6.75614657546723,-32.5171307001481,
17.8903484102689));
#28220=CARTESIAN_POINT('Ctrl Pts',(-6.6835788188904,-32.6119400264773,17.8845517954654));
#28221=CARTESIAN_POINT('Ctrl Pts',(-6.61516741615517,-32.7099381918354,
17.8787551806619));
#28222=CARTESIAN_POINT('Ctrl Pts',(-6.55119212035181,-32.8107194767969,
17.8729585658584));
#28223=CARTESIAN_POINT('Ctrl Pts',(-6.48720453022862,-32.9115201291928,
17.8671608371024));
#28224=CARTESIAN_POINT('Ctrl Pts',(-6.42765496159749,-33.0151046191435,
17.8613631083465));
#28225=CARTESIAN_POINT('Ctrl Pts',(-6.37277863245117,-33.1210401412491,
17.8555653795906));
#28226=CARTESIAN_POINT('Ctrl Pts',(-6.31784438904388,-33.2270874634253,
17.8497615321459));
#28227=CARTESIAN_POINT('Ctrl Pts',(-6.2675934242897,-33.3354904093112,17.8439576847012));
#28228=CARTESIAN_POINT('Ctrl Pts',(-6.22221405330886,-33.4457933403235,
17.8381538372565));
#28229=CARTESIAN_POINT('Ctrl Pts',(-6.1768101584289,-33.5561558811958,17.8323468532993));
#28230=CARTESIAN_POINT('Ctrl Pts',(-6.13628324099394,-33.6684200677715,
17.826539869342));
#28231=CARTESIAN_POINT('Ctrl Pts',(-6.1007720966111,-33.7821138158952,17.8207328853847));
#28232=CARTESIAN_POINT('Ctrl Pts',(-6.0652035360177,-33.8959913898091,17.8149165124027));
#28233=CARTESIAN_POINT('Ctrl Pts',(-6.03466705613968,-34.0113027473889,
17.8091001394206));
#28234=CARTESIAN_POINT('Ctrl Pts',(-6.00925069731334,-34.127563754131,17.8032837664386));
#28235=CARTESIAN_POINT('Ctrl Pts',(-5.98745130943369,-34.227279799162,17.7982951143837));
#28236=CARTESIAN_POINT('Ctrl Pts',(-5.96941762182638,-34.3276941337255,
17.7933064623287));
#28237=CARTESIAN_POINT('Ctrl Pts',(-5.95517470999492,-34.4284990172053,
17.7883178102738));
#28238=CARTESIAN_POINT('Ctrl Pts',(-5.93851906885877,-34.5463801066818,
17.7824840875517));
#28239=CARTESIAN_POINT('Ctrl Pts',(-5.9269944808512,-34.6651770682635,17.7766503648296));
#28240=CARTESIAN_POINT('Ctrl Pts',(-5.92069314400233,-34.7844064597202,
17.7708166421075));
#28241=CARTESIAN_POINT('Ctrl Pts',(-5.91439976709298,-34.9034852388912,
17.764990288628));
#28242=CARTESIAN_POINT('Ctrl Pts',(-5.9133165382126,-35.0229949586629,17.7591639351485));
#28243=CARTESIAN_POINT('Ctrl Pts',(-5.91748427346542,-35.1424441736183,
17.753337581669));
#28244=CARTESIAN_POINT('Ctrl Pts',(-5.92164781989202,-35.261773334882,17.7475170840274));
#28245=CARTESIAN_POINT('Ctrl Pts',(-5.93105181658592,-35.3810417080726,
17.7416965863859));
#28246=CARTESIAN_POINT('Ctrl Pts',(-5.94568508665268,-35.4997555236408,
17.7358760887443));
#28247=CARTESIAN_POINT('Ctrl Pts',(-5.96083644705803,-35.6226723970781,
17.7298495166177));
#28248=CARTESIAN_POINT('Ctrl Pts',(-5.98159424722097,-35.7449942738863,
17.7238229444911));
#28249=CARTESIAN_POINT('Ctrl Pts',(-6.00788719817211,-35.8661757197485,
17.7177963723644));
#28250=CARTESIAN_POINT('Ctrl Pts',(-6.03325190179439,-35.9830789712902,
17.7119825625667));
#28251=CARTESIAN_POINT('Ctrl Pts',(-6.06376744677097,-36.0989205224302,
17.706168752769));
#28252=CARTESIAN_POINT('Ctrl Pts',(-6.09931751766941,-36.2132193420974,
17.7003549429713));
#28253=CARTESIAN_POINT('Ctrl Pts',(-6.13486190666894,-36.3274998936059,
17.6945420623836));
#28254=CARTESIAN_POINT('Ctrl Pts',(-6.17543910039763,-36.4402378157443,
17.6887291817958));
#28255=CARTESIAN_POINT('Ctrl Pts',(-6.22088278486858,-36.5509668192122,
17.6829163012081));
#28256=CARTESIAN_POINT('Ctrl Pts',(-6.26632982913655,-36.6617040092297,
17.6771029908555));
#28257=CARTESIAN_POINT('Ctrl Pts',(-6.31664392498955,-36.7704316089549,
17.6712896805029));
#28258=CARTESIAN_POINT('Ctrl Pts',(-6.37161068595107,-36.8767034890189,
17.6654763701502));
#28259=CARTESIAN_POINT('Ctrl Pts',(-6.42659435971158,-36.9830080680251,
17.6596612710921));
#28260=CARTESIAN_POINT('Ctrl Pts',(-6.48623335900731,-37.0868550634284,
17.6538461720339));
#28261=CARTESIAN_POINT('Ctrl Pts',(-6.55026775161833,-37.1878236707915,
17.6480310729758));
#28262=CARTESIAN_POINT('Ctrl Pts',(-6.61437088710802,-37.2889006710422,
17.642209731231));
#28263=CARTESIAN_POINT('Ctrl Pts',(-6.68287861686422,-37.3870927713628,
17.6363883894862));
#28264=CARTESIAN_POINT('Ctrl Pts',(-6.75548806402465,-37.4820087222477,
17.6305670477413));
#28265=CARTESIAN_POINT('Ctrl Pts',(-6.82814390425031,-37.5769853187106,
17.6247419865096));
#28266=CARTESIAN_POINT('Ctrl Pts',(-6.90490642128588,-37.6686812851157,
17.6189169252779));
#28267=CARTESIAN_POINT('Ctrl Pts',(-6.98543397023575,-37.7567402221086,
17.6130918640462));
#28268=CARTESIAN_POINT('Ctrl Pts',(-7.06607372756671,-37.8449218618398,
17.6072586860806));
#28269=CARTESIAN_POINT('Ctrl Pts',(-7.15048870197217,-37.9294560696016,
17.6014255081149));
#28270=CARTESIAN_POINT('Ctrl Pts',(-7.23830202914566,-38.0100248035156,
17.5955923301492));
#28271=CARTESIAN_POINT('Ctrl Pts',(-7.26015042859291,-38.0300707115591,
17.5941410060013));
#28272=CARTESIAN_POINT('Ctrl Pts',(-7.28220904940426,-38.0498713440633,
17.5926896818533));
#28273=CARTESIAN_POINT('Ctrl Pts',(-7.3044717991109,-38.0694222124386,17.5912383577053));
#28274=CARTESIAN_POINT('Ctrl Pts',(-7.39387079096929,-38.1479312890683,
17.5854103752055));
#28275=CARTESIAN_POINT('Ctrl Pts',(-7.48684366641138,-38.2226553293975,
17.5795823927056));
#28276=CARTESIAN_POINT('Ctrl Pts',(-7.58303683313338,-38.293252806878,17.5737544102058));
#28277=CARTESIAN_POINT('Ctrl Pts',(-7.67911044836402,-38.363762543888,17.5679336708816));
#28278=CARTESIAN_POINT('Ctrl Pts',(-7.77839606833716,-38.4301556801732,
17.5621129315574));
#28279=CARTESIAN_POINT('Ctrl Pts',(-7.88050527017014,-38.4921293060572,
17.5562921922332));
#28280=CARTESIAN_POINT('Ctrl Pts',(-7.98251404491423,-38.5540419792482,
17.5504771777594));
#28281=CARTESIAN_POINT('Ctrl Pts',(-8.08734053018008,-38.6115435794294,
17.5446621632855));
#28282=CARTESIAN_POINT('Ctrl Pts',(-8.19456589800467,-38.6643734393962,
17.5388471488117));
#28283=CARTESIAN_POINT('Ctrl Pts',(-8.30573107092183,-38.7191444384382,
17.5328184719919));
#28284=CARTESIAN_POINT('Ctrl Pts',(-8.41947443517335,-38.7688935336658,
17.5267897951722));
#28285=CARTESIAN_POINT('Ctrl Pts',(-8.53529918504936,-38.8133812453888,
17.5207611183524));
#28286=CARTESIAN_POINT('Ctrl Pts',(-8.64689736879917,-38.8562455540343,
17.514952434248));
#28287=CARTESIAN_POINT('Ctrl Pts',(-8.76042727961783,-38.8942255869599,
17.5091437501435));
#28288=CARTESIAN_POINT('Ctrl Pts',(-8.87542318440409,-38.9271557119402,
17.5033350660391));
#28289=CARTESIAN_POINT('Ctrl Pts',(-8.990403470318,-38.960081364314,17.4975271708767));
#28290=CARTESIAN_POINT('Ctrl Pts',(-9.1068489625418,-38.9879583606301,17.4917192757142));
#28291=CARTESIAN_POINT('Ctrl Pts',(-9.22427893354455,-39.0106709946164,
17.4859113805518));
#28292=CARTESIAN_POINT('Ctrl Pts',(-9.34172052787383,-39.0333858767201,
17.4801029105185));
#28293=CARTESIAN_POINT('Ctrl Pts',(-9.46014639463344,-39.0509353026474,
17.4742944404853));
#28294=CARTESIAN_POINT('Ctrl Pts',(-9.57906641146543,-39.06325484237,17.468485970452));
#28295=CARTESIAN_POINT('Ctrl Pts',(-9.69802612153923,-39.0755784941209,
17.4626755616619));
#28296=CARTESIAN_POINT('Ctrl Pts',(-9.81747990460743,-39.0826687457922,
17.4568651528717));
#28297=CARTESIAN_POINT('Ctrl Pts',(-9.93693395963507,-39.0845131502485,
17.4510547440815));
#28298=CARTESIAN_POINT('Ctrl Pts',(-10.0565213697727,-39.0863596137455,
17.4452378487162));
#28299=CARTESIAN_POINT('Ctrl Pts',(-10.1761086447797,-39.0829485339201,
17.4394209533509));
#28300=CARTESIAN_POINT('Ctrl Pts',(-10.2952032565593,-39.0743195796742,
17.4336040579856));
#28301=CARTESIAN_POINT('Ctrl Pts',(-10.4143768272869,-39.0656849044882,
17.4277833060567));
#28302=CARTESIAN_POINT('Ctrl Pts',(-10.5330566804442,-39.051825512261,17.4219625541279));
#28303=CARTESIAN_POINT('Ctrl Pts',(-10.6507583154515,-39.0328325795737,
17.416141802199));
#28304=CARTESIAN_POINT('Ctrl Pts',(-10.7686287585406,-39.0138124071582,
17.4103127021281));
#28305=CARTESIAN_POINT('Ctrl Pts',(-10.8855177855614,-38.9896440811116,
17.4044836020572));
#28306=CARTESIAN_POINT('Ctrl Pts',(-11.0009537873615,-38.960469229216,17.3986545019863));
#28307=CARTESIAN_POINT('Ctrl Pts',(-11.0306298219521,-38.9529690221703,
17.3971559697032));
#28308=CARTESIAN_POINT('Ctrl Pts',(-11.0602099213474,-38.9451381902407,
17.39565743742));
#28309=CARTESIAN_POINT('Ctrl Pts',(-11.0896862802715,-38.9369796558514,
17.3941589051369));
#28310=CARTESIAN_POINT('Ctrl Pts',(-11.2031719139894,-38.9055688412473,
17.3883894718687));
#28311=CARTESIAN_POINT('Ctrl Pts',(-11.3155007485516,-38.8691909052908,
17.3826200386006));
#28312=CARTESIAN_POINT('Ctrl Pts',(-11.4262003987351,-38.8279468939169,
17.3768506053324));
#28313=CARTESIAN_POINT('Ctrl Pts',(-11.5367586810991,-38.7867555527722,
17.3710885398581));
#28314=CARTESIAN_POINT('Ctrl Pts',(-11.6456915287877,-38.7407106345995,
17.3653264743838));
#28315=CARTESIAN_POINT('Ctrl Pts',(-11.7525390974166,-38.689963646437,17.3595644089094));
#28316=CARTESIAN_POINT('Ctrl Pts',(-11.8592793964961,-38.6392676056813,
17.3538081282571));
#28317=CARTESIAN_POINT('Ctrl Pts',(-11.9639382054807,-38.5838790596371,
17.3480518476048));
#28318=CARTESIAN_POINT('Ctrl Pts',(-12.0660738167459,-38.5239982950843,
17.3422955669525));
#28319=CARTESIAN_POINT('Ctrl Pts',(-12.1734329020074,-38.46105507648,17.3362448955198));
#28320=CARTESIAN_POINT('Ctrl Pts',(-12.2780034320631,-38.3931481539316,
17.3301942240872));
#28321=CARTESIAN_POINT('Ctrl Pts',(-12.3792994209464,-38.3205661061759,
17.3241435526545));
#28322=CARTESIAN_POINT('Ctrl Pts',(-12.4755642992349,-38.2515890215929,
17.3183934024714));
#28323=CARTESIAN_POINT('Ctrl Pts',(-12.5688717047298,-38.1783903109183,
17.3126432522882));
#28324=CARTESIAN_POINT('Ctrl Pts',(-12.6588334620962,-38.1012625849543,
17.3068931021051));
#28325=CARTESIAN_POINT('Ctrl Pts',(-12.7487854232299,-38.0241432576829,
17.3011435780748));
#28326=CARTESIAN_POINT('Ctrl Pts',(-12.8353921438226,-37.9430960365249,
17.2953940540445));
#28327=CARTESIAN_POINT('Ctrl Pts',(-12.9182989111097,-37.8584535094026,
17.2896445300142));
#28328=CARTESIAN_POINT('Ctrl Pts',(-13.001217134618,-37.7737992862083,17.2838942115033));
#28329=CARTESIAN_POINT('Ctrl Pts',(-13.0804340967645,-37.6855490671484,
17.2781438929923));
#28330=CARTESIAN_POINT('Ctrl Pts',(-13.1556328407124,-37.5940713896532,
17.2723935744814));
#28331=CARTESIAN_POINT('Ctrl Pts',(-13.2308605571474,-37.5025584677418,
17.2666410404943));
#28332=CARTESIAN_POINT('Ctrl Pts',(-13.3020667131398,-37.407815936993,17.2608885065071));
#28333=CARTESIAN_POINT('Ctrl Pts',(-13.3689759047412,-37.3102437865457,
17.25513597252));
#28334=CARTESIAN_POINT('Ctrl Pts',(-13.4359686747336,-37.2125497556341,
17.2493762528604));
#28335=CARTESIAN_POINT('Ctrl Pts',(-13.4986535321635,-37.1120193945602,
17.2436165332008));
#28336=CARTESIAN_POINT('Ctrl Pts',(-13.5567994624573,-37.0090800342106,
17.2378568135413));
#28337=CARTESIAN_POINT('Ctrl Pts',(-13.6149876492351,-36.9060658645764,
17.2320929081115));
#28338=CARTESIAN_POINT('Ctrl Pts',(-13.6686301558586,-36.8006395816176,
17.2263290026817));
#28339=CARTESIAN_POINT('Ctrl Pts',(-13.7175436244579,-36.6932496567998,
17.2205650972519));
#28340=CARTESIAN_POINT('Ctrl Pts',(-13.7665358558739,-36.5856868075665,
17.2147919105047));
#28341=CARTESIAN_POINT('Ctrl Pts',(-13.8107836979585,-36.4761543910992,
17.2090187237575));
#28342=CARTESIAN_POINT('Ctrl Pts',(-13.850153190532,-36.3651173610485,17.2032455370104));
#28343=CARTESIAN_POINT('Ctrl Pts',(-13.8641694595514,-36.325586120421,17.2011901755297));
#28344=CARTESIAN_POINT('Ctrl Pts',(-13.8775678722885,-36.2858642738188,
17.1991348140491));
#28345=CARTESIAN_POINT('Ctrl Pts',(-13.8903439517821,-36.2459730883259,
17.1970794525685));
#28346=CARTESIAN_POINT('Ctrl Pts',(-13.9364879357336,-36.1018961651894,
17.1896560041449));
#28347=CARTESIAN_POINT('Ctrl Pts',(-13.9746350341868,-35.9552204518296,
17.1822325557212));
#28348=CARTESIAN_POINT('Ctrl Pts',(-14.0045492121205,-35.8067283357521,
17.1748091072976));
#28349=CARTESIAN_POINT('Ctrl Pts',(-14.0339663193344,-35.6607036477675,
17.167509011047));
#28350=CARTESIAN_POINT('Ctrl Pts',(-14.0554218917175,-35.5129222631596,
17.1602089147964));
#28351=CARTESIAN_POINT('Ctrl Pts',(-14.0687370244314,-35.3641483571585,
17.1529088185457));
#28352=CARTESIAN_POINT('Ctrl Pts',(-14.0793913123442,-35.2451048551138,
17.1470675453931));
#28353=CARTESIAN_POINT('Ctrl Pts',(-14.0848344029928,-35.1254262216438,
17.1412262722404));
#28354=CARTESIAN_POINT('Ctrl Pts',(-14.0849962778219,-35.0055145427062,
17.1353849990878));
#28355=CARTESIAN_POINT('',(-13.1750507821943,-32.429732011932,17.));
#28356=CARTESIAN_POINT('Ctrl Pts',(-14.0811726754193,-35.0055088132717,
17.1353849714045));
#28357=CARTESIAN_POINT('Ctrl Pts',(-14.0735476212511,-34.0799540937817,
17.090256647603));
#28358=CARTESIAN_POINT('Ctrl Pts',(-13.7580895933996,-33.1499595688096,
17.0451283238015));
#28359=CARTESIAN_POINT('Ctrl Pts',(-13.1750507821943,-32.429732011932,17.));
#28360=CARTESIAN_POINT('',(-11.4626266916477,-31.1858227412875,17.00000010299));
#28361=CARTESIAN_POINT('Origin',(-10.,-35.,17.));
#28362=CARTESIAN_POINT('',(-14.0849987341496,-34.9967841025477,17.2396150285694));
#28363=CARTESIAN_POINT('Ctrl Pts',(-14.0849987341496,-34.9967841025477,
17.2396150285694));
#28364=CARTESIAN_POINT('Ctrl Pts',(-14.0848792956189,-34.8450671234211,
17.2322291344928));
#28365=CARTESIAN_POINT('Ctrl Pts',(-14.0763040577088,-34.6937076409018,
17.2248432404161));
#28366=CARTESIAN_POINT('Ctrl Pts',(-14.0594139179449,-34.5435094274846,
17.2174573463394));
#28367=CARTESIAN_POINT('Ctrl Pts',(-14.0421958750279,-34.3903952839183,
17.2099280633986));
#28368=CARTESIAN_POINT('Ctrl Pts',(-14.0163369470605,-34.2384876988639,
17.2023987804579));
#28369=CARTESIAN_POINT('Ctrl Pts',(-13.9820349515489,-34.0886149855068,
17.1948694975171));
#28370=CARTESIAN_POINT('Ctrl Pts',(-13.9743904293648,-34.0552144423323,
17.1931915260285));
#28371=CARTESIAN_POINT('Ctrl Pts',(-13.9663267596094,-34.0219148823929,
17.1915135545398));
#28372=CARTESIAN_POINT('Ctrl Pts',(-13.9578464551255,-33.9887253401522,
17.1898355830512));
#28373=CARTESIAN_POINT('Ctrl Pts',(-13.9285722574743,-33.8741543101436,
17.1840431885559));
#28374=CARTESIAN_POINT('Ctrl Pts',(-13.8942699070934,-33.7606632797219,
17.1782507940605));
#28375=CARTESIAN_POINT('Ctrl Pts',(-13.8550346975133,-33.6487293087733,
17.1724583995652));
#28376=CARTESIAN_POINT('Ctrl Pts',(-13.8158484446736,-33.5369350063114,
17.1666732326788));
#28377=CARTESIAN_POINT('Ctrl Pts',(-13.7717417078434,-33.4266942862656,
17.1608880657925));
#28378=CARTESIAN_POINT('Ctrl Pts',(-13.7228604057983,-33.3184723020601,
17.1551028989061));
#28379=CARTESIAN_POINT('Ctrl Pts',(-13.6740269923903,-33.2103563421034,
17.1493233997034));
#28380=CARTESIAN_POINT('Ctrl Pts',(-13.620428486564,-33.1042555587027,17.1435439005007));
#28381=CARTESIAN_POINT('Ctrl Pts',(-13.562259834161,-33.0006176268849,17.137764401298));
#28382=CARTESIAN_POINT('Ctrl Pts',(-13.504130973168,-32.8970505906315,17.1319888556754));
#28383=CARTESIAN_POINT('Ctrl Pts',(-13.4414383856446,-32.7959434139872,
17.1262133100527));
#28384=CARTESIAN_POINT('Ctrl Pts',(-13.3744238446957,-32.6977209733941,
17.1204377644301));
#28385=CARTESIAN_POINT('Ctrl Pts',(-13.3074334204694,-32.5995338804036,
17.1146642972703));
#28386=CARTESIAN_POINT('Ctrl Pts',(-13.2361243672596,-32.5042298006227,
17.1088908301104));
#28387=CARTESIAN_POINT('Ctrl Pts',(-13.1607825295344,-32.4122058039732,
17.1031173629506));
#28388=CARTESIAN_POINT('Ctrl Pts',(-13.0854495234263,-32.3201925944339,
17.0973445725602));
#28389=CARTESIAN_POINT('Ctrl Pts',(-13.0060849345761,-32.2314590230699,
17.0915717821698));
#28390=CARTESIAN_POINT('Ctrl Pts',(-12.9230153063086,-32.146369589613,17.0857989917794));
#28391=CARTESIAN_POINT('Ctrl Pts',(-12.839935258194,-32.0612694829545,17.0800254772784));
#28392=CARTESIAN_POINT('Ctrl Pts',(-12.7531495356343,-31.9798147183417,
17.0742519627774));
#28393=CARTESIAN_POINT('Ctrl Pts',(-12.663021482694,-31.9023328805841,17.0684784482765));
#28394=CARTESIAN_POINT('Ctrl Pts',(-12.5728043165972,-31.8247744334812,
17.0626992252743));
#28395=CARTESIAN_POINT('Ctrl Pts',(-12.47923853297,-31.7511970295599,17.0569200022721));
#28396=CARTESIAN_POINT('Ctrl Pts',(-12.3827206515411,-31.6818879921378,
17.0511407792699));
#28397=CARTESIAN_POINT('Ctrl Pts',(-12.2861553775729,-31.6125449223557,
17.045358718534));
#28398=CARTESIAN_POINT('Ctrl Pts',(-12.1866354641117,-31.547474620243,17.039576657798));
#28399=CARTESIAN_POINT('Ctrl Pts',(-12.0845849864714,-31.4869200928277,
17.033794597062));
#28400=CARTESIAN_POINT('Ctrl Pts',(-11.9823703793501,-31.4262681745584,
17.0280032369416));
#28401=CARTESIAN_POINT('Ctrl Pts',(-11.877617440471,-31.37014673806,17.0222118768211));
#28402=CARTESIAN_POINT('Ctrl Pts',(-11.7707738116355,-31.3187522349038,
17.0164205167007));
#28403=CARTESIAN_POINT('Ctrl Pts',(-11.6697948503699,-31.2701787860231,
17.0109470454638));
#28404=CARTESIAN_POINT('Ctrl Pts',(-11.5669488707751,-31.2258272805034,
17.0054735742269));
#28405=CARTESIAN_POINT('Ctrl Pts',(-11.4626266916477,-31.1858227412875,
17.00000010299));
#28406=CARTESIAN_POINT('Ctrl Pts',(-7.51282745730981,-31.7594448403263,
18.0469656703996));
#28407=CARTESIAN_POINT('Ctrl Pts',(-7.41799591346389,-31.8322294097635,
18.041156532831));
#28408=CARTESIAN_POINT('Ctrl Pts',(-7.32640799980818,-31.9091448038285,
18.0353473952624));
#28409=CARTESIAN_POINT('Ctrl Pts',(-7.23842903445172,-31.9898586740419,
18.0295382576938));
#28410=CARTESIAN_POINT('Ctrl Pts',(-7.15040482328216,-32.070614053776,18.0237261326026));
#28411=CARTESIAN_POINT('Ctrl Pts',(-7.06599354704681,-32.1551715127752,
18.0179140075113));
#28412=CARTESIAN_POINT('Ctrl Pts',(-6.98552277878798,-32.2431626666062,
18.01210188242));
#28413=CARTESIAN_POINT('Ctrl Pts',(-6.90492116054487,-32.3312968989904,
18.0062803064873));
#28414=CARTESIAN_POINT('Ctrl Pts',(-6.82827311668664,-32.4228756697515,
18.0004587305545));
#28415=CARTESIAN_POINT('Ctrl Pts',(-6.75586551560998,-32.5174979461858,
17.9946371546218));
#28416=CARTESIAN_POINT('Ctrl Pts',(-6.68752493647219,-32.6068054370391,
17.9891425675228));
#28417=CARTESIAN_POINT('Ctrl Pts',(-6.62296160326281,-32.6988236305518,
17.9836479804239));
#28418=CARTESIAN_POINT('Ctrl Pts',(-6.56237960878621,-32.793194379672,17.978153393325));
#28419=CARTESIAN_POINT('Ctrl Pts',(-6.49815825728457,-32.893234285969,17.9723287285466));
#28420=CARTESIAN_POINT('Ctrl Pts',(-6.43820408463767,-32.9962410126016,
17.9665040637681));
#28421=CARTESIAN_POINT('Ctrl Pts',(-6.38280235811278,-33.1018150196766,
17.9606793989897));
#28422=CARTESIAN_POINT('Ctrl Pts',(-6.32747055204339,-33.2072557857295,
17.9548620853037));
#28423=CARTESIAN_POINT('Ctrl Pts',(-6.27667995239707,-33.3152570295018,
17.9490447716177));
#28424=CARTESIAN_POINT('Ctrl Pts',(-6.23067250817717,-33.4253904422402,
17.9432274579317));
#28425=CARTESIAN_POINT('Ctrl Pts',(-6.18471114847212,-33.5354135370728,
17.9374159713044));
#28426=CARTESIAN_POINT('Ctrl Pts',(-6.14352356912006,-33.6475641775767,
17.9316044846772));
#28427=CARTESIAN_POINT('Ctrl Pts',(-6.10730546100739,-33.7613902042624,
17.9257929980499));
#28428=CARTESIAN_POINT('Ctrl Pts',(-6.06972578762955,-33.8794953491098,
17.9197630373294));
#28429=CARTESIAN_POINT('Ctrl Pts',(-6.03749676689774,-33.9994039233524,
17.9137330766088));
#28430=CARTESIAN_POINT('Ctrl Pts',(-6.01078198013274,-34.1205884979338,
17.9077031158882));
#28431=CARTESIAN_POINT('Ctrl Pts',(-5.98506416668024,-34.2372505663912,
17.9018981882165));
#28432=CARTESIAN_POINT('Ctrl Pts',(-5.9644564835091,-34.3550946687381,17.8960932605447));
#28433=CARTESIAN_POINT('Ctrl Pts',(-5.94905366228232,-34.4736362769607,
17.890288332873));
#28434=CARTESIAN_POINT('Ctrl Pts',(-5.93365313903662,-34.5921601996979,
17.8844842712513));
#28435=CARTESIAN_POINT('Ctrl Pts',(-5.92345598603055,-34.7113810166986,
17.8786802096296));
#28436=CARTESIAN_POINT('Ctrl Pts',(-5.91850534177189,-34.8308067529261,
17.8728761480078));
#28437=CARTESIAN_POINT('Ctrl Pts',(-5.91355426889453,-34.9502428288387,
17.8670715838799));
#28438=CARTESIAN_POINT('Ctrl Pts',(-5.91385062479059,-35.0698834514069,
17.861267019752));
#28439=CARTESIAN_POINT('Ctrl Pts',(-5.91938544634027,-35.1892349451354,
17.8554624556242));
#28440=CARTESIAN_POINT('Ctrl Pts',(-5.92492205202479,-35.3086249114969,
17.8496560204106));
#28441=CARTESIAN_POINT('Ctrl Pts',(-5.93570046273317,-35.427725156134,17.8438495851971));
#28442=CARTESIAN_POINT('Ctrl Pts',(-5.95165976113041,-35.5460460698049,
17.8380431499836));
#28443=CARTESIAN_POINT('Ctrl Pts',(-5.96763667162035,-35.6644975580691,
17.8322303070024));
#28444=CARTESIAN_POINT('Ctrl Pts',(-5.98880582772998,-35.782167593892,17.8264174640213));
#28445=CARTESIAN_POINT('Ctrl Pts',(-6.01505496204245,-35.8985755641333,
17.8206046210402));
#28446=CARTESIAN_POINT('Ctrl Pts',(-6.04132128348752,-36.0150597547633,
17.8147879719867));
#28447=CARTESIAN_POINT('Ctrl Pts',(-6.07267410054133,-36.1302798411067,
17.8089713229333));
#28448=CARTESIAN_POINT('Ctrl Pts',(-6.10895140066696,-36.2437707978677,
17.8031546738798));
#28449=CARTESIAN_POINT('Ctrl Pts',(-6.14528050704745,-36.3574238268174,
17.7973297182875));
#28450=CARTESIAN_POINT('Ctrl Pts',(-6.18654799227187,-36.4693424159406,
17.7915047626952));
#28451=CARTESIAN_POINT('Ctrl Pts',(-6.23254386823653,-36.5790817886474,
17.7856798071029));
#28452=CARTESIAN_POINT('Ctrl Pts',(-6.24466704261493,-36.6080058937677,
17.7841445183208));
#28453=CARTESIAN_POINT('Ctrl Pts',(-6.25711845065319,-36.6367787457519,
17.7826092295387));
#28454=CARTESIAN_POINT('Ctrl Pts',(-6.26989372793288,-36.6653925060134,
17.7810739407566));
#28455=CARTESIAN_POINT('Ctrl Pts',(-6.31836098739686,-36.7739483136465,
17.7752493125997));
#28456=CARTESIAN_POINT('Ctrl Pts',(-6.37164893828561,-36.8805610015775,
17.7694246844429));
#28457=CARTESIAN_POINT('Ctrl Pts',(-6.42957968551216,-36.9847729789305,
17.7636000562861));
#28458=CARTESIAN_POINT('Ctrl Pts',(-6.48743749358682,-37.0888537455947,
17.7577827617726));
#28459=CARTESIAN_POINT('Ctrl Pts',(-6.54992627449195,-37.1905394601524,
17.751965467259));
#28460=CARTESIAN_POINT('Ctrl Pts',(-6.61682033094515,-37.2893930040283,
17.7461481727455));
#28461=CARTESIAN_POINT('Ctrl Pts',(-6.68364757915551,-37.3881478211726,
17.7403366880639));
#28462=CARTESIAN_POINT('Ctrl Pts',(-6.75487112287933,-37.4840757586115,
17.7345252033824));
#28463=CARTESIAN_POINT('Ctrl Pts',(-6.8302199657713,-37.5767653239294,17.7287137187008));
#28464=CARTESIAN_POINT('Ctrl Pts',(-6.90840155476272,-37.672939561268,17.7226837507627));
#28465=CARTESIAN_POINT('Ctrl Pts',(-6.9910244955403,-37.7656267619708,17.7166537828247));
#28466=CARTESIAN_POINT('Ctrl Pts',(-7.07773723570448,-37.8544010468769,
17.7106238148867));
#28467=CARTESIAN_POINT('Ctrl Pts',(-7.16121441223064,-37.9398628445097,
17.7048188467003));
#28468=CARTESIAN_POINT('Ctrl Pts',(-7.248481334466,-38.0216981875071,17.6990138785139));
#28469=CARTESIAN_POINT('Ctrl Pts',(-7.33918460599718,-38.0995622979765,
17.6932089103274));
#28470=CARTESIAN_POINT('Ctrl Pts',(-7.42987458756949,-38.1774149996973,
17.6874047926924));
#28471=CARTESIAN_POINT('Ctrl Pts',(-7.52399960751364,-38.2512973602683,
17.6816006750573));
#28472=CARTESIAN_POINT('Ctrl Pts',(-7.62117176851912,-38.320903678987,17.6757965574222));
#28473=CARTESIAN_POINT('Ctrl Pts',(-7.71835259959821,-38.390516208249,17.6699919219214));
#28474=CARTESIAN_POINT('Ctrl Pts',(-7.81858078047582,-38.4558516993873,
17.6641872864207));
#28475=CARTESIAN_POINT('Ctrl Pts',(-7.92143844123699,-38.5166471029139,
17.6583826509199));
#28476=CARTESIAN_POINT('Ctrl Pts',(-8.02432952738108,-38.5774622629626,
17.6525761291021));
#28477=CARTESIAN_POINT('Ctrl Pts',(-8.12985144163544,-38.6337341935927,
17.6467696072842));
#28478=CARTESIAN_POINT('Ctrl Pts',(-8.23756124598365,-38.685245532979,17.6409630854663));
#28479=CARTESIAN_POINT('Ctrl Pts',(-8.3453903198527,-38.7368139120451,17.6351501339546));
#28480=CARTESIAN_POINT('Ctrl Pts',(-8.45541175130916,-38.7836110012543,
17.6293371824428));
#28481=CARTESIAN_POINT('Ctrl Pts',(-8.56716198730639,-38.8254673216981,
17.623524230931));
#28482=CARTESIAN_POINT('Ctrl Pts',(-8.6789856402559,-38.8673511406385,17.6177074604636));
#28483=CARTESIAN_POINT('Ctrl Pts',(-8.79253997245018,-38.9042876003803,
17.6118906899963));
#28484=CARTESIAN_POINT('Ctrl Pts',(-8.90734721116404,-38.9361573752899,
17.606073919529));
#28485=CARTESIAN_POINT('Ctrl Pts',(-9.02231874944238,-38.968072758736,17.6002488247359));
#28486=CARTESIAN_POINT('Ctrl Pts',(-9.13854637673725,-38.9949068934395,
17.5944237299428));
#28487=CARTESIAN_POINT('Ctrl Pts',(-9.2555429677009,-39.0165916804002,17.5885986351497));
#28488=CARTESIAN_POINT('Ctrl Pts',(-9.28636761622221,-39.0223048890572,
17.5870639194958));
#28489=CARTESIAN_POINT('Ctrl Pts',(-9.31724562117584,-39.027660938676,17.585529203842));
#28490=CARTESIAN_POINT('Ctrl Pts',(-9.34816804465764,-39.0326591849541,
17.5839944881881));
#28491=CARTESIAN_POINT('Ctrl Pts',(-9.46537473536423,-39.0516042688004,
17.5781773845232));
#28492=CARTESIAN_POINT('Ctrl Pts',(-9.58359963525702,-39.0654662622646,
17.5723602808582));
#28493=CARTESIAN_POINT('Ctrl Pts',(-9.70236375059238,-39.0741425678342,
17.5665431771933));
#28494=CARTESIAN_POINT('Ctrl Pts',(-9.82097756406794,-39.0828078931101,
17.5607334353606));
#28495=CARTESIAN_POINT('Ctrl Pts',(-9.9401288311714,-39.0863005533965,17.554923693528));
#28496=CARTESIAN_POINT('Ctrl Pts',(-10.0593293837626,-39.0845691356889,
17.5491139516953));
#28497=CARTESIAN_POINT('Ctrl Pts',(-10.1784103425818,-39.0828394551106,
17.5433100387697));
#28498=CARTESIAN_POINT('Ctrl Pts',(-10.2975400816037,-39.075896128858,17.5375061258441));
#28499=CARTESIAN_POINT('Ctrl Pts',(-10.4162269551722,-39.0637396720002,
17.5317022129185));
#28500=CARTESIAN_POINT('Ctrl Pts',(-10.5395944260109,-39.0511038067876,
17.5256694138644));
#28501=CARTESIAN_POINT('Ctrl Pts',(-10.6624829335618,-39.0328351491251,
17.5196366148103));
#28502=CARTESIAN_POINT('Ctrl Pts',(-10.7843417756888,-39.0089940108348,
17.5136038157562));
#28503=CARTESIAN_POINT('Ctrl Pts',(-10.901445632305,-38.9860831642259,17.5078064191693));
#28504=CARTESIAN_POINT('Ctrl Pts',(-11.0175982323764,-38.9580266446692,
17.5020090225824));
#28505=CARTESIAN_POINT('Ctrl Pts',(-11.132318464172,-38.9249305593469,17.4962116259955));
#28506=CARTESIAN_POINT('Ctrl Pts',(-11.2470221211626,-38.8918392557545,
17.4904150670178));
#28507=CARTESIAN_POINT('Ctrl Pts',(-11.360293428187,-38.8537099477184,17.4846185080401));
#28508=CARTESIAN_POINT('Ctrl Pts',(-11.4716650242463,-38.8106990246424,
17.4788219490624));
#28509=CARTESIAN_POINT('Ctrl Pts',(-11.5830469735196,-38.7676841032282,
17.4730248512308));
#28510=CARTESIAN_POINT('Ctrl Pts',(-11.6925284788183,-38.7197868119969,
17.4672277533992));
#28511=CARTESIAN_POINT('Ctrl Pts',(-11.7996614171169,-38.6672119905646,
17.4614306555676));
#28512=CARTESIAN_POINT('Ctrl Pts',(-11.9068297523597,-38.6146197983027,
17.4556316423629));
#28513=CARTESIAN_POINT('Ctrl Pts',(-12.0116476101418,-38.5573471826325,
17.4498326291582));
#28514=CARTESIAN_POINT('Ctrl Pts',(-12.1136913478998,-38.4956449885269,
17.4440336159536));
#28515=CARTESIAN_POINT('Ctrl Pts',(-12.2158496459546,-38.4338735239122,
17.4382280924359));
#28516=CARTESIAN_POINT('Ctrl Pts',(-12.3152272569984,-38.3676627666107,
17.4324225689182));
#28517=CARTESIAN_POINT('Ctrl Pts',(-12.4114293004768,-38.2973070419362,
17.4266170454005));
#28518=CARTESIAN_POINT('Ctrl Pts',(-12.5076952582291,-38.226904574647,17.4208076648356));
#28519=CARTESIAN_POINT('Ctrl Pts',(-12.6007811283544,-38.1523519114076,
17.4149982842707));
#28520=CARTESIAN_POINT('Ctrl Pts',(-12.6903262170624,-38.0739827334887,
17.4091889037058));
#28521=CARTESIAN_POINT('Ctrl Pts',(-12.7800013460207,-37.9954997453357,
17.4033710865721));
#28522=CARTESIAN_POINT('Ctrl Pts',(-12.8661251357339,-37.9131894620869,
17.3975532694385));
#28523=CARTESIAN_POINT('Ctrl Pts',(-12.9483746417885,-37.8274214350992,
17.3917354523048));
#28524=CARTESIAN_POINT('Ctrl Pts',(-12.971090887545,-37.8037334195407,17.3901286467431));
#28525=CARTESIAN_POINT('Ctrl Pts',(-12.993511849102,-37.7797818359811,17.3885218411814));
#28526=CARTESIAN_POINT('Ctrl Pts',(-13.0156312901188,-37.7555748805025,
17.3869150356197));
#28527=CARTESIAN_POINT('Ctrl Pts',(-13.0950952824613,-37.6686115018474,
17.3811425938679));
#28528=CARTESIAN_POINT('Ctrl Pts',(-13.1709347279013,-37.5780543125062,
17.3753701521162));
#28529=CARTESIAN_POINT('Ctrl Pts',(-13.2428032938079,-37.4842406883529,
17.3695977103644));
#28530=CARTESIAN_POINT('Ctrl Pts',(-13.314557702329,-37.3905760795297,17.3638344376681));
#28531=CARTESIAN_POINT('Ctrl Pts',(-13.3823535340787,-37.2936656586178,
17.3580711649717));
#28532=CARTESIAN_POINT('Ctrl Pts',(-13.4458822746592,-37.1938824829943,
17.3523078922753));
#28533=CARTESIAN_POINT('Ctrl Pts',(-13.509353084695,-37.0941902975851,17.3465498749881));
#28534=CARTESIAN_POINT('Ctrl Pts',(-13.5685643151663,-36.9916309131642,
17.3407918577009));
#28535=CARTESIAN_POINT('Ctrl Pts',(-13.623248700849,-36.8866090882311,17.3350338404137));
#28536=CARTESIAN_POINT('Ctrl Pts',(-13.6778967281546,-36.7816570898684,
17.3292796514983));
#28537=CARTESIAN_POINT('Ctrl Pts',(-13.7280237029789,-36.674246274176,17.323525462583));
#28538=CARTESIAN_POINT('Ctrl Pts',(-13.7734069587951,-36.5648082704653,
17.3177712736676));
#28539=CARTESIAN_POINT('Ctrl Pts',(-13.818771248082,-36.4554160029863,17.3120194895377));
#28540=CARTESIAN_POINT('Ctrl Pts',(-13.8593956025279,-36.3439986168261,
17.3062677054078));
#28541=CARTESIAN_POINT('Ctrl Pts',(-13.8951047222278,-36.2310094243662,
17.3005159212779));
#28542=CARTESIAN_POINT('Ctrl Pts',(-13.9308168475328,-36.1180107217059,
17.2947636530254));
#28543=CARTESIAN_POINT('Ctrl Pts',(-13.9616127765773,-36.0034403426354,
17.289011384773));
#28544=CARTESIAN_POINT('Ctrl Pts',(-13.987366634355,-35.8877681697565,17.2832591165205));
#28545=CARTESIAN_POINT('Ctrl Pts',(-14.013121424051,-35.7720918112122,17.2775066401188));
#28546=CARTESIAN_POINT('Ctrl Pts',(-14.0338336962148,-35.6553139878288,
17.2717541637171));
#28547=CARTESIAN_POINT('Ctrl Pts',(-14.0494286499008,-35.5379150577577,
17.2660016873154));
#28548=CARTESIAN_POINT('Ctrl Pts',(-14.0650341474827,-35.4204367531582,
17.26024532161));
#28549=CARTESIAN_POINT('Ctrl Pts',(-14.0755153712924,-35.3023369175002,
17.2544889559045));
#28550=CARTESIAN_POINT('Ctrl Pts',(-14.0808493937001,-35.1841011296474,
17.2487325901991));
#28551=CARTESIAN_POINT('Ctrl Pts',(-14.0836655963984,-35.1216762053895,
17.2456934029979));
#28552=CARTESIAN_POINT('Ctrl Pts',(-14.0850478813473,-35.0592134171758,
17.2426542157967));
#28553=CARTESIAN_POINT('Ctrl Pts',(-14.08499873415,-34.996784103083,17.2396150285955));
#28554=CARTESIAN_POINT('Origin',(-10.,-35.,32.7603849714045));
#28555=CARTESIAN_POINT('',(-7.51282745730977,-31.7594448403263,19.2967866684593));
#28556=CARTESIAN_POINT('',(-7.51282745730979,-31.7594448403263,19.1927507934385));
#28557=CARTESIAN_POINT('',(-7.5128274573098,-31.7594448403263,32.7603849714045));
#28558=CARTESIAN_POINT('',(-14.0849999333383,-34.9992620122689,18.3853849714444));
#28559=CARTESIAN_POINT('Ctrl Pts',(-7.5128274573098,-31.7594448403263,19.1927507934385));
#28560=CARTESIAN_POINT('Ctrl Pts',(-7.41816098010506,-31.83210271875,19.1869272043147));
#28561=CARTESIAN_POINT('Ctrl Pts',(-7.3267948839667,-31.9088247975322,19.1811036151909));
#28562=CARTESIAN_POINT('Ctrl Pts',(-7.23907769086388,-31.9892637108318,
19.1752800260671));
#28563=CARTESIAN_POINT('Ctrl Pts',(-7.20189342113841,-32.0233626387928,
19.1728113434624));
#28564=CARTESIAN_POINT('Ctrl Pts',(-7.1653643842384,-32.0581290534056,19.1703426608576));
#28565=CARTESIAN_POINT('Ctrl Pts',(-7.12951495513338,-32.093534688458,19.1678739782529));
#28566=CARTESIAN_POINT('Ctrl Pts',(-7.04494813447614,-32.1770546234885,
19.1620504925153));
#28567=CARTESIAN_POINT('Ctrl Pts',(-6.96389309800936,-32.2644031799116,
19.1562270067777));
#28568=CARTESIAN_POINT('Ctrl Pts',(-6.88671566354767,-32.3552531991889,
19.15040352104));
#28569=CARTESIAN_POINT('Ctrl Pts',(-6.80963560306152,-32.4459885939309,
19.1445873827345));
#28570=CARTESIAN_POINT('Ctrl Pts',(-6.73642367590697,-32.5402163562413,
19.1387712444289));
#28571=CARTESIAN_POINT('Ctrl Pts',(-6.66740974472798,-32.6375717597214,
19.1329551061234));
#28572=CARTESIAN_POINT('Ctrl Pts',(-6.59846489787046,-32.734829708501,19.1271447898883));
#28573=CARTESIAN_POINT('Ctrl Pts',(-6.53370992188484,-32.8352087388302,
19.1213344736532));
#28574=CARTESIAN_POINT('Ctrl Pts',(-6.47343477594744,-32.9383107119396,
19.1155241574181));
#28575=CARTESIAN_POINT('Ctrl Pts',(-6.41087650802344,-33.0453180158119,
19.1094937560959));
#28576=CARTESIAN_POINT('Ctrl Pts',(-6.35314444740412,-33.1552582804184,
19.1034633547736));
#28577=CARTESIAN_POINT('Ctrl Pts',(-6.30051393217922,-33.2676525077226,
19.0974329534514));
#28578=CARTESIAN_POINT('Ctrl Pts',(-6.2498612881276,-33.3758229249181,19.0916291764912));
#28579=CARTESIAN_POINT('Ctrl Pts',(-6.20393386227847,-33.4862657887406,
19.0858253995311));
#28580=CARTESIAN_POINT('Ctrl Pts',(-6.16293019111039,-33.5985292433633,
19.0800216225709));
#28581=CARTESIAN_POINT('Ctrl Pts',(-6.12193257350797,-33.7107761240019,
19.0742187024497));
#28582=CARTESIAN_POINT('Ctrl Pts',(-6.08585740503899,-33.8248426774518,
19.0684157823286));
#28583=CARTESIAN_POINT('Ctrl Pts',(-6.05485451372902,-33.9402584786111,
19.0626128622074));
#28584=CARTESIAN_POINT('Ctrl Pts',(-6.02384888208821,-34.0556844813182,
19.0568094291689));
#28585=CARTESIAN_POINT('Ctrl Pts',(-5.99791652494864,-34.1724595744584,
19.0510059961304));
#28586=CARTESIAN_POINT('Ctrl Pts',(-5.97715680626476,-34.2901002615735,
19.0452025630919));
#28587=CARTESIAN_POINT('Ctrl Pts',(-5.95639035287169,-34.4077791127807,
19.039397247348));
#28588=CARTESIAN_POINT('Ctrl Pts',(-5.94079994615834,-34.5263237144956,
19.0335919316042));
#28589=CARTESIAN_POINT('Ctrl Pts',(-5.93043336647939,-34.6452431602693,
19.0277866158603));
#28590=CARTESIAN_POINT('Ctrl Pts',(-5.92005530381182,-34.7642943322906,
19.0219748696083));
#28591=CARTESIAN_POINT('Ctrl Pts',(-5.91491265380358,-34.8837207701175,
19.0161631233563));
#28592=CARTESIAN_POINT('Ctrl Pts',(-5.9150011230657,-35.0030290997907,19.0103513771044));
#28593=CARTESIAN_POINT('Ctrl Pts',(-5.91508965044777,-35.1224158091395,
19.0045358128223));
#28594=CARTESIAN_POINT('Ctrl Pts',(-5.92041612296338,-35.2416838488016,
18.9987202485403));
#28595=CARTESIAN_POINT('Ctrl Pts',(-5.93092429633697,-35.3603441658459,
18.9929046842583));
#28596=CARTESIAN_POINT('Ctrl Pts',(-5.94144752526976,-35.4791744931636,
18.9870807877411));
#28597=CARTESIAN_POINT('Ctrl Pts',(-5.95716721945902,-35.5973949566152,
18.9812568912238));
#28598=CARTESIAN_POINT('Ctrl Pts',(-5.97797589018163,-35.7145257588357,
18.9754329947066));
#28599=CARTESIAN_POINT('Ctrl Pts',(-5.98350027717661,-35.7456222132476,
18.9738868383659));
#28600=CARTESIAN_POINT('Ctrl Pts',(-5.98938307315799,-35.7766419460926,
18.9723406820251));
#28601=CARTESIAN_POINT('Ctrl Pts',(-5.99562167962237,-35.807576168104,18.9707945256844));
#28602=CARTESIAN_POINT('Ctrl Pts',(-6.01911979901596,-35.9240919391059,
18.9649708266736));
#28603=CARTESIAN_POINT('Ctrl Pts',(-6.04774543284499,-36.0397691373127,
18.9591471276627));
#28604=CARTESIAN_POINT('Ctrl Pts',(-6.08142546428526,-36.1541224406657,
18.9533234286519));
#28605=CARTESIAN_POINT('Ctrl Pts',(-6.11506300070686,-36.2683314613219,
18.9475070775617));
#28606=CARTESIAN_POINT('Ctrl Pts',(-6.15374213614125,-36.3812195212681,
18.9416907264714));
#28607=CARTESIAN_POINT('Ctrl Pts',(-6.19733862407877,-36.4923107786506,
18.9358743753812));
#28608=CARTESIAN_POINT('Ctrl Pts',(-6.24089146718125,-36.6032908215792,
18.9300638470923));
#28609=CARTESIAN_POINT('Ctrl Pts',(-6.28935172115923,-36.7124772625115,
18.9242533188033));
#28610=CARTESIAN_POINT('Ctrl Pts',(-6.34254532110293,-36.8194093194809,
18.9184427905143));
#28611=CARTESIAN_POINT('Ctrl Pts',(-6.39775106084799,-36.9303862662133,
18.9124124689561));
#28612=CARTESIAN_POINT('Ctrl Pts',(-6.45805518470405,-37.0389344794742,
18.9063821473978));
#28613=CARTESIAN_POINT('Ctrl Pts',(-6.52320802133764,-37.1445611525692,
18.9003518258395));
#28614=CARTESIAN_POINT('Ctrl Pts',(-6.58591548063397,-37.2462233463577,
18.8945478399627));
#28615=CARTESIAN_POINT('Ctrl Pts',(-6.65311400581338,-37.3451789767769,
18.8887438540858));
#28616=CARTESIAN_POINT('Ctrl Pts',(-6.72453449292813,-37.4410142793483,
18.882939868209));
#28617=CARTESIAN_POINT('Ctrl Pts',(-6.79594441768056,-37.536835408855,18.8771367406825));
#28618=CARTESIAN_POINT('Ctrl Pts',(-6.87157481873301,-37.6295368009083,
18.871333613156));
#28619=CARTESIAN_POINT('Ctrl Pts',(-6.95111436096877,-37.718735250095,18.8655304856295));
#28620=CARTESIAN_POINT('Ctrl Pts',(-7.03066090970844,-37.8079415566224,
18.8597268469153));
#28621=CARTESIAN_POINT('Ctrl Pts',(-7.11411701251287,-37.8936440020054,
18.8539232082011));
#28622=CARTESIAN_POINT('Ctrl Pts',(-7.20113273869939,-37.9754944217087,
18.8481195694869));
#28623=CARTESIAN_POINT('Ctrl Pts',(-7.28817666363465,-38.0573713662659,
18.8423140500167));
#28624=CARTESIAN_POINT('Ctrl Pts',(-7.37878220883528,-38.1353935229219,
18.8365085305465));
#28625=CARTESIAN_POINT('Ctrl Pts',(-7.47256496897134,-38.209251807498,18.8307030110763));
#28626=CARTESIAN_POINT('Ctrl Pts',(-7.56645154505005,-38.2831918519564,
18.8248910649935));
#28627=CARTESIAN_POINT('Ctrl Pts',(-7.66352203557086,-38.3529585709188,
18.8190791189106));
#28628=CARTESIAN_POINT('Ctrl Pts',(-7.76336142554086,-38.418285079867,18.8132671728277));
#28629=CARTESIAN_POINT('Ctrl Pts',(-7.86326636786683,-38.4836544807697,
18.8074514107483));
#28630=CARTESIAN_POINT('Ctrl Pts',(-7.96594347988446,-38.5445776577864,
18.801635648669));
#28631=CARTESIAN_POINT('Ctrl Pts',(-8.07095288110995,-38.6008335442092,
18.7958198865897));
#28632=CARTESIAN_POINT('Ctrl Pts',(-8.17611264840499,-38.6571699851007,
18.7899957967485));
#28633=CARTESIAN_POINT('Ctrl Pts',(-8.2836110039876,-38.7088256198026,18.7841717069073));
#28634=CARTESIAN_POINT('Ctrl Pts',(-8.3929877162259,-38.7556273137519,18.7783476170661));
#28635=CARTESIAN_POINT('Ctrl Pts',(-8.42198752222565,-38.7680361713342,
18.7768034357494));
#28636=CARTESIAN_POINT('Ctrl Pts',(-8.45111928958413,-38.7801040804447,
18.7752592544327));
#28637=CARTESIAN_POINT('Ctrl Pts',(-8.48037427685997,-38.7918284061348,
18.773715073116));
#28638=CARTESIAN_POINT('Ctrl Pts',(-8.59070779361214,-38.8360460320986,
18.7678912813103));
#28639=CARTESIAN_POINT('Ctrl Pts',(-8.70315067803467,-38.8755152456379,
18.7620674895045));
#28640=CARTESIAN_POINT('Ctrl Pts',(-8.81725691625265,-38.9100311760711,
18.7562436976988));
#28641=CARTESIAN_POINT('Ctrl Pts',(-8.93121923080606,-38.9445035711176,
18.7504272515165));
#28642=CARTESIAN_POINT('Ctrl Pts',(-9.04684033888211,-38.9740349923122,
18.7446108053342));
#28643=CARTESIAN_POINT('Ctrl Pts',(-9.16365413058495,-38.9984685301641,
18.7387943591519));
#28644=CARTESIAN_POINT('Ctrl Pts',(-9.28035102411723,-39.0228776168289,
18.7329837336173));
#28645=CARTESIAN_POINT('Ctrl Pts',(-9.39823782950199,-39.0421988859875,
18.7271731080826));
#28646=CARTESIAN_POINT('Ctrl Pts',(-9.51683372619434,-39.0563253508387,
18.7213624825479));
#28647=CARTESIAN_POINT('Ctrl Pts',(-9.63991293020297,-39.0709858416131,
18.7153321966312));
#28648=CARTESIAN_POINT('Ctrl Pts',(-9.76375546640057,-39.0800508870034,
18.7093019107145));
#28649=CARTESIAN_POINT('Ctrl Pts',(-9.8878123230821,-39.0834591861739,18.7032716247979));
#28650=CARTESIAN_POINT('Ctrl Pts',(-10.0072157643847,-39.0867396388697,
18.6974675369808));
#28651=CARTESIAN_POINT('Ctrl Pts',(-10.126817292495,-39.0847800627728,18.6916634491637));
#28652=CARTESIAN_POINT('Ctrl Pts',(-10.2461233180407,-39.0775787315902,
18.6858593613466));
#28653=CARTESIAN_POINT('Ctrl Pts',(-10.3654117315051,-39.0703784634756,
18.6800561303351));
#28654=CARTESIAN_POINT('Ctrl Pts',(-10.4844043217039,-39.0579380037031,
18.6742528993236));
#28655=CARTESIAN_POINT('Ctrl Pts',(-10.6026099100317,-39.0403076982244,
18.6684496683121));
#28656=CARTESIAN_POINT('Ctrl Pts',(-10.7208259397154,-39.0226758354227,
18.6626459246886));
#28657=CARTESIAN_POINT('Ctrl Pts',(-10.8382544254531,-38.999853275678,18.6568421810651));
#28658=CARTESIAN_POINT('Ctrl Pts',(-10.9544123405207,-38.9719418530817,
18.6510384374416));
#28659=CARTESIAN_POINT('Ctrl Pts',(-11.0706079237318,-38.9440213792599,
18.6452328117574));
#28660=CARTESIAN_POINT('Ctrl Pts',(-11.1855317200458,-38.9110088559792,
18.6394271860732));
#28661=CARTESIAN_POINT('Ctrl Pts',(-11.2987144917996,-38.8730563730457,
18.633621560389));
#28662=CARTESIAN_POINT('Ctrl Pts',(-11.4120225795509,-38.8350618691121,
18.6278095067143));
#28663=CARTESIAN_POINT('Ctrl Pts',(-11.5235854076105,-38.792116617767,18.6219974530397));
#28664=CARTESIAN_POINT('Ctrl Pts',(-11.6329522546071,-38.7444214418484,
18.616185399365));
#28665=CARTESIAN_POINT('Ctrl Pts',(-11.7423909255862,-38.6966949432979,
18.6103695287673));
#28666=CARTESIAN_POINT('Ctrl Pts',(-11.8496303775063,-38.6442124868736,
18.6045536581696));
#28667=CARTESIAN_POINT('Ctrl Pts',(-11.9542445799809,-38.5872208074797,
18.5987377875719));
#28668=CARTESIAN_POINT('Ctrl Pts',(-12.0590085890829,-38.530147516497,18.5929135886981));
#28669=CARTESIAN_POINT('Ctrl Pts',(-12.1611394969088,-38.4685523244996,
18.5870893898243));
#28670=CARTESIAN_POINT('Ctrl Pts',(-12.2602402068397,-38.4027252618137,
18.5812651909505));
#28671=CARTESIAN_POINT('Ctrl Pts',(-12.2864981079149,-38.3852836057319,
18.5797220008162));
#28672=CARTESIAN_POINT('Ctrl Pts',(-12.3125434566103,-38.3675450700787,
18.5781788106819));
#28673=CARTESIAN_POINT('Ctrl Pts',(-12.3383692710118,-38.3495155100981,
18.5766356205475));
#28674=CARTESIAN_POINT('Ctrl Pts',(-12.4353485685863,-38.2818121635428,
18.5708407405517));
#28675=CARTESIAN_POINT('Ctrl Pts',(-12.5295492744555,-38.2097788486512,
18.5650458605559));
#28676=CARTESIAN_POINT('Ctrl Pts',(-12.6205578782234,-38.1336721919947,
18.5592509805601));
#28677=CARTESIAN_POINT('Ctrl Pts',(-12.7114513203758,-38.0576618401399,
18.5534634333627));
#28678=CARTESIAN_POINT('Ctrl Pts',(-12.7991603788963,-37.9775886587321,
18.5476758861653));
#28679=CARTESIAN_POINT('Ctrl Pts',(-12.8833004316501,-37.8937525154799,
18.5418883389678));
#28680=CARTESIAN_POINT('Ctrl Pts',(-12.9673565359973,-37.8100000174171,
18.5361065661353));
#28681=CARTESIAN_POINT('Ctrl Pts',(-13.0478504263204,-37.7224923146416,
18.5303247933027));
#28682=CARTESIAN_POINT('Ctrl Pts',(-13.1244310249679,-37.6315690700071,
18.5245430204702));
#28683=CARTESIAN_POINT('Ctrl Pts',(-13.2012298936544,-37.5403866759209,
18.5187447684274));
#28684=CARTESIAN_POINT('Ctrl Pts',(-13.2740928125809,-37.4457695142884,
18.5129465163847));
#28685=CARTESIAN_POINT('Ctrl Pts',(-13.3427031763758,-37.3480972029809,
18.507148264342));
#28686=CARTESIAN_POINT('Ctrl Pts',(-13.4110441711698,-37.2508083598766,
18.501372776635));
#28687=CARTESIAN_POINT('Ctrl Pts',(-13.4751657043617,-37.1504886541793,
18.4955972889281));
#28688=CARTESIAN_POINT('Ctrl Pts',(-13.534796089474,-37.0475452634409,18.4898218012211));
#28689=CARTESIAN_POINT('Ctrl Pts',(-13.5944184924182,-36.9446156527821,
18.4840470866253));
#28690=CARTESIAN_POINT('Ctrl Pts',(-13.6495507358493,-36.8390634126814,
18.4782723720295));
#28691=CARTESIAN_POINT('Ctrl Pts',(-13.6999659003013,-36.7313224242202,
18.4724976574336));
#28692=CARTESIAN_POINT('Ctrl Pts',(-13.7503865306814,-36.6235697546606,
18.4667223167529));
#28693=CARTESIAN_POINT('Ctrl Pts',(-13.7960888906862,-36.5136282391173,
18.4609469760721));
#28694=CARTESIAN_POINT('Ctrl Pts',(-13.8368935305175,-36.4019532928999,
18.4551716353914));
#28695=CARTESIAN_POINT('Ctrl Pts',(-13.8779822997752,-36.2895007356427,
18.4493560800625));
#28696=CARTESIAN_POINT('Ctrl Pts',(-13.9141047250615,-36.1752909100815,
18.4435405247335));
#28697=CARTESIAN_POINT('Ctrl Pts',(-13.945128495028,-36.0598047733983,18.4377249694046));
#28698=CARTESIAN_POINT('Ctrl Pts',(-13.975982656681,-35.9449500044988,18.4319412079722));
#28699=CARTESIAN_POINT('Ctrl Pts',(-14.0017937405414,-35.8288332630182,
18.4261574465398));
#28700=CARTESIAN_POINT('Ctrl Pts',(-14.0224831018297,-35.7119372833998,
18.4203736851074));
#28701=CARTESIAN_POINT('Ctrl Pts',(-14.0433430602509,-35.5940774210066,
18.4145422328303));
#28702=CARTESIAN_POINT('Ctrl Pts',(-14.0589963984069,-35.4754258368058,
18.4087107805531));
#28703=CARTESIAN_POINT('Ctrl Pts',(-14.0694159822337,-35.356480803889,18.4028793282759));
#28704=CARTESIAN_POINT('Ctrl Pts',(-14.0798355660604,-35.2375357709721,
18.3970478759987));
#28705=CARTESIAN_POINT('Ctrl Pts',(-14.0850214380849,-35.1182977151717,
18.3912164237215));
#28706=CARTESIAN_POINT('Ctrl Pts',(-14.0849999333383,-34.9992620122689,
18.3853849714444));
#28707=CARTESIAN_POINT('Ctrl Pts',(-14.0849999333382,-34.9992620114549,
18.3853849714045));
#28708=CARTESIAN_POINT('Ctrl Pts',(-14.0849927683375,-34.9596014672289,
18.3834420369294));
#28709=CARTESIAN_POINT('Ctrl Pts',(-14.0844080317122,-34.9199467334781,
18.3814991024543));
#28710=CARTESIAN_POINT('Ctrl Pts',(-14.0832461448359,-34.8803090618181,
18.3795561679791));
#28711=CARTESIAN_POINT('Ctrl Pts',(-14.0797629590262,-34.7614804750833,
18.3737315030043));
#28712=CARTESIAN_POINT('Ctrl Pts',(-14.0710827252895,-34.6426127214269,
18.3679068380296));
#28713=CARTESIAN_POINT('Ctrl Pts',(-14.0571956019598,-34.5241966294384,
18.3620821730548));
#28714=CARTESIAN_POINT('Ctrl Pts',(-14.0433260050548,-34.4059299860188,
18.3562648591742));
#28715=CARTESIAN_POINT('Ctrl Pts',(-14.024262636187,-34.2881142723218,18.3504475452937));
#28716=CARTESIAN_POINT('Ctrl Pts',(-14.0000476499133,-34.1712396013183,
18.3446302314131));
#28717=CARTESIAN_POINT('Ctrl Pts',(-13.9758569191974,-34.0544820008057,
18.3388187445931));
#28718=CARTESIAN_POINT('Ctrl Pts',(-13.9465249191627,-33.9386639651413,
18.3330072577732));
#28719=CARTESIAN_POINT('Ctrl Pts',(-13.9121454499452,-33.8242691726109,
18.3271957709532));
#28720=CARTESIAN_POINT('Ctrl Pts',(-13.876473537939,-33.7055738853948,18.3211658103056));
#28721=CARTESIAN_POINT('Ctrl Pts',(-13.8353672565244,-33.5884113956389,
18.315135849658));
#28722=CARTESIAN_POINT('Ctrl Pts',(-13.7889894075899,-33.4733093734578,
18.3091058890104));
#28723=CARTESIAN_POINT('Ctrl Pts',(-13.744342338888,-33.3625028567672,18.3033009611517));
#28724=CARTESIAN_POINT('Ctrl Pts',(-13.6948102801032,-33.2536061857114,
18.2974960332931));
#28725=CARTESIAN_POINT('Ctrl Pts',(-13.6405886331091,-33.1470727471169,
18.2916911054345));
#28726=CARTESIAN_POINT('Ctrl Pts',(-13.5863750755856,-33.0405552025272,
18.2858870436284));
#28727=CARTESIAN_POINT('Ctrl Pts',(-13.5274735063545,-32.9364005528948,
18.2800829818223));
#28728=CARTESIAN_POINT('Ctrl Pts',(-13.4641261137532,-32.835039199428,18.2742789200162));
#28729=CARTESIAN_POINT('Ctrl Pts',(-13.400773236667,-32.7336690703071,18.2684743557065));
#28730=CARTESIAN_POINT('Ctrl Pts',(-13.3329739872578,-32.635093064334,18.2626697913969));
#28731=CARTESIAN_POINT('Ctrl Pts',(-13.2610145152082,-32.5397135671631,
18.2568652270872));
#28732=CARTESIAN_POINT('Ctrl Pts',(-13.1890318472518,-32.4443033247147,
18.2510587916947));
#28733=CARTESIAN_POINT('Ctrl Pts',(-13.1128865353371,-32.3520919659564,
18.2452523563022));
#28734=CARTESIAN_POINT('Ctrl Pts',(-13.0329053126748,-32.2634491847677,
18.2394459209098));
#28735=CARTESIAN_POINT('Ctrl Pts',(-12.9528358257594,-32.1747085807572,
18.2336330777547));
#28736=CARTESIAN_POINT('Ctrl Pts',(-12.8689222519123,-32.0895447184489,
18.2278202345997));
#28737=CARTESIAN_POINT('Ctrl Pts',(-12.7815286256401,-32.0082908723031,
18.2220073914446));
#28738=CARTESIAN_POINT('Ctrl Pts',(-12.6940777767297,-31.926983823657,18.21619074222));
#28739=CARTESIAN_POINT('Ctrl Pts',(-12.6031426475152,-31.8495921538102,
18.2103740929954));
#28740=CARTESIAN_POINT('Ctrl Pts',(-12.5091195271677,-31.7764081836582,
18.2045574437708));
#28741=CARTESIAN_POINT('Ctrl Pts',(-12.414962136009,-31.7031197022861,18.1987324880126));
#28742=CARTESIAN_POINT('Ctrl Pts',(-12.3177082834953,-31.6340511495191,
18.1929075322544));
#28743=CARTESIAN_POINT('Ctrl Pts',(-12.2177824212526,-31.5694510450974,
18.1870825764962));
#28744=CARTESIAN_POINT('Ctrl Pts',(-12.1914449027408,-31.5524243574323,
18.1855472894677));
#28745=CARTESIAN_POINT('Ctrl Pts',(-12.1649218871643,-31.5357078392217,
18.1840120024392));
#28746=CARTESIAN_POINT('Ctrl Pts',(-12.1382214026234,-31.5193054955422,
18.1824767154107));
#28747=CARTESIAN_POINT('Ctrl Pts',(-12.0369241125928,-31.4570776748317,
18.1766520864543));
#28748=CARTESIAN_POINT('Ctrl Pts',(-11.9327453225741,-31.3991755625065,
18.170827457498));
#28749=CARTESIAN_POINT('Ctrl Pts',(-11.8260902324513,-31.345876375525,18.1650028285416));
#28750=CARTESIAN_POINT('Ctrl Pts',(-11.7195694289784,-31.2926442961636,
18.159185533224));
#28751=CARTESIAN_POINT('Ctrl Pts',(-11.6105788886912,-31.2440037959266,
18.1533682379065));
#28752=CARTESIAN_POINT('Ctrl Pts',(-11.4995517045763,-31.2001882039629,
18.147550942589));
#28753=CARTESIAN_POINT('Ctrl Pts',(-11.3886354051343,-31.1564163713509,
18.1417394570998));
#28754=CARTESIAN_POINT('Ctrl Pts',(-11.2756868858487,-31.1174600096547,
18.1359279716107));
#28755=CARTESIAN_POINT('Ctrl Pts',(-11.161162156784,-31.0835057199515,18.1301164861215));
#28756=CARTESIAN_POINT('Ctrl Pts',(-11.0423318833288,-31.0482749225214,
18.1240865184849));
#28757=CARTESIAN_POINT('Ctrl Pts',(-10.9218049596498,-31.0184298841488,
18.1180565508483));
#28758=CARTESIAN_POINT('Ctrl Pts',(-10.8001120045011,-30.9941235939868,
18.1120265832116));
#28759=CARTESIAN_POINT('Ctrl Pts',(-10.6829598281673,-30.9707242543323,
18.1062216142141));
#28760=CARTESIAN_POINT('Ctrl Pts',(-10.5647275148102,-30.9524578148195,
18.1004166452166));
#28761=CARTESIAN_POINT('Ctrl Pts',(-10.4459014118456,-30.9394092879343,
18.0946116762191));
#28762=CARTESIAN_POINT('Ctrl Pts',(-10.3270927194324,-30.9263626729359,
18.088807557773));
#28763=CARTESIAN_POINT('Ctrl Pts',(-10.2076908160468,-30.9185324946725,
18.0830034393269));
#28764=CARTESIAN_POINT('Ctrl Pts',(-10.0881884590293,-30.9159520331301,
18.0771993208808));
#28765=CARTESIAN_POINT('Ctrl Pts',(-9.96867543957385,-30.9133713413495,
18.07139468457));
#28766=CARTESIAN_POINT('Ctrl Pts',(-9.84906235675006,-30.9160413064066,
18.0655900482592));
#28767=CARTESIAN_POINT('Ctrl Pts',(-9.72984262241596,-30.9239430829125,
18.0597854119484));
#28768=CARTESIAN_POINT('Ctrl Pts',(-9.61058414560315,-30.9318474272349,
18.0539788893223));
#28769=CARTESIAN_POINT('Ctrl Pts',(-9.49171967855415,-30.9449869373111,
18.0481723666963));
#28770=CARTESIAN_POINT('Ctrl Pts',(-9.37373752527892,-30.9632909056069,
18.0423658440703));
#28771=CARTESIAN_POINT('Ctrl Pts',(-9.255624727833,-30.9816151422796,18.0365528917572));
#28772=CARTESIAN_POINT('Ctrl Pts',(-9.13839659792394,-31.0051151896328,
18.030739939444));
#28773=CARTESIAN_POINT('Ctrl Pts',(-9.02253141690564,-31.0336691805822,
18.0249269871308));
#28774=CARTESIAN_POINT('Ctrl Pts',(-8.90659011559562,-31.0622419307317,
18.0191102158652));
#28775=CARTESIAN_POINT('Ctrl Pts',(-8.79201393718519,-31.0958751223193,
18.0132934445995));
#28776=CARTESIAN_POINT('Ctrl Pts',(-8.67926458013119,-31.1343974660211,
18.0074766733338));
#28777=CARTESIAN_POINT('Ctrl Pts',(-8.56635386875424,-31.172974938611,18.0016515777529));
#28778=CARTESIAN_POINT('Ctrl Pts',(-8.45527557556923,-31.2164553803592,
17.995826482172));
#28779=CARTESIAN_POINT('Ctrl Pts',(-8.3464701931264,-31.2646199419898,17.9900013865911));
#28780=CARTESIAN_POINT('Ctrl Pts',(-8.31780379968252,-31.2773096108531,
17.9884666786748));
#28781=CARTESIAN_POINT('Ctrl Pts',(-8.2892950364283,-31.2903241790584,17.9869319707585));
#28782=CARTESIAN_POINT('Ctrl Pts',(-8.2609516437956,-31.303659131684,17.9853972628422));
#28783=CARTESIAN_POINT('Ctrl Pts',(-8.15351027992575,-31.3542079673793,
17.9795796420018));
#28784=CARTESIAN_POINT('Ctrl Pts',(-8.04809906399801,-31.4095278223734,
17.9737620211614));
#28785=CARTESIAN_POINT('Ctrl Pts',(-7.94517137702572,-31.4694328599776,
17.9679444003209));
#28786=CARTESIAN_POINT('Ctrl Pts',(-7.84238877816553,-31.5292534547165,
17.9621349800692));
#28787=CARTESIAN_POINT('Ctrl Pts',(-7.74208309268596,-31.5936461665222,
17.9563255598174));
#28788=CARTESIAN_POINT('Ctrl Pts',(-7.64468617915615,-31.6623778216608,
17.9505161395657));
#28789=CARTESIAN_POINT('Ctrl Pts',(-7.60011108377388,-31.6938338501174,
17.9478573750068));
#28790=CARTESIAN_POINT('Ctrl Pts',(-7.55614494409697,-31.7261980482037,
17.9451986104479));
#28791=CARTESIAN_POINT('Ctrl Pts',(-7.51282745730979,-31.7594448403263,
17.9425398458891));
#28792=CARTESIAN_POINT('',(-14.0849995332614,-35.001952755595,18.4896150286338));
#28793=CARTESIAN_POINT('Ctrl Pts',(-14.0849995332617,-35.0019527548048,
18.4896150285955));
#28794=CARTESIAN_POINT('Ctrl Pts',(-14.0850575830891,-34.8805173769074,
18.4837275465484));
#28795=CARTESIAN_POINT('Ctrl Pts',(-14.0796963945017,-34.7590902192459,
18.4778400645013));
#28796=CARTESIAN_POINT('Ctrl Pts',(-14.068944624063,-34.6381787094313,18.4719525824541));
#28797=CARTESIAN_POINT('Ctrl Pts',(-14.0581894969497,-34.5172294513599,
18.4660632623505));
#28798=CARTESIAN_POINT('Ctrl Pts',(-14.0420404715241,-34.3967965517054,
18.4601739422469));
#28799=CARTESIAN_POINT('Ctrl Pts',(-14.0205780196417,-34.2773815751216,
18.4542846221433));
#28800=CARTESIAN_POINT('Ctrl Pts',(-13.999104411433,-34.1579045258323,18.4483922407316));
#28801=CARTESIAN_POINT('Ctrl Pts',(-13.9723119464262,-34.039446838248,18.44249985932));
#28802=CARTESIAN_POINT('Ctrl Pts',(-13.9403319704358,-33.9224987411787,
18.4366074779083));
#28803=CARTESIAN_POINT('Ctrl Pts',(-13.9083066257222,-33.805384734484,18.4307067372089));
#28804=CARTESIAN_POINT('Ctrl Pts',(-13.8710791744484,-33.689784973889,18.4248059965095));
#28805=CARTESIAN_POINT('Ctrl Pts',(-13.8288306955208,-33.5761739906022,
18.4189052558101));
#28806=CARTESIAN_POINT('Ctrl Pts',(-13.7865496100022,-33.4624753244695,
18.4129999610287));
#28807=CARTESIAN_POINT('Ctrl Pts',(-13.7392399260949,-33.3507688546655,
18.4070946662472));
#28808=CARTESIAN_POINT('Ctrl Pts',(-13.687129973312,-33.241507020229,18.4011893714658));
#28809=CARTESIAN_POINT('Ctrl Pts',(-13.634928187988,-33.132052635399,18.3952736698773));
#28810=CARTESIAN_POINT('Ctrl Pts',(-13.5779094167131,-33.0250518383686,
18.3893579682888));
#28811=CARTESIAN_POINT('Ctrl Pts',(-13.5163471857879,-32.9209311052778,
18.3834422667002));
#28812=CARTESIAN_POINT('Ctrl Pts',(-13.4777388784652,-32.8556325415087,
18.3797322772875));
#28813=CARTESIAN_POINT('Ctrl Pts',(-13.437344457819,-32.7914661462019,18.3760222878747));
#28814=CARTESIAN_POINT('Ctrl Pts',(-13.3952395708656,-32.7285305953132,
18.3723122984619));
#28815=CARTESIAN_POINT('Ctrl Pts',(-13.3291450185491,-32.629736907412,18.3664885068054));
#28816=CARTESIAN_POINT('Ctrl Pts',(-13.2586283616502,-32.5336711932551,
18.3606647151489));
#28817=CARTESIAN_POINT('Ctrl Pts',(-13.1839420305572,-32.4407543794994,
18.3548409234924));
#28818=CARTESIAN_POINT('Ctrl Pts',(-13.1093499023061,-32.3479547629308,
18.3490244774602));
#28819=CARTESIAN_POINT('Ctrl Pts',(-13.0305988139817,-32.2582964624724,
18.3432080314279));
#28820=CARTESIAN_POINT('Ctrl Pts',(-12.9479848629971,-32.1721721679812,
18.3373915853957));
#28821=CARTESIAN_POINT('Ctrl Pts',(-12.8654535856495,-32.0861340600067,
18.3315809600117));
#28822=CARTESIAN_POINT('Ctrl Pts',(-12.7790674169178,-32.0036232154057,
18.3257703346277));
#28823=CARTESIAN_POINT('Ctrl Pts',(-12.6891627840684,-31.9249994275153,
18.3199597092437));
#28824=CARTESIAN_POINT('Ctrl Pts',(-12.5958594629035,-31.8434034040375,
18.3139294232707));
#28825=CARTESIAN_POINT('Ctrl Pts',(-12.498766690014,-31.7659944728829,18.3078991372978));
#28826=CARTESIAN_POINT('Ctrl Pts',(-12.3983029695353,-31.6931332251936,
18.3018688513249));
#28827=CARTESIAN_POINT('Ctrl Pts',(-12.3016076812011,-31.6230050304569,
18.2960647636591));
#28828=CARTESIAN_POINT('Ctrl Pts',(-12.2017901417147,-31.557089754572,18.2902606759933));
#28829=CARTESIAN_POINT('Ctrl Pts',(-12.0992567518518,-31.4956675257898,
18.2844565883275));
#28830=CARTESIAN_POINT('Ctrl Pts',(-11.9967384980758,-31.4342543642216,
18.2786533574672));
#28831=CARTESIAN_POINT('Ctrl Pts',(-11.8915055413924,-31.3773331404906,
18.272850126607));
#28832=CARTESIAN_POINT('Ctrl Pts',(-11.7839916953017,-31.3251396446811,
18.2670468957467));
#28833=CARTESIAN_POINT('Ctrl Pts',(-11.6764683522758,-31.272941538505,18.2612431522743));
#28834=CARTESIAN_POINT('Ctrl Pts',(-11.5666640865868,-31.225472168885,18.2554394088018));
#28835=CARTESIAN_POINT('Ctrl Pts',(-11.4550350563148,-31.1829202281201,
18.2496356653294));
#28836=CARTESIAN_POINT('Ctrl Pts',(-11.3433698265356,-31.140354488442,18.2438300397958));
#28837=CARTESIAN_POINT('Ctrl Pts',(-11.229879036659,-31.1027094943694,18.2380244142623));
#28838=CARTESIAN_POINT('Ctrl Pts',(-11.1150358409108,-31.0701246745623,
18.2322187887288));
#28839=CARTESIAN_POINT('Ctrl Pts',(-11.0000654907144,-31.0375037768251,
18.2264067352035));
#28840=CARTESIAN_POINT('Ctrl Pts',(-10.8837401387693,-31.0099543481992,
18.2205946816783));
#28841=CARTESIAN_POINT('Ctrl Pts',(-10.7665451741307,-30.987565141212,18.2147826281531));
#28842=CARTESIAN_POINT('Ctrl Pts',(-10.6492732445727,-30.9651612306621,
18.2089667577042));
#28843=CARTESIAN_POINT('Ctrl Pts',(-10.5311309680637,-30.9479243495558,
18.2031508872553));
#28844=CARTESIAN_POINT('Ctrl Pts',(-10.4126092794624,-30.935891416005,18.1973350168064));
#28845=CARTESIAN_POINT('Ctrl Pts',(-10.2939178687895,-30.9238412513935,
18.1915108180794));
#28846=CARTESIAN_POINT('Ctrl Pts',(-10.1748463677846,-30.9170099314566,
18.1856866193525));
#28847=CARTESIAN_POINT('Ctrl Pts',(-10.0558862779217,-30.9153823038208,
18.1798624206255));
#28848=CARTESIAN_POINT('Ctrl Pts',(-10.0243663698065,-30.9149510442817,
18.1783192290481));
#28849=CARTESIAN_POINT('Ctrl Pts',(-9.99285425617415,-30.9148848268477,
18.1767760374708));
#28850=CARTESIAN_POINT('Ctrl Pts',(-9.96135900559659,-30.9151827613036,
18.1752328458934));
#28851=CARTESIAN_POINT('Ctrl Pts',(-9.84254216014076,-30.9163067286177,
18.1694111060503));
#28852=CARTESIAN_POINT('Ctrl Pts',(-9.72358249997705,-30.9226209291842,
18.1635893662072));
#28853=CARTESIAN_POINT('Ctrl Pts',(-9.6049700399353,-30.9341450676824,18.1577676263641));
#28854=CARTESIAN_POINT('Ctrl Pts',(-9.48649777117739,-30.9456555854887,
18.1519527673932));
#28855=CARTESIAN_POINT('Ctrl Pts',(-9.36837228927801,-30.9623637587939,
18.1461379084223));
#28856=CARTESIAN_POINT('Ctrl Pts',(-9.25108406035002,-30.9842373183493,
18.1403230494514));
#28857=CARTESIAN_POINT('Ctrl Pts',(-9.13390674299997,-31.0060901935528,
18.134513689201));
#28858=CARTESIAN_POINT('Ctrl Pts',(-9.0175655031429,-31.033098666387,18.1287043289505));
#28859=CARTESIAN_POINT('Ctrl Pts',(-8.90254549512174,-31.0651787067616,
18.1228949687001));
#28860=CARTESIAN_POINT('Ctrl Pts',(-8.78760708024051,-31.0972359901284,
18.1170897295061));
#28861=CARTESIAN_POINT('Ctrl Pts',(-8.67398842467963,-31.134357574507,18.1112844903121));
#28862=CARTESIAN_POINT('Ctrl Pts',(-8.56216366771447,-31.1764085362634,
18.1054792511181));
#28863=CARTESIAN_POINT('Ctrl Pts',(-8.45038370261397,-31.2184426543347,
18.0996763372365));
#28864=CARTESIAN_POINT('Ctrl Pts',(-8.34039658894526,-31.2654020799654,
18.0938734233548));
#28865=CARTESIAN_POINT('Ctrl Pts',(-8.23265998151875,-31.3171024642172,
18.0880705094732));
#28866=CARTESIAN_POINT('Ctrl Pts',(-8.12494812156206,-31.3687909727128,
18.0822689285409));
#28867=CARTESIAN_POINT('Ctrl Pts',(-8.01948610574778,-31.4252180931851,
18.0764673476085));
#28868=CARTESIAN_POINT('Ctrl Pts',(-7.91670964774879,-31.4861522075911,
18.0706657666762));
#28869=CARTESIAN_POINT('Ctrl Pts',(-7.81391283532173,-31.547098389732,18.0648630367661));
#28870=CARTESIAN_POINT('Ctrl Pts',(-7.71380299386624,-31.612553139466,18.059060306856));
#28871=CARTESIAN_POINT('Ctrl Pts',(-7.61678904282017,-31.6822401332257,
18.053257576946));
#28872=CARTESIAN_POINT('Ctrl Pts',(-7.58172493086275,-31.7074273617101,
18.0511602747638));
#28873=CARTESIAN_POINT('Ctrl Pts',(-7.54706496700791,-31.733167060793,18.0490629725817));
#28874=CARTESIAN_POINT('Ctrl Pts',(-7.51282745730981,-31.7594448403263,
18.0469656703996));
#28875=CARTESIAN_POINT('Ctrl Pts',(-7.51282745730977,-31.7594448403263,
19.2967866684593));
#28876=CARTESIAN_POINT('Ctrl Pts',(-7.41811230182008,-31.8321400800316,
19.2909817497243));
#28877=CARTESIAN_POINT('Ctrl Pts',(-7.32652932999714,-31.9090354648001,
19.2851768309894));
#28878=CARTESIAN_POINT('Ctrl Pts',(-7.23846562792,-31.9898251027854,19.2793719122544));
#28879=CARTESIAN_POINT('Ctrl Pts',(-7.15042629203376,-32.0705923872279,
19.2735685996721));
#28880=CARTESIAN_POINT('Ctrl Pts',(-7.06590459032354,-32.1552515065383,
19.2677652870899));
#28881=CARTESIAN_POINT('Ctrl Pts',(-6.98525340953167,-32.2434572386303,
19.2619619745077));
#28882=CARTESIAN_POINT('Ctrl Pts',(-6.90460550996115,-32.3316593821508,
19.256158898028));
#28883=CARTESIAN_POINT('Ctrl Pts',(-6.82782809357387,-32.4234075500423,
19.2503558215484));
#28884=CARTESIAN_POINT('Ctrl Pts',(-6.75523570142573,-32.5183212039634,
19.2445527450688));
#28885=CARTESIAN_POINT('Ctrl Pts',(-6.68262913065411,-32.6132533962591,
19.2387485351421));
#28886=CARTESIAN_POINT('Ctrl Pts',(-6.61420945765297,-32.7113519797587,
19.2329443252153));
#28887=CARTESIAN_POINT('Ctrl Pts',(-6.55024921419173,-32.8122055590583,
19.2271401152886));
#28888=CARTESIAN_POINT('Ctrl Pts',(-6.48622215928464,-32.9131644877608,
19.2213298424134));
#28889=CARTESIAN_POINT('Ctrl Pts',(-6.4266640565776,-33.0168838145444,19.2155195695383));
#28890=CARTESIAN_POINT('Ctrl Pts',(-6.37180269974769,-33.1229253210269,
19.2097092966631));
#28891=CARTESIAN_POINT('Ctrl Pts',(-6.31691165533461,-33.2290242106335,
19.2038958796266));
#28892=CARTESIAN_POINT('Ctrl Pts',(-6.26672259176406,-33.3374474129976,
19.1980824625901));
#28893=CARTESIAN_POINT('Ctrl Pts',(-6.22141541612506,-33.4477359945864,
19.1922690455535));
#28894=CARTESIAN_POINT('Ctrl Pts',(-6.17603645820562,-33.5581993115407,
19.1864464180481));
#28895=CARTESIAN_POINT('Ctrl Pts',(-6.13555497936683,-33.6705335279456,
19.1806237905427));
#28896=CARTESIAN_POINT('Ctrl Pts',(-6.10010137767713,-33.7842632951152,
19.1748011630372));
#28897=CARTESIAN_POINT('Ctrl Pts',(-6.07133916713093,-33.8765280962299,
19.1700774782701));
#28898=CARTESIAN_POINT('Ctrl Pts',(-6.04588510475766,-33.969711018008,19.1653537935029));
#28899=CARTESIAN_POINT('Ctrl Pts',(-6.02378394272223,-34.0635541308509,
19.1606301087357));
#28900=CARTESIAN_POINT('Ctrl Pts',(-5.99653648754323,-34.179248772017,19.154806505942));
#28901=CARTESIAN_POINT('Ctrl Pts',(-5.97429877815729,-34.2963201807641,
19.1489829031483));
#28902=CARTESIAN_POINT('Ctrl Pts',(-5.95720681340291,-34.4142967898294,
19.1431593003546));
#28903=CARTESIAN_POINT('Ctrl Pts',(-5.9401364129236,-34.532124552341,19.1373430449767));
#28904=CARTESIAN_POINT('Ctrl Pts',(-5.92819890229578,-34.6508548430926,
19.1315267895989));
#28905=CARTESIAN_POINT('Ctrl Pts',(-5.92147985714887,-34.7700033818561,
19.125710534221));
#28906=CARTESIAN_POINT('Ctrl Pts',(-5.91476753790458,-34.8890326504776,
19.1199001010346));
#28907=CARTESIAN_POINT('Ctrl Pts',(-5.91326331491269,-35.0084789288646,
19.1140896678482));
#28908=CARTESIAN_POINT('Ctrl Pts',(-5.91700120472805,-35.1278508420302,
19.1082792346619));
#28909=CARTESIAN_POINT('Ctrl Pts',(-5.92088057325785,-35.2517409688533,
19.1022488772246));
#28910=CARTESIAN_POINT('Ctrl Pts',(-5.93040678586944,-35.3755505462157,
19.0962185197873));
#28911=CARTESIAN_POINT('Ctrl Pts',(-5.94555850193402,-35.498727519554,19.09018816235));
#28912=CARTESIAN_POINT('Ctrl Pts',(-5.96014120915312,-35.6172786942639,
19.0843842694735));
#28913=CARTESIAN_POINT('Ctrl Pts',(-5.97993446342108,-35.7352434801594,
19.078580376597));
#28914=CARTESIAN_POINT('Ctrl Pts',(-6.00486629169651,-35.8521335885747,
19.0727764837204));
#28915=CARTESIAN_POINT('Ctrl Pts',(-6.02979443675131,-35.9690064286191,
19.0669734482627));
#28916=CARTESIAN_POINT('Ctrl Pts',(-6.05985956098728,-36.0848045076697,
19.061170412805));
#28917=CARTESIAN_POINT('Ctrl Pts',(-6.09493856249193,-36.1990496942527,
19.0553673773472));
#28918=CARTESIAN_POINT('Ctrl Pts',(-6.13002066030497,-36.3133049648835,
19.0495638296746));
#28919=CARTESIAN_POINT('Ctrl Pts',(-6.17011739543714,-36.4260066801526,
19.0437602820019));
#28920=CARTESIAN_POINT('Ctrl Pts',(-6.21505597183103,-36.5366924557725,
19.0379567343293));
#28921=CARTESIAN_POINT('Ctrl Pts',(-6.26000912017273,-36.6474141227685,
19.032151304777));
#28922=CARTESIAN_POINT('Ctrl Pts',(-6.30980707868948,-36.756118171914,19.0263458752247));
#28923=CARTESIAN_POINT('Ctrl Pts',(-6.36422941753683,-36.8623633565165,
19.0205404456723));
#28924=CARTESIAN_POINT('Ctrl Pts',(-6.4187120216759,-36.9687261931196,19.0147285874013));
#28925=CARTESIAN_POINT('Ctrl Pts',(-6.47782904156566,-37.0726243664797,
19.0089167291304));
#28926=CARTESIAN_POINT('Ctrl Pts',(-6.54131462508069,-37.1736422146525,
19.0031048708594));
#28927=CARTESIAN_POINT('Ctrl Pts',(-6.60484190473565,-37.2747264094523,
18.9972891954689));
#28928=CARTESIAN_POINT('Ctrl Pts',(-6.67274323037939,-37.3729261765179,
18.9914735200785));
#28929=CARTESIAN_POINT('Ctrl Pts',(-6.74471103920186,-37.4678571234384,
18.985657844688));
#28930=CARTESIAN_POINT('Ctrl Pts',(-6.81678193082489,-37.5629240443177,
18.9798338392384));
#28931=CARTESIAN_POINT('Ctrl Pts',(-6.89293067143959,-37.6547124867205,
18.9740098337888));
#28932=CARTESIAN_POINT('Ctrl Pts',(-6.97281120843644,-37.7428731323617,
18.9681858283392));
#28933=CARTESIAN_POINT('Ctrl Pts',(-6.9940028118998,-37.766261375778,18.9666407709485));
#28934=CARTESIAN_POINT('Ctrl Pts',(-7.01545686835546,-37.7893945098375,
18.9650957135579));
#28935=CARTESIAN_POINT('Ctrl Pts',(-7.03716652044213,-37.8122664831788,
18.9635506561672));
#28936=CARTESIAN_POINT('Ctrl Pts',(-7.11899448754544,-37.8984754686886,
18.9577270296609));
#28937=CARTESIAN_POINT('Ctrl Pts',(-7.20472012898345,-37.9812490979073,
18.9519034031545));
#28938=CARTESIAN_POINT('Ctrl Pts',(-7.29402358378522,-38.0602151288577,
18.9460797766482));
#28939=CARTESIAN_POINT('Ctrl Pts',(-7.38321437281215,-38.1390815357892,
18.940263497264));
#28940=CARTESIAN_POINT('Ctrl Pts',(-7.47597369417695,-38.2141496307771,
18.9344472178798));
#28941=CARTESIAN_POINT('Ctrl Pts',(-7.57194341428716,-38.2850823759194,
18.9286309384956));
#28942=CARTESIAN_POINT('Ctrl Pts',(-7.6678170714414,-38.3559441194045,18.9228204810414));
#28943=CARTESIAN_POINT('Ctrl Pts',(-7.76689440795815,-38.4226785064943,
18.9170100235872));
#28944=CARTESIAN_POINT('Ctrl Pts',(-7.86878309388657,-38.4849877329908,
18.911199566133));
#28945=CARTESIAN_POINT('Ctrl Pts',(-7.97452765582091,-38.5496549902068,
18.9051692176941));
#28946=CARTESIAN_POINT('Ctrl Pts',(-8.08330022028003,-38.6095552419705,
18.8991388692552));
#28947=CARTESIAN_POINT('Ctrl Pts',(-8.19462736983438,-38.6644037258808,
18.8931085208162));
#28948=CARTESIAN_POINT('Ctrl Pts',(-8.30177434702584,-38.7171927290848,
18.8873046031804));
#28949=CARTESIAN_POINT('Ctrl Pts',(-8.41128712709699,-38.7653023007235,
18.8815006855446));
#28950=CARTESIAN_POINT('Ctrl Pts',(-8.52271786244398,-38.8085249751128,
18.8756967679088));
#28951=CARTESIAN_POINT('Ctrl Pts',(-8.63413213865007,-38.8517412651945,
18.8698937075544));
#28952=CARTESIAN_POINT('Ctrl Pts',(-8.74746342615259,-38.8900719458933,
18.8640906472));
#28953=CARTESIAN_POINT('Ctrl Pts',(-8.86224434573965,-38.9233578821207,
18.8582875868457));
#28954=CARTESIAN_POINT('Ctrl Pts',(-8.97703539878588,-38.9566467570044,
18.8524840141668));
#28955=CARTESIAN_POINT('Ctrl Pts',(-9.09327594618063,-38.9848898881663,
18.8466804414879));
#28956=CARTESIAN_POINT('Ctrl Pts',(-9.21048453883426,-39.0079783353432,
18.840876868809));
#28957=CARTESIAN_POINT('Ctrl Pts',(-9.32773113946557,-39.031074269558,18.8350714141686));
#28958=CARTESIAN_POINT('Ctrl Pts',(-9.4459460092339,-39.0490121165882,18.8292659595283));
#28959=CARTESIAN_POINT('Ctrl Pts',(-9.56463926691708,-39.0617343625709,
18.8234605048879));
#28960=CARTESIAN_POINT('Ctrl Pts',(-9.68346396042756,-39.0744706966236,
18.8176486215358));
#28961=CARTESIAN_POINT('Ctrl Pts',(-9.80276769302514,-39.0819798576253,
18.8118367381837));
#28962=CARTESIAN_POINT('Ctrl Pts',(-9.92205708305286,-39.0842563462273,
18.8060248548316));
#28963=CARTESIAN_POINT('Ctrl Pts',(-10.0414248202914,-39.0865343299876,
18.8002091543349));
#28964=CARTESIAN_POINT('Ctrl Pts',(-10.1607777889321,-39.083572807119,18.7943934538383));
#28965=CARTESIAN_POINT('Ctrl Pts',(-10.2796258959687,-39.0754183047024,
18.7885777533416));
#28966=CARTESIAN_POINT('Ctrl Pts',(-10.3986442306876,-39.0672521224865,
18.7827537229418));
#28967=CARTESIAN_POINT('Ctrl Pts',(-10.5171558561783,-39.0538781605604,
18.776929692542));
#28968=CARTESIAN_POINT('Ctrl Pts',(-10.6346789156901,-39.0353943641209,
18.7711056621422));
#28969=CARTESIAN_POINT('Ctrl Pts',(-10.6658518154301,-39.0304915515527,
18.7695608426277));
#28970=CARTESIAN_POINT('Ctrl Pts',(-10.6969552370849,-39.0252295000134,
18.7680160231133));
#28971=CARTESIAN_POINT('Ctrl Pts',(-10.7279803646265,-39.0196106265058,
18.7664712035988));
#28972=CARTESIAN_POINT('Ctrl Pts',(-10.8449353797245,-38.9984292329712,
18.7606477178001));
#28973=CARTESIAN_POINT('Ctrl Pts',(-10.9611538213096,-38.9721050356772,
18.7548242320015));
#28974=CARTESIAN_POINT('Ctrl Pts',(-11.0761490389905,-38.9407014915976,
18.7490007462028));
#28975=CARTESIAN_POINT('Ctrl Pts',(-11.1909991683903,-38.909337569046,18.7431846078362));
#28976=CARTESIAN_POINT('Ctrl Pts',(-11.3046287530725,-38.8729071528003,
18.7373684694695));
#28977=CARTESIAN_POINT('Ctrl Pts',(-11.416559605072,-38.8315250077845,18.7315523311029));
#28978=CARTESIAN_POINT('Ctrl Pts',(-11.5283784120568,-38.790184287121,18.7257420148067));
#28979=CARTESIAN_POINT('Ctrl Pts',(-11.6385014884079,-38.7439018393689,
18.7199316985106));
#28980=CARTESIAN_POINT('Ctrl Pts',(-11.7464647136278,-38.6928425371322,
18.7141213822144));
#28981=CARTESIAN_POINT('Ctrl Pts',(-11.8585174041288,-38.639849194454,18.7080909809151));
#28982=CARTESIAN_POINT('Ctrl Pts',(-11.9682429529133,-38.5817100820163,
18.7020605796157));
#28983=CARTESIAN_POINT('Ctrl Pts',(-12.0751436498692,-38.5186650639706,
18.6960301783164));
#28984=CARTESIAN_POINT('Ctrl Pts',(-12.1780269867652,-38.4579892964976,
18.6902264012956));
#28985=CARTESIAN_POINT('Ctrl Pts',(-12.2782935745585,-38.3927699262819,
18.6844226242748));
#28986=CARTESIAN_POINT('Ctrl Pts',(-12.3755244157646,-38.3232677818837,
18.6786188472541));
#28987=CARTESIAN_POINT('Ctrl Pts',(-12.4727409023177,-38.2537758984187,
18.6728159270726));
#28988=CARTESIAN_POINT('Ctrl Pts',(-12.5669222014561,-38.1800027355907,
18.6670130068911));
#28989=CARTESIAN_POINT('Ctrl Pts',(-12.6576790313083,-38.1022519508487,
18.6612100867096));
#28990=CARTESIAN_POINT('Ctrl Pts',(-12.7484438831084,-38.024494293756,18.6554066536111));
#28991=CARTESIAN_POINT('Ctrl Pts',(-12.8357833536778,-37.9427585814093,
18.6496032205126));
#28992=CARTESIAN_POINT('Ctrl Pts',(-12.9193424301072,-37.8573877538367,
18.6437997874141));
#28993=CARTESIAN_POINT('Ctrl Pts',(-13.0029286141271,-37.7719892309192,
18.6379944716106));
#28994=CARTESIAN_POINT('Ctrl Pts',(-13.0827316794739,-37.682953539143,18.6321891558071));
#28995=CARTESIAN_POINT('Ctrl Pts',(-13.1584350028544,-37.5906588607426,
18.6263838400036));
#28996=CARTESIAN_POINT('Ctrl Pts',(-13.2342221822704,-37.4982619481802,
18.6205720936929));
#28997=CARTESIAN_POINT('Ctrl Pts',(-13.3059002958618,-37.4025991591309,
18.6147603473822));
#28998=CARTESIAN_POINT('Ctrl Pts',(-13.3731943052379,-37.3040801156016,
18.6089486010715));
#28999=CARTESIAN_POINT('Ctrl Pts',(-13.4405325234464,-37.2054963499384,
18.6031330367312));
#29000=CARTESIAN_POINT('Ctrl Pts',(-13.503480686763,-37.1040529390479,18.5973174723909));
#29001=CARTESIAN_POINT('Ctrl Pts',(-13.5618090734252,-37.000185272535,18.5915019080506));
#29002=CARTESIAN_POINT('Ctrl Pts',(-13.6202210299261,-36.896168789903,18.5856780114762));
#29003=CARTESIAN_POINT('Ctrl Pts',(-13.6739998151822,-36.7897214822269,
18.5798541149018));
#29004=CARTESIAN_POINT('Ctrl Pts',(-13.7229632272811,-36.6813000351848,
18.5740302183273));
#29005=CARTESIAN_POINT('Ctrl Pts',(-13.7359622668343,-36.6525157936851,
18.5724840625617));
#29006=CARTESIAN_POINT('Ctrl Pts',(-13.7486221793541,-36.6235924987563,
18.570937906796));
#29007=CARTESIAN_POINT('Ctrl Pts',(-13.760940146646,-36.5945388716951,18.5693917510303));
#29008=CARTESIAN_POINT('Ctrl Pts',(-13.8139041428435,-36.4696159719389,
18.5627436908306));
#29009=CARTESIAN_POINT('Ctrl Pts',(-13.8606921368581,-36.3419281838578,
18.5560956306309));
#29010=CARTESIAN_POINT('Ctrl Pts',(-13.9010386242277,-36.2120736991964,
18.5494475704312));
#29011=CARTESIAN_POINT('Ctrl Pts',(-13.9400043386838,-36.0866632087167,
18.5430270259844));
#29012=CARTESIAN_POINT('Ctrl Pts',(-13.9729620104295,-35.9592321474535,
18.5366064815376));
#29013=CARTESIAN_POINT('Ctrl Pts',(-13.9997194876352,-35.8303427125178,
18.5301859370908));
#29014=CARTESIAN_POINT('Ctrl Pts',(-14.0264024397389,-35.701812261286,18.5237832751867));
#29015=CARTESIAN_POINT('Ctrl Pts',(-14.0469195642965,-35.5718317830148,
18.5173806132826));
#29016=CARTESIAN_POINT('Ctrl Pts',(-14.0611283190673,-35.4409782036222,
18.5109779513786));
#29017=CARTESIAN_POINT('Ctrl Pts',(-14.0752785314931,-35.31066376193,18.5046016694668));
#29018=CARTESIAN_POINT('Ctrl Pts',(-14.0831721511011,-35.1794836454211,
18.498225387555));
#29019=CARTESIAN_POINT('Ctrl Pts',(-14.0847177083086,-35.0480233633797,
18.4918491056432));
#29020=CARTESIAN_POINT('Ctrl Pts',(-14.0848982154794,-35.0326699856684,
18.4911044133067));
#29021=CARTESIAN_POINT('Ctrl Pts',(-14.0849921906863,-35.0173128016336,
18.4903597209703));
#29022=CARTESIAN_POINT('Ctrl Pts',(-14.0849995332614,-35.001952755595,18.4896150286338));
#29023=CARTESIAN_POINT('Origin',(-10.,-35.,32.7603849714045));
#29024=CARTESIAN_POINT('',(-7.51282745730979,-31.7594448403263,20.5469196554144));
#29025=CARTESIAN_POINT('',(-7.51282745730978,-31.7594448403263,20.4426717943404));
#29026=CARTESIAN_POINT('',(-7.5128274573098,-31.7594448403263,32.7603849714045));
#29027=CARTESIAN_POINT('',(-14.0849992317303,-34.9974946531383,19.6353849713615));
#29028=CARTESIAN_POINT('Ctrl Pts',(-7.51282745730978,-31.7594448403263,
20.4426717943404));
#29029=CARTESIAN_POINT('Ctrl Pts',(-7.41801457216884,-31.83221508894,20.4368682884277));
#29030=CARTESIAN_POINT('Ctrl Pts',(-7.32640772298353,-31.9091424187619,
20.4310647825151));
#29031=CARTESIAN_POINT('Ctrl Pts',(-7.23838002126121,-31.9899036405738,
20.4252612766024));
#29032=CARTESIAN_POINT('Ctrl Pts',(-7.15032437497231,-32.070690500194,20.4194559283555));
#29033=CARTESIAN_POINT('Ctrl Pts',(-7.06585043653951,-32.1553133963662,
20.4136505801085));
#29034=CARTESIAN_POINT('Ctrl Pts',(-6.98529490154283,-32.2434118607713,
20.4078452318615));
#29035=CARTESIAN_POINT('Ctrl Pts',(-6.90465041251276,-32.3316076085443,
20.4020334730167));
#29036=CARTESIAN_POINT('Ctrl Pts',(-6.82793323981866,-32.4232862840495,
20.3962217141718));
#29037=CARTESIAN_POINT('Ctrl Pts',(-6.7554402684333,-32.5180537579762,20.390409955327));
#29038=CARTESIAN_POINT('Ctrl Pts',(-6.68290012777349,-32.6128828946118,
20.3845944149231));
#29039=CARTESIAN_POINT('Ctrl Pts',(-6.61458989548414,-32.7108044981316,
20.3787788745193));
#29040=CARTESIAN_POINT('Ctrl Pts',(-6.55076260764328,-32.8113962416261,
20.3729633341154));
#29041=CARTESIAN_POINT('Ctrl Pts',(-6.48684340383313,-32.9121328445987,
20.3671394189075));
#29042=CARTESIAN_POINT('Ctrl Pts',(-6.42742023329891,-33.015546909901,20.3613155036995));
#29043=CARTESIAN_POINT('Ctrl Pts',(-6.37269984728246,-33.1211922391859,
20.3554915884915));
#29044=CARTESIAN_POINT('Ctrl Pts',(-6.35659889460636,-33.1522773716401,
20.3537779568822));
#29045=CARTESIAN_POINT('Ctrl Pts',(-6.34090477651809,-33.1835555567077,
20.3520643252729));
#29046=CARTESIAN_POINT('Ctrl Pts',(-6.32562195109587,-33.215015139075,20.3503506936635));
#29047=CARTESIAN_POINT('Ctrl Pts',(-6.27368491830175,-33.3219271344658,
20.3445271015834));
#29048=CARTESIAN_POINT('Ctrl Pts',(-6.22633417308424,-33.4312802038204,
20.3387035095032));
#29049=CARTESIAN_POINT('Ctrl Pts',(-6.18380574197683,-33.5426440431278,
20.332879917423));
#29050=CARTESIAN_POINT('Ctrl Pts',(-6.14133096681192,-33.6538673803851,
20.3270636726706));
#29051=CARTESIAN_POINT('Ctrl Pts',(-6.10366654908498,-33.767096063685,20.3212474279182));
#29052=CARTESIAN_POINT('Ctrl Pts',(-6.071002103367,-33.8818763358852,20.3154311831658));
#29053=CARTESIAN_POINT('Ctrl Pts',(-6.0383703549341,-33.9965417124183,20.3096207605055));
#29054=CARTESIAN_POINT('Ctrl Pts',(-6.01072873281045,-34.1127551975689,
20.3038103378452));
#29055=CARTESIAN_POINT('Ctrl Pts',(-5.98821810023126,-34.2300448138444,
20.297999915185));
#29056=CARTESIAN_POINT('Ctrl Pts',(-5.96485538495364,-34.3517741299987,
20.2919695537645));
#29057=CARTESIAN_POINT('Ctrl Pts',(-5.94701993528333,-34.4746622366628,
20.2859391923441));
#29058=CARTESIAN_POINT('Ctrl Pts',(-5.93481189984071,-34.5981658173782,
20.2799088309237));
#29059=CARTESIAN_POINT('Ctrl Pts',(-5.92306235444929,-34.7170310463039,
20.2741049482623));
#29060=CARTESIAN_POINT('Ctrl Pts',(-5.91652519881065,-34.8364659100945,
20.2683010656008));
#29061=CARTESIAN_POINT('Ctrl Pts',(-5.91523720607281,-34.9559782173449,
20.2624971829394));
#29062=CARTESIAN_POINT('Ctrl Pts',(-5.91394940358339,-35.0754728715235,
20.256694157565));
#29063=CARTESIAN_POINT('Ctrl Pts',(-5.91790922646807,-35.1950445382098,
20.2508911321906));
#29064=CARTESIAN_POINT('Ctrl Pts',(-5.92710133590371,-35.3141997326585,
20.2450881068162));
#29065=CARTESIAN_POINT('Ctrl Pts',(-5.93629425692309,-35.43336544748,20.2392845690849));
#29066=CARTESIAN_POINT('Ctrl Pts',(-5.95072035158373,-35.5521142098069,
20.2334810313536));
#29067=CARTESIAN_POINT('Ctrl Pts',(-5.97031234403708,-35.6699570100985,
20.2276774936223));
#29068=CARTESIAN_POINT('Ctrl Pts',(-5.98991068998727,-35.7878380256896,
20.2218720738589));
#29069=CARTESIAN_POINT('Ctrl Pts',(-6.01467819849276,-35.9048120923528,
20.2160666540955));
#29070=CARTESIAN_POINT('Ctrl Pts',(-6.04449648579143,-36.020400386654,20.2102612343321));
#29071=CARTESIAN_POINT('Ctrl Pts',(-6.07434779422287,-36.1361166848333,
20.2044493855764));
#29072=CARTESIAN_POINT('Ctrl Pts',(-6.1092609440807,-36.2504437517881,20.1986375368208));
#29073=CARTESIAN_POINT('Ctrl Pts',(-6.14906762696214,-36.3629177738547,
20.1928256880652));
#29074=CARTESIAN_POINT('Ctrl Pts',(-6.18890045518272,-36.4754656697343,
20.1870100220421));
#29075=CARTESIAN_POINT('Ctrl Pts',(-6.23363306476521,-36.5861577191303,
20.1811943560189));
#29076=CARTESIAN_POINT('Ctrl Pts',(-6.28304959839844,-36.6945514781304,
20.1753786899958));
#29077=CARTESIAN_POINT('Ctrl Pts',(-6.33253691615743,-36.8031005000943,
20.1695546936265));
#29078=CARTESIAN_POINT('Ctrl Pts',(-6.38672136438866,-36.9093442984082,
20.1637306972571));
#29079=CARTESIAN_POINT('Ctrl Pts',(-6.44534184579712,-37.012866216806,20.1579067008877));
#29080=CARTESIAN_POINT('Ctrl Pts',(-6.46089433286163,-37.0403314176725,
20.1563615476235));
#29081=CARTESIAN_POINT('Ctrl Pts',(-6.47675883432838,-37.067605196216,20.1548163943593));
#29082=CARTESIAN_POINT('Ctrl Pts',(-6.49292998448124,-37.0946801441388,
20.1532712410951));
#29083=CARTESIAN_POINT('Ctrl Pts',(-6.553878124316,-37.1967240740028,20.1474476468347));
#29084=CARTESIAN_POINT('Ctrl Pts',(-6.6193819464649,-37.2962702709819,20.1416240525744));
#29085=CARTESIAN_POINT('Ctrl Pts',(-6.6892109379969,-37.3928854521102,20.135800458314));
#29086=CARTESIAN_POINT('Ctrl Pts',(-6.75895182974484,-37.4893787386442,
20.1299842113944));
#29087=CARTESIAN_POINT('Ctrl Pts',(-6.83300680024026,-37.5829480363693,
20.1241679644748));
#29088=CARTESIAN_POINT('Ctrl Pts',(-6.91110027968808,-37.6731860238032,
20.1183517175552));
#29089=CARTESIAN_POINT('Ctrl Pts',(-6.9891155869673,-37.7633336823235,20.1125412927432));
#29090=CARTESIAN_POINT('Ctrl Pts',(-7.0711610953141,-37.8501563574677,20.1067308679311));
#29091=CARTESIAN_POINT('Ctrl Pts',(-7.15691927225585,-37.9332775142372,
20.1009204431191));
#29092=CARTESIAN_POINT('Ctrl Pts',(-7.24592356174802,-38.019544967253,20.094890082511));
#29093=CARTESIAN_POINT('Ctrl Pts',(-7.33892687397448,-38.1018247827203,
20.088859721903));
#29094=CARTESIAN_POINT('Ctrl Pts',(-7.43552969293042,-38.1797353732911,
20.082829361295));
#29095=CARTESIAN_POINT('Ctrl Pts',(-7.52850450245271,-38.2547199585896,
20.0770254765332));
#29096=CARTESIAN_POINT('Ctrl Pts',(-7.62481298225817,-38.3256573019792,
20.0712215917715));
#29097=CARTESIAN_POINT('Ctrl Pts',(-7.72406363516667,-38.3922468458574,
20.0654177070097));
#29098=CARTESIAN_POINT('Ctrl Pts',(-7.82329962745752,-38.4588265535903,
20.0596146795575));
#29099=CARTESIAN_POINT('Ctrl Pts',(-7.92547658957685,-38.5210595115568,
20.0538116521054));
#29100=CARTESIAN_POINT('Ctrl Pts',(-8.03017337674044,-38.578688038136,20.0480086246532));
#29101=CARTESIAN_POINT('Ctrl Pts',(-8.13487940727622,-38.6363216525688,
20.0422050848687));
#29102=CARTESIAN_POINT('Ctrl Pts',(-8.24210534743277,-38.6893498304572,
20.0364015450843));
#29103=CARTESIAN_POINT('Ctrl Pts',(-8.35140532536104,-38.7375607819475,
20.0305980052998));
#29104=CARTESIAN_POINT('Ctrl Pts',(-8.46074074771617,-38.7857873675631,
20.0247925835101));
#29105=CARTESIAN_POINT('Ctrl Pts',(-8.57215117204004,-38.8291934552923,
20.0189871617203));
#29106=CARTESIAN_POINT('Ctrl Pts',(-8.68517123033586,-38.8676155841117,
20.0131817399305));
#29107=CARTESIAN_POINT('Ctrl Pts',(-8.79831644740283,-38.9060802617184,
20.0073698891982));
#29108=CARTESIAN_POINT('Ctrl Pts',(-8.91307446965551,-38.9395498320075,
20.0015580384659));
#29109=CARTESIAN_POINT('Ctrl Pts',(-9.02896511595014,-38.9679108172889,
19.9957461877336));
#29110=CARTESIAN_POINT('Ctrl Pts',(-9.14493187956705,-38.9962904301501,
19.9899305197604));
#29111=CARTESIAN_POINT('Ctrl Pts',(-9.26203234915435,-39.0195546963855,
19.9841148517872));
#29112=CARTESIAN_POINT('Ctrl Pts',(-9.37977815200525,-39.0376416209552,
19.978299183814));
#29113=CARTESIAN_POINT('Ctrl Pts',(-9.49769261252338,-39.0557544530175,
19.9724751855482));
#29114=CARTESIAN_POINT('Ctrl Pts',(-9.61625384679987,-39.0686750974766,
19.9666511872824));
#29115=CARTESIAN_POINT('Ctrl Pts',(-9.7349702512338,-39.0763935325566,19.9608271890166));
#29116=CARTESIAN_POINT('Ctrl Pts',(-9.76646625873928,-39.0784412688435,
19.9592820555199));
#29117=CARTESIAN_POINT('Ctrl Pts',(-9.79797320079258,-39.0801231238753,
19.9577369220233));
#29118=CARTESIAN_POINT('Ctrl Pts',(-9.82948194037072,-39.0814395244007,
19.9561917885266));
#29119=CARTESIAN_POINT('Ctrl Pts',(-9.94823818709877,-39.0864010299283,
19.9503681898295));
#29120=CARTESIAN_POINT('Ctrl Pts',(-10.0674026593695,-39.0861831193878,
19.9445445911324));
#29121=CARTESIAN_POINT('Ctrl Pts',(-10.1864866122855,-39.0807410777257,
19.9387209924352));
#29122=CARTESIAN_POINT('Ctrl Pts',(-10.3054203237308,-39.0753059019791,
19.9329047410423));
#29123=CARTESIAN_POINT('Ctrl Pts',(-10.4242733135602,-39.0646597229128,
19.9270884896494));
#29124=CARTESIAN_POINT('Ctrl Pts',(-10.5425538518512,-39.0488097408796,
19.9212722382566));
#29125=CARTESIAN_POINT('Ctrl Pts',(-10.6607159911385,-39.0329756247032,
19.9154618089404));
#29126=CARTESIAN_POINT('Ctrl Pts',(-10.7783064164573,-39.0119481221722,
19.9096513796243));
#29127=CARTESIAN_POINT('Ctrl Pts',(-10.894836144462,-38.9857864060389,19.9038409503081));
#29128=CARTESIAN_POINT('Ctrl Pts',(-11.0157766202502,-38.9586344470429,
19.8978105913769));
#29129=CARTESIAN_POINT('Ctrl Pts',(-11.1355740679262,-38.9259519471033,
19.8917802324456));
#29130=CARTESIAN_POINT('Ctrl Pts',(-11.2536903398068,-38.8878638777451,
19.8857498735144));
#29131=CARTESIAN_POINT('Ctrl Pts',(-11.3673707651204,-38.8512062025995,
19.879945984201));
#29132=CARTESIAN_POINT('Ctrl Pts',(-11.4794935867999,-38.8095417843649,
19.8741420948877));
#29133=CARTESIAN_POINT('Ctrl Pts',(-11.5895928221178,-38.7630333057085,
19.8683382055744));
#29134=CARTESIAN_POINT('Ctrl Pts',(-11.6996757945346,-38.7165316968799,
19.8625351735611));
#29135=CARTESIAN_POINT('Ctrl Pts',(-11.8077353989698,-38.6651876094302,
19.8567321415478));
#29136=CARTESIAN_POINT('Ctrl Pts',(-11.9133252612175,-38.6092120254686,
19.8509291095345));
#29137=CARTESIAN_POINT('Ctrl Pts',(-12.0189244457598,-38.5532314995468,
19.8451255651843));
#29138=CARTESIAN_POINT('Ctrl Pts',(-12.1220530937882,-38.4926188553773,
19.8393220208342));
#29139=CARTESIAN_POINT('Ctrl Pts',(-12.2222896591848,-38.42763091226,19.8335184764841));
#29140=CARTESIAN_POINT('Ctrl Pts',(-12.3225587298375,-38.3626218945006,
19.8277130501292));
#29141=CARTESIAN_POINT('Ctrl Pts',(-12.4199335102169,-38.2932349780552,
19.8219076237743));
#29142=CARTESIAN_POINT('Ctrl Pts',(-12.5140221879713,-38.2197697803396,
19.8161021974194));
#29143=CARTESIAN_POINT('Ctrl Pts',(-12.6082150593581,-38.1462232273962,
19.8102903421458));
#29144=CARTESIAN_POINT('Ctrl Pts',(-12.6991142422774,-38.0685896297487,
19.8044784868722));
#29145=CARTESIAN_POINT('Ctrl Pts',(-12.7863616089684,-37.9872083931436,
19.7986666315986));
#29146=CARTESIAN_POINT('Ctrl Pts',(-12.8736662798165,-37.9057737052613,
19.7928509590927));
#29147=CARTESIAN_POINT('Ctrl Pts',(-12.9573140722942,-37.8205867670632,
19.7870352865868));
#29148=CARTESIAN_POINT('Ctrl Pts',(-13.0369854269177,-37.7320220564061,
19.7812196140809));
#29149=CARTESIAN_POINT('Ctrl Pts',(-13.1167709010918,-37.6433304875448,
19.7753956113296));
#29150=CARTESIAN_POINT('Ctrl Pts',(-13.1925683103788,-37.5512518034839,
19.7695716085784));
#29151=CARTESIAN_POINT('Ctrl Pts',(-13.2640997931654,-37.4561916741691,
19.7637476058271));
#29152=CARTESIAN_POINT('Ctrl Pts',(-13.2830768747935,-37.4309725152294,
19.7622025158708));
#29153=CARTESIAN_POINT('Ctrl Pts',(-13.3017539546748,-37.405543660053,19.7606574259145));
#29154=CARTESIAN_POINT('Ctrl Pts',(-13.3201263815374,-37.3799129838335,
19.7591123359582));
#29155=CARTESIAN_POINT('Ctrl Pts',(-13.3898878294926,-37.2825914324391,
19.7532455164367));
#29156=CARTESIAN_POINT('Ctrl Pts',(-13.4554778697672,-37.1820448960581,
19.7473786969153));
#29157=CARTESIAN_POINT('Ctrl Pts',(-13.5165873062648,-37.0786627233433,
19.7415118773939));
#29158=CARTESIAN_POINT('Ctrl Pts',(-13.5776176346634,-36.975414382122,19.7356526526559));
#29159=CARTESIAN_POINT('Ctrl Pts',(-13.6341786944696,-36.8693380470425,
19.729793427918));
#29160=CARTESIAN_POINT('Ctrl Pts',(-13.6860029550964,-36.7608541152011,
19.72393420318));
#29161=CARTESIAN_POINT('Ctrl Pts',(-13.7377717268428,-36.6524863384548,
19.7180812519869));
#29162=CARTESIAN_POINT('Ctrl Pts',(-13.7848136180123,-36.5417164522241,
19.7122283007938));
#29163=CARTESIAN_POINT('Ctrl Pts',(-13.8269059431142,-36.4289912185024,
19.7063753496006));
#29164=CARTESIAN_POINT('Ctrl Pts',(-13.8694507206623,-36.3150542957704,
19.700459484751));
#29165=CARTESIAN_POINT('Ctrl Pts',(-13.9069386754605,-36.1991200917361,
19.6945436199013));
#29166=CARTESIAN_POINT('Ctrl Pts',(-13.9391887252632,-36.0816733271922,
19.6886277550516));
#29167=CARTESIAN_POINT('Ctrl Pts',(-13.9710477424299,-35.9656506075172,
19.6827836202067));
#29168=CARTESIAN_POINT('Ctrl Pts',(-13.9977950643991,-35.8481522013055,
19.6769394853618));
#29169=CARTESIAN_POINT('Ctrl Pts',(-14.0193056312597,-35.7296624168231,
19.671095350517));
#29170=CARTESIAN_POINT('Ctrl Pts',(-14.041212224163,-35.6089911444811,19.6651436206649));
#29171=CARTESIAN_POINT('Ctrl Pts',(-14.0576872017008,-35.4872920340612,
19.6591918908128));
#29172=CARTESIAN_POINT('Ctrl Pts',(-14.0686527751091,-35.3650884763954,
19.6532401609607));
#29173=CARTESIAN_POINT('Ctrl Pts',(-14.0796183485174,-35.2428849187295,
19.6472884311087));
#29174=CARTESIAN_POINT('Ctrl Pts',(-14.0850744735076,-35.1201773507321,
19.6413367012566));
#29175=CARTESIAN_POINT('Ctrl Pts',(-14.0849992317308,-34.9974946540251,
19.6353849714045));
#29176=CARTESIAN_POINT('Ctrl Pts',(-14.0849992317303,-34.9974946531383,
19.6353849713615));
#29177=CARTESIAN_POINT('Ctrl Pts',(-14.0849166368598,-34.862822689068,19.6288516038181));
#29178=CARTESIAN_POINT('Ctrl Pts',(-14.0781702967129,-34.7283970591762,
19.6223182362747));
#29179=CARTESIAN_POINT('Ctrl Pts',(-14.0648574522931,-34.5948347342912,
19.6157848687313));
#29180=CARTESIAN_POINT('Ctrl Pts',(-14.051492035593,-34.4607449732116,19.6092257009893));
#29181=CARTESIAN_POINT('Ctrl Pts',(-14.0315082632746,-34.3275255447684,
19.6026665332472));
#29182=CARTESIAN_POINT('Ctrl Pts',(-14.0050544114292,-34.1957835108058,
19.5961073655052));
#29183=CARTESIAN_POINT('Ctrl Pts',(-13.9784604821396,-34.063343881366,19.5895134659041));
#29184=CARTESIAN_POINT('Ctrl Pts',(-13.945327873669,-33.9323975267073,19.582919566303));
#29185=CARTESIAN_POINT('Ctrl Pts',(-13.9058559311413,-33.8035408719191,
19.576325666702));
#29186=CARTESIAN_POINT('Ctrl Pts',(-13.8773364431503,-33.7104386432608,
19.5715614055979));
#29187=CARTESIAN_POINT('Ctrl Pts',(-13.8455085702689,-33.6184269108994,
19.5667971444938));
#29188=CARTESIAN_POINT('Ctrl Pts',(-13.81046272572,-33.5277232543104,19.5620328833897));
#29189=CARTESIAN_POINT('Ctrl Pts',(-13.767624377055,-33.4168514828874,19.5562092805936));
#29190=CARTESIAN_POINT('Ctrl Pts',(-13.7198739334846,-33.3076721551263,
19.5503856777975));
#29191=CARTESIAN_POINT('Ctrl Pts',(-13.6673654194799,-33.200651262261,19.5445620750014));
#29192=CARTESIAN_POINT('Ctrl Pts',(-13.6149231534501,-33.0937653935446,
19.5387458196211));
#29193=CARTESIAN_POINT('Ctrl Pts',(-13.5577349352383,-32.9890329066717,
19.5329295642409));
#29194=CARTESIAN_POINT('Ctrl Pts',(-13.4960035835794,-32.8869018140181,
19.5271133088607));
#29195=CARTESIAN_POINT('Ctrl Pts',(-13.4343340262757,-32.784872956693,19.521302875672));
#29196=CARTESIAN_POINT('Ctrl Pts',(-13.3681305927617,-32.6854406606044,
19.5154924424833));
#29197=CARTESIAN_POINT('Ctrl Pts',(-13.2976426612025,-32.589029681017,19.5096820092946));
#29198=CARTESIAN_POINT('Ctrl Pts',(-13.2244867693012,-32.4889695566128,
19.5036516518582));
#29199=CARTESIAN_POINT('Ctrl Pts',(-13.1467158332367,-32.3921643828436,
19.4976212944218));
#29200=CARTESIAN_POINT('Ctrl Pts',(-13.064659181786,-32.2990577385855,19.4915909369854));
#29201=CARTESIAN_POINT('Ctrl Pts',(-12.9856840928256,-32.2094476291906,
19.4857870441068));
#29202=CARTESIAN_POINT('Ctrl Pts',(-12.9027396703876,-32.1232636027136,
19.4799831512281));
#29203=CARTESIAN_POINT('Ctrl Pts',(-12.8161610266563,-32.0408680205266,
19.4741792583494));
#29204=CARTESIAN_POINT('Ctrl Pts',(-12.7295951733336,-31.9584846107775,
19.4683762228896));
#29205=CARTESIAN_POINT('Ctrl Pts',(-12.6393964621359,-31.8798888137317,
19.4625731874298));
#29206=CARTESIAN_POINT('Ctrl Pts',(-12.5459364683641,-31.8054057379608,
19.45677015197));
#29207=CARTESIAN_POINT('Ctrl Pts',(-12.4524682251862,-31.7309160878139,
19.4509666042954));
#29208=CARTESIAN_POINT('Ctrl Pts',(-12.3557384464404,-31.6605401352099,
19.4451630566208));
#29209=CARTESIAN_POINT('Ctrl Pts',(-12.2561508300465,-31.5945619324263,
19.4393595089461));
#29210=CARTESIAN_POINT('Ctrl Pts',(-12.156530921008,-31.5285623353094,19.4335540793919));
#29211=CARTESIAN_POINT('Ctrl Pts',(-12.0540516715701,-31.4669635494739,
19.4277486498377));
#29212=CARTESIAN_POINT('Ctrl Pts',(-11.9491441581158,-31.4100052853962,
19.4219432202834));
#29213=CARTESIAN_POINT('Ctrl Pts',(-11.8441204739503,-31.3529839478376,
19.4161313620106));
#29214=CARTESIAN_POINT('Ctrl Pts',(-11.7366635174216,-31.3006135843589,
19.4103195037378));
#29215=CARTESIAN_POINT('Ctrl Pts',(-11.6272274070774,-31.2530871419719,
19.404507645465));
#29216=CARTESIAN_POINT('Ctrl Pts',(-11.5177194211509,-31.20552948511,19.3986919700729));
#29217=CARTESIAN_POINT('Ctrl Pts',(-11.4062300731225,-31.1628222309038,
19.3928762946807));
#29218=CARTESIAN_POINT('Ctrl Pts',(-11.2932302505084,-31.1251089668005,
19.3870606192885));
#29219=CARTESIAN_POINT('Ctrl Pts',(-11.1800685730566,-31.0873416842563,
19.3812366138372));
#29220=CARTESIAN_POINT('Ctrl Pts',(-11.0653924939827,-31.0545827808194,
19.375412608386));
#29221=CARTESIAN_POINT('Ctrl Pts',(-10.9496848632193,-31.0269251629786,
19.3695886029348));
#29222=CARTESIAN_POINT('Ctrl Pts',(-10.9189886474781,-31.0195878404656,
19.3680435455636));
#29223=CARTESIAN_POINT('Ctrl Pts',(-10.8882198672476,-31.0126092612386,
19.3664984881925));
#29224=CARTESIAN_POINT('Ctrl Pts',(-10.8573875990132,-31.0059905477004,
19.3649534308213));
#29225=CARTESIAN_POINT('Ctrl Pts',(-10.7411646752692,-30.9810411591901,
19.3591293025521));
#29226=CARTESIAN_POINT('Ctrl Pts',(-10.62366441418,-30.9611287597988,19.3533051742829));
#29227=CARTESIAN_POINT('Ctrl Pts',(-10.5053611158976,-30.9463799952957,
19.3474810460137));
#29228=CARTESIAN_POINT('Ctrl Pts',(-10.3872094763206,-30.9316501379454,
19.3416643839755));
#29229=CARTESIAN_POINT('Ctrl Pts',(-10.2682572490579,-30.9220707984628,
19.3358477219373));
#29230=CARTESIAN_POINT('Ctrl Pts',(-10.148990417942,-30.9177179353502,19.3300310598991));
#29231=CARTESIAN_POINT('Ctrl Pts',(-10.0298630331131,-30.9133701615872,
19.3242211986782));
#29232=CARTESIAN_POINT('Ctrl Pts',(-9.91042218245955,-30.9142367134684,
19.3184113374573));
#29233=CARTESIAN_POINT('Ctrl Pts',(-9.79115967193203,-30.9203418381717,
19.3126014762363));
#29234=CARTESIAN_POINT('Ctrl Pts',(-9.67197562219243,-30.9264429464167,
19.3067954372248));
#29235=CARTESIAN_POINT('Ctrl Pts',(-9.55297008553151,-30.9377757534022,
19.3009893982133));
#29236=CARTESIAN_POINT('Ctrl Pts',(-9.43463534023889,-30.954312443911,19.2951833592017));
#29237=CARTESIAN_POINT('Ctrl Pts',(-9.3163505181675,-30.9708421578986,19.2893797696497));
#29238=CARTESIAN_POINT('Ctrl Pts',(-9.19873632821924,-30.992571331977,19.2835761800977));
#29239=CARTESIAN_POINT('Ctrl Pts',(-9.08227975844286,-31.0194203238427,
19.2777725905457));
#29240=CARTESIAN_POINT('Ctrl Pts',(-8.9658448366947,-31.0462643247686,19.2719700798188));
#29241=CARTESIAN_POINT('Ctrl Pts',(-8.85056750435854,-31.0782261572829,
19.2661675690919));
#29242=CARTESIAN_POINT('Ctrl Pts',(-8.73692375970745,-31.115175240605,19.260365058365));
#29243=CARTESIAN_POINT('Ctrl Pts',(-8.62322686242791,-31.1521416054845,
19.2545598337299));
#29244=CARTESIAN_POINT('Ctrl Pts',(-8.51116546951101,-31.1940997595864,
19.2487546090947));
#29245=CARTESIAN_POINT('Ctrl Pts',(-8.40119959948887,-31.2408694782802,
19.2429493844596));
#29246=CARTESIAN_POINT('Ctrl Pts',(-8.29121022613133,-31.2876491932063,
19.2371429190563));
#29247=CARTESIAN_POINT('Ctrl Pts',(-8.18331763951256,-31.3392423514837,
19.2313364536531));
#29248=CARTESIAN_POINT('Ctrl Pts',(-8.07795982296281,-31.3954214451819,
19.2255299882498));
#29249=CARTESIAN_POINT('Ctrl Pts',(-7.97248668849355,-31.4516620289186,
19.2197171674614));
#29250=CARTESIAN_POINT('Ctrl Pts',(-7.86955422295094,-31.5124983750139,
19.2139043466729));
#29251=CARTESIAN_POINT('Ctrl Pts',(-7.76957409372478,-31.5776579252482,
19.2080915258845));
#29252=CARTESIAN_POINT('Ctrl Pts',(-7.68162090265582,-31.6349792191501,
19.2029779484025));
#29253=CARTESIAN_POINT('Ctrl Pts',(-7.59595220320821,-31.6956454061462,
19.1978643709205));
#29254=CARTESIAN_POINT('Ctrl Pts',(-7.5128274573098,-31.7594448403263,19.1927507934385));
#29255=CARTESIAN_POINT('',(-14.0849997388207,-35.001460765222,19.7396150285601));
#29256=CARTESIAN_POINT('Ctrl Pts',(-14.0849997388207,-35.0014607652219,
19.7396150285601));
#29257=CARTESIAN_POINT('Ctrl Pts',(-14.0850418772244,-34.8836215905298,
19.7338448932755));
#29258=CARTESIAN_POINT('Ctrl Pts',(-14.0799808576064,-34.7655803559852,
19.7280747579908));
#29259=CARTESIAN_POINT('Ctrl Pts',(-14.0697904347131,-34.6478199075505,
19.7223046227062));
#29260=CARTESIAN_POINT('Ctrl Pts',(-14.059612412446,-34.530202760656,19.7165415090428));
#29261=CARTESIAN_POINT('Ctrl Pts',(-14.0443174331435,-34.4128661318137,
19.7107783953795));
#29262=CARTESIAN_POINT('Ctrl Pts',(-14.0239312542375,-34.2962939099519,
19.7050152817162));
#29263=CARTESIAN_POINT('Ctrl Pts',(-14.0035643214882,-34.179831741439,19.6992576088855));
#29264=CARTESIAN_POINT('Ctrl Pts',(-13.9781158193059,-34.0641329527669,
19.6934999360549));
#29265=CARTESIAN_POINT('Ctrl Pts',(-13.9476633382702,-33.9496766366128,
19.6877422632243));
#29266=CARTESIAN_POINT('Ctrl Pts',(-13.917229973243,-33.8352921683947,19.6819882046713));
#29267=CARTESIAN_POINT('Ctrl Pts',(-13.8817989824691,-33.7221490230879,
19.6762341461184));
#29268=CARTESIAN_POINT('Ctrl Pts',(-13.8414989710686,-33.6107157759194,
19.6704800875654));
#29269=CARTESIAN_POINT('Ctrl Pts',(-13.8012118048751,-33.4993180469328,
19.6647278630584));
#29270=CARTESIAN_POINT('Ctrl Pts',(-13.7560588442483,-33.3896295240911,
19.6589756385515));
#29271=CARTESIAN_POINT('Ctrl Pts',(-13.7062182517548,-33.2821026601221,
19.6532234140445));
#29272=CARTESIAN_POINT('Ctrl Pts',(-13.6563812419505,-33.1745835255022,
19.6474716030244));
#29273=CARTESIAN_POINT('Ctrl Pts',(-13.6018574456382,-33.0692261185813,
19.6417197920044));
#29274=CARTESIAN_POINT('Ctrl Pts',(-13.5428724621768,-32.9664612822105,
19.6359679809843));
#29275=CARTESIAN_POINT('Ctrl Pts',(-13.4838771573901,-32.8636784638169,
19.6302151634994));
#29276=CARTESIAN_POINT('Ctrl Pts',(-13.4204193215166,-32.7634894786887,
19.6244623460145));
#29277=CARTESIAN_POINT('Ctrl Pts',(-13.3527692482539,-32.6662983549813,
19.6187095285296));
#29278=CARTESIAN_POINT('Ctrl Pts',(-13.2850503479888,-32.5690083492862,
19.6129508581436));
#29279=CARTESIAN_POINT('Ctrl Pts',(-13.2131309321623,-32.47472263748,19.6071921877577));
#29280=CARTESIAN_POINT('Ctrl Pts',(-13.1373232306751,-32.3838142370492,
19.6014335173717));
#29281=CARTESIAN_POINT('Ctrl Pts',(-13.0614743849762,-32.2928564965856,
19.5956717214992));
#29282=CARTESIAN_POINT('Ctrl Pts',(-12.9817333318425,-32.205280024942,19.5899099256267));
#29283=CARTESIAN_POINT('Ctrl Pts',(-12.8984497562577,-32.1214215295654,
19.5841481297542));
#29284=CARTESIAN_POINT('Ctrl Pts',(-12.8150375631549,-32.0374335288036,
19.578377435754));
#29285=CARTESIAN_POINT('Ctrl Pts',(-12.7280722279227,-31.957175253068,19.5726067417539));
#29286=CARTESIAN_POINT('Ctrl Pts',(-12.6379373769759,-31.8809438294328,
19.5668360477537));
#29287=CARTESIAN_POINT('Ctrl Pts',(-12.5752148457861,-31.827896336744,19.5628203697933));
#29288=CARTESIAN_POINT('Ctrl Pts',(-12.5109581856905,-31.7767979505961,
19.5588046918329));
#29289=CARTESIAN_POINT('Ctrl Pts',(-12.4453045397188,-31.7277361493867,
19.5547890138725));
#29290=CARTESIAN_POINT('Ctrl Pts',(-12.3500926002635,-31.6565859615001,
19.5489654151801));
#29291=CARTESIAN_POINT('Ctrl Pts',(-12.2516191999004,-31.5894800129192,
19.5431418164876));
#29292=CARTESIAN_POINT('Ctrl Pts',(-12.1502624676698,-31.526731176524,19.5373182177951));
#29293=CARTESIAN_POINT('Ctrl Pts',(-12.0490336114812,-31.4640615067777,
19.5315019664069));
#29294=CARTESIAN_POINT('Ctrl Pts',(-11.9449290029249,-31.4057382286165,
19.5256857150186));
#29295=CARTESIAN_POINT('Ctrl Pts',(-11.8383585485305,-31.3520330529122,
19.5198694636304));
#29296=CARTESIAN_POINT('Ctrl Pts',(-11.7318947713275,-31.2983816361728,
19.5140590343189));
#29297=CARTESIAN_POINT('Ctrl Pts',(-11.6229704212492,-31.2493393082513,
19.5082486050074));
#29298=CARTESIAN_POINT('Ctrl Pts',(-11.5120224840164,-31.2051333346442,
19.5024381756959));
#29299=CARTESIAN_POINT('Ctrl Pts',(-11.3968750743293,-31.1592541278692,
19.4964078167629));
#29300=CARTESIAN_POINT('Ctrl Pts',(-11.2795482429684,-31.1185848652021,
19.4903774578299));
#29301=CARTESIAN_POINT('Ctrl Pts',(-11.1605567056453,-31.0833262667179,
19.4843470988969));
#29302=CARTESIAN_POINT('Ctrl Pts',(-11.0460338855338,-31.0493918019448,
19.4785432095883));
#29303=CARTESIAN_POINT('Ctrl Pts',(-10.92996956717,-31.0204690622736,19.4727393202796));
#29304=CARTESIAN_POINT('Ctrl Pts',(-10.8128401996152,-30.9966868958462,
19.4669354309709));
#29305=CARTESIAN_POINT('Ctrl Pts',(-10.6957281333917,-30.9729082423135,
19.4611323989623));
#29306=CARTESIAN_POINT('Ctrl Pts',(-10.5775517308993,-30.9542687332049,
19.4553293669537));
#29307=CARTESIAN_POINT('Ctrl Pts',(-10.4587985297507,-30.9408462816618,
19.4495263349451));
#29308=CARTESIAN_POINT('Ctrl Pts',(-10.3400348441456,-30.9274226450803,
19.4437227905996));
#29309=CARTESIAN_POINT('Ctrl Pts',(-10.220694664407,-30.9192170277171,19.4379192462542));
#29310=CARTESIAN_POINT('Ctrl Pts',(-10.1012709185177,-30.9162554926804,
19.4321157019087));
#29311=CARTESIAN_POINT('Ctrl Pts',(-9.98180844524824,-30.9132929972612,
19.4263102755585));
#29312=CARTESIAN_POINT('Ctrl Pts',(-9.86226275993423,-30.9155779763552,
19.4205048492082));
#29313=CARTESIAN_POINT('Ctrl Pts',(-9.74312641610772,-30.9230843813125,
19.4146994228579));
#29314=CARTESIAN_POINT('Ctrl Pts',(-9.62385814090777,-30.9305990988491,
19.4088875675889));
#29315=CARTESIAN_POINT('Ctrl Pts',(-9.50500051979866,-30.9433467583186,
19.4030757123199));
#29316=CARTESIAN_POINT('Ctrl Pts',(-9.38704077165203,-30.9612494525679,
19.3972638570509));
#29317=CARTESIAN_POINT('Ctrl Pts',(-9.26900354742514,-30.9791639053247,
19.3914481845496));
#29318=CARTESIAN_POINT('Ctrl Pts',(-9.15186577032583,-31.0022400570877,
19.3856325120482));
#29319=CARTESIAN_POINT('Ctrl Pts',(-9.0361026309011,-31.030349277097,19.3798168395469));
#29320=CARTESIAN_POINT('Ctrl Pts',(-8.92017367482114,-31.0584987601543,
19.3739928368001));
#29321=CARTESIAN_POINT('Ctrl Pts',(-8.80562367724287,-31.091695587492,19.3681688340534));
#29322=CARTESIAN_POINT('Ctrl Pts',(-8.69291102659217,-31.1297618399386,
19.3623448313066));
#29323=CARTESIAN_POINT('Ctrl Pts',(-8.66300870733518,-31.1398606995342,
19.3607997413058));
#29324=CARTESIAN_POINT('Ctrl Pts',(-8.63323558515604,-31.1503020232743,
19.3592546513049));
#29325=CARTESIAN_POINT('Ctrl Pts',(-8.60359994560332,-31.1610819378266,
19.3577095613041));
#29326=CARTESIAN_POINT('Ctrl Pts',(-8.49191615464733,-31.2017067308648,
19.3518867914478));
#29327=CARTESIAN_POINT('Ctrl Pts',(-8.38182657333516,-31.2472748149992,
19.3460640215914));
#29328=CARTESIAN_POINT('Ctrl Pts',(-8.27379995922212,-31.2976415058481,
19.3402412517351));
#29329=CARTESIAN_POINT('Ctrl Pts',(-8.16589302622355,-31.3479523961729,
19.3344249328408));
#29330=CARTESIAN_POINT('Ctrl Pts',(-8.06004488446533,-31.4030511558678,
19.3286086139465));
#29331=CARTESIAN_POINT('Ctrl Pts',(-7.95670750152521,-31.4627438931176,
19.3227922950522));
#29332=CARTESIAN_POINT('Ctrl Pts',(-7.85348150489727,-31.5223722881742,
19.3169822455088));
#29333=CARTESIAN_POINT('Ctrl Pts',(-7.75276123275879,-31.5865846031199,
19.3111721959653));
#29334=CARTESIAN_POINT('Ctrl Pts',(-7.65497622498272,-31.6551399887882,
19.3053621464219));
#29335=CARTESIAN_POINT('Ctrl Pts',(-7.60686687164105,-31.6888686282556,
19.3025036537677));
#29336=CARTESIAN_POINT('Ctrl Pts',(-7.55946765824416,-31.7236478174602,
19.2996451611135));
#29337=CARTESIAN_POINT('Ctrl Pts',(-7.51282745730977,-31.7594448403263,
19.2967866684593));
#29338=CARTESIAN_POINT('Ctrl Pts',(-7.51282745730979,-31.7594448403263,
20.5469196554144));
#29339=CARTESIAN_POINT('Ctrl Pts',(-7.47644412383199,-31.7873695703737,
20.5446751958479));
#29340=CARTESIAN_POINT('Ctrl Pts',(-7.44055213223825,-31.8158910003058,
20.5424307362813));
#29341=CARTESIAN_POINT('Ctrl Pts',(-7.40517161094806,-31.8449895988491,
20.5401862767148));
#29342=CARTESIAN_POINT('Ctrl Pts',(-7.31337143933769,-31.9204903614861,
20.534362683227));
#29343=CARTESIAN_POINT('Ctrl Pts',(-7.22472119483735,-32.0001228138231,
20.5285390897392));
#29344=CARTESIAN_POINT('Ctrl Pts',(-7.13961488664204,-32.0835943349252,
20.5227154962513));
#29345=CARTESIAN_POINT('Ctrl Pts',(-7.05461595269594,-32.1669605443049,
20.5168992500917));
#29346=CARTESIAN_POINT('Ctrl Pts',(-6.97315235089349,-32.2541559053276,
20.5110830039321));
#29347=CARTESIAN_POINT('Ctrl Pts',(-6.89558569267423,-32.3448471214502,
20.5052667577725));
#29348=CARTESIAN_POINT('Ctrl Pts',(-6.81809667910428,-32.4354475551693,
20.4994563337071));
#29349=CARTESIAN_POINT('Ctrl Pts',(-6.74449711271978,-32.5295365738911,
20.4936459096417));
#29350=CARTESIAN_POINT('Ctrl Pts',(-6.67511189826874,-32.6267439853724,
20.4878354855764));
#29351=CARTESIAN_POINT('Ctrl Pts',(-6.60310030684887,-32.7276309027648,
20.4818051246834));
#29352=CARTESIAN_POINT('Ctrl Pts',(-6.53562873542885,-32.8318766390586,
20.4757747637905));
#29353=CARTESIAN_POINT('Ctrl Pts',(-6.47301484396659,-32.9390291828558,
20.4697444028976));
#29354=CARTESIAN_POINT('Ctrl Pts',(-6.41275248611149,-33.0421574949379,
20.4639405188451));
#29355=CARTESIAN_POINT('Ctrl Pts',(-6.35698974170198,-33.1479778309798,
20.4581366347925));
#29356=CARTESIAN_POINT('Ctrl Pts',(-6.30596534631192,-33.2560582070059,
20.45233275074));
#29357=CARTESIAN_POINT('Ctrl Pts',(-6.25494848776096,-33.3641226184252,
20.4465297239821));
#29358=CARTESIAN_POINT('Ctrl Pts',(-6.20866876061912,-33.4744460367868,
20.4407266972242));
#29359=CARTESIAN_POINT('Ctrl Pts',(-6.16731807849836,-33.5865735644914,
20.4349236704663));
#29360=CARTESIAN_POINT('Ctrl Pts',(-6.12596374553521,-33.6987109919102,
20.4291201313605));
#29361=CARTESIAN_POINT('Ctrl Pts',(-6.0895394641378,-33.8126524622339,20.4233165922547));
#29362=CARTESIAN_POINT('Ctrl Pts',(-6.05818807864224,-33.9279254799027,
20.4175130531489));
#29363=CARTESIAN_POINT('Ctrl Pts',(-6.02682652624944,-34.0432358792983,
20.4117076320214));
#29364=CARTESIAN_POINT('Ctrl Pts',(-6.00054124856552,-34.1598782909817,
20.405902210894));
#29365=CARTESIAN_POINT('Ctrl Pts',(-5.97942439191471,-34.2773681575867,
20.4000967897665));
#29366=CARTESIAN_POINT('Ctrl Pts',(-5.95828415028766,-34.3949881334113,
20.3942849396692));
#29367=CARTESIAN_POINT('Ctrl Pts',(-5.94232382666853,-34.5134570353053,
20.3884730895719));
#29368=CARTESIAN_POINT('Ctrl Pts',(-5.93158393261422,-34.6322831216313,
20.3826612394745));
#29369=CARTESIAN_POINT('Ctrl Pts',(-5.92083698453664,-34.7511872536041,
20.3768455721211));
#29370=CARTESIAN_POINT('Ctrl Pts',(-5.91531731341602,-34.8704486302597,
20.3710299047677));
#29371=CARTESIAN_POINT('Ctrl Pts',(-5.91501330217641,-34.9895750969147,
20.3652142374143));
#29372=CARTESIAN_POINT('Ctrl Pts',(-5.91470885547333,-35.1088721994499,
20.3593902397415));
#29373=CARTESIAN_POINT('Ctrl Pts',(-5.91963496330141,-35.2280335997395,
20.3535662420687));
#29374=CARTESIAN_POINT('Ctrl Pts',(-5.92972813549782,-35.3465717083692,
20.3477422443959));
#29375=CARTESIAN_POINT('Ctrl Pts',(-5.93240591213912,-35.3780205504394,
20.3461971043127));
#29376=CARTESIAN_POINT('Ctrl Pts',(-5.93544710454838,-35.4094255757416,
20.3446519642295));
#29377=CARTESIAN_POINT('Ctrl Pts',(-5.93884992651983,-35.4407778132711,
20.3431068241463));
#29378=CARTESIAN_POINT('Ctrl Pts',(-5.95167507597797,-35.5589435990619,
20.3372832304741));
#29379=CARTESIAN_POINT('Ctrl Pts',(-5.96968252705702,-35.6767397184615,
20.3314596368018));
#29380=CARTESIAN_POINT('Ctrl Pts',(-5.99284352153497,-35.7936762293881,
20.3256360431296));
#29381=CARTESIAN_POINT('Ctrl Pts',(-6.01597529497144,-35.9104652075031,
20.3198197967874));
#29382=CARTESIAN_POINT('Ctrl Pts',(-6.04424760092048,-36.0263963372128,
20.3140035504453));
#29383=CARTESIAN_POINT('Ctrl Pts',(-6.07757990198573,-36.1409844760967,
20.3081873041032));
#29384=CARTESIAN_POINT('Ctrl Pts',(-6.11087883722424,-36.2554579115889,
20.3023768798574));
#29385=CARTESIAN_POINT('Ctrl Pts',(-6.14922757782333,-36.3685906408246,
20.2965664556116));
#29386=CARTESIAN_POINT('Ctrl Pts',(-6.1924946066162,-36.4799079969219,20.2907560313658));
#29387=CARTESIAN_POINT('Ctrl Pts',(-6.23739938196257,-36.5954389452481,
20.2847256705413));
#29388=CARTESIAN_POINT('Ctrl Pts',(-6.28760204993146,-36.7090139340734,
20.2786953097168));
#29389=CARTESIAN_POINT('Ctrl Pts',(-6.34289869087207,-36.82011950563,20.2726649488923));
#29390=CARTESIAN_POINT('Ctrl Pts',(-6.39611860780277,-36.9270523895845,
20.2668610646656));
#29391=CARTESIAN_POINT('Ctrl Pts',(-6.45405658032985,-37.0316975960583,
20.261057180439));
#29392=CARTESIAN_POINT('Ctrl Pts',(-6.51648217566361,-37.1336186556015,
20.2552532962123));
#29393=CARTESIAN_POINT('Ctrl Pts',(-6.57889855005348,-37.2355246602883,
20.2494502692829));
#29394=CARTESIAN_POINT('Ctrl Pts',(-6.64580101578983,-37.3347069701451,
20.2436472423535));
#29395=CARTESIAN_POINT('Ctrl Pts',(-6.71691430969483,-37.4307557158451,
20.2378442154241));
#29396=CARTESIAN_POINT('Ctrl Pts',(-6.78803388214217,-37.5268129416207,
20.2320406761496));
#29397=CARTESIAN_POINT('Ctrl Pts',(-6.86336477893826,-37.6197357249787,
20.2262371368751));
#29398=CARTESIAN_POINT('Ctrl Pts',(-6.9425901204879,-37.709145590156,20.2204335976005));
#29399=CARTESIAN_POINT('Ctrl Pts',(-7.02184115387228,-37.7985844498878,
20.2146281763073));
#29400=CARTESIAN_POINT('Ctrl Pts',(-7.10498887301,-37.8845078203705,20.2088227550141));
#29401=CARTESIAN_POINT('Ctrl Pts',(-7.19167851935393,-37.966573016351,20.2030173337209));
#29402=CARTESIAN_POINT('Ctrl Pts',(-7.27846416642655,-38.0487290919111,
20.197205483463));
#29403=CARTESIAN_POINT('Ctrl Pts',(-7.36879927334768,-38.1270181836673,
20.1913936332051));
#29404=CARTESIAN_POINT('Ctrl Pts',(-7.46229476855321,-38.2011368540391,
20.1855817829472));
#29405=CARTESIAN_POINT('Ctrl Pts',(-7.55585167208242,-38.2753042059362,
20.1797661154361));
#29406=CARTESIAN_POINT('Ctrl Pts',(-7.65257276777595,-38.3452954425188,
20.173950447925));
#29407=CARTESIAN_POINT('Ctrl Pts',(-7.75204006358966,-38.4108504986724,
20.1681347804138));
#29408=CARTESIAN_POINT('Ctrl Pts',(-7.85164983553608,-38.4764994553469,
20.1623107825886));
#29409=CARTESIAN_POINT('Ctrl Pts',(-7.95401330969173,-38.5376993398648,
20.1564867847634));
#29410=CARTESIAN_POINT('Ctrl Pts',(-8.05868787733256,-38.5942359747775,
20.1506627869382));
#29411=CARTESIAN_POINT('Ctrl Pts',(-8.08645861221458,-38.6092354530143,
20.1491176484847));
#29412=CARTESIAN_POINT('Ctrl Pts',(-8.11439191096311,-38.6239069627225,
20.1475725100313));
#29413=CARTESIAN_POINT('Ctrl Pts',(-8.14247929138295,-38.6382470802653,
20.1460273715779));
#29414=CARTESIAN_POINT('Ctrl Pts',(-8.24834003862632,-38.6922946822824,
20.1402037771796));
#29415=CARTESIAN_POINT('Ctrl Pts',(-8.35673235688323,-38.741805317745,20.1343801827814));
#29416=CARTESIAN_POINT('Ctrl Pts',(-8.46723070838592,-38.7865344708169,
20.1285565883832));
#29417=CARTESIAN_POINT('Ctrl Pts',(-8.57758964987418,-38.8312071914463,
20.1227403413106));
#29418=CARTESIAN_POINT('Ctrl Pts',(-8.69004896458759,-38.8711102764148,
20.1169240942381));
#29419=CARTESIAN_POINT('Ctrl Pts',(-8.80415874560844,-38.9060451474983,
20.1111078471656));
#29420=CARTESIAN_POINT('Ctrl Pts',(-8.91815430215916,-38.9409450485985,
20.1052974221859));
#29421=CARTESIAN_POINT('Ctrl Pts',(-9.03379665011463,-38.9708865105447,
20.0994869972062));
#29422=CARTESIAN_POINT('Ctrl Pts',(-9.15061669875019,-38.9957193354336,
20.0936765722265));
#29423=CARTESIAN_POINT('Ctrl Pts',(-9.27185860709382,-39.0214921296951,
20.0876462116758));
#29424=CARTESIAN_POINT('Ctrl Pts',(-9.39436871862172,-39.041761734177,20.0816158511251));
#29425=CARTESIAN_POINT('Ctrl Pts',(-9.51760581090146,-39.0564172426322,
20.0755854905744));
#29426=CARTESIAN_POINT('Ctrl Pts',(-9.63621462391286,-39.0705223503542,
20.0697816056099));
#29427=CARTESIAN_POINT('Ctrl Pts',(-9.75549635563586,-39.0794273897883,
20.0639777206454));
#29428=CARTESIAN_POINT('Ctrl Pts',(-9.87495964064826,-39.0830858316393,
20.0581738356809));
#29429=CARTESIAN_POINT('Ctrl Pts',(-9.99440527963151,-39.0867437330984,
20.0523708080135));
#29430=CARTESIAN_POINT('Ctrl Pts',(-10.1140320105376,-39.0851565656684,
20.046567780346));
#29431=CARTESIAN_POINT('Ctrl Pts',(-10.2333461411369,-39.0783298761155,
20.0407647526786));
#29432=CARTESIAN_POINT('Ctrl Pts',(-10.3526708058821,-39.0715025838399,
20.0349612126666));
#29433=CARTESIAN_POINT('Ctrl Pts',(-10.4716824077565,-39.059434873021,20.0291576726547));
#29434=CARTESIAN_POINT('Ctrl Pts',(-10.589890698599,-39.0421843060042,20.0233541326428));
#29435=CARTESIAN_POINT('Ctrl Pts',(-10.7081373229486,-39.0249281448388,
20.0175487106136));
#29436=CARTESIAN_POINT('Ctrl Pts',(-10.8255797143336,-39.0024858438039,
20.0117432885844));
#29437=CARTESIAN_POINT('Ctrl Pts',(-10.9417367948808,-38.9749662651609,
20.0059378665552));
#29438=CARTESIAN_POINT('Ctrl Pts',(-11.0580225084692,-38.9474162111731,
20.0001260155672));
#29439=CARTESIAN_POINT('Ctrl Pts',(-11.1730196724962,-38.9147777505631,
19.9943141645791));
#29440=CARTESIAN_POINT('Ctrl Pts',(-11.2862612255628,-38.8772099581547,
19.9885023135911));
#29441=CARTESIAN_POINT('Ctrl Pts',(-11.3995771562069,-38.8396174910458,
19.9826866453524));
#29442=CARTESIAN_POINT('Ctrl Pts',(-11.5111347988012,-38.7970893894815,
19.9768709771136));
#29443=CARTESIAN_POINT('Ctrl Pts',(-11.6204875142691,-38.7498326917475,
19.9710553088749));
#29444=CARTESIAN_POINT('Ctrl Pts',(-11.7299968654689,-38.702508303994,19.9652313103314));
#29445=CARTESIAN_POINT('Ctrl Pts',(-11.837294619651,-38.6504419787779,19.9594073117878));
#29446=CARTESIAN_POINT('Ctrl Pts',(-11.9419590228879,-38.5938864970147,
19.9535833132443));
#29447=CARTESIAN_POINT('Ctrl Pts',(-11.9697269311232,-38.5788820888373,
19.9520381818327));
#29448=CARTESIAN_POINT('Ctrl Pts',(-11.9973096492124,-38.5635619394124,
19.950493050421));
#29449=CARTESIAN_POINT('Ctrl Pts',(-12.0246996641969,-38.5479312662171,
19.9489479190094));
#29450=CARTESIAN_POINT('Ctrl Pts',(-12.1279324851569,-38.4890193419862,
19.943124326928));
#29451=CARTESIAN_POINT('Ctrl Pts',(-12.2287584359163,-38.4255030880873,
19.9373007348465));
#29452=CARTESIAN_POINT('Ctrl Pts',(-12.3267397463782,-38.357604377026,19.931477142765));
#29453=CARTESIAN_POINT('Ctrl Pts',(-12.4245974388409,-38.2897913302895,
19.9256608980113));
#29454=CARTESIAN_POINT('Ctrl Pts',(-12.5196172966492,-38.2176070542147,
19.9198446532575));
#29455=CARTESIAN_POINT('Ctrl Pts',(-12.6113866122977,-38.1413189842982,
19.9140284085038));
#29456=CARTESIAN_POINT('Ctrl Pts',(-12.7030640663699,-38.0651072791481,
19.9082179858422));
#29457=CARTESIAN_POINT('Ctrl Pts',(-12.7914971391326,-37.9848002118877,
19.9024075631806));
#29458=CARTESIAN_POINT('Ctrl Pts',(-12.876303071105,-37.9007077831371,19.896597140519));
#29459=CARTESIAN_POINT('Ctrl Pts',(-12.9643191157427,-37.8134322495691,
19.8905667790991));
#29460=CARTESIAN_POINT('Ctrl Pts',(-13.048427633254,-37.7220793771287,19.8845364176792));
#29461=CARTESIAN_POINT('Ctrl Pts',(-13.1282391859743,-37.6270410341932,
19.8785060562593));
#29462=CARTESIAN_POINT('Ctrl Pts',(-13.2050533028845,-37.535571990723,19.8727021735965));
#29463=CARTESIAN_POINT('Ctrl Pts',(-13.2778871054155,-37.4406896514441,
19.8668982909338));
#29464=CARTESIAN_POINT('Ctrl Pts',(-13.3464323293442,-37.3427794742826,
19.861094408271));
#29465=CARTESIAN_POINT('Ctrl Pts',(-13.4149674285101,-37.2448837593589,
19.8552913828954));
#29466=CARTESIAN_POINT('Ctrl Pts',(-13.4792149747097,-37.1439614303904,
19.8494883575197));
#29467=CARTESIAN_POINT('Ctrl Pts',(-13.5389089831636,-37.0404284375796,
19.843685332144));
#29468=CARTESIAN_POINT('Ctrl Pts',(-13.598608262082,-36.9368863037015,19.8378817944115));
#29469=CARTESIAN_POINT('Ctrl Pts',(-13.6537529999346,-36.8307334014606,
19.8320782566789));
#29470=CARTESIAN_POINT('Ctrl Pts',(-13.7041226041859,-36.7224113135831,
19.8262747189463));
#29471=CARTESIAN_POINT('Ctrl Pts',(-13.7545085428211,-36.614054097882,19.8204692991816));
#29472=CARTESIAN_POINT('Ctrl Pts',(-13.8001160960937,-36.5035266676226,
19.8146638794168));
#29473=CARTESIAN_POINT('Ctrl Pts',(-13.840772604059,-36.3912910565048,19.8088584596521));
#29474=CARTESIAN_POINT('Ctrl Pts',(-13.8814741355335,-36.2789311543118,
19.8030466108953));
#29475=CARTESIAN_POINT('Ctrl Pts',(-13.9172135383115,-36.1648596794967,
19.7972347621384));
#29476=CARTESIAN_POINT('Ctrl Pts',(-13.9478678321096,-36.049554467474,19.7914229133815));
#29477=CARTESIAN_POINT('Ctrl Pts',(-13.9785422598863,-35.9341735220908,
19.7856072473571));
#29478=CARTESIAN_POINT('Ctrl Pts',(-14.0041248398133,-35.8175576236468,
19.7797915813328));
#29479=CARTESIAN_POINT('Ctrl Pts',(-14.0245439016398,-35.7001938187202,
19.7739759153084));
#29480=CARTESIAN_POINT('Ctrl Pts',(-14.044992211682,-35.5826619021581,19.7681519189378));
#29481=CARTESIAN_POINT('Ctrl Pts',(-14.0602621890924,-35.4643803443969,
19.7623279225673));
#29482=CARTESIAN_POINT('Ctrl Pts',(-14.0703340625699,-35.3458404532196,
19.7565039261967));
#29483=CARTESIAN_POINT('Ctrl Pts',(-14.0730062119097,-35.314390863165,19.7549587729448));
#29484=CARTESIAN_POINT('Ctrl Pts',(-14.0753127595707,-35.2829230824219,
19.7534136196929));
#29485=CARTESIAN_POINT('Ctrl Pts',(-14.0772539509858,-35.2514462550343,
19.751868466441));
#29486=CARTESIAN_POINT('Ctrl Pts',(-14.0823853229758,-35.1682399781399,
19.7477839871591));
#29487=CARTESIAN_POINT('Ctrl Pts',(-14.0849699104865,-35.0848750437508,
19.7436995078773));
#29488=CARTESIAN_POINT('Ctrl Pts',(-14.0849997388204,-35.0014607659441,
19.7396150285955));
#29489=CARTESIAN_POINT('Origin',(-10.,-35.,32.7603849714045));
#29490=CARTESIAN_POINT('',(-7.51282745730979,-31.7594448403263,21.7969517045595));
#29491=CARTESIAN_POINT('',(-7.5128274573098,-31.7594448403263,21.6925401901332));
#29492=CARTESIAN_POINT('',(-7.5128274573098,-31.7594448403263,32.7603849714045));
#29493=CARTESIAN_POINT('',(-14.084998525967,-35.0034702806205,20.8853849714301));
#29494=CARTESIAN_POINT('Ctrl Pts',(-7.5128274573098,-31.7594448403263,21.6925401901332));
#29495=CARTESIAN_POINT('Ctrl Pts',(-7.41823831723824,-31.8320433613915,
21.6867304612017));
#29496=CARTESIAN_POINT('Ctrl Pts',(-7.32673657161299,-31.9088588456523,
21.6809207322703));
#29497=CARTESIAN_POINT('Ctrl Pts',(-7.2387160725769,-31.9895953640491,21.6751110033388));
#29498=CARTESIAN_POINT('Ctrl Pts',(-7.14889638448983,-32.0719821827907,
21.6691825202445));
#29499=CARTESIAN_POINT('Ctrl Pts',(-7.06270218204445,-32.1584518535685,
21.6632540371501));
#29500=CARTESIAN_POINT('Ctrl Pts',(-6.98051726194745,-32.2486459706896,
21.6573255540558));
#29501=CARTESIAN_POINT('Ctrl Pts',(-6.90006210464625,-32.3369417538096,
21.6515218489557));
#29502=CARTESIAN_POINT('Ctrl Pts',(-6.82344940572467,-32.4288064278047,
21.6457181438557));
#29503=CARTESIAN_POINT('Ctrl Pts',(-6.75100196095492,-32.5238665742167,
21.6399144387556));
#29504=CARTESIAN_POINT('Ctrl Pts',(-6.67856311686816,-32.6189154354525,
21.6341114226492));
#29505=CARTESIAN_POINT('Ctrl Pts',(-6.61028879098722,-32.7171586899447,
21.6283084065428));
#29506=CARTESIAN_POINT('Ctrl Pts',(-6.54646067508267,-32.8181908581983,
21.6225053904363));
#29507=CARTESIAN_POINT('Ctrl Pts',(-6.48262507317079,-32.9192348758938,
21.6167016937298));
#29508=CARTESIAN_POINT('Ctrl Pts',(-6.42323693620976,-33.0230681125113,
21.6108979970233));
#29509=CARTESIAN_POINT('Ctrl Pts',(-6.36853356044624,-33.1292577680517,
21.6050943003168));
#29510=CARTESIAN_POINT('Ctrl Pts',(-6.31177027222353,-33.2394461054181,
21.5990720593799));
#29511=CARTESIAN_POINT('Ctrl Pts',(-6.26005172010707,-33.3521713939478,
21.593049818443));
#29512=CARTESIAN_POINT('Ctrl Pts',(-6.21358913516407,-33.4669253890784,
21.5870275775062));
#29513=CARTESIAN_POINT('Ctrl Pts',(-6.16874567483564,-33.5776804457435,
21.5812151991619));
#29514=CARTESIAN_POINT('Ctrl Pts',(-6.1287980621215,-33.6903247673409,21.5754028208176));
#29515=CARTESIAN_POINT('Ctrl Pts',(-6.09388554052908,-33.8043851667396,
21.5695904424734));
#29516=CARTESIAN_POINT('Ctrl Pts',(-6.05894890485997,-33.9185243476498,
21.5637740495197));
#29517=CARTESIAN_POINT('Ctrl Pts',(-6.02905438772444,-34.0340811599237,
21.557957656566));
#29518=CARTESIAN_POINT('Ctrl Pts',(-6.0042902724017,-34.1505715022579,21.5521412636124));
#29519=CARTESIAN_POINT('Ctrl Pts',(-5.97949171870993,-34.267223842602,21.5463167820561));
#29520=CARTESIAN_POINT('Ctrl Pts',(-5.95983786975095,-34.3848119025423,
21.5404923004999));
#29521=CARTESIAN_POINT('Ctrl Pts',(-5.9453652930546,-34.502845704802,21.5346678189437));
#29522=CARTESIAN_POINT('Ctrl Pts',(-5.94384095292056,-34.515277745463,21.5340543489872));
#29523=CARTESIAN_POINT('Ctrl Pts',(-5.94237404403647,-34.5277147308241,
21.5334408790307));
#29524=CARTESIAN_POINT('Ctrl Pts',(-5.94096457550326,-34.540156088786,21.5328274090742));
#29525=CARTESIAN_POINT('Ctrl Pts',(-5.92758466681395,-34.6582603455175,
21.5270038154231));
#29526=CARTESIAN_POINT('Ctrl Pts',(-5.91934211447388,-34.7771395042762,
21.521180221772));
#29527=CARTESIAN_POINT('Ctrl Pts',(-5.91631621890907,-34.8963092286898,
21.5153566281209));
#29528=CARTESIAN_POINT('Ctrl Pts',(-5.91329414096097,-35.0153286027953,
21.5095403817982));
#29529=CARTESIAN_POINT('Ctrl Pts',(-5.91547563943895,-35.134637408806,21.5037241354755));
#29530=CARTESIAN_POINT('Ctrl Pts',(-5.9228884422849,-35.2537446471277,21.4979078891528));
#29531=CARTESIAN_POINT('Ctrl Pts',(-5.93029382487437,-35.3727326584477,
21.4920974649247));
#29532=CARTESIAN_POINT('Ctrl Pts',(-5.94292006911669,-35.4915190982697,
21.4862870406966));
#29533=CARTESIAN_POINT('Ctrl Pts',(-5.96074286670504,-35.609612016881,21.4804766164685));
#29534=CARTESIAN_POINT('Ctrl Pts',(-5.9792402941338,-35.7321749973018,21.4744462556367));
#29535=CARTESIAN_POINT('Ctrl Pts',(-6.00333545989816,-35.8539904686384,
21.4684158948049));
#29536=CARTESIAN_POINT('Ctrl Pts',(-6.03294191300147,-35.9745127676842,
21.4623855339731));
#29537=CARTESIAN_POINT('Ctrl Pts',(-6.06143646425158,-36.0905087235307,
21.4565816497599));
#29538=CARTESIAN_POINT('Ctrl Pts',(-6.09503569746211,-36.2053064561403,
21.4507777655466));
#29539=CARTESIAN_POINT('Ctrl Pts',(-6.13361042261971,-36.3184296097726,
21.4449738813333));
#29540=CARTESIAN_POINT('Ctrl Pts',(-6.17217944987885,-36.4315360539081,
21.4391708544156));
#29541=CARTESIAN_POINT('Ctrl Pts',(-6.21572237578022,-36.5429680245935,
21.4333678274979));
#29542=CARTESIAN_POINT('Ctrl Pts',(-6.26406044065362,-36.6522652961649,
21.4275648005802));
#29543=CARTESIAN_POINT('Ctrl Pts',(-6.31240277327407,-36.7615722175455,
21.4217612613158));
#29544=CARTESIAN_POINT('Ctrl Pts',(-6.36554092144129,-36.8687436916215,
21.4159577220514));
#29545=CARTESIAN_POINT('Ctrl Pts',(-6.4232486413134,-36.9733410040167,21.4101541827869));
#29546=CARTESIAN_POINT('Ctrl Pts',(-6.48097507512801,-37.0779722361039,
21.4043487615022));
#29547=CARTESIAN_POINT('Ctrl Pts',(-6.54327383057665,-37.1800272889913,
21.3985433402175));
#29548=CARTESIAN_POINT('Ctrl Pts',(-6.60987386278575,-37.2790940686546,
21.3927379189327));
#29549=CARTESIAN_POINT('Ctrl Pts',(-6.67654764837054,-37.3782705556135,
21.3869260686809));
#29550=CARTESIAN_POINT('Ctrl Pts',(-6.74753199064943,-37.4744518247513,
21.381114218429));
#29551=CARTESIAN_POINT('Ctrl Pts',(-6.82251376542751,-37.5672565569304,
21.3753023681772));
#29552=CARTESIAN_POINT('Ctrl Pts',(-6.89754478864049,-37.6601222437593,
21.3694867006707));
#29553=CARTESIAN_POINT('Ctrl Pts',(-6.97657820348194,-37.7496066716158,
21.3636710331642));
#29554=CARTESIAN_POINT('Ctrl Pts',(-7.05926316405889,-37.8353645024474,
21.3578553656577));
#29555=CARTESIAN_POINT('Ctrl Pts',(-7.14206656191993,-37.9212451721183,
21.352031367835));
#29556=CARTESIAN_POINT('Ctrl Pts',(-7.22853165020971,-38.0033883102641,
21.3462073700123));
#29557=CARTESIAN_POINT('Ctrl Pts',(-7.31827350938968,-38.0814879570686,
21.3403833721896));
#29558=CARTESIAN_POINT('Ctrl Pts',(-7.34208251677673,-38.1022082216663,
21.3388382336283));
#29559=CARTESIAN_POINT('Ctrl Pts',(-7.36612200403376,-38.1226441107511,
21.337293095067));
#29560=CARTESIAN_POINT('Ctrl Pts',(-7.39038444532554,-38.1427904252115,
21.3357479565057));
#29561=CARTESIAN_POINT('Ctrl Pts',(-7.4818290593393,-38.2187214466398,21.3299243628435));
#29562=CARTESIAN_POINT('Ctrl Pts',(-7.57673789068995,-38.2907805045122,
21.3241007691813));
#29563=CARTESIAN_POINT('Ctrl Pts',(-7.67474932401576,-38.3586357786808,
21.3182771755191));
#29564=CARTESIAN_POINT('Ctrl Pts',(-7.77263710135612,-38.4264054433393,
21.3124609291855));
#29565=CARTESIAN_POINT('Ctrl Pts',(-7.87361936226491,-38.489981642841,21.306644682852));
#29566=CARTESIAN_POINT('Ctrl Pts',(-7.97730064829635,-38.5490720382401,
21.3008284365185));
#29567=CARTESIAN_POINT('Ctrl Pts',(-8.08087814878458,-38.6081032838252,
21.2950180122798));
#29568=CARTESIAN_POINT('Ctrl Pts',(-8.1871489468936,-38.662657457206,21.2892075880411));
#29569=CARTESIAN_POINT('Ctrl Pts',(-8.29568826514955,-38.7124852202333,
21.2833971638025));
#29570=CARTESIAN_POINT('Ctrl Pts',(-8.40833602135342,-38.7641990672694,
21.2773668029748));
#29571=CARTESIAN_POINT('Ctrl Pts',(-8.52342705879202,-38.8108213702415,
21.271336442147));
#29572=CARTESIAN_POINT('Ctrl Pts',(-8.64045761121957,-38.8521253215737,
21.2653060813193));
#29573=CARTESIAN_POINT('Ctrl Pts',(-8.75309295697439,-38.8918780591524,
21.2595021970962));
#29574=CARTESIAN_POINT('Ctrl Pts',(-8.86752434411707,-38.9267045656859,
21.2536983128731));
#29575=CARTESIAN_POINT('Ctrl Pts',(-8.98328254519098,-38.9564517711059,
21.24789442865));
#29576=CARTESIAN_POINT('Ctrl Pts',(-9.09902364753772,-38.9861945825447,
21.2420914017228));
#29577=CARTESIAN_POINT('Ctrl Pts',(-9.21609077868371,-39.0108594833107,
21.2362883747956));
#29578=CARTESIAN_POINT('Ctrl Pts',(-9.33400102962214,-39.0303437038863,
21.2304853478684));
#29579=CARTESIAN_POINT('Ctrl Pts',(-9.4519216908,-39.0498296447143,21.2246818085947));
#29580=CARTESIAN_POINT('Ctrl Pts',(-9.57068521687892,-39.0641339293542,
21.2188782693211));
#29581=CARTESIAN_POINT('Ctrl Pts',(-9.68980066117877,-39.0732052943836,
21.2130747300474));
#29582=CARTESIAN_POINT('Ctrl Pts',(-9.80895473322567,-39.0822796011508,
21.2072693087538));
#29583=CARTESIAN_POINT('Ctrl Pts',(-9.92846054350984,-39.0861175824163,
21.2014638874602));
#29584=CARTESIAN_POINT('Ctrl Pts',(-10.0478248515515,-39.0847200373556,
21.1956584661665));
#29585=CARTESIAN_POINT('Ctrl Pts',(-10.1673213445136,-39.0833209446431,
21.1898466159063));
#29586=CARTESIAN_POINT('Ctrl Pts',(-10.2866756138942,-39.0766747573613,
21.184034765646));
#29587=CARTESIAN_POINT('Ctrl Pts',(-10.4053970920895,-39.064834338288,21.1782229153857));
#29588=CARTESIAN_POINT('Ctrl Pts',(-10.5241965471874,-39.052986142364,21.1724072478711));
#29589=CARTESIAN_POINT('Ctrl Pts',(-10.642361980158,-39.0359369785404,21.1665915803565));
#29590=CARTESIAN_POINT('Ctrl Pts',(-10.7594122392775,-39.0137909824548,
21.1607759128418));
#29591=CARTESIAN_POINT('Ctrl Pts',(-10.8766301602534,-38.9916132646213,
21.1549519150115));
#29592=CARTESIAN_POINT('Ctrl Pts',(-10.9927293230292,-38.9643242359031,
21.1491279171812));
#29593=CARTESIAN_POINT('Ctrl Pts',(-11.1072428327699,-38.9320781158669,
21.1433039193508));
#29594=CARTESIAN_POINT('Ctrl Pts',(-11.137623893087,-38.9235230438931,21.1417587808797));
#29595=CARTESIAN_POINT('Ctrl Pts',(-11.1678934506138,-38.9146193209484,
21.1402136424085));
#29596=CARTESIAN_POINT('Ctrl Pts',(-11.198043031576,-38.90537039146,21.1386685039373));
#29597=CARTESIAN_POINT('Ctrl Pts',(-11.3116761558621,-38.870511374501,21.1328449101648));
#29598=CARTESIAN_POINT('Ctrl Pts',(-11.4239698392151,-38.8306325165478,
21.1270213163923));
#29599=CARTESIAN_POINT('Ctrl Pts',(-11.5344483324554,-38.7858543705516,
21.1211977226198));
#29600=CARTESIAN_POINT('Ctrl Pts',(-11.6447874406743,-38.7411327188346,
21.1153814761755));
#29601=CARTESIAN_POINT('Ctrl Pts',(-11.7533155387002,-38.6915242253266,
21.1095652297312));
#29602=CARTESIAN_POINT('Ctrl Pts',(-11.8595713467469,-38.6371993905143,
21.1037489832868));
#29603=CARTESIAN_POINT('Ctrl Pts',(-11.9657207921482,-38.582928935159,21.097938558937));
#29604=CARTESIAN_POINT('Ctrl Pts',(-12.06960211107,-38.5239517153247,21.0921281345872));
#29605=CARTESIAN_POINT('Ctrl Pts',(-12.1707739167292,-38.4604863245573,
21.0863177102374));
#29606=CARTESIAN_POINT('Ctrl Pts',(-12.2757752819967,-38.3946186390456,
21.0802873494512));
#29607=CARTESIAN_POINT('Ctrl Pts',(-12.3778575445062,-38.3239164647101,
21.074256988665));
#29608=CARTESIAN_POINT('Ctrl Pts',(-12.4765548626641,-38.2486768094433,
21.0682266278788));
#29609=CARTESIAN_POINT('Ctrl Pts',(-12.5715455007079,-38.1762628574395,
21.0624227435443));
#29610=CARTESIAN_POINT('Ctrl Pts',(-12.663400505583,-38.0996463676855,21.0566188592098));
#29611=CARTESIAN_POINT('Ctrl Pts',(-12.7517346404905,-38.0191358810634,
21.0508149748753));
#29612=CARTESIAN_POINT('Ctrl Pts',(-12.840055727498,-37.9386372867044,21.0450119478368));
#29613=CARTESIAN_POINT('Ctrl Pts',(-12.9248566770818,-37.8542461143283,
21.0392089207983));
#29614=CARTESIAN_POINT('Ctrl Pts',(-13.0057868226452,-37.7663099206005,
21.0334058937598));
#29615=CARTESIAN_POINT('Ctrl Pts',(-13.0867241134889,-37.6783659630319,
21.0276023543751));
#29616=CARTESIAN_POINT('Ctrl Pts',(-13.1637896442939,-37.5868766622893,
21.0217988149904));
#29617=CARTESIAN_POINT('Ctrl Pts',(-13.2366714207157,-37.4922245312817,
21.0159952756057));
#29618=CARTESIAN_POINT('Ctrl Pts',(-13.3095768318412,-37.3975417057001,
21.0101898542013));
#29619=CARTESIAN_POINT('Ctrl Pts',(-13.3782955413343,-37.2996943334015,
21.004384432797));
#29620=CARTESIAN_POINT('Ctrl Pts',(-13.4425578411275,-37.1990953845823,
20.9985790113926));
#29621=CARTESIAN_POINT('Ctrl Pts',(-13.5068913054552,-37.0983850317615,
20.9927671610227));
#29622=CARTESIAN_POINT('Ctrl Pts',(-13.5667582893279,-36.9949173644387,
20.9869553106528));
#29623=CARTESIAN_POINT('Ctrl Pts',(-13.621934094346,-36.889131656665,20.9811434602829));
#29624=CARTESIAN_POINT('Ctrl Pts',(-13.6771461391229,-36.7832764682823,
20.9753277926592));
#29625=CARTESIAN_POINT('Ctrl Pts',(-13.7276606964019,-36.6751005764842,
20.9695121250354));
#29626=CARTESIAN_POINT('Ctrl Pts',(-13.7733011123659,-36.5650634860663,
20.9636964574116));
#29627=CARTESIAN_POINT('Ctrl Pts',(-13.8190069032839,-36.4548687794312,
20.9578724594737));
#29628=CARTESIAN_POINT('Ctrl Pts',(-13.8598244785776,-36.3428079353696,
20.9520484615358));
#29629=CARTESIAN_POINT('Ctrl Pts',(-13.8956268882903,-36.2293559888128,
20.9462244635979));
#29630=CARTESIAN_POINT('Ctrl Pts',(-13.9051254566608,-36.1992565882477,
20.9446793261882));
#29631=CARTESIAN_POINT('Ctrl Pts',(-13.9142713021348,-36.1690593277715,
20.9431341887785));
#29632=CARTESIAN_POINT('Ctrl Pts',(-13.9230626605209,-36.1387731826954,
20.9415890513689));
#29633=CARTESIAN_POINT('Ctrl Pts',(-13.964019680971,-35.9976766412109,20.9343905933257));
#29634=CARTESIAN_POINT('Ctrl Pts',(-13.9973850464863,-35.8542851090668,
20.9271921352824));
#29635=CARTESIAN_POINT('Ctrl Pts',(-14.0229437096185,-35.7093299015557,
20.9199936772392));
#29636=CARTESIAN_POINT('Ctrl Pts',(-14.0481513699877,-35.5663653959087,
20.9128940772094));
#29637=CARTESIAN_POINT('Ctrl Pts',(-14.0657652703003,-35.4218798148452,
20.9057944771795));
#29638=CARTESIAN_POINT('Ctrl Pts',(-14.0756251114202,-35.2765952840546,
20.8986948771497));
#29639=CARTESIAN_POINT('Ctrl Pts',(-14.0817866583225,-35.1858050329981,
20.8942582419098));
#29640=CARTESIAN_POINT('Ctrl Pts',(-14.0849210219501,-35.0947031891774,
20.88982160667));
#29641=CARTESIAN_POINT('Ctrl Pts',(-14.084998525967,-35.0034702806205,20.8853849714301));
#29642=CARTESIAN_POINT('Ctrl Pts',(-14.0849985259674,-35.0034702800941,
20.8853849714045));
#29643=CARTESIAN_POINT('Ctrl Pts',(-14.0851010661903,-34.8827662884805,
20.8795151642127));
#29644=CARTESIAN_POINT('Ctrl Pts',(-14.0798491529874,-34.7619569640071,
20.8736453570208));
#29645=CARTESIAN_POINT('Ctrl Pts',(-14.0692436282641,-34.6415571261249,
20.867775549829));
#29646=CARTESIAN_POINT('Ctrl Pts',(-14.0588381189795,-34.5234279751741,
20.8620164445676));
#29647=CARTESIAN_POINT('Ctrl Pts',(-14.04327920392,-34.4056934318941,20.8562573393062));
#29648=CARTESIAN_POINT('Ctrl Pts',(-14.0226202175467,-34.2888378628019,
20.8504982340449));
#29649=CARTESIAN_POINT('Ctrl Pts',(-14.0019643520304,-34.1719999465367,
20.8447399987847));
#29650=CARTESIAN_POINT('Ctrl Pts',(-13.9762100191969,-34.05604114935,20.8389817635246));
#29651=CARTESIAN_POINT('Ctrl Pts',(-13.9454620141881,-33.9414375339175,
20.8332235282644));
#29652=CARTESIAN_POINT('Ctrl Pts',(-13.9147111095555,-33.82682311104,20.8274647499864));
#29653=CARTESIAN_POINT('Ctrl Pts',(-13.8789657046189,-33.7135645250196,
20.8217059717084));
#29654=CARTESIAN_POINT('Ctrl Pts',(-13.8383807969433,-33.6021238046032,
20.8159471934304));
#29655=CARTESIAN_POINT('Ctrl Pts',(-13.7964261779445,-33.4869220403567,
20.8099940605445));
#29656=CARTESIAN_POINT('Ctrl Pts',(-13.7492997768626,-33.3736634658438,
20.8040409276587));
#29657=CARTESIAN_POINT('Ctrl Pts',(-13.6972267955546,-33.2628359253561,
20.7980877947729));
#29658=CARTESIAN_POINT('Ctrl Pts',(-13.6467793219724,-33.1554679721394,
20.7923204946021));
#29659=CARTESIAN_POINT('Ctrl Pts',(-13.5916897458874,-33.05038188159,20.7865531944314));
#29660=CARTESIAN_POINT('Ctrl Pts',(-13.532208994307,-32.947994975509,20.7807858942606));
#29661=CARTESIAN_POINT('Ctrl Pts',(-13.4698533786046,-32.8406594358778,
20.7747398450172));
#29662=CARTESIAN_POINT('Ctrl Pts',(-13.4026717823479,-32.7362909683151,
20.7686937957739));
#29663=CARTESIAN_POINT('Ctrl Pts',(-13.3310026043436,-32.6353337127924,
20.7626477465305));
#29664=CARTESIAN_POINT('Ctrl Pts',(-13.2593334263393,-32.5343764572698,
20.7566016972871));
#29665=CARTESIAN_POINT('Ctrl Pts',(-13.1831770448846,-32.4368307748664,
20.7505556480437));
#29666=CARTESIAN_POINT('Ctrl Pts',(-13.1029170864551,-32.3430975639694,
20.7445095988004));
#29667=CARTESIAN_POINT('Ctrl Pts',(-13.0256101762356,-32.2528131299729,
20.7386860051282));
#29668=CARTESIAN_POINT('Ctrl Pts',(-12.9442348728726,-32.1657599620686,
20.732862411456));
#29669=CARTESIAN_POINT('Ctrl Pts',(-12.8590915555345,-32.0823261873418,
20.7270388177838));
#29670=CARTESIAN_POINT('Ctrl Pts',(-12.7740556591628,-31.998997676739,20.7212225714418));
#29671=CARTESIAN_POINT('Ctrl Pts',(-12.6852614933123,-31.9192797601209,
20.7154063250997));
#29672=CARTESIAN_POINT('Ctrl Pts',(-12.593049462095,-31.8435273663266,20.7095900787576));
#29673=CARTESIAN_POINT('Ctrl Pts',(-12.5009297356559,-31.767850801118,20.7037796545119));
#29674=CARTESIAN_POINT('Ctrl Pts',(-12.4053992638164,-31.6961321195937,
20.6979692302662));
#29675=CARTESIAN_POINT('Ctrl Pts',(-12.3068346109939,-31.6286888192395,
20.6921588060204));
#29676=CARTESIAN_POINT('Ctrl Pts',(-12.2045390821434,-31.5586926504347,
20.6861284451959));
#29677=CARTESIAN_POINT('Ctrl Pts',(-12.0989754538823,-31.4933022356453,
20.6800980843714));
#29678=CARTESIAN_POINT('Ctrl Pts',(-11.9906019499155,-31.432826205945,20.6740677235469));
#29679=CARTESIAN_POINT('Ctrl Pts',(-11.8862985278559,-31.3746214176948,
20.6682638393203));
#29680=CARTESIAN_POINT('Ctrl Pts',(-11.7793928683359,-31.3209687582943,
20.6624599550937));
#29681=CARTESIAN_POINT('Ctrl Pts',(-11.6703216060448,-31.2720983472763,
20.6566560708672));
#29682=CARTESIAN_POINT('Ctrl Pts',(-11.5612664547734,-31.2232351549531,
20.6508530439378));
#29683=CARTESIAN_POINT('Ctrl Pts',(-11.4500467094183,-31.1791529731452,
20.6450500170085));
#29684=CARTESIAN_POINT('Ctrl Pts',(-11.3371209849973,-31.140034654109,20.6392469900792));
#29685=CARTESIAN_POINT('Ctrl Pts',(-11.2241852904441,-31.1009128813441,
20.6334434508047));
#29686=CARTESIAN_POINT('Ctrl Pts',(-11.1095437032182,-31.0667559763748,
20.6276399115302));
#29687=CARTESIAN_POINT('Ctrl Pts',(-10.9936714594704,-31.0376973827541,
20.6218363722558));
#29688=CARTESIAN_POINT('Ctrl Pts',(-10.877761639734,-31.0086293657775,20.6160309509626));
#29689=CARTESIAN_POINT('Ctrl Pts',(-10.7606207656496,-30.9846630475094,
20.6102255296695));
#29690=CARTESIAN_POINT('Ctrl Pts',(-10.6427351271284,-30.9658809442017,
20.6044201083764));
#29691=CARTESIAN_POINT('Ctrl Pts',(-10.5247189412156,-30.9470780414597,
20.5986082581185));
#29692=CARTESIAN_POINT('Ctrl Pts',(-10.4059567480696,-30.9334708775643,
20.5927964078607));
#29693=CARTESIAN_POINT('Ctrl Pts',(-10.2869409962033,-30.9250902016489,
20.5869845576029));
#29694=CARTESIAN_POINT('Ctrl Pts',(-10.1678470741772,-30.9167040212623,
20.5811688900919));
#29695=CARTESIAN_POINT('Ctrl Pts',(-10.0484996690212,-30.9135511760909,
20.5753532225808));
#29696=CARTESIAN_POINT('Ctrl Pts',(-9.92939060816214,-30.9156102886987,
20.5695375550698));
#29697=CARTESIAN_POINT('Ctrl Pts',(-9.81011093646856,-30.9176723507623,
20.5637135572446));
#29698=CARTESIAN_POINT('Ctrl Pts',(-9.69107069661965,-30.9249612466002,
20.5578895594195));
#29699=CARTESIAN_POINT('Ctrl Pts',(-9.57275612268976,-30.9374038264552,
20.5520655615944));
#29700=CARTESIAN_POINT('Ctrl Pts',(-9.54136661957653,-30.9407049108958,
20.5505204231402));
#29701=CARTESIAN_POINT('Ctrl Pts',(-9.51002813342651,-30.9443684696613,
20.5489752846861));
#29702=CARTESIAN_POINT('Ctrl Pts',(-9.47874959801868,-30.9483925389502,
20.547430146232));
#29703=CARTESIAN_POINT('Ctrl Pts',(-9.3608661673276,-30.96355856533,20.5416067846362));
#29704=CARTESIAN_POINT('Ctrl Pts',(-9.24345509214536,-30.9838981280243,
20.5357834230404));
#29705=CARTESIAN_POINT('Ctrl Pts',(-9.12700558914339,-31.0093727612551,
20.5299600614446));
#29706=CARTESIAN_POINT('Ctrl Pts',(-9.01069687702149,-31.0348165949037,
20.5241437404646));
#29707=CARTESIAN_POINT('Ctrl Pts',(-8.89534782060662,-31.0653830669002,
20.5183274194846));
#29708=CARTESIAN_POINT('Ctrl Pts',(-8.78144188802837,-31.1009820303379,
20.5125110985045));
#29709=CARTESIAN_POINT('Ctrl Pts',(-8.66746504168588,-31.1366031564184,
20.5066911564909));
#29710=CARTESIAN_POINT('Ctrl Pts',(-8.55493352306209,-31.1772629828042,
20.5008712144772));
#29711=CARTESIAN_POINT('Ctrl Pts',(-8.44432160893254,-31.2228198687955,
20.4950512724635));
#29712=CARTESIAN_POINT('Ctrl Pts',(-8.33397539404962,-31.2682673232633,
20.4892453104466));
#29713=CARTESIAN_POINT('Ctrl Pts',(-8.22553995871077,-31.3185882042552,
20.4834393484298));
#29714=CARTESIAN_POINT('Ctrl Pts',(-8.11947019380578,-31.3735923218679,
20.4776333864129));
#29715=CARTESIAN_POINT('Ctrl Pts',(-8.01301732572882,-31.4287951035576,
20.4718064544008));
#29716=CARTESIAN_POINT('Ctrl Pts',(-7.90894763984181,-31.4887148755145,
20.4659795223887));
#29717=CARTESIAN_POINT('Ctrl Pts',(-7.80769898378764,-31.5531113661282,
20.4601525903766));
#29718=CARTESIAN_POINT('Ctrl Pts',(-7.70645032773347,-31.617507856742,20.4543256583645));
#29719=CARTESIAN_POINT('Ctrl Pts',(-7.60802305871064,-31.6863808514964,
20.4484987263525));
#29720=CARTESIAN_POINT('Ctrl Pts',(-7.51282745730978,-31.7594448403263,
20.4426717943404));
#29721=CARTESIAN_POINT('',(-14.0849985032409,-34.9965030699667,20.9896150285484));
#29722=CARTESIAN_POINT('Ctrl Pts',(-14.0849985032409,-34.9965030699667,
20.9896150285484));
#29723=CARTESIAN_POINT('Ctrl Pts',(-14.0848731076929,-34.8500201203563,
20.9824905060981));
#29724=CARTESIAN_POINT('Ctrl Pts',(-14.0768649533835,-34.7038771885051,
20.9753659836478));
#29725=CARTESIAN_POINT('Ctrl Pts',(-14.0611057921053,-34.5588143867611,
20.9682414611975));
#29726=CARTESIAN_POINT('Ctrl Pts',(-14.0451084213714,-34.4115588711768,
20.9610092471901));
#29727=CARTESIAN_POINT('Ctrl Pts',(-14.0211239958772,-34.2654163151662,
20.9537770331828));
#29728=CARTESIAN_POINT('Ctrl Pts',(-13.9893392113733,-34.1211384314923,
20.9465448191755));
#29729=CARTESIAN_POINT('Ctrl Pts',(-13.9714671903031,-34.0400135342429,
20.9424782734009));
#29730=CARTESIAN_POINT('Ctrl Pts',(-13.9511298671933,-33.9594777773168,
20.9384117276262));
#29731=CARTESIAN_POINT('Ctrl Pts',(-13.928367028479,-33.8796618860545,20.9343451818516));
#29732=CARTESIAN_POINT('Ctrl Pts',(-13.8957689635323,-33.7653596393175,
20.9285215881894));
#29733=CARTESIAN_POINT('Ctrl Pts',(-13.8581254755735,-33.6522969933898,
20.9226979945272));
#29734=CARTESIAN_POINT('Ctrl Pts',(-13.8155476565818,-33.5409519951856,
20.9168744008649));
#29735=CARTESIAN_POINT('Ctrl Pts',(-13.773023555835,-33.4297474752401,20.9110581545314));
#29736=CARTESIAN_POINT('Ctrl Pts',(-13.7255776507743,-33.3202566708117,
20.9052419081978));
#29737=CARTESIAN_POINT('Ctrl Pts',(-13.6733712581103,-33.2129441530581,
20.8994256618642));
#29738=CARTESIAN_POINT('Ctrl Pts',(-13.6212171243352,-33.1057390557306,
20.8936152376256));
#29739=CARTESIAN_POINT('Ctrl Pts',(-13.5643121604877,-33.0007082723686,
20.8878048133869));
#29740=CARTESIAN_POINT('Ctrl Pts',(-13.502866161484,-32.8982974390436,20.8819943891482));
#29741=CARTESIAN_POINT('Ctrl Pts',(-13.4390943041823,-32.7920101436161,
20.8759640283205));
#29742=CARTESIAN_POINT('Ctrl Pts',(-13.3704310041942,-32.6885454768558,
20.8699336674928));
#29743=CARTESIAN_POINT('Ctrl Pts',(-13.2971639702753,-32.5883750803414,
20.8639033066651));
#29744=CARTESIAN_POINT('Ctrl Pts',(-13.2266485576182,-32.49196668944,20.8580994224419));
#29745=CARTESIAN_POINT('Ctrl Pts',(-13.1518692340175,-32.3986099506225,
20.8522955382188));
#29746=CARTESIAN_POINT('Ctrl Pts',(-13.0731268378526,-32.3086961452727,
20.8464916539957));
#29747=CARTESIAN_POINT('Ctrl Pts',(-12.9943960727838,-32.2187956211559,
20.8406886270685));
#29748=CARTESIAN_POINT('Ctrl Pts',(-12.9117036682537,-32.1323373262523,
20.8348856001413));
#29749=CARTESIAN_POINT('Ctrl Pts',(-12.8253901565031,-32.0496787524855,
20.8290825732141));
#29750=CARTESIAN_POINT('Ctrl Pts',(-12.7390690241739,-31.9670128808329,
20.8232790339404));
#29751=CARTESIAN_POINT('Ctrl Pts',(-12.6491264439008,-31.8881476797638,
20.8174754946667));
#29752=CARTESIAN_POINT('Ctrl Pts',(-12.5559386644153,-31.8134026699712,
20.811671955393));
#29753=CARTESIAN_POINT('Ctrl Pts',(-12.4627206652216,-31.7386334212452,
20.8058665340994));
#29754=CARTESIAN_POINT('Ctrl Pts',(-12.3662556922375,-31.6679872764169,
20.8000611128057));
#29755=CARTESIAN_POINT('Ctrl Pts',(-12.2669512843041,-31.601742082391,20.7942556915121));
#29756=CARTESIAN_POINT('Ctrl Pts',(-12.1675369059325,-31.5354235279458,
20.7884438412518));
#29757=CARTESIAN_POINT('Ctrl Pts',(-12.0652771559888,-31.473515879256,20.7826319909915));
#29758=CARTESIAN_POINT('Ctrl Pts',(-11.9606067648305,-31.4162525041933,
20.7768201407312));
#29759=CARTESIAN_POINT('Ctrl Pts',(-11.8558676255988,-31.3589515182392,
20.7710044732166));
#29760=CARTESIAN_POINT('Ctrl Pts',(-11.7487150575697,-31.3063010604908,
20.7651888057019));
#29761=CARTESIAN_POINT('Ctrl Pts',(-11.6396049709043,-31.2584868649989,
20.7593731381873));
#29762=CARTESIAN_POINT('Ctrl Pts',(-11.5303385958221,-31.2106041808352,
20.7535491403569));
#29763=CARTESIAN_POINT('Ctrl Pts',(-11.4191094850817,-31.1675717325015,
20.7477251425266));
#29764=CARTESIAN_POINT('Ctrl Pts',(-11.3063900618776,-31.1295258680328,
20.7419011446962));
#29765=CARTESIAN_POINT('Ctrl Pts',(-11.2764849825327,-31.119432092148,20.7403560062252));
#29766=CARTESIAN_POINT('Ctrl Pts',(-11.2464750655715,-31.1096890290316,
20.7388108677542));
#29767=CARTESIAN_POINT('Ctrl Pts',(-11.2163692495621,-31.1002986205711,
20.7372657292832));
#29768=CARTESIAN_POINT('Ctrl Pts',(-11.1028985208735,-31.0649055759061,
20.731442004453));
#29769=CARTESIAN_POINT('Ctrl Pts',(-10.9876987634977,-31.0344121023845,
20.7256182796227));
#29770=CARTESIAN_POINT('Ctrl Pts',(-10.8712307300107,-31.0089873446599,
20.7197945547924));
#29771=CARTESIAN_POINT('Ctrl Pts',(-10.7549102796124,-30.9835948040524,
20.7139782095261));
#29772=CARTESIAN_POINT('Ctrl Pts',(-10.6373251451302,-30.9632582903934,
20.7081618642598));
#29773=CARTESIAN_POINT('Ctrl Pts',(-10.5189523332168,-30.9480975485769,
20.7023455189935));
#29774=CARTESIAN_POINT('Ctrl Pts',(-10.4006986643929,-30.9329520661564,
20.6965350279206));
#29775=CARTESIAN_POINT('Ctrl Pts',(-10.2816592980966,-30.9229720433083,
20.6907245368478));
#29776=CARTESIAN_POINT('Ctrl Pts',(-10.1623219706432,-30.9182262951204,
20.6849140457749));
#29777=CARTESIAN_POINT('Ctrl Pts',(-10.0430738621628,-30.9134840949487,
20.6791078987414));
#29778=CARTESIAN_POINT('Ctrl Pts',(-9.92352864244225,-30.9139683984217,
20.6733017517079));
#29779=CARTESIAN_POINT('Ctrl Pts',(-9.80417911364261,-30.9196961901758,
20.6674956046744));
#29780=CARTESIAN_POINT('Ctrl Pts',(-9.68487740632811,-30.9254216868934,
20.661691784073));
#29781=CARTESIAN_POINT('Ctrl Pts',(-9.56577164121818,-30.9363864744827,
20.6558879634716));
#29782=CARTESIAN_POINT('Ctrl Pts',(-9.44735408758601,-30.9525554363905,
20.6500841428702));
#29783=CARTESIAN_POINT('Ctrl Pts',(-9.32895603536141,-30.9687217355384,
20.6442812780619));
#29784=CARTESIAN_POINT('Ctrl Pts',(-9.21124637356511,-30.9900904489027,
20.6384784132535));
#29785=CARTESIAN_POINT('Ctrl Pts',(-9.0947110799995,-31.0165747187472,20.6326755484451));
#29786=CARTESIAN_POINT('Ctrl Pts',(-8.97816747584504,-31.0430608772888,
20.6268722698117));
#29787=CARTESIAN_POINT('Ctrl Pts',(-8.86279880443876,-31.0746632265921,
20.6210689911782));
#29788=CARTESIAN_POINT('Ctrl Pts',(-8.74907907121573,-31.1112441796984,
20.6152657125448));
#29789=CARTESIAN_POINT('Ctrl Pts',(-8.63525960069849,-31.1478572159374,
20.6094573441763));
#29790=CARTESIAN_POINT('Ctrl Pts',(-8.52309234690806,-31.1894574539382,
20.6036489758079));
#29791=CARTESIAN_POINT('Ctrl Pts',(-8.41303458871639,-31.235857895431,20.5978406074394));
#29792=CARTESIAN_POINT('Ctrl Pts',(-8.30292908366268,-31.2822784670401,
20.5920297191999));
#29793=CARTESIAN_POINT('Ctrl Pts',(-8.19493526746047,-31.3335032179248,
20.5862188309604));
#29794=CARTESIAN_POINT('Ctrl Pts',(-8.08948741778155,-31.3892983129058,
20.5804079427208));
#29795=CARTESIAN_POINT('Ctrl Pts',(-7.98388384719028,-31.4451758037168,
20.574588473208));
#29796=CARTESIAN_POINT('Ctrl Pts',(-7.8808341093746,-31.5056369195399,20.5687690036951));
#29797=CARTESIAN_POINT('Ctrl Pts',(-7.78074545052058,-31.5704031950366,
20.5629495341823));
#29798=CARTESIAN_POINT('Ctrl Pts',(-7.6888465203333,-31.6298699867642,20.5576062412596));
#29799=CARTESIAN_POINT('Ctrl Pts',(-7.59944376850164,-31.6929655797273,
20.552262948337));
#29800=CARTESIAN_POINT('Ctrl Pts',(-7.51282745730979,-31.7594448403263,
20.5469196554144));
#29801=CARTESIAN_POINT('Ctrl Pts',(-7.51282745730979,-31.7594448403263,
21.7969517045595));
#29802=CARTESIAN_POINT('Ctrl Pts',(-7.41803123744738,-31.8322022980998,
21.7911462658977));
#29803=CARTESIAN_POINT('Ctrl Pts',(-7.32646761151655,-31.9090941156954,
21.7853408272359));
#29804=CARTESIAN_POINT('Ctrl Pts',(-7.23850334801992,-31.989790498802,21.7795353885741));
#29805=CARTESIAN_POINT('Ctrl Pts',(-7.15044160797137,-32.0705763046453,
21.7737235166845));
#29806=CARTESIAN_POINT('Ctrl Pts',(-7.06598749294522,-32.1551748152077,
21.7679116447949));
#29807=CARTESIAN_POINT('Ctrl Pts',(-6.98547103052354,-32.2432192520646,
21.7620997729053));
#29808=CARTESIAN_POINT('Ctrl Pts',(-6.90490156944531,-32.3313216427452,
21.7562840754452));
#29809=CARTESIAN_POINT('Ctrl Pts',(-6.82827518425165,-32.4228741645268,
21.7504683779852));
#29810=CARTESIAN_POINT('Ctrl Pts',(-6.75588066911818,-32.5174781437017,
21.7446526805251));
#29811=CARTESIAN_POINT('Ctrl Pts',(-6.68338258582743,-32.612217464066,21.738828663083));
#29812=CARTESIAN_POINT('Ctrl Pts',(-6.61512868904173,-32.7100166212431,
21.7330046456408));
#29813=CARTESIAN_POINT('Ctrl Pts',(-6.55136372612828,-32.810449166944,21.7271806281987));
#29814=CARTESIAN_POINT('Ctrl Pts',(-6.53487643022944,-32.8364173636337,
21.7256747495076));
#29815=CARTESIAN_POINT('Ctrl Pts',(-6.51868899898723,-32.8625614964342,
21.7241688708165));
#29816=CARTESIAN_POINT('Ctrl Pts',(-6.50280514828376,-32.8888739570719,
21.7226629921254));
#29817=CARTESIAN_POINT('Ctrl Pts',(-6.44137849223948,-32.990630546166,21.7168393984561));
#29818=CARTESIAN_POINT('Ctrl Pts',(-6.38429762830078,-33.0952344137322,
21.7110158047867));
#29819=CARTESIAN_POINT('Ctrl Pts',(-6.33183666579974,-33.2022784549245,
21.7051922111174));
#29820=CARTESIAN_POINT('Ctrl Pts',(-6.27944189059527,-33.3091874441587,
21.6993759647765));
#29821=CARTESIAN_POINT('Ctrl Pts',(-6.23165560181353,-33.4185301202355,
21.6935597184356));
#29822=CARTESIAN_POINT('Ctrl Pts',(-6.1887078171446,-33.5298718093631,21.6877434720947));
#29823=CARTESIAN_POINT('Ctrl Pts',(-6.14580302344499,-33.6411020448458,
21.6819330478485));
#29824=CARTESIAN_POINT('Ctrl Pts',(-6.10772724468424,-33.7543269338045,
21.6761226236022));
#29825=CARTESIAN_POINT('Ctrl Pts',(-6.07466360223702,-33.8690892323454,
21.670312199356));
#29826=CARTESIAN_POINT('Ctrl Pts',(-6.04034843251884,-33.9881955213142,
21.664281838531));
#29827=CARTESIAN_POINT('Ctrl Pts',(-6.011432532949,-34.108957505296,21.6582514777061));
#29828=CARTESIAN_POINT('Ctrl Pts',(-5.98806495335417,-34.2308432009695,
21.6522211168811));
#29829=CARTESIAN_POINT('Ctrl Pts',(-5.96557496798386,-34.3481513501263,
21.64641723265));
#29830=CARTESIAN_POINT('Ctrl Pts',(-5.94822415578494,-34.4664998916385,
21.6406133484188));
#29831=CARTESIAN_POINT('Ctrl Pts',(-5.93609381245938,-34.5854020032983,
21.6348094641876));
#29832=CARTESIAN_POINT('Ctrl Pts',(-5.92396526091524,-34.7042865518447,
21.6290064372522));
#29833=CARTESIAN_POINT('Ctrl Pts',(-5.91705568616423,-34.8237241018089,
21.6232034103168));
#29834=CARTESIAN_POINT('Ctrl Pts',(-5.91539460443504,-34.9432218129771,
21.6174003833814));
#29835=CARTESIAN_POINT('Ctrl Pts',(-5.91373337604969,-35.0627300745444,
21.6115968440994));
#29836=CARTESIAN_POINT('Ctrl Pts',(-5.91732156768746,-35.1822980995589,
21.6057933048173));
#29837=CARTESIAN_POINT('Ctrl Pts',(-5.92613656673855,-35.3014327904114,
21.5999897655353));
#29838=CARTESIAN_POINT('Ctrl Pts',(-5.93495442439102,-35.4206061152548,
21.5941843442331));
#29839=CARTESIAN_POINT('Ctrl Pts',(-5.94900243029894,-35.5393454194489,
21.588378922931));
#29840=CARTESIAN_POINT('Ctrl Pts',(-5.96820615034603,-35.6571631105687,
21.5825735016289));
#29841=CARTESIAN_POINT('Ctrl Pts',(-5.98743113673578,-35.7751112738776,
21.5767616513599));
#29842=CARTESIAN_POINT('Ctrl Pts',(-6.01182316813919,-35.8921353836473,
21.5709498010909));
#29843=CARTESIAN_POINT('Ctrl Pts',(-6.0412567294959,-36.0077582637907,21.565137950822));
#29844=CARTESIAN_POINT('Ctrl Pts',(-6.07070962297388,-36.1234570856632,
21.5593222832985));
#29845=CARTESIAN_POINT('Ctrl Pts',(-6.10521052322106,-36.2377524550219,
21.5535066157751));
#29846=CARTESIAN_POINT('Ctrl Pts',(-6.14458462288469,-36.3501841614768,
21.5476909482517));
#29847=CARTESIAN_POINT('Ctrl Pts',(-6.18401512169475,-36.4627769142116,
21.5418669504124));
#29848=CARTESIAN_POINT('Ctrl Pts',(-6.22833260108735,-36.5735002981215,
21.5360429525732));
#29849=CARTESIAN_POINT('Ctrl Pts',(-6.27731485981466,-36.6819156777447,
21.530218954734));
#29850=CARTESIAN_POINT('Ctrl Pts',(-6.29031012021684,-36.710678869284,21.5286738163416));
#29851=CARTESIAN_POINT('Ctrl Pts',(-6.30363347546049,-36.7392797521074,
21.5271286779493));
#29852=CARTESIAN_POINT('Ctrl Pts',(-6.3172802545401,-36.7677104616989,21.525583539557));
#29853=CARTESIAN_POINT('Ctrl Pts',(-6.36871467403733,-36.8748652002055,
21.5197599458878));
#29854=CARTESIAN_POINT('Ctrl Pts',(-6.42491268003565,-36.979946017943,21.5139363522187));
#29855=CARTESIAN_POINT('Ctrl Pts',(-6.48568403854074,-37.0825004977269,
21.5081127585495));
#29856=CARTESIAN_POINT('Ctrl Pts',(-6.54637872494984,-37.1849255898006,
21.5022965122088));
#29857=CARTESIAN_POINT('Ctrl Pts',(-6.61163508121168,-37.2848303352914,
21.4964802658682));
#29858=CARTESIAN_POINT('Ctrl Pts',(-6.68121564602919,-37.3817840816998,
21.4906640195275));
#29859=CARTESIAN_POINT('Ctrl Pts',(-6.75072656031707,-37.4786407768727,
21.4848535952815));
#29860=CARTESIAN_POINT('Ctrl Pts',(-6.82455283531835,-37.5725520196744,
21.4790431710355));
#29861=CARTESIAN_POINT('Ctrl Pts',(-6.90241242590179,-37.6631140082228,
21.4732327467896));
#29862=CARTESIAN_POINT('Ctrl Pts',(-6.98321916307485,-37.7571039554041,
21.4672023859645));
#29863=CARTESIAN_POINT('Ctrl Pts',(-7.06837035901945,-37.8474857005277,
21.4611720251395));
#29864=CARTESIAN_POINT('Ctrl Pts',(-7.15750278192183,-37.9338429687388,
21.4551416643144));
#29865=CARTESIAN_POINT('Ctrl Pts',(-7.24328774218333,-38.0169569981856,
21.4493377800836));
#29866=CARTESIAN_POINT('Ctrl Pts',(-7.33275996413809,-38.096343076676,21.4435338958528));
#29867=CARTESIAN_POINT('Ctrl Pts',(-7.42555684708142,-38.1716663526277,
21.4377300116219));
#29868=CARTESIAN_POINT('Ctrl Pts',(-7.51834002293257,-38.2469785025258,
21.4319269846869));
#29869=CARTESIAN_POINT('Ctrl Pts',(-7.61444656619898,-38.3182287860612,
21.4261239577518));
#29870=CARTESIAN_POINT('Ctrl Pts',(-7.71348045926837,-38.3851223596574,
21.4203209308168));
#29871=CARTESIAN_POINT('Ctrl Pts',(-7.81252309599461,-38.4520218392564,
21.4145173915352));
#29872=CARTESIAN_POINT('Ctrl Pts',(-7.91449325799974,-38.5145636155634,
21.4087138522535));
#29873=CARTESIAN_POINT('Ctrl Pts',(-8.01896613726248,-38.5724963029634,
21.4029103129719));
#29874=CARTESIAN_POINT('Ctrl Pts',(-8.12347289586164,-38.6304477772583,
21.3971048916702));
#29875=CARTESIAN_POINT('Ctrl Pts',(-8.23048362888832,-38.683786992155,21.3912994703684));
#29876=CARTESIAN_POINT('Ctrl Pts',(-8.33954972603607,-38.7323089217927,
21.3854940490667));
#29877=CARTESIAN_POINT('Ctrl Pts',(-8.4487366037914,-38.7808845849763,21.3796821987982));
#29878=CARTESIAN_POINT('Ctrl Pts',(-8.5599830157061,-38.8246321483105,21.3738703485297));
#29879=CARTESIAN_POINT('Ctrl Pts',(-8.67282106268532,-38.8633950184195,
21.3680584982612));
#29880=CARTESIAN_POINT('Ctrl Pts',(-8.7857332222997,-38.9021833481896,21.3622428307383));
#29881=CARTESIAN_POINT('Ctrl Pts',(-8.90023870817414,-38.9359803492066,
21.3564271632153));
#29882=CARTESIAN_POINT('Ctrl Pts',(-9.0158567905939,-38.9646799547227,21.3506114956924));
#29883=CARTESIAN_POINT('Ctrl Pts',(-9.13164048343237,-38.9934206693247,
21.3447874978537));
#29884=CARTESIAN_POINT('Ctrl Pts',(-9.24853955488159,-39.017049334478,21.338963500015));
#29885=CARTESIAN_POINT('Ctrl Pts',(-9.36606534026731,-39.035511348911,21.3331395021762));
#29886=CARTESIAN_POINT('Ctrl Pts',(-9.39724557222105,-39.0404094220485,
21.3315943637803));
#29887=CARTESIAN_POINT('Ctrl Pts',(-9.42846990349015,-39.0449441143995,
21.3300492253844));
#29888=CARTESIAN_POINT('Ctrl Pts',(-9.45972919594527,-39.0491150216172,
21.3285040869885));
#29889=CARTESIAN_POINT('Ctrl Pts',(-9.57754480302673,-39.0648350820324,
21.3226804933035));
#29890=CARTESIAN_POINT('Ctrl Pts',(-9.69623706723093,-39.0754341682929,
21.3168568996185));
#29891=CARTESIAN_POINT('Ctrl Pts',(-9.81532332052963,-39.0808233880015,
21.3110333059335));
#29892=CARTESIAN_POINT('Ctrl Pts',(-9.93425932883225,-39.0862058084089,
21.3052170595769));
#29893=CARTESIAN_POINT('Ctrl Pts',(-10.0535879332335,-39.0863914175503,
21.2994008132203));
#29894=CARTESIAN_POINT('Ctrl Pts',(-10.172818780773,-39.0813427531895,21.2935845668637));
#29895=CARTESIAN_POINT('Ctrl Pts',(-10.2919302775763,-39.0762991425695,
21.2877741426018));
#29896=CARTESIAN_POINT('Ctrl Pts',(-10.4109438065621,-39.0660316990324,
21.2819637183399));
#29897=CARTESIAN_POINT('Ctrl Pts',(-10.5293670326174,-39.0505549675048,
21.276153294078));
#29898=CARTESIAN_POINT('Ctrl Pts',(-10.6522728223295,-39.0344924097286,
21.2701229332589));
#29899=CARTESIAN_POINT('Ctrl Pts',(-10.7745422900069,-39.0128183870614,
21.2640925724398));
#29900=CARTESIAN_POINT('Ctrl Pts',(-10.8956281649261,-38.9856085093987,
21.2580622116207));
#29901=CARTESIAN_POINT('Ctrl Pts',(-11.0121665318719,-38.9594205274418,
21.252258327374));
#29902=CARTESIAN_POINT('Ctrl Pts',(-11.127608170754,-38.9281050992437,21.2464544431272));
#29903=CARTESIAN_POINT('Ctrl Pts',(-11.2414742568698,-38.891781940131,21.2406505588804));
#29904=CARTESIAN_POINT('Ctrl Pts',(-11.3553235237461,-38.8554641463376,
21.2348475319295));
#29905=CARTESIAN_POINT('Ctrl Pts',(-11.4675973117569,-38.8141402167147,
21.2290445049786));
#29906=CARTESIAN_POINT('Ctrl Pts',(-11.5778319398096,-38.7679797464578,
21.2232414780276));
#29907=CARTESIAN_POINT('Ctrl Pts',(-11.6880763004256,-38.7218152007149,
21.2174379387301));
#29908=CARTESIAN_POINT('Ctrl Pts',(-11.7962807664614,-38.6708134230554,
21.2116343994327));
#29909=CARTESIAN_POINT('Ctrl Pts',(-11.902002221956,-38.6151919102137,21.2058308601352));
#29910=CARTESIAN_POINT('Ctrl Pts',(-12.0077579616846,-38.5595523599646,
21.2000254388177));
#29911=CARTESIAN_POINT('Ctrl Pts',(-12.1110287282994,-38.499290285125,21.1942200175002));
#29912=CARTESIAN_POINT('Ctrl Pts',(-12.2113971322542,-38.4346685027027,
21.1884145961827));
#29913=CARTESIAN_POINT('Ctrl Pts',(-12.3118766849232,-38.3699751576396,
21.1826027458986));
#29914=CARTESIAN_POINT('Ctrl Pts',(-12.4094471157842,-38.3009126891299,
21.1767908956145));
#29915=CARTESIAN_POINT('Ctrl Pts',(-12.5037209694124,-38.2277865956913,
21.1709790453304));
#29916=CARTESIAN_POINT('Ctrl Pts',(-12.598056742612,-38.1546124726434,21.1651633777919));
#29917=CARTESIAN_POINT('Ctrl Pts',(-12.6890913158667,-38.077369672845,21.1593477102534));
#29918=CARTESIAN_POINT('Ctrl Pts',(-12.7764724594871,-37.9964021228316,
21.153532042715));
#29919=CARTESIAN_POINT('Ctrl Pts',(-12.8639787671569,-37.9153185955488,
21.147708044861));
#29920=CARTESIAN_POINT('Ctrl Pts',(-12.9478209140806,-37.8304999584517,
21.1418840470069));
#29921=CARTESIAN_POINT('Ctrl Pts',(-13.0276853651523,-37.7423249861463,
21.1360600491529));
#29922=CARTESIAN_POINT('Ctrl Pts',(-13.0488738375391,-37.7189316873654,
21.1345149109086));
#29923=CARTESIAN_POINT('Ctrl Pts',(-13.0697825624144,-37.6953023131244,
21.1329697726644));
#29924=CARTESIAN_POINT('Ctrl Pts',(-13.0904061924061,-37.6714442846405,
21.1314246344201));
#29925=CARTESIAN_POINT('Ctrl Pts',(-13.1692726209871,-37.5802092547126,
21.125515900844));
#29926=CARTESIAN_POINT('Ctrl Pts',(-13.2442376687118,-37.4853140263686,
21.119607167268));
#29927=CARTESIAN_POINT('Ctrl Pts',(-13.314940660894,-37.3871307912956,21.113698433692));
#29928=CARTESIAN_POINT('Ctrl Pts',(-13.3839459164573,-37.2913051547967,
21.1079315819947));
#29929=CARTESIAN_POINT('Ctrl Pts',(-13.4488911827427,-37.1923479648596,
21.1021647302974));
#29930=CARTESIAN_POINT('Ctrl Pts',(-13.5094788137209,-37.0906418765642,
21.0963978786002));
#29931=CARTESIAN_POINT('Ctrl Pts',(-13.5700104610653,-36.9890297658072,
21.090636355537));
#29932=CARTESIAN_POINT('Ctrl Pts',(-13.6261922654264,-36.8846741604791,
21.0848748324737));
#29933=CARTESIAN_POINT('Ctrl Pts',(-13.6777687647333,-36.777988164514,21.0791133094105));
#29934=CARTESIAN_POINT('Ctrl Pts',(-13.7293102997855,-36.6713744921147,
21.0733556921448));
#29935=CARTESIAN_POINT('Ctrl Pts',(-13.7762525571488,-36.5624339432972,
21.067598074879));
#29936=CARTESIAN_POINT('Ctrl Pts',(-13.8183854556858,-36.4516051501037,
21.0618404576133));
#29937=CARTESIAN_POINT('Ctrl Pts',(-13.8624295242089,-36.3357491057475,
21.0558216718618));
#29938=CARTESIAN_POINT('Ctrl Pts',(-13.9012174237302,-36.2178298958137,
21.0498028861103));
#29939=CARTESIAN_POINT('Ctrl Pts',(-13.9345650358115,-36.0983728779288,
21.0437841003588));
#29940=CARTESIAN_POINT('Ctrl Pts',(-13.9664521067682,-35.9841477755052,
21.0380289222111));
#29941=CARTESIAN_POINT('Ctrl Pts',(-13.9933652579074,-35.8685171612166,
21.0322737440633));
#29942=CARTESIAN_POINT('Ctrl Pts',(-14.0151946311413,-35.7519555000491,
21.0265185659155));
#29943=CARTESIAN_POINT('Ctrl Pts',(-14.0370247942173,-35.6353896213848,
21.0207631795308));
#29944=CARTESIAN_POINT('Ctrl Pts',(-14.0537707443996,-35.517893038846,21.0150077931461));
#29945=CARTESIAN_POINT('Ctrl Pts',(-14.0653740111778,-35.3999489332902,
21.0092524067614));
#29946=CARTESIAN_POINT('Ctrl Pts',(-14.0769833472101,-35.2819431353887,
21.0034940099398));
#29947=CARTESIAN_POINT('Ctrl Pts',(-14.0834446009025,-35.1634897617954,
20.9977356131181));
#29948=CARTESIAN_POINT('Ctrl Pts',(-14.0847513050877,-35.0450752214036,
20.9919772162965));
#29949=CARTESIAN_POINT('Ctrl Pts',(-14.0849299821657,-35.0288833668764,
20.9911898203962));
#29950=CARTESIAN_POINT('Ctrl Pts',(-14.0850123618426,-35.0126922365669,
20.9904024244958));
#29951=CARTESIAN_POINT('Ctrl Pts',(-14.0849985032417,-34.9965030709352,
20.9896150285955));
#29952=CARTESIAN_POINT('Origin',(-10.,-35.,32.7603849714045));
#29953=CARTESIAN_POINT('',(-7.5128274573098,-31.7594448403263,23.0467784921743));
#29954=CARTESIAN_POINT('',(-7.5128274573098,-31.7594448403263,22.9427600101556));
#29955=CARTESIAN_POINT('',(-7.5128274573098,-31.7594448403263,32.7603849714045));
#29956=CARTESIAN_POINT('',(-14.084999774902,-34.998643884102,22.1353849714381));
#29957=CARTESIAN_POINT('Ctrl Pts',(-7.5128274573098,-31.7594448403263,22.9427600101556));
#29958=CARTESIAN_POINT('Ctrl Pts',(-7.41810522499216,-31.8321455115984,
22.9369372163922));
#29959=CARTESIAN_POINT('Ctrl Pts',(-7.32667862096095,-31.9089218128983,
22.9311144226289));
#29960=CARTESIAN_POINT('Ctrl Pts',(-7.23889864961535,-31.9894279060444,
22.9252916288655));
#29961=CARTESIAN_POINT('Ctrl Pts',(-7.1740346877293,-32.0489169224724,22.9209889449281));
#29962=CARTESIAN_POINT('Ctrl Pts',(-7.11116115321496,-32.1104417111689,
22.9166862609907));
#29963=CARTESIAN_POINT('Ctrl Pts',(-7.05040557842172,-32.1738510746611,
22.9123835770532));
#29964=CARTESIAN_POINT('Ctrl Pts',(-6.96817416518498,-32.2596743359857,
22.9065599833816));
#29965=CARTESIAN_POINT('Ctrl Pts',(-6.88955900838773,-32.3492279583017,
22.9007363897099));
#29966=CARTESIAN_POINT('Ctrl Pts',(-6.81491676329803,-32.4421747957923,
22.8949127960382));
#29967=CARTESIAN_POINT('Ctrl Pts',(-6.74036869048768,-32.5350043670414,
22.8890965496949));
#29968=CARTESIAN_POINT('Ctrl Pts',(-6.66978381322937,-32.6312183229924,
22.8832803033517));
#29969=CARTESIAN_POINT('Ctrl Pts',(-6.60348180785171,-32.7304429572259,
22.8774640570084));
#29970=CARTESIAN_POINT('Ctrl Pts',(-6.53724617114727,-32.8295682670529,
22.8716536327598));
#29971=CARTESIAN_POINT('Ctrl Pts',(-6.47528510307415,-32.9316979222035,
22.8658432085113));
#29972=CARTESIAN_POINT('Ctrl Pts',(-6.41787746912875,-33.0364259184272,
22.8600327842627));
#29973=CARTESIAN_POINT('Ctrl Pts',(-6.35829683750231,-33.1451180859168,
22.8540024234386));
#29974=CARTESIAN_POINT('Ctrl Pts',(-6.30362144545683,-33.2566088367515,
22.8479720626146));
#29975=CARTESIAN_POINT('Ctrl Pts',(-6.25411329246123,-33.3704117776922,
22.8419417017905));
#29976=CARTESIAN_POINT('Ctrl Pts',(-6.20646447061099,-33.4799407285985,
22.836137817557));
#29977=CARTESIAN_POINT('Ctrl Pts',(-6.16360194235758,-33.5916109199821,
22.8303339333235));
#29978=CARTESIAN_POINT('Ctrl Pts',(-6.12571170368782,-33.7049651753491,
22.8245300490901));
#29979=CARTESIAN_POINT('Ctrl Pts',(-6.08782706181152,-33.8183026870804,
22.8187270221524));
#29980=CARTESIAN_POINT('Ctrl Pts',(-6.05491337832605,-33.933323380932,22.8129239952147));
#29981=CARTESIAN_POINT('Ctrl Pts',(-6.02710744688961,-34.0495528623643,
22.807120968277));
#29982=CARTESIAN_POINT('Ctrl Pts',(-5.9992990604802,-34.1657926056442,22.8013174289927));
#29983=CARTESIAN_POINT('Ctrl Pts',(-5.97659941775086,-34.2832409515463,
22.7955138897084));
#29984=CARTESIAN_POINT('Ctrl Pts',(-5.95909450684952,-34.401411831535,22.7897103504241));
#29985=CARTESIAN_POINT('Ctrl Pts',(-5.94158391930971,-34.519621032962,22.7839049291197));
#29986=CARTESIAN_POINT('Ctrl Pts',(-5.92927147367318,-34.6385528307428,
22.7780995078153));
#29987=CARTESIAN_POINT('Ctrl Pts',(-5.92219138970122,-34.7577151722184,
22.7722940865109));
#29988=CARTESIAN_POINT('Ctrl Pts',(-5.9151034651916,-34.8770094749575,22.7664822362398));
#29989=CARTESIAN_POINT('Ctrl Pts',(-5.91325949261094,-34.996534423144,22.7606703859686));
#29990=CARTESIAN_POINT('Ctrl Pts',(-5.91664156972958,-35.1157969340679,
22.7548585356975));
#29991=CARTESIAN_POINT('Ctrl Pts',(-5.92002586821463,-35.2351377772491,
22.7490428681719));
#29992=CARTESIAN_POINT('Ctrl Pts',(-5.92864302289948,-35.3542154335524,
22.7432272006463));
#29993=CARTESIAN_POINT('Ctrl Pts',(-5.9424233196004,-35.4725425723439,22.7374115331207));
#29994=CARTESIAN_POINT('Ctrl Pts',(-5.95622335508832,-35.5910392019845,
22.7315875352794));
#29995=CARTESIAN_POINT('Ctrl Pts',(-5.975201229148,-35.7087827666983,22.725763537438));
#29996=CARTESIAN_POINT('Ctrl Pts',(-5.999236257892,-35.8252966011283,22.7199395395967));
#29997=CARTESIAN_POINT('Ctrl Pts',(-6.00561288201903,-35.8562083564531,
22.7183944012261));
#29998=CARTESIAN_POINT('Ctrl Pts',(-6.01234519332932,-35.8870336423358,
22.7168492628555));
#29999=CARTESIAN_POINT('Ctrl Pts',(-6.01943035767116,-35.9177637618527,
22.7153041244849));
#30000=CARTESIAN_POINT('Ctrl Pts',(-6.04613419145459,-36.0335849290314,
22.7094805308136));
#30001=CARTESIAN_POINT('Ctrl Pts',(-6.07794029159739,-36.1484264116932,
22.7036569371423));
#30002=CARTESIAN_POINT('Ctrl Pts',(-6.11476218449411,-36.2618051026062,
22.6978333434711));
#30003=CARTESIAN_POINT('Ctrl Pts',(-6.15153762110352,-36.3750407494597,
22.6920170971283));
#30004=CARTESIAN_POINT('Ctrl Pts',(-6.19331613887172,-36.486816890333,22.6862008507854));
#30005=CARTESIAN_POINT('Ctrl Pts',(-6.23996041545217,-36.5966613049214,
22.6803846044426));
#30006=CARTESIAN_POINT('Ctrl Pts',(-6.28655800085441,-36.7063957646448,
22.6745741801945));
#30007=CARTESIAN_POINT('Ctrl Pts',(-6.33801149682606,-36.8142019711841,
22.6687637559463));
#30008=CARTESIAN_POINT('Ctrl Pts',(-6.39413419703498,-36.9196241327425,
22.6629533316982));
#30009=CARTESIAN_POINT('Ctrl Pts',(-6.45238125753123,-37.0290367411715,
22.6569229708739));
#30010=CARTESIAN_POINT('Ctrl Pts',(-6.5156578460597,-37.1358808302093,22.6508926100497));
#30011=CARTESIAN_POINT('Ctrl Pts',(-6.58370077591591,-37.2396706480022,
22.6448622492255));
#30012=CARTESIAN_POINT('Ctrl Pts',(-6.64918828143554,-37.3395625292006,
22.6390583649924));
#30013=CARTESIAN_POINT('Ctrl Pts',(-6.71909033052298,-37.4366250425797,
22.6332544807594));
#30014=CARTESIAN_POINT('Ctrl Pts',(-6.79312651017591,-37.5304520189609,
22.6274505965263));
#30015=CARTESIAN_POINT('Ctrl Pts',(-6.86715175389339,-37.6242651360944,
22.6216475695891));
#30016=CARTESIAN_POINT('Ctrl Pts',(-6.94530966089996,-37.7148433461959,
22.6158445426518));
#30017=CARTESIAN_POINT('Ctrl Pts',(-7.02727844659211,-37.8018121931893,
22.6100415157145));
#30018=CARTESIAN_POINT('Ctrl Pts',(-7.10925446927085,-37.8887887186224,
22.6042379764306));
#30019=CARTESIAN_POINT('Ctrl Pts',(-7.19504175951718,-37.9721549501883,
22.5984344371467));
#30020=CARTESIAN_POINT('Ctrl Pts',(-7.28428091920406,-38.0515725248142,
22.5926308978629));
#30021=CARTESIAN_POINT('Ctrl Pts',(-7.37354901810982,-38.1310158536335,
22.5868254765589));
#30022=CARTESIAN_POINT('Ctrl Pts',(-7.46627090781355,-38.2065077075568,
22.5810200552549));
#30023=CARTESIAN_POINT('Ctrl Pts',(-7.56205380769615,-38.2777497408178,
22.5752146339509));
#30024=CARTESIAN_POINT('Ctrl Pts',(-7.65794277827479,-38.3490706680365,
22.5694027836801));
#30025=CARTESIAN_POINT('Ctrl Pts',(-7.7568991974959,-38.4161321366073,22.5635909334094));
#30026=CARTESIAN_POINT('Ctrl Pts',(-7.85850085185827,-38.4786788294564,
22.5577790831387));
#30027=CARTESIAN_POINT('Ctrl Pts',(-7.96016923873276,-38.5412666033093,
22.5519634156135));
#30028=CARTESIAN_POINT('Ctrl Pts',(-8.06448596486752,-38.599333497768,22.5461477480883));
#30029=CARTESIAN_POINT('Ctrl Pts',(-8.17100522620586,-38.6526706828612,
22.540332080563));
#30030=CARTESIAN_POINT('Ctrl Pts',(-8.27767706488404,-38.7060842677126,
22.5345080827221));
#30031=CARTESIAN_POINT('Ctrl Pts',(-8.38655736429783,-38.7547544550232,
22.5286840848811));
#30032=CARTESIAN_POINT('Ctrl Pts',(-8.4971813007853,-38.7985208907272,22.5228600870402));
#30033=CARTESIAN_POINT('Ctrl Pts',(-8.52653043416117,-38.8101323646961,
22.5213149486656));
#30034=CARTESIAN_POINT('Ctrl Pts',(-8.55600222174986,-38.8213989527676,
22.519769810291));
#30035=CARTESIAN_POINT('Ctrl Pts',(-8.58558783611663,-38.8323182580076,
22.5182246719164));
#30036=CARTESIAN_POINT('Ctrl Pts',(-8.69709538742309,-38.8734728872202,
22.5124010782454));
#30037=CARTESIAN_POINT('Ctrl Pts',(-8.81058043544505,-38.9098231007045,
22.5065774845743));
#30038=CARTESIAN_POINT('Ctrl Pts',(-8.92559152155281,-38.9411764007008,
22.5007538909033));
#30039=CARTESIAN_POINT('Ctrl Pts',(-9.04045750409189,-38.972490143852,22.4949376445607));
#30040=CARTESIAN_POINT('Ctrl Pts',(-9.15684530480536,-38.9988194062653,
22.4891213982181));
#30041=CARTESIAN_POINT('Ctrl Pts',(-9.27428469714738,-39.0200201864177,
22.4833051518755));
#30042=CARTESIAN_POINT('Ctrl Pts',(-9.39160653200965,-39.0411997444721,
22.4774947276276));
#30043=CARTESIAN_POINT('Ctrl Pts',(-9.50997746485374,-39.0572609608792,
22.4716843033797));
#30044=CARTESIAN_POINT('Ctrl Pts',(-9.62891393896168,-39.068110142966,22.4658738791318));
#30045=CARTESIAN_POINT('Ctrl Pts',(-9.75235240462994,-39.079369989036,22.4598435183075));
#30046=CARTESIAN_POINT('Ctrl Pts',(-9.87639963886841,-39.0850153142075,
22.4538131574831));
#30047=CARTESIAN_POINT('Ctrl Pts',(-10.0005051034775,-39.0849999687724,
22.4477827966588));
#30048=CARTESIAN_POINT('Ctrl Pts',(-10.1199496558406,-39.0849851996514,
22.441978912426));
#30049=CARTESIAN_POINT('Ctrl Pts',(-10.2394476985915,-39.0797272772861,
22.4361750281932));
#30050=CARTESIAN_POINT('Ctrl Pts',(-10.3585058113548,-39.0692380838708,
22.4303711439604));
#30051=CARTESIAN_POINT('Ctrl Pts',(-10.4775463379617,-39.0587504398216,
22.4245681170234));
#30052=CARTESIAN_POINT('Ctrl Pts',(-10.5961466571589,-39.0430330972343,
22.4187650900863));
#30053=CARTESIAN_POINT('Ctrl Pts',(-10.7138171940898,-39.0221499242845,
22.4129620631493));
#30054=CARTESIAN_POINT('Ctrl Pts',(-10.8314981200985,-39.0012649075689,
22.4071585238657));
#30055=CARTESIAN_POINT('Ctrl Pts',(-10.9482486985517,-38.9752132250327,
22.401354984582));
#30056=CARTESIAN_POINT('Ctrl Pts',(-11.0635889233761,-38.944109988587,22.3955514452984));
#30057=CARTESIAN_POINT('Ctrl Pts',(-11.1789665516905,-38.9129966657244,
22.3897460239947));
#30058=CARTESIAN_POINT('Ctrl Pts',(-11.292932522737,-38.8768286372834,22.3839406026909));
#30059=CARTESIAN_POINT('Ctrl Pts',(-11.4050220006962,-38.8357708713581,
22.3781351813872));
#30060=CARTESIAN_POINT('Ctrl Pts',(-11.5172356073774,-38.7946676377574,
22.3723233311167));
#30061=CARTESIAN_POINT('Ctrl Pts',(-11.6275681893694,-38.7486639985343,
22.3665114808462));
#30062=CARTESIAN_POINT('Ctrl Pts',(-11.735574764776,-38.6979731253584,22.3606996305757));
#30063=CARTESIAN_POINT('Ctrl Pts',(-11.8436522794811,-38.6472489581448,
22.3548839630508));
#30064=CARTESIAN_POINT('Ctrl Pts',(-11.9494003842303,-38.5918316149719,
22.3490682955258));
#30065=CARTESIAN_POINT('Ctrl Pts',(-12.0524000461147,-38.531979480505,22.3432526280009));
#30066=CARTESIAN_POINT('Ctrl Pts',(-12.1555472438929,-38.4720416143183,
22.3374286301602));
#30067=CARTESIAN_POINT('Ctrl Pts',(-12.2559377985724,-38.4076564975345,
22.3316046323195));
#30068=CARTESIAN_POINT('Ctrl Pts',(-12.3531827952385,-38.339124994994,22.3257806344788));
#30069=CARTESIAN_POINT('Ctrl Pts',(-12.3789824229897,-38.3209432137672,
22.3242354961018));
#30070=CARTESIAN_POINT('Ctrl Pts',(-12.4045608326993,-38.302469794208,22.3226903577249));
#30071=CARTESIAN_POINT('Ctrl Pts',(-12.4299111807624,-38.283710805416,22.321145219348));
#30072=CARTESIAN_POINT('Ctrl Pts',(-12.5246533662664,-38.2136025926385,
22.3153705535969));
#30073=CARTESIAN_POINT('Ctrl Pts',(-12.6165244936633,-38.1392680574621,
22.3095958878458));
#30074=CARTESIAN_POINT('Ctrl Pts',(-12.705119863426,-38.0609723168461,22.3038212220948));
#30075=CARTESIAN_POINT('Ctrl Pts',(-12.7936030129361,-37.9827757503496,
22.2980538708845));
#30076=CARTESIAN_POINT('Ctrl Pts',(-12.8788183458607,-37.9006282274634,
22.2922865196743));
#30077=CARTESIAN_POINT('Ctrl Pts',(-12.9603911014523,-37.8148373889875,
22.286519168464));
#30078=CARTESIAN_POINT('Ctrl Pts',(-13.0418827354362,-37.7291318668737,
22.280757552708));
#30079=CARTESIAN_POINT('Ctrl Pts',(-13.1197387110851,-37.6397905343191,
22.2749959369519));
#30080=CARTESIAN_POINT('Ctrl Pts',(-13.1936188085971,-37.5471599685483,
22.2692343211959));
#30081=CARTESIAN_POINT('Ctrl Pts',(-13.2674469120441,-37.4545945927248,
22.2634767602507));
#30082=CARTESIAN_POINT('Ctrl Pts',(-13.3373044441074,-37.3587449120252,
22.2577191993056));
#30083=CARTESIAN_POINT('Ctrl Pts',(-13.4028898721003,-37.2599923713051,
22.2519616383604));
#30084=CARTESIAN_POINT('Ctrl Pts',(-13.4684512490783,-37.1612760444041,
22.2462061887865));
#30085=CARTESIAN_POINT('Ctrl Pts',(-13.5297434061283,-37.0596593195178,
22.2404507392125));
#30086=CARTESIAN_POINT('Ctrl Pts',(-13.586507122281,-36.955554054949,22.2346952896386));
#30087=CARTESIAN_POINT('Ctrl Pts',(-13.6432640019227,-36.851461328615,22.2289405332397));
#30088=CARTESIAN_POINT('Ctrl Pts',(-13.6954933261915,-36.7448810238551,
22.2231857768409));
#30089=CARTESIAN_POINT('Ctrl Pts',(-13.7429813543258,-36.63625046407,22.217431020442));
#30090=CARTESIAN_POINT('Ctrl Pts',(-13.7904753584461,-36.5276062340037,
22.2116755398534));
#30091=CARTESIAN_POINT('Ctrl Pts',(-13.8332267144446,-36.4169116175228,
22.2059200592648));
#30092=CARTESIAN_POINT('Ctrl Pts',(-13.8710697362876,-36.3046241208862,
22.2001645786762));
#30093=CARTESIAN_POINT('Ctrl Pts',(-13.9089487815479,-36.1922297358682,
22.1944036193476));
#30094=CARTESIAN_POINT('Ctrl Pts',(-13.9419100289835,-36.0782398375382,
22.1886426600189));
#30095=CARTESIAN_POINT('Ctrl Pts',(-13.9698376062256,-35.9631273956215,
22.1828817006903));
#30096=CARTESIAN_POINT('Ctrl Pts',(-13.9977791248229,-35.8479574899511,
22.1771178655096));
#30097=CARTESIAN_POINT('Ctrl Pts',(-14.0206818886153,-35.7316643327201,
22.171354030329));
#30098=CARTESIAN_POINT('Ctrl Pts',(-14.0384814547981,-35.6147296472856,
22.1655901951483));
#30099=CARTESIAN_POINT('Ctrl Pts',(-14.0563077963075,-35.4976190606882,
22.159817689612));
#30100=CARTESIAN_POINT('Ctrl Pts',(-14.0690155630157,-35.3798654318944,
22.1540451840757));
#30101=CARTESIAN_POINT('Ctrl Pts',(-14.0765923082484,-35.2619544852256,
22.1482726785393));
#30102=CARTESIAN_POINT('Ctrl Pts',(-14.0822309269687,-35.1742050821785,
22.1439767761723));
#30103=CARTESIAN_POINT('Ctrl Pts',(-14.085028897281,-35.0863686218627,22.1396808738052));
#30104=CARTESIAN_POINT('Ctrl Pts',(-14.084999774902,-34.998643884102,22.1353849714381));
#30105=CARTESIAN_POINT('Ctrl Pts',(-14.0849997749018,-34.9986438834154,
22.1353849714045));
#30106=CARTESIAN_POINT('Ctrl Pts',(-14.0849741968582,-34.9215957126599,
22.1316119031962));
#30107=CARTESIAN_POINT('Ctrl Pts',(-14.0827689216963,-34.8445868960997,
22.1278388349879));
#30108=CARTESIAN_POINT('Ctrl Pts',(-14.0783897720535,-34.7677030624194,
22.1240657667795));
#30109=CARTESIAN_POINT('Ctrl Pts',(-14.0716307137146,-34.6490356590298,
22.1182421731102));
#30110=CARTESIAN_POINT('Ctrl Pts',(-14.0596772245187,-34.5304721392025,
22.1124185794409));
#30111=CARTESIAN_POINT('Ctrl Pts',(-14.0425329433292,-34.4125032748195,
22.1065949857715));
#30112=CARTESIAN_POINT('Ctrl Pts',(-14.025410292197,-34.2946832456818,22.1007787394306));
#30113=CARTESIAN_POINT('Ctrl Pts',(-14.0031099329978,-34.1774567802964,
22.0949624930897));
#30114=CARTESIAN_POINT('Ctrl Pts',(-13.9756874615845,-34.0613125079135,
22.0891462467488));
#30115=CARTESIAN_POINT('Ctrl Pts',(-13.9482924402164,-33.9452844965879,
22.0833358225026));
#30116=CARTESIAN_POINT('Ctrl Pts',(-13.9157855999802,-33.8303369183369,
22.0775253982564));
#30117=CARTESIAN_POINT('Ctrl Pts',(-13.8782739859287,-33.7169505504195,
22.0717149740101));
#30118=CARTESIAN_POINT('Ctrl Pts',(-13.8393424796786,-33.5992722738948,
22.0656846131852));
#30119=CARTESIAN_POINT('Ctrl Pts',(-13.7950198958776,-33.4832761765968,
22.0596542523602));
#30120=CARTESIAN_POINT('Ctrl Pts',(-13.7454836013007,-33.3694854823133,
22.0536238915353));
#30121=CARTESIAN_POINT('Ctrl Pts',(-13.697807694782,-33.2599683181874,22.0478200073041));
#30122=CARTESIAN_POINT('Ctrl Pts',(-13.6453028057686,-33.1524942999704,
22.0420161230729));
#30123=CARTESIAN_POINT('Ctrl Pts',(-13.5881767206801,-33.0475111213712,
22.0362122388418));
#30124=CARTESIAN_POINT('Ctrl Pts',(-13.5310590737252,-32.9425434499099,
22.0304092119063));
#30125=CARTESIAN_POINT('Ctrl Pts',(-13.4693217832893,-32.84006624496,22.0246061849709));
#30126=CARTESIAN_POINT('Ctrl Pts',(-13.4032187691399,-32.7405029299922,
22.0188031580355));
#30127=CARTESIAN_POINT('Ctrl Pts',(-13.3371099187855,-32.6409308246247,
22.0129996187535));
#30128=CARTESIAN_POINT('Ctrl Pts',(-13.266634804225,-32.5442734609492,22.0071960794715));
#30129=CARTESIAN_POINT('Ctrl Pts',(-13.1920905142082,-32.4509250405094,
22.0013925401894));
#30130=CARTESIAN_POINT('Ctrl Pts',(-13.1175220503471,-32.357546348265,21.9955871188873));
#30131=CARTESIAN_POINT('Ctrl Pts',(-13.0388820413454,-32.2674790522316,
21.9897816975851));
#30132=CARTESIAN_POINT('Ctrl Pts',(-12.9565072374636,-32.1810835495132,
21.983976276283));
#30133=CARTESIAN_POINT('Ctrl Pts',(-12.8740412111105,-32.0945923717715,
21.978164426014));
#30134=CARTESIAN_POINT('Ctrl Pts',(-12.7878324161339,-32.0117813994789,
21.9723525757451));
#30135=CARTESIAN_POINT('Ctrl Pts',(-12.698253880029,-31.9329735901189,21.9665407254761));
#30136=CARTESIAN_POINT('Ctrl Pts',(-12.6086165082604,-31.8541140193662,
21.9607250579527));
#30137=CARTESIAN_POINT('Ctrl Pts',(-12.51560530498,-31.7792631032794,21.9549093904292));
#30138=CARTESIAN_POINT('Ctrl Pts',(-12.4196244006124,-31.7087019642759,
21.9490937229058));
#30139=CARTESIAN_POINT('Ctrl Pts',(-12.3235060139627,-31.6380397540596,
21.9432697250666));
#30140=CARTESIAN_POINT('Ctrl Pts',(-12.2244097740045,-31.5716798116975,
21.9374457272273));
#30141=CARTESIAN_POINT('Ctrl Pts',(-12.1227667446957,-31.5098586923143,
21.9316217293881));
#30142=CARTESIAN_POINT('Ctrl Pts',(-12.0958002946327,-31.4934572121535,
21.9300765909958));
#30143=CARTESIAN_POINT('Ctrl Pts',(-12.0686547041485,-31.4773749483047,
21.9285314526034));
#30144=CARTESIAN_POINT('Ctrl Pts',(-12.0413382690486,-31.4616157541446,
21.9269863142111));
#30145=CARTESIAN_POINT('Ctrl Pts',(-11.9383832073534,-31.4022196872316,
21.9211627205419));
#30146=CARTESIAN_POINT('Ctrl Pts',(-11.8326676330743,-31.3472250375885,
21.9153391268728));
#30147=CARTESIAN_POINT('Ctrl Pts',(-11.7246040083446,-31.2968977850454,
21.9095155332036));
#30148=CARTESIAN_POINT('Ctrl Pts',(-11.6166767219297,-31.2466340278071,
21.903699286863));
#30149=CARTESIAN_POINT('Ctrl Pts',(-11.5064076441365,-31.2010261262243,
21.8978830405223));
#30150=CARTESIAN_POINT('Ctrl Pts',(-11.3942359259922,-31.1602954302873,
21.8920667941816));
#30151=CARTESIAN_POINT('Ctrl Pts',(-11.2821764923571,-31.1196055060018,
21.8862563699356));
#30152=CARTESIAN_POINT('Ctrl Pts',(-11.1682185888553,-31.0837832135761,
21.8804459456896));
#30153=CARTESIAN_POINT('Ctrl Pts',(-11.0528230019126,-31.053002568199,21.8746355214437));
#30154=CARTESIAN_POINT('Ctrl Pts',(-10.9330594532589,-31.0210568117114,
21.8686051606186));
#30155=CARTESIAN_POINT('Ctrl Pts',(-10.8117476384181,-30.9945421063119,
21.8625747997936));
#30156=CARTESIAN_POINT('Ctrl Pts',(-10.689422392675,-30.9735969197709,21.8565444389685));
#30157=CARTESIAN_POINT('Ctrl Pts',(-10.571691201226,-30.9534383519167,21.8507405547377));
#30158=CARTESIAN_POINT('Ctrl Pts',(-10.4530217657443,-30.9384385838515,
21.8449366705069));
#30159=CARTESIAN_POINT('Ctrl Pts',(-10.3339024252768,-30.9286692383946,
21.8391327862761));
#30160=CARTESIAN_POINT('Ctrl Pts',(-10.21480068001,-30.9189013359745,21.833329759341));
#30161=CARTESIAN_POINT('Ctrl Pts',(-10.0952495687778,-30.9143623530944,
21.827526732406));
#30162=CARTESIAN_POINT('Ctrl Pts',(-9.97574242032107,-30.9150720239118,
21.8217237054709));
#30163=CARTESIAN_POINT('Ctrl Pts',(-9.85622472063311,-30.9157817573857,
21.8159201661893));
#30164=CARTESIAN_POINT('Ctrl Pts',(-9.73675139978788,-30.9217410634859,
21.8101166269077));
#30165=CARTESIAN_POINT('Ctrl Pts',(-9.61781500981382,-30.9329175526827,
21.8043130876261));
#30166=CARTESIAN_POINT('Ctrl Pts',(-9.49884005015554,-30.9440976662846,
21.7985076663243));
#30167=CARTESIAN_POINT('Ctrl Pts',(-9.38040277399139,-30.9604982895504,
21.7927022450226));
#30168=CARTESIAN_POINT('Ctrl Pts',(-9.26298920128755,-30.9820353308446,
21.7868968237208));
#30169=CARTESIAN_POINT('Ctrl Pts',(-9.14544560391974,-31.0035962224185,
21.7810849734524));
#30170=CARTESIAN_POINT('Ctrl Pts',(-9.02892837476259,-31.0303048122552,
21.7752731231839));
#30171=CARTESIAN_POINT('Ctrl Pts',(-8.9139121062226,-31.0620261444507,21.7694612729154));
#30172=CARTESIAN_POINT('Ctrl Pts',(-8.79882029437999,-31.0937683113873,
21.7636456053925));
#30173=CARTESIAN_POINT('Ctrl Pts',(-8.68523179408255,-31.1305296521297,
21.7578299378695));
#30174=CARTESIAN_POINT('Ctrl Pts',(-8.57360325758762,-31.1721262647215,
21.7520142703466));
#30175=CARTESIAN_POINT('Ctrl Pts',(-8.46181482526753,-31.2137824599693,
21.7461902725079));
#30176=CARTESIAN_POINT('Ctrl Pts',(-8.35199233491958,-31.260287592335,21.7403662746692));
#30177=CARTESIAN_POINT('Ctrl Pts',(-8.24456992798524,-31.3114108032655,
21.7345422768305));
#30178=CARTESIAN_POINT('Ctrl Pts',(-8.21607017744642,-31.3249740699977,
21.7329971384346));
#30179=CARTESIAN_POINT('Ctrl Pts',(-8.18773921196682,-31.338862147366,21.7314520000386));
#30180=CARTESIAN_POINT('Ctrl Pts',(-8.15958480185818,-31.353070209279,21.7299068616426));
#30181=CARTESIAN_POINT('Ctrl Pts',(-8.05345316483866,-31.4066293093942,
21.7240822655402));
#30182=CARTESIAN_POINT('Ctrl Pts',(-7.94949028075317,-31.4649115462035,
21.7182576694377));
#30183=CARTESIAN_POINT('Ctrl Pts',(-7.84814493422774,-31.5277176416786,
21.7124330733352));
#30184=CARTESIAN_POINT('Ctrl Pts',(-7.74693946603362,-31.590437051261,21.7066165164256));
#30185=CARTESIAN_POINT('Ctrl Pts',(-7.64834469086719,-31.6576676818168,
21.700799959516));
#30186=CARTESIAN_POINT('Ctrl Pts',(-7.55278652953408,-31.7291635274795,
21.6949834026064));
#30187=CARTESIAN_POINT('Ctrl Pts',(-7.53940697095604,-31.7391740053057,
21.6941689984486));
#30188=CARTESIAN_POINT('Ctrl Pts',(-7.52608690363846,-31.7492680251774,
21.6933545942909));
#30189=CARTESIAN_POINT('Ctrl Pts',(-7.5128274573098,-31.7594448403263,21.6925401901332));
#30190=CARTESIAN_POINT('',(-14.0849992774348,-35.002429682444,22.2396150286382));
#30191=CARTESIAN_POINT('Ctrl Pts',(-14.0849992774354,-35.0024296815638,
22.2396150285955));
#30192=CARTESIAN_POINT('Ctrl Pts',(-14.085070989627,-34.8818606921073,22.233766442302));
#30193=CARTESIAN_POINT('Ctrl Pts',(-14.0798004648248,-34.7612723331048,
22.2279178560085));
#30194=CARTESIAN_POINT('Ctrl Pts',(-14.0692091476505,-34.6411658981124,
22.2220692697149));
#30195=CARTESIAN_POINT('Ctrl Pts',(-14.0586166826974,-34.5210464472109,
22.2162200496114));
#30196=CARTESIAN_POINT('Ctrl Pts',(-14.0427023124912,-34.4014094220384,
22.2103708295078));
#30197=CARTESIAN_POINT('Ctrl Pts',(-14.0215393834306,-34.2827510979325,
22.2045216094042));
#30198=CARTESIAN_POINT('Ctrl Pts',(-14.0003694708715,-34.1640536180835,
22.1986704591321));
#30199=CARTESIAN_POINT('Ctrl Pts',(-13.9739476225001,-34.0463358750017,
22.19281930886));
#30200=CARTESIAN_POINT('Ctrl Pts',(-13.9423982256987,-33.9300835406406,
22.1869681585879));
#30201=CARTESIAN_POINT('Ctrl Pts',(-13.9108091820572,-33.8136851167132,
22.1811096554139));
#30202=CARTESIAN_POINT('Ctrl Pts',(-13.8740798226738,-33.6987561662509,
22.1752511522399));
#30203=CARTESIAN_POINT('Ctrl Pts',(-13.832384485157,-33.5857672900376,22.169392649066));
#30204=CARTESIAN_POINT('Ctrl Pts',(-13.7906628672974,-33.4727071975545,
22.1635304533095));
#30205=CARTESIAN_POINT('Ctrl Pts',(-13.7439691883523,-33.3615899841287,
22.1576682575531));
#30206=CARTESIAN_POINT('Ctrl Pts',(-13.6925253126231,-33.2528646830776,
22.1518060617967));
#30207=CARTESIAN_POINT('Ctrl Pts',(-13.6409886366956,-33.143943251207,22.145933291158));
#30208=CARTESIAN_POINT('Ctrl Pts',(-13.5846848248018,-33.0374227087693,
22.1400605205193));
#30209=CARTESIAN_POINT('Ctrl Pts',(-13.5238813533309,-32.9337267345176,
22.1341877498806));
#30210=CARTESIAN_POINT('Ctrl Pts',(-13.4639491572571,-32.8315166581756,
22.1283991323412));
#30211=CARTESIAN_POINT('Ctrl Pts',(-13.3996456789967,-32.7320509915328,
22.1226105148018));
#30212=CARTESIAN_POINT('Ctrl Pts',(-13.3312658119027,-32.635704525562,22.1168218972623));
#30213=CARTESIAN_POINT('Ctrl Pts',(-13.2624727782426,-32.5387759125325,
22.1109983035913));
#30214=CARTESIAN_POINT('Ctrl Pts',(-13.1893348551765,-32.4446959552913,
22.1051747099203));
#30215=CARTESIAN_POINT('Ctrl Pts',(-13.1121159531807,-32.3538784430873,
22.0993511162492));
#30216=CARTESIAN_POINT('Ctrl Pts',(-13.0349944742999,-32.263175510665,22.0935348699066));
#30217=CARTESIAN_POINT('Ctrl Pts',(-12.9538025194292,-32.1757271448803,
22.087718623564));
#30218=CARTESIAN_POINT('Ctrl Pts',(-12.8688468720517,-32.0919177066804,
22.0819023772214));
#30219=CARTESIAN_POINT('Ctrl Pts',(-12.7839762657458,-32.0081921621904,
22.0760919529735));
#30220=CARTESIAN_POINT('Ctrl Pts',(-12.6953497508832,-31.9280985839322,
22.0702815287256));
#30221=CARTESIAN_POINT('Ctrl Pts',(-12.6033135194904,-31.8519873381388,
22.0644711044777));
#30222=CARTESIAN_POINT('Ctrl Pts',(-12.5077935263662,-31.7729951242591,
22.0584407436534));
#30223=CARTESIAN_POINT('Ctrl Pts',(-12.4086008771729,-31.6982930201086,
22.052410382829));
#30224=CARTESIAN_POINT('Ctrl Pts',(-12.3061638909232,-31.6282299740045,
22.0463800220047));
#30225=CARTESIAN_POINT('Ctrl Pts',(-12.2075740342512,-31.5607982198471,
22.0405761377719));
#30226=CARTESIAN_POINT('Ctrl Pts',(-12.105979502287,-31.4976636093401,22.0347722535391));
#30227=CARTESIAN_POINT('Ctrl Pts',(-12.0017942403327,-31.4390949437859,
22.0289683693063));
#30228=CARTESIAN_POINT('Ctrl Pts',(-11.8976243676558,-31.38053492945,22.0231653423693));
#30229=CARTESIAN_POINT('Ctrl Pts',(-11.7908648818679,-31.3265397188664,
22.0173623154322));
#30230=CARTESIAN_POINT('Ctrl Pts',(-11.6819559081383,-31.2773330362388,
22.0115592884952));
#30231=CARTESIAN_POINT('Ctrl Pts',(-11.573037318885,-31.2281220091757,22.0057557492116));
#30232=CARTESIAN_POINT('Ctrl Pts',(-11.4619692365034,-31.1837005187882,
21.9999522099279));
#30233=CARTESIAN_POINT('Ctrl Pts',(-11.3492128233251,-31.1442445931601,
21.9941486706443));
#30234=CARTESIAN_POINT('Ctrl Pts',(-11.2364198445569,-31.1047758724355,
21.9883432493405));
#30235=CARTESIAN_POINT('Ctrl Pts',(-11.1219378313496,-31.0702760537414,
21.9825378280368));
#30236=CARTESIAN_POINT('Ctrl Pts',(-11.0062435766426,-31.0408714513841,
21.976732406733));
#30237=CARTESIAN_POINT('Ctrl Pts',(-10.8904212012571,-31.0114342861514,
21.9709205564625));
#30238=CARTESIAN_POINT('Ctrl Pts',(-10.7733843007257,-30.9871037007735,
21.965108706192));
#30239=CARTESIAN_POINT('Ctrl Pts',(-10.6556204998703,-30.9679550151133,
21.9592968559216));
#30240=CARTESIAN_POINT('Ctrl Pts',(-10.5377793511181,-30.9487937524935,
21.9534811883966));
#30241=CARTESIAN_POINT('Ctrl Pts',(-10.4192107558225,-30.9348212154259,
21.9476655208716));
#30242=CARTESIAN_POINT('Ctrl Pts',(-10.3004064516107,-30.9260607559966,
21.9418498533467));
#30243=CARTESIAN_POINT('Ctrl Pts',(-10.1814319730621,-30.9172877481552,
21.936025855506));
#30244=CARTESIAN_POINT('Ctrl Pts',(-10.0622215184187,-30.913741731258,21.9302018576653));
#30245=CARTESIAN_POINT('Ctrl Pts',(-9.94326595421711,-30.9153939910869,
21.9243778598246));
#30246=CARTESIAN_POINT('Ctrl Pts',(-9.91170639454354,-30.9158323446269,
21.9228327214477));
#30247=CARTESIAN_POINT('Ctrl Pts',(-9.88016474084331,-30.916636306858,21.9212875830708));
#30248=CARTESIAN_POINT('Ctrl Pts',(-9.84865006826418,-30.9178047329698,
21.9197424446939));
#30249=CARTESIAN_POINT('Ctrl Pts',(-9.72988906658467,-30.9222078710662,
21.913919690835));
#30250=CARTESIAN_POINT('Ctrl Pts',(-9.61112888813309,-30.9318049790338,
21.908096936976));
#30251=CARTESIAN_POINT('Ctrl Pts',(-9.49286006789792,-30.9466021550719,
21.9022741831171));
#30252=CARTESIAN_POINT('Ctrl Pts',(-9.37473174463704,-30.9613817528637,
21.8964583463755));
#30253=CARTESIAN_POINT('Ctrl Pts',(-9.25709402033374,-30.9813490857124,
21.8906425096338));
#30254=CARTESIAN_POINT('Ctrl Pts',(-9.14043642792352,-31.0064582804785,
21.8848266728922));
#30255=CARTESIAN_POINT('Ctrl Pts',(-9.02388987404794,-31.0315435754868,
21.8790163718553));
#30256=CARTESIAN_POINT('Ctrl Pts',(-8.9083219934234,-31.0617609132255,21.8732060708184));
#30257=CARTESIAN_POINT('Ctrl Pts',(-8.79421556330646,-31.0970128244859,
21.8673957697815));
#30258=CARTESIAN_POINT('Ctrl Pts',(-8.67893007358786,-31.132628993084,21.861525431013));
#30259=CARTESIAN_POINT('Ctrl Pts',(-8.5651368289882,-31.1733843249257,21.8556550922445));
#30260=CARTESIAN_POINT('Ctrl Pts',(-8.4533218646113,-31.2191255316381,21.849784753476));
#30261=CARTESIAN_POINT('Ctrl Pts',(-8.34277849542931,-31.2643465548582,
21.8439811740595));
#30262=CARTESIAN_POINT('Ctrl Pts',(-8.23416902713381,-31.314440469642,21.8381775946431));
#30263=CARTESIAN_POINT('Ctrl Pts',(-8.12794568099241,-31.3692097793063,
21.8323740152266));
#30264=CARTESIAN_POINT('Ctrl Pts',(-8.01988948276489,-31.4249241170376,
21.8264702967821));
#30265=CARTESIAN_POINT('Ctrl Pts',(-7.91430292008785,-31.4854765379561,
21.8205665783376));
#30266=CARTESIAN_POINT('Ctrl Pts',(-7.81163757497356,-31.5506094890934,
21.814662859893));
#30267=CARTESIAN_POINT('Ctrl Pts',(-7.70897222985925,-31.6157424402308,
21.8087591414485));
#30268=CARTESIAN_POINT('Ctrl Pts',(-7.60922847440342,-31.6854556776709,
21.802855423004));
#30269=CARTESIAN_POINT('Ctrl Pts',(-7.51282745730979,-31.7594448403263,
21.7969517045595));
#30270=CARTESIAN_POINT('Ctrl Pts',(-7.5128274573098,-31.7594448403263,23.0467784921743));
#30271=CARTESIAN_POINT('Ctrl Pts',(-7.41657407421678,-31.8333206917696,
23.0408768761477));
#30272=CARTESIAN_POINT('Ctrl Pts',(-7.32354678406087,-31.9115410529426,
23.0349752601211));
#30273=CARTESIAN_POINT('Ctrl Pts',(-7.23415358548507,-31.9937866657014,
23.0290736440946));
#30274=CARTESIAN_POINT('Ctrl Pts',(-7.1462441309189,-32.074667169736,23.0232699828069));
#30275=CARTESIAN_POINT('Ctrl Pts',(-7.06184936093566,-32.1594400346389,
23.0174663215192));
#30276=CARTESIAN_POINT('Ctrl Pts',(-6.98132346380725,-32.2477614620387,
23.0116626602315));
#30277=CARTESIAN_POINT('Ctrl Pts',(-6.90080651065365,-32.3360730796177,
23.0058596435538));
#30278=CARTESIAN_POINT('Ctrl Pts',(-6.82415785080753,-32.4279321741339,
23.0000566268762));
#30279=CARTESIAN_POINT('Ctrl Pts',(-6.75169352034171,-32.5229594241898,
22.9942536101985));
#30280=CARTESIAN_POINT('Ctrl Pts',(-6.67922013687654,-32.6179985460402,
22.9884498685475));
#30281=CARTESIAN_POINT('Ctrl Pts',(-6.61093236983824,-32.7162062857298,
22.9826461268965));
#30282=CARTESIAN_POINT('Ctrl Pts',(-6.54710441122387,-32.8171722346895,
22.9768423852455));
#30283=CARTESIAN_POINT('Ctrl Pts',(-6.48139054620653,-32.9211213956109,
22.9708671621031));
#30284=CARTESIAN_POINT('Ctrl Pts',(-6.42040438537492,-33.0279939058608,
22.9648919389606));
#30285=CARTESIAN_POINT('Ctrl Pts',(-6.36439501581763,-33.1373133921703,
22.9589167158182));
#30286=CARTESIAN_POINT('Ctrl Pts',(-6.30991131226698,-33.2436550727046,
22.9531042546369));
#30287=CARTESIAN_POINT('Ctrl Pts',(-6.26013688993258,-33.3523117422711,
22.9472917934555));
#30288=CARTESIAN_POINT('Ctrl Pts',(-6.21525217972208,-33.4628243636781,
22.9414793322742));
#30289=CARTESIAN_POINT('Ctrl Pts',(-6.16848216054422,-33.5779788873091,
22.9354227281512));
#30290=CARTESIAN_POINT('Ctrl Pts',(-6.12702175079582,-33.695148202419,22.9293661240282));
#30291=CARTESIAN_POINT('Ctrl Pts',(-6.09101724819159,-33.8137964567308,
22.9233095199051));
#30292=CARTESIAN_POINT('Ctrl Pts',(-6.05501274558735,-33.9324447110427,
22.9172529157821));
#30293=CARTESIAN_POINT('Ctrl Pts',(-6.02446420547396,-34.0525714086231,
22.9111963116591));
#30294=CARTESIAN_POINT('Ctrl Pts',(-5.99945759808046,-34.1736311414121,
22.9051397075361));
#30295=CARTESIAN_POINT('Ctrl Pts',(-5.97541304809779,-34.2900334486156,
22.8993161138646));
#30296=CARTESIAN_POINT('Ctrl Pts',(-5.95641431380095,-34.4076737573629,
22.8934925201932));
#30297=CARTESIAN_POINT('Ctrl Pts',(-5.94258432963637,-34.526076928302,22.8876689265217));
#30298=CARTESIAN_POINT('Ctrl Pts',(-5.92877179405107,-34.6443307160538,
22.8818526801787));
#30299=CARTESIAN_POINT('Ctrl Pts',(-5.92011508514747,-34.7633450496746,
22.8760364338357));
#30300=CARTESIAN_POINT('Ctrl Pts',(-5.91668638256212,-34.8826334730583,
22.8702201874927));
#30301=CARTESIAN_POINT('Ctrl Pts',(-5.91326111212698,-35.0018024880719,
22.8644097632444));
#30302=CARTESIAN_POINT('Ctrl Pts',(-5.91505344874563,-35.1212446412101,
22.858599338996));
#30303=CARTESIAN_POINT('Ctrl Pts',(-5.92208383683804,-35.2404678070397,
22.8527889147477));
#30304=CARTESIAN_POINT('Ctrl Pts',(-5.92938033966113,-35.3642038162922,
22.8467585539235));
#30305=CARTESIAN_POINT('Ctrl Pts',(-5.94231932317023,-35.4877034872365,
22.8407281930994));
#30306=CARTESIAN_POINT('Ctrl Pts',(-5.96086422097446,-35.6104155622162,
22.8346978322752));
#30307=CARTESIAN_POINT('Ctrl Pts',(-5.97871264549017,-35.7285190551857,
22.828893948042));
#30308=CARTESIAN_POINT('Ctrl Pts',(-6.0017534391838,-35.8458926032994,22.8230900638088));
#30309=CARTESIAN_POINT('Ctrl Pts',(-6.0299011822913,-35.9620500910181,22.8172861795755));
#30310=CARTESIAN_POINT('Ctrl Pts',(-6.05804476767621,-36.0781904210341,
22.8114831526381));
#30311=CARTESIAN_POINT('Ctrl Pts',(-6.09129370616843,-36.1931146511285,
22.8056801257006));
#30312=CARTESIAN_POINT('Ctrl Pts',(-6.12951174889391,-36.3063482300098,
22.7998770987631));
#30313=CARTESIAN_POINT('Ctrl Pts',(-6.16773316587283,-36.4195918062318,
22.7940735594791));
#30314=CARTESIAN_POINT('Ctrl Pts',(-6.21092442877709,-36.5311440475486,
22.788270020195));
#30315=CARTESIAN_POINT('Ctrl Pts',(-6.25890004806749,-36.6405475152066,
22.782466480911));
#30316=CARTESIAN_POINT('Ctrl Pts',(-6.30689122529183,-36.7499864611335,
22.7766610596068));
#30317=CARTESIAN_POINT('Ctrl Pts',(-6.35966968060255,-36.857274873811,22.7708556383026));
#30318=CARTESIAN_POINT('Ctrl Pts',(-6.41700289212973,-36.9619777585369,
22.7650502169985));
#30319=CARTESIAN_POINT('Ctrl Pts',(-6.47439959488187,-37.0667965920162,
22.7592383667275));
#30320=CARTESIAN_POINT('Ctrl Pts',(-6.53636092581258,-37.1690238239168,
22.7534265164566));
#30321=CARTESIAN_POINT('Ctrl Pts',(-6.60260966410572,-37.2682512880129,
22.7476146661857));
#30322=CARTESIAN_POINT('Ctrl Pts',(-6.66890191492579,-37.3675439252401,
22.7417989986603));
#30323=CARTESIAN_POINT('Ctrl Pts',(-6.73948694036625,-37.4638325422618,
22.735983331135));
#30324=CARTESIAN_POINT('Ctrl Pts',(-6.81404668775415,-37.5567413815616,
22.7301676636096));
#30325=CARTESIAN_POINT('Ctrl Pts',(-6.88871323392924,-37.6497833027415,
22.7243436657685));
#30326=CARTESIAN_POINT('Ctrl Pts',(-6.96736559735218,-37.7394354776297,
22.7185196679274));
#30327=CARTESIAN_POINT('Ctrl Pts',(-7.04964821814089,-37.8253582716676,
22.7126956700862));
#30328=CARTESIAN_POINT('Ctrl Pts',(-7.07147824594466,-37.8481540572764,
22.7111505317134));
#30329=CARTESIAN_POINT('Ctrl Pts',(-7.09356361386344,-37.8706875610459,
22.7096053933405));
#30330=CARTESIAN_POINT('Ctrl Pts',(-7.11589729903294,-37.8929529222361,
22.7080602549676));
#30331=CARTESIAN_POINT('Ctrl Pts',(-7.20007248353159,-37.9768705951097,
22.7022366612962));
#30332=CARTESIAN_POINT('Ctrl Pts',(-7.28804902917364,-38.0572467206924,
22.6964130676248));
#30333=CARTESIAN_POINT('Ctrl Pts',(-7.3794969313009,-38.1337180260736,22.6905894739534));
#30334=CARTESIAN_POINT('Ctrl Pts',(-7.47082945831606,-38.2100928515441,
22.6847732276105));
#30335=CARTESIAN_POINT('Ctrl Pts',(-7.56562432034595,-38.2825723958907,
22.6789569812675));
#30336=CARTESIAN_POINT('Ctrl Pts',(-7.66351422578759,-38.3508296326288,
22.6731407349246));
#30337=CARTESIAN_POINT('Ctrl Pts',(-7.76130614289356,-38.4190185434961,
22.6673303106763));
#30338=CARTESIAN_POINT('Ctrl Pts',(-7.86218660699052,-38.4829933227464,
22.661519886428));
#30339=CARTESIAN_POINT('Ctrl Pts',(-7.96575522545239,-38.5424671060189,
22.6557094621798));
#30340=CARTESIAN_POINT('Ctrl Pts',(-8.07324413034172,-38.6041920950022,
22.6496791013556));
#30341=CARTESIAN_POINT('Ctrl Pts',(-8.18362837108424,-38.6610683238982,
22.6436487405314));
#30342=CARTESIAN_POINT('Ctrl Pts',(-8.29642684731877,-38.7128241964122,
22.6376183797072));
#30343=CARTESIAN_POINT('Ctrl Pts',(-8.4049890572478,-38.7626363222892,22.631814495474));
#30344=CARTESIAN_POINT('Ctrl Pts',(-8.51578703002208,-38.8077055712258,
22.6260106112409));
#30345=CARTESIAN_POINT('Ctrl Pts',(-8.62836736862794,-38.8478369150154,
22.6202067270077));
#30346=CARTESIAN_POINT('Ctrl Pts',(-8.74093107791384,-38.8879623309764,
22.6144037000703));
#30347=CARTESIAN_POINT('Ctrl Pts',(-8.85527624493528,-38.9231511552279,
22.6086006731329));
#30348=CARTESIAN_POINT('Ctrl Pts',(-8.97093128201469,-38.9532572106636,
22.6027976461955));
#30349=CARTESIAN_POINT('Ctrl Pts',(-9.08659653022495,-38.9833659241494,
22.5969941069114));
#30350=CARTESIAN_POINT('Ctrl Pts',(-9.2035714832416,-39.0083908737143,22.5911905676274));
#30351=CARTESIAN_POINT('Ctrl Pts',(-9.32137187388081,-39.0282364461933,
22.5853870283434));
#30352=CARTESIAN_POINT('Ctrl Pts',(-9.43921046581199,-39.0480884543599,
22.5795816070393));
#30353=CARTESIAN_POINT('Ctrl Pts',(-9.55787462526471,-39.0627576772715,
22.5737761857352));
#30354=CARTESIAN_POINT('Ctrl Pts',(-9.67687307520163,-39.0722001412591,
22.5679707644311));
#30355=CARTESIAN_POINT('Ctrl Pts',(-9.79600330490789,-39.0816530619015,
22.5621589141603));
#30356=CARTESIAN_POINT('Ctrl Pts',(-9.91546815674197,-39.0858676376544,
22.5563470638894));
#30357=CARTESIAN_POINT('Ctrl Pts',(-10.034774289896,-39.0848519861511,22.5505352136186));
#30358=CARTESIAN_POINT('Ctrl Pts',(-10.1541587839587,-39.0838356675624,
22.5447195460932));
#30359=CARTESIAN_POINT('Ctrl Pts',(-10.2733839448912,-39.0775823016864,
22.5389038785679));
#30360=CARTESIAN_POINT('Ctrl Pts',(-10.3919611550581,-39.0661519220174,
22.5330882110426));
#30361=CARTESIAN_POINT('Ctrl Pts',(-10.5107082142745,-39.0547051695637,
22.5272642132015));
#30362=CARTESIAN_POINT('Ctrl Pts',(-10.6288050673409,-39.0380666591211,
22.5214402153605));
#30363=CARTESIAN_POINT('Ctrl Pts',(-10.7457727487356,-39.0163475954209,
22.5156162175194));
#30364=CARTESIAN_POINT('Ctrl Pts',(-10.7768049121916,-39.0105854094323,
22.514071079146));
#30365=CARTESIAN_POINT('Ctrl Pts',(-10.8077576788359,-39.0044658909878,
22.5125259407726));
#30366=CARTESIAN_POINT('Ctrl Pts',(-10.8386222972362,-38.9979917011643,
22.5109808023992));
#30367=CARTESIAN_POINT('Ctrl Pts',(-10.9549503876449,-38.9735906173943,
22.5051572087275));
#30368=CARTESIAN_POINT('Ctrl Pts',(-11.0704001978095,-38.9440688376194,
22.4993336150558));
#30369=CARTESIAN_POINT('Ctrl Pts',(-11.1844870002162,-38.9095032352358,
22.4935100213841));
#30370=CARTESIAN_POINT('Ctrl Pts',(-11.2984298651754,-38.8749812424938,
22.4876937750409));
#30371=CARTESIAN_POINT('Ctrl Pts',(-11.411012755344,-38.8354282014154,22.4818775286977));
#30372=CARTESIAN_POINT('Ctrl Pts',(-11.521760819328,-38.7909720400919,22.4760612823544));
#30373=CARTESIAN_POINT('Ctrl Pts',(-11.6323980238884,-38.7465603796313,
22.4702508581059));
#30374=CARTESIAN_POINT('Ctrl Pts',(-11.7412036793262,-38.6972555141252,
22.4644404338573));
#30375=CARTESIAN_POINT('Ctrl Pts',(-11.8477183799131,-38.6432350718189,
22.4586300096088));
#30376=CARTESIAN_POINT('Ctrl Pts',(-11.9582648822223,-38.5871698440405,
22.4525996487847));
#30377=CARTESIAN_POINT('Ctrl Pts',(-12.0663431391598,-38.5260251272257,
22.4465692879606));
#30378=CARTESIAN_POINT('Ctrl Pts',(-12.1714622737272,-38.4600544206384,
22.4405389271365));
#30379=CARTESIAN_POINT('Ctrl Pts',(-12.2726335478099,-38.3965613138407,
22.4347350429031));
#30380=CARTESIAN_POINT('Ctrl Pts',(-12.3710635802308,-38.3285984071227,
22.4289311586696));
#30381=CARTESIAN_POINT('Ctrl Pts',(-12.4663407192961,-38.2564380013048,
22.4231272744361));
#30382=CARTESIAN_POINT('Ctrl Pts',(-12.5616037849091,-38.1842882543505,
22.4173242474984));
#30383=CARTESIAN_POINT('Ctrl Pts',(-12.653714557903,-38.1079424877804,22.4115212205607));
#30384=CARTESIAN_POINT('Ctrl Pts',(-12.7422922727754,-38.0277149949551,
22.405718193623));
#30385=CARTESIAN_POINT('Ctrl Pts',(-12.8308778081336,-37.9474804188814,
22.3999146543387));
#30386=CARTESIAN_POINT('Ctrl Pts',(-12.9159293625085,-37.8633637092838,
22.3941111150545));
#30387=CARTESIAN_POINT('Ctrl Pts',(-12.9971015101761,-37.7757174816072,
22.3883075757702));
#30388=CARTESIAN_POINT('Ctrl Pts',(-13.0782999810252,-37.6880428312805,
22.3825021544657));
#30389=CARTESIAN_POINT('Ctrl Pts',(-13.1556162658785,-37.5968366859967,
22.3766967331613));
#30390=CARTESIAN_POINT('Ctrl Pts',(-13.2287442862499,-37.5024858309306,
22.3708913118569));
#30391=CARTESIAN_POINT('Ctrl Pts',(-13.3019532891348,-37.4080304910262,
22.3650794615857));
#30392=CARTESIAN_POINT('Ctrl Pts',(-13.3709645191656,-37.3104238129581,
22.3592676113146));
#30393=CARTESIAN_POINT('Ctrl Pts',(-13.4355143342349,-37.210082862534,22.3534557610435));
#30394=CARTESIAN_POINT('Ctrl Pts',(-13.5001065459694,-37.1096760076348,
22.3476400935178));
#30395=CARTESIAN_POINT('Ctrl Pts',(-13.5602313018458,-37.0065316557953,
22.3418244259922));
#30396=CARTESIAN_POINT('Ctrl Pts',(-13.615670969756,-36.9010913808819,22.3360087584666));
#30397=CARTESIAN_POINT('Ctrl Pts',(-13.6711900490038,-36.7955000741607,
22.3301847606253));
#30398=CARTESIAN_POINT('Ctrl Pts',(-13.7220104723456,-36.6876066484729,
22.3243607627839));
#30399=CARTESIAN_POINT('Ctrl Pts',(-13.7679626967566,-36.5778726551438,
22.3185367649426));
#30400=CARTESIAN_POINT('Ctrl Pts',(-13.7801540723524,-36.5487596286159,
22.316991626572));
#30401=CARTESIAN_POINT('Ctrl Pts',(-13.7920030629536,-36.5195171306536,
22.3154464882014));
#30402=CARTESIAN_POINT('Ctrl Pts',(-13.8035070969918,-36.4901539394079,
22.3139013498308));
#30403=CARTESIAN_POINT('Ctrl Pts',(-13.852406599943,-36.3653415951289,22.3073335234437));
#30404=CARTESIAN_POINT('Ctrl Pts',(-13.8952013288729,-36.2380114730684,
22.3007656970567));
#30405=CARTESIAN_POINT('Ctrl Pts',(-13.9316569522707,-36.1087373943643,
22.2941978706696));
#30406=CARTESIAN_POINT('Ctrl Pts',(-13.9679980306451,-35.9798694999738,
22.2876506806552));
#30407=CARTESIAN_POINT('Ctrl Pts',(-13.9980396583831,-35.8490700313153,
22.2811034906407));
#30408=CARTESIAN_POINT('Ctrl Pts',(-14.0215963303967,-35.7169295330366,
22.2745563006263));
#30409=CARTESIAN_POINT('Ctrl Pts',(-14.0450149575283,-35.5855633936945,
22.268047477919));
#30410=CARTESIAN_POINT('Ctrl Pts',(-14.0620243166783,-35.4528720959649,
22.2615386552118));
#30411=CARTESIAN_POINT('Ctrl Pts',(-14.0724898512344,-35.319454866284,22.2550298325046));
#30412=CARTESIAN_POINT('Ctrl Pts',(-14.0807516711158,-35.2141311377364,
22.2498915645492));
#30413=CARTESIAN_POINT('Ctrl Pts',(-14.0849362747585,-35.1083554128431,
22.2447532965937));
#30414=CARTESIAN_POINT('Ctrl Pts',(-14.0849992774348,-35.002429682444,22.2396150286382));
#30415=CARTESIAN_POINT('Origin',(-10.,-35.,32.7603849714045));
#30416=CARTESIAN_POINT('',(-7.51282745730979,-31.7594448403263,24.2969436976378));
#30417=CARTESIAN_POINT('',(-7.51282745730979,-31.7594448403263,24.1926554185755));
#30418=CARTESIAN_POINT('',(-7.5128274573098,-31.7594448403263,32.7603849714045));
#30419=CARTESIAN_POINT('',(-14.0849994926668,-34.9979640942378,23.3853849713652));
#30420=CARTESIAN_POINT('Ctrl Pts',(-7.51282745730979,-31.7594448403263,
24.1926554185755));
#30421=CARTESIAN_POINT('Ctrl Pts',(-7.41801607719479,-31.832213933811,24.1868522096254));
#30422=CARTESIAN_POINT('Ctrl Pts',(-7.32640223554429,-31.90914642333,24.1810490006754));
#30423=CARTESIAN_POINT('Ctrl Pts',(-7.23836090041157,-31.9899211831541,
24.1752457917253));
#30424=CARTESIAN_POINT('Ctrl Pts',(-7.15029814958328,-32.070715591109,24.1694411711683));
#30425=CARTESIAN_POINT('Ctrl Pts',(-7.06580993423397,-32.1553538520102,
24.1636365506114));
#30426=CARTESIAN_POINT('Ctrl Pts',(-6.98523507237383,-32.2434772935535,
24.1578319300544));
#30427=CARTESIAN_POINT('Ctrl Pts',(-6.90457409534944,-32.3316949178787,
24.152021105753));
#30428=CARTESIAN_POINT('Ctrl Pts',(-6.82783509921019,-32.4234048588342,
24.1462102814516));
#30429=CARTESIAN_POINT('Ctrl Pts',(-6.75531735975733,-32.5182144403458,
24.1403994571501));
#30430=CARTESIAN_POINT('Ctrl Pts',(-6.68275726123609,-32.6130794020386,
24.1345852386295));
#30431=CARTESIAN_POINT('Ctrl Pts',(-6.61442356434731,-32.7110472762526,
24.1287710201089));
#30432=CARTESIAN_POINT('Ctrl Pts',(-6.55057188569452,-32.811696848186,24.1229568015883));
#30433=CARTESIAN_POINT('Ctrl Pts',(-6.48662276134335,-32.9125000240345,
24.1171337098384));
#30434=CARTESIAN_POINT('Ctrl Pts',(-6.42716951938448,-33.0159927176018,
24.1113106180885));
#30435=CARTESIAN_POINT('Ctrl Pts',(-6.37242173268631,-33.1217292755001,
24.1054875263386));
#30436=CARTESIAN_POINT('Ctrl Pts',(-6.33911654257133,-33.1860529016281,
24.101945115047));
#30437=CARTESIAN_POINT('Ctrl Pts',(-6.30755179619556,-33.2512065136336,
24.0984027037555));
#30438=CARTESIAN_POINT('Ctrl Pts',(-6.2777657820977,-33.317086625201,24.0948602924639));
#30439=CARTESIAN_POINT('Ctrl Pts',(-6.22879867214836,-33.4253911017918,
24.0890366987924));
#30440=CARTESIAN_POINT('Ctrl Pts',(-6.18448346565954,-33.5360091682236,
24.0832131051209));
#30441=CARTESIAN_POINT('Ctrl Pts',(-6.14504422535159,-33.6485041711108,
24.0773895114494));
#30442=CARTESIAN_POINT('Ctrl Pts',(-6.10565474350347,-33.7608572448422,
24.0715732651064));
#30443=CARTESIAN_POINT('Ctrl Pts',(-6.07112912604358,-33.8750821631195,
24.0657570187633));
#30444=CARTESIAN_POINT('Ctrl Pts',(-6.04164439422476,-33.9907201090739,
24.0599407724202));
#30445=CARTESIAN_POINT('Ctrl Pts',(-6.01218917678524,-34.1062423008062,
24.0541303481719));
#30446=CARTESIAN_POINT('Ctrl Pts',(-5.98776490699332,-34.2231743129421,
24.0483199239235));
#30447=CARTESIAN_POINT('Ctrl Pts',(-5.96849937054934,-34.341040460469,24.0425094996752));
#30448=CARTESIAN_POINT('Ctrl Pts',(-5.94850459370308,-34.4633680854682,
24.036479138851));
#30449=CARTESIAN_POINT('Ctrl Pts',(-5.93406695235356,-34.5867015380663,
24.0304487780268));
#30450=CARTESIAN_POINT('Ctrl Pts',(-5.92527156445518,-34.7104949455321,
24.0244184172027));
#30451=CARTESIAN_POINT('Ctrl Pts',(-5.91680649666943,-34.8296391604019,
24.0186145329694));
#30452=CARTESIAN_POINT('Ctrl Pts',(-5.91356755497437,-34.9492089610531,
24.0128106487361));
#30453=CARTESIAN_POINT('Ctrl Pts',(-5.91557791684955,-35.0687113285635,
24.0070067645029));
#30454=CARTESIAN_POINT('Ctrl Pts',(-5.91758798177279,-35.1881960442961,
24.0012037375654));
#30455=CARTESIAN_POINT('Ctrl Pts',(-5.92484580141723,-35.3076129385274,
23.9954007106278));
#30456=CARTESIAN_POINT('Ctrl Pts',(-5.93732242544666,-35.4264691374782,
23.9895976836903));
#30457=CARTESIAN_POINT('Ctrl Pts',(-5.94980015103154,-35.5453358301887,
23.9837941444062));
#30458=CARTESIAN_POINT('Ctrl Pts',(-5.96749755448325,-35.6636413230681,
23.9779906051221));
#30459=CARTESIAN_POINT('Ctrl Pts',(-5.99033389170718,-35.7808986489986,
23.972187065838));
#30460=CARTESIAN_POINT('Ctrl Pts',(-6.01317763448897,-35.8981940001126,
23.9663816445338));
#30461=CARTESIAN_POINT('Ctrl Pts',(-6.04116354730942,-36.0144401076764,
23.9605762232295));
#30462=CARTESIAN_POINT('Ctrl Pts',(-6.07416007869851,-36.1291615970779,
23.9547708019253));
#30463=CARTESIAN_POINT('Ctrl Pts',(-6.10719315069184,-36.2440101299099,
23.9489589516543));
#30464=CARTESIAN_POINT('Ctrl Pts',(-6.1452478041883,-36.3573302817817,23.9431471013834));
#30465=CARTESIAN_POINT('Ctrl Pts',(-6.18814299626949,-36.4686630597624,
23.9373352511124));
#30466=CARTESIAN_POINT('Ctrl Pts',(-6.23106636214315,-36.5800689617095,
23.931519583587));
#30467=CARTESIAN_POINT('Ctrl Pts',(-6.27883643523255,-36.689484516827,23.9257039160616));
#30468=CARTESIAN_POINT('Ctrl Pts',(-6.33122523149382,-36.7964734058628,
23.9198882485362));
#30469=CARTESIAN_POINT('Ctrl Pts',(-6.38368906904874,-36.9036155449295,
23.914064250695));
#30470=CARTESIAN_POINT('Ctrl Pts',(-6.44078463980518,-37.0083237229024,
23.9082402528538));
#30471=CARTESIAN_POINT('Ctrl Pts',(-6.50223944854652,-37.1101886467081,
23.9024162550126));
#30472=CARTESIAN_POINT('Ctrl Pts',(-6.51854374428008,-37.1372139662335,
23.9008711166403));
#30473=CARTESIAN_POINT('Ctrl Pts',(-6.53515464754064,-37.1640393303594,
23.8993259782679));
#30474=CARTESIAN_POINT('Ctrl Pts',(-6.55206659039437,-37.1906574818819,
23.8977808398955));
#30475=CARTESIAN_POINT('Ctrl Pts',(-6.6158073434136,-37.290980728992,23.891957246224));
#30476=CARTESIAN_POINT('Ctrl Pts',(-6.68403312025819,-37.3886814839584,
23.8861336525526));
#30477=CARTESIAN_POINT('Ctrl Pts',(-6.75650153965794,-37.4833329897053,
23.8803100588811));
#30478=CARTESIAN_POINT('Ctrl Pts',(-6.82887852938234,-37.5778650785184,
23.8744938125381));
#30479=CARTESIAN_POINT('Ctrl Pts',(-6.90548726917389,-37.6693552485029,
23.8686775661951));
#30480=CARTESIAN_POINT('Ctrl Pts',(-6.9860410544455,-37.7574039374948,23.8628613198521));
#30481=CARTESIAN_POINT('Ctrl Pts',(-7.06651420493347,-37.8453644892631,
23.8570508956037));
#30482=CARTESIAN_POINT('Ctrl Pts',(-7.15092427078452,-37.9298901137794,
23.8512404713554));
#30483=CARTESIAN_POINT('Ctrl Pts',(-7.23894345024624,-38.0106131815731,
23.8454300471071));
#30484=CARTESIAN_POINT('Ctrl Pts',(-7.33029433770584,-38.0943917844471,
23.8393996862829));
#30485=CARTESIAN_POINT('Ctrl Pts',(-7.42553268961703,-38.1740739175939,
23.8333693254587));
#30486=CARTESIAN_POINT('Ctrl Pts',(-7.52424861234076,-38.2492891632638,
23.8273389646346));
#30487=CARTESIAN_POINT('Ctrl Pts',(-7.61925715398036,-38.3216796206792,
23.8215350804014));
#30488=CARTESIAN_POINT('Ctrl Pts',(-7.7174864152581,-38.3899323876538,23.8157311961681));
#30489=CARTESIAN_POINT('Ctrl Pts',(-7.8185367544231,-38.4537578241963,23.8099273119349));
#30490=CARTESIAN_POINT('Ctrl Pts',(-7.91957216737257,-38.5175738330394,
23.8041242849974));
#30491=CARTESIAN_POINT('Ctrl Pts',(-8.02342748437325,-38.5769635939781,
23.7983212580599));
#30492=CARTESIAN_POINT('Ctrl Pts',(-8.12967461049804,-38.6316811447847,
23.7925182311225));
#30493=CARTESIAN_POINT('Ctrl Pts',(-8.23593111713296,-38.6864035265787,
23.7867146918384));
#30494=CARTESIAN_POINT('Ctrl Pts',(-8.34457948971135,-38.7364526911092,
23.7809111525543));
#30495=CARTESIAN_POINT('Ctrl Pts',(-8.45516818201529,-38.7816292327702,
23.7751076132703));
#30496=CARTESIAN_POINT('Ctrl Pts',(-8.56579273694218,-38.8268204246566,
23.7693021919661));
#30497=CARTESIAN_POINT('Ctrl Pts',(-8.67835848515975,-38.8671356968,23.763496770662));
#30498=CARTESIAN_POINT('Ctrl Pts',(-8.79239572533486,-38.9024244920063,
23.7576913493578));
#30499=CARTESIAN_POINT('Ctrl Pts',(-8.90655925119832,-38.937752366287,23.7518794990869));
#30500=CARTESIAN_POINT('Ctrl Pts',(-9.02219713140498,-38.9680425319197,
23.746067648816));
#30501=CARTESIAN_POINT('Ctrl Pts',(-9.13882623637793,-38.9931948047709,
23.7402557985451));
#30502=CARTESIAN_POINT('Ctrl Pts',(-9.25553194397294,-39.0183635977698,
23.7344401310197));
#30503=CARTESIAN_POINT('Ctrl Pts',(-9.37322977127301,-39.0383877090656,
23.7286244634944));
#30504=CARTESIAN_POINT('Ctrl Pts',(-9.49142982089655,-39.0532186436123,
23.722808795969));
#30505=CARTESIAN_POINT('Ctrl Pts',(-9.6097991793283,-39.0680708218714,23.7169847981279));
#30506=CARTESIAN_POINT('Ctrl Pts',(-9.72867179037029,-39.0777149433081,
23.7111608002867));
#30507=CARTESIAN_POINT('Ctrl Pts',(-9.84755596115319,-39.0821545555038,
23.7053368024456));
#30508=CARTESIAN_POINT('Ctrl Pts',(-9.87909657967911,-39.0833324088188,
23.7037916640728));
#30509=CARTESIAN_POINT('Ctrl Pts',(-9.91063803235721,-39.0841442161781,
23.7022465256999));
#30510=CARTESIAN_POINT('Ctrl Pts',(-9.94217119733299,-39.084590656306,23.700701387327));
#30511=CARTESIAN_POINT('Ctrl Pts',(-10.0610190256045,-39.0862732796548,
23.6948777936556));
#30512=CARTESIAN_POINT('Ctrl Pts',(-10.1801320038195,-39.0827672038154,
23.6890541999841));
#30513=CARTESIAN_POINT('Ctrl Pts',(-10.2990203400898,-39.0740412168034,
23.6832306063127));
#30514=CARTESIAN_POINT('Ctrl Pts',(-10.4177586810645,-39.0653262389201,
23.6774143599696));
#30515=CARTESIAN_POINT('Ctrl Pts',(-10.5362725401565,-39.0514044782802,
23.6715981136266));
#30516=CARTESIAN_POINT('Ctrl Pts',(-10.6540705740894,-39.0322967009026,
23.6657818672836));
#30517=CARTESIAN_POINT('Ctrl Pts',(-10.7717506915403,-39.0132080505157,
23.6599714430353));
#30518=CARTESIAN_POINT('Ctrl Pts',(-10.8887160085574,-38.9889437757082,
23.654161018787));
#30519=CARTESIAN_POINT('Ctrl Pts',(-11.0044793614783,-38.9595765193218,
23.6483505945386));
#30520=CARTESIAN_POINT('Ctrl Pts',(-11.1246245967473,-38.9290976515391,
23.6423202337145));
#30521=CARTESIAN_POINT('Ctrl Pts',(-11.2434746293564,-38.893121885162,23.6362898728903));
#30522=CARTESIAN_POINT('Ctrl Pts',(-11.3604949638244,-38.8517889938843,
23.6302595120661));
#30523=CARTESIAN_POINT('Ctrl Pts',(-11.4731204756289,-38.8120084031377,
23.6244556278329));
#30524=CARTESIAN_POINT('Ctrl Pts',(-11.584050823736,-38.7672659642261,23.6186517435996));
#30525=CARTESIAN_POINT('Ctrl Pts',(-11.692824692563,-38.7177371558852,23.6128478593664));
#30526=CARTESIAN_POINT('Ctrl Pts',(-11.8015824943263,-38.6682156634789,
23.6070448324289));
#30527=CARTESIAN_POINT('Ctrl Pts',(-11.9081840787501,-38.613909376808,23.6012418054915));
#30528=CARTESIAN_POINT('Ctrl Pts',(-12.012189064078,-38.5550415145825,23.595438778554));
#30529=CARTESIAN_POINT('Ctrl Pts',(-12.1162032319582,-38.4961684549405,
23.5896352392699));
#30530=CARTESIAN_POINT('Ctrl Pts',(-12.2176199895532,-38.4327332201492,
23.5838316999859));
#30531=CARTESIAN_POINT('Ctrl Pts',(-12.3160250385777,-38.3650041635459,
23.5780281607018));
#30532=CARTESIAN_POINT('Ctrl Pts',(-12.414461999212,-38.2972531431993,23.5722227393977));
#30533=CARTESIAN_POINT('Ctrl Pts',(-12.5098849727227,-38.2252057631901,
23.5664173180935));
#30534=CARTESIAN_POINT('Ctrl Pts',(-12.601910564254,-38.1491723381903,23.5606118967893));
#30535=CARTESIAN_POINT('Ctrl Pts',(-12.6940380656104,-38.0730547132098,
23.5548000465184));
#30536=CARTESIAN_POINT('Ctrl Pts',(-12.7827603601641,-37.9929424924071,
23.5489881962475));
#30537=CARTESIAN_POINT('Ctrl Pts',(-12.8677288227596,-37.9091848341268,
23.5431763459766));
#30538=CARTESIAN_POINT('Ctrl Pts',(-12.9527530930979,-37.8253721633667,
23.5373606784512));
#30539=CARTESIAN_POINT('Ctrl Pts',(-13.0340183439926,-37.7379095851885,
23.5315450109258));
#30540=CARTESIAN_POINT('Ctrl Pts',(-13.1112154716858,-37.6471802524087,
23.5257293434004));
#30541=CARTESIAN_POINT('Ctrl Pts',(-13.1885231759284,-37.5563209596571,
23.5199053455592));
#30542=CARTESIAN_POINT('Ctrl Pts',(-13.2617508764712,-37.4621858938875,
23.5140813477181));
#30543=CARTESIAN_POINT('Ctrl Pts',(-13.330632012287,-37.3651882374832,23.508257349877));
#30544=CARTESIAN_POINT('Ctrl Pts',(-13.3489065530774,-37.3394542305226,
23.5067122115042));
#30545=CARTESIAN_POINT('Ctrl Pts',(-13.3668754008444,-37.3135188728409,
23.5051670731314));
#30546=CARTESIAN_POINT('Ctrl Pts',(-13.3845341229849,-37.2873901657458,
23.5036219347586));
#30547=CARTESIAN_POINT('Ctrl Pts',(-13.4520539487644,-37.1874845362861,
23.4977139492936));
#30548=CARTESIAN_POINT('Ctrl Pts',(-13.5152498617656,-37.084434171241,23.4918059638286));
#30549=CARTESIAN_POINT('Ctrl Pts',(-13.5738211458681,-36.9786428220743,
23.4858979783636));
#30550=CARTESIAN_POINT('Ctrl Pts',(-13.6323130634339,-36.872994824605,23.4799979984656));
#30551=CARTESIAN_POINT('Ctrl Pts',(-13.6861926320066,-36.7646135732612,
23.4740980185677));
#30552=CARTESIAN_POINT('Ctrl Pts',(-13.7352017518379,-36.6539325479193,
23.4681980386698));
#30553=CARTESIAN_POINT('Ctrl Pts',(-13.7841547944734,-36.5433781659767,
23.4623048096446));
#30554=CARTESIAN_POINT('Ctrl Pts',(-13.8282483207181,-36.4305296035672,
23.4564115806194));
#30555=CARTESIAN_POINT('Ctrl Pts',(-13.8672698330024,-36.3158453703796,
23.4505183515942));
#30556=CARTESIAN_POINT('Ctrl Pts',(-13.9062483904799,-36.201287381379,23.4446316098243));
#30557=CARTESIAN_POINT('Ctrl Pts',(-13.9401659294039,-36.0848981168257,
23.4387448680545));
#30558=CARTESIAN_POINT('Ctrl Pts',(-13.9688580865626,-35.9671558761266,
23.4328581262846));
#30559=CARTESIAN_POINT('Ctrl Pts',(-13.9975315945567,-35.8494901648578,
23.4269752107456));
#30560=CARTESIAN_POINT('Ctrl Pts',(-14.020986387276,-35.7304736079701,23.4210922952066));
#30561=CARTESIAN_POINT('Ctrl Pts',(-14.0391079923918,-35.6105993987847,
23.4152093796675));
#30562=CARTESIAN_POINT('Ctrl Pts',(-14.0572220478134,-35.4907751307399,
23.409328915027));
#30563=CARTESIAN_POINT('Ctrl Pts',(-14.0700072787421,-35.370094309224,23.4034484503864));
#30564=CARTESIAN_POINT('Ctrl Pts',(-14.0774004327815,-35.2490596530013,
23.3975679857458));
#30565=CARTESIAN_POINT('Ctrl Pts',(-14.0825060895164,-35.1654740271091,
23.3935069809654));
#30566=CARTESIAN_POINT('Ctrl Pts',(-14.0850412353373,-35.0817198648656,
23.3894459761849));
#30567=CARTESIAN_POINT('Ctrl Pts',(-14.0849994926672,-34.9979640950489,
23.3853849714045));
#30568=CARTESIAN_POINT('Ctrl Pts',(-14.0849994926668,-34.9979640942378,
23.3853849713652));
#30569=CARTESIAN_POINT('Ctrl Pts',(-14.0849319581215,-34.8624575358837,
23.3788147639339));
#30570=CARTESIAN_POINT('Ctrl Pts',(-14.0781173618785,-34.7271788853858,
23.3722445565027));
#30571=CARTESIAN_POINT('Ctrl Pts',(-14.0646509392799,-34.5927681964646,
23.3656743490714));
#30572=CARTESIAN_POINT('Ctrl Pts',(-14.0514755036666,-34.4612618988816,
23.3592461128904));
#30573=CARTESIAN_POINT('Ctrl Pts',(-14.0319329338457,-34.330586641113,23.3528178767094));
#30574=CARTESIAN_POINT('Ctrl Pts',(-14.006163324473,-34.2013258376235,23.3463896405285));
#30575=CARTESIAN_POINT('Ctrl Pts',(-13.9795400103922,-34.0677828366469,
23.3397484474721));
#30576=CARTESIAN_POINT('Ctrl Pts',(-13.9462701124896,-33.9357499211005,
23.3331072544157));
#30577=CARTESIAN_POINT('Ctrl Pts',(-13.9065621511345,-33.8058487703296,
23.3264660613593));
#30578=CARTESIAN_POINT('Ctrl Pts',(-13.8668541897794,-33.6759476195587,
23.3198248683029));
#30579=CARTESIAN_POINT('Ctrl Pts',(-13.8207083428049,-33.5481784751292,
23.3131836752465));
#30580=CARTESIAN_POINT('Ctrl Pts',(-13.7683854637982,-33.4231372931563,
23.3065424821901));
#30581=CARTESIAN_POINT('Ctrl Pts',(-13.7225040710322,-33.3134899707813,
23.3007188885187));
#30582=CARTESIAN_POINT('Ctrl Pts',(-13.671759167446,-33.2056699869793,23.2948952948472));
#30583=CARTESIAN_POINT('Ctrl Pts',(-13.6163175769508,-33.1001389043836,
23.2890717011758));
#30584=CARTESIAN_POINT('Ctrl Pts',(-13.5609459342572,-32.994740964924,23.2832554548328));
#30585=CARTESIAN_POINT('Ctrl Pts',(-13.500889578707,-32.8916265412277,23.2774392084898));
#30586=CARTESIAN_POINT('Ctrl Pts',(-13.4363636137902,-32.7912378774936,
23.2716229621468));
#30587=CARTESIAN_POINT('Ctrl Pts',(-13.3719022397202,-32.6909497033657,
23.2658125378984));
#30588=CARTESIAN_POINT('Ctrl Pts',(-13.3029803764778,-32.5933822027107,
23.2600021136501));
#30589=CARTESIAN_POINT('Ctrl Pts',(-13.2298590274944,-32.4989530867029,
23.2541916894018));
#30590=CARTESIAN_POINT('Ctrl Pts',(-13.1539698842108,-32.4009496333409,
23.2481613285776));
#30591=CARTESIAN_POINT('Ctrl Pts',(-13.0735572636369,-32.3063272444996,
23.2421309677534));
#30592=CARTESIAN_POINT('Ctrl Pts',(-12.9889626109017,-32.2155202441692,
23.2361006069293));
#30593=CARTESIAN_POINT('Ctrl Pts',(-12.9075449999923,-32.1281235969616,
23.230296722696));
#30594=CARTESIAN_POINT('Ctrl Pts',(-12.822254116813,-32.0442612501225,23.2244928384628));
#30595=CARTESIAN_POINT('Ctrl Pts',(-12.7334349445223,-31.9642861788264,
23.2186889542296));
#30596=CARTESIAN_POINT('Ctrl Pts',(-12.6446288917731,-31.8843229207035,
23.2128859272921));
#30597=CARTESIAN_POINT('Ctrl Pts',(-12.5522958897155,-31.8082460693974,
23.2070829003546));
#30598=CARTESIAN_POINT('Ctrl Pts',(-12.4568163427328,-31.7363703552515,
23.2012798734172));
#30599=CARTESIAN_POINT('Ctrl Pts',(-12.3613283659046,-31.6644882952318,
23.1954763341331));
#30600=CARTESIAN_POINT('Ctrl Pts',(-12.2626936180526,-31.5968083554396,
23.1896727948491));
#30601=CARTESIAN_POINT('Ctrl Pts',(-12.1613234809668,-31.5336033391111,
23.183869255565));
#30602=CARTESIAN_POINT('Ctrl Pts',(-12.0599204707276,-31.4703778261329,
23.1780638342609));
#30603=CARTESIAN_POINT('Ctrl Pts',(-11.9557806534257,-31.4116303385939,
23.1722584129567));
#30604=CARTESIAN_POINT('Ctrl Pts',(-11.849341555226,-31.3575885992774,23.1664529916525));
#30605=CARTESIAN_POINT('Ctrl Pts',(-11.7427845855771,-31.3034870137366,
23.1606411413816));
#30606=CARTESIAN_POINT('Ctrl Pts',(-11.6339236168275,-31.254101763351,23.1548292911107));
#30607=CARTESIAN_POINT('Ctrl Pts',(-11.5232179180481,-31.209613189378,23.1490174408398));
#30608=CARTESIAN_POINT('Ctrl Pts',(-11.4124395071714,-31.1650953950707,
23.1432017733144));
#30609=CARTESIAN_POINT('Ctrl Pts',(-11.2998143375937,-31.1254808174257,
23.137386105789));
#30610=CARTESIAN_POINT('Ctrl Pts',(-11.1858170787973,-31.0908999941633,
23.1315704382637));
#30611=CARTESIAN_POINT('Ctrl Pts',(-11.0716565312373,-31.0562696376056,
23.1257464404226));
#30612=CARTESIAN_POINT('Ctrl Pts',(-10.9561203658598,-31.0266875277412,
23.1199224425814));
#30613=CARTESIAN_POINT('Ctrl Pts',(-10.8396938113801,-31.0022332105124,
23.1140984447403));
#30614=CARTESIAN_POINT('Ctrl Pts',(-10.8088052118552,-30.9957453468553,
23.1125533063674));
#30615=CARTESIAN_POINT('Ctrl Pts',(-10.7778539682478,-30.9896181299179,
23.1110081679946));
#30616=CARTESIAN_POINT('Ctrl Pts',(-10.7468491860047,-30.9838524313262,
23.1094630296217));
#30617=CARTESIAN_POINT('Ctrl Pts',(-10.6299803966585,-30.9621193254829,
23.1036388167762));
#30618=CARTESIAN_POINT('Ctrl Pts',(-10.5119736988937,-30.9454566791178,
23.0978146039308));
#30619=CARTESIAN_POINT('Ctrl Pts',(-10.3933067302598,-30.9339780108892,
23.0919903910854));
#30620=CARTESIAN_POINT('Ctrl Pts',(-10.2747924252673,-30.9225141098305,
23.0861736710204));
#30621=CARTESIAN_POINT('Ctrl Pts',(-10.1556199421272,-30.9162209598722,
23.0803569509554));
#30622=CARTESIAN_POINT('Ctrl Pts',(-10.0362771935465,-30.9151610845434,
23.0745402308903));
#30623=CARTESIAN_POINT('Ctrl Pts',(-9.91707555089145,-30.9141024623673,
23.0687303882744));
#30624=CARTESIAN_POINT('Ctrl Pts',(-9.79770444961418,-30.9182647993533,
23.0629205456584));
#30625=CARTESIAN_POINT('Ctrl Pts',(-9.67865617645128,-30.9276587634302,
23.0571107030424));
#30626=CARTESIAN_POINT('Ctrl Pts',(-9.55968699035048,-30.9370464868367,
23.0513047200656));
#30627=CARTESIAN_POINT('Ctrl Pts',(-9.44104061140693,-30.9516588936954,
23.0454987370889));
#30628=CARTESIAN_POINT('Ctrl Pts',(-9.32320835253115,-30.9714545967662,
23.0396927541121));
#30629=CARTESIAN_POINT('Ctrl Pts',(-9.20542656315506,-30.9912418210109,
23.0338892579336));
#30630=CARTESIAN_POINT('Ctrl Pts',(-9.08845860212028,-31.0162078574589,
23.0280857617551));
#30631=CARTESIAN_POINT('Ctrl Pts',(-8.97278905483393,-31.0462596602545,
23.0222822655766));
#30632=CARTESIAN_POINT('Ctrl Pts',(-8.85714175272616,-31.0763056835883,
23.016479885507));
#30633=CARTESIAN_POINT('Ctrl Pts',(-8.74279276210235,-31.1114354233229,
23.0106775054373));
#30634=CARTESIAN_POINT('Ctrl Pts',(-8.6302142686793,-31.1515052227825,23.0048751253677));
#30635=CARTESIAN_POINT('Ctrl Pts',(-8.51759076243682,-31.1915910435495,
22.9990704253036));
#30636=CARTESIAN_POINT('Ctrl Pts',(-8.40673955371437,-31.2366207361975,
22.9932657252394));
#30637=CARTESIAN_POINT('Ctrl Pts',(-8.2981153940833,-31.2864015041817,22.9874610251753));
#30638=CARTESIAN_POINT('Ctrl Pts',(-8.18946829498385,-31.3361927849686,
22.981655099263));
#30639=CARTESIAN_POINT('Ctrl Pts',(-8.08304954846559,-31.3907369597228,
22.9758491733506));
#30640=CARTESIAN_POINT('Ctrl Pts',(-7.97929057964607,-31.4497945920704,
22.9700432474382));
#30641=CARTESIAN_POINT('Ctrl Pts',(-7.87543494661103,-31.5089072438516,
22.9642319125932));
#30642=CARTESIAN_POINT('Ctrl Pts',(-7.7742443891795,-31.5725415388876,22.9584205777482));
#30643=CARTESIAN_POINT('Ctrl Pts',(-7.67612259938703,-31.6404138905335,
22.9526092429032));
#30644=CARTESIAN_POINT('Ctrl Pts',(-7.62068930273178,-31.6787579546953,
22.9493261653207));
#30645=CARTESIAN_POINT('Ctrl Pts',(-7.56623488510624,-31.7184538738265,
22.9460430877381));
#30646=CARTESIAN_POINT('Ctrl Pts',(-7.5128274573098,-31.7594448403263,22.9427600101556));
#30647=CARTESIAN_POINT('',(-14.0849999165586,-35.0008256610752,23.4896150285502));
#30648=CARTESIAN_POINT('Ctrl Pts',(-14.0849999165586,-35.0008256610752,
23.4896150285502));
#30649=CARTESIAN_POINT('Ctrl Pts',(-14.0850238118884,-34.8826023086252,
23.4838237303793));
#30650=CARTESIAN_POINT('Ctrl Pts',(-14.0799112176567,-34.7641789032605,
23.4780324322084));
#30651=CARTESIAN_POINT('Ctrl Pts',(-14.0696361080072,-34.6460410357058,
23.4722411340375));
#30652=CARTESIAN_POINT('Ctrl Pts',(-14.0593738341097,-34.5280507469535,
23.4664570704042));
#30653=CARTESIAN_POINT('Ctrl Pts',(-14.043961904424,-34.4103456948312,23.4606730067709));
#30654=CARTESIAN_POINT('Ctrl Pts',(-14.023426288869,-34.2934124979611,23.4548889431376));
#30655=CARTESIAN_POINT('Ctrl Pts',(-14.0029108151613,-34.1765939921055,
23.4491105526591));
#30656=CARTESIAN_POINT('Ctrl Pts',(-13.9772817220656,-34.0605462405772,
23.4433321621806));
#30657=CARTESIAN_POINT('Ctrl Pts',(-13.9466168096245,-33.9457510929628,
23.4375537717021));
#30658=CARTESIAN_POINT('Ctrl Pts',(-13.9159728587045,-33.8310344155189,
23.4317793311404));
#30659=CARTESIAN_POINT('Ctrl Pts',(-13.8803000416625,-33.7175690370024,
23.4260048905788));
#30660=CARTESIAN_POINT('Ctrl Pts',(-13.8397271776587,-33.6058263375213,
23.4202304500171));
#30661=CARTESIAN_POINT('Ctrl Pts',(-13.7991689235688,-33.4941238755552,
23.4144580887782));
#30662=CARTESIAN_POINT('Ctrl Pts',(-13.7537142708979,-33.3841432475838,
23.4086857275393));
#30663=CARTESIAN_POINT('Ctrl Pts',(-13.7035416294541,-33.2763398249944,
23.4029133663003));
#30664=CARTESIAN_POINT('Ctrl Pts',(-13.6533748668638,-33.1685490340008,
23.3971416814234));
#30665=CARTESIAN_POINT('Ctrl Pts',(-13.5984913891949,-33.0629353158317,
23.3913699965464));
#30666=CARTESIAN_POINT('Ctrl Pts',(-13.5391171100777,-32.9599325792623,
23.3855983116695));
#30667=CARTESIAN_POINT('Ctrl Pts',(-13.4797353646703,-32.8569168901429,
23.3798259010056));
#30668=CARTESIAN_POINT('Ctrl Pts',(-13.4158619018825,-32.7565131933414,
23.3740534903418));
#30669=CARTESIAN_POINT('Ctrl Pts',(-13.3477674386447,-32.6591287569048,
23.3682810796779));
#30670=CARTESIAN_POINT('Ctrl Pts',(-13.2796050587149,-32.561647190269,23.3625029116732));
#30671=CARTESIAN_POINT('Ctrl Pts',(-13.2072135061458,-32.467191238724,23.3567247436684));
#30672=CARTESIAN_POINT('Ctrl Pts',(-13.1309056247077,-32.3761373951417,
23.3509465756637));
#30673=CARTESIAN_POINT('Ctrl Pts',(-13.0545602420009,-32.285038803434,23.3451655679964));
#30674=CARTESIAN_POINT('Ctrl Pts',(-12.974294975624,-32.197345955219,23.3393845603292));
#30675=CARTESIAN_POINT('Ctrl Pts',(-12.8904603476396,-32.1133992346147,
23.3336035526619));
#30676=CARTESIAN_POINT('Ctrl Pts',(-12.8064891229381,-32.0293157346542,
23.327813125657));
#30677=CARTESIAN_POINT('Ctrl Pts',(-12.7189372206995,-31.9489908384761,
23.3220226986521));
#30678=CARTESIAN_POINT('Ctrl Pts',(-12.6281895523734,-31.8727256793183,
23.3162322716472));
#30679=CARTESIAN_POINT('Ctrl Pts',(-12.539728024013,-31.7983818128125,23.3105877186558));
#30680=CARTESIAN_POINT('Ctrl Pts',(-12.4482301579867,-31.7278957223736,
23.3049431656644));
#30681=CARTESIAN_POINT('Ctrl Pts',(-12.3540776653063,-31.6615058266179,
23.2992986126729));
#30682=CARTESIAN_POINT('Ctrl Pts',(-12.2569387313005,-31.5930100967772,
23.2934750190015));
#30683=CARTESIAN_POINT('Ctrl Pts',(-12.1566511797001,-31.5286470550448,
23.28765142533));
#30684=CARTESIAN_POINT('Ctrl Pts',(-12.0536016281221,-31.4687190209537,
23.2818278316586));
#30685=CARTESIAN_POINT('Ctrl Pts',(-11.9506820888601,-31.4088665949791,
23.2760115853156));
#30686=CARTESIAN_POINT('Ctrl Pts',(-11.8450078304297,-31.3534382509536,
23.2701953389725));
#30687=CARTESIAN_POINT('Ctrl Pts',(-11.7369961000552,-31.3026942852405,
23.2643790926295));
#30688=CARTESIAN_POINT('Ctrl Pts',(-11.6290924900188,-31.2520011145171,
23.2585686683812));
#30689=CARTESIAN_POINT('Ctrl Pts',(-11.5188564302838,-31.2059831663772,
23.2527582441329));
#30690=CARTESIAN_POINT('Ctrl Pts',(-11.406731010566,-31.164855561532,23.2469478198845));
#30691=CARTESIAN_POINT('Ctrl Pts',(-11.2903614117966,-31.1221711917768,
23.2409174590603));
#30692=CARTESIAN_POINT('Ctrl Pts',(-11.1719569820493,-31.0847549248091,
23.2348870982362));
#30693=CARTESIAN_POINT('Ctrl Pts',(-11.0520377807444,-31.0527932017835,
23.228856737412));
#30694=CARTESIAN_POINT('Ctrl Pts',(-10.9366222721191,-31.022031835135,23.2230528531788));
#30695=CARTESIAN_POINT('Ctrl Pts',(-10.8198041478446,-30.9963228131414,
23.2172489689455));
#30696=CARTESIAN_POINT('Ctrl Pts',(-10.7020632302898,-30.9757817876418,
23.2114450847123));
#30697=CARTESIAN_POINT('Ctrl Pts',(-10.5843397043275,-30.9552437962714,
23.2056420577748));
#30698=CARTESIAN_POINT('Ctrl Pts',(-10.4656940583079,-30.9398723534558,
23.1998390308374));
#30699=CARTESIAN_POINT('Ctrl Pts',(-10.3466157934321,-30.9297318894521,
23.1940360038999));
#30700=CARTESIAN_POINT('Ctrl Pts',(-10.2275270151908,-30.9195905301514,
23.1882324646158));
#30701=CARTESIAN_POINT('Ctrl Pts',(-10.1080059490354,-30.9146811025631,
23.1824289253318));
#30702=CARTESIAN_POINT('Ctrl Pts',(-9.98854605372797,-30.9150160579122,
23.1766253860477));
#30703=CARTESIAN_POINT('Ctrl Pts',(-9.86904741896954,-30.9153511218835,
23.1708199647435));
#30704=CARTESIAN_POINT('Ctrl Pts',(-9.74961040263558,-30.9209339499408,
23.1650145434394));
#30705=CARTESIAN_POINT('Ctrl Pts',(-9.63072665119035,-30.9317249117275,
23.1592091221352));
#30706=CARTESIAN_POINT('Ctrl Pts',(-9.51171124699436,-30.9425278235055,
23.1533972718643));
#30707=CARTESIAN_POINT('Ctrl Pts',(-9.39325073757438,-30.9585503445543,
23.1475854215933));
#30708=CARTESIAN_POINT('Ctrl Pts',(-9.27583000575991,-30.9797011529686,
23.1417735713224));
#30709=CARTESIAN_POINT('Ctrl Pts',(-9.15833215137828,-31.0008658533474,
23.135957903797));
#30710=CARTESIAN_POINT('Ctrl Pts',(-9.0418758320683,-31.0271654593759,23.1301422362716));
#30711=CARTESIAN_POINT('Ctrl Pts',(-8.92693250720849,-31.0584582767762,
23.1243265687463));
#30712=CARTESIAN_POINT('Ctrl Pts',(-8.81182453844754,-31.0897959177584,
23.1185025709051));
#30713=CARTESIAN_POINT('Ctrl Pts',(-8.69823427728588,-31.1261409215892,
23.112678573064));
#30714=CARTESIAN_POINT('Ctrl Pts',(-8.58661502727573,-31.1673027879994,
23.1068545752229));
#30715=CARTESIAN_POINT('Ctrl Pts',(-8.55700183183212,-31.1782232555237,
23.1053094368501));
#30716=CARTESIAN_POINT('Ctrl Pts',(-8.52752724292256,-31.1894825129037,
23.1037642984773));
#30717=CARTESIAN_POINT('Ctrl Pts',(-8.49819943683016,-31.2010764592502,
23.1022191601045));
#30718=CARTESIAN_POINT('Ctrl Pts',(-8.38767210566969,-31.2447704179209,
23.0963960166999));
#30719=CARTESIAN_POINT('Ctrl Pts',(-8.27887501034288,-31.2933624204465,
23.0905728732953));
#30720=CARTESIAN_POINT('Ctrl Pts',(-8.17227282463346,-31.3466948700626,
23.0847497298907));
#30721=CARTESIAN_POINT('Ctrl Pts',(-8.06578901651658,-31.399968096062,23.078933052861));
#30722=CARTESIAN_POINT('Ctrl Pts',(-7.96149563547643,-31.4579711253596,
23.0731163758314));
#30723=CARTESIAN_POINT('Ctrl Pts',(-7.85983920555744,-31.5204976255316,
23.0672996988017));
#30724=CARTESIAN_POINT('Ctrl Pts',(-7.75829239057437,-31.5829567041119,
23.0614892938266));
#30725=CARTESIAN_POINT('Ctrl Pts',(-7.6593772139506,-31.6499293338582,23.0556788888515));
#30726=CARTESIAN_POINT('Ctrl Pts',(-7.56351647800449,-31.7211628513992,
23.0498684838764));
#30727=CARTESIAN_POINT('Ctrl Pts',(-7.54652346404085,-31.733790254541,23.0488384866424));
#30728=CARTESIAN_POINT('Ctrl Pts',(-7.52962636762599,-31.746551435824,23.0478084894084));
#30729=CARTESIAN_POINT('Ctrl Pts',(-7.5128274573098,-31.7594448403263,23.0467784921743));
#30730=CARTESIAN_POINT('Ctrl Pts',(-7.51282745730979,-31.7594448403263,
24.2969436976378));
#30731=CARTESIAN_POINT('Ctrl Pts',(-7.44658657932097,-31.8102856638332,
24.2928610902636));
#30732=CARTESIAN_POINT('Ctrl Pts',(-7.38197060909365,-31.8631081695722,
24.2887784828894));
#30733=CARTESIAN_POINT('Ctrl Pts',(-7.31909951636833,-31.9177933883558,
24.2846958755152));
#30734=CARTESIAN_POINT('Ctrl Pts',(-7.22941768704527,-31.9957985612396,
24.2788722818435));
#30735=CARTESIAN_POINT('Ctrl Pts',(-7.14299859653699,-32.0778469307783,
24.2730486881718));
#30736=CARTESIAN_POINT('Ctrl Pts',(-7.0602280293541,-32.1636351150452,24.2672250945002));
#30737=CARTESIAN_POINT('Ctrl Pts',(-6.97756188953619,-32.2493150647749,
24.2614088481569));
#30738=CARTESIAN_POINT('Ctrl Pts',(-6.89853539850233,-32.3387251533123,
24.2555926018137));
#30739=CARTESIAN_POINT('Ctrl Pts',(-6.82350083292988,-32.4315222326049,
24.2497763554704));
#30740=CARTESIAN_POINT('Ctrl Pts',(-6.74854137737154,-32.5242264215092,
24.2439659312219));
#30741=CARTESIAN_POINT('Ctrl Pts',(-6.67756615311754,-32.6203105406969,
24.2381555069733));
#30742=CARTESIAN_POINT('Ctrl Pts',(-6.61088972602085,-32.7193955733602,
24.2323450827247));
#30743=CARTESIAN_POINT('Ctrl Pts',(-6.54168945825155,-32.8222311794476,
24.2263147219007));
#30744=CARTESIAN_POINT('Ctrl Pts',(-6.47712016569874,-32.9282990467605,
24.2202843610766));
#30745=CARTESIAN_POINT('Ctrl Pts',(-6.41748691440709,-33.0371385704651,
24.2142540002525));
#30746=CARTESIAN_POINT('Ctrl Pts',(-6.36009325305609,-33.1418905105289,
24.208450116019));
#30747=CARTESIAN_POINT('Ctrl Pts',(-6.30727177640957,-33.2492092860382,
24.2026462317856));
#30748=CARTESIAN_POINT('Ctrl Pts',(-6.25924920886292,-33.3586564897599,
24.1968423475521));
#30749=CARTESIAN_POINT('Ctrl Pts',(-6.21123373476303,-33.4680875269592,
24.1910393206144));
#30750=CARTESIAN_POINT('Ctrl Pts',(-6.1680159241084,-33.5796459933206,24.1852362936767));
#30751=CARTESIAN_POINT('Ctrl Pts',(-6.12977506487752,-33.6928718687305,
24.179433266739));
#30752=CARTESIAN_POINT('Ctrl Pts',(-6.09153082937867,-33.8061077408011,
24.1736297274547));
#30753=CARTESIAN_POINT('Ctrl Pts',(-6.05826454962939,-33.9210109277316,
24.1678261881704));
#30754=CARTESIAN_POINT('Ctrl Pts',(-6.03010597741508,-34.037105172179,24.1620226488861));
#30755=CARTESIAN_POINT('Ctrl Pts',(-6.00193827370416,-34.153237064636,24.1562172275817));
#30756=CARTESIAN_POINT('Ctrl Pts',(-5.97888166787577,-34.2705603861392,
24.1504118062773));
#30757=CARTESIAN_POINT('Ctrl Pts',(-5.96101490017246,-34.3885882211053,
24.1446063849729));
#30758=CARTESIAN_POINT('Ctrl Pts',(-5.94312834667766,-34.5067467609741,
24.1387945347017));
#30759=CARTESIAN_POINT('Ctrl Pts',(-5.93044316449474,-34.6256109676421,
24.1329826844306));
#30760=CARTESIAN_POINT('Ctrl Pts',(-5.92298628051657,-34.7446881688134,
24.1271708341594));
#30761=CARTESIAN_POINT('Ctrl Pts',(-5.91552449881696,-34.8638435805297,
24.1213551666338));
#30762=CARTESIAN_POINT('Ctrl Pts',(-5.91329786176668,-34.9832118580281,
24.1155394991082));
#30763=CARTESIAN_POINT('Ctrl Pts',(-5.9162811760783,-35.1023013545734,24.1097238315826));
#30764=CARTESIAN_POINT('Ctrl Pts',(-5.91926876366553,-35.221561433963,24.1038998337412));
#30765=CARTESIAN_POINT('Ctrl Pts',(-5.92748116972549,-35.3405415294495,
24.0980758358999));
#30766=CARTESIAN_POINT('Ctrl Pts',(-5.94084147361191,-35.4587559892262,
24.0922518380585));
#30767=CARTESIAN_POINT('Ctrl Pts',(-5.94438603505235,-35.4901189297243,
24.0907066996879));
#30768=CARTESIAN_POINT('Ctrl Pts',(-5.94829266398164,-35.5214280420674,
24.0891615613173));
#30769=CARTESIAN_POINT('Ctrl Pts',(-5.95255932733317,-35.5526744079856,
24.0876164229467));
#30770=CARTESIAN_POINT('Ctrl Pts',(-5.9686402908021,-35.6704412968797,24.0817928292753));
#30771=CARTESIAN_POINT('Ctrl Pts',(-5.98989138186709,-35.7876956583138,
24.0759692356039));
#30772=CARTESIAN_POINT('Ctrl Pts',(-6.01627033365602,-35.9039485303328,
24.0701456419325));
#30773=CARTESIAN_POINT('Ctrl Pts',(-6.04261600447901,-36.020054732086,24.0643293955896));
#30774=CARTESIAN_POINT('Ctrl Pts',(-6.07407657866469,-36.1351615628471,
24.0585131492466));
#30775=CARTESIAN_POINT('Ctrl Pts',(-6.11055816232707,-36.2487862873044,
24.0526969029036));
#30776=CARTESIAN_POINT('Ctrl Pts',(-6.1470032277229,-36.3622972727855,24.0468864786554));
#30777=CARTESIAN_POINT('Ctrl Pts',(-6.18845917976378,-36.4743287168403,
24.0410760544071));
#30778=CARTESIAN_POINT('Ctrl Pts',(-6.23478145327106,-36.5844097624568,
24.0352656301588));
#30779=CARTESIAN_POINT('Ctrl Pts',(-6.28285712064225,-36.6986576033384,
24.0292352693346));
#30780=CARTESIAN_POINT('Ctrl Pts',(-6.33617468997626,-36.8108040380477,
24.0232049085104));
#30781=CARTESIAN_POINT('Ctrl Pts',(-6.39451615077476,-36.9203414313543,
24.0171745476863));
#30782=CARTESIAN_POINT('Ctrl Pts',(-6.4506665361896,-37.0257650317805,24.0113706634531));
#30783=CARTESIAN_POINT('Ctrl Pts',(-6.51147005382736,-37.128771634547,24.0055667792199));
#30784=CARTESIAN_POINT('Ctrl Pts',(-6.57668431458383,-37.2289312950344,
23.9997628949867));
#30785=CARTESIAN_POINT('Ctrl Pts',(-6.64188894249658,-37.3290761608688,
23.9939598680493));
#30786=CARTESIAN_POINT('Ctrl Pts',(-6.71150279512863,-37.4263745786108,
23.9881568411119));
#30787=CARTESIAN_POINT('Ctrl Pts',(-6.78523940407023,-37.5204244306976,
23.9823538141745));
#30788=CARTESIAN_POINT('Ctrl Pts',(-6.8589825231833,-37.6144825864027,23.9765502748905));
#30789=CARTESIAN_POINT('Ctrl Pts',(-6.93684887036415,-37.7052912848328,
23.9707467356065));
#30790=CARTESIAN_POINT('Ctrl Pts',(-7.01851124291595,-37.7924809384097,
23.9649431963225));
#30791=CARTESIAN_POINT('Ctrl Pts',(-7.10020009762288,-37.8796988665745,
23.9591377750184));
#30792=CARTESIAN_POINT('Ctrl Pts',(-7.1856871469023,-37.9632951179562,23.9533323537143));
#30793=CARTESIAN_POINT('Ctrl Pts',(-7.27460831114308,-38.0429369271001,
23.9475269324102));
#30794=CARTESIAN_POINT('Ctrl Pts',(-7.36362794734274,-38.1226669321761,
23.9417150821393));
#30795=CARTESIAN_POINT('Ctrl Pts',(-7.45608898519387,-38.1984334812067,
23.9359032318685));
#30796=CARTESIAN_POINT('Ctrl Pts',(-7.55159412814588,-38.2699439883078,
23.9300913815976));
#30797=CARTESIAN_POINT('Ctrl Pts',(-7.64716199938854,-38.3415014638939,
23.9242757140723));
#30798=CARTESIAN_POINT('Ctrl Pts',(-7.74577762104494,-38.4087971008214,
23.918460046547));
#30799=CARTESIAN_POINT('Ctrl Pts',(-7.84701598392944,-38.4715824671963,
23.9126443790216));
#30800=CARTESIAN_POINT('Ctrl Pts',(-7.94839935983691,-38.5344577668288,
23.9068203811806));
#30801=CARTESIAN_POINT('Ctrl Pts',(-8.05241262046843,-38.5928097020728,
23.9009963833395));
#30802=CARTESIAN_POINT('Ctrl Pts',(-8.1586074155696,-38.6464363905058,23.8951723854985));
#30803=CARTESIAN_POINT('Ctrl Pts',(-8.1867814735695,-38.660663843262,23.8936272471251));
#30804=CARTESIAN_POINT('Ctrl Pts',(-8.21510898346397,-38.6745589665825,
23.8920821087517));
#30805=CARTESIAN_POINT('Ctrl Pts',(-8.24358137181638,-38.688118572195,23.8905369703783));
#30806=CARTESIAN_POINT('Ctrl Pts',(-8.35089319804208,-38.7392244373991,
23.8847133767068));
#30807=CARTESIAN_POINT('Ctrl Pts',(-8.46061043672435,-38.7857252081772,
23.8788897830354));
#30808=CARTESIAN_POINT('Ctrl Pts',(-8.57230096503302,-38.8273882041876,
23.8730661893639));
#30809=CARTESIAN_POINT('Ctrl Pts',(-8.68385057915002,-38.86899863614,23.8672499430209));
#30810=CARTESIAN_POINT('Ctrl Pts',(-8.79736815192777,-38.90578329173,23.8614336966779));
#30811=CARTESIAN_POINT('Ctrl Pts',(-8.91239846827213,-38.9375560831794,
23.8556174503349));
#30812=CARTESIAN_POINT('Ctrl Pts',(-9.0273136386351,-38.9692970698893,23.8498070260865));
#30813=CARTESIAN_POINT('Ctrl Pts',(-9.14373814878656,-38.9960360648753,
23.8439966018382));
#30814=CARTESIAN_POINT('Ctrl Pts',(-9.26119894214271,-39.0176358716177,
23.8381861775899));
#30815=CARTESIAN_POINT('Ctrl Pts',(-9.38310586947834,-39.0400532757214,
23.8321558167657));
#30816=CARTESIAN_POINT('Ctrl Pts',(-9.50612866105545,-39.0569345899521,
23.8261254559415));
#30817=CARTESIAN_POINT('Ctrl Pts',(-9.62972324000022,-39.0681838848562,
23.8200950951174));
#30818=CARTESIAN_POINT('Ctrl Pts',(-9.74867609356334,-39.0790107005698,
23.8142912108841));
#30819=CARTESIAN_POINT('Ctrl Pts',(-9.86815811762749,-39.0846208606733,
23.8084873266509));
#30820=CARTESIAN_POINT('Ctrl Pts',(-9.9876768500406,-39.0849814124394,23.8026834424177));
#30821=CARTESIAN_POINT('Ctrl Pts',(-10.1071779282588,-39.085341910948,23.7968804154802));
#30822=CARTESIAN_POINT('Ctrl Pts',(-10.2267152958181,-39.0804543419597,
23.7910773885428));
#30823=CARTESIAN_POINT('Ctrl Pts',(-10.3457956016437,-39.070337873185,23.7852743616053));
#30824=CARTESIAN_POINT('Ctrl Pts',(-10.4648864210151,-39.0602205112318,
23.7794708223212));
#30825=CARTESIAN_POINT('Ctrl Pts',(-10.5835196915284,-39.0448733661736,
23.7736672830372));
#30826=CARTESIAN_POINT('Ctrl Pts',(-10.7012069401969,-39.0243675064561,
23.7678637437531));
#30827=CARTESIAN_POINT('Ctrl Pts',(-10.8189323534677,-39.0038549969274,
23.762058322449));
#30828=CARTESIAN_POINT('Ctrl Pts',(-10.9357107327008,-38.9781805157537,
23.7562529011448));
#30829=CARTESIAN_POINT('Ctrl Pts',(-11.0510641872897,-38.9474661587146,
23.7504474798406));
#30830=CARTESIAN_POINT('Ctrl Pts',(-11.1665453851525,-38.916717788368,23.7446356295697));
#30831=CARTESIAN_POINT('Ctrl Pts',(-11.2805981137806,-38.8809185067376,
23.7388237792988));
#30832=CARTESIAN_POINT('Ctrl Pts',(-11.3927598792847,-38.8402402162697,
23.7330119290279));
#30833=CARTESIAN_POINT('Ctrl Pts',(-11.5049953132385,-38.7995352080822,
23.7271962615025));
#30834=CARTESIAN_POINT('Ctrl Pts',(-11.6153369340792,-38.7539449646672,
23.7213805939771));
#30835=CARTESIAN_POINT('Ctrl Pts',(-11.7233439859836,-38.7036887701283,
23.7155649264518));
#30836=CARTESIAN_POINT('Ctrl Pts',(-11.8315057463271,-38.6533605890174,
23.7097409286107));
#30837=CARTESIAN_POINT('Ctrl Pts',(-11.937325902232,-38.5983533046048,23.7039169307695));
#30838=CARTESIAN_POINT('Ctrl Pts',(-12.0403898357863,-38.5389312395157,
23.6980929329284));
#30839=CARTESIAN_POINT('Ctrl Pts',(-12.0677332591422,-38.523166241748,23.6965477945556));
#30840=CARTESIAN_POINT('Ctrl Pts',(-12.094882848487,-38.5070907303515,23.6950026561827));
#30841=CARTESIAN_POINT('Ctrl Pts',(-12.1218312375957,-38.4907101282065,
23.6934575178098));
#30842=CARTESIAN_POINT('Ctrl Pts',(-12.2233991431152,-38.4289719870394,
23.6876339241383));
#30843=CARTESIAN_POINT('Ctrl Pts',(-12.3224340400302,-38.3626976832686,
23.6818103304668));
#30844=CARTESIAN_POINT('Ctrl Pts',(-12.4185044472203,-38.292121085072,23.6759867367953));
#30845=CARTESIAN_POINT('Ctrl Pts',(-12.5144536473216,-38.2216335297374,
23.6701704904523));
#30846=CARTESIAN_POINT('Ctrl Pts',(-12.6074454705769,-38.1468547157318,
23.6643542441092));
#30847=CARTESIAN_POINT('Ctrl Pts',(-12.6970747462037,-38.0680633652828,
23.6585379977662));
#30848=CARTESIAN_POINT('Ctrl Pts',(-12.7866143024312,-37.9893508854102,
23.6527275735178));
#30849=CARTESIAN_POINT('Ctrl Pts',(-12.8727977022076,-37.9066341276154,
23.6469171492694));
#30850=CARTESIAN_POINT('Ctrl Pts',(-12.9552508859334,-37.8202335366401,
23.641106725021));
#30851=CARTESIAN_POINT('Ctrl Pts',(-13.040825093205,-37.7305625045902,23.6350763641969));
#30852=CARTESIAN_POINT('Ctrl Pts',(-13.1223807507815,-37.6369235130602,
23.6290460033727));
#30853=CARTESIAN_POINT('Ctrl Pts',(-13.1995393829107,-37.5397190272161,
23.6230156425486));
#30854=CARTESIAN_POINT('Ctrl Pts',(-13.2738002408485,-37.4461651588414,
23.6172117583153));
#30855=CARTESIAN_POINT('Ctrl Pts',(-13.3439881105524,-37.3493091269306,
23.611407874082));
#30856=CARTESIAN_POINT('Ctrl Pts',(-13.4098054814972,-37.249544749133,23.6056039898487));
#30857=CARTESIAN_POINT('Ctrl Pts',(-13.4756131305124,-37.1497951076009,
23.5998009629112));
#30858=CARTESIAN_POINT('Ctrl Pts',(-13.5370513397981,-37.0471383152607,
23.5939979359737));
#30859=CARTESIAN_POINT('Ctrl Pts',(-13.5938657035847,-36.9419975037567,
23.5881949090362));
#30860=CARTESIAN_POINT('Ctrl Pts',(-13.6506850834855,-36.8368474094186,
23.5823913697521));
#30861=CARTESIAN_POINT('Ctrl Pts',(-13.7028796120812,-36.7292132191305,
23.576587830468));
#30862=CARTESIAN_POINT('Ctrl Pts',(-13.7502409658695,-36.6195424347372,
23.5707842911839));
#30863=CARTESIAN_POINT('Ctrl Pts',(-13.7976176783925,-36.5098360853874,
23.5649788698797));
#30864=CARTESIAN_POINT('Ctrl Pts',(-13.8401579372119,-36.3980922031405,
23.5591734485755));
#30865=CARTESIAN_POINT('Ctrl Pts',(-13.8777018974908,-36.2847774103697,
23.5533680272713));
#30866=CARTESIAN_POINT('Ctrl Pts',(-13.9152874342306,-36.1713371319542,
23.5475561770003));
#30867=CARTESIAN_POINT('Ctrl Pts',(-13.9478654997089,-36.0563228583936,
23.5417443267294));
#30868=CARTESIAN_POINT('Ctrl Pts',(-13.975326345867,-35.9402156368918,23.5359324764584));
#30869=CARTESIAN_POINT('Ctrl Pts',(-14.0028052284563,-35.8240321555435,
23.530116808933));
#30870=CARTESIAN_POINT('Ctrl Pts',(-14.0251601218921,-35.7067546968224,
23.5243011414076));
#30871=CARTESIAN_POINT('Ctrl Pts',(-14.0423328227829,-35.5888720997399,
23.5184854738822));
#30872=CARTESIAN_POINT('Ctrl Pts',(-14.0595301217134,-35.4708206485661,
23.512661476041));
#30873=CARTESIAN_POINT('Ctrl Pts',(-14.0715303713908,-35.3521627337771,
23.5068374781998));
#30874=CARTESIAN_POINT('Ctrl Pts',(-14.0783273651944,-35.2333900218666,
23.5010134803587));
#30875=CARTESIAN_POINT('Ctrl Pts',(-14.0801306446992,-35.2018789739962,
23.4994683419862));
#30876=CARTESIAN_POINT('Ctrl Pts',(-14.0815679668199,-35.1703598310385,
23.4979232036138));
#30877=CARTESIAN_POINT('Ctrl Pts',(-14.0826398292009,-35.1388417265166,
23.4963780652414));
#30878=CARTESIAN_POINT('Ctrl Pts',(-14.0842036685506,-35.0928570432686,
23.4941237196927));
#30879=CARTESIAN_POINT('Ctrl Pts',(-14.0849906149495,-35.0468457909019,
23.4918693741441));
#30880=CARTESIAN_POINT('Ctrl Pts',(-14.0849999165584,-35.0008256619994,
23.4896150285955));
#30881=CARTESIAN_POINT('Origin',(-10.,-35.,32.7603849714045));
#30882=CARTESIAN_POINT('',(-7.5128274573098,-31.7594448403263,25.5469376127646));
#30883=CARTESIAN_POINT('',(-7.5128274573098,-31.7594448403263,25.442544535095));
#30884=CARTESIAN_POINT('',(-7.5128274573098,-31.7594448403263,32.7603849714045));
#30885=CARTESIAN_POINT('',(-14.0849984277889,-35.0035839868969,24.6353849714293));
#30886=CARTESIAN_POINT('Ctrl Pts',(-7.5128274573098,-31.7594448403263,25.442544535095));
#30887=CARTESIAN_POINT('Ctrl Pts',(-7.41827395874041,-31.8320160060276,
25.4367332032128));
#30888=CARTESIAN_POINT('Ctrl Pts',(-7.32679695411755,-31.908807538792,25.4309218713305));
#30889=CARTESIAN_POINT('Ctrl Pts',(-7.23879181561765,-31.9895258907441,
25.4251105394482));
#30890=CARTESIAN_POINT('Ctrl Pts',(-7.15085584740807,-32.0701807996754,
25.4193037751573));
#30891=CARTESIAN_POINT('Ctrl Pts',(-7.06638661541144,-32.1547561116215,
25.4134970108664));
#30892=CARTESIAN_POINT('Ctrl Pts',(-6.98574673250876,-32.2429178032894,
25.4076902465755));
#30893=CARTESIAN_POINT('Ctrl Pts',(-6.90514184249712,-32.3310412380507,
25.4018860020734));
#30894=CARTESIAN_POINT('Ctrl Pts',(-6.82836327281571,-32.4227476575573,
25.3960817575712));
#30895=CARTESIAN_POINT('Ctrl Pts',(-6.75573670076481,-32.517666290517,25.3902775130691));
#30896=CARTESIAN_POINT('Ctrl Pts',(-6.68312451340452,-32.6125661235371,
25.3844744181774));
#30897=CARTESIAN_POINT('Ctrl Pts',(-6.61466293637587,-32.7106765806863,
25.3786713232856));
#30898=CARTESIAN_POINT('Ctrl Pts',(-6.55063685704201,-32.811594437038,25.3728682283939));
#30899=CARTESIAN_POINT('Ctrl Pts',(-6.48660834875909,-32.9125161218974,
25.3670649133509));
#30900=CARTESIAN_POINT('Ctrl Pts',(-6.42701589139308,-33.0162450728324,
25.3612615983078));
#30901=CARTESIAN_POINT('Ctrl Pts',(-6.37210024043593,-33.1223503163383,
25.3554582832648));
#30902=CARTESIAN_POINT('Ctrl Pts',(-6.31716954611168,-33.2284846258773,
25.3496533784856));
#30903=CARTESIAN_POINT('Ctrl Pts',(-6.2669183936464,-33.3369961600095,25.3438484737064));
#30904=CARTESIAN_POINT('Ctrl Pts',(-6.22154062098647,-33.447431250751,25.3380435689272));
#30905=CARTESIAN_POINT('Ctrl Pts',(-6.17611367088984,-33.557986023759,25.3322323731751));
#30906=CARTESIAN_POINT('Ctrl Pts',(-6.13557080051017,-33.6704681372962,
25.326421177423));
#30907=CARTESIAN_POINT('Ctrl Pts',(-6.10005697200426,-33.7844057509237,
25.3206099816709));
#30908=CARTESIAN_POINT('Ctrl Pts',(-6.06452142162713,-33.8984130539729,
25.3147952315274));
#30909=CARTESIAN_POINT('Ctrl Pts',(-6.03402114392668,-34.0138772360793,
25.3089804813839));
#30910=CARTESIAN_POINT('Ctrl Pts',(-6.00865026741219,-34.1303148200807,
25.3031657312405));
#30911=CARTESIAN_POINT('Ctrl Pts',(-5.98324158955583,-34.2469258902807,
25.297342317409));
#30912=CARTESIAN_POINT('Ctrl Pts',(-5.9629776421869,-34.3645128566708,25.2915189035776));
#30913=CARTESIAN_POINT('Ctrl Pts',(-5.94790090175037,-34.4825853713273,
25.2856954897461));
#30914=CARTESIAN_POINT('Ctrl Pts',(-5.9406875692008,-34.5390761172393,25.2829093291223));
#30915=CARTESIAN_POINT('Ctrl Pts',(-5.93466085033665,-34.5956779772144,
25.2801231684984));
#30916=CARTESIAN_POINT('Ctrl Pts',(-5.92982117855723,-34.6523372877647,
25.2773370078746));
#30917=CARTESIAN_POINT('Ctrl Pts',(-5.91970536480497,-34.7707657802292,
25.2715134142015));
#30918=CARTESIAN_POINT('Ctrl Pts',(-5.91474633401457,-34.8898271180746,
25.2656898205283));
#30919=CARTESIAN_POINT('Ctrl Pts',(-5.91500999150824,-35.0090349611213,
25.2598662268552));
#30920=CARTESIAN_POINT('Ctrl Pts',(-5.91527331635881,-35.1280924057676,
25.2540499805105));
#30921=CARTESIAN_POINT('Ctrl Pts',(-5.9207462228401,-35.2472955832397,25.2482337341658));
#30922=CARTESIAN_POINT('Ctrl Pts',(-5.93144287956194,-35.3661529157781,
25.2424174878211));
#30923=CARTESIAN_POINT('Ctrl Pts',(-5.94212882887143,-35.4848912714712,
25.236607063571));
#30924=CARTESIAN_POINT('Ctrl Pts',(-5.95802808957765,-35.6032840665822,
25.230796639321));
#30925=CARTESIAN_POINT('Ctrl Pts',(-5.97910278763899,-35.7208402094968,
25.2249862150709));
#30926=CARTESIAN_POINT('Ctrl Pts',(-6.0009752066032,-35.84284609552,25.2189558542474));
#30927=CARTESIAN_POINT('Ctrl Pts',(-6.02842260533274,-35.9639502916357,
25.2129254934239));
#30928=CARTESIAN_POINT('Ctrl Pts',(-6.06134350857702,-36.0836097279794,
25.2068951326003));
#30929=CARTESIAN_POINT('Ctrl Pts',(-6.09302803242764,-36.1987752274389,
25.2010912483653));
#30930=CARTESIAN_POINT('Ctrl Pts',(-6.12978223035001,-36.3126020999863,
25.1952873641303));
#30931=CARTESIAN_POINT('Ctrl Pts',(-6.17146381683887,-36.4246177361756,
25.1894834798954));
#30932=CARTESIAN_POINT('Ctrl Pts',(-6.21313924651174,-36.5366168264576,
25.1836804529561));
#30933=CARTESIAN_POINT('Ctrl Pts',(-6.25974047496469,-36.6468048298346,
25.1778774260169));
#30934=CARTESIAN_POINT('Ctrl Pts',(-6.31107611100897,-36.7547266286323,
25.1720743990777));
#30935=CARTESIAN_POINT('Ctrl Pts',(-6.36241627945318,-36.8626579557965,
25.1662708597918));
#30936=CARTESIAN_POINT('Ctrl Pts',(-6.41849151115981,-36.9683223118065,
25.160467320506));
#30937=CARTESIAN_POINT('Ctrl Pts',(-6.47906354243825,-37.0712873923752,
25.1546637812202));
#30938=CARTESIAN_POINT('Ctrl Pts',(-6.53965521652011,-37.1742858633189,
25.1488583599142));
#30939=CARTESIAN_POINT('Ctrl Pts',(-6.60474638338353,-37.2745829661884,
25.1430529386083));
#30940=CARTESIAN_POINT('Ctrl Pts',(-6.67405472993515,-37.3717742431634,
25.1372475173023));
#30941=CARTESIAN_POINT('Ctrl Pts',(-6.74343982906545,-37.4690731504816,
25.1314356670296));
#30942=CARTESIAN_POINT('Ctrl Pts',(-6.8170511926523,-37.5632590338801,25.1256238167569));
#30943=CARTESIAN_POINT('Ctrl Pts',(-6.89456529351481,-37.6539593598541,
25.1198119664842));
#30944=CARTESIAN_POINT('Ctrl Pts',(-6.97213030605494,-37.7447192582891,
25.113996298957));
#30945=CARTESIAN_POINT('Ctrl Pts',(-7.05360288281086,-37.8319887422407,
25.1081806314299));
#30946=CARTESIAN_POINT('Ctrl Pts',(-7.13862278213925,-37.9154322864899,
25.1023649639027));
#30947=CARTESIAN_POINT('Ctrl Pts',(-7.22376446329271,-37.9989953546056,
25.0965409660598));
#30948=CARTESIAN_POINT('Ctrl Pts',(-7.31246330611885,-38.0787212727478,
25.0907169682169));
#30949=CARTESIAN_POINT('Ctrl Pts',(-7.40432609491705,-38.1543148191757,
25.084892970374));
#30950=CARTESIAN_POINT('Ctrl Pts',(-7.42869779323927,-38.1743701988648,
25.083347832018));
#30951=CARTESIAN_POINT('Ctrl Pts',(-7.45329203647413,-38.1941349514844,
25.0818026936621));
#30952=CARTESIAN_POINT('Ctrl Pts',(-7.47810115818965,-38.2136040875745,
25.0802575553061));
#30953=CARTESIAN_POINT('Ctrl Pts',(-7.57160621141045,-38.2869828483039,
25.0744339616351));
#30954=CARTESIAN_POINT('Ctrl Pts',(-7.66846731883909,-38.3563955273518,
25.0686103679641));
#30955=CARTESIAN_POINT('Ctrl Pts',(-7.76831384647973,-38.4215204094358,
25.062786774293));
#30956=CARTESIAN_POINT('Ctrl Pts',(-7.86803440289478,-38.4865631268076,
25.0569705279504));
#30957=CARTESIAN_POINT('Ctrl Pts',(-7.97073254893948,-38.5473285858543,
25.0511542816078));
#30958=CARTESIAN_POINT('Ctrl Pts',(-8.07600490987609,-38.6035354713363,
25.0453380352652));
#30959=CARTESIAN_POINT('Ctrl Pts',(-8.18117189259851,-38.6596860934158,
25.0395276110173));
#30960=CARTESIAN_POINT('Ctrl Pts',(-8.28890760584245,-38.7112870285497,
25.0337171867694));
#30961=CARTESIAN_POINT('Ctrl Pts',(-8.39878055358211,-38.7581007549576,
25.0279067625215));
#30962=CARTESIAN_POINT('Ctrl Pts',(-8.51281241966153,-38.8066864777424,
25.0218764016972));
#30963=CARTESIAN_POINT('Ctrl Pts',(-8.62914613917075,-38.8501151747488,
25.0158460408728));
#30964=CARTESIAN_POINT('Ctrl Pts',(-8.74727187910843,-38.8881740258285,
25.0098156800485));
#30965=CARTESIAN_POINT('Ctrl Pts',(-8.86096128169724,-38.9248035364225,
25.0040117958157));
#30966=CARTESIAN_POINT('Ctrl Pts',(-8.97631010603435,-38.9564591313934,
24.9982079115829));
#30967=CARTESIAN_POINT('Ctrl Pts',(-9.09284507948462,-38.9830007469475,
24.9924040273501));
#30968=CARTESIAN_POINT('Ctrl Pts',(-9.20936283947303,-39.0095384420213,
24.9866010004131));
#30969=CARTESIAN_POINT('Ctrl Pts',(-9.32706600210986,-39.0309635692546,
24.980797973476));
#30970=CARTESIAN_POINT('Ctrl Pts',(-9.44546900642645,-39.0471867237831,
24.974994946539));
#30971=CARTESIAN_POINT('Ctrl Pts',(-9.56388246449013,-39.0634113106466,
24.9691914072554));
#30972=CARTESIAN_POINT('Ctrl Pts',(-9.68299548250737,-39.0744329562123,
24.9633878679718));
#30973=CARTESIAN_POINT('Ctrl Pts',(-9.80231588616976,-39.080213963892,24.9575843286881));
#30974=CARTESIAN_POINT('Ctrl Pts',(-9.92167498404754,-39.085996846285,24.9517789073844));
#30975=CARTESIAN_POINT('Ctrl Pts',(-10.0412411936723,-39.0865356911639,
24.9459734860807));
#30976=CARTESIAN_POINT('Ctrl Pts',(-10.1605214844387,-39.0818449080083,
24.9401680647769));
#30977=CARTESIAN_POINT('Ctrl Pts',(-10.2799338670867,-39.0771489302446,
24.9343562145064));
#30978=CARTESIAN_POINT('Ctrl Pts',(-10.3990592905948,-39.0672117805131,
24.9285443642359));
#30979=CARTESIAN_POINT('Ctrl Pts',(-10.5174088328726,-39.0520998383141,
24.9227325139655));
#30980=CARTESIAN_POINT('Ctrl Pts',(-10.6358361077652,-39.0369779705104,
24.9169168464405));
#30981=CARTESIAN_POINT('Ctrl Pts',(-10.7534860850764,-39.016674610663,24.9111011789156));
#30982=CARTESIAN_POINT('Ctrl Pts',(-10.8698806698468,-38.9913071317836,
24.9052855113906));
#30983=CARTESIAN_POINT('Ctrl Pts',(-10.9864419772915,-38.96590331673,24.8994615135499));
#30984=CARTESIAN_POINT('Ctrl Pts',(-11.1017439096846,-38.9354210084424,
24.8936375157092));
#30985=CARTESIAN_POINT('Ctrl Pts',(-11.215324005556,-38.9000272513816,24.8878135178685));
#30986=CARTESIAN_POINT('Ctrl Pts',(-11.2454574241779,-38.8906370946827,
24.8862683794916));
#30987=CARTESIAN_POINT('Ctrl Pts',(-11.2754697617168,-38.8809014966569,
24.8847232411146));
#30988=CARTESIAN_POINT('Ctrl Pts',(-11.3053526426733,-38.8708241342466,
24.8831781027377));
#30989=CARTESIAN_POINT('Ctrl Pts',(-11.4179805852676,-38.8328427697088,
24.8773545090664));
#30990=CARTESIAN_POINT('Ctrl Pts',(-11.529131078261,-38.7898804367481,24.8715309153951));
#30991=CARTESIAN_POINT('Ctrl Pts',(-11.6383318802172,-38.7420707703441,
24.8657073217238));
#30992=CARTESIAN_POINT('Ctrl Pts',(-11.7473949091413,-38.6943214229359,
24.859891075381));
#30993=CARTESIAN_POINT('Ctrl Pts',(-11.8545127688016,-38.6417370682555,
24.8540748290381));
#30994=CARTESIAN_POINT('Ctrl Pts',(-11.9592290599098,-38.5845008705265,
24.8482585826953));
#30995=CARTESIAN_POINT('Ctrl Pts',(-12.0638405294327,-38.5273219665473,
24.8424481584471));
#30996=CARTESIAN_POINT('Ctrl Pts',(-12.1660548565831,-38.4655006778096,
24.836637734199));
#30997=CARTESIAN_POINT('Ctrl Pts',(-12.2654368545928,-38.3992676943502,
24.8308273099508));
#30998=CARTESIAN_POINT('Ctrl Pts',(-12.3685806667888,-38.3305276554705,
24.8247969491266));
#30999=CARTESIAN_POINT('Ctrl Pts',(-12.4686730836362,-38.2570355191049,
24.8187665883024));
#31000=CARTESIAN_POINT('Ctrl Pts',(-12.5652566366224,-38.179101034611,24.8127362274781));
#31001=CARTESIAN_POINT('Ctrl Pts',(-12.6582128919258,-38.1040934622701,
24.8069323432451));
#31002=CARTESIAN_POINT('Ctrl Pts',(-12.7479187422822,-38.0249714780818,
24.801128459012));
#31003=CARTESIAN_POINT('Ctrl Pts',(-12.8339976115558,-37.9420541357521,
24.795324574779));
#31004=CARTESIAN_POINT('Ctrl Pts',(-12.9200637660598,-37.8591490412006,
24.7895215478417));
#31005=CARTESIAN_POINT('Ctrl Pts',(-13.0025037108978,-37.7724499866039,
24.7837185209044));
#31006=CARTESIAN_POINT('Ctrl Pts',(-13.0809765035836,-37.6823140726555,
24.7779154939671));
#31007=CARTESIAN_POINT('Ctrl Pts',(-13.1594562245964,-37.5921702006485,
24.7721119546833));
#31008=CARTESIAN_POINT('Ctrl Pts',(-13.2339678289217,-37.4985891739701,
24.7663084153994));
#31009=CARTESIAN_POINT('Ctrl Pts',(-13.3042099961916,-37.4019619691135,
24.7605048761155));
#31010=CARTESIAN_POINT('Ctrl Pts',(-13.3744749421769,-37.3053034291816,
24.7546994548116));
#31011=CARTESIAN_POINT('Ctrl Pts',(-13.4404674576149,-37.2055970765999,
24.7488940335076));
#31012=CARTESIAN_POINT('Ctrl Pts',(-13.5019293327585,-37.1032631666926,
24.7430886122036));
#31013=CARTESIAN_POINT('Ctrl Pts',(-13.56345927124,-37.0008159314518,24.7372767619329));
#31014=CARTESIAN_POINT('Ctrl Pts',(-13.62044834417,-36.8957356809831,24.7314649116622));
#31015=CARTESIAN_POINT('Ctrl Pts',(-13.6726840601652,-36.7884677224396,
24.7256530613915));
#31016=CARTESIAN_POINT('Ctrl Pts',(-13.7249540848592,-36.681129309725,24.7198373938663));
#31017=CARTESIAN_POINT('Ctrl Pts',(-13.772464372894,-36.5716007010673,24.7140217263411));
#31018=CARTESIAN_POINT('Ctrl Pts',(-13.8150510174271,-36.460346100905,24.7082060588159));
#31019=CARTESIAN_POINT('Ctrl Pts',(-13.8576986627298,-36.3489321405416,
24.702382060975));
#31020=CARTESIAN_POINT('Ctrl Pts',(-13.8954084592957,-36.2357876401169,
24.6965580631341));
#31021=CARTESIAN_POINT('Ctrl Pts',(-13.928066613758,-36.1213909567496,24.6907340652932));
#31022=CARTESIAN_POINT('Ctrl Pts',(-13.936731000161,-36.09104089306,24.6891889269185));
#31023=CARTESIAN_POINT('Ctrl Pts',(-13.9450400971673,-36.0606027397414,
24.6876437885439));
#31024=CARTESIAN_POINT('Ctrl Pts',(-13.9529923889216,-36.0300855173858,
24.6860986501693));
#31025=CARTESIAN_POINT('Ctrl Pts',(-13.9915465443555,-35.882132478129,24.6786075385624));
#31026=CARTESIAN_POINT('Ctrl Pts',(-14.0218101378458,-35.7319372299034,
24.6711164269556));
#31027=CARTESIAN_POINT('Ctrl Pts',(-14.0435706506774,-35.5803114620445,
24.6636253153487));
#31028=CARTESIAN_POINT('Ctrl Pts',(-14.0649246235175,-35.4315184370933,
24.6562741561627));
#31029=CARTESIAN_POINT('Ctrl Pts',(-14.0780902876876,-35.281347638357,24.6489229969766));
#31030=CARTESIAN_POINT('Ctrl Pts',(-14.0829121862388,-35.1305874399128,
24.6415718377906));
#31031=CARTESIAN_POINT('Ctrl Pts',(-14.0842649181091,-35.0882932848111,
24.6395095490035));
#31032=CARTESIAN_POINT('Ctrl Pts',(-14.0849612552969,-35.0459528838747,
24.6374472602164));
#31033=CARTESIAN_POINT('Ctrl Pts',(-14.0849984277889,-35.0035839868969,
24.6353849714293));
#31034=CARTESIAN_POINT('Ctrl Pts',(-14.0849984277894,-35.0035839863873,
24.6353849714045));
#31035=CARTESIAN_POINT('Ctrl Pts',(-14.0851020062225,-34.8855261338036,
24.6296385535608));
#31036=CARTESIAN_POINT('Ctrl Pts',(-14.0800834836686,-34.7673454041044,
24.6238921357172));
#31037=CARTESIAN_POINT('Ctrl Pts',(-14.0699376947858,-34.64952580614,24.6181457178735));
#31038=CARTESIAN_POINT('Ctrl Pts',(-14.0597976023172,-34.5317723586983,
24.6124025263907));
#31039=CARTESIAN_POINT('Ctrl Pts',(-14.0445360024405,-34.4143800553256,
24.606659334908));
#31040=CARTESIAN_POINT('Ctrl Pts',(-14.024199795063,-34.2978312101673,24.6009161434252));
#31041=CARTESIAN_POINT('Ctrl Pts',(-14.003869129897,-34.1813141279799,24.5951745171302));
#31042=CARTESIAN_POINT('Ctrl Pts',(-13.9784666777729,-34.065640458642,24.5894328908351));
#31043=CARTESIAN_POINT('Ctrl Pts',(-13.9480909112641,-33.9512849975357,
24.5836912645401));
#31044=CARTESIAN_POINT('Ctrl Pts',(-13.9177158689797,-33.8369322629124,
24.577949775138));
#31045=CARTESIAN_POINT('Ctrl Pts',(-13.8823678558292,-33.7238980779719,
24.5722082857358));
#31046=CARTESIAN_POINT('Ctrl Pts',(-13.8421957448839,-33.612643932512,24.5664667963337));
#31047=CARTESIAN_POINT('Ctrl Pts',(-13.8020146008844,-33.5013647705742,
24.5607240159069));
#31048=CARTESIAN_POINT('Ctrl Pts',(-13.7570073454803,-33.391866836607,24.5549812354801));
#31049=CARTESIAN_POINT('Ctrl Pts',(-13.7073714148722,-33.284592703703,24.5492384550533));
#31050=CARTESIAN_POINT('Ctrl Pts',(-13.657683486109,-33.1772061913812,24.5434896585413));
#31051=CARTESIAN_POINT('Ctrl Pts',(-13.6033573785645,-33.0720485102435,
24.5377408620293));
#31052=CARTESIAN_POINT('Ctrl Pts',(-13.5446370465651,-32.9695386711099,
24.5319920655174));
#31053=CARTESIAN_POINT('Ctrl Pts',(-13.4858820406438,-32.866968300674,24.5262398743835));
#31054=CARTESIAN_POINT('Ctrl Pts',(-13.4227278681906,-32.7670492372735,
24.5204876832497));
#31055=CARTESIAN_POINT('Ctrl Pts',(-13.3554614679228,-32.6701709639363,
24.5147354921159));
#31056=CARTESIAN_POINT('Ctrl Pts',(-13.2880945699607,-32.5731479520216,
24.5089747070638));
#31057=CARTESIAN_POINT('Ctrl Pts',(-13.216603432795,-32.4791751304297,24.5032139220117));
#31058=CARTESIAN_POINT('Ctrl Pts',(-13.1413149418207,-32.3886085248868,
24.4974531369597));
#31059=CARTESIAN_POINT('Ctrl Pts',(-13.1045735045829,-32.3444112350974,
24.49464182384));
#31060=CARTESIAN_POINT('Ctrl Pts',(-13.0669282755438,-32.3010245830022,
24.4918305107204));
#31061=CARTESIAN_POINT('Ctrl Pts',(-13.0284202510578,-32.2584865889471,
24.4890191976008));
#31062=CARTESIAN_POINT('Ctrl Pts',(-12.9486514461778,-32.1703697615308,
24.4831956039294));
#31063=CARTESIAN_POINT('Ctrl Pts',(-12.8649049617741,-32.0855952341254,
24.477372010258));
#31064=CARTESIAN_POINT('Ctrl Pts',(-12.777491772723,-32.0045426972737,24.4715484165866));
#31065=CARTESIAN_POINT('Ctrl Pts',(-12.690188868394,-31.9235924202366,24.4657321702437));
#31066=CARTESIAN_POINT('Ctrl Pts',(-12.599228757394,-31.8463550690208,24.4599159239007));
#31067=CARTESIAN_POINT('Ctrl Pts',(-12.5049615082197,-31.773176044105,24.4540996775577));
#31068=CARTESIAN_POINT('Ctrl Pts',(-12.4107886210817,-31.7000702717967,
24.4482892533095));
#31069=CARTESIAN_POINT('Ctrl Pts',(-12.3133155022263,-31.6310149930897,
24.4424788290612));
#31070=CARTESIAN_POINT('Ctrl Pts',(-12.2129273337946,-31.566317193545,24.4366684048129));
#31071=CARTESIAN_POINT('Ctrl Pts',(-12.1087392655482,-31.4991704484687,
24.4306380439887));
#31072=CARTESIAN_POINT('Ctrl Pts',(-12.001411434772,-31.4367178844015,24.4246076831645));
#31073=CARTESIAN_POINT('Ctrl Pts',(-11.891410407136,-31.379255370538,24.4185773223403));
#31074=CARTESIAN_POINT('Ctrl Pts',(-11.7855405846588,-31.3239509222747,
24.4127734381071));
#31075=CARTESIAN_POINT('Ctrl Pts',(-11.6771951282978,-31.273268676305,24.406969553874));
#31076=CARTESIAN_POINT('Ctrl Pts',(-11.5668168564593,-31.2274266159139,
24.4011656696408));
#31077=CARTESIAN_POINT('Ctrl Pts',(-11.4564548886719,-31.1815913268852,
24.3953626427034));
#31078=CARTESIAN_POINT('Ctrl Pts',(-11.3440610795513,-31.1405949582078,
24.389559615766));
#31079=CARTESIAN_POINT('Ctrl Pts',(-11.2300989151555,-31.1046076373575,
24.3837565888286));
#31080=CARTESIAN_POINT('Ctrl Pts',(-11.1161266890924,-31.0686171392032,
24.3779530495446));
#31081=CARTESIAN_POINT('Ctrl Pts',(-11.0005862218465,-31.0376366911359,
24.3721495102606));
#31082=CARTESIAN_POINT('Ctrl Pts',(-10.8839562508819,-31.0117865720944,
24.3663459709766));
#31083=CARTESIAN_POINT('Ctrl Pts',(-10.7672884581778,-30.9859280701607,
24.3605405496725));
#31084=CARTESIAN_POINT('Ctrl Pts',(-10.6495308575516,-30.9652032943032,
24.3547351283683));
#31085=CARTESIAN_POINT('Ctrl Pts',(-10.5311718307159,-30.949681310532,24.3489297070642));
#31086=CARTESIAN_POINT('Ctrl Pts',(-10.4126817322134,-30.9341421376005,
24.3431178567934));
#31087=CARTESIAN_POINT('Ctrl Pts',(-10.2935892831711,-30.9238173105511,
24.3373060065225));
#31088=CARTESIAN_POINT('Ctrl Pts',(-10.174387593082,-30.9187239780457,24.3314941562517));
#31089=CARTESIAN_POINT('Ctrl Pts',(-10.0551076106827,-30.9136273002122,
24.3256784887263));
#31090=CARTESIAN_POINT('Ctrl Pts',(-9.93571865174241,-30.9137689594669,
24.319862821201));
#31091=CARTESIAN_POINT('Ctrl Pts',(-9.81671176650925,-30.9191140148904,
24.3140471536757));
#31092=CARTESIAN_POINT('Ctrl Pts',(-9.69753441676367,-30.9244667265287,
24.3082231558346));
#31093=CARTESIAN_POINT('Ctrl Pts',(-9.57874063835113,-30.935037674659,24.3023991579936));
#31094=CARTESIAN_POINT('Ctrl Pts',(-9.46081446167688,-30.9507403201001,
24.2965751601525));
#31095=CARTESIAN_POINT('Ctrl Pts',(-9.42952800419933,-30.9549063175294,
24.2950300217791));
#31096=CARTESIAN_POINT('Ctrl Pts',(-9.39830254646571,-30.9594332434406,
24.2934848834058));
#31097=CARTESIAN_POINT('Ctrl Pts',(-9.36714696466196,-30.964318888259,24.2919397450324));
#31098=CARTESIAN_POINT('Ctrl Pts',(-9.24972281422751,-30.9827326895398,
24.2861161798703));
#31099=CARTESIAN_POINT('Ctrl Pts',(-9.13291364202334,-31.0063053837757,
24.2802926147083));
#31100=CARTESIAN_POINT('Ctrl Pts',(-9.01720746820394,-31.0349850139696,
24.2744690495462));
#31101=CARTESIAN_POINT('Ctrl Pts',(-8.90164192701255,-31.0636297861119,
24.2686525625136));
#31102=CARTESIAN_POINT('Ctrl Pts',(-8.78717711113497,-31.0973690534386,
24.2628360754809));
#31103=CARTESIAN_POINT('Ctrl Pts',(-8.67429385790801,-31.1360993510677,
24.2570195884483));
#31104=CARTESIAN_POINT('Ctrl Pts',(-8.56153930379801,-31.1747854919688,
24.2512097328399));
#31105=CARTESIAN_POINT('Ctrl Pts',(-8.4503631069613,-31.2184512041946,24.2453998772315));
#31106=CARTESIAN_POINT('Ctrl Pts',(-8.34123302693219,-31.2669426566071,
24.2395900216232));
#31107=CARTESIAN_POINT('Ctrl Pts',(-8.23217569903826,-31.3154017819409,
24.2337840391852));
#31108=CARTESIAN_POINT('Ctrl Pts',(-8.12516214700283,-31.3686800843982,
24.2279780567473));
#31109=CARTESIAN_POINT('Ctrl Pts',(-8.02064187895397,-31.4265749722921,
24.2221720743094));
#31110=CARTESIAN_POINT('Ctrl Pts',(-7.91616129546325,-31.4844478784873,
24.2163682963037));
#31111=CARTESIAN_POINT('Ctrl Pts',(-7.81417247073959,-31.5469336882283,
24.210564518298));
#31112=CARTESIAN_POINT('Ctrl Pts',(-7.71510143287545,-31.6137833002077,
24.2047607402923));
#31113=CARTESIAN_POINT('Ctrl Pts',(-7.64622177178903,-31.6602608451711,
24.2007256330533));
#31114=CARTESIAN_POINT('Ctrl Pts',(-7.57875203275188,-31.7088467835586,
24.1966905258144));
#31115=CARTESIAN_POINT('Ctrl Pts',(-7.51282745730979,-31.7594448403263,
24.1926554185755));
#31116=CARTESIAN_POINT('',(-14.084998667809,-34.9967009094586,24.7396150285614));
#31117=CARTESIAN_POINT('Ctrl Pts',(-14.084998667809,-34.9967009094586,24.7396150285614));
#31118=CARTESIAN_POINT('Ctrl Pts',(-14.0848838734084,-34.854560229187,24.7327077308575));
#31119=CARTESIAN_POINT('Ctrl Pts',(-14.0773464015934,-34.7127316992153,
24.7258004331536));
#31120=CARTESIAN_POINT('Ctrl Pts',(-14.0625068059482,-34.5719071927434,
24.7188931354498));
#31121=CARTESIAN_POINT('Ctrl Pts',(-14.0474942948948,-34.4294417569901,
24.7119053518465));
#31122=CARTESIAN_POINT('Ctrl Pts',(-14.0250085659472,-34.2880039250404,
24.7049175682433));
#31123=CARTESIAN_POINT('Ctrl Pts',(-13.9952238380687,-34.1482890844142,
24.6979297846401));
#31124=CARTESIAN_POINT('Ctrl Pts',(-13.9681220732687,-34.0211595445654,
24.6915714499774));
#31125=CARTESIAN_POINT('Ctrl Pts',(-13.9349776994646,-33.8954563163519,
24.6852131153147));
#31126=CARTESIAN_POINT('Ctrl Pts',(-13.8959562242754,-33.7716881102385,
24.6788547806521));
#31127=CARTESIAN_POINT('Ctrl Pts',(-13.8602164861204,-33.658328908492,24.673031186981));
#31128=CARTESIAN_POINT('Ctrl Pts',(-13.8194674520747,-33.5463480602667,
24.66720759331));
#31129=CARTESIAN_POINT('Ctrl Pts',(-13.7738333631692,-33.4362203649393,
24.661383999639));
#31130=CARTESIAN_POINT('Ctrl Pts',(-13.7282568484454,-33.3262316120577,
24.6555677532964));
#31131=CARTESIAN_POINT('Ctrl Pts',(-13.677807692304,-33.2180917356995,24.6497515069538));
#31132=CARTESIAN_POINT('Ctrl Pts',(-13.6226599695282,-33.1122606787011,
24.6439352606112));
#31133=CARTESIAN_POINT('Ctrl Pts',(-13.5675674499272,-33.0065355591748,
24.6381248363633));
#31134=CARTESIAN_POINT('Ctrl Pts',(-13.5077859079211,-32.9031150213197,
24.6323144121154));
#31135=CARTESIAN_POINT('Ctrl Pts',(-13.4435373555386,-32.802438742376,24.6265039878675));
#31136=CARTESIAN_POINT('Ctrl Pts',(-13.3768568625529,-32.6979516580294,
24.6204736270431));
#31137=CARTESIAN_POINT('Ctrl Pts',(-13.3053646778812,-32.5964211032718,
24.6144432662188));
#31138=CARTESIAN_POINT('Ctrl Pts',(-13.2293614153236,-32.4983106009699,
24.6084129053945));
#31139=CARTESIAN_POINT('Ctrl Pts',(-13.1562125358369,-32.403884742556,24.6026090211617));
#31140=CARTESIAN_POINT('Ctrl Pts',(-13.0788855771601,-32.3126270336723,
24.5968051369289));
#31141=CARTESIAN_POINT('Ctrl Pts',(-12.9976920602387,-32.2249203052918,
24.5910012526961));
#31142=CARTESIAN_POINT('Ctrl Pts',(-12.9165105364681,-32.137226532133,24.585198225759));
#31143=CARTESIAN_POINT('Ctrl Pts',(-12.8314638675763,-32.0530829959458,
24.579395198822));
#31144=CARTESIAN_POINT('Ctrl Pts',(-12.7429023208597,-31.9728376557868,
24.573592171885));
#31145=CARTESIAN_POINT('Ctrl Pts',(-12.6543329550848,-31.8925852308035,
24.5677886326013));
#31146=CARTESIAN_POINT('Ctrl Pts',(-12.5622483970904,-31.8162319603357,
24.5619850933177));
#31147=CARTESIAN_POINT('Ctrl Pts',(-12.4670335692747,-31.7440868610984,
24.5561815540341));
#31148=CARTESIAN_POINT('Ctrl Pts',(-12.3717878644006,-31.6719183660468,
24.5503761327304));
#31149=CARTESIAN_POINT('Ctrl Pts',(-12.2734101961745,-31.603961002706,24.5445707114266));
#31150=CARTESIAN_POINT('Ctrl Pts',(-12.1723156152313,-31.5404812664444,
24.5387652901229));
#31151=CARTESIAN_POINT('Ctrl Pts',(-12.0711090813969,-31.4769312322505,
24.5329534398524));
#31152=CARTESIAN_POINT('Ctrl Pts',(-11.9671799751828,-31.4178689401148,
24.5271415895819));
#31153=CARTESIAN_POINT('Ctrl Pts',(-11.8609693010197,-31.36351567298,24.5213297393114));
#31154=CARTESIAN_POINT('Ctrl Pts',(-11.7546888671157,-31.3091267063276,
24.5155140717865));
#31155=CARTESIAN_POINT('Ctrl Pts',(-11.646124251332,-31.2594530937943,24.5096984042615));
#31156=CARTESIAN_POINT('Ctrl Pts',(-11.5357363154174,-31.2146679181995,
24.5038827367366));
#31157=CARTESIAN_POINT('Ctrl Pts',(-11.4251902607043,-31.1698185926765,
24.4980587388959));
#31158=CARTESIAN_POINT('Ctrl Pts',(-11.3128160564153,-31.1298718163044,
24.4922347410552));
#31159=CARTESIAN_POINT('Ctrl Pts',(-11.1990897082743,-31.0949508490275,
24.4864107432145));
#31160=CARTESIAN_POINT('Ctrl Pts',(-11.1689174881278,-31.0856861260357,
24.4848656048375));
#31161=CARTESIAN_POINT('Ctrl Pts',(-11.138650147959,-31.0767748751365,24.4833204664606));
#31162=CARTESIAN_POINT('Ctrl Pts',(-11.1082966765157,-31.0682187908247,
24.4817753280836));
#31163=CARTESIAN_POINT('Ctrl Pts',(-10.9938903537229,-31.0359697564614,
24.475951493395));
#31164=CARTESIAN_POINT('Ctrl Pts',(-10.8778908004923,-31.0086663255076,
24.4701276587064));
#31165=CARTESIAN_POINT('Ctrl Pts',(-10.7607632878861,-30.986464872484,24.4643038240178));
#31166=CARTESIAN_POINT('Ctrl Pts',(-10.6437847222405,-30.9642916522716,
24.458487395296));
#31167=CARTESIAN_POINT('Ctrl Pts',(-10.5256814480284,-30.9472075803738,
24.4526709665742));
#31168=CARTESIAN_POINT('Ctrl Pts',(-10.4069336155649,-30.9353191967236,
24.4468545378524));
#31169=CARTESIAN_POINT('Ctrl Pts',(-10.2883058386614,-30.9234428323796,
24.4410439896137));
#31170=CARTESIAN_POINT('Ctrl Pts',(-10.1690352039896,-30.9167517461939,
24.4352334413749));
#31171=CARTESIAN_POINT('Ctrl Pts',(-10.0496111757909,-30.9153012679958,
24.4294228931361));
#31172=CARTESIAN_POINT('Ctrl Pts',(-9.93027871601185,-30.9138519019524,
24.4236168001374));
#31173=CARTESIAN_POINT('Ctrl Pts',(-9.81079350370928,-30.9176351517055,
24.4178107071387));
#31174=CARTESIAN_POINT('Ctrl Pts',(-9.69164860837947,-30.9266543948143,
24.41200461414));
#31175=CARTESIAN_POINT('Ctrl Pts',(-9.57255221940145,-30.9356699660027,
24.4062008849218));
#31176=CARTESIAN_POINT('Ctrl Pts',(-9.45379627834284,-30.9499172604491,
24.4003971557037));
#31177=CARTESIAN_POINT('Ctrl Pts',(-9.33587187471168,-30.9693475921135,
24.3945934264856));
#31178=CARTESIAN_POINT('Ctrl Pts',(-9.21796765035289,-30.9887745988516,
24.388790690404));
#31179=CARTESIAN_POINT('Ctrl Pts',(-9.10089508298854,-31.0133828117266,
24.3829879543224));
#31180=CARTESIAN_POINT('Ctrl Pts',(-8.98513753636315,-31.0430720021839,
24.3771852182408));
#31181=CARTESIAN_POINT('Ctrl Pts',(-8.86937247998878,-31.0727631187218,
24.3713821057078));
#31182=CARTESIAN_POINT('Ctrl Pts',(-8.75492300914663,-31.1075357657944,
24.3655789931748));
#31183=CARTESIAN_POINT('Ctrl Pts',(-8.64225911212408,-31.1472393428361,
24.3597758806418));
#31184=CARTESIAN_POINT('Ctrl Pts',(-8.52950544824127,-31.1869745543725,
24.3539681443811));
#31185=CARTESIAN_POINT('Ctrl Pts',(-8.41854058517941,-31.2316484066746,
24.3481604081203));
#31186=CARTESIAN_POINT('Ctrl Pts',(-8.30981632203141,-31.2810614236413,
24.3423526718595));
#31187=CARTESIAN_POINT('Ctrl Pts',(-8.20104516977009,-31.3304957507783,
24.3365424309176));
#31188=CARTESIAN_POINT('Ctrl Pts',(-8.09451690735335,-31.3846731312039,
24.3307321899758));
#31189=CARTESIAN_POINT('Ctrl Pts',(-7.99065905712731,-31.4433479260271,
24.3249219490339));
#31190=CARTESIAN_POINT('Ctrl Pts',(-7.8866674396989,-31.5020982930207,24.3191042245973));
#31191=CARTESIAN_POINT('Ctrl Pts',(-7.78535345118204,-31.5653574290668,
24.3132865001607));
#31192=CARTESIAN_POINT('Ctrl Pts',(-7.68711615261122,-31.6328360140189,
24.3074687757241));
#31193=CARTESIAN_POINT('Ctrl Pts',(-7.62787447660817,-31.6735287501286,
24.303960416362));
#31194=CARTESIAN_POINT('Ctrl Pts',(-7.56975108065747,-31.7157551433316,
24.3004520569999));
#31195=CARTESIAN_POINT('Ctrl Pts',(-7.51282745730979,-31.7594448403263,
24.2969436976378));
#31196=CARTESIAN_POINT('Ctrl Pts',(-7.5128274573098,-31.7594448403263,25.5469376127646));
#31197=CARTESIAN_POINT('Ctrl Pts',(-7.41802267680316,-31.8322088685169,
25.5411329166442));
#31198=CARTESIAN_POINT('Ctrl Pts',(-7.32644265542362,-31.9091144685266,
25.5353282205238));
#31199=CARTESIAN_POINT('Ctrl Pts',(-7.23845612486566,-31.9898338209149,
25.5295235244034));
#31200=CARTESIAN_POINT('Ctrl Pts',(-7.1503751931797,-32.0706397774443,25.5237126003995));
#31201=CARTESIAN_POINT('Ctrl Pts',(-7.06589575190499,-32.1552673801606,
25.5179016763955));
#31202=CARTESIAN_POINT('Ctrl Pts',(-6.98535008939967,-32.243351506536,25.5120907523916));
#31203=CARTESIAN_POINT('Ctrl Pts',(-6.90475677099751,-32.3314877490392,
25.5062763902784));
#31204=CARTESIAN_POINT('Ctrl Pts',(-6.8281021292086,-32.4230842760319,25.5004620281651));
#31205=CARTESIAN_POINT('Ctrl Pts',(-6.75567743765626,-32.5177437458096,
25.4946476660519));
#31206=CARTESIAN_POINT('Ctrl Pts',(-6.68314294086342,-32.6125467316399,
25.4888244886103));
#31207=CARTESIAN_POINT('Ctrl Pts',(-6.61485143510181,-32.7104215998079,
25.4830013111688));
#31208=CARTESIAN_POINT('Ctrl Pts',(-6.55105043615599,-32.8109426900923,
25.4771781337273));
#31209=CARTESIAN_POINT('Ctrl Pts',(-6.51450889549698,-32.8685153859499,
25.4738429527935));
#31210=CARTESIAN_POINT('Ctrl Pts',(-6.47943954707083,-32.9269556736248,
25.4705077718596));
#31211=CARTESIAN_POINT('Ctrl Pts',(-6.44588189144434,-32.9861803778797,
25.4671725909258));
#31212=CARTESIAN_POINT('Ctrl Pts',(-6.38728652428349,-33.0895932422775,
25.4613489972415));
#31213=CARTESIAN_POINT('Ctrl Pts',(-6.33311386295757,-33.1957323819947,
25.4555254035572));
#31214=CARTESIAN_POINT('Ctrl Pts',(-6.28362667866039,-33.3041832833601,
25.4497018098729));
#31215=CARTESIAN_POINT('Ctrl Pts',(-6.23420192979541,-33.4124973578078,
25.4438855635169));
#31216=CARTESIAN_POINT('Ctrl Pts',(-6.1894510682932,-33.5231170245795,25.4380693171609));
#31217=CARTESIAN_POINT('Ctrl Pts',(-6.14959202975056,-33.6356014282331,
25.4322530708049));
#31218=CARTESIAN_POINT('Ctrl Pts',(-6.10977289032432,-33.7479732343811,
25.4264426465434));
#31219=CARTESIAN_POINT('Ctrl Pts',(-6.07483596799803,-33.8622056813432,
25.420632222282));
#31220=CARTESIAN_POINT('Ctrl Pts',(-6.04495169710551,-33.9778366462393,
25.4148217980205));
#31221=CARTESIAN_POINT('Ctrl Pts',(-6.01393624484356,-34.0978444819544,
25.4087914372012));
#31222=CARTESIAN_POINT('Ctrl Pts',(-5.9883636943945,-34.219358393308,25.4027610763819));
#31223=CARTESIAN_POINT('Ctrl Pts',(-5.96836835913738,-34.3418424866376,
25.3967307155626));
#31224=CARTESIAN_POINT('Ctrl Pts',(-5.9491239698242,-34.4597265604176,25.3909268313159));
#31225=CARTESIAN_POINT('Ctrl Pts',(-5.9350455056025,-34.5785088186769,25.3851229470693));
#31226=CARTESIAN_POINT('Ctrl Pts',(-5.92620079771629,-34.6977003812893,
25.3793190628226));
#31227=CARTESIAN_POINT('Ctrl Pts',(-5.91735739628789,-34.8168743380351,
25.3735160358716));
#31228=CARTESIAN_POINT('Ctrl Pts',(-5.91374624398939,-34.9364570717935,
25.3677130089207));
#31229=CARTESIAN_POINT('Ctrl Pts',(-5.91538324624638,-35.055955115541,25.3619099819697));
#31230=CARTESIAN_POINT('Ctrl Pts',(-5.91702039303356,-35.1754637097173,
25.3561064426721));
#31231=CARTESIAN_POINT('Ctrl Pts',(-5.92390661004875,-35.2948871906974,
25.3503029033744));
#31232=CARTESIAN_POINT('Ctrl Pts',(-5.9360056866268,-35.4137332726169,25.3444993640768));
#31233=CARTESIAN_POINT('Ctrl Pts',(-5.94810868679438,-35.5326178949358,
25.338693942759));
#31234=CARTESIAN_POINT('Ctrl Pts',(-5.96542786715174,-35.6509243397802,
25.3328885214412));
#31235=CARTESIAN_POINT('Ctrl Pts',(-5.98787536717209,-35.7681672543499,
25.3270831001234));
#31236=CARTESIAN_POINT('Ctrl Pts',(-6.01034772572099,-35.8855400045957,
25.3212712498389));
#31237=CARTESIAN_POINT('Ctrl Pts',(-6.03795966314973,-36.0018464723642,
25.3154593995543));
#31238=CARTESIAN_POINT('Ctrl Pts',(-6.07057254486996,-36.1166131267678,
25.3096475492698));
#31239=CARTESIAN_POINT('Ctrl Pts',(-6.10320684690608,-36.2314551605266,
25.3038318817307));
#31240=CARTESIAN_POINT('Ctrl Pts',(-6.1408485062443,-36.3447549801565,25.2980162141917));
#31241=CARTESIAN_POINT('Ctrl Pts',(-6.18331008292999,-36.4560573741911,
25.2922005466526));
#31242=CARTESIAN_POINT('Ctrl Pts',(-6.22583248123856,-36.5675191968847,
25.2863765487979));
#31243=CARTESIAN_POINT('Ctrl Pts',(-6.27318841536203,-36.6769775099537,
25.2805525509432));
#31244=CARTESIAN_POINT('Ctrl Pts',(-6.32514366484224,-36.7839999764436,
25.2747285530885));
#31245=CARTESIAN_POINT('Ctrl Pts',(-6.33892767454405,-36.8123936177247,
25.2731834148448));
#31246=CARTESIAN_POINT('Ctrl Pts',(-6.35303517529878,-36.8406159585932,
25.2716382766011));
#31247=CARTESIAN_POINT('Ctrl Pts',(-6.36746128086554,-36.8686592664231,
25.2700931383574));
#31248=CARTESIAN_POINT('Ctrl Pts',(-6.42183297051223,-36.9743539061123,
25.2642695446883));
#31249=CARTESIAN_POINT('Ctrl Pts',(-6.48090920439806,-37.0778439671083,
25.2584459510193));
#31250=CARTESIAN_POINT('Ctrl Pts',(-6.54448733684962,-37.1786824538715,
25.2526223573502));
#31251=CARTESIAN_POINT('Ctrl Pts',(-6.6079852560432,-37.279393717905,25.2468061110096));
#31252=CARTESIAN_POINT('Ctrl Pts',(-6.67597356092467,-37.3774597191691,
25.2409898646691));
#31253=CARTESIAN_POINT('Ctrl Pts',(-6.74820299708228,-37.472456521724,25.2351736183285));
#31254=CARTESIAN_POINT('Ctrl Pts',(-6.82036013117569,-37.5673582319552,
25.2293631940825));
#31255=CARTESIAN_POINT('Ctrl Pts',(-6.89674970512961,-37.659196532226,25.2235527698366));
#31256=CARTESIAN_POINT('Ctrl Pts',(-6.97707863859834,-37.7475755572471,
25.2177423455907));
#31257=CARTESIAN_POINT('Ctrl Pts',(-7.06044818839508,-37.8392999112166,
25.2117119847656));
#31258=CARTESIAN_POINT('Ctrl Pts',(-7.14806097694068,-37.9272975549707,
25.2056816239406));
#31259=CARTESIAN_POINT('Ctrl Pts',(-7.23954242393988,-38.011162395284,25.1996512631155));
#31260=CARTESIAN_POINT('Ctrl Pts',(-7.32758818820707,-38.0918776026046,
25.1938473788847));
#31261=CARTESIAN_POINT('Ctrl Pts',(-7.41921694001888,-38.1687645312801,
25.1880434946539));
#31262=CARTESIAN_POINT('Ctrl Pts',(-7.51405697676403,-38.2414984629372,
25.182239610423));
#31263=CARTESIAN_POINT('Ctrl Pts',(-7.60888300462153,-38.3142216510149,
25.176436583488));
#31264=CARTESIAN_POINT('Ctrl Pts',(-7.70691905016476,-38.3827928135887,
25.170633556553));
#31265=CARTESIAN_POINT('Ctrl Pts',(-7.80776111059125,-38.4469281471716,
25.1648305296179));
#31266=CARTESIAN_POINT('Ctrl Pts',(-7.90861207431753,-38.511069143234,25.1590269903362));
#31267=CARTESIAN_POINT('Ctrl Pts',(-8.01226920092535,-38.5707733124886,
25.1532234510546));
#31268=CARTESIAN_POINT('Ctrl Pts',(-8.11830090735696,-38.6258010873111,
25.1474199117729));
#31269=CARTESIAN_POINT('Ctrl Pts',(-8.22436699863475,-38.6808467069994,
25.1416144904711));
#31270=CARTESIAN_POINT('Ctrl Pts',(-8.33280883894015,-38.731212728281,25.1358090691693));
#31271=CARTESIAN_POINT('Ctrl Pts',(-8.44317233125726,-38.7767065824389,
25.1300036478676));
#31272=CARTESIAN_POINT('Ctrl Pts',(-8.55365804092722,-38.8222508168294,
25.124191797599));
#31273=CARTESIAN_POINT('Ctrl Pts',(-8.66606927263863,-38.8629119585548,
25.1183799473305));
#31274=CARTESIAN_POINT('Ctrl Pts',(-8.77993398439098,-38.8985463852,25.1125680970619));
#31275=CARTESIAN_POINT('Ctrl Pts',(-8.89387348309799,-38.9342042167281,
25.1067524295389));
#31276=CARTESIAN_POINT('Ctrl Pts',(-9.00926796929501,-38.9648286535075,
25.1009367620158));
#31277=CARTESIAN_POINT('Ctrl Pts',(-9.1256339694926,-38.9903269345625,25.0951210944928));
#31278=CARTESIAN_POINT('Ctrl Pts',(-9.24216665142073,-39.0158617391519,
25.089297096654));
#31279=CARTESIAN_POINT('Ctrl Pts',(-9.35967322399059,-39.0362556628802,
25.0834730988152));
#31280=CARTESIAN_POINT('Ctrl Pts',(-9.47766370192668,-39.0514676096095,
25.0776491009763));
#31281=CARTESIAN_POINT('Ctrl Pts',(-9.50896721934635,-39.0555034220561,
25.0761039625805));
#31282=CARTESIAN_POINT('Ctrl Pts',(-9.54030479206342,-39.0591747752014,
25.0745588241847));
#31283=CARTESIAN_POINT('Ctrl Pts',(-9.5716672742707,-39.0624815170126,25.0730136857889));
#31284=CARTESIAN_POINT('Ctrl Pts',(-9.68987180102332,-39.0749445563952,
25.0671900921193));
#31285=CARTESIAN_POINT('Ctrl Pts',(-9.80881134156663,-39.0822643809811,
25.0613664984498));
#31286=CARTESIAN_POINT('Ctrl Pts',(-9.92800095875183,-39.0843654510902,
25.0555429047802));
#31287=CARTESIAN_POINT('Ctrl Pts',(-10.0470402005301,-39.0864638703873,
25.0497266584391));
#31288=CARTESIAN_POINT('Ctrl Pts',(-10.1663284867357,-39.0833566239609,
25.043910412098));
#31289=CARTESIAN_POINT('Ctrl Pts',(-10.2853746173914,-39.0750197947677,
25.0380941657569));
#31290=CARTESIAN_POINT('Ctrl Pts',(-10.4043015822128,-39.0666913107866,
25.0322837415105));
#31291=CARTESIAN_POINT('Ctrl Pts',(-10.5229864687091,-39.0531436864692,
25.0264733172641));
#31292=CARTESIAN_POINT('Ctrl Pts',(-10.6409375306042,-39.034405046827,25.0206628930177));
#31293=CARTESIAN_POINT('Ctrl Pts',(-10.7633532842126,-39.0149571109073,
25.0146325321928));
#31294=CARTESIAN_POINT('Ctrl Pts',(-10.8849781138591,-38.9899174057335,
25.008602171368));
#31295=CARTESIAN_POINT('Ctrl Pts',(-11.0052670436135,-38.9593766139412,
25.0025718105431));
#31296=CARTESIAN_POINT('Ctrl Pts',(-11.1210383950901,-38.9299828139616,
24.9967679263119));
#31297=CARTESIAN_POINT('Ctrl Pts',(-11.2355719480392,-38.8954937836691,
24.9909640420807));
#31298=CARTESIAN_POINT('Ctrl Pts',(-11.34839236355,-38.8560424056175,24.9851601578495));
#31299=CARTESIAN_POINT('Ctrl Pts',(-11.4611961142788,-38.8165968549562,
24.9793571309141));
#31300=CARTESIAN_POINT('Ctrl Pts',(-11.5722868454571,-38.7721905489741,
24.9735541039786));
#31301=CARTESIAN_POINT('Ctrl Pts',(-11.6812057324157,-38.723005813223,24.9677510770432));
#31302=CARTESIAN_POINT('Ctrl Pts',(-11.7901342357727,-38.6738167349743,
24.9619475377612));
#31303=CARTESIAN_POINT('Ctrl Pts',(-11.8968901414922,-38.6198485562083,
24.9561439984792));
#31304=CARTESIAN_POINT('Ctrl Pts',(-12.001036504013,-38.5613309182955,24.9503404591972));
#31305=CARTESIAN_POINT('Ctrl Pts',(-12.1052166399838,-38.5027943037957,
24.9445350378952));
#31306=CARTESIAN_POINT('Ctrl Pts',(-12.206785193959,-38.4397054959587,24.9387296165931));
#31307=CARTESIAN_POINT('Ctrl Pts',(-12.3053321875756,-38.372338729269,24.932924195291));
#31308=CARTESIAN_POINT('Ctrl Pts',(-12.4039883128662,-38.3048973601207,
24.9271123450222));
#31309=CARTESIAN_POINT('Ctrl Pts',(-12.4996158614001,-38.2331688063547,
24.9213004947534));
#31310=CARTESIAN_POINT('Ctrl Pts',(-12.5918359553017,-38.1574691417028,
24.9154886444846));
#31311=CARTESIAN_POINT('Ctrl Pts',(-12.6841166198558,-38.081719757105,24.9096729769614));
#31312=CARTESIAN_POINT('Ctrl Pts',(-12.7729850694245,-38.0019943392835,
24.9038573094381));
#31313=CARTESIAN_POINT('Ctrl Pts',(-12.8580986988468,-37.9186464033264,
24.8980416419149));
#31314=CARTESIAN_POINT('Ctrl Pts',(-12.9433342443526,-37.835179080451,24.8922176440759));
#31315=CARTESIAN_POINT('Ctrl Pts',(-13.0248039568207,-37.7480791799022,
24.8863936462369));
#31316=CARTESIAN_POINT('Ctrl Pts',(-13.1022048725458,-37.6577339838203,
24.8805696483979));
#31317=CARTESIAN_POINT('Ctrl Pts',(-13.1227397576548,-37.6337649105307,
24.8790245100054));
#31318=CARTESIAN_POINT('Ctrl Pts',(-13.1429884873955,-37.6095675710598,
24.877479371613));
#31319=CARTESIAN_POINT('Ctrl Pts',(-13.1629459212134,-37.5851495313578,
24.8759342332205));
#31320=CARTESIAN_POINT('Ctrl Pts',(-13.2378042578983,-37.4935599084697,
24.8701385737653));
#31321=CARTESIAN_POINT('Ctrl Pts',(-13.3088098080699,-37.3985584740394,
24.8643429143101));
#31322=CARTESIAN_POINT('Ctrl Pts',(-13.3756340199529,-37.3005042845726,
24.8585472548549));
#31323=CARTESIAN_POINT('Ctrl Pts',(-13.4423779072389,-37.2025679590211,
24.8527585619467));
#31324=CARTESIAN_POINT('Ctrl Pts',(-13.5049502169776,-37.1015865095326,
24.8469698690384));
#31325=CARTESIAN_POINT('Ctrl Pts',(-13.5630617794871,-36.9979528912259,
24.8411811761302));
#31326=CARTESIAN_POINT('Ctrl Pts',(-13.6211175348196,-36.8944187969974,
24.8353980423671));
#31327=CARTESIAN_POINT('Ctrl Pts',(-13.6747208597772,-36.7882379551329,
24.829614908604));
#31328=CARTESIAN_POINT('Ctrl Pts',(-13.7236255579147,-36.6798326417964,
24.8238317748409));
#31329=CARTESIAN_POINT('Ctrl Pts',(-13.7724951073974,-36.5715052412387,
24.8180527975164));
#31330=CARTESIAN_POINT('Ctrl Pts',(-13.8166725773331,-36.460956923271,24.8122738201918));
#31331=CARTESIAN_POINT('Ctrl Pts',(-13.8559577878748,-36.3486343233536,
24.8064948428673));
#31332=CARTESIAN_POINT('Ctrl Pts',(-13.8952293775639,-36.236350667598,24.8007178692128));
#31333=CARTESIAN_POINT('Ctrl Pts',(-13.92961193999,-36.1222943399894,24.7949408955583));
#31334=CARTESIAN_POINT('Ctrl Pts',(-13.9589537101831,-36.006931239275,24.7891639219038));
#31335=CARTESIAN_POINT('Ctrl Pts',(-13.9882886312204,-35.8915950674005,
24.7833882967497));
#31336=CARTESIAN_POINT('Ctrl Pts',(-14.0125850024543,-35.7749531295744,
24.7776126715957));
#31337=CARTESIAN_POINT('Ctrl Pts',(-14.0317413883318,-35.6574848877446,
24.7718370464417));
#31338=CARTESIAN_POINT('Ctrl Pts',(-14.0509049499055,-35.5399726440644,
24.7660592578247));
#31339=CARTESIAN_POINT('Ctrl Pts',(-14.0649246106826,-35.4216338849925,
24.7602814692077));
#31340=CARTESIAN_POINT('Ctrl Pts',(-14.0737504068468,-35.3029564700018,
24.7545036805907));
#31341=CARTESIAN_POINT('Ctrl Pts',(-14.0813314046055,-35.2010174267331,
24.7495407965923));
#31342=CARTESIAN_POINT('Ctrl Pts',(-14.0850811474127,-35.0988287954618,
24.7445779125939));
#31343=CARTESIAN_POINT('Ctrl Pts',(-14.0849986678096,-34.9967009101602,
24.7396150285955));
#31344=CARTESIAN_POINT('Origin',(-10.,-35.,32.7603849714045));
#31345=CARTESIAN_POINT('',(-7.5128274573098,-31.7594448403263,26.796772721093));
#31346=CARTESIAN_POINT('',(-7.51282745730979,-31.7594448403263,26.6927653424671));
#31347=CARTESIAN_POINT('',(-7.5128274573098,-31.7594448403263,32.7603849714045));
#31348=CARTESIAN_POINT('',(-14.0849995364304,-34.9980538850391,25.8853849714457));
#31349=CARTESIAN_POINT('Ctrl Pts',(-7.51282745730979,-31.7594448403263,
26.6927653424671));
#31350=CARTESIAN_POINT('Ctrl Pts',(-7.41550409810477,-31.8341419137751,
26.6867866480316));
#31351=CARTESIAN_POINT('Ctrl Pts',(-7.32165094663543,-31.9131486832113,
26.680807953596));
#31352=CARTESIAN_POINT('Ctrl Pts',(-7.23165018155787,-31.9960918318412,
26.6748292591604));
#31353=CARTESIAN_POINT('Ctrl Pts',(-7.14164941648032,-32.079034980471,26.6688505647248));
#31354=CARTESIAN_POINT('Ctrl Pts',(-7.05550131791785,-32.165914133754,26.6628718702893));
#31355=CARTESIAN_POINT('Ctrl Pts',(-6.97354327202869,-32.2563191377791,
26.6568931758537));
#31356=CARTESIAN_POINT('Ctrl Pts',(-6.89371140426106,-32.3443788303763,
26.6510695823501));
#31357=CARTESIAN_POINT('Ctrl Pts',(-6.81759735210981,-32.4360676753925,
26.6452459888466));
#31358=CARTESIAN_POINT('Ctrl Pts',(-6.74554833174319,-32.5310388137963,
26.639422395343));
#31359=CARTESIAN_POINT('Ctrl Pts',(-6.67359021195502,-32.625890131953,26.6336061491707));
#31360=CARTESIAN_POINT('Ctrl Pts',(-6.60568716782213,-32.7240151844941,
26.6277899029984));
#31361=CARTESIAN_POINT('Ctrl Pts',(-6.5421484417945,-32.8250315861108,26.6219736568261));
#31362=CARTESIAN_POINT('Ctrl Pts',(-6.47867331841221,-32.9259468697044,
26.616163232751));
#31363=CARTESIAN_POINT('Ctrl Pts',(-6.41955403829092,-33.0297474009458,
26.610352808676));
#31364=CARTESIAN_POINT('Ctrl Pts',(-6.3650581573562,-33.1360196351363,26.6045423846009));
#31365=CARTESIAN_POINT('Ctrl Pts',(-6.3084994923243,-33.2463144976595,26.5985120237128));
#31366=CARTESIAN_POINT('Ctrl Pts',(-6.25692142388314,-33.3592715215538,
26.5924816628246));
#31367=CARTESIAN_POINT('Ctrl Pts',(-6.21057243011051,-33.4743972690896,
26.5864513019365));
#31368=CARTESIAN_POINT('Ctrl Pts',(-6.16596412375978,-33.5851993425957,
26.5806474178819));
#31369=CARTESIAN_POINT('Ctrl Pts',(-6.12619937404884,-33.6980097669418,
26.5748435338272));
#31370=CARTESIAN_POINT('Ctrl Pts',(-6.09145149069811,-33.8123664073318,
26.5690396497726));
#31371=CARTESIAN_POINT('Ctrl Pts',(-6.05670873999147,-33.9267061559898,
26.5632366230155));
#31372=CARTESIAN_POINT('Ctrl Pts',(-6.02698150062196,-34.0425912758967,
26.5574335962583));
#31373=CARTESIAN_POINT('Ctrl Pts',(-6.00239342359869,-34.1595437784673,
26.5516305695011));
#31374=CARTESIAN_POINT('Ctrl Pts',(-5.97780317571153,-34.2765066066915,
26.5458270303988));
#31375=CARTESIAN_POINT('Ctrl Pts',(-5.95835307631765,-34.3945366053273,
26.5400234912965));
#31376=CARTESIAN_POINT('Ctrl Pts',(-5.94411566812738,-34.513145518178,26.5342199521942));
#31377=CARTESIAN_POINT('Ctrl Pts',(-5.92987364291467,-34.6317928944909,
26.5284145310731));
#31378=CARTESIAN_POINT('Ctrl Pts',(-5.92084771939816,-34.7510191531632,
26.522609109952));
#31379=CARTESIAN_POINT('Ctrl Pts',(-5.91705852648728,-34.8703314846627,
26.5168036888309));
#31380=CARTESIAN_POINT('Ctrl Pts',(-5.91326513739649,-34.9897759435095,
26.510991838744));
#31381=CARTESIAN_POINT('Ctrl Pts',(-5.91472006756795,-35.1093062570726,
26.5051799886571));
#31382=CARTESIAN_POINT('Ctrl Pts',(-5.92139181534436,-35.2284300244276,
26.4993681385702));
#31383=CARTESIAN_POINT('Ctrl Pts',(-5.92806794515974,-35.3476320328986,
26.4935524712297));
#31384=CARTESIAN_POINT('Ctrl Pts',(-5.93996767580205,-35.4664265580115,
26.4877368038892));
#31385=CARTESIAN_POINT('Ctrl Pts',(-5.95700787211379,-35.5843283784398,
26.4819211365486));
#31386=CARTESIAN_POINT('Ctrl Pts',(-5.97407247666817,-35.7023990805048,
26.4760971388921));
#31387=CARTESIAN_POINT('Ctrl Pts',(-5.99629216755737,-35.8195741258997,
26.4702731412356));
#31388=CARTESIAN_POINT('Ctrl Pts',(-6.02353315362947,-35.9353803609848,
26.4644491435791));
#31389=CARTESIAN_POINT('Ctrl Pts',(-6.03076034401834,-35.966104421669,26.4629040034811));
#31390=CARTESIAN_POINT('Ctrl Pts',(-6.03834070087973,-35.9967322307021,
26.4613588633832));
#31391=CARTESIAN_POINT('Ctrl Pts',(-6.0462711511454,-36.0272551726494,26.4598137232852));
#31392=CARTESIAN_POINT('Ctrl Pts',(-6.07616081668759,-36.1422953652745,
26.4539901295173));
#31393=CARTESIAN_POINT('Ctrl Pts',(-6.11112377217277,-36.2562154530518,
26.4481665357494));
#31394=CARTESIAN_POINT('Ctrl Pts',(-6.15106024591779,-36.3685348988775,
26.4423429419815));
#31395=CARTESIAN_POINT('Ctrl Pts',(-6.19094633387794,-36.4807126370635,
26.4365266955409));
#31396=CARTESIAN_POINT('Ctrl Pts',(-6.23579332401346,-36.591293368582,26.4307104491003));
#31397=CARTESIAN_POINT('Ctrl Pts',(-6.28545091568015,-36.6998088422463,
26.4248942026596));
#31398=CARTESIAN_POINT('Ctrl Pts',(-6.33505879983332,-36.8082156913439,
26.4190837783127));
#31399=CARTESIAN_POINT('Ctrl Pts',(-6.38946753686421,-36.9145610261199,
26.4132733539657));
#31400=CARTESIAN_POINT('Ctrl Pts',(-6.44847791428129,-37.0183943803559,
26.4074629296187));
#31401=CARTESIAN_POINT('Ctrl Pts',(-6.50972195512672,-37.1261580393306,
26.4014325688311));
#31402=CARTESIAN_POINT('Ctrl Pts',(-6.57592273228872,-37.2312153708464,
26.3954022080435));
#31403=CARTESIAN_POINT('Ctrl Pts',(-6.64680375531957,-37.3330880704896,
26.3893718472559));
#31404=CARTESIAN_POINT('Ctrl Pts',(-6.71502276801676,-37.4311348352412,
26.3835679629221));
#31405=CARTESIAN_POINT('Ctrl Pts',(-6.78757656904055,-37.5262314933653,
26.3777640785882));
#31406=CARTESIAN_POINT('Ctrl Pts',(-6.86417364421405,-37.6179797681339,
26.3719601942544));
#31407=CARTESIAN_POINT('Ctrl Pts',(-6.94075940518792,-37.70971449071,26.3661571672157));
#31408=CARTESIAN_POINT('Ctrl Pts',(-7.02138699097805,-37.7981015001445,
26.3603541401771));
#31409=CARTESIAN_POINT('Ctrl Pts',(-7.1057244066607,-37.8827753623549,26.3545511131384));
#31410=CARTESIAN_POINT('Ctrl Pts',(-7.19006926846154,-37.9674567003882,
26.3487475737528));
#31411=CARTESIAN_POINT('Ctrl Pts',(-7.27812432320579,-38.0484239500613,
26.3429440343671));
#31412=CARTESIAN_POINT('Ctrl Pts',(-7.36952097272954,-38.1253487944692,
26.3371404949814));
#31413=CARTESIAN_POINT('Ctrl Pts',(-7.46094726112563,-38.2022985847111,
26.3313350735753));
#31414=CARTESIAN_POINT('Ctrl Pts',(-7.55571698716796,-38.2752030997859,
26.3255296521691));
#31415=CARTESIAN_POINT('Ctrl Pts',(-7.65342928716088,-38.3437749460222,
26.319724230763));
#31416=CARTESIAN_POINT('Ctrl Pts',(-7.75124979447971,-38.4124227292298,
26.3139123803902));
#31417=CARTESIAN_POINT('Ctrl Pts',(-7.85201904580789,-38.4767280316185,
26.3081005300173));
#31418=CARTESIAN_POINT('Ctrl Pts',(-7.95530794312085,-38.5364472840034,
26.3022886796444));
#31419=CARTESIAN_POINT('Ctrl Pts',(-8.05866468113677,-38.5962057603144,
26.296473012017));
#31420=CARTESIAN_POINT('Ctrl Pts',(-8.1645439996482,-38.6513719996173,26.2906573443896));
#31421=CARTESIAN_POINT('Ctrl Pts',(-8.27249450183565,-38.7017495530913,
26.2848416767622));
#31422=CARTESIAN_POINT('Ctrl Pts',(-8.38059963144689,-38.7521992669644,
26.2790176788196));
#31423=CARTESIAN_POINT('Ctrl Pts',(-8.49078149029422,-38.7978464485358,
26.273193680877));
#31424=CARTESIAN_POINT('Ctrl Pts',(-8.60257100685233,-38.8385436312631,
26.2673696829345));
#31425=CARTESIAN_POINT('Ctrl Pts',(-8.63222935586338,-38.8493408087289,
26.2658245455286));
#31426=CARTESIAN_POINT('Ctrl Pts',(-8.66200079536442,-38.8597898475114,
26.2642794081227));
#31427=CARTESIAN_POINT('Ctrl Pts',(-8.69187643515746,-38.8698885951799,
26.2627342707168));
#31428=CARTESIAN_POINT('Ctrl Pts',(-8.80447715652083,-38.9079505841522,
26.2569106770561));
#31429=CARTESIAN_POINT('Ctrl Pts',(-8.91892204726395,-38.941155419342,26.2510870833954));
#31430=CARTESIAN_POINT('Ctrl Pts',(-9.03475450883762,-38.9693231339601,
26.2452634897346));
#31431=CARTESIAN_POINT('Ctrl Pts',(-9.1504408305565,-38.9974553108224,26.2394472434023));
#31432=CARTESIAN_POINT('Ctrl Pts',(-9.26751084787404,-39.0205629115739,
26.2336309970699));
#31433=CARTESIAN_POINT('Ctrl Pts',(-9.38549053968945,-39.0385149650817,
26.2278147507376));
#31434=CARTESIAN_POINT('Ctrl Pts',(-9.50335213318378,-39.0564490484851,
26.2220043264999));
#31435=CARTESIAN_POINT('Ctrl Pts',(-9.62212118830161,-39.0692377902069,
26.2161939022621));
#31436=CARTESIAN_POINT('Ctrl Pts',(-9.74131174708171,-39.0768008766436,
26.2103834780244));
#31437=CARTESIAN_POINT('Ctrl Pts',(-9.8650139153479,-39.0846502415646,26.2043531171962));
#31438=CARTESIAN_POINT('Ctrl Pts',(-9.98916969180361,-39.0868704250354,
26.1983227563681));
#31439=CARTESIAN_POINT('Ctrl Pts',(-10.1132274744215,-39.0834304866174,
26.1922923955399));
#31440=CARTESIAN_POINT('Ctrl Pts',(-10.2326261352612,-39.0801197387399,
26.186488511317));
#31441=CARTESIAN_POINT('Ctrl Pts',(-10.3519335851697,-39.0715663581694,
26.1806846270941));
#31442=CARTESIAN_POINT('Ctrl Pts',(-10.4706569195449,-39.0577958381472,
26.1748807428712));
#31443=CARTESIAN_POINT('Ctrl Pts',(-10.5893627172164,-39.0440273521778,
26.1690777159439));
#31444=CARTESIAN_POINT('Ctrl Pts',(-10.7074841654304,-39.0250433063251,
26.1632746890167));
#31445=CARTESIAN_POINT('Ctrl Pts',(-10.8245336381544,-39.0009210539014,
26.1574716620894));
#31446=CARTESIAN_POINT('Ctrl Pts',(-10.9415934451254,-38.9767966717347,
26.1516681228155));
#31447=CARTESIAN_POINT('Ctrl Pts',(-11.0575806884786,-38.9475332634557,
26.1458645835415));
#31448=CARTESIAN_POINT('Ctrl Pts',(-11.1720187213541,-38.9132591425557,
26.1400610442675));
#31449=CARTESIAN_POINT('Ctrl Pts',(-11.2864938651518,-38.8789739069571,
26.1342556229733));
#31450=CARTESIAN_POINT('Ctrl Pts',(-11.3994184083611,-38.8396748442417,
26.1284502016791));
#31451=CARTESIAN_POINT('Ctrl Pts',(-11.510332244344,-38.7955396864866,26.1226447803849));
#31452=CARTESIAN_POINT('Ctrl Pts',(-11.6213689071394,-38.7513556531273,
26.1168329301237));
#31453=CARTESIAN_POINT('Ctrl Pts',(-11.7303900384525,-38.7023249856986,
26.1110210798625));
#31454=CARTESIAN_POINT('Ctrl Pts',(-11.8369567081506,-38.648673053643,26.1052092296012));
#31455=CARTESIAN_POINT('Ctrl Pts',(-11.943593371412,-38.5949858827091,26.0993935620854));
#31456=CARTESIAN_POINT('Ctrl Pts',(-12.0477720070184,-38.5366716013178,
26.0935778945696));
#31457=CARTESIAN_POINT('Ctrl Pts',(-12.1490808715626,-38.4740000586476,
26.0877622270538));
#31458=CARTESIAN_POINT('Ctrl Pts',(-12.2505348501211,-38.4112387457567,
26.0819382292219));
#31459=CARTESIAN_POINT('Ctrl Pts',(-12.3491105167004,-38.3441079433072,
26.0761142313901));
#31460=CARTESIAN_POINT('Ctrl Pts',(-12.4444274066281,-38.2729191333923,
26.0702902335582));
#31461=CARTESIAN_POINT('Ctrl Pts',(-12.4697154987112,-38.254032352867,26.0687450950883));
#31462=CARTESIAN_POINT('Ctrl Pts',(-12.4947744094188,-38.2348601493782,
26.0671999566183));
#31463=CARTESIAN_POINT('Ctrl Pts',(-12.5195974652232,-38.21540877856,26.0656548181484));
#31464=CARTESIAN_POINT('Ctrl Pts',(-12.6121091278228,-38.1429165492224,
26.0598963277381));
#31465=CARTESIAN_POINT('Ctrl Pts',(-12.7016553977147,-38.066298478211,26.0541378373279));
#31466=CARTESIAN_POINT('Ctrl Pts',(-12.7878402403067,-37.9858284938232,
26.0483793469177));
#31467=CARTESIAN_POINT('Ctrl Pts',(-12.8739158144014,-37.9054605324131,
26.0426281573457));
#31468=CARTESIAN_POINT('Ctrl Pts',(-12.9566381307634,-37.8212506493314,
26.0368769677737));
#31469=CARTESIAN_POINT('Ctrl Pts',(-13.0356421573583,-37.7335145312342,
26.0311257782017));
#31470=CARTESIAN_POINT('Ctrl Pts',(-13.1145677909286,-37.645865470721,26.0253802953407));
#31471=CARTESIAN_POINT('Ctrl Pts',(-13.1897821930235,-37.5546974420572,
26.0196348124797));
#31472=CARTESIAN_POINT('Ctrl Pts',(-13.2609558687923,-37.4603641644661,
26.0138893296186));
#31473=CARTESIAN_POINT('Ctrl Pts',(-13.3320794864131,-37.3660972337247,
26.0081478876931));
#31474=CARTESIAN_POINT('Ctrl Pts',(-13.3991677787653,-37.2686698146862,
26.0024064457676));
#31475=CARTESIAN_POINT('Ctrl Pts',(-13.4619308537099,-37.168469451971,25.996665003842));
#31476=CARTESIAN_POINT('Ctrl Pts',(-13.5246713353126,-37.068305159207,25.9909256287107));
#31477=CARTESIAN_POINT('Ctrl Pts',(-13.5830894723226,-36.9653702610003,
25.9851862535794));
#31478=CARTESIAN_POINT('Ctrl Pts',(-13.6369384953953,-36.8600815521669,
25.979446878448));
#31479=CARTESIAN_POINT('Ctrl Pts',(-13.6907815551996,-36.754804503059,25.973708138898));
#31480=CARTESIAN_POINT('Ctrl Pts',(-13.7400563170544,-36.6471745343663,
25.9679693993481));
#31481=CARTESIAN_POINT('Ctrl Pts',(-13.7845621812999,-36.5376326270843,
25.9622306597981));
#31482=CARTESIAN_POINT('Ctrl Pts',(-13.8290742097712,-36.4280755478458,
25.9564911254116));
#31483=CARTESIAN_POINT('Ctrl Pts',(-13.8688158713989,-36.3166063917855,
25.9507515910251));
#31484=CARTESIAN_POINT('Ctrl Pts',(-13.9036351727091,-36.2036849414976,
25.9450120566386));
#31485=CARTESIAN_POINT('Ctrl Pts',(-13.9384862376508,-36.0906604795121,
25.9392672864074));
#31486=CARTESIAN_POINT('Ctrl Pts',(-13.9684058548621,-35.9761814789232,
25.9335225161761));
#31487=CARTESIAN_POINT('Ctrl Pts',(-13.993292283104,-35.8607216400799,25.9277777459449));
#31488=CARTESIAN_POINT('Ctrl Pts',(-14.0181915929177,-35.74520203757,25.9220300021383));
#31489=CARTESIAN_POINT('Ctrl Pts',(-14.0380524566317,-35.6287009980468,
25.9162822583318));
#31490=CARTESIAN_POINT('Ctrl Pts',(-14.0528247789729,-35.5116994341827,
25.9105345145252));
#31491=CARTESIAN_POINT('Ctrl Pts',(-14.0676173085854,-35.3945378222046,
25.9047789082976));
#31492=CARTESIAN_POINT('Ctrl Pts',(-14.0773073680108,-35.2768747353253,
25.8990233020699));
#31493=CARTESIAN_POINT('Ctrl Pts',(-14.0818969247299,-35.1591932658148,
25.8932676958423));
#31494=CARTESIAN_POINT('Ctrl Pts',(-14.0839921694523,-35.1054688011184,
25.8906401210434));
#31495=CARTESIAN_POINT('Ctrl Pts',(-14.0850251129975,-35.0517404692523,
25.8880125462446));
#31496=CARTESIAN_POINT('Ctrl Pts',(-14.0849995364304,-34.9980538850391,
25.8853849714457));
#31497=CARTESIAN_POINT('Ctrl Pts',(-14.08499953643,-34.9980538841979,25.8853849714045));
#31498=CARTESIAN_POINT('Ctrl Pts',(-14.0849449953633,-34.883569313474,25.879781769463));
#31499=CARTESIAN_POINT('Ctrl Pts',(-14.080078085778,-34.7692049070056,25.8741785675215));
#31500=CARTESIAN_POINT('Ctrl Pts',(-14.0704266820107,-34.6552513576889,
25.8685753655799));
#31501=CARTESIAN_POINT('Ctrl Pts',(-14.0603956578551,-34.5368156530634,
25.8627517718956));
#31502=CARTESIAN_POINT('Ctrl Pts',(-14.0451750474139,-34.4186271289466,
25.8569281782113));
#31503=CARTESIAN_POINT('Ctrl Pts',(-14.0247820306556,-34.3011762699278,
25.851104584527));
#31504=CARTESIAN_POINT('Ctrl Pts',(-14.0044147427164,-34.18387359261,25.845288338171));
#31505=CARTESIAN_POINT('Ctrl Pts',(-13.9788880972798,-34.0673071280727,
25.839472091815));
#31506=CARTESIAN_POINT('Ctrl Pts',(-13.9482711523948,-33.9519637853742,
25.8336558454589));
#31507=CARTESIAN_POINT('Ctrl Pts',(-13.9176848552396,-33.8367359019949,
25.8278454211974));
#31508=CARTESIAN_POINT('Ctrl Pts',(-13.8820184994982,-33.7227290971593,
25.8220349969359));
#31509=CARTESIAN_POINT('Ctrl Pts',(-13.8413923561576,-33.6104210112218,
25.8162245726744));
#31510=CARTESIAN_POINT('Ctrl Pts',(-13.7992284293919,-33.4938618322967,
25.8101942118551));
#31511=CARTESIAN_POINT('Ctrl Pts',(-13.7517218964776,-33.3791329548536,
25.8041638510358));
#31512=CARTESIAN_POINT('Ctrl Pts',(-13.6990644946249,-33.2667525091306,
25.7981334902165));
#31513=CARTESIAN_POINT('Ctrl Pts',(-13.6483846971398,-33.1585926297946,
25.7923296059699));
#31514=CARTESIAN_POINT('Ctrl Pts',(-13.5929341350944,-33.0526083705815,
25.7865257217232));
#31515=CARTESIAN_POINT('Ctrl Pts',(-13.5329328695643,-32.9492415210093,
25.7807218374765));
#31516=CARTESIAN_POINT('Ctrl Pts',(-13.4729404668619,-32.8458899398248,
25.7749188105255));
#31517=CARTESIAN_POINT('Ctrl Pts',(-13.4083989023823,-32.7451553524743,
25.7691157835745));
#31518=CARTESIAN_POINT('Ctrl Pts',(-13.3395736832622,-32.6474540144638,
25.7633127566235));
#31519=CARTESIAN_POINT('Ctrl Pts',(-13.2707423875942,-32.5497440504456,
25.7575092173258));
#31520=CARTESIAN_POINT('Ctrl Pts',(-13.1976269205012,-32.4550682020675,
25.7517056780282));
#31521=CARTESIAN_POINT('Ctrl Pts',(-13.1205351353065,-32.3638123228196,
25.7459021387305));
#31522=CARTESIAN_POINT('Ctrl Pts',(-13.0434183501445,-32.2725268503538,
25.7400967174127));
#31523=CARTESIAN_POINT('Ctrl Pts',(-12.9623229457867,-32.184663864449,25.7342912960949));
#31524=CARTESIAN_POINT('Ctrl Pts',(-12.8775954891559,-32.100574332598,25.7284858747771));
#31525=CARTESIAN_POINT('Ctrl Pts',(-12.792774204709,-32.0163916793736,25.7226740244925));
#31526=CARTESIAN_POINT('Ctrl Pts',(-12.7043131294084,-31.9359911091633,
25.7168621742079));
#31527=CARTESIAN_POINT('Ctrl Pts',(-12.6125940604785,-31.8596851630525,
25.7110503239233));
#31528=CARTESIAN_POINT('Ctrl Pts',(-12.5208147499716,-31.7833290987866,
25.7052346563843));
#31529=CARTESIAN_POINT('Ctrl Pts',(-12.4257735085496,-31.7110732611334,
25.6994189888452));
#31530=CARTESIAN_POINT('Ctrl Pts',(-12.3278820701145,-31.6431875137805,
25.6936033213061));
#31531=CARTESIAN_POINT('Ctrl Pts',(-12.2298504127658,-31.5752045274259,
25.6877793234514));
#31532=CARTESIAN_POINT('Ctrl Pts',(-12.1289607539607,-31.5116043423405,
25.6819553255967));
#31533=CARTESIAN_POINT('Ctrl Pts',(-12.0256505210766,-31.4526115286789,
25.6761313277419));
#31534=CARTESIAN_POINT('Ctrl Pts',(-11.9982417555253,-31.4369604150019,
25.6745861894984));
#31535=CARTESIAN_POINT('Ctrl Pts',(-11.9706627263405,-31.4216333392667,
25.673041051255));
#31536=CARTESIAN_POINT('Ctrl Pts',(-11.9429218324976,-31.4066339244652,
25.6714959130115));
#31537=CARTESIAN_POINT('Ctrl Pts',(-11.8383669847753,-31.3501014443163,
25.6656723193424));
#31538=CARTESIAN_POINT('Ctrl Pts',(-11.7311741295239,-31.2980448797148,
25.6598487256734));
#31539=CARTESIAN_POINT('Ctrl Pts',(-11.6217629113311,-31.2507187276185,
25.6540251320044));
#31540=CARTESIAN_POINT('Ctrl Pts',(-11.5124897316419,-31.2034522844928,
25.6482088856638));
#31541=CARTESIAN_POINT('Ctrl Pts',(-11.4010041272226,-31.1609045441083,
25.6423926393232));
#31542=CARTESIAN_POINT('Ctrl Pts',(-11.287751189864,-31.1232846541171,25.6365763929826));
#31543=CARTESIAN_POINT('Ctrl Pts',(-11.1746116193209,-31.0857024218435,
25.6307659687367));
#31544=CARTESIAN_POINT('Ctrl Pts',(-11.0597086205532,-31.0530383547416,
25.6249555444908));
#31545=CARTESIAN_POINT('Ctrl Pts',(-10.943507606343,-31.0254536866741,25.6191451202449));
#31546=CARTESIAN_POINT('Ctrl Pts',(-10.8229081433312,-30.996824881849,25.6131147594198));
#31547=CARTESIAN_POINT('Ctrl Pts',(-10.7009108695577,-30.9736677832646,
25.6070843985947));
#31548=CARTESIAN_POINT('Ctrl Pts',(-10.5780542375612,-30.9561060475777,
25.6010540377696));
#31549=CARTESIAN_POINT('Ctrl Pts',(-10.4598116166339,-30.9392038614938,
25.5952501535388));
#31550=CARTESIAN_POINT('Ctrl Pts',(-10.3407734622321,-30.9274844009111,
25.589446269308));
#31551=CARTESIAN_POINT('Ctrl Pts',(-10.2214299038253,-30.9210057860188,
25.5836423850772));
#31552=CARTESIAN_POINT('Ctrl Pts',(-10.1021039737383,-30.9145281280872,
25.5778393581421));
#31553=CARTESIAN_POINT('Ctrl Pts',(-9.98247313698508,-30.9132897984763,
25.5720363312071));
#31554=CARTESIAN_POINT('Ctrl Pts',(-9.86303107899964,-30.9172969107857,
25.5662333042721));
#31555=CARTESIAN_POINT('Ctrl Pts',(-9.74357847552941,-30.9213043768812,
25.5604297649904));
#31556=CARTESIAN_POINT('Ctrl Pts',(-9.62431509209281,-30.9305581919947,
25.5546262257088));
#31557=CARTESIAN_POINT('Ctrl Pts',(-9.50573239939212,-30.9450123873199,
25.5488226864271));
#31558=CARTESIAN_POINT('Ctrl Pts',(-9.38711125170683,-30.959471269972,25.5430172651253));
#31559=CARTESIAN_POINT('Ctrl Pts',(-9.26917163888798,-30.9791338373683,
25.5372118438236));
#31560=CARTESIAN_POINT('Ctrl Pts',(-9.15239707538142,-31.0039026185317,
25.5314064225218));
#31561=CARTESIAN_POINT('Ctrl Pts',(-9.03549319485371,-31.0286988288278,
25.5255945722533));
#31562=CARTESIAN_POINT('Ctrl Pts',(-8.91975733864368,-31.0586124552982,
25.5197827219847));
#31563=CARTESIAN_POINT('Ctrl Pts',(-8.80566019442701,-31.0934954974013,
25.5139708717162));
#31564=CARTESIAN_POINT('Ctrl Pts',(-8.69148811059312,-31.1284014508739,
25.5081552041931));
#31565=CARTESIAN_POINT('Ctrl Pts',(-8.57895726625642,-31.1682831841049,
25.5023395366701));
#31566=CARTESIAN_POINT('Ctrl Pts',(-8.46851906514466,-31.2129442641843,
25.4965238691471));
#31567=CARTESIAN_POINT('Ctrl Pts',(-8.35792267323427,-31.2576693164387,
25.4906998713083));
#31568=CARTESIAN_POINT('Ctrl Pts',(-8.24942527752503,-31.307187210643,25.4848758734695));
#31569=CARTESIAN_POINT('Ctrl Pts',(-8.14345448376809,-31.3612551963405,
25.4790518756307));
#31570=CARTESIAN_POINT('Ctrl Pts',(-8.11533985412562,-31.3755997278808,
25.4775067372348));
#31571=CARTESIAN_POINT('Ctrl Pts',(-8.08740290818025,-31.3902642888718,
25.4759615988389));
#31572=CARTESIAN_POINT('Ctrl Pts',(-8.05965128011236,-31.4052438406437,
25.474416460443));
#31573=CARTESIAN_POINT('Ctrl Pts',(-7.95507361046443,-31.4616919384936,
25.4685938480784));
#31574=CARTESIAN_POINT('Ctrl Pts',(-7.852792633018,-31.5227983519528,25.4627712357138));
#31575=CARTESIAN_POINT('Ctrl Pts',(-7.75325101340967,-31.5883517192924,
25.4569486233492));
#31576=CARTESIAN_POINT('Ctrl Pts',(-7.67116836825394,-31.6424074380085,
25.4521472605978));
#31577=CARTESIAN_POINT('Ctrl Pts',(-7.59094821434825,-31.699486039335,25.4473458978464));
#31578=CARTESIAN_POINT('Ctrl Pts',(-7.5128274573098,-31.7594448403263,25.442544535095));
#31579=CARTESIAN_POINT('',(-14.0849990113761,-35.0028420162714,25.9896150286377));
#31580=CARTESIAN_POINT('Ctrl Pts',(-14.0849990113767,-35.0028420154021,
25.9896150285955));
#31581=CARTESIAN_POINT('Ctrl Pts',(-14.0850823687409,-34.8830274816084,
25.9837992556086));
#31582=CARTESIAN_POINT('Ctrl Pts',(-14.079890102243,-34.7631670279784,25.9779834826216));
#31583=CARTESIAN_POINT('Ctrl Pts',(-14.0694367788947,-34.6437566806534,
25.9721677096347));
#31584=CARTESIAN_POINT('Ctrl Pts',(-14.0589841763813,-34.5243545675665,
25.9663523376888));
#31585=CARTESIAN_POINT('Ctrl Pts',(-14.0432712736033,-34.4054029029652,
25.960536965743));
#31586=CARTESIAN_POINT('Ctrl Pts',(-14.0223646062431,-34.2873935346609,
25.9547215937972));
#31587=CARTESIAN_POINT('Ctrl Pts',(-14.0014545368584,-34.1693649633554,
25.9489052755486));
#31588=CARTESIAN_POINT('Ctrl Pts',(-13.9753490922789,-34.0522793926447,
25.9430889573));
#31589=CARTESIAN_POINT('Ctrl Pts',(-13.9441660016668,-33.9366188118573,
25.9372726390513));
#31590=CARTESIAN_POINT('Ctrl Pts',(-13.9129706122758,-33.8209126139139,
25.9314540268155));
#31591=CARTESIAN_POINT('Ctrl Pts',(-13.8766936982193,-33.7066329152009,
25.9256354145796));
#31592=CARTESIAN_POINT('Ctrl Pts',(-13.8355027712762,-33.5942462905856,
25.9198168023438));
#31593=CARTESIAN_POINT('Ctrl Pts',(-13.7942616422543,-33.4817226930344,
25.9139910985843));
#31594=CARTESIAN_POINT('Ctrl Pts',(-13.7480946838732,-33.3710971564586,
25.9081653948248));
#31595=CARTESIAN_POINT('Ctrl Pts',(-13.6972175587036,-33.2628162665931,
25.9023396910654));
#31596=CARTESIAN_POINT('Ctrl Pts',(-13.6463043684081,-33.1544586199548,
25.8965098576555));
#31597=CARTESIAN_POINT('Ctrl Pts',(-13.5906745492271,-33.0484492884319,
25.8906800242457));
#31598=CARTESIAN_POINT('Ctrl Pts',(-13.5305888844623,-32.9452087383602,
25.8848501908358));
#31599=CARTESIAN_POINT('Ctrl Pts',(-13.4704104788133,-32.8418088388009,
25.8790113592081));
#31600=CARTESIAN_POINT('Ctrl Pts',(-13.405762716197,-32.741186592108,25.8731725275803));
#31601=CARTESIAN_POINT('Ctrl Pts',(-13.3369488314327,-32.6437322952601,
25.8673336959526));
#31602=CARTESIAN_POINT('Ctrl Pts',(-13.3133690745061,-32.6103386184028,
25.865332962656));
#31603=CARTESIAN_POINT('Ctrl Pts',(-13.2893004869779,-32.5773166103989,
25.8633322293594));
#31604=CARTESIAN_POINT('Ctrl Pts',(-13.2647562933768,-32.5446810095516,
25.8613314960627));
#31605=CARTESIAN_POINT('Ctrl Pts',(-13.1933147821542,-32.4496875996201,
25.855507902402));
#31606=CARTESIAN_POINT('Ctrl Pts',(-13.1176086426052,-32.3576616547356,
25.8496843087413));
#31607=CARTESIAN_POINT('Ctrl Pts',(-13.0379131029185,-32.2690095241623,
25.8438607150805));
#31608=CARTESIAN_POINT('Ctrl Pts',(-12.9583181109923,-32.1804692414192,
25.8380444687481));
#31609=CARTESIAN_POINT('Ctrl Pts',(-12.8747440004701,-32.0952946077671,
25.8322282224158));
#31610=CARTESIAN_POINT('Ctrl Pts',(-12.7875080441697,-32.0138613723256,
25.8264119760834));
#31611=CARTESIAN_POINT('Ctrl Pts',(-12.7003594115419,-31.9325096520013,
25.8206015518457));
#31612=CARTESIAN_POINT('Ctrl Pts',(-12.6095565220285,-31.8548921563931,
25.8147911276079));
#31613=CARTESIAN_POINT('Ctrl Pts',(-12.5154551039248,-31.7813495654019,
25.8089807033701));
#31614=CARTESIAN_POINT('Ctrl Pts',(-12.4177917522681,-31.7050232350398,
25.802950342542));
#31615=CARTESIAN_POINT('Ctrl Pts',(-12.3165755254786,-31.633086725002,25.7969199817138));
#31616=CARTESIAN_POINT('Ctrl Pts',(-12.2122442084415,-31.5658770315818,
25.7908896208857));
#31617=CARTESIAN_POINT('Ctrl Pts',(-12.1118311648171,-31.5011914695758,
25.7850857366627));
#31618=CARTESIAN_POINT('Ctrl Pts',(-12.0085331665854,-31.4408843266798,
25.7792818524398));
#31619=CARTESIAN_POINT('Ctrl Pts',(-11.9027714187935,-31.3852128793216,
25.7734779682169));
#31620=CARTESIAN_POINT('Ctrl Pts',(-11.7970252931406,-31.3295496552303,
25.7676749412896));
#31621=CARTESIAN_POINT('Ctrl Pts',(-11.6888165028904,-31.2785209550916,
25.7618719143624));
#31622=CARTESIAN_POINT('Ctrl Pts',(-11.5785911791187,-31.2323382729857,
25.7560688874351));
#31623=CARTESIAN_POINT('Ctrl Pts',(-11.4683561236013,-31.1861515134309,
25.7502653481611));
#31624=CARTESIAN_POINT('Ctrl Pts',(-11.3561045572124,-31.1448117803874,
25.7444618088871));
#31625=CARTESIAN_POINT('Ctrl Pts',(-11.2423023240401,-31.108482309473,25.7386582696131));
#31626=CARTESIAN_POINT('Ctrl Pts',(-11.1284631861273,-31.0721410573337,
25.7328528483189));
#31627=CARTESIAN_POINT('Ctrl Pts',(-11.0130727701459,-31.0408134227405,
25.7270474270246));
#31628=CARTESIAN_POINT('Ctrl Pts',(-10.8966111730242,-31.0146125151489,
25.7212420057303));
#31629=CARTESIAN_POINT('Ctrl Pts',(-10.7800206054583,-30.988382592476,25.7154301554691));
#31630=CARTESIAN_POINT('Ctrl Pts',(-10.6623568875434,-30.9672908190116,
25.7096183052078));
#31631=CARTESIAN_POINT('Ctrl Pts',(-10.5441095368113,-30.9513990302882,
25.7038064549466));
#31632=CARTESIAN_POINT('Ctrl Pts',(-10.4257845205817,-30.9354968037523,
25.6979907874307));
#31633=CARTESIAN_POINT('Ctrl Pts',(-10.3068755138776,-30.9248014002655,
25.6921751199149));
#31634=CARTESIAN_POINT('Ctrl Pts',(-10.1878747114574,-30.9193225938829,
25.6863594523991));
#31635=CARTESIAN_POINT('Ctrl Pts',(-10.0687034532317,-30.9138359397015,
25.6805354545672));
#31636=CARTESIAN_POINT('Ctrl Pts',(-9.94944054373476,-30.9135807976243,
25.6747114567353));
#31637=CARTESIAN_POINT('Ctrl Pts',(-9.83057587023469,-30.9185149192661,
25.6688874589035));
#31638=CARTESIAN_POINT('Ctrl Pts',(-9.79904042241721,-30.9198239687169,
25.6673423204337));
#31639=CARTESIAN_POINT('Ctrl Pts',(-9.76753296246046,-30.9214979935786,
25.665797181964));
#31640=CARTESIAN_POINT('Ctrl Pts',(-9.73606253046786,-30.9235355990544,
25.6642520434943));
#31641=CARTESIAN_POINT('Ctrl Pts',(-9.61746471748103,-30.9312144117639,
25.6584291160139));
#31642=CARTESIAN_POINT('Ctrl Pts',(-9.49901105975285,-30.9440855036799,
25.6526061885334));
#31643=CARTESIAN_POINT('Ctrl Pts',(-9.38119211766201,-30.9621414332896,
25.646783261053));
#31644=CARTESIAN_POINT('Ctrl Pts',(-9.26351389261787,-30.9801757978009,
25.6409672881857));
#31645=CARTESIAN_POINT('Ctrl Pts',(-9.14646927572767,-31.0033826255236,
25.6351513153183));
#31646=CARTESIAN_POINT('Ctrl Pts',(-9.03054638179244,-31.0317025461611,
25.629335342451));
#31647=CARTESIAN_POINT('Ctrl Pts',(-8.91473456843547,-31.0599953298539,
25.6235249426125));
#31648=CARTESIAN_POINT('Ctrl Pts',(-8.80004273454173,-31.093391365418,25.617714542774));
#31649=CARTESIAN_POINT('Ctrl Pts',(-8.68695080781059,-31.1317798900669,
25.6119041429355));
#31650=CARTESIAN_POINT('Ctrl Pts',(-8.57394311493053,-31.1701398219297,
25.6060980708361));
#31651=CARTESIAN_POINT('Ctrl Pts',(-8.46253334325251,-31.2134847125031,
25.6002919987367));
#31652=CARTESIAN_POINT('Ctrl Pts',(-8.35318755702693,-31.2616536038418,
25.5944859266373));
#31653=CARTESIAN_POINT('Ctrl Pts',(-8.2438906130624,-31.3098009792388,25.5886824479775));
#31654=CARTESIAN_POINT('Ctrl Pts',(-8.13665619309796,-31.3627679035355,
25.5828789693176));
#31655=CARTESIAN_POINT('Ctrl Pts',(-8.03193110999552,-31.4203450104519,
25.5770754906578));
#31656=CARTESIAN_POINT('Ctrl Pts',(-7.92720867010922,-31.4779206641469,
25.5712721584753));
#31657=CARTESIAN_POINT('Ctrl Pts',(-7.82499580308749,-31.5401060801663,
25.5654688262928));
#31658=CARTESIAN_POINT('Ctrl Pts',(-7.72571506550866,-31.6066457543095,
25.5596654941103));
#31659=CARTESIAN_POINT('Ctrl Pts',(-7.65313415233258,-31.6552907425472,
25.5554228669951));
#31660=CARTESIAN_POINT('Ctrl Pts',(-7.5821198585115,-31.7062619290058,25.5511802398798));
#31661=CARTESIAN_POINT('Ctrl Pts',(-7.5128274573098,-31.7594448403263,25.5469376127646));
#31662=CARTESIAN_POINT('Ctrl Pts',(-7.5128274573098,-31.7594448403263,26.796772721093));
#31663=CARTESIAN_POINT('Ctrl Pts',(-7.41816755880118,-31.8320976695064,
26.7909660993717));
#31664=CARTESIAN_POINT('Ctrl Pts',(-7.32661924854595,-31.9089587491885,
26.7851594776504));
#31665=CARTESIAN_POINT('Ctrl Pts',(-7.23857278924136,-31.9897267965047,
26.7793528559291));
#31666=CARTESIAN_POINT('Ctrl Pts',(-7.15056342287312,-32.0704608171938,
26.7735486804691));
#31667=CARTESIAN_POINT('Ctrl Pts',(-7.0660532747713,-32.1550982576077,26.7677445050092));
#31668=CARTESIAN_POINT('Ctrl Pts',(-6.98539899898841,-32.243298020333,26.7619403295492));
#31669=CARTESIAN_POINT('Ctrl Pts',(-6.90475998799386,-32.3314810901961,
26.756137252599));
#31670=CARTESIAN_POINT('Ctrl Pts',(-6.8279756735518,-32.4232248404266,26.7503341756489));
#31671=CARTESIAN_POINT('Ctrl Pts',(-6.75536488494574,-32.5181523072201,
26.7445310986987));
#31672=CARTESIAN_POINT('Ctrl Pts',(-6.68275070259049,-32.6130842108201,
26.738727750519));
#31673=CARTESIAN_POINT('Ctrl Pts',(-6.61431068192869,-32.7111998024259,
26.7329244023393));
#31674=CARTESIAN_POINT('Ctrl Pts',(-6.55032209091048,-32.8120906500635,
26.7271210541596));
#31675=CARTESIAN_POINT('Ctrl Pts',(-6.48631540787171,-32.9130100234001,
26.7213160651516));
#31676=CARTESIAN_POINT('Ctrl Pts',(-6.42676287608266,-33.0167058685485,
26.7155110761436));
#31677=CARTESIAN_POINT('Ctrl Pts',(-6.37189698958961,-33.1227430794238,
26.7097060871355));
#31678=CARTESIAN_POINT('Ctrl Pts',(-6.31697141161673,-33.2288956537506,
26.703894782575));
#31679=CARTESIAN_POINT('Ctrl Pts',(-6.26674284636288,-33.3373943163327,
26.6980834780146));
#31680=CARTESIAN_POINT('Ctrl Pts',(-6.22139666957394,-33.4477816289925,
26.6922721734541));
#31681=CARTESIAN_POINT('Ctrl Pts',(-6.17602239898176,-33.5582373310881,
26.6864572685537));
#31682=CARTESIAN_POINT('Ctrl Pts',(-6.13553667971406,-33.6705836302412,
26.6806423636534));
#31683=CARTESIAN_POINT('Ctrl Pts',(-6.10007525591783,-33.7843470929185,
26.6748274587531));
#31684=CARTESIAN_POINT('Ctrl Pts',(-6.06456135891672,-33.8982788943946,
26.6690039493845));
#31685=CARTESIAN_POINT('Ctrl Pts',(-6.0340867052915,-34.0136316523845,26.6631804400158));
#31686=CARTESIAN_POINT('Ctrl Pts',(-6.00873617634326,-34.1299206415683,
26.6573569306472));
#31687=CARTESIAN_POINT('Ctrl Pts',(-5.99755206376073,-34.1812248628646,
26.6547877225436));
#31688=CARTESIAN_POINT('Ctrl Pts',(-5.98736462608227,-34.2327112275932,
26.6522185144401));
#31689=CARTESIAN_POINT('Ctrl Pts',(-5.97817793786512,-34.2843378586755,
26.6496493063365));
#31690=CARTESIAN_POINT('Ctrl Pts',(-5.95735457765622,-34.4013593478113,
26.6438257119652));
#31691=CARTESIAN_POINT('Ctrl Pts',(-5.94160927488649,-34.5194791313175,
26.6380021175938));
#31692=CARTESIAN_POINT('Ctrl Pts',(-5.93105180598832,-34.6382188583562,
26.6321785232225));
#31693=CARTESIAN_POINT('Ctrl Pts',(-5.92050765688948,-34.7568087777705,
26.6263622761718));
#31694=CARTESIAN_POINT('Ctrl Pts',(-5.9151383592276,-34.8760166818923,26.620546029121));
#31695=CARTESIAN_POINT('Ctrl Pts',(-5.91500264167212,-34.9953543079937,
26.6147297820702));
#31696=CARTESIAN_POINT('Ctrl Pts',(-5.91486705997048,-35.1145724766296,
26.6089193571072));
#31697=CARTESIAN_POINT('Ctrl Pts',(-5.91995463682205,-35.2339197029306,
26.6031089321442));
#31698=CARTESIAN_POINT('Ctrl Pts',(-5.9302722289381,-35.3529034846067,26.5972985071812));
#31699=CARTESIAN_POINT('Ctrl Pts',(-5.94098036146807,-35.4763910278991,
26.5912681466223));
#31700=CARTESIAN_POINT('Ctrl Pts',(-5.95732230389187,-35.5994866223381,
26.5852377860635));
#31701=CARTESIAN_POINT('Ctrl Pts',(-5.97924629213039,-35.7216402293753,
26.5792074255046));
#31702=CARTESIAN_POINT('Ctrl Pts',(-6.00034690533139,-35.8392062481651,
26.5734035405439));
#31703=CARTESIAN_POINT('Ctrl Pts',(-6.02661776934589,-35.9558993199064,
26.5675996555832));
#31704=CARTESIAN_POINT('Ctrl Pts',(-6.05796008286243,-36.0712358711759,
26.5617957706225));
#31705=CARTESIAN_POINT('Ctrl Pts',(-6.0892977668033,-36.1865553860741,26.5559927429542));
#31706=CARTESIAN_POINT('Ctrl Pts',(-6.12570530346265,-36.3005183850366,
26.5501897152858));
#31707=CARTESIAN_POINT('Ctrl Pts',(-6.1670334008828,-36.412654257082,26.5443866876175));
#31708=CARTESIAN_POINT('Ctrl Pts',(-6.20836514716021,-36.5248000296023,
26.5385831475999));
#31709=CARTESIAN_POINT('Ctrl Pts',(-6.25461817674669,-36.6351179713057,
26.5327796075822));
#31710=CARTESIAN_POINT('Ctrl Pts',(-6.30559444797943,-36.7431559359964,
26.5269760675646));
#31711=CARTESIAN_POINT('Ctrl Pts',(-6.35658725023713,-36.8512289361702,
26.521170645525));
#31712=CARTESIAN_POINT('Ctrl Pts',(-6.41230616617751,-36.957020119787,26.5153652234854));
#31713=CARTESIAN_POINT('Ctrl Pts',(-6.47250675904511,-37.060101073981,26.5095598014457));
#31714=CARTESIAN_POINT('Ctrl Pts',(-6.53277401847907,-37.1632961807596,
26.5037479504403));
#31715=CARTESIAN_POINT('Ctrl Pts',(-6.59753265544521,-37.2637747143913,
26.4979360994349));
#31716=CARTESIAN_POINT('Ctrl Pts',(-6.66649429157606,-37.3611363137068,
26.4921242484294));
#31717=CARTESIAN_POINT('Ctrl Pts',(-6.73550122207792,-37.4585618606409,
26.4863085801692));
#31718=CARTESIAN_POINT('Ctrl Pts',(-6.80871639961766,-37.5528660743705,
26.480492911909));
#31719=CARTESIAN_POINT('Ctrl Pts',(-6.88581152381396,-37.6436821168193,
26.4746772436487));
#31720=CARTESIAN_POINT('Ctrl Pts',(-6.96301707836893,-37.734628243346,26.4688532450779));
#31721=CARTESIAN_POINT('Ctrl Pts',(-7.04411339557444,-37.8220759276561,
26.463029246507));
#31722=CARTESIAN_POINT('Ctrl Pts',(-7.12873567890862,-37.905695475859,26.4572052479362));
#31723=CARTESIAN_POINT('Ctrl Pts',(-7.15118632765622,-37.9278800947463,
26.4556601165468));
#31724=CARTESIAN_POINT('Ctrl Pts',(-7.17388497955515,-37.9497954881707,
26.4541149851574));
#31725=CARTESIAN_POINT('Ctrl Pts',(-7.19682445279163,-37.9714359914918,
26.452569853768));
#31726=CARTESIAN_POINT('Ctrl Pts',(-7.28328323016378,-38.0529989567602,
26.4467462601123));
#31727=CARTESIAN_POINT('Ctrl Pts',(-7.37344419473058,-38.1309168275642,
26.4409226664566));
#31728=CARTESIAN_POINT('Ctrl Pts',(-7.46696744324481,-38.2048355755667,
26.4350990728009));
#31729=CARTESIAN_POINT('Ctrl Pts',(-7.56037269831285,-38.2786610641076,
26.4292828264721));
#31730=CARTESIAN_POINT('Ctrl Pts',(-7.65713148251871,-38.3484972142308,
26.4234665801434));
#31731=CARTESIAN_POINT('Ctrl Pts',(-7.75686762006312,-38.4140272591294,
26.4176503338146));
#31732=CARTESIAN_POINT('Ctrl Pts',(-7.85650392120851,-38.4794917081079,
26.4118399095791));
#31733=CARTESIAN_POINT('Ctrl Pts',(-7.95911130735749,-38.5406584040014,
26.4060294853436));
#31734=CARTESIAN_POINT('Ctrl Pts',(-8.0642816225373,-38.5972516402322,26.400219061108));
#31735=CARTESIAN_POINT('Ctrl Pts',(-8.1734328520136,-38.6559870476907,26.3941887002785));
#31736=CARTESIAN_POINT('Ctrl Pts',(-8.28534451683555,-38.7097956467526,
26.388158339449));
#31737=CARTESIAN_POINT('Ctrl Pts',(-8.39952820533579,-38.7584192201622,
26.3821279786195));
#31738=CARTESIAN_POINT('Ctrl Pts',(-8.50942360415092,-38.8052166836339,
26.3763240943952));
#31739=CARTESIAN_POINT('Ctrl Pts',(-8.6214230382177,-38.8472113819989,26.3705202101709));
#31740=CARTESIAN_POINT('Ctrl Pts',(-8.73506790151208,-38.8842208724807,
26.3647163259466));
#31741=CARTESIAN_POINT('Ctrl Pts',(-8.84869597827336,-38.9212248962743,
26.3589132990166));
#31742=CARTESIAN_POINT('Ctrl Pts',(-8.96396861275618,-38.953245050178,26.3531102720866));
#31743=CARTESIAN_POINT('Ctrl Pts',(-9.08041036321069,-38.9801482258717,
26.3473072451566));
#31744=CARTESIAN_POINT('Ctrl Pts',(-9.19686239428267,-39.0070537768411,
26.3415037058786));
#31745=CARTESIAN_POINT('Ctrl Pts',(-9.31448334867906,-39.028841359432,26.3357001666006));
#31746=CARTESIAN_POINT('Ctrl Pts',(-9.43278650524778,-39.0454287598932,
26.3298966273226));
#31747=CARTESIAN_POINT('Ctrl Pts',(-9.5511280261813,-39.0620215394592,26.3240912060229));
#31748=CARTESIAN_POINT('Ctrl Pts',(-9.67015178509111,-39.0734107264371,
26.3182857847233));
#31749=CARTESIAN_POINT('Ctrl Pts',(-9.78936547859593,-39.0795659203392,
26.3124803634237));
#31750=CARTESIAN_POINT('Ctrl Pts',(-9.9087111902775,-39.0857279305512,26.3066685131551));
#31751=CARTESIAN_POINT('Ctrl Pts',(-10.0282468483653,-39.0866443569785,
26.3008566628865));
#31752=CARTESIAN_POINT('Ctrl Pts',(-10.1474795239155,-39.0823369275484,
26.2950448126179));
#31753=CARTESIAN_POINT('Ctrl Pts',(-10.266790512154,-39.0780266689746,26.2892291450936));
#31754=CARTESIAN_POINT('Ctrl Pts',(-10.3857977154447,-39.0684857540623,
26.2834134775692));
#31755=CARTESIAN_POINT('Ctrl Pts',(-10.5040143587992,-39.0537876764977,
26.2775978100449));
#31756=CARTESIAN_POINT('Ctrl Pts',(-10.6224003347691,-39.0390685455192,
26.2717738122029));
#31757=CARTESIAN_POINT('Ctrl Pts',(-10.7399930894212,-39.0191775755394,
26.2659498143608));
#31758=CARTESIAN_POINT('Ctrl Pts',(-10.8563169082389,-38.9942391456527,
26.2601258165188));
#31759=CARTESIAN_POINT('Ctrl Pts',(-10.8871782527635,-38.9876228439833,
26.2585806780791));
#31760=CARTESIAN_POINT('Ctrl Pts',(-10.9179503703753,-38.9806515367974,
26.2570355396394));
#31761=CARTESIAN_POINT('Ctrl Pts',(-10.9486245864041,-38.9733281256485,
26.2554904011996));
#31762=CARTESIAN_POINT('Ctrl Pts',(-11.064235046025,-38.9457263467434,26.2496668076959));
#31763=CARTESIAN_POINT('Ctrl Pts',(-11.1788262582109,-38.9130300575665,
26.2438432141922));
#31764=CARTESIAN_POINT('Ctrl Pts',(-11.2919158013149,-38.8753294779041,
26.2380196206885));
#31765=CARTESIAN_POINT('Ctrl Pts',(-11.4048626651036,-38.8376764631426,
26.232203374516));
#31766=CARTESIAN_POINT('Ctrl Pts',(-11.5163112441204,-38.7950318436155,
26.2263871283435));
#31767=CARTESIAN_POINT('Ctrl Pts',(-11.6257903978905,-38.7475366018395,
26.2205708821711));
#31768=CARTESIAN_POINT('Ctrl Pts',(-11.7351599623722,-38.700088903085,26.2147604580959));
#31769=CARTESIAN_POINT('Ctrl Pts',(-11.8425636510252,-38.6478004030813,
26.2089500340206));
#31770=CARTESIAN_POINT('Ctrl Pts',(-11.9475471345948,-38.5908613393629,
26.2031396099454));
#31771=CARTESIAN_POINT('Ctrl Pts',(-12.056504464562,-38.5317670119255,26.1971092490573));
#31772=CARTESIAN_POINT('Ctrl Pts',(-12.1628543243545,-38.4676632389247,
26.1910788881692));
#31773=CARTESIAN_POINT('Ctrl Pts',(-12.2661130189758,-38.3988169684801,
26.1850485272811));
#31774=CARTESIAN_POINT('Ctrl Pts',(-12.3654937197915,-38.3325562954159,
26.1792446432263));
#31775=CARTESIAN_POINT('Ctrl Pts',(-12.4620108822091,-38.261903167245,26.1734407591716));
#31776=CARTESIAN_POINT('Ctrl Pts',(-12.5552605252404,-38.187141140293,26.1676368751168));
#31777=CARTESIAN_POINT('Ctrl Pts',(-12.6484963942748,-38.1123901565138,
26.1618338483594));
#31778=CARTESIAN_POINT('Ctrl Pts',(-12.7384653852574,-38.0335317362996,
26.1560308216021));
#31779=CARTESIAN_POINT('Ctrl Pts',(-12.8247955503814,-37.9508905602454,
26.1502277948447));
#31780=CARTESIAN_POINT('Ctrl Pts',(-12.9111333375348,-37.8682420878601,
26.1444242557423));
#31781=CARTESIAN_POINT('Ctrl Pts',(-12.9938313650825,-37.7818104779888,
26.1386207166398));
#31782=CARTESIAN_POINT('Ctrl Pts',(-13.0725540690073,-37.6919577435441,
26.1328171775373));
#31783=CARTESIAN_POINT('Ctrl Pts',(-13.1513023017699,-37.6020758709247,
26.127011756416));
#31784=CARTESIAN_POINT('Ctrl Pts',(-13.2260723781308,-37.5087709743006,
26.1212063352947));
#31785=CARTESIAN_POINT('Ctrl Pts',(-13.2965690092148,-37.4124381375456,
26.1154009141734));
#31786=CARTESIAN_POINT('Ctrl Pts',(-13.3671437087831,-37.3159986211034,
26.1095890640864));
#31787=CARTESIAN_POINT('Ctrl Pts',(-13.4334352754196,-37.2165248010505,
26.1037772139993));
#31788=CARTESIAN_POINT('Ctrl Pts',(-13.4951916760395,-37.114440859363,26.0979653639123));
#31789=CARTESIAN_POINT('Ctrl Pts',(-13.5569886385876,-37.0122898684067,
26.0921496965716));
#31790=CARTESIAN_POINT('Ctrl Pts',(-13.6142443075444,-36.9075256991544,
26.0863340292309));
#31791=CARTESIAN_POINT('Ctrl Pts',(-13.6667533185855,-36.8005957626969,
26.0805183618902));
#31792=CARTESIAN_POINT('Ctrl Pts',(-13.7193375431195,-36.6935126606428,
26.0746943642335));
#31793=CARTESIAN_POINT('Ctrl Pts',(-13.7671613759936,-36.5842579722473,
26.0688703665769));
#31794=CARTESIAN_POINT('Ctrl Pts',(-13.8100680749183,-36.4732977514706,
26.0630463689202));
#31795=CARTESIAN_POINT('Ctrl Pts',(-13.8214514690779,-36.4438593663049,
26.0615012288239));
#31796=CARTESIAN_POINT('Ctrl Pts',(-13.8324890351795,-36.4143010065942,
26.0599560887275));
#31797=CARTESIAN_POINT('Ctrl Pts',(-13.8431784448527,-36.3846315181374,
26.0584109486312));
#31798=CARTESIAN_POINT('Ctrl Pts',(-13.8896767283399,-36.2555710435782,
26.0516896829651));
#31799=CARTESIAN_POINT('Ctrl Pts',(-13.9297065577542,-36.1240650714574,
26.044968417299));
#31800=CARTESIAN_POINT('Ctrl Pts',(-13.963040544028,-35.9907243039264,26.0382471516329));
#31801=CARTESIAN_POINT('Ctrl Pts',(-13.9962417189144,-35.8579148011589,
26.0315526652608));
#31802=CARTESIAN_POINT('Ctrl Pts',(-14.0228002009898,-35.7232852282394,
26.0248581788888));
#31803=CARTESIAN_POINT('Ctrl Pts',(-14.0425382248911,-35.5874603818931,
26.0181636925167));
#31804=CARTESIAN_POINT('Ctrl Pts',(-14.0621325522581,-35.4526243660297,
26.0115179432672));
#31805=CARTESIAN_POINT('Ctrl Pts',(-14.0750052824874,-35.3166105657448,
26.0048721940178));
#31806=CARTESIAN_POINT('Ctrl Pts',(-14.0810301740175,-35.1800492120466,
25.9982264447683));
#31807=CARTESIAN_POINT('Ctrl Pts',(-14.0836324814554,-35.1210648096409,
25.9953559727248));
#31808=CARTESIAN_POINT('Ctrl Pts',(-14.084957868942,-35.0619784836735,25.9924855006812));
#31809=CARTESIAN_POINT('Ctrl Pts',(-14.0849990113761,-35.0028420162714,
25.9896150286377));
#31810=CARTESIAN_POINT('Origin',(-10.,-35.,32.7603849714045));
#31811=CARTESIAN_POINT('',(-7.5128274573098,-31.7594448403263,28.0469627561459));
#31812=CARTESIAN_POINT('',(-7.5128274573098,-31.7594448403263,27.9426390119128));
#31813=CARTESIAN_POINT('',(-7.5128274573098,-31.7594448403263,32.7603849714045));
#31814=CARTESIAN_POINT('',(-14.0849997205636,-34.9984890415501,27.1353849713726));
#31815=CARTESIAN_POINT('Ctrl Pts',(-7.5128274573098,-31.7594448403263,27.9426390119128));
#31816=CARTESIAN_POINT('Ctrl Pts',(-7.41802049582305,-31.8322105424504,
27.9368359551733));
#31817=CARTESIAN_POINT('Ctrl Pts',(-7.32640238267038,-31.9091456963177,
27.9310328984338));
#31818=CARTESIAN_POINT('Ctrl Pts',(-7.23834991095762,-31.98993126562,27.9252298416944));
#31819=CARTESIAN_POINT('Ctrl Pts',(-7.15028255297934,-32.0707304926358,
27.9194258038826));
#31820=CARTESIAN_POINT('Ctrl Pts',(-7.06578233601788,-32.1553811534852,
27.9136217660707));
#31821=CARTESIAN_POINT('Ctrl Pts',(-6.98519017205803,-32.243526401116,27.9078177282589));
#31822=CARTESIAN_POINT('Ctrl Pts',(-6.90451492792515,-32.3317625151792,
27.9020077072294));
#31823=CARTESIAN_POINT('Ctrl Pts',(-6.82775606013463,-32.4235001100291,
27.8961976861998));
#31824=CARTESIAN_POINT('Ctrl Pts',(-6.75521520865047,-32.5183479982425,
27.8903876651703));
#31825=CARTESIAN_POINT('Ctrl Pts',(-6.68263681144322,-32.6132449778641,
27.8845746369877));
#31826=CARTESIAN_POINT('Ctrl Pts',(-6.6142810139752,-32.7112551234008,27.8787616088051));
#31827=CARTESIAN_POINT('Ctrl Pts',(-6.55040599104204,-32.811958370286,27.8729485806225));
#31828=CARTESIAN_POINT('Ctrl Pts',(-6.48642767990506,-32.9128244579346,
27.8671261525648));
#31829=CARTESIAN_POINT('Ctrl Pts',(-6.42694482512305,-33.0163919944017,
27.8613037245071));
#31830=CARTESIAN_POINT('Ctrl Pts',(-6.37216980895975,-33.1222159056545,
27.8554812964494));
#31831=CARTESIAN_POINT('Ctrl Pts',(-6.32164664401443,-33.2198253505782,
27.8501108280544));
#31832=CARTESIAN_POINT('Ctrl Pts',(-6.2751283719363,-33.319353988852,27.8447403596593));
#31833=CARTESIAN_POINT('Ctrl Pts',(-6.23274456499622,-33.4204394638272,
27.8393698912643));
#31834=CARTESIAN_POINT('Ctrl Pts',(-6.18678478500024,-33.5300536425917,
27.8335463099551));
#31835=CARTESIAN_POINT('Ctrl Pts',(-6.14553895250771,-33.641852162612,27.8277227286458));
#31836=CARTESIAN_POINT('Ctrl Pts',(-6.10921899689708,-33.7553923566467,
27.8218991473366));
#31837=CARTESIAN_POINT('Ctrl Pts',(-6.07294486555298,-33.8687892989613,
27.8160829135402));
#31838=CARTESIAN_POINT('Ctrl Pts',(-6.04158437312784,-33.9839231591374,
27.8102666797439));
#31839=CARTESIAN_POINT('Ctrl Pts',(-6.01530181397272,-34.1003304127231,
27.8044504459475));
#31840=CARTESIAN_POINT('Ctrl Pts',(-5.98904556462065,-34.2166211383903,
27.798640034414));
#31841=CARTESIAN_POINT('Ctrl Pts',(-5.96785722556352,-34.3341823255599,
27.7928296228804));
#31842=CARTESIAN_POINT('Ctrl Pts',(-5.95185140895948,-34.4525349464517,
27.7870192113468));
#31843=CARTESIAN_POINT('Ctrl Pts',(-5.93523968978527,-34.5753678234253,
27.7809888458197));
#31844=CARTESIAN_POINT('Ctrl Pts',(-5.9242107531769,-34.6990528109013,27.7749584802926));
#31845=CARTESIAN_POINT('Ctrl Pts',(-5.91883462375985,-34.8230418925887,
27.7689281147654));
#31846=CARTESIAN_POINT('Ctrl Pts',(-5.91366041625262,-34.9423740714693,
27.7631242435858));
#31847=CARTESIAN_POINT('Ctrl Pts',(-5.9137220661502,-35.0619874689632,27.7573203724061));
#31848=CARTESIAN_POINT('Ctrl Pts',(-5.91902913880518,-35.1813886161775,
27.7515165012264));
#31849=CARTESIAN_POINT('Ctrl Pts',(-5.92433542745309,-35.3007721244129,
27.7457134874453));
#31850=CARTESIAN_POINT('Ctrl Pts',(-5.93488557970118,-35.4199430368987,
27.7399104736641));
#31851=CARTESIAN_POINT('Ctrl Pts',(-5.95063705693842,-35.5384094681185,
27.7341074598829));
#31852=CARTESIAN_POINT('Ctrl Pts',(-5.96638992462875,-35.6568863568982,
27.7283039338438));
#31853=CARTESIAN_POINT('Ctrl Pts',(-5.98734497637511,-35.7746582359709,
27.7225004078047));
#31854=CARTESIAN_POINT('Ctrl Pts',(-6.0134080625052,-35.8912405533309,27.7166968817657));
#31855=CARTESIAN_POINT('Ctrl Pts',(-6.0394796002739,-36.007860675562,27.7108914737812));
#31856=CARTESIAN_POINT('Ctrl Pts',(-6.07066237761633,-36.1232900706205,
27.7050860657967));
#31857=CARTESIAN_POINT('Ctrl Pts',(-6.10681177669693,-36.2370571765017,
27.6992806578123));
#31858=CARTESIAN_POINT('Ctrl Pts',(-6.14300120770635,-36.3509502683411,
27.6934688209055));
#31859=CARTESIAN_POINT('Ctrl Pts',(-6.18416811529114,-36.4631770071668,
27.6876569839987));
#31860=CARTESIAN_POINT('Ctrl Pts',(-6.23011886103203,-36.5732835720408,
27.6818451470919));
#31861=CARTESIAN_POINT('Ctrl Pts',(-6.27609978720983,-36.6834624548757,
27.6760294929722));
#31862=CARTESIAN_POINT('Ctrl Pts',(-6.32687063571257,-36.7915180217742,
27.6702138388526));
#31863=CARTESIAN_POINT('Ctrl Pts',(-6.38219147051755,-36.8970204121211,
27.6643981847329));
#31864=CARTESIAN_POINT('Ctrl Pts',(-6.43759154701612,-37.0026739243394,
27.6585742002567));
#31865=CARTESIAN_POINT('Ctrl Pts',(-6.49755441363915,-37.1057666087602,
27.6527502157804));
#31866=CARTESIAN_POINT('Ctrl Pts',(-6.5617963858949,-37.2058968488927,27.6469262313042));
#31867=CARTESIAN_POINT('Ctrl Pts',(-6.5788415583959,-37.2324641717144,27.6453809671014));
#31868=CARTESIAN_POINT('Ctrl Pts',(-6.59618775340684,-37.2588231209837,
27.6438357028987));
#31869=CARTESIAN_POINT('Ctrl Pts',(-6.61382920342114,-37.2849665941533,
27.6422904386959));
#31870=CARTESIAN_POINT('Ctrl Pts',(-6.68031409498706,-37.3834928478019,
27.6364668401324));
#31871=CARTESIAN_POINT('Ctrl Pts',(-6.75120994305795,-37.4792738392738,
27.630643241569));
#31872=CARTESIAN_POINT('Ctrl Pts',(-6.82626268160111,-37.5718896620583,
27.6248196430055));
#31873=CARTESIAN_POINT('Ctrl Pts',(-6.90122073068663,-37.6643886371141,
27.6190033917208));
#31874=CARTESIAN_POINT('Ctrl Pts',(-6.98032498424699,-37.753730071613,27.6131871404361));
#31875=CARTESIAN_POINT('Ctrl Pts',(-7.06327782028086,-37.8395224667443,
27.6073708891513));
#31876=CARTESIAN_POINT('Ctrl Pts',(-7.14614762075709,-37.9252289839273,
27.6015604599179));
#31877=CARTESIAN_POINT('Ctrl Pts',(-7.23285805758641,-38.0073932372909,
27.5957500306845));
#31878=CARTESIAN_POINT('Ctrl Pts',(-7.32307130845913,-38.0856567826648,
27.5899396014511));
#31879=CARTESIAN_POINT('Ctrl Pts',(-7.41669920838254,-38.1668826704699,
27.5839092424793));
#31880=CARTESIAN_POINT('Ctrl Pts',(-7.51410004835411,-38.2439063774664,
27.5778788835075));
#31881=CARTESIAN_POINT('Ctrl Pts',(-7.61485386994085,-38.316368938804,27.5718485245357));
#31882=CARTESIAN_POINT('Ctrl Pts',(-7.71182388933896,-38.3861101741029,
27.5660446352413));
#31883=CARTESIAN_POINT('Ctrl Pts',(-7.81189922859877,-38.4516264129335,
27.5602407459469));
#31884=CARTESIAN_POINT('Ctrl Pts',(-7.91467240495817,-38.5126391533087,
27.5544368566526));
#31885=CARTESIAN_POINT('Ctrl Pts',(-8.01743040097529,-38.5736428816603,
27.5486338246347));
#31886=CARTESIAN_POINT('Ctrl Pts',(-8.12288509059288,-38.630144226035,27.5428307926168));
#31887=CARTESIAN_POINT('Ctrl Pts',(-8.23060175399589,-38.6819091307415,
27.5370277605988));
#31888=CARTESIAN_POINT('Ctrl Pts',(-8.33832792790142,-38.7336786058667,
27.5312242162206));
#31889=CARTESIAN_POINT('Ctrl Pts',(-8.44831610461033,-38.7807106329853,
27.5254206718423));
#31890=CARTESIAN_POINT('Ctrl Pts',(-8.56010940666761,-38.8228183424318,
27.519617127464));
#31891=CARTESIAN_POINT('Ctrl Pts',(-8.67193896211582,-38.8649397069652,
27.5138117010574));
#31892=CARTESIAN_POINT('Ctrl Pts',(-8.7855744251755,-38.9021334340867,27.5080062746507));
#31893=CARTESIAN_POINT('Ctrl Pts',(-8.90054211814158,-38.9342619849242,
27.5022008482441));
#31894=CARTESIAN_POINT('Ctrl Pts',(-9.01563712681007,-38.9664261150528,
27.4963889928841));
#31895=CARTESIAN_POINT('Ctrl Pts',(-9.13206691674238,-38.9935137624922,
27.490577137524));
#31896=CARTESIAN_POINT('Ctrl Pts',(-9.24934577711996,-39.0154381127932,
27.484765282164));
#31897=CARTESIAN_POINT('Ctrl Pts',(-9.36670166677805,-39.0373768631057,
27.4789496095514));
#31898=CARTESIAN_POINT('Ctrl Pts',(-9.48490733414273,-39.0541455052459,
27.4731339369387));
#31899=CARTESIAN_POINT('Ctrl Pts',(-9.6034717294852,-39.0657090809209,27.4673182643261));
#31900=CARTESIAN_POINT('Ctrl Pts',(-9.72220595452643,-39.0772892200724,
27.4614942614392));
#31901=CARTESIAN_POINT('Ctrl Pts',(-9.84129952682653,-39.0836493899837,
27.4556702585523));
#31902=CARTESIAN_POINT('Ctrl Pts',(-9.96026103792287,-39.084806704716,27.4498462556654));
#31903=CARTESIAN_POINT('Ctrl Pts',(-9.99182115669804,-39.0851137367138,
27.4483011658194));
#31904=CARTESIAN_POINT('Ctrl Pts',(-10.0233720090006,-39.0850548621266,
27.4467560759735));
#31905=CARTESIAN_POINT('Ctrl Pts',(-10.0549044960451,-39.0846310110356,
27.4452109861275));
#31906=CARTESIAN_POINT('Ctrl Pts',(-10.1737535104524,-39.0830334749978,
27.4393873920321));
#31907=CARTESIAN_POINT('Ctrl Pts',(-10.2927243949168,-39.0762418979449,
27.4335637979367));
#31908=CARTESIAN_POINT('Ctrl Pts',(-10.4113266827035,-39.0642385953701,
27.4277402038413));
#31909=CARTESIAN_POINT('Ctrl Pts',(-10.5297793364882,-39.0522504367039,
27.4219239570552));
#31910=CARTESIAN_POINT('Ctrl Pts',(-10.647863915865,-39.035063671483,27.4161077102691));
#31911=CARTESIAN_POINT('Ctrl Pts',(-10.7650898376149,-39.0127126162209,
27.410291463483));
#31912=CARTESIAN_POINT('Ctrl Pts',(-10.8821984159523,-38.9903839344157,
27.4044810387731));
#31913=CARTESIAN_POINT('Ctrl Pts',(-10.9984496477625,-38.9629013226206,
27.3986706140632));
#31914=CARTESIAN_POINT('Ctrl Pts',(-11.1133585593696,-38.9303508390827,
27.3928601893533));
#31915=CARTESIAN_POINT('Ctrl Pts',(-11.2326169981954,-38.896568256031,27.3868298286952));
#31916=CARTESIAN_POINT('Ctrl Pts',(-11.3504290441579,-38.8573266081899,
27.3807994680371));
#31917=CARTESIAN_POINT('Ctrl Pts',(-11.4662642624002,-38.8127803651414,
27.374769107379));
#31918=CARTESIAN_POINT('Ctrl Pts',(-11.5777491790476,-38.7699070985428,
27.3689652226406));
#31919=CARTESIAN_POINT('Ctrl Pts',(-11.6874026581689,-38.7221206494065,
27.3631613379023));
#31920=CARTESIAN_POINT('Ctrl Pts',(-11.7947684020336,-38.6696091594422,
27.3573574531639));
#31921=CARTESIAN_POINT('Ctrl Pts',(-11.9021182871135,-38.6171054258477,
27.351554425706));
#31922=CARTESIAN_POINT('Ctrl Pts',(-12.0071807422314,-38.5598782187373,
27.3457513982482));
#31923=CARTESIAN_POINT('Ctrl Pts',(-12.1095217128741,-38.4981628239567,
27.3399483707903));
#31924=CARTESIAN_POINT('Ctrl Pts',(-12.2118717194142,-38.4364419801953,
27.3341448309711));
#31925=CARTESIAN_POINT('Ctrl Pts',(-12.3114994140395,-38.3702323717587,
27.3283412911518));
#31926=CARTESIAN_POINT('Ctrl Pts',(-12.4079980612437,-38.2998136821715,
27.3225377513326));
#31927=CARTESIAN_POINT('Ctrl Pts',(-12.5045280020695,-38.2293721564526,
27.3167323294789));
#31928=CARTESIAN_POINT('Ctrl Pts',(-12.5979265477428,-38.1547190755532,
27.3109269076252));
#31929=CARTESIAN_POINT('Ctrl Pts',(-12.6878190123209,-38.0761752155893,
27.3051214857715));
#31930=CARTESIAN_POINT('Ctrl Pts',(-12.7778110247604,-37.9975443753284,
27.2993096349326));
#31931=CARTESIAN_POINT('Ctrl Pts',(-12.8642888982836,-37.9150144243233,
27.2934977840937));
#31932=CARTESIAN_POINT('Ctrl Pts',(-12.9469137752778,-37.82894400812,27.2876859332547));
#31933=CARTESIAN_POINT('Ctrl Pts',(-13.0295929208927,-37.7428170602407,
27.2818702651498));
#31934=CARTESIAN_POINT('Ctrl Pts',(-13.1084137611082,-37.6531453220559,
27.2760545970449));
#31935=CARTESIAN_POINT('Ctrl Pts',(-13.1830778827183,-37.5603203300661,
27.27023892894));
#31936=CARTESIAN_POINT('Ctrl Pts',(-13.2578489527708,-37.4673623761114,
27.2644149305068));
#31937=CARTESIAN_POINT('Ctrl Pts',(-13.3284511793682,-37.3712424811903,
27.2585909320737));
#31938=CARTESIAN_POINT('Ctrl Pts',(-13.394629504484,-37.2723810259916,27.2527669336405));
#31939=CARTESIAN_POINT('Ctrl Pts',(-13.4121869161231,-37.2461526308014,
27.25122180028));
#31940=CARTESIAN_POINT('Ctrl Pts',(-13.4294331970442,-37.2197313982307,
27.2496766669195));
#31941=CARTESIAN_POINT('Ctrl Pts',(-13.446364137165,-37.1931254487746,27.248131533559));
#31942=CARTESIAN_POINT('Ctrl Pts',(-13.5116281814714,-37.0905669463098,
27.2421754761057));
#31943=CARTESIAN_POINT('Ctrl Pts',(-13.5724057739584,-36.9849433669533,
27.2362194186525));
#31944=CARTESIAN_POINT('Ctrl Pts',(-13.6284046856138,-36.8766737695763,
27.2302633611992));
#31945=CARTESIAN_POINT('Ctrl Pts',(-13.6843233506168,-36.7685593229424,
27.2243158387988));
#31946=CARTESIAN_POINT('Ctrl Pts',(-13.7354767897766,-36.6578067427523,
27.2183683163984));
#31947=CARTESIAN_POINT('Ctrl Pts',(-13.7816163114275,-36.5448634480579,
27.212420793998));
#31948=CARTESIAN_POINT('Ctrl Pts',(-13.8276986056336,-36.4320602383912,
27.2064806483865));
#31949=CARTESIAN_POINT('Ctrl Pts',(-13.8687792179631,-36.3170720760405,
27.200540502775));
#31950=CARTESIAN_POINT('Ctrl Pts',(-13.9046557782775,-36.2003700484284,
27.1946003571635));
#31951=CARTESIAN_POINT('Ctrl Pts',(-13.9404859563607,-36.0838188964964,
27.1886678911401));
#31952=CARTESIAN_POINT('Ctrl Pts',(-13.9711253765799,-35.9655586593393,
27.1827354251167));
#31953=CARTESIAN_POINT('Ctrl Pts',(-13.9964203633776,-35.8460787665346,
27.1768029590934));
#31954=CARTESIAN_POINT('Ctrl Pts',(-14.0216960800848,-35.7266898952583,
27.1708750125093));
#31955=CARTESIAN_POINT('Ctrl Pts',(-14.0416353885848,-35.6060835916905,
27.1649470659253));
#31956=CARTESIAN_POINT('Ctrl Pts',(-14.0561348461714,-35.4847629417297,
27.1590191193412));
#31957=CARTESIAN_POINT('Ctrl Pts',(-14.0706246910155,-35.3635227240301,
27.153095102823));
#31958=CARTESIAN_POINT('Ctrl Pts',(-14.0796818242725,-35.2415694834072,
27.1471710863049));
#31959=CARTESIAN_POINT('Ctrl Pts',(-14.0832542386772,-35.1194144979658,
27.1412470697867));
#31960=CARTESIAN_POINT('Ctrl Pts',(-14.0844325971236,-35.0791217596222,
27.1392930369926));
#31961=CARTESIAN_POINT('Ctrl Pts',(-14.0850146333961,-35.0388071211363,
27.1373390041986));
#31962=CARTESIAN_POINT('Ctrl Pts',(-14.0849997205638,-34.9984890422085,
27.1353849714045));
#31963=CARTESIAN_POINT('Ctrl Pts',(-14.0849997205636,-34.9984890415501,
27.1353849713726));
#31964=CARTESIAN_POINT('Ctrl Pts',(-14.0849517284631,-34.868738473512,27.1290965550657));
#31965=CARTESIAN_POINT('Ctrl Pts',(-14.0787177200191,-34.7391739922796,
27.1228081387587));
#31966=CARTESIAN_POINT('Ctrl Pts',(-14.0663757191564,-34.6103674671502,
27.1165197224518));
#31967=CARTESIAN_POINT('Ctrl Pts',(-14.0539812320581,-34.481013172683,27.1102045636981));
#31968=CARTESIAN_POINT('Ctrl Pts',(-14.0354267799426,-34.3524235763946,
27.1038894049444));
#31969=CARTESIAN_POINT('Ctrl Pts',(-14.0108419948859,-34.2251635707713,
27.0975742461907));
#31970=CARTESIAN_POINT('Ctrl Pts',(-13.9862032613468,-34.0976243077068,
27.0912452295477));
#31971=CARTESIAN_POINT('Ctrl Pts',(-13.9555078254915,-33.9714207437558,
27.0849162129047));
#31972=CARTESIAN_POINT('Ctrl Pts',(-13.9189352633586,-33.8471030394676,
27.0785871962617));
#31973=CARTESIAN_POINT('Ctrl Pts',(-13.8822472544181,-33.7223929075987,
27.0722382011232));
#31974=CARTESIAN_POINT('Ctrl Pts',(-13.8396450934937,-33.5995808195232,
27.0658892059847));
#31975=CARTESIAN_POINT('Ctrl Pts',(-13.7913574442726,-33.4791996417153,
27.0595402108463));
#31976=CARTESIAN_POINT('Ctrl Pts',(-13.7698384569852,-33.4255527759707,
27.0567108342277));
#31977=CARTESIAN_POINT('Ctrl Pts',(-13.7471909664105,-33.3723883587508,
27.0538814576091));
#31978=CARTESIAN_POINT('Ctrl Pts',(-13.7234381112611,-33.3197519136723,
27.0510520809905));
#31979=CARTESIAN_POINT('Ctrl Pts',(-13.6745485457436,-33.2114123934716,
27.0452284866185));
#31980=CARTESIAN_POINT('Ctrl Pts',(-13.6208477443864,-33.1050337219617,
27.0394048922465));
#31981=CARTESIAN_POINT('Ctrl Pts',(-13.5625152041965,-33.0010726826948,
27.0335812978744));
#31982=CARTESIAN_POINT('Ctrl Pts',(-13.5042562590829,-32.8972428055648,
27.0277650508229));
#31983=CARTESIAN_POINT('Ctrl Pts',(-13.4413773960105,-32.7958248468748,
27.0219488037714));
#31984=CARTESIAN_POINT('Ctrl Pts',(-13.3741058400978,-32.6972549468476,
27.01613255672));
#31985=CARTESIAN_POINT('Ctrl Pts',(-13.306901623295,-32.5987837157041,27.0103221317562));
#31986=CARTESIAN_POINT('Ctrl Pts',(-13.2353136900053,-32.5031552070109,
27.0045117067924));
#31987=CARTESIAN_POINT('Ctrl Pts',(-13.1596144708337,-32.4107797707228,
26.9987012818287));
#31988=CARTESIAN_POINT('Ctrl Pts',(-13.0810498927768,-32.3149077491324,
26.9926709212701));
#31989=CARTESIAN_POINT('Ctrl Pts',(-12.9980568586636,-32.2225403266311,
26.9866405607115));
#31990=CARTESIAN_POINT('Ctrl Pts',(-12.9109886684102,-32.1341022397184,
26.9806102001529));
#31991=CARTESIAN_POINT('Ctrl Pts',(-12.827190402101,-32.048985524447,26.9748063151914));
#31992=CARTESIAN_POINT('Ctrl Pts',(-12.7396178642165,-31.967508644902,26.96900243023));
#31993=CARTESIAN_POINT('Ctrl Pts',(-12.6486256467501,-31.8900149223223,
26.9631985452686));
#31994=CARTESIAN_POINT('Ctrl Pts',(-12.5576468697513,-31.8125326463466,
26.9573955175994));
#31995=CARTESIAN_POINT('Ctrl Pts',(-12.4632497284872,-31.7390326219744,
26.9515924899303));
#31996=CARTESIAN_POINT('Ctrl Pts',(-12.3658231673449,-31.6698189627508,
26.9457894622612));
#31997=CARTESIAN_POINT('Ctrl Pts',(-12.2683880044126,-31.600599192654,26.9399859222428));
#31998=CARTESIAN_POINT('Ctrl Pts',(-12.1679232227137,-31.5356667766415,
26.9341823822244));
#31999=CARTESIAN_POINT('Ctrl Pts',(-12.0648475752946,-31.4752830623155,
26.9283788422061));
#32000=CARTESIAN_POINT('Ctrl Pts',(-11.9617385016158,-31.414879766238,26.9225734201657));
#32001=CARTESIAN_POINT('Ctrl Pts',(-11.8560172305229,-31.3590283117683,
26.9167679981253));
#32002=CARTESIAN_POINT('Ctrl Pts',(-11.748127405517,-31.3079442617858,26.910962576085));
#32003=CARTESIAN_POINT('Ctrl Pts',(-11.6401181025483,-31.2568036409615,
26.9051507250788));
#32004=CARTESIAN_POINT('Ctrl Pts',(-11.5299358213997,-31.2104411377206,
26.8993388740726));
#32005=CARTESIAN_POINT('Ctrl Pts',(-11.4180446327388,-31.169024351479,26.8935270230664));
#32006=CARTESIAN_POINT('Ctrl Pts',(-11.3060799533475,-31.127580362471,26.8877113548054));
#32007=CARTESIAN_POINT('Ctrl Pts',(-11.1924045190183,-31.0910886842026,
26.8818956865444));
#32008=CARTESIAN_POINT('Ctrl Pts',(-11.0774964206742,-31.0596667065546,
26.8760800182834));
#32009=CARTESIAN_POINT('Ctrl Pts',(-10.9624237290091,-31.02819972035,26.8702560197118));
#32010=CARTESIAN_POINT('Ctrl Pts',(-10.8461152459811,-31.0018170189197,
26.8644320211401));
#32011=CARTESIAN_POINT('Ctrl Pts',(-10.7290582106451,-30.98058472841,26.8586080225685));
#32012=CARTESIAN_POINT('Ctrl Pts',(-10.698002485515,-30.9749517121965,26.8570628911864));
#32013=CARTESIAN_POINT('Ctrl Pts',(-10.6668940924327,-30.9696809307097,
26.8555177598042));
#32014=CARTESIAN_POINT('Ctrl Pts',(-10.6357421573044,-30.9647730039779,
26.8539726284221));
#32015=CARTESIAN_POINT('Ctrl Pts',(-10.5183157488948,-30.9462727019427,
26.8481482959054));
#32016=CARTESIAN_POINT('Ctrl Pts',(-10.3998917399521,-30.9328725381076,
26.8423239633887));
#32017=CARTESIAN_POINT('Ctrl Pts',(-10.2809507483721,-30.9246728135045,
26.836499630872));
#32018=CARTESIAN_POINT('Ctrl Pts',(-10.1586484735487,-30.9162413639382,
26.8305107021885));
#32019=CARTESIAN_POINT('Ctrl Pts',(-10.0357999672896,-30.913308807926,26.8245217735049));
#32020=CARTESIAN_POINT('Ctrl Pts',(-9.91293956784619,-30.9159278310547,
26.8185328448214));
#32021=CARTESIAN_POINT('Ctrl Pts',(-9.79375532453327,-30.9184684893241,
26.8127231133161));
#32022=CARTESIAN_POINT('Ctrl Pts',(-9.67456033602679,-30.9262332574045,
26.8069133818107));
#32023=CARTESIAN_POINT('Ctrl Pts',(-9.5558470133928,-30.9392176708807,26.8011036503054));
#32024=CARTESIAN_POINT('Ctrl Pts',(-9.43721248743642,-30.9521934658747,
26.7952977750441));
#32025=CARTESIAN_POINT('Ctrl Pts',(-9.31905939593694,-30.9703819717122,
26.7894918997828));
#32026=CARTESIAN_POINT('Ctrl Pts',(-9.20187755966171,-30.993726722972,26.7836860245215));
#32027=CARTESIAN_POINT('Ctrl Pts',(-9.08474584711726,-31.0170614886739,
26.7778826326838));
#32028=CARTESIAN_POINT('Ctrl Pts',(-8.96858496299047,-31.0455480321735,
26.772079240846));
#32029=CARTESIAN_POINT('Ctrl Pts',(-8.85387639939024,-31.0790784639163,
26.7662758490082));
#32030=CARTESIAN_POINT('Ctrl Pts',(-8.73918983038655,-31.1126024664239,
26.7604735699318));
#32031=CARTESIAN_POINT('Ctrl Pts',(-8.6259554189508,-31.1511683167176,26.7546712908555));
#32032=CARTESIAN_POINT('Ctrl Pts',(-8.51464069226473,-31.1946179262886,
26.7488690117791));
#32033=CARTESIAN_POINT('Ctrl Pts',(-8.40328786556716,-31.2380824074823,
26.74306474674));
#32034=CARTESIAN_POINT('Ctrl Pts',(-8.29385641732616,-31.2864338402305,
26.7372604817009));
#32035=CARTESIAN_POINT('Ctrl Pts',(-8.18679484698842,-31.3394656027989,
26.7314562166618));
#32036=CARTESIAN_POINT('Ctrl Pts',(-8.07971027020371,-31.3925087613559,
26.7256507043449));
#32037=CARTESIAN_POINT('Ctrl Pts',(-7.97499694650878,-31.4502340620241,
26.719845192028));
#32038=CARTESIAN_POINT('Ctrl Pts',(-7.87307862470323,-31.5123890034429,
26.7140396797111));
#32039=CARTESIAN_POINT('Ctrl Pts',(-7.77108031664891,-31.5745927245171,
26.7082296111855));
#32040=CARTESIAN_POINT('Ctrl Pts',(-7.67188173069061,-31.6412328026179,
26.7024195426598));
#32041=CARTESIAN_POINT('Ctrl Pts',(-7.57587736468658,-31.7120136178869,
26.6966094741342));
#32042=CARTESIAN_POINT('Ctrl Pts',(-7.55470415351006,-31.7276239199108,
26.6953280969118));
#32043=CARTESIAN_POINT('Ctrl Pts',(-7.5336861810716,-31.7434354708017,26.6940467196895));
#32044=CARTESIAN_POINT('Ctrl Pts',(-7.51282745730979,-31.7594448403263,
26.6927653424671));
#32045=CARTESIAN_POINT('',(-14.0849999969885,-35.0001568555874,27.2396150285597));
#32046=CARTESIAN_POINT('Ctrl Pts',(-14.0849999969885,-35.0001568555874,
27.2396150285597));
#32047=CARTESIAN_POINT('Ctrl Pts',(-14.0850045558159,-34.8814310263966,
27.2337980380925));
#32048=CARTESIAN_POINT('Ctrl Pts',(-14.0798288721944,-34.7625114247042,
27.2279810476253));
#32049=CARTESIAN_POINT('Ctrl Pts',(-14.0694482081679,-34.6438872635826,
27.222164057158));
#32050=CARTESIAN_POINT('Ctrl Pts',(-14.0590806442284,-34.525412802598,27.2163544075585));
#32051=CARTESIAN_POINT('Ctrl Pts',(-14.0435211992775,-34.4072334448657,
27.2105447579589));
#32052=CARTESIAN_POINT('Ctrl Pts',(-14.0227971296609,-34.2898392762253,
27.2047351083594));
#32053=CARTESIAN_POINT('Ctrl Pts',(-14.0020937767413,-34.1725624599908,
27.1989312663427));
#32054=CARTESIAN_POINT('Ctrl Pts',(-13.9762361401773,-34.056069672273,27.1931274243259));
#32055=CARTESIAN_POINT('Ctrl Pts',(-13.9453032933436,-33.9408461284912,
27.1873235823092));
#32056=CARTESIAN_POINT('Ctrl Pts',(-13.9134326019726,-33.8221291535458,
27.181343775191));
#32057=CARTESIAN_POINT('Ctrl Pts',(-13.8761740797712,-33.7047600549076,
27.1753639680729));
#32058=CARTESIAN_POINT('Ctrl Pts',(-13.8336711624622,-33.5892589117398,
27.1693841609547));
#32059=CARTESIAN_POINT('Ctrl Pts',(-13.7924649395073,-33.4772815191688,
27.1635867879521));
#32060=CARTESIAN_POINT('Ctrl Pts',(-13.7463298222171,-33.3670601722282,
27.1577894149496));
#32061=CARTESIAN_POINT('Ctrl Pts',(-13.6954469887969,-33.2590529723762,
27.151992041947));
#32062=CARTESIAN_POINT('Ctrl Pts',(-13.6445714584235,-33.1510612744448,
27.1461955010224));
#32063=CARTESIAN_POINT('Ctrl Pts',(-13.5889497414525,-33.0452834618998,
27.1403989600978));
#32064=CARTESIAN_POINT('Ctrl Pts',(-13.5288104726773,-32.9421560681327,
27.1346024191732));
#32065=CARTESIAN_POINT('Ctrl Pts',(-13.4686655518633,-32.8390189821953,
27.1288053334753));
#32066=CARTESIAN_POINT('Ctrl Pts',(-13.4040024414123,-32.7385331639236,
27.1230082477773));
#32067=CARTESIAN_POINT('Ctrl Pts',(-13.3350945511629,-32.6411084520895,
27.1172111620793));
#32068=CARTESIAN_POINT('Ctrl Pts',(-13.2661638185421,-32.5436514448037,
27.1114121546974));
#32069=CARTESIAN_POINT('Ctrl Pts',(-13.1929857441635,-32.4492578959464,
27.1056131473155));
#32070=CARTESIAN_POINT('Ctrl Pts',(-13.1158752651503,-32.3583061623222,
27.0998141399336));
#32071=CARTESIAN_POINT('Ctrl Pts',(-13.0386792579379,-32.2672535482718,
27.0940087004991));
#32072=CARTESIAN_POINT('Ctrl Pts',(-12.9575424053558,-32.1796506814067,
27.0882032610646));
#32073=CARTESIAN_POINT('Ctrl Pts',(-12.8728179817518,-32.0958405960204,
27.0823978216301));
#32074=CARTESIAN_POINT('Ctrl Pts',(-12.788037129969,-32.0119746914229,27.0765885156556));
#32075=CARTESIAN_POINT('Ctrl Pts',(-12.6996642516753,-31.9319068727521,
27.0707792096811));
#32076=CARTESIAN_POINT('Ctrl Pts',(-12.6080860379959,-31.8559401693971,
27.0649699037065));
#32077=CARTESIAN_POINT('Ctrl Pts',(-12.5163779129181,-31.7798657008841,
27.0591523567429));
#32078=CARTESIAN_POINT('Ctrl Pts',(-12.4214557029949,-31.7079042043729,
27.0533348097792));
#32079=CARTESIAN_POINT('Ctrl Pts',(-12.3237354633827,-31.6403157148003,
27.0475172628155));
#32080=CARTESIAN_POINT('Ctrl Pts',(-12.3029678679135,-31.6259517466461,
27.0462809123682));
#32081=CARTESIAN_POINT('Ctrl Pts',(-12.2820739874267,-31.6117851206942,
27.0450445619208));
#32082=CARTESIAN_POINT('Ctrl Pts',(-12.2610579524706,-31.5978180625414,
27.0438082114734));
#32083=CARTESIAN_POINT('Ctrl Pts',(-12.162065909123,-31.5320288863724,27.0379846173779));
#32084=CARTESIAN_POINT('Ctrl Pts',(-12.0600404855395,-31.4704577095777,
27.0321610232824));
#32085=CARTESIAN_POINT('Ctrl Pts',(-11.9553764945523,-31.4133960680677,
27.0263374291869));
#32086=CARTESIAN_POINT('Ctrl Pts',(-11.8508445523827,-31.3564064181015,
27.0205211824007));
#32087=CARTESIAN_POINT('Ctrl Pts',(-11.7436810193416,-31.3039151810071,
27.0147049356145));
#32088=CARTESIAN_POINT('Ctrl Pts',(-11.6343101665915,-31.2561710403151,
27.0088886888283));
#32089=CARTESIAN_POINT('Ctrl Pts',(-11.5250487943121,-31.2084746916157,
27.0030782641183));
#32090=CARTESIAN_POINT('Ctrl Pts',(-11.4135848699965,-31.1655161485198,
26.9972678394083));
#32091=CARTESIAN_POINT('Ctrl Pts',(-11.3003672508535,-31.1274982229949,
26.9914574146983));
#32092=CARTESIAN_POINT('Ctrl Pts',(-11.1828641232246,-31.0880412445762,
26.9854270540403));
#32093=CARTESIAN_POINT('Ctrl Pts',(-11.0634723095887,-31.0539065124743,
26.9793966933822));
#32094=CARTESIAN_POINT('Ctrl Pts',(-10.942716815981,-31.0252660460269,26.9733663327241));
#32095=CARTESIAN_POINT('Ctrl Pts',(-10.8264964095787,-30.9977011994877,
26.9675624479857));
#32096=CARTESIAN_POINT('Ctrl Pts',(-10.7090133376739,-30.9752254787958,
26.9617585632473));
#32097=CARTESIAN_POINT('Ctrl Pts',(-10.5907504313402,-30.9579412513088,
26.9559546785088));
#32098=CARTESIAN_POINT('Ctrl Pts',(-10.4725049933901,-30.9406595768414,
26.9501516510509));
#32099=CARTESIAN_POINT('Ctrl Pts',(-10.3534803540188,-30.9285679296409,
26.944348623593));
#32100=CARTESIAN_POINT('Ctrl Pts',(-10.2341676060109,-30.9217172079054,
26.9385455961351));
#32101=CARTESIAN_POINT('Ctrl Pts',(-10.1148443236319,-30.9148658813053,
26.9327420563158));
#32102=CARTESIAN_POINT('Ctrl Pts',(-9.9952332897256,-30.9132564236021,26.9269385164965));
#32103=CARTESIAN_POINT('Ctrl Pts',(-9.87582811879394,-30.9168876645483,
26.9211349766772));
#32104=CARTESIAN_POINT('Ctrl Pts',(-9.75638422586779,-30.9205200830724,
26.9153295548235));
#32105=CARTESIAN_POINT('Ctrl Pts',(-9.63714673662399,-30.9293965677822,
26.9095241329698));
#32106=CARTESIAN_POINT('Ctrl Pts',(-9.5186060167919,-30.9434639366904,26.9037187111162));
#32107=CARTESIAN_POINT('Ctrl Pts',(-9.39993402371848,-30.9575468839512,
26.8979068602772));
#32108=CARTESIAN_POINT('Ctrl Pts',(-9.28196074598802,-30.9768321416398,
26.8920950094382));
#32109=CARTESIAN_POINT('Ctrl Pts',(-9.16516836187053,-31.0012150425438,
26.8862831585993));
#32110=CARTESIAN_POINT('Ctrl Pts',(-9.04829926766458,-31.0256139583146,
26.8804674904943));
#32111=CARTESIAN_POINT('Ctrl Pts',(-8.93261300650044,-31.0551170845889,
26.8746518223894));
#32112=CARTESIAN_POINT('Ctrl Pts',(-8.81857694830981,-31.0895697713762,
26.8688361542845));
#32113=CARTESIAN_POINT('Ctrl Pts',(-8.70437754555023,-31.1240718079863,
26.8630121558513));
#32114=CARTESIAN_POINT('Ctrl Pts',(-8.59183344762659,-31.163537421163,26.8571881574181));
#32115=CARTESIAN_POINT('Ctrl Pts',(-8.48139252878395,-31.2077636745099,
26.8513641589849));
#32116=CARTESIAN_POINT('Ctrl Pts',(-8.45209204905866,-31.219497101333,26.8498190256249));
#32117=CARTESIAN_POINT('Ctrl Pts',(-8.42293947080304,-31.2315653620464,
26.8482738922649));
#32118=CARTESIAN_POINT('Ctrl Pts',(-8.39394285394541,-31.2439641317465,
26.8467287589049));
#32119=CARTESIAN_POINT('Ctrl Pts',(-8.28465587810226,-31.2906945503794,
26.84090521911));
#32120=CARTESIAN_POINT('Ctrl Pts',(-8.17723389000758,-31.3422740639199,
26.8350816793151));
#32121=CARTESIAN_POINT('Ctrl Pts',(-8.07213713139233,-31.3985322769954,
26.8292581395202));
#32122=CARTESIAN_POINT('Ctrl Pts',(-7.96718840949689,-31.45471124613,26.8234428026208));
#32123=CARTESIAN_POINT('Ctrl Pts',(-7.86455875598442,-31.5155556089732,
26.8176274657214));
#32124=CARTESIAN_POINT('Ctrl Pts',(-7.76468852804543,-31.5808469435622,
26.811812128822));
#32125=CARTESIAN_POINT('Ctrl Pts',(-7.67859497325255,-31.6371316162613,
26.8067989929123));
#32126=CARTESIAN_POINT('Ctrl Pts',(-7.59455190212405,-31.6967201573034,
26.8017858570026));
#32127=CARTESIAN_POINT('Ctrl Pts',(-7.5128274573098,-31.7594448403263,26.796772721093));
#32128=CARTESIAN_POINT('Ctrl Pts',(-7.5128274573098,-31.7594448403263,28.0469627561459));
#32129=CARTESIAN_POINT('Ctrl Pts',(-7.41670716853337,-31.8332185399736,
28.0410436622024));
#32130=CARTESIAN_POINT('Ctrl Pts',(-7.32400111322147,-31.9111734129659,
28.035124568259));
#32131=CARTESIAN_POINT('Ctrl Pts',(-7.23507124736889,-31.9929426355864,
28.0292054743155));
#32132=CARTESIAN_POINT('Ctrl Pts',(-7.14757771632443,-32.0733911772461,
28.0233819815583));
#32133=CARTESIAN_POINT('Ctrl Pts',(-7.0634570630503,-32.157791240188,28.017558488801));
#32134=CARTESIAN_POINT('Ctrl Pts',(-6.9830865523076,-32.2458289361166,28.0117349960438));
#32135=CARTESIAN_POINT('Ctrl Pts',(-6.90281746241604,-32.3337555358487,
28.0059188520465));
#32136=CARTESIAN_POINT('Ctrl Pts',(-6.82628937539092,-32.4253103394787,
28.0001027080492));
#32137=CARTESIAN_POINT('Ctrl Pts',(-6.75384496521342,-32.5201406309773,
27.994286564052));
#32138=CARTESIAN_POINT('Ctrl Pts',(-6.68147308973758,-32.6148759739921,
27.9884762434477));
#32139=CARTESIAN_POINT('Ctrl Pts',(-6.6131770034937,-32.7128799579496,27.9826659228433));
#32140=CARTESIAN_POINT('Ctrl Pts',(-6.54926069551753,-32.8137650509381,
27.9768556022391));
#32141=CARTESIAN_POINT('Ctrl Pts',(-6.48292341778096,-32.9184713871606,
27.9708252030519));
#32142=CARTESIAN_POINT('Ctrl Pts',(-6.42130456768723,-33.0262810731424,
27.9647948038647));
#32143=CARTESIAN_POINT('Ctrl Pts',(-6.36469640883172,-33.1367252483761,
27.9587644046776));
#32144=CARTESIAN_POINT('Ctrl Pts',(-6.31021557311453,-33.2430189538857,
27.9529606266698));
#32145=CARTESIAN_POINT('Ctrl Pts',(-6.26037582611707,-33.3517523185486,
27.9471568486621));
#32146=CARTESIAN_POINT('Ctrl Pts',(-6.2153917105462,-33.4624808634044,27.9413530706543));
#32147=CARTESIAN_POINT('Ctrl Pts',(-6.17041424570425,-33.5731930374697,
27.9355501507129));
#32148=CARTESIAN_POINT('Ctrl Pts',(-6.13029113829591,-33.6858994268841,
27.9297472307714));
#32149=CARTESIAN_POINT('Ctrl Pts',(-6.0951889167183,-33.8001352560057,27.92394431083));
#32150=CARTESIAN_POINT('Ctrl Pts',(-6.06008359989467,-33.9143811582219,
27.9181408791983));
#32151=CARTESIAN_POINT('Ctrl Pts',(-6.03000016910789,-34.0301563779248,
27.9123374475666));
#32152=CARTESIAN_POINT('Ctrl Pts',(-6.00505518761999,-34.1469812745092,
27.9065340159349));
#32153=CARTESIAN_POINT('Ctrl Pts',(-5.98010211894736,-34.2638440458268,
27.9007287028256));
#32154=CARTESIAN_POINT('Ctrl Pts',(-5.96029089787606,-34.3817567716713,
27.8949233897163));
#32155=CARTESIAN_POINT('Ctrl Pts',(-5.94568680155446,-34.5002305642496,
27.8891180766071));
#32156=CARTESIAN_POINT('Ctrl Pts',(-5.93106653291073,-34.618835552644,27.8833063347951));
#32157=CARTESIAN_POINT('Ctrl Pts',(-5.92166494899037,-34.7380024424444,
27.8774945929831));
#32158=CARTESIAN_POINT('Ctrl Pts',(-5.91749537449755,-34.8572380206389,
27.8716828511711));
#32159=CARTESIAN_POINT('Ctrl Pts',(-5.91332306155652,-34.9765519090919,
27.8658672923859));
#32160=CARTESIAN_POINT('Ctrl Pts',(-5.91438959772116,-35.0959341683828,
27.8600517336007));
#32161=CARTESIAN_POINT('Ctrl Pts',(-5.92065623563793,-35.2148940486851,
27.8542361748155));
#32162=CARTESIAN_POINT('Ctrl Pts',(-5.92693185045036,-35.3340243378172,
27.848412285301));
#32163=CARTESIAN_POINT('Ctrl Pts',(-5.93842239579202,-35.4527306352959,
27.8425883957865));
#32164=CARTESIAN_POINT('Ctrl Pts',(-5.9550375820364,-35.5705296112053,27.836764506272));
#32165=CARTESIAN_POINT('Ctrl Pts',(-5.9594486824461,-35.6018035977411,27.8352183447637));
#32166=CARTESIAN_POINT('Ctrl Pts',(-5.96422070613784,-35.6330137040189,
27.8336721832554));
#32167=CARTESIAN_POINT('Ctrl Pts',(-5.96935137004129,-35.6641510534599,
27.8321260217472));
#32168=CARTESIAN_POINT('Ctrl Pts',(-5.98867604478963,-35.7814300570737,
27.8263023956399));
#32169=CARTESIAN_POINT('Ctrl Pts',(-6.01315479434023,-35.8980540344452,
27.8204787695327));
#32170=CARTESIAN_POINT('Ctrl Pts',(-6.04273187030218,-36.0135353716955,
27.8146551434255));
#32171=CARTESIAN_POINT('Ctrl Pts',(-6.07227163203181,-36.1288710184978,
27.8088388643642));
#32172=CARTESIAN_POINT('Ctrl Pts',(-6.10689682662744,-36.243066500305,27.803022585303));
#32173=CARTESIAN_POINT('Ctrl Pts',(-6.14650027023396,-36.3556418526636,
27.7972063062418));
#32174=CARTESIAN_POINT('Ctrl Pts',(-6.18606407243592,-36.4681045217632,
27.7913958490347));
#32175=CARTESIAN_POINT('Ctrl Pts',(-6.23059607581365,-36.5789499045739,
27.7855853918275));
#32176=CARTESIAN_POINT('Ctrl Pts',(-6.27993877240317,-36.6877113091198,
27.7797749346204));
#32177=CARTESIAN_POINT('Ctrl Pts',(-6.33114879748764,-36.8005886879414,
27.7737445860604));
#32178=CARTESIAN_POINT('Ctrl Pts',(-6.38754070981686,-36.9112208059573,
27.7677142375003));
#32179=CARTESIAN_POINT('Ctrl Pts',(-6.44888257438587,-37.0191062452233,
27.7616838889402));
#32180=CARTESIAN_POINT('Ctrl Pts',(-6.507921139498,-37.1229407402376,27.755879971361));
#32181=CARTESIAN_POINT('Ctrl Pts',(-6.57154441183006,-37.2242307183596,
27.7500760537818));
#32182=CARTESIAN_POINT('Ctrl Pts',(-6.63949822635043,-37.3225530842799,
27.7442721362026));
#32183=CARTESIAN_POINT('Ctrl Pts',(-6.70744200441555,-37.4208609284544,
27.7384690758345));
#32184=CARTESIAN_POINT('Ctrl Pts',(-6.77971482060832,-37.5162016962512,
27.7326660154663));
#32185=CARTESIAN_POINT('Ctrl Pts',(-6.8560192153665,-37.6081813253406,27.7268629550981));
#32186=CARTESIAN_POINT('Ctrl Pts',(-6.93233034760052,-37.7001690759875,
27.7210593823351));
#32187=CARTESIAN_POINT('Ctrl Pts',(-7.01267350544634,-37.7887947835733,
27.7152558095721));
#32188=CARTESIAN_POINT('Ctrl Pts',(-7.09671140830339,-37.8736980275117,
27.7094522368091));
#32189=CARTESIAN_POINT('Ctrl Pts',(-7.18077656368583,-37.9586288045955,
27.7036467820141));
#32190=CARTESIAN_POINT('Ctrl Pts',(-7.268538559853,-38.0398344272183,27.6978413272192));
#32191=CARTESIAN_POINT('Ctrl Pts',(-7.35962426946815,-38.1169923005388,
27.6920358724243));
#32192=CARTESIAN_POINT('Ctrl Pts',(-7.45081084511643,-38.1942356165555,
27.6862239888142));
#32193=CARTESIAN_POINT('Ctrl Pts',(-7.54532816924453,-38.2674219719774,
27.680412105204));
#32194=CARTESIAN_POINT('Ctrl Pts',(-7.64277101897887,-38.3362698528497,
27.6746002215939));
#32195=CARTESIAN_POINT('Ctrl Pts',(-7.74027786850679,-38.4051629525368,
27.6687845207786));
#32196=CARTESIAN_POINT('Ctrl Pts',(-7.84071372757151,-38.4697116826011,
27.6629688199633));
#32197=CARTESIAN_POINT('Ctrl Pts',(-7.9436468895561,-38.5296794309353,27.6571531191479));
#32198=CARTESIAN_POINT('Ctrl Pts',(-8.04672748556019,-38.5897330727368,
27.6513290883432));
#32199=CARTESIAN_POINT('Ctrl Pts',(-8.15231216368047,-38.6451924472694,
27.6455050575385));
#32200=CARTESIAN_POINT('Ctrl Pts',(-8.2599471695437,-38.6958681182127,27.6396810267338));
#32201=CARTESIAN_POINT('Ctrl Pts',(-8.28849726270323,-38.7093097965473,
27.6381362075488));
#32202=CARTESIAN_POINT('Ctrl Pts',(-8.31719151868609,-38.7224151763029,
27.6365913883637));
#32203=CARTESIAN_POINT('Ctrl Pts',(-8.34602128478285,-38.7351813088,27.6350465691787));
#32204=CARTESIAN_POINT('Ctrl Pts',(-8.45470265264603,-38.7833065949174,
27.62922296792));
#32205=CARTESIAN_POINT('Ctrl Pts',(-8.56566144290904,-38.826762146425,27.6233993666612));
#32206=CARTESIAN_POINT('Ctrl Pts',(-8.67845927465491,-38.8653272967828,
27.6175757654025));
#32207=CARTESIAN_POINT('Ctrl Pts',(-8.79111479934749,-38.9038437928995,
27.6117595112666));
#32208=CARTESIAN_POINT('Ctrl Pts',(-8.90560436781489,-38.9374820284921,
27.6059432571308));
#32209=CARTESIAN_POINT('Ctrl Pts',(-9.0214678015652,-38.9660685491588,27.600127002995));
#32210=CARTESIAN_POINT('Ctrl Pts',(-9.1372152594184,-38.9946264555571,27.5943165707588));
#32211=CARTESIAN_POINT('Ctrl Pts',(-9.25433345259775,-39.0181426092948,
27.5885061385227));
#32212=CARTESIAN_POINT('Ctrl Pts',(-9.37234571723612,-39.0364929210056,
27.5826957062866));
#32213=CARTESIAN_POINT('Ctrl Pts',(-9.49482476247991,-39.055537794563,27.5766653483834));
#32214=CARTESIAN_POINT('Ctrl Pts',(-9.61826647373684,-39.0690178991552,
27.5706349904802));
#32215=CARTESIAN_POINT('Ctrl Pts',(-9.742124335769,-39.0768523571252,27.5646046325771));
#32216=CARTESIAN_POINT('Ctrl Pts',(-9.86133081533922,-39.0843925983228,
27.5588007399182));
#32217=CARTESIAN_POINT('Ctrl Pts',(-9.98092230874842,-39.0867035537119,
27.5529968472594));
#32218=CARTESIAN_POINT('Ctrl Pts',(-10.1004056308461,-39.0837658734671,
27.5471929546006));
#32219=CARTESIAN_POINT('Ctrl Pts',(-10.2198713070446,-39.0808286270737,
27.5413899190899));
#32220=CARTESIAN_POINT('Ctrl Pts',(-10.3392284355992,-39.0726442965989,
27.5355868835792));
#32221=CARTESIAN_POINT('Ctrl Pts',(-10.4579843811548,-39.0592456573381,
27.5297838480685));
#32222=CARTESIAN_POINT('Ctrl Pts',(-10.5767508144459,-39.0458458347985,
27.5239803000722));
#32223=CARTESIAN_POINT('Ctrl Pts',(-10.694915553396,-39.0272308336835,27.518176752076));
#32224=CARTESIAN_POINT('Ctrl Pts',(-10.8119922711789,-39.0034851756371,
27.5123732040798));
#32225=CARTESIAN_POINT('Ctrl Pts',(-10.9291069581476,-38.9797318166291,
27.5065677739331));
#32226=CARTESIAN_POINT('Ctrl Pts',(-11.0451325222156,-38.950844572643,27.5007623437865));
#32227=CARTESIAN_POINT('Ctrl Pts',(-11.1595946230855,-38.9169586811851,
27.4949569136399));
#32228=CARTESIAN_POINT('Ctrl Pts',(-11.2741834829013,-38.8830352634207,
27.4891450543765));
#32229=CARTESIAN_POINT('Ctrl Pts',(-11.3872050316689,-38.8441022645142,
27.4833331951132));
#32230=CARTESIAN_POINT('Ctrl Pts',(-11.4982016944126,-38.8003442847799,
27.4775213358498));
#32231=CARTESIAN_POINT('Ctrl Pts',(-11.6092712621196,-38.756557563876,27.471705659234));
#32232=CARTESIAN_POINT('Ctrl Pts',(-11.7183129230101,-38.7079397166031,
27.4658899826181));
#32233=CARTESIAN_POINT('Ctrl Pts',(-11.8248921394382,-38.654722107003,27.4600743060023));
#32234=CARTESIAN_POINT('Ctrl Pts',(-11.9316240202275,-38.6014282683534,
27.4542502989954));
#32235=CARTESIAN_POINT('Ctrl Pts',(-12.0358860607236,-38.5435217142231,
27.4484262919884));
#32236=CARTESIAN_POINT('Ctrl Pts',(-12.1372710941066,-38.4812781087262,
27.4426022849815));
#32237=CARTESIAN_POINT('Ctrl Pts',(-12.1641676219605,-38.4647654459286,
27.4410572288578));
#32238=CARTESIAN_POINT('Ctrl Pts',(-12.1908618425745,-38.4479477693427,
27.439512172734));
#32239=CARTESIAN_POINT('Ctrl Pts',(-12.2173465433403,-38.4308307021386,
27.4379671166103));
#32240=CARTESIAN_POINT('Ctrl Pts',(-12.3171719194025,-38.3663135423699,
27.4321435352924));
#32241=CARTESIAN_POINT('Ctrl Pts',(-12.4143401001004,-38.2973318601452,
27.4263199539746));
#32242=CARTESIAN_POINT('Ctrl Pts',(-12.5084262226572,-38.2241313381259,
27.4204963726567));
#32243=CARTESIAN_POINT('Ctrl Pts',(-12.6023936383654,-38.1510231719509,
27.4146801388516));
#32244=CARTESIAN_POINT('Ctrl Pts',(-12.6932864107806,-38.0737070015131,
27.4088639050465));
#32245=CARTESIAN_POINT('Ctrl Pts',(-12.7807072149309,-37.9924726205651,
27.4030476712414));
#32246=CARTESIAN_POINT('Ctrl Pts',(-12.8680405076606,-37.9113195582017,
27.397237259699));
#32247=CARTESIAN_POINT('Ctrl Pts',(-12.9519084489252,-37.8262563645648,
27.3914268481565));
#32248=CARTESIAN_POINT('Ctrl Pts',(-13.0319459642009,-37.737613681688,27.385616436614));
#32249=CARTESIAN_POINT('Ctrl Pts',(-13.1150133113598,-37.6456154170462,
27.3795860710902));
#32250=CARTESIAN_POINT('Ctrl Pts',(-13.19395414564,-37.5497615791823,27.3735557055663));
#32251=CARTESIAN_POINT('Ctrl Pts',(-13.268401237959,-37.4504649248068,27.3675253400425));
#32252=CARTESIAN_POINT('Ctrl Pts',(-13.3400521739576,-37.3548977507787,
27.3617214688537));
#32253=CARTESIAN_POINT('Ctrl Pts',(-13.4075405737231,-37.2561420694291,
27.355917597665));
#32254=CARTESIAN_POINT('Ctrl Pts',(-13.4705799071922,-37.1545997558234,
27.3501137264762));
#32255=CARTESIAN_POINT('Ctrl Pts',(-13.5336099279418,-37.0530724429327,
27.3443107126859));
#32256=CARTESIAN_POINT('Ctrl Pts',(-13.5921919741503,-36.9487596632861,
27.3385076988955));
#32257=CARTESIAN_POINT('Ctrl Pts',(-13.646083412917,-36.8420914054551,27.3327046851052));
#32258=CARTESIAN_POINT('Ctrl Pts',(-13.6999796089217,-36.7354137315404,
27.3269011590569));
#32259=CARTESIAN_POINT('Ctrl Pts',(-13.7491841900861,-36.6263805305119,
27.3210976330085));
#32260=CARTESIAN_POINT('Ctrl Pts',(-13.7935012606565,-36.5154448803562,
27.3152941069602));
#32261=CARTESIAN_POINT('Ctrl Pts',(-13.8378327021985,-36.4044732564084,
27.3094886989665));
#32262=CARTESIAN_POINT('Ctrl Pts',(-13.8772733297251,-36.2915983354265,
27.3036832909728));
#32263=CARTESIAN_POINT('Ctrl Pts',(-13.9116762352757,-36.1772909709921,
27.297877882979));
#32264=CARTESIAN_POINT('Ctrl Pts',(-13.9461172386843,-36.062857022315,27.2920660460629));
#32265=CARTESIAN_POINT('Ctrl Pts',(-13.9755092666319,-35.9469878550576,
27.2862542091468));
#32266=CARTESIAN_POINT('Ctrl Pts',(-13.9997558868884,-35.8301673598144,
27.2804423722307));
#32267=CARTESIAN_POINT('Ctrl Pts',(-14.0240184323186,-35.7132701369014,
27.2746267181016));
#32268=CARTESIAN_POINT('Ctrl Pts',(-14.0431287744825,-35.5954207437815,
27.2688110639726));
#32269=CARTESIAN_POINT('Ctrl Pts',(-14.0570422211961,-35.4771094375846,
27.2629954098435));
#32270=CARTESIAN_POINT('Ctrl Pts',(-14.0709755975632,-35.3586286619967,
27.2571714253579));
#32271=CARTESIAN_POINT('Ctrl Pts',(-14.0796971908158,-35.2396850585239,
27.2513474408724));
#32272=CARTESIAN_POINT('Ctrl Pts',(-14.083214363765,-35.1207702759093,27.2455234563868));
#32273=CARTESIAN_POINT('Ctrl Pts',(-14.0841475669969,-35.0892188961329,
27.2439781922718));
#32274=CARTESIAN_POINT('Ctrl Pts',(-14.0847146691044,-35.0576695226078,
27.2424329281568));
#32275=CARTESIAN_POINT('Ctrl Pts',(-14.0849164197722,-35.0261312739004,
27.2408876640418));
#32276=CARTESIAN_POINT('Ctrl Pts',(-14.0849718051372,-35.0174732732323,
27.2404634522263));
#32277=CARTESIAN_POINT('Ctrl Pts',(-14.0849996645284,-35.0088150963167,
27.2400392404109));
#32278=CARTESIAN_POINT('Ctrl Pts',(-14.0849999969885,-35.0001568563172,
27.2396150285955));
#32279=CARTESIAN_POINT('Origin',(-10.,-35.,32.7603849714045));
#32280=CARTESIAN_POINT('',(-7.51282745730978,-31.7594448403263,29.2969304815276));
#32281=CARTESIAN_POINT('',(-7.5128274573098,-31.7594448403263,29.1925543292906));
#32282=CARTESIAN_POINT('',(-7.5128274573098,-31.7594448403263,32.7603849714045));
#32283=CARTESIAN_POINT('',(-14.0823965473396,-35.0044045793917,29.7396160305011));
#32284=CARTESIAN_POINT('Ctrl Pts',(-14.0849976445926,-35.0043867611016,
29.7396150285955));
#32285=CARTESIAN_POINT('Ctrl Pts',(-14.0851248049252,-34.8859737344617,
29.7338650871352));
#32286=CARTESIAN_POINT('Ctrl Pts',(-14.0800989948151,-34.7674775508307,
29.7281151456748));
#32287=CARTESIAN_POINT('Ctrl Pts',(-14.0699255136412,-34.649384379395,29.7223652042145));
#32288=CARTESIAN_POINT('Ctrl Pts',(-14.0597547176425,-34.5313223773153,
29.7166167803862));
#32289=CARTESIAN_POINT('Ctrl Pts',(-14.0444389866147,-34.4136635905276,
29.7108683565578));
#32290=CARTESIAN_POINT('Ctrl Pts',(-14.0240356521059,-34.2968911388837,
29.7051199327294));
#32291=CARTESIAN_POINT('Ctrl Pts',(-14.0036326709799,-34.1801207097214,
29.6993716084629));
#32292=CARTESIAN_POINT('Ctrl Pts',(-13.9781423333174,-34.0642369953368,
29.6936232841964));
#32293=CARTESIAN_POINT('Ctrl Pts',(-13.9476733383978,-33.9497142230312,
29.6878749599299));
#32294=CARTESIAN_POINT('Ctrl Pts',(-13.9171973565982,-33.8351651893778,
29.6821253175086));
#32295=CARTESIAN_POINT('Ctrl Pts',(-13.8817405552409,-33.7219781204337,
29.6763756750873));
#32296=CARTESIAN_POINT('Ctrl Pts',(-13.8414616644281,-33.6106126239492,
29.670626032666));
#32297=CARTESIAN_POINT('Ctrl Pts',(-13.8011379470234,-33.4991231882111,
29.664869991437));
#32298=CARTESIAN_POINT('Ctrl Pts',(-13.7559815663988,-33.3894597649086,
29.6591139502081));
#32299=CARTESIAN_POINT('Ctrl Pts',(-13.7061997024199,-33.2820626420667,
29.6533579089791));
#32300=CARTESIAN_POINT('Ctrl Pts',(-13.6563885438708,-33.1746023204554,
29.6475984805577));
#32301=CARTESIAN_POINT('Ctrl Pts',(-13.6019466741219,-33.0694113236932,
29.6418390521363));
#32302=CARTESIAN_POINT('Ctrl Pts',(-13.5431267044342,-32.9669042923844,
29.6360796237149));
#32303=CARTESIAN_POINT('Ctrl Pts',(-13.4842097594284,-32.8642282597649,
29.630310699838));
#32304=CARTESIAN_POINT('Ctrl Pts',(-13.4209005215424,-32.7642453812295,
29.6245417759611));
#32305=CARTESIAN_POINT('Ctrl Pts',(-13.3534945117023,-32.6673406678251,
29.6187728520842));
#32306=CARTESIAN_POINT('Ctrl Pts',(-13.3031282057788,-32.5949326963054,
29.6144622663439));
#32307=CARTESIAN_POINT('Ctrl Pts',(-13.2504754795845,-32.5242426933336,
29.6101516806035));
#32308=CARTESIAN_POINT('Ctrl Pts',(-13.1956733769003,-32.4554181742041,
29.6058410948631));
#32309=CARTESIAN_POINT('Ctrl Pts',(-13.1215713269672,-32.3623553590318,
29.6000124272732));
#32310=CARTESIAN_POINT('Ctrl Pts',(-13.0432819943138,-32.2723830731251,
29.5941837596833));
#32311=CARTESIAN_POINT('Ctrl Pts',(-12.961092379355,-32.1859003356445,29.5883550920934));
#32312=CARTESIAN_POINT('Ctrl Pts',(-12.8790067593268,-32.0995270252039,
29.5825337995458));
#32313=CARTESIAN_POINT('Ctrl Pts',(-12.7930309513319,-32.0166347736365,
29.5767125069981));
#32314=CARTESIAN_POINT('Ctrl Pts',(-12.7034931198539,-31.9375908256892,
29.5708912144504));
#32315=CARTESIAN_POINT('Ctrl Pts',(-12.6140453627667,-31.8586263953642,
29.5650757780796));
#32316=CARTESIAN_POINT('Ctrl Pts',(-12.521043014877,-31.7835028349162,29.5592603417089));
#32317=CARTESIAN_POINT('Ctrl Pts',(-12.4248516983507,-31.7125512565204,
29.5534449053381));
#32318=CARTESIAN_POINT('Ctrl Pts',(-12.3251366707921,-31.6390005572414,
29.5474164360446));
#32319=CARTESIAN_POINT('Ctrl Pts',(-12.2219948707104,-31.5699336732242,
29.5413879667511));
#32320=CARTESIAN_POINT('Ctrl Pts',(-12.1158723210058,-31.5056746972839,
29.5353594974577));
#32321=CARTESIAN_POINT('Ctrl Pts',(-12.0136171483038,-31.4437574826985,
29.5295507209964));
#32322=CARTESIAN_POINT('Ctrl Pts',(-11.9085950596014,-31.3863041064149,
29.5237419445352));
#32323=CARTESIAN_POINT('Ctrl Pts',(-11.801234779685,-31.3335605461902,29.5179331680739));
#32324=CARTESIAN_POINT('Ctrl Pts',(-11.6938913330252,-31.2808252557454,
29.5121253023836));
#32325=CARTESIAN_POINT('Ctrl Pts',(-11.5842107899159,-31.2327984923111,
29.5063174366933));
#32326=CARTESIAN_POINT('Ctrl Pts',(-11.4726455446039,-31.1896797903643,
29.500509571003));
#32327=CARTESIAN_POINT('Ctrl Pts',(-11.3610715960219,-31.1465577247023,
29.4947012522377));
#32328=CARTESIAN_POINT('Ctrl Pts',(-11.2476130330501,-31.1083446286469,
29.4888929334724));
#32329=CARTESIAN_POINT('Ctrl Pts',(-11.1327406516267,-31.075191263749,29.4830846147071));
#32330=CARTESIAN_POINT('Ctrl Pts',(-11.0178323368642,-31.0420275281154,
29.4772744790361));
#32331=CARTESIAN_POINT('Ctrl Pts',(-10.901509715417,-31.0139267843516,29.4714643433651));
#32332=CARTESIAN_POINT('Ctrl Pts',(-10.7842564873658,-30.9909893038276,
29.4656542076941));
#32333=CARTESIAN_POINT('Ctrl Pts',(-10.6668759668052,-30.9680269219043,
29.4598377644206));
#32334=CARTESIAN_POINT('Ctrl Pts',(-10.5485632231643,-30.950239070429,29.4540213211471));
#32335=CARTESIAN_POINT('Ctrl Pts',(-10.4298099984691,-30.9376745126448,
29.4482048778736));
#32336=CARTESIAN_POINT('Ctrl Pts',(-10.310980176034,-30.9251018505186,29.4423846829007));
#32337=CARTESIAN_POINT('Ctrl Pts',(-10.1917097125356,-30.9177592172505,
29.4365644879278));
#32338=CARTESIAN_POINT('Ctrl Pts',(-10.0724916561893,-30.9156432624239,
29.4307442929548));
#32339=CARTESIAN_POINT('Ctrl Pts',(-9.95310565333495,-30.9135243267803,
29.4249158988764));
#32340=CARTESIAN_POINT('Ctrl Pts',(-9.83377261098454,-30.9166467554624,
29.419087504798));
#32341=CARTESIAN_POINT('Ctrl Pts',(-9.7149818984416,-30.9249552540145,29.4132591107195));
#32342=CARTESIAN_POINT('Ctrl Pts',(-9.68442702794396,-30.9270923326788,
29.4117599545779));
#32343=CARTESIAN_POINT('Ctrl Pts',(-9.65390799075907,-30.9295722576534,
29.4102607984363));
#32344=CARTESIAN_POINT('Ctrl Pts',(-9.62343300298483,-30.9323935420497,
29.4087616422947));
#32345=CARTESIAN_POINT('Ctrl Pts',(-9.50487393027754,-30.943369390977,29.4029293655663));
#32346=CARTESIAN_POINT('Ctrl Pts',(-9.38661087693688,-30.9595500719646,
29.3970970888379));
#32347=CARTESIAN_POINT('Ctrl Pts',(-9.26913546796359,-30.9809127857421,
29.3912648121095));
#32348=CARTESIAN_POINT('Ctrl Pts',(-9.15179778034071,-31.002250455114,29.3854393728038));
#32349=CARTESIAN_POINT('Ctrl Pts',(-9.03524629757056,-31.0287580038616,
29.3796139334981));
#32350=CARTESIAN_POINT('Ctrl Pts',(-8.91996853885142,-31.0603607978738,
29.3737884941924));
#32351=CARTESIAN_POINT('Ctrl Pts',(-8.8047989632097,-31.0919339340618,29.3679685218038));
#32352=CARTESIAN_POINT('Ctrl Pts',(-8.69090112407866,-31.1285926969889,
29.3621485494153));
#32353=CARTESIAN_POINT('Ctrl Pts',(-8.57875273316241,-31.170211336574,29.3563285770267));
#32354=CARTESIAN_POINT('Ctrl Pts',(-8.46668768181303,-31.2117990485695,
29.3505129295684));
#32355=CARTESIAN_POINT('Ctrl Pts',(-8.35636987120471,-31.2583391599235,
29.3446972821102));
#32356=CARTESIAN_POINT('Ctrl Pts',(-8.24826156776168,-31.3096561860689,
29.3388816346519));
#32357=CARTESIAN_POINT('Ctrl Pts',(-8.14019980301785,-31.3609511211486,
29.3330684907263));
#32358=CARTESIAN_POINT('Ctrl Pts',(-8.03434601938491,-31.4170187044427,
29.3272553468007));
#32359=CARTESIAN_POINT('Ctrl Pts',(-7.93114175266072,-31.4776356587632,
29.3214422028751));
#32360=CARTESIAN_POINT('Ctrl Pts',(-7.82794668659896,-31.5382472090811,
29.3156295771914));
#32361=CARTESIAN_POINT('Ctrl Pts',(-7.72740101990802,-31.6034071207539,
29.3098169515077));
#32362=CARTESIAN_POINT('Ctrl Pts',(-7.62992054908888,-31.6728468029908,
29.304004325824));
#32363=CARTESIAN_POINT('Ctrl Pts',(-7.59037664873343,-31.7010156849423,
29.3016463777252));
#32364=CARTESIAN_POINT('Ctrl Pts',(-7.55133683318268,-31.729888342261,29.2992884296264));
#32365=CARTESIAN_POINT('Ctrl Pts',(-7.51282745730978,-31.7594448403263,
29.2969304815276));
#32366=CARTESIAN_POINT('',(-11.0579044229731,-38.9456385074984,30.));
#32367=CARTESIAN_POINT('Ctrl Pts',(-11.057904422973,-38.9456385074984,30.));
#32368=CARTESIAN_POINT('Ctrl Pts',(-12.3607928946041,-38.596308107828,29.9343068491439));
#32369=CARTESIAN_POINT('Ctrl Pts',(-13.821306101938,-37.2193037646235,29.8475124055022));
#32370=CARTESIAN_POINT('Ctrl Pts',(-14.083832240564,-35.4385219893524,29.7607179618605));
#32371=CARTESIAN_POINT('Ctrl Pts',(-14.0807387137482,-35.0044159360451,
29.739616669075));
#32372=CARTESIAN_POINT('',(-8.94137284034965,-38.9454446564172,29.9999998970666));
#32373=CARTESIAN_POINT('Origin',(-10.,-35.,30.));
#32374=CARTESIAN_POINT('',(-14.084999315681,-34.9976354946767,29.6353849714467));
#32375=CARTESIAN_POINT('Ctrl Pts',(-8.94137284034965,-38.9454446564172,
29.9999998970666));
#32376=CARTESIAN_POINT('Ctrl Pts',(-9.05557825458975,-38.9760878319834,
29.9942072407224));
#32377=CARTESIAN_POINT('Ctrl Pts',(-9.17130798408894,-39.0018198448346,
29.9884145843782));
#32378=CARTESIAN_POINT('Ctrl Pts',(-9.28809962572047,-39.0224896341819,
29.982621928034));
#32379=CARTESIAN_POINT('Ctrl Pts',(-9.40474452355768,-39.0431334528067,
29.9768365499193));
#32380=CARTESIAN_POINT('Ctrl Pts',(-9.52244827714246,-39.0587276246669,
29.9710511718046));
#32381=CARTESIAN_POINT('Ctrl Pts',(-9.64073400885775,-39.0691710393652,
29.9652657936899));
#32382=CARTESIAN_POINT('Ctrl Pts',(-9.75890283044874,-39.0796041321009,
29.9594861336721));
#32383=CARTESIAN_POINT('Ctrl Pts',(-9.87765207688717,-39.0848965571337,
29.9537064736543));
#32384=CARTESIAN_POINT('Ctrl Pts',(-9.9964960350032,-39.0849984972126,29.9479268136365));
#32385=CARTESIAN_POINT('Ctrl Pts',(-10.1152571170041,-39.0851003662034,
29.9421511840783));
#32386=CARTESIAN_POINT('Ctrl Pts',(-10.2341123674742,-39.080018949806,29.93637555452));
#32387=CARTESIAN_POINT('Ctrl Pts',(-10.3525729593925,-39.0697564187928,
29.9305999249618));
#32388=CARTESIAN_POINT('Ctrl Pts',(-10.4709899614492,-39.059497664076,29.9248264206579));
#32389=CARTESIAN_POINT('Ctrl Pts',(-10.5890121825612,-39.0440616202775,
29.9190529163541));
#32390=CARTESIAN_POINT('Ctrl Pts',(-10.7061533900576,-39.0235025027593,
29.9132794120503));
#32391=CARTESIAN_POINT('Ctrl Pts',(-10.8232799176483,-39.0029459616692,
29.9075066312706));
#32392=CARTESIAN_POINT('Ctrl Pts',(-10.9395252442958,-38.9772676949977,
29.901733850491));
#32393=CARTESIAN_POINT('Ctrl Pts',(-11.0544115373312,-38.9465733630509,
29.8959610697114));
#32394=CARTESIAN_POINT('Ctrl Pts',(-11.1693113107022,-38.915875429544,29.8901876115748));
#32395=CARTESIAN_POINT('Ctrl Pts',(-11.2828513343666,-38.8801603677232,
29.8844141534383));
#32396=CARTESIAN_POINT('Ctrl Pts',(-11.3945678743728,-38.839584019626,29.8786406953018));
#32397=CARTESIAN_POINT('Ctrl Pts',(-11.5063934549401,-38.7989680671178,
29.8728616020004));
#32398=CARTESIAN_POINT('Ctrl Pts',(-11.6163916076045,-38.7534814918166,
29.8670825086991));
#32399=CARTESIAN_POINT('Ctrl Pts',(-11.7241173983454,-38.7033287994347,
29.8613034153977));
#32400=CARTESIAN_POINT('Ctrl Pts',(-11.8318953367984,-38.6531518292254,
29.855521524563));
#32401=CARTESIAN_POINT('Ctrl Pts',(-11.9373983553712,-38.5983044328783,
29.8497396337283));
#32402=CARTESIAN_POINT('Ctrl Pts',(-12.0402066034073,-38.5390368768089,
29.8439577428936));
#32403=CARTESIAN_POINT('Ctrl Pts',(-12.1431790206705,-38.4796746794139,
29.8381666192535));
#32404=CARTESIAN_POINT('Ctrl Pts',(-12.243447720281,-38.415878441,29.8323754956134));
#32405=CARTESIAN_POINT('Ctrl Pts',(-12.3406218494647,-38.3479418092029,
29.8265843719733));
#32406=CARTESIAN_POINT('Ctrl Pts',(-12.4324632565271,-38.2837334040672,
29.8211110536318));
#32407=CARTESIAN_POINT('Ctrl Pts',(-12.5215404659313,-38.2158271156631,
29.8156377352903));
#32408=CARTESIAN_POINT('Ctrl Pts',(-12.6075527252282,-38.1445021521944,
29.8101644169488));
#32409=CARTESIAN_POINT('Ctrl Pts',(-12.6979864758416,-38.0695107031664,
29.8044097406971));
#32410=CARTESIAN_POINT('Ctrl Pts',(-12.78534229383,-37.9904821524985,29.7986550644455));
#32411=CARTESIAN_POINT('Ctrl Pts',(-12.8692326440361,-37.907701675619,29.7929003881939));
#32412=CARTESIAN_POINT('Ctrl Pts',(-12.9530187460856,-37.8250240676881,
29.7871528631151));
#32413=CARTESIAN_POINT('Ctrl Pts',(-13.0333476462293,-37.7386040943328,
29.7814053380363));
#32414=CARTESIAN_POINT('Ctrl Pts',(-13.1098640485527,-37.6487677511476,
29.7756578129575));
#32415=CARTESIAN_POINT('Ctrl Pts',(-13.1876741568812,-37.5574124941984,
29.7698131112279));
#32416=CARTESIAN_POINT('Ctrl Pts',(-13.2615413177147,-37.462524548608,29.7639684094983));
#32417=CARTESIAN_POINT('Ctrl Pts',(-13.3311298526084,-37.3644870278903,
29.7581237077686));
#32418=CARTESIAN_POINT('Ctrl Pts',(-13.3994484814726,-37.2682385725532,
29.752385664729));
#32419=CARTESIAN_POINT('Ctrl Pts',(-13.463643061243,-37.1689548732471,29.7466476216893));
#32420=CARTESIAN_POINT('Ctrl Pts',(-13.5234363250196,-37.0670320422123,
29.7409095786496));
#32421=CARTESIAN_POINT('Ctrl Pts',(-13.583209723368,-36.9651430735317,29.73517344199));
#32422=CARTESIAN_POINT('Ctrl Pts',(-13.6385845006397,-36.860617077093,29.7294373053303));
#32423=CARTESIAN_POINT('Ctrl Pts',(-13.6893274390699,-36.7538780024066,
29.7237011686706));
#32424=CARTESIAN_POINT('Ctrl Pts',(-13.7400661989603,-36.6471477173861,
29.7179655043658));
#32425=CARTESIAN_POINT('Ctrl Pts',(-13.7861736993804,-36.5382050952904,
29.712229840061));
#32426=CARTESIAN_POINT('Ctrl Pts',(-13.8274636531967,-36.4274967542725,
29.7064941757563));
#32427=CARTESIAN_POINT('Ctrl Pts',(-13.8701221202582,-36.3131190986384,
29.7005684087305));
#32428=CARTESIAN_POINT('Ctrl Pts',(-13.907637959032,-36.1968570825576,29.6946426417047));
#32429=CARTESIAN_POINT('Ctrl Pts',(-13.9398609751301,-36.0792221720512,
29.6887168746789));
#32430=CARTESIAN_POINT('Ctrl Pts',(-13.9710834565762,-35.9652398620303,
29.6829751045586));
#32431=CARTESIAN_POINT('Ctrl Pts',(-13.9973368939361,-35.8499690830318,
29.6772333344383));
#32432=CARTESIAN_POINT('Ctrl Pts',(-14.0185365737413,-35.7338860984535,
29.6714915643181));
#32433=CARTESIAN_POINT('Ctrl Pts',(-14.0407552795788,-35.61222323794,29.6654737988395));
#32434=CARTESIAN_POINT('Ctrl Pts',(-14.0574222078387,-35.4896686666685,
29.659456033361));
#32435=CARTESIAN_POINT('Ctrl Pts',(-14.0685010078323,-35.3667758842506,
29.6534382678824));
#32436=CARTESIAN_POINT('Ctrl Pts',(-14.0795798078258,-35.2438831018327,
29.6474205024038));
#32437=CARTESIAN_POINT('Ctrl Pts',(-14.0850705212451,-35.1206526339226,
29.6414027369253));
#32438=CARTESIAN_POINT('Ctrl Pts',(-14.084999315681,-34.9976354946767,29.6353849714467));
#32439=CARTESIAN_POINT('Ctrl Pts',(-14.0849993156805,-34.9976354938135,
29.6353849714045));
#32440=CARTESIAN_POINT('Ctrl Pts',(-14.0849113602667,-34.8456808034869,
29.6279516357298));
#32441=CARTESIAN_POINT('Ctrl Pts',(-14.076345106143,-34.6939815686482,29.6205183000551));
#32442=CARTESIAN_POINT('Ctrl Pts',(-14.0593832455855,-34.543236751194,29.6130849643803));
#32443=CARTESIAN_POINT('Ctrl Pts',(-14.0461086539941,-34.4252617283806,
29.6072675309148));
#32444=CARTESIAN_POINT('Ctrl Pts',(-14.0276649934632,-34.3076716578208,
29.6014500974494));
#32445=CARTESIAN_POINT('Ctrl Pts',(-14.0040819085924,-34.1909554590241,
29.5956326639839));
#32446=CARTESIAN_POINT('Ctrl Pts',(-13.9805289239898,-34.0743882309371,
29.589822655599));
#32447=CARTESIAN_POINT('Ctrl Pts',(-13.9518496417305,-33.9586930538953,
29.5840126472142));
#32448=CARTESIAN_POINT('Ctrl Pts',(-13.9181254752496,-33.8443539641396,
29.5782026388294));
#32449=CARTESIAN_POINT('Ctrl Pts',(-13.8844355082274,-33.7301308249135,
29.5723985223364));
#32450=CARTESIAN_POINT('Ctrl Pts',(-13.8457109491444,-33.6172614276375,
29.5665944058434));
#32451=CARTESIAN_POINT('Ctrl Pts',(-13.8020841697217,-33.5062192375213,
29.5607902893504));
#32452=CARTESIAN_POINT('Ctrl Pts',(-13.7567392439761,-33.3908038909825,
29.5547575902863));
#32453=CARTESIAN_POINT('Ctrl Pts',(-13.7060981315312,-33.2773630695008,
29.5487248912222));
#32454=CARTESIAN_POINT('Ctrl Pts',(-13.650366626008,-33.166411034139,29.5426921921581));
#32455=CARTESIAN_POINT('Ctrl Pts',(-13.596808482337,-33.05978579596,29.5368947502953));
#32456=CARTESIAN_POINT('Ctrl Pts',(-13.53854972168,-32.955459273906,29.5310973084325));
#32457=CARTESIAN_POINT('Ctrl Pts',(-13.4758216114673,-32.8538664707767,
29.5252998665696));
#32458=CARTESIAN_POINT('Ctrl Pts',(-13.4131031963228,-32.7522893695255,
29.519503320742));
#32459=CARTESIAN_POINT('Ctrl Pts',(-13.3459170202657,-32.6534454952016,
29.5137067749143));
#32460=CARTESIAN_POINT('Ctrl Pts',(-13.2745391055131,-32.5577431243897,
29.5079102290867));
#32461=CARTESIAN_POINT('Ctrl Pts',(-13.2031552746485,-32.4620328213492,
29.5021132028161));
#32462=CARTESIAN_POINT('Ctrl Pts',(-13.127579259126,-32.3694648676279,29.4963161765455));
#32463=CARTESIAN_POINT('Ctrl Pts',(-13.048128600517,-32.280416018081,29.490519150275));
#32464=CARTESIAN_POINT('Ctrl Pts',(-12.9686524918513,-32.191338643934,29.4847202670702));
#32465=CARTESIAN_POINT('Ctrl Pts',(-12.885299544286,-32.1057829209723,29.4789213838654));
#32466=CARTESIAN_POINT('Ctrl Pts',(-12.7984250584702,-32.0240896868141,
29.4731225006606));
#32467=CARTESIAN_POINT('Ctrl Pts',(-12.7114543284358,-31.9423059485061,
29.4673171931417));
#32468=CARTESIAN_POINT('Ctrl Pts',(-12.620954571213,-31.864393520882,29.4615118856228));
#32469=CARTESIAN_POINT('Ctrl Pts',(-12.5273152611175,-31.7906538717485,
29.4557065781039));
#32470=CARTESIAN_POINT('Ctrl Pts',(-12.4336145483529,-31.7168658688707,
29.4498974638358));
#32471=CARTESIAN_POINT('Ctrl Pts',(-12.3367705145969,-31.6472563318031,
29.4440883495676));
#32472=CARTESIAN_POINT('Ctrl Pts',(-12.237201387277,-31.5820832437337,29.4382792352994));
#32473=CARTESIAN_POINT('Ctrl Pts',(-12.1374888867239,-31.5168163105478,
29.4324617562749));
#32474=CARTESIAN_POINT('Ctrl Pts',(-12.0350438114514,-31.4559987848715,
29.4266442772504));
#32475=CARTESIAN_POINT('Ctrl Pts',(-11.9303088245547,-31.3998426642928,
29.4208267982258));
#32476=CARTESIAN_POINT('Ctrl Pts',(-11.9013754803315,-31.3843293729363,
29.4192197027545));
#32477=CARTESIAN_POINT('Ctrl Pts',(-11.8722674942299,-31.3691715354047,
29.4176126072832));
#32478=CARTESIAN_POINT('Ctrl Pts',(-11.8429944425675,-31.3543729641301,
29.4160055118119));
#32479=CARTESIAN_POINT('Ctrl Pts',(-11.7368984678678,-31.3007376663264,
29.4101808249146));
#32480=CARTESIAN_POINT('Ctrl Pts',(-11.6282885062496,-31.2516513740434,
29.4043561380172));
#32481=CARTESIAN_POINT('Ctrl Pts',(-11.5175912617084,-31.2073568896631,
29.3985314511199));
#32482=CARTESIAN_POINT('Ctrl Pts',(-11.4070336019806,-31.1631182588621,
29.3927141089206));
#32483=CARTESIAN_POINT('Ctrl Pts',(-11.2943942699428,-31.1236595682043,
29.3868967667213));
#32484=CARTESIAN_POINT('Ctrl Pts',(-11.180124143974,-31.0891775794841,29.381079424522));
#32485=CARTESIAN_POINT('Ctrl Pts',(-11.0659683568885,-31.0547300935008,
29.3752679031652));
#32486=CARTESIAN_POINT('Ctrl Pts',(-10.9501854106313,-31.0252495201162,
29.3694563818085));
#32487=CARTESIAN_POINT('Ctrl Pts',(-10.8332451644592,-31.0008841607294,
29.3636448604517));
#32488=CARTESIAN_POINT('Ctrl Pts',(-10.7119096655413,-30.9756030181433,
29.3576149104014));
#32489=CARTESIAN_POINT('Ctrl Pts',(-10.5893285799952,-30.9558293168082,
29.351584960351));
#32490=CARTESIAN_POINT('Ctrl Pts',(-10.466043334308,-30.9416716975401,29.3455550103007));
#32491=CARTESIAN_POINT('Ctrl Pts',(-10.3473577671624,-30.9280422882552,
29.3397500330904));
#32492=CARTESIAN_POINT('Ctrl Pts',(-10.2280200838256,-30.9196174540592,
29.33394505588));
#32493=CARTESIAN_POINT('Ctrl Pts',(-10.1085219886427,-30.9164417503872,
29.3281400786697));
#32494=CARTESIAN_POINT('Ctrl Pts',(-9.98904161281289,-30.9132665176131,
29.3223359622299));
#32495=CARTESIAN_POINT('Ctrl Pts',(-9.86940128034394,-30.9153388782924,
29.3165318457901));
#32496=CARTESIAN_POINT('Ctrl Pts',(-9.75009481274481,-30.9226513029442,
29.3107277293503));
#32497=CARTESIAN_POINT('Ctrl Pts',(-9.6307779101942,-30.9299643671656,29.3049231052627));
#32498=CARTESIAN_POINT('Ctrl Pts',(-9.51179533798562,-30.9425183816275,
29.299118481175));
#32499=CARTESIAN_POINT('Ctrl Pts',(-9.3936372666126,-30.9602538154534,29.2933138570874));
#32500=CARTESIAN_POINT('Ctrl Pts',(-9.27544100576304,-30.9779949814898,
29.2875073569065));
#32501=CARTESIAN_POINT('Ctrl Pts',(-9.15807017916034,-31.0009208368988,
29.2817008567256));
#32502=CARTESIAN_POINT('Ctrl Pts',(-9.04200558532037,-31.0289205873664,
29.2758943565448));
#32503=CARTESIAN_POINT('Ctrl Pts',(-8.92581277050846,-31.0569512702234,
29.2700814417023));
#32504=CARTESIAN_POINT('Ctrl Pts',(-8.81092946592161,-31.0900669411032,
29.2642685268598));
#32505=CARTESIAN_POINT('Ctrl Pts',(-8.69782225691509,-31.1281066484968,
29.2584556120173));
#32506=CARTESIAN_POINT('Ctrl Pts',(-8.58464091024233,-31.1661712895367,
29.2526388870203));
#32507=CARTESIAN_POINT('Ctrl Pts',(-8.47323835756487,-31.2091662482557,
29.2468221620233));
#32508=CARTESIAN_POINT('Ctrl Pts',(-8.36406057817883,-31.2568826884358,
29.2410054370263));
#32509=CARTESIAN_POINT('Ctrl Pts',(-8.25472678958248,-31.3046673128582,
29.2351804002403));
#32510=CARTESIAN_POINT('Ctrl Pts',(-8.14762448475744,-31.3571867058625,
29.2293553634542));
#32511=CARTESIAN_POINT('Ctrl Pts',(-8.04317458259696,-31.4141863844024,
29.2235303266682));
#32512=CARTESIAN_POINT('Ctrl Pts',(-8.01565456857819,-31.4292044162055,
29.2219955708599));
#32513=CARTESIAN_POINT('Ctrl Pts',(-7.98831852233574,-31.4445332365823,
29.2204608150517));
#32514=CARTESIAN_POINT('Ctrl Pts',(-7.96117378602652,-31.4601677060608,
29.2189260592434));
#32515=CARTESIAN_POINT('Ctrl Pts',(-7.85816142420679,-31.5194994162102,
29.2131017690818));
#32516=CARTESIAN_POINT('Ctrl Pts',(-7.75757567177424,-31.583426782036,29.2072774789202));
#32517=CARTESIAN_POINT('Ctrl Pts',(-7.65985340609903,-31.651725979097,29.2014531887587));
#32518=CARTESIAN_POINT('Ctrl Pts',(-7.61008386709288,-31.686510472976,29.1984869022693));
#32519=CARTESIAN_POINT('Ctrl Pts',(-7.56105674097248,-31.7224281736847,
29.19552061578));
#32520=CARTESIAN_POINT('Ctrl Pts',(-7.5128274573098,-31.7594448403263,29.1925543292906));
#32521=CARTESIAN_POINT('Origin',(-10.,-35.,23.));
#32522=CARTESIAN_POINT('',(-13.1787500647504,-33.8227349116068,17.9149431671188));
#32523=CARTESIAN_POINT('',(-13.1787501240207,-33.8227350716434,17.5703580349972));
#32524=CARTESIAN_POINT('',(-13.1787501240207,-33.8227350716434,23.));
#32525=CARTESIAN_POINT('',(-6.62123117139838,-35.2726284383003,17.));
#32526=CARTESIAN_POINT('Ctrl Pts',(-13.1787501240207,-33.8227350716434,
17.5703580349972));
#32527=CARTESIAN_POINT('Ctrl Pts',(-13.1427561410128,-33.7255471955804,
17.5642606734842));
#32528=CARTESIAN_POINT('Ctrl Pts',(-13.1022543457953,-33.6298857670595,
17.5581633119711));
#32529=CARTESIAN_POINT('Ctrl Pts',(-13.0573978208791,-33.5361954955036,
17.5520659504581));
#32530=CARTESIAN_POINT('Ctrl Pts',(-13.01258486052,-33.4425962157308,17.545974510689));
#32531=CARTESIAN_POINT('Ctrl Pts',(-12.9634257646823,-33.3509646690272,
17.5398830709199));
#32532=CARTESIAN_POINT('Ctrl Pts',(-12.9101220782721,-33.2617265600448,
17.5337916311508));
#32533=CARTESIAN_POINT('Ctrl Pts',(-12.8568522287991,-33.1725450990076,
17.5277040581999));
#32534=CARTESIAN_POINT('Ctrl Pts',(-12.7994432384854,-33.085754420227,17.521616485249));
#32535=CARTESIAN_POINT('Ctrl Pts',(-12.7381426726736,-33.001755829088,17.5155289122981));
#32536=CARTESIAN_POINT('Ctrl Pts',(-12.6768617435676,-32.9177841456227,
17.5094432894088));
#32537=CARTESIAN_POINT('Ctrl Pts',(-12.6116919681767,-32.8366031166276,
17.5033576665195));
#32538=CARTESIAN_POINT('Ctrl Pts',(-12.5429238704387,-32.7585845428272,
17.4972720436302));
#32539=CARTESIAN_POINT('Ctrl Pts',(-12.4741600755362,-32.6805708506667,
17.4911868015197));
#32540=CARTESIAN_POINT('Ctrl Pts',(-12.4017986884822,-32.6057195403265,
17.4851015594092));
#32541=CARTESIAN_POINT('Ctrl Pts',(-12.3261695030696,-32.53436813261,17.4790163172987));
#32542=CARTESIAN_POINT('Ctrl Pts',(-12.2505255555982,-32.4630027978142,
17.47292988741));
#32543=CARTESIAN_POINT('Ctrl Pts',(-12.171612852793,-32.3951390161126,17.4668434575212));
#32544=CARTESIAN_POINT('Ctrl Pts',(-12.0897962284543,-32.3310757249337,
17.4607570276325));
#32545=CARTESIAN_POINT('Ctrl Pts',(-12.0078921757233,-32.2669439763894,
17.4546640938482));
#32546=CARTESIAN_POINT('Ctrl Pts',(-11.9230783421455,-32.2066210909662,
17.4485711600638));
#32547=CARTESIAN_POINT('Ctrl Pts',(-11.8357506295315,-32.1503641129655,
17.4424782262795));
#32548=CARTESIAN_POINT('Ctrl Pts',(-11.7483725193403,-32.094074668577,17.4363817762105));
#32549=CARTESIAN_POINT('Ctrl Pts',(-11.6584780096167,-32.0418560193866,
17.4302853261415));
#32550=CARTESIAN_POINT('Ctrl Pts',(-11.5664880974162,-31.9939194782652,
17.4241888760725));
#32551=CARTESIAN_POINT('Ctrl Pts',(-11.4743515815419,-31.9459065410165,
17.418082710134));
#32552=CARTESIAN_POINT('Ctrl Pts',(-11.3801133808725,-31.9021895209563,
17.4119765441955));
#32553=CARTESIAN_POINT('Ctrl Pts',(-11.284215100619,-31.8629318404213,17.405870378257));
#32554=CARTESIAN_POINT('Ctrl Pts',(-11.2229049351904,-31.8378334248755,
17.4019665538836));
#32555=CARTESIAN_POINT('Ctrl Pts',(-11.1609165924618,-31.8145567073918,
17.3980627295102));
#32556=CARTESIAN_POINT('Ctrl Pts',(-11.0983682718265,-31.7931335852666,
17.3941589051368));
#32557=CARTESIAN_POINT('Ctrl Pts',(-11.0015147354448,-31.7599607499757,
17.3881139915062));
#32558=CARTESIAN_POINT('Ctrl Pts',(-10.9029758716802,-31.7311176974456,
17.3820690778757));
#32559=CARTESIAN_POINT('Ctrl Pts',(-10.8031787497248,-31.706778331407,17.3760241642451));
#32560=CARTESIAN_POINT('Ctrl Pts',(-10.7035144749785,-31.6824713652691,
17.3699872974388));
#32561=CARTESIAN_POINT('Ctrl Pts',(-10.6025956903531,-31.6626562751579,
17.3639504306325));
#32562=CARTESIAN_POINT('Ctrl Pts',(-10.5008673376754,-31.6474581326179,
17.3579135638262));
#32563=CARTESIAN_POINT('Ctrl Pts',(-10.3992439061861,-31.6322756652278,
17.3518829233592));
#32564=CARTESIAN_POINT('Ctrl Pts',(-10.2968129954217,-31.6217007449999,
17.3458522828922));
#32565=CARTESIAN_POINT('Ctrl Pts',(-10.1940315703266,-31.6158078050713,
17.3398216424252));
#32566=CARTESIAN_POINT('Ctrl Pts',(-10.0913190575091,-31.6099188162059,
17.3337950453461));
#32567=CARTESIAN_POINT('Ctrl Pts',(-9.98825693183714,-31.6087055948162,
17.327768448267));
#32568=CARTESIAN_POINT('Ctrl Pts',(-9.88530824168519,-31.6121908461257,
17.3217418511879));
#32569=CARTESIAN_POINT('Ctrl Pts',(-9.782394873529,-31.6156749016352,17.3157173218519));
#32570=CARTESIAN_POINT('Ctrl Pts',(-9.67959529947481,-31.6238542132337,
17.3096927925158));
#32571=CARTESIAN_POINT('Ctrl Pts',(-9.57737257670802,-31.6366993706209,
17.3036682631798));
#32572=CARTESIAN_POINT('Ctrl Pts',(-9.47515720184965,-31.6495436046807,
17.2976441668951));
#32573=CARTESIAN_POINT('Ctrl Pts',(-9.37351902910539,-31.6670529636749,
17.2916200706104));
#32574=CARTESIAN_POINT('Ctrl Pts',(-9.2729149678679,-31.6891462704388,17.2855959743257));
#32575=CARTESIAN_POINT('Ctrl Pts',(-9.17229085089137,-31.7112439815735,
17.2795706771182));
#32576=CARTESIAN_POINT('Ctrl Pts',(-9.07270168135648,-31.7379273619785,
17.2735453799108));
#32577=CARTESIAN_POINT('Ctrl Pts',(-8.97459215180163,-31.7690645615622,
17.2675200827034));
#32578=CARTESIAN_POINT('Ctrl Pts',(-8.87636670556745,-31.8002385498329,
17.2614876665907));
#32579=CARTESIAN_POINT('Ctrl Pts',(-8.77962480708826,-31.8358767325254,
17.2554552504781));
#32580=CARTESIAN_POINT('Ctrl Pts',(-8.68479394402274,-31.8757980070391,
17.2494228343654));
#32581=CARTESIAN_POINT('Ctrl Pts',(-8.58990614490615,-31.915743250118,17.2433867964155));
#32582=CARTESIAN_POINT('Ctrl Pts',(-8.49693205876363,-31.9599765155484,
17.2373507584656));
#32583=CARTESIAN_POINT('Ctrl Pts',(-8.40627520250295,-32.0082703443755,
17.2313147205157));
#32584=CARTESIAN_POINT('Ctrl Pts',(-8.31545155112396,-32.0566530266576,
17.2252675771546));
#32585=CARTESIAN_POINT('Ctrl Pts',(-8.22695402074023,-32.109110971783,17.2192204337935));
#32586=CARTESIAN_POINT('Ctrl Pts',(-8.14115796984813,-32.1653727988603,
17.2131732904325));
#32587=CARTESIAN_POINT('Ctrl Pts',(-8.0650455726394,-32.2152844496377,17.2078086778111));
#32588=CARTESIAN_POINT('Ctrl Pts',(-7.99105895925869,-32.2681890221868,
17.2024440651898));
#32589=CARTESIAN_POINT('Ctrl Pts',(-7.91943702063162,-32.3238716863009,
17.1970794525685));
#32590=CARTESIAN_POINT('Ctrl Pts',(-7.83581776040074,-32.3888816995757,
17.1908162188803));
#32591=CARTESIAN_POINT('Ctrl Pts',(-7.75513118295744,-32.4579052413955,
17.1845529851921));
#32592=CARTESIAN_POINT('Ctrl Pts',(-7.67777316876516,-32.5306544173014,
17.178289751504));
#32593=CARTESIAN_POINT('Ctrl Pts',(-7.60052793358127,-32.6032975333504,
17.1720356488837));
#32594=CARTESIAN_POINT('Ctrl Pts',(-7.52660189303604,-32.6796552011327,
17.1657815462635));
#32595=CARTESIAN_POINT('Ctrl Pts',(-7.45635876139179,-32.7593986718401,
17.1595274436433));
#32596=CARTESIAN_POINT('Ctrl Pts',(-7.3862020003943,-32.8390440903256,17.1532810310403));
#32597=CARTESIAN_POINT('Ctrl Pts',(-7.3197193970536,-32.9220667257876,17.1470346184372));
#32598=CARTESIAN_POINT('Ctrl Pts',(-7.25723821870783,-33.0081006868863,
17.1407882058342));
#32599=CARTESIAN_POINT('Ctrl Pts',(-7.19483021640349,-33.0940338876461,
17.1345491088381));
#32600=CARTESIAN_POINT('Ctrl Pts',(-7.13641453710058,-33.1829710653652,
17.1283100118421));
#32601=CARTESIAN_POINT('Ctrl Pts',(-7.08227801460293,-33.2745135531014,
17.1220709148461));
#32602=CARTESIAN_POINT('Ctrl Pts',(-7.02817855180624,-33.3659933745071,
17.1158360888867));
#32603=CARTESIAN_POINT('Ctrl Pts',(-6.97835261871944,-33.4600746128199,
17.1096012629272));
#32604=CARTESIAN_POINT('Ctrl Pts',(-6.93304349073857,-33.5563300817711,
17.1033664369678));
#32605=CARTESIAN_POINT('Ctrl Pts',(-6.88775601855788,-33.6525395447784,
17.0971345909851));
#32606=CARTESIAN_POINT('Ctrl Pts',(-6.84698122377164,-33.7509208080942,
17.0909027450024));
#32607=CARTESIAN_POINT('Ctrl Pts',(-6.81091594762553,-33.8510230770852,
17.0846708990196));
#32608=CARTESIAN_POINT('Ctrl Pts',(-6.77486046283198,-33.9510981693368,
17.0784407449191));
#32609=CARTESIAN_POINT('Ctrl Pts',(-6.74351208542603,-34.0528929604214,
17.0722105908187));
#32610=CARTESIAN_POINT('Ctrl Pts',(-6.71701891222609,-34.1559382488118,
17.0659804367182));
#32611=CARTESIAN_POINT('Ctrl Pts',(-6.6905202480665,-34.2590048943087,17.0597489913596));
#32612=CARTESIAN_POINT('Ctrl Pts',(-6.6688789034052,-34.3633221685375,17.053517546001));
#32613=CARTESIAN_POINT('Ctrl Pts',(-6.65219258767227,-34.4684074939735,
17.0472861006425));
#32614=CARTESIAN_POINT('Ctrl Pts',(-6.63550481518413,-34.5735019936094,
17.0410541112638));
#32615=CARTESIAN_POINT('Ctrl Pts',(-6.62377298967071,-34.6793642816695,
17.0348221218852));
#32616=CARTESIAN_POINT('Ctrl Pts',(-6.61704319803061,-34.7855044557361,
17.0285901325065));
#32617=CARTESIAN_POINT('Ctrl Pts',(-6.61030887275071,-34.8917161329553,
17.0223539448411));
#32618=CARTESIAN_POINT('Ctrl Pts',(-6.60858333145876,-34.9982056700471,
17.0161177571757));
#32619=CARTESIAN_POINT('Ctrl Pts',(-6.61186057071778,-35.1044809563661,
17.0098815695103));
#32620=CARTESIAN_POINT('Ctrl Pts',(-6.61359155708732,-35.1606138955556,
17.0065877130069));
#32621=CARTESIAN_POINT('Ctrl Pts',(-6.61671733632887,-35.2166870797046,
17.0032938565034));
#32622=CARTESIAN_POINT('Ctrl Pts',(-6.62123117139838,-35.2726284383002,
17.));
#32623=CARTESIAN_POINT('',(-13.1787501240207,-33.8227350716434,17.));
#32624=CARTESIAN_POINT('Origin',(-10.,-35.,17.));
#32625=CARTESIAN_POINT('',(-13.1787501240207,-33.8227350716434,16.));
#32626=CARTESIAN_POINT('',(-13.1787501240207,-33.8227350716434,23.));
#32627=CARTESIAN_POINT('Origin',(-10.,-35.,16.));
#32628=CARTESIAN_POINT('',(-10.7859688154841,-38.3003672135327,16.9983147074305));
#32629=CARTESIAN_POINT('Origin',(-10.,-35.,17.));
#32630=CARTESIAN_POINT('Ctrl Pts',(-10.7851704499296,-38.2975615880613,
16.9966427327388));
#32631=CARTESIAN_POINT('Ctrl Pts',(-10.743310784149,-38.3075286415149,16.9992508007924));
#32632=CARTESIAN_POINT('Ctrl Pts',(-10.7012668042908,-38.3166973331851,
17.0018967864938));
#32633=CARTESIAN_POINT('Ctrl Pts',(-10.4536050921614,-38.3657864213433,
17.0175939914567));
#32634=CARTESIAN_POINT('Ctrl Pts',(-10.2448259397233,-38.3873780071541,
17.0312412363625));
#32635=CARTESIAN_POINT('Ctrl Pts',(-9.87026006962071,-38.3912897903155,
17.0553063052265));
#32636=CARTESIAN_POINT('Ctrl Pts',(-9.70520066741884,-38.3809441326568,
17.0657713163129));
#32637=CARTESIAN_POINT('Ctrl Pts',(-9.47799215449731,-38.3499292672403,
17.0798307027395));
#32638=CARTESIAN_POINT('Ctrl Pts',(-9.41470309195617,-38.3394530452039,
17.0837111912157));
#32639=CARTESIAN_POINT('Ctrl Pts',(-9.31979469515452,-38.3209615248075,
17.0894789550261));
#32640=CARTESIAN_POINT('Ctrl Pts',(-9.28793387478838,-38.3142761877813,
17.0914064393494));
#32641=CARTESIAN_POINT('Ctrl Pts',(-9.23261394171108,-38.3018338584622,
17.0947390357368));
#32642=CARTESIAN_POINT('Ctrl Pts',(-9.2091112994877,-38.2962832552482,17.0961504272415));
#32643=CARTESIAN_POINT('Ctrl Pts',(-9.155972702891,-38.2831324826891,17.0993322820044));
#32644=CARTESIAN_POINT('Ctrl Pts',(-9.1263760784018,-38.2753812461509,17.1010979086763));
#32645=CARTESIAN_POINT('Ctrl Pts',(-9.04609325646344,-38.2531898497246,
17.1058720754798));
#32646=CARTESIAN_POINT('Ctrl Pts',(-8.99563138749464,-38.2379663945757,
17.1088561314373));
#32647=CARTESIAN_POINT('Ctrl Pts',(-8.76968187411001,-38.164010562092,17.1221720717703));
#32648=CARTESIAN_POINT('Ctrl Pts',(-8.59882344241059,-38.0921445722062,
17.1320944660758));
#32649=CARTESIAN_POINT('Ctrl Pts',(-8.29718144020483,-37.9351050419574,
17.1502153077104));
#32650=CARTESIAN_POINT('Ctrl Pts',(-8.16476885351069,-37.854181934104,17.1584174494901));
#32651=CARTESIAN_POINT('Ctrl Pts',(-7.9757713259831,-37.7200724455312,17.1711242245388));
#32652=CARTESIAN_POINT('Ctrl Pts',(-7.91470806847342,-37.6735466616793,
17.1754029777835));
#32653=CARTESIAN_POINT('Ctrl Pts',(-7.83652006488241,-37.6096640687498,
17.1811898260787));
#32654=CARTESIAN_POINT('Ctrl Pts',(-7.81792477349181,-37.5941356203807,
17.1825901036778));
#32655=CARTESIAN_POINT('Ctrl Pts',(-7.7874099083126,-37.5680932035323,17.184931071396));
#32656=CARTESIAN_POINT('Ctrl Pts',(-7.77539469403909,-37.5576920898364,
17.185864133032));
#32657=CARTESIAN_POINT('Ctrl Pts',(-7.75262087849325,-37.5376957961096,
17.1876553464526));
#32658=CARTESIAN_POINT('Ctrl Pts',(-7.74184944242308,-37.528115683896,17.188512393171));
#32659=CARTESIAN_POINT('Ctrl Pts',(-7.71229652554076,-37.5014917769243,
17.1908903428796));
#32660=CARTESIAN_POINT('Ctrl Pts',(-7.69364509275221,-37.4843057895331,
17.1924210383931));
#32661=CARTESIAN_POINT('Ctrl Pts',(-7.61451756643669,-37.4097362461635,
17.1990378438738));
#32662=CARTESIAN_POINT('Ctrl Pts',(-7.55598058899076,-37.3503451320522,
17.2042454098228));
#32663=CARTESIAN_POINT('Ctrl Pts',(-7.36537999728428,-37.1421371666012,
17.2221251233073));
#32664=CARTESIAN_POINT('Ctrl Pts',(-7.24423963964011,-36.9838752006094,
17.2350787935645));
#32665=CARTESIAN_POINT('Ctrl Pts',(-7.08015664818693,-36.7252385742279,
17.2546065819693));
#32666=CARTESIAN_POINT('Ctrl Pts',(-7.02697486690723,-36.6318878458345,
17.2613681618698));
#32667=CARTESIAN_POINT('Ctrl Pts',(-6.94433807822268,-36.4693383033307,
17.272621959888));
#32668=CARTESIAN_POINT('Ctrl Pts',(-6.91258980521957,-36.4014008782826,
17.2771806671139));
#32669=CARTESIAN_POINT('Ctrl Pts',(-6.86963337246016,-36.3009176606076,
17.2837169481035));
#32670=CARTESIAN_POINT('Ctrl Pts',(-6.85662736934266,-36.2691692622874,
17.2857530480205));
#32671=CARTESIAN_POINT('Ctrl Pts',(-6.83436650218949,-36.2123867170112,
17.2893444951596));
#32672=CARTESIAN_POINT('Ctrl Pts',(-6.82492124245694,-36.1874308137927,
17.2909059816516));
#32673=CARTESIAN_POINT('Ctrl Pts',(-6.80551948703197,-36.1342808994909,
17.2941967983839));
#32674=CARTESIAN_POINT('Ctrl Pts',(-6.79563932667782,-36.1060613293273,
17.2959235384772));
#32675=CARTESIAN_POINT('Ctrl Pts',(-6.76978587126011,-36.0289633729162,
17.3005880348398));
#32676=CARTESIAN_POINT('Ctrl Pts',(-6.754548971306,-35.9798453703461,17.3035021502739));
#32677=CARTESIAN_POINT('Ctrl Pts',(-6.67131670554485,-35.6882486125514,
17.3205003365769));
#32678=CARTESIAN_POINT('Ctrl Pts',(-6.6293955554992,-35.4391531640892,17.333727087924));
#32679=CARTESIAN_POINT('Ctrl Pts',(-6.60889389514483,-35.0694671655412,
17.3533940834857));
#32680=CARTESIAN_POINT('Ctrl Pts',(-6.60853713860263,-34.9509815624263,
17.3597169713223));
#32681=CARTESIAN_POINT('Ctrl Pts',(-6.61764102105995,-34.7667172823524,
17.3698807385786));
#32682=CARTESIAN_POINT('Ctrl Pts',(-6.6228320213891,-34.7008204603456,17.3735823273943));
#32683=CARTESIAN_POINT('Ctrl Pts',(-6.63239785953204,-34.6124692984434,
17.378684005663));
#32684=CARTESIAN_POINT('Ctrl Pts',(-6.63507874324607,-34.5898425955063,
17.3800028587966));
#32685=CARTESIAN_POINT('Ctrl Pts',(-6.63995072011255,-34.5519928678066,
17.3822321999947));
#32686=CARTESIAN_POINT('Ctrl Pts',(-6.64201774271023,-34.5367541650539,
17.3831360751198));
#32687=CARTESIAN_POINT('Ctrl Pts',(-6.64650987282731,-34.5052480139126,
17.3850188527511));
#32688=CARTESIAN_POINT('Ctrl Pts',(-6.64894979124846,-34.4889833327116,
17.3859984918382));
#32689=CARTESIAN_POINT('Ctrl Pts',(-6.65589118590911,-34.444900542759,17.3886733059703));
#32690=CARTESIAN_POINT('Ctrl Pts',(-6.66062125647275,-34.4171203706953,
17.3903802186767));
#32691=CARTESIAN_POINT('Ctrl Pts',(-6.69129122312531,-34.2496399665877,
17.4007866703774));
#32692=CARTESIAN_POINT('Ctrl Pts',(-6.72564565888985,-34.1116362216724,
17.4098446557825));
#32693=CARTESIAN_POINT('Ctrl Pts',(-6.8285199248545,-33.7869285076647,17.4317545759383));
#32694=CARTESIAN_POINT('Ctrl Pts',(-6.90500801021866,-33.6032665645102,
17.4446235142211));
#32695=CARTESIAN_POINT('Ctrl Pts',(-7.04728568991387,-33.331597609153,17.4638622851735));
#32696=CARTESIAN_POINT('Ctrl Pts',(-7.10198759315005,-33.2382916739901,
17.4705173604536));
#32697=CARTESIAN_POINT('Ctrl Pts',(-7.18221228691058,-33.1153313416155,
17.4793444461009));
#32698=CARTESIAN_POINT('Ctrl Pts',(-7.20391901803817,-33.0832749603318,
17.4816515973875));
#32699=CARTESIAN_POINT('Ctrl Pts',(-7.2417591886613,-33.029404104059,17.4855403539966));
#32700=CARTESIAN_POINT('Ctrl Pts',(-7.25761367514143,-33.0073992201757,
17.4871322078223));
#32701=CARTESIAN_POINT('Ctrl Pts',(-7.28829108222011,-32.9658809982845,
17.4901430954114));
#32702=CARTESIAN_POINT('Ctrl Pts',(-7.30306476304412,-32.9463335855415,
17.49156387896));
#32703=CARTESIAN_POINT('Ctrl Pts',(-7.34205426499023,-32.8958920610367,
17.4952397728289));
#32704=CARTESIAN_POINT('Ctrl Pts',(-7.36659742194331,-32.8652548647136,
17.4974819577439));
#32705=CARTESIAN_POINT('Ctrl Pts',(-7.45796147147842,-32.755179448133,17.5055816764898));
#32706=CARTESIAN_POINT('Ctrl Pts',(-7.52789198927584,-32.6783919661395,
17.5113151602841));
#32707=CARTESIAN_POINT('Ctrl Pts',(-7.78132600292532,-32.424567658594,17.5307906942772));
#32708=CARTESIAN_POINT('Ctrl Pts',(-7.98116525377509,-32.2651027509197,
17.5439231045514));
#32709=CARTESIAN_POINT('Ctrl Pts',(-8.25195591528014,-32.0950108486595,
17.5612419288636));
#32710=CARTESIAN_POINT('Ctrl Pts',(-8.30791132282685,-32.0620661754796,
17.564801953498));
#32711=CARTESIAN_POINT('Ctrl Pts',(-8.40358858683736,-32.009374805817,17.5709153478751));
#32712=CARTESIAN_POINT('Ctrl Pts',(-8.4428155412199,-31.9887636050222,17.5734289693904));
#32713=CARTESIAN_POINT('Ctrl Pts',(-8.49991066293199,-31.9601777889932,
17.577113822043));
#32714=CARTESIAN_POINT('Ctrl Pts',(-8.51746301095371,-31.9515789119634,
17.5782501433891));
#32715=CARTESIAN_POINT('Ctrl Pts',(-8.54837976707107,-31.9367629871929,
17.5802594855762));
#32716=CARTESIAN_POINT('Ctrl Pts',(-8.56171186708872,-31.9304805704015,
17.5811285728894));
#32717=CARTESIAN_POINT('Ctrl Pts',(-8.59145379517805,-31.9167017493821,
17.5830733786653));
#32718=CARTESIAN_POINT('Ctrl Pts',(-8.60788263331463,-31.9092493276539,
17.584151532289));
#32719=CARTESIAN_POINT('Ctrl Pts',(-8.65695942033241,-31.8874578635176,
17.5873820370072));
#32720=CARTESIAN_POINT('Ctrl Pts',(-8.68977401939683,-31.8735028845947,
17.5895548905233));
#32721=CARTESIAN_POINT('Ctrl Pts',(-8.88703087619828,-31.7932666623742,
17.6026667935407));
#32722=CARTESIAN_POINT('Ctrl Pts',(-9.05623637117996,-31.7394571049311,
17.6141062712943));
#32723=CARTESIAN_POINT('Ctrl Pts',(-9.38864232342969,-31.6618012127062,
17.6361100763141));
#32724=CARTESIAN_POINT('Ctrl Pts',(-9.55093775625886,-31.6361212093345,
17.6466475337112));
#32725=CARTESIAN_POINT('Ctrl Pts',(-9.81202945562476,-31.6140497751506,
17.6630089955334));
#32726=CARTESIAN_POINT('Ctrl Pts',(-9.90991152828183,-31.6100326312856,
17.669015680292));
#32727=CARTESIAN_POINT('Ctrl Pts',(-10.0454778836812,-31.6103460946026,
17.677155675251));
#32728=CARTESIAN_POINT('Ctrl Pts',(-10.0831148528553,-31.6110600582777,
17.6793967067006));
#32729=CARTESIAN_POINT('Ctrl Pts',(-10.1478084975021,-31.613365725654,17.6832177877439));
#32730=CARTESIAN_POINT('Ctrl Pts',(-10.1748717170049,-31.6146552603872,
17.6848069267013));
#32731=CARTESIAN_POINT('Ctrl Pts',(-10.2302215503355,-31.6179581476324,
17.6880389357425));
#32732=CARTESIAN_POINT('Ctrl Pts',(-10.2585042251357,-31.620002264818,17.6896807312807));
#32733=CARTESIAN_POINT('Ctrl Pts',(-10.3308235983518,-31.6261421884174,
17.6938558611301));
#32734=CARTESIAN_POINT('Ctrl Pts',(-10.3748125349363,-31.6307453935645,
17.6963735194634));
#32735=CARTESIAN_POINT('Ctrl Pts',(-10.5787240470861,-31.6561268122918,
17.7079589752589));
#32736=CARTESIAN_POINT('Ctrl Pts',(-10.7371303936744,-31.6874396847406,
17.7167017768494));
#32737=CARTESIAN_POINT('Ctrl Pts',(-11.080734111676,-31.7812420173593,17.7357197583529));
#32738=CARTESIAN_POINT('Ctrl Pts',(-11.2639619996605,-31.8486856309957,
17.7458951436701));
#32739=CARTESIAN_POINT('Ctrl Pts',(-11.5182586887286,-31.9680536253725,
17.7611965963785));
#32740=CARTESIAN_POINT('Ctrl Pts',(-11.5947203668731,-32.007564046601,17.7659666375772));
#32741=CARTESIAN_POINT('Ctrl Pts',(-11.6912088833232,-32.0621717811038,
17.7723107866141));
#32742=CARTESIAN_POINT('Ctrl Pts',(-11.7126918010815,-32.0746438082891,
17.7737447764485));
#32743=CARTESIAN_POINT('Ctrl Pts',(-11.7476204917344,-32.0954384735782,
17.7761148612058));
#32744=CARTESIAN_POINT('Ctrl Pts',(-11.7611489165214,-32.1036213098265,
17.7770424477029));
#32745=CARTESIAN_POINT('Ctrl Pts',(-11.7882289210827,-32.1202608552763,
17.7789196386815));
#32746=CARTESIAN_POINT('Ctrl Pts',(-11.8017789396394,-32.128719302198,17.7798693394958));
#32747=CARTESIAN_POINT('Ctrl Pts',(-11.8369774714619,-32.1510388532362,
17.7823625913552));
#32748=CARTESIAN_POINT('Ctrl Pts',(-11.8585285872754,-32.1650507500312,
17.7839153010184));
#32749=CARTESIAN_POINT('Ctrl Pts',(-11.9529827620085,-32.2280019438361,
17.7908296431376));
#32750=CARTESIAN_POINT('Ctrl Pts',(-12.024122872019,-32.2795149174791,17.7963271991821));
#32751=CARTESIAN_POINT('Ctrl Pts',(-12.264603946402,-32.4683063331739,17.8157385601154));
#32752=CARTESIAN_POINT('Ctrl Pts',(-12.4226538947103,-32.619105570469,17.8299665660269));
#32753=CARTESIAN_POINT('Ctrl Pts',(-12.6570594593548,-32.8904474021813,
17.8527151022909));
#32754=CARTESIAN_POINT('Ctrl Pts',(-12.7422797865341,-33.0024798730737,
17.8614577830914));
#32755=CARTESIAN_POINT('Ctrl Pts',(-12.8435903142834,-33.1544211308715,
17.8724712358748));
#32756=CARTESIAN_POINT('Ctrl Pts',(-12.8662282162011,-33.1897781109792,
17.874979389166));
#32757=CARTESIAN_POINT('Ctrl Pts',(-12.9027949185996,-33.2492962550207,
17.8791132148106));
#32758=CARTESIAN_POINT('Ctrl Pts',(-12.9170923761371,-33.2732243688142,
17.8807520415042));
#32759=CARTESIAN_POINT('Ctrl Pts',(-12.9446665028586,-33.3206922763181,
17.8839589219604));
#32760=CARTESIAN_POINT('Ctrl Pts',(-12.9579599999856,-33.3442198382113,
17.8855274906737));
#32761=CARTESIAN_POINT('Ctrl Pts',(-12.9867520348804,-33.3966311670291,
17.8889770496842));
#32762=CARTESIAN_POINT('Ctrl Pts',(-13.0021159329327,-33.4255860253796,
17.8908532632633));
#32763=CARTESIAN_POINT('Ctrl Pts',(-13.054485713031,-33.5278372263349,17.8973810303638));
#32764=CARTESIAN_POINT('Ctrl Pts',(-13.0892479075963,-33.6022536010355,
17.9019570521331));
#32765=CARTESIAN_POINT('Ctrl Pts',(-13.1415533580126,-33.7257353107587,
17.9093181297542));
#32766=CARTESIAN_POINT('Ctrl Pts',(-13.1607152904065,-33.7740389631084,
17.9121418218122));
#32767=CARTESIAN_POINT('Ctrl Pts',(-13.1787500647504,-33.822734911607,17.9149431671188));
#32768=CARTESIAN_POINT('Origin',(-10.,-35.,23.));
#32769=CARTESIAN_POINT('',(-13.1787501240201,-33.8227350716418,19.1603160842799));
#32770=CARTESIAN_POINT('',(-13.1787501466517,-33.8227351327498,18.8205587414464));
#32771=CARTESIAN_POINT('',(-13.1787501240207,-33.8227350716434,23.));
#32772=CARTESIAN_POINT('',(-13.3897489495918,-34.9973314346088,17.6410178032058));
#32773=CARTESIAN_POINT('Ctrl Pts',(-13.1787501466517,-33.8227351327498,
18.8205587414464));
#32774=CARTESIAN_POINT('Ctrl Pts',(-13.1278271796848,-33.6852372822515,
18.8127838077241));
#32775=CARTESIAN_POINT('Ctrl Pts',(-13.0680253938338,-33.5511580716046,
18.8050413658075));
#32776=CARTESIAN_POINT('Ctrl Pts',(-12.9630852026426,-33.351753700127,18.7927313675143));
#32777=CARTESIAN_POINT('Ctrl Pts',(-12.9240518693691,-33.2834602661968,
18.7883601853884));
#32778=CARTESIAN_POINT('Ctrl Pts',(-12.8696313405074,-33.1954955301696,
18.7824417043482));
#32779=CARTESIAN_POINT('Ctrl Pts',(-12.856349561064,-33.1745445718325,18.7810097829634));
#32780=CARTESIAN_POINT('Ctrl Pts',(-12.8350989407793,-33.1418231972354,
18.778735021485));
#32781=CARTESIAN_POINT('Ctrl Pts',(-12.8272836961893,-33.129953498025,18.777901784375));
#32782=CARTESIAN_POINT('Ctrl Pts',(-12.8107581297681,-33.1051950537516,
18.7761460391324));
#32783=CARTESIAN_POINT('Ctrl Pts',(-12.8020333898203,-33.0923166144302,
18.7752225204624));
#32784=CARTESIAN_POINT('Ctrl Pts',(-12.7797669685693,-33.0599318206986,
18.7728750921918));
#32785=CARTESIAN_POINT('Ctrl Pts',(-12.7661085176199,-33.0405070709123,
18.7714438298795));
#32786=CARTESIAN_POINT('Ctrl Pts',(-12.7084889622472,-32.9603647996441,
18.7654467896085));
#32787=CARTESIAN_POINT('Ctrl Pts',(-12.6627265461189,-32.9009740531532,
18.7607807708712));
#32788=CARTESIAN_POINT('Ctrl Pts',(-12.5210053560613,-32.7291462777544,
18.7467189387252));
#32789=CARTESIAN_POINT('Ctrl Pts',(-12.4196220096114,-32.6214139919694,
18.7371537613859));
#32790=CARTESIAN_POINT('Ctrl Pts',(-12.161386459057,-32.3806575304665,18.7144213291779));
#32791=CARTESIAN_POINT('Ctrl Pts',(-11.9988122774959,-32.2545824963507,
18.7013678505348));
#32792=CARTESIAN_POINT('Ctrl Pts',(-11.7811823494712,-32.1154550106523,
18.6856404447628));
#32793=CARTESIAN_POINT('Ctrl Pts',(-11.7358926817733,-32.0879753730936,
18.6824518638282));
#32794=CARTESIAN_POINT('Ctrl Pts',(-11.663607711314,-32.0464022467577,18.6774915253318));
#32795=CARTESIAN_POINT('Ctrl Pts',(-11.637036245979,-32.0315925608539,18.675694715312));
#32796=CARTESIAN_POINT('Ctrl Pts',(-11.5869891390892,-32.0045750904019,
18.6723586935983));
#32797=CARTESIAN_POINT('Ctrl Pts',(-11.5635631207946,-31.9922807075084,
18.6708165433615));
#32798=CARTESIAN_POINT('Ctrl Pts',(-11.5105247638211,-31.9652324017662,
18.6673671587087));
#32799=CARTESIAN_POINT('Ctrl Pts',(-11.4808353161526,-31.9506350965688,
18.6654654149995));
#32800=CARTESIAN_POINT('Ctrl Pts',(-11.3890990613947,-31.9071872962696,
18.6596740261626));
#32801=CARTESIAN_POINT('Ctrl Pts',(-11.3263868349768,-31.8797779793758,
18.6558326136647));
#32802=CARTESIAN_POINT('Ctrl Pts',(-11.1754896755044,-31.8191985269537,
18.6468276740873));
#32803=CARTESIAN_POINT('Ctrl Pts',(-11.0866668015975,-31.7877685571224,
18.6417153030131));
#32804=CARTESIAN_POINT('Ctrl Pts',(-10.7881320092118,-31.6959350202277,
18.6249532813954));
#32805=CARTESIAN_POINT('Ctrl Pts',(-10.5739249964252,-31.6520753753334,
18.613625428358));
#32806=CARTESIAN_POINT('Ctrl Pts',(-10.26961590203,-31.6198470445316,18.5969872147209));
#32807=CARTESIAN_POINT('Ctrl Pts',(-10.1819112909128,-31.6139945922539,
18.5921246758359));
#32808=CARTESIAN_POINT('Ctrl Pts',(-10.0684446739674,-31.6108440048291,
18.5856377460135));
#32809=CARTESIAN_POINT('Ctrl Pts',(-10.0427971848497,-31.6104231311858,
18.5841585211107));
#32810=CARTESIAN_POINT('Ctrl Pts',(-10.001196762476,-31.6102126783775,18.5817347061495));
#32811=CARTESIAN_POINT('Ctrl Pts',(-9.98524528787591,-31.6102445820032,
18.5807994637303));
#32812=CARTESIAN_POINT('Ctrl Pts',(-9.95354951481549,-31.6105317002119,
18.5789284808173));
#32813=CARTESIAN_POINT('Ctrl Pts',(-9.93780564695028,-31.6107840377502,
18.5779929044681));
#32814=CARTESIAN_POINT('Ctrl Pts',(-9.8973398152633,-31.6117146543137,18.575573209462));
#32815=CARTESIAN_POINT('Ctrl Pts',(-9.87262284234043,-31.6125538116422,
18.5740808191472));
#32816=CARTESIAN_POINT('Ctrl Pts',(-9.7625826134207,-31.6174957686995,18.56737896883));
#32817=CARTESIAN_POINT('Ctrl Pts',(-9.67742886540143,-31.6245522551736,
18.5620387286689));
#32818=CARTESIAN_POINT('Ctrl Pts',(-9.40238391878068,-31.6578468389858,
18.5444696605795));
#32819=CARTESIAN_POINT('Ctrl Pts',(-9.21442544796143,-31.696970124836,18.5319858923283));
#32820=CARTESIAN_POINT('Ctrl Pts',(-8.87115991819229,-31.7993950796104,
18.5090954006666));
#32821=CARTESIAN_POINT('Ctrl Pts',(-8.71525221256635,-31.8587283404383,
18.4986581401984));
#32822=CARTESIAN_POINT('Ctrl Pts',(-8.52413059969507,-31.9480853491866,
18.4859064923559));
#32823=CARTESIAN_POINT('Ctrl Pts',(-8.48431059322875,-31.9676643614449,
18.4832510396663));
#32824=CARTESIAN_POINT('Ctrl Pts',(-8.41970955662775,-32.0010185171241,
18.4789434730602));
#32825=CARTESIAN_POINT('Ctrl Pts',(-8.39469755452233,-32.0143322436214,
18.4772757746419));
#32826=CARTESIAN_POINT('Ctrl Pts',(-8.34619330226916,-32.0409365044549,
18.4740408938562));
#32827=CARTESIAN_POINT('Ctrl Pts',(-8.32268711817533,-32.0541970666111,
18.4724728198936));
#32828=CARTESIAN_POINT('Ctrl Pts',(-8.26703283162491,-32.0864755335199,
18.4687578621645));
#32829=CARTESIAN_POINT('Ctrl Pts',(-8.23503541868252,-32.1057470382195,
18.4666201622408));
#32830=CARTESIAN_POINT('Ctrl Pts',(-8.12182354356072,-32.1765085121722,
18.4590427891796));
#32831=CARTESIAN_POINT('Ctrl Pts',(-8.04248633201922,-32.2309219177966,
18.4537082799207));
#32832=CARTESIAN_POINT('Ctrl Pts',(-7.83825290124936,-32.3841658422554,
18.4397773625463));
#32833=CARTESIAN_POINT('Ctrl Pts',(-7.71782266634565,-32.4885445099542,
18.4313585204422));
#32834=CARTESIAN_POINT('Ctrl Pts',(-7.4742422944954,-32.7317015465711,18.4131103908508));
#32835=CARTESIAN_POINT('Ctrl Pts',(-7.35424700723463,-32.87288774716,18.4033037390942));
#32836=CARTESIAN_POINT('Ctrl Pts',(-7.22611945710972,-33.0513597652028,
18.3908923618807));
#32837=CARTESIAN_POINT('Ctrl Pts',(-7.20629453394378,-33.0798902103678,
18.388907466408));
#32838=CARTESIAN_POINT('Ctrl Pts',(-7.17683217255581,-33.1237124707789,
18.3858493179413));
#32839=CARTESIAN_POINT('Ctrl Pts',(-7.166872199568,-33.1387857971824,18.3847957682614));
#32840=CARTESIAN_POINT('Ctrl Pts',(-7.14890008985113,-33.1664631434829,
18.3828568725705));
#32841=CARTESIAN_POINT('Ctrl Pts',(-7.14085007775999,-33.1790415167915,
18.3819739705732));
#32842=CARTESIAN_POINT('Ctrl Pts',(-7.12235598055536,-33.2083640464982,
18.3799118918268));
#32843=CARTESIAN_POINT('Ctrl Pts',(-7.11197474349381,-33.225146606345,18.3787289008106));
#32844=CARTESIAN_POINT('Ctrl Pts',(-7.07842552556662,-33.2804568130526,
18.3748235298702));
#32845=CARTESIAN_POINT('Ctrl Pts',(-7.05587829782229,-33.3193533471446,
18.372066755563));
#32846=CARTESIAN_POINT('Ctrl Pts',(-7.00207386331143,-33.4165789693409,
18.3651716934198));
#32847=CARTESIAN_POINT('Ctrl Pts',(-6.97173886628657,-33.4753961479894,
18.3609969811496));
#32848=CARTESIAN_POINT('Ctrl Pts',(-6.82654717612096,-33.7783640672862,
18.3396011187023));
#32849=CARTESIAN_POINT('Ctrl Pts',(-6.73939664834711,-34.0347579820041,
18.3219444666333));
#32850=CARTESIAN_POINT('Ctrl Pts',(-6.66497278660186,-34.3867439103519,
18.2995451818813));
#32851=CARTESIAN_POINT('Ctrl Pts',(-6.64987894258677,-34.4754233464817,
18.2940398668148));
#32852=CARTESIAN_POINT('Ctrl Pts',(-6.63352859880435,-34.601663725078,18.286398292647));
#32853=CARTESIAN_POINT('Ctrl Pts',(-6.62934178848976,-34.6388007865018,
18.2841738239773));
#32854=CARTESIAN_POINT('Ctrl Pts',(-6.62318771767488,-34.7028911956753,
18.2803738919918));
#32855=CARTESIAN_POINT('Ctrl Pts',(-6.62092713086152,-34.7298122142041,
18.2787895410305));
#32856=CARTESIAN_POINT('Ctrl Pts',(-6.61695247586294,-34.785059057254,18.2755613450546));
#32857=CARTESIAN_POINT('Ctrl Pts',(-6.61527177715232,-34.8133851881557,
18.273918648314));
#32858=CARTESIAN_POINT('Ctrl Pts',(-6.61187090757798,-34.8861437963664,
18.2697293008994));
#32859=CARTESIAN_POINT('Ctrl Pts',(-6.61066890199132,-34.9305957643352,
18.2671986266567));
#32860=CARTESIAN_POINT('Ctrl Pts',(-6.6089920360372,-35.1585030551804,18.2543525370803));
#32861=CARTESIAN_POINT('Ctrl Pts',(-6.62253531671405,-35.3417609369562,
18.2444724383207));
#32862=CARTESIAN_POINT('Ctrl Pts',(-6.6795570276113,-35.7068858323845,18.2248183471407));
#32863=CARTESIAN_POINT('Ctrl Pts',(-6.72335585861298,-35.8880452831363,
18.215077091432));
#32864=CARTESIAN_POINT('Ctrl Pts',(-6.8051404964262,-36.1352546474058,18.2008170043095));
#32865=CARTESIAN_POINT('Ctrl Pts',(-6.83080086226466,-36.2050334632,18.1966764071039));
#32866=CARTESIAN_POINT('Ctrl Pts',(-6.86789828736187,-36.296510253193,18.191024706514));
#32867=CARTESIAN_POINT('Ctrl Pts',(-6.87730805220173,-36.3190128509112,
18.1896160472342));
#32868=CARTESIAN_POINT('Ctrl Pts',(-6.89255644117843,-36.354400098528,18.1873687046291));
#32869=CARTESIAN_POINT('Ctrl Pts',(-6.89823447317542,-36.3673535383788,
18.1865392029941));
#32870=CARTESIAN_POINT('Ctrl Pts',(-6.9103819001591,-36.394600738888,18.1847790829892));
#32871=CARTESIAN_POINT('Ctrl Pts',(-6.91686974382693,-36.4088857369226,
18.1838473230294));
#32872=CARTESIAN_POINT('Ctrl Pts',(-6.93364271801762,-36.4451459355761,
18.1814602314316));
#32873=CARTESIAN_POINT('Ctrl Pts',(-6.94406492355331,-36.4670564034257,
18.1799971218698));
#32874=CARTESIAN_POINT('Ctrl Pts',(-6.98974975120966,-36.560499542065,18.1736740466874));
#32875=CARTESIAN_POINT('Ctrl Pts',(-7.0272934993271,-36.6308830568857,18.1687008904929));
#32876=CARTESIAN_POINT('Ctrl Pts',(-7.15070409073578,-36.8437983042673,
18.1531361019726));
#32877=CARTESIAN_POINT('Ctrl Pts',(-7.24460716391243,-36.9813853731174,
18.1423405209087));
#32878=CARTESIAN_POINT('Ctrl Pts',(-7.45995554359306,-37.2518324796645,
18.120148132963));
#32879=CARTESIAN_POINT('Ctrl Pts',(-7.58265348968885,-37.3830706828012,
18.1088100265218));
#32880=CARTESIAN_POINT('Ctrl Pts',(-7.75439721099543,-37.5397819128541,
18.0946538037738));
#32881=CARTESIAN_POINT('Ctrl Pts',(-7.79445456941998,-37.5746444180604,
18.0914574223302));
#32882=CARTESIAN_POINT('Ctrl Pts',(-7.85876832258284,-37.6280145971421,
18.0864859461972));
#32883=CARTESIAN_POINT('Ctrl Pts',(-7.88248242294936,-37.6471594626543,
18.0846857165856));
#32884=CARTESIAN_POINT('Ctrl Pts',(-7.92729346366907,-37.6823487651706,
18.0813436725575));
#32885=CARTESIAN_POINT('Ctrl Pts',(-7.94832646812252,-37.6984705040206,
18.0797989098084));
#32886=CARTESIAN_POINT('Ctrl Pts',(-7.99607813897189,-37.7341909293101,
18.0763439285654));
#32887=CARTESIAN_POINT('Ctrl Pts',(-8.02289966232174,-37.7536479855994,
18.0744392084099));
#32888=CARTESIAN_POINT('Ctrl Pts',(-8.10605431856967,-37.8121291796384,
18.0686389853354));
#32889=CARTESIAN_POINT('Ctrl Pts',(-8.16329055996146,-37.8498421139435,
18.0647918084539));
#32890=CARTESIAN_POINT('Ctrl Pts',(-8.301926517572,-37.9352762695603,18.0557735704154));
#32891=CARTESIAN_POINT('Ctrl Pts',(-8.38425282610886,-37.9813860867071,
18.0506537823879));
#32892=CARTESIAN_POINT('Ctrl Pts',(-8.6635497587908,-38.1228447160072,18.0338528189895));
#32893=CARTESIAN_POINT('Ctrl Pts',(-8.86779853617199,-38.2025567598758,
18.022495284381));
#32894=CARTESIAN_POINT('Ctrl Pts',(-9.16245346482691,-38.2858133747848,
18.0058434992633));
#32895=CARTESIAN_POINT('Ctrl Pts',(-9.24749747447466,-38.3063259537656,
18.0010028974775));
#32896=CARTESIAN_POINT('Ctrl Pts',(-9.35832415173827,-38.32856006576,17.9945425827067));
#32897=CARTESIAN_POINT('Ctrl Pts',(-9.38347143557366,-38.3333095342386,
17.9930666638767));
#32898=CARTESIAN_POINT('Ctrl Pts',(-9.4243652360559,-38.3405544116143,17.9906468381062));
#32899=CARTESIAN_POINT('Ctrl Pts',(-9.44008027195994,-38.3432243469305,
17.9897122181947));
#32900=CARTESIAN_POINT('Ctrl Pts',(-9.47126875699553,-38.3482971087787,
17.9878469954287));
#32901=CARTESIAN_POINT('Ctrl Pts',(-9.48674103188765,-38.350703725545,17.9869165919148));
#32902=CARTESIAN_POINT('Ctrl Pts',(-9.52655937792873,-38.3566149698747,
17.984510053648));
#32903=CARTESIAN_POINT('Ctrl Pts',(-9.5509276317461,-38.3599619059399,17.9830256788122));
#32904=CARTESIAN_POINT('Ctrl Pts',(-9.65953938558319,-38.3736769313171,
17.976364511486));
#32905=CARTESIAN_POINT('Ctrl Pts',(-9.74411280584278,-38.3811431427272,
17.9710575386435));
#32906=CARTESIAN_POINT('Ctrl Pts',(-10.0176372067226,-38.3949695261054,
17.9536853377977));
#32907=CARTESIAN_POINT('Ctrl Pts',(-10.2068697736873,-38.3887069160527,
17.9413671592005));
#32908=CARTESIAN_POINT('Ctrl Pts',(-10.564789248577,-38.3467569961094,17.9183047714037));
#32909=CARTESIAN_POINT('Ctrl Pts',(-10.7332443929623,-38.3139305723157,
17.9075520350472));
#32910=CARTESIAN_POINT('Ctrl Pts',(-10.941327119456,-38.2567283914272,17.8945066813705));
#32911=CARTESIAN_POINT('Ctrl Pts',(-10.9839064843871,-38.2441185048608,
17.8918488944142));
#32912=CARTESIAN_POINT('Ctrl Pts',(-11.0531433294776,-38.2221253479804,
17.8875445302911));
#32913=CARTESIAN_POINT('Ctrl Pts',(-11.0799519537448,-38.2132392504568,
17.8858821730731));
#32914=CARTESIAN_POINT('Ctrl Pts',(-11.1319910531298,-38.1952652886215,
17.8826627483972));
#32915=CARTESIAN_POINT('Ctrl Pts',(-11.1572308448781,-38.1862110478725,
17.8811047254976));
#32916=CARTESIAN_POINT('Ctrl Pts',(-11.2169974784316,-38.1639671388135,
17.8774222671109));
#32917=CARTESIAN_POINT('Ctrl Pts',(-11.2514216383299,-38.1505102687802,
17.8753067864029));
#32918=CARTESIAN_POINT('Ctrl Pts',(-11.37266383406,-38.1008141957698,17.8678688735315));
#32919=CARTESIAN_POINT('Ctrl Pts',(-11.4581892171857,-38.0615259219255,
17.862647119791));
#32920=CARTESIAN_POINT('Ctrl Pts',(-11.6786908915289,-37.948893036407,17.8491294299995));
#32921=CARTESIAN_POINT('Ctrl Pts',(-11.8105097499169,-37.8698485908608,
17.8409977537255));
#32922=CARTESIAN_POINT('Ctrl Pts',(-12.0954276728645,-37.6715302788106,
17.8226034464986));
#32923=CARTESIAN_POINT('Ctrl Pts',(-12.2445504355825,-37.5475219854541,
17.8123746483425));
#32924=CARTESIAN_POINT('Ctrl Pts',(-12.4071665466224,-37.3868766637562,
17.7994609296924));
#32925=CARTESIAN_POINT('Ctrl Pts',(-12.4316913777557,-37.3618864987385,
17.7974601089233));
#32926=CARTESIAN_POINT('Ctrl Pts',(-12.468134756586,-37.3235823382524,17.7943969570222));
#32927=CARTESIAN_POINT('Ctrl Pts',(-12.4803430552487,-37.3105459001232,
17.7933550618218));
#32928=CARTESIAN_POINT('Ctrl Pts',(-12.5025788884134,-37.2864224081972,
17.7914268454443));
#32929=CARTESIAN_POINT('Ctrl Pts',(-12.5126369302576,-37.2753646186839,
17.7905427873545));
#32930=CARTESIAN_POINT('Ctrl Pts',(-12.5359491360268,-37.2493921740165,
17.7884661795447));
#32931=CARTESIAN_POINT('Ctrl Pts',(-12.5491451686072,-37.2344265572653,
17.7872696071724));
#32932=CARTESIAN_POINT('Ctrl Pts',(-12.5923860692065,-37.1845054573929,
17.7832806932646));
#32933=CARTESIAN_POINT('Ctrl Pts',(-12.6218488895095,-37.1490550445159,
17.7804521145876));
#32934=CARTESIAN_POINT('Ctrl Pts',(-12.693263742535,-37.0594719215604,17.7733368634722));
#32935=CARTESIAN_POINT('Ctrl Pts',(-12.7343149033388,-37.0046484076015,
17.7690110799991));
#32936=CARTESIAN_POINT('Ctrl Pts',(-12.924817613039,-36.7334862321096,17.7478820424465));
#32937=CARTESIAN_POINT('Ctrl Pts',(-13.0504372340232,-36.5014631297012,
17.7306880273113));
#32938=CARTESIAN_POINT('Ctrl Pts',(-13.1824802009045,-36.1708462768496,
17.7084873475608));
#32939=CARTESIAN_POINT('Ctrl Pts',(-13.2134182675029,-36.0830543445701,
17.7027833940108));
#32940=CARTESIAN_POINT('Ctrl Pts',(-13.2518542173537,-35.9577546765959,
17.6949101000677));
#32941=CARTESIAN_POINT('Ctrl Pts',(-13.2623896988519,-35.9212293417552,
17.6926460526183));
#32942=CARTESIAN_POINT('Ctrl Pts',(-13.2793418861227,-35.8585151524786,
17.6888099965516));
#32943=CARTESIAN_POINT('Ctrl Pts',(-13.2860644253252,-35.8324134357044,
17.6872284409606));
#32944=CARTESIAN_POINT('Ctrl Pts',(-13.2992080677314,-35.7787377920279,
17.6840058317488));
#32945=CARTESIAN_POINT('Ctrl Pts',(-13.305596490129,-35.7511579978445,17.6823659162278));
#32946=CARTESIAN_POINT('Ctrl Pts',(-13.3177838770018,-35.6953733685506,
17.6790795065311));
#32947=CARTESIAN_POINT('Ctrl Pts',(-13.3235704614071,-35.6671682210812,
17.6774335128797));
#32948=CARTESIAN_POINT('Ctrl Pts',(-13.3368339124911,-35.5980579803883,
17.6734362028842));
#32949=CARTESIAN_POINT('Ctrl Pts',(-13.3439189242645,-35.5570819803451,
17.6710966870807));
#32950=CARTESIAN_POINT('Ctrl Pts',(-13.3766779417949,-35.344380267151,17.6590918149364));
#32951=CARTESIAN_POINT('Ctrl Pts',(-13.3898844254065,-35.1709939538293,
17.6497907008939));
#32952=CARTESIAN_POINT('Ctrl Pts',(-13.3897489685498,-34.9973556256544,
17.6405626171251));
#32953=CARTESIAN_POINT('Ctrl Pts',(-13.3897489495918,-34.9973314346088,
17.6410178032058));
#32954=CARTESIAN_POINT('Ctrl Pts',(-13.3896451068354,-34.8654250268716,
17.6332792606915));
#32955=CARTESIAN_POINT('Ctrl Pts',(-13.381838229504,-34.7338444491851,17.6255407181773));
#32956=CARTESIAN_POINT('Ctrl Pts',(-13.3664638492093,-34.6033563129622,
17.617802175663));
#32957=CARTESIAN_POINT('Ctrl Pts',(-13.3507856217542,-34.4702893118427,
17.6099106946808));
#32958=CARTESIAN_POINT('Ctrl Pts',(-13.3272378167578,-34.338358106954,17.6020192136986));
#32959=CARTESIAN_POINT('Ctrl Pts',(-13.2960126784577,-34.2083526757789,
17.5941277327164));
#32960=CARTESIAN_POINT('Ctrl Pts',(-13.2922017700226,-34.1924860112503,
17.5931646077127));
#32961=CARTESIAN_POINT('Ctrl Pts',(-13.2882765642279,-34.1766480068593,
17.5922014827091));
#32962=CARTESIAN_POINT('Ctrl Pts',(-13.2842374593052,-34.1608400787715,
17.5912383577054));
#32963=CARTESIAN_POINT('Ctrl Pts',(-13.258626776551,-34.0606070224349,17.5851314876452));
#32964=CARTESIAN_POINT('Ctrl Pts',(-13.2283809689128,-33.9613816652927,
17.579024617585));
#32965=CARTESIAN_POINT('Ctrl Pts',(-13.1935957197208,-33.8636235476387,
17.5729177475248));
#32966=CARTESIAN_POINT('Ctrl Pts',(-13.1887356065883,-33.8499650135632,
17.5720645100156));
#32967=CARTESIAN_POINT('Ctrl Pts',(-13.1837869610759,-33.8363351084987,
17.5712112725064));
#32968=CARTESIAN_POINT('Ctrl Pts',(-13.1787501240207,-33.8227350716434,
17.5703580349972));
#32969=CARTESIAN_POINT('Ctrl Pts',(-13.1787500647504,-33.822734911607,17.9149431671188));
#32970=CARTESIAN_POINT('Ctrl Pts',(-13.2574736629433,-34.0352976090998,
17.9271713202471));
#32971=CARTESIAN_POINT('Ctrl Pts',(-13.3147214038581,-34.2553371507137,
17.9389318292027));
#32972=CARTESIAN_POINT('Ctrl Pts',(-13.3598256104917,-34.54563607905,17.9548343611894));
#32973=CARTESIAN_POINT('Ctrl Pts',(-13.3681327220865,-34.6119848253376,
17.9584977817604));
#32974=CARTESIAN_POINT('Ctrl Pts',(-13.3787671453846,-34.7236151964397,
17.9647713098526));
#32975=CARTESIAN_POINT('Ctrl Pts',(-13.3821578507305,-34.7687774939372,
17.9673394228452));
#32976=CARTESIAN_POINT('Ctrl Pts',(-13.3857286033999,-34.8337516451611,
17.9710941787719));
#32977=CARTESIAN_POINT('Ctrl Pts',(-13.3866414449915,-34.8535200578378,
17.9722445405624));
#32978=CARTESIAN_POINT('Ctrl Pts',(-13.3879395062227,-34.8882228830459,
17.9742796982406));
#32979=CARTESIAN_POINT('Ctrl Pts',(-13.3883991777765,-34.9031536159209,
17.9751604929724));
#32980=CARTESIAN_POINT('Ctrl Pts',(-13.3891957335569,-34.9361074688981,
17.9771163142488));
#32981=CARTESIAN_POINT('Ctrl Pts',(-13.389487559345,-34.9541303058339,17.9781936029256));
#32982=CARTESIAN_POINT('Ctrl Pts',(-13.3899283133611,-35.0077826861086,
17.9814215909546));
#32983=CARTESIAN_POINT('Ctrl Pts',(-13.3896592322845,-35.043412119444,17.9835927777448));
#32984=CARTESIAN_POINT('Ctrl Pts',(-13.384777880587,-35.252728184127,17.9964846924534));
#32985=CARTESIAN_POINT('Ctrl Pts',(-13.3673786748111,-35.4258458803741,
18.0076865605367));
#32986=CARTESIAN_POINT('Ctrl Pts',(-13.307491412664,-35.7606544881738,18.0296124871599));
#32987=CARTESIAN_POINT('Ctrl Pts',(-13.2661681023012,-35.9220894308829,
18.0403063602688));
#32988=CARTESIAN_POINT('Ctrl Pts',(-13.1817368252688,-36.173320122958,18.0568624955752));
#32989=CARTESIAN_POINT('Ctrl Pts',(-13.1462568947524,-36.2653852359981,
18.0629138888606));
#32990=CARTESIAN_POINT('Ctrl Pts',(-13.0917431188089,-36.3903052130589,
18.0710985399781));
#32991=CARTESIAN_POINT('Ctrl Pts',(-13.0761015147676,-36.4245784432275,
18.0733415370835));
#32992=CARTESIAN_POINT('Ctrl Pts',(-13.0482555855393,-36.4829950076799,
18.0771615828884));
#32993=CARTESIAN_POINT('Ctrl Pts',(-13.0363278852742,-36.5072655186889,
18.0787478132954));
#32994=CARTESIAN_POINT('Ctrl Pts',(-13.0113552853821,-36.5565800938483,
18.0819699714671));
#32995=CARTESIAN_POINT('Ctrl Pts',(-12.9982853213871,-36.581609131581,18.0836048782435));
#32996=CARTESIAN_POINT('Ctrl Pts',(-12.9641062008404,-36.6451155957622,
18.0877537861169));
#32997=CARTESIAN_POINT('Ctrl Pts',(-12.9425594472246,-36.6833523224569,
18.0902523715505));
#32998=CARTESIAN_POINT('Ctrl Pts',(-12.8419742782966,-36.8540140932111,
18.1014226665075));
#32999=CARTESIAN_POINT('Ctrl Pts',(-12.7546946868513,-36.9813758409625,
18.1097989087319));
#33000=CARTESIAN_POINT('Ctrl Pts',(-12.6379670212617,-37.1290113202829,
18.1198578482986));
#33001=CARTESIAN_POINT('Ctrl Pts',(-12.6164971619536,-37.1553426282019,
18.1216670540787));
#33002=CARTESIAN_POINT('Ctrl Pts',(-12.4712559637912,-37.3281018902216,
18.1336623432424));
#33003=CARTESIAN_POINT('Ctrl Pts',(-12.335657144121,-37.4641145648641,18.143694985248));
#33004=CARTESIAN_POINT('Ctrl Pts',(-12.1380088740832,-37.6313184438488,
18.1579324884406));
#33005=CARTESIAN_POINT('Ctrl Pts',(-12.0854417220138,-37.6731723370791,
18.1616886154957));
#33006=CARTESIAN_POINT('Ctrl Pts',(-12.0128229667522,-37.7275452489114,
18.1668889927681));
#33007=CARTESIAN_POINT('Ctrl Pts',(-11.9938305113286,-37.7414593204963,
18.1682501142065));
#33008=CARTESIAN_POINT('Ctrl Pts',(-11.9633409847396,-37.7633118506042,
18.1704394914702));
#33009=CARTESIAN_POINT('Ctrl Pts',(-11.9519367615474,-37.7713792720609,
18.171259344059));
#33010=CARTESIAN_POINT('Ctrl Pts',(-11.9275144520872,-37.7884302522046,
18.1730178204206));
#33011=CARTESIAN_POINT('Ctrl Pts',(-11.9144827582823,-37.7973936047479,
18.1739577879707));
#33012=CARTESIAN_POINT('Ctrl Pts',(-11.8806732143477,-37.8203013107773,
18.176399679444));
#33013=CARTESIAN_POINT('Ctrl Pts',(-11.8598031859927,-37.8341071348051,
18.1779101307904));
#33014=CARTESIAN_POINT('Ctrl Pts',(-11.7642922454333,-37.8957797503511,
18.1848298470815));
#33015=CARTESIAN_POINT('Ctrl Pts',(-11.6879485776571,-37.9409343059859,
18.1903799206523));
#33016=CARTESIAN_POINT('Ctrl Pts',(-11.4265037944314,-38.0820345128476,
18.2092412651861));
#33017=CARTESIAN_POINT('Ctrl Pts',(-11.2343381561607,-38.1639000220664,
18.2228388566312));
#33018=CARTESIAN_POINT('Ctrl Pts',(-10.895315268362,-38.2727060105552,18.2454863242625));
#33019=CARTESIAN_POINT('Ctrl Pts',(-10.751956360791,-38.3085895427248,18.2546898537724));
#33020=CARTESIAN_POINT('Ctrl Pts',(-10.5638877520947,-38.3428025811365,
18.2662342924794));
#33021=CARTESIAN_POINT('Ctrl Pts',(-10.5209294173895,-38.3497658574244,
18.2688370541273));
#33022=CARTESIAN_POINT('Ctrl Pts',(-10.4499501385651,-38.3598726121073,
18.2730831189388));
#33023=CARTESIAN_POINT('Ctrl Pts',(-10.4220038630253,-38.3634969760628,
18.2747411051786));
#33024=CARTESIAN_POINT('Ctrl Pts',(-10.3670785386468,-38.3699249129996,
18.2779736614267));
#33025=CARTESIAN_POINT('Ctrl Pts',(-10.3401046693868,-38.3727539858738,
18.2795489050284));
#33026=CARTESIAN_POINT('Ctrl Pts',(-10.275258016893,-38.3787693559963,18.2833078970419));
#33027=CARTESIAN_POINT('Ctrl Pts',(-10.2373594976023,-38.3816430873576,
18.285481901486));
#33028=CARTESIAN_POINT('Ctrl Pts',(-10.0985283019247,-38.3898247199358,
18.2933699948383));
#33029=CARTESIAN_POINT('Ctrl Pts',(-9.99741648630631,-38.3912557102519,
18.2989667259291));
#33030=CARTESIAN_POINT('Ctrl Pts',(-9.63032288922031,-38.3800294606252,
18.3189619407942));
#33031=CARTESIAN_POINT('Ctrl Pts',(-9.36616538847495,-38.3405840724596,
18.332661166564));
#33032=CARTESIAN_POINT('Ctrl Pts',(-9.02426850672867,-38.2474804654496,
18.3519248469663));
#33033=CARTESIAN_POINT('Ctrl Pts',(-8.94012669182979,-38.2210010048482,
18.3568037818863));
#33034=CARTESIAN_POINT('Ctrl Pts',(-8.832912255196,-38.1826046598288,18.3633115135663));
#33035=CARTESIAN_POINT('Ctrl Pts',(-8.80880492608107,-38.1736604159552,
18.3647942356018));
#33036=CARTESIAN_POINT('Ctrl Pts',(-8.76989507419001,-38.1587184009094,
18.3672225731859));
#33037=CARTESIAN_POINT('Ctrl Pts',(-8.75502865536089,-38.1528885792252,
18.3681587857228));
#33038=CARTESIAN_POINT('Ctrl Pts',(-8.72558067395743,-38.1410998975053,
18.3700310598773));
#33039=CARTESIAN_POINT('Ctrl Pts',(-8.71099840431787,-38.1351440229613,
18.3709669474307));
#33040=CARTESIAN_POINT('Ctrl Pts',(-8.67364480995784,-38.1195829472141,
18.3733858808067));
#33041=CARTESIAN_POINT('Ctrl Pts',(-8.6509363965119,-38.1098300871039,18.3748771684393));
#33042=CARTESIAN_POINT('Ctrl Pts',(-8.5505332316712,-38.0654020824224,18.381556861461));
#33043=CARTESIAN_POINT('Ctrl Pts',(-8.47405861599768,-38.0280595242528,
18.3868748474453));
#33044=CARTESIAN_POINT('Ctrl Pts',(-8.23161809754652,-37.898158582785,18.4043133548527));
#33045=CARTESIAN_POINT('Ctrl Pts',(-8.07200105003478,-37.7945157955768,
18.4166851830328));
#33046=CARTESIAN_POINT('Ctrl Pts',(-7.7889267376143,-37.5748576077641,18.4395875901524));
#33047=CARTESIAN_POINT('Ctrl Pts',(-7.6638036435863,-37.4618969002117,18.4501384093483));
#33048=CARTESIAN_POINT('Ctrl Pts',(-7.51690801857805,-37.3079499707143,
18.4629997505395));
#33049=CARTESIAN_POINT('Ctrl Pts',(-7.48687169763568,-37.2752066438739,
18.4656588844473));
#33050=CARTESIAN_POINT('Ctrl Pts',(-7.43873051083282,-37.2206098095412,
18.4699716966451));
#33051=CARTESIAN_POINT('Ctrl Pts',(-7.42024165763747,-37.1991035197149,
18.4716409983953));
#33052=CARTESIAN_POINT('Ctrl Pts',(-7.3846780533992,-37.1566699912887,18.4748785611568));
#33053=CARTESIAN_POINT('Ctrl Pts',(-7.36757926060233,-37.1357657756271,
18.4764477199936));
#33054=CARTESIAN_POINT('Ctrl Pts',(-7.32742284928981,-37.0854573778795,
18.4801646435222));
#33055=CARTESIAN_POINT('Ctrl Pts',(-7.30459775569439,-37.055871591215,18.4823032285057));
#33056=CARTESIAN_POINT('Ctrl Pts',(-7.22480663496711,-36.9488329423689,
18.4898807817139));
#33057=CARTESIAN_POINT('Ctrl Pts',(-7.17064980608984,-36.8693388486506,
18.495214702772));
#33058=CARTESIAN_POINT('Ctrl Pts',(-7.03604808777771,-36.652483273502,18.5091409839819));
#33059=CARTESIAN_POINT('Ctrl Pts',(-6.96176965723963,-36.5115791388387,
18.5175561156818));
#33060=CARTESIAN_POINT('Ctrl Pts',(-6.82305328459711,-36.1965333013897,
18.5358082816679));
#33061=CARTESIAN_POINT('Ctrl Pts',(-6.7624614118829,-36.0212795028723,18.5456225529541));
#33062=CARTESIAN_POINT('Ctrl Pts',(-6.70785374268399,-35.8083225048791,
18.5580422966834));
#33063=CARTESIAN_POINT('Ctrl Pts',(-6.69974185301445,-35.774537422732,18.5600273869828));
#33064=CARTESIAN_POINT('Ctrl Pts',(-6.68820203150838,-35.7229978848826,
18.5630861173421));
#33065=CARTESIAN_POINT('Ctrl Pts',(-6.68439425470741,-35.7053298771089,
18.5641400686341));
#33066=CARTESIAN_POINT('Ctrl Pts',(-6.6776977075306,-35.6730049726649,18.566079585272));
#33067=CARTESIAN_POINT('Ctrl Pts',(-6.67476427489355,-35.6583582323194,
18.5669627045738));
#33068=CARTESIAN_POINT('Ctrl Pts',(-6.66817914558223,-35.6243112561122,
18.569025384291));
#33069=CARTESIAN_POINT('Ctrl Pts',(-6.66460001719369,-35.60489806064,18.5702087600021));
#33070=CARTESIAN_POINT('Ctrl Pts',(-6.65341850820725,-35.5411307161891,
18.5741171559401));
#33071=CARTESIAN_POINT('Ctrl Pts',(-6.64653007681595,-35.4966580252875,
18.5768766383884));
#33072=CARTESIAN_POINT('Ctrl Pts',(-6.63169189566488,-35.3863894336289,
18.5837805623838));
#33073=CARTESIAN_POINT('Ctrl Pts',(-6.62478263028336,-35.3204732486462,
18.587961534498));
#33074=CARTESIAN_POINT('Ctrl Pts',(-6.59944757504377,-34.983849319207,18.6094602550772));
#33075=CARTESIAN_POINT('Ctrl Pts',(-6.61164025555888,-34.7117881422173,
18.6272151811768));
#33076=CARTESIAN_POINT('Ctrl Pts',(-6.67065558785496,-34.3568047009002,
18.6496033405606));
#33077=CARTESIAN_POINT('Ctrl Pts',(-6.68857958873701,-34.2701154978643,
18.655017960122));
#33078=CARTESIAN_POINT('Ctrl Pts',(-6.71880925266393,-34.1481960826065,
18.6625563139971));
#33079=CARTESIAN_POINT('Ctrl Pts',(-6.7283328481143,-34.1123194010776,18.6647651953944));
#33080=CARTESIAN_POINT('Ctrl Pts',(-6.74578859275448,-34.0506633339324,
18.6685463835757));
#33081=CARTESIAN_POINT('Ctrl Pts',(-6.75344253429222,-34.0248094171066,
18.6701273667004));
#33082=CARTESIAN_POINT('Ctrl Pts',(-6.76980080030374,-33.9718819409708,
18.673355494956));
#33083=CARTESIAN_POINT('Ctrl Pts',(-6.77853899142676,-33.9448210318468,
18.6750014057077));
#33084=CARTESIAN_POINT('Ctrl Pts',(-6.80192063656046,-33.8754107135872,
18.6792131744246));
#33085=CARTESIAN_POINT('Ctrl Pts',(-6.81706535669886,-33.833235242997,18.681762680768));
#33086=CARTESIAN_POINT('Ctrl Pts',(-6.9019704603064,-33.6107593076599,18.695179582384));
#33087=CARTESIAN_POINT('Ctrl Pts',(-6.98622468615936,-33.4363676811077,
18.7055577256501));
#33088=CARTESIAN_POINT('Ctrl Pts',(-7.1886866603987,-33.095194185605,18.7266282824366));
#33089=CARTESIAN_POINT('Ctrl Pts',(-7.30799856086935,-32.9300042637491,
18.7372713487305));
#33090=CARTESIAN_POINT('Ctrl Pts',(-7.47612085504177,-32.7365415700979,
18.7515098503233));
#33091=CARTESIAN_POINT('Ctrl Pts',(-7.51179091238259,-32.6973873712854,
18.7544956269074));
#33092=CARTESIAN_POINT('Ctrl Pts',(-7.56323019788442,-32.6435149984917,
18.7587797369064));
#33093=CARTESIAN_POINT('Ctrl Pts',(-7.57824655962961,-32.6280854034999,
18.7600278961994));
#33094=CARTESIAN_POINT('Ctrl Pts',(-7.60407813739368,-32.6020439887711,
18.7621730236245));
#33095=CARTESIAN_POINT('Ctrl Pts',(-7.61481960187461,-32.5913594983349,
18.7630644850142));
#33096=CARTESIAN_POINT('Ctrl Pts',(-7.63777718931109,-32.5688278497078,
18.7649693705438));
#33097=CARTESIAN_POINT('Ctrl Pts',(-7.65001126983398,-32.5570002921701,
18.7659840955195));
#33098=CARTESIAN_POINT('Ctrl Pts',(-7.68451809053389,-32.5241391253324,
18.7688437503801));
#33099=CARTESIAN_POINT('Ctrl Pts',(-7.70698713908062,-32.503315113735,18.7707030147454));
#33100=CARTESIAN_POINT('Ctrl Pts',(-7.75895290914514,-32.45644713967,18.7749904932201));
#33101=CARTESIAN_POINT('Ctrl Pts',(-7.78862684921236,-32.4306067331975,
18.7774297813377));
#33102=CARTESIAN_POINT('Ctrl Pts',(-7.89086491244491,-32.344659745318,18.7857851952846));
#33103=CARTESIAN_POINT('Ctrl Pts',(-7.9654802216647,-32.2870661386771,18.7918007486963));
#33104=CARTESIAN_POINT('Ctrl Pts',(-8.27333827740561,-32.0692885299454,
18.8160346946936));
#33105=CARTESIAN_POINT('Ctrl Pts',(-8.52387278761695,-31.9354396280636,
18.8343522476638));
#33106=CARTESIAN_POINT('Ctrl Pts',(-8.83698466013862,-31.8155793734949,
18.8547560357336));
#33107=CARTESIAN_POINT('Ctrl Pts',(-8.88624770630459,-31.7980169127796,
18.8579028433028));
#33108=CARTESIAN_POINT('Ctrl Pts',(-8.96463871014907,-31.7720984692396,
18.8628130766327));
#33109=CARTESIAN_POINT('Ctrl Pts',(-8.99350455856831,-31.7629815712283,
18.8646007410966));
#33110=CARTESIAN_POINT('Ctrl Pts',(-9.0475873805674,-31.7466936343888,18.8679131964173));
#33111=CARTESIAN_POINT('Ctrl Pts',(-9.07277271641578,-31.7394261658924,
18.8694409808716));
#33112=CARTESIAN_POINT('Ctrl Pts',(-9.12999083630758,-31.7236319293576,
18.872879752454));
#33113=CARTESIAN_POINT('Ctrl Pts',(-9.16206972925407,-31.7152813436048,
18.8747850187413));
#33114=CARTESIAN_POINT('Ctrl Pts',(-9.26110465546569,-31.6910464568305,
18.8806016352486));
#33115=CARTESIAN_POINT('Ctrl Pts',(-9.32842784161424,-31.6767287799142,
18.8844640931337));
#33116=CARTESIAN_POINT('Ctrl Pts',(-9.48956637990019,-31.6475566437947,
18.8935307373691));
#33117=CARTESIAN_POINT('Ctrl Pts',(-9.58366231910807,-31.634575287889,18.8986827212484));
#33118=CARTESIAN_POINT('Ctrl Pts',(-9.81192811106071,-31.6128058270445,
18.9109842334276));
#33119=CARTESIAN_POINT('Ctrl Pts',(-9.94631440408638,-31.6080133025493,
18.9180618170391));
#33120=CARTESIAN_POINT('Ctrl Pts',(-10.2452954378598,-31.6151269838291,
18.9339608201663));
#33121=CARTESIAN_POINT('Ctrl Pts',(-10.4094393189859,-31.6310412971696,
18.94279341346));
#33122=CARTESIAN_POINT('Ctrl Pts',(-10.5998792455353,-31.6636301120385,
18.9537924781046));
#33123=CARTESIAN_POINT('Ctrl Pts',(-10.6279396037921,-31.6687973824746,
18.9554327660765));
#33124=CARTESIAN_POINT('Ctrl Pts',(-10.6721884930077,-31.6775246727265,
18.9580551671047));
#33125=CARTESIAN_POINT('Ctrl Pts',(-10.6884224815881,-31.6808503902108,
18.9590249308205));
#33126=CARTESIAN_POINT('Ctrl Pts',(-10.7196327192991,-31.6874829773589,
18.9609052200413));
#33127=CARTESIAN_POINT('Ctrl Pts',(-10.7346119324671,-31.6907726656868,
18.9618148278932));
#33128=CARTESIAN_POINT('Ctrl Pts',(-10.7716311645891,-31.6991664348316,
18.9640798298665));
#33129=CARTESIAN_POINT('Ctrl Pts',(-10.7936432026019,-31.7043896945485,
18.9654415773468));
#33130=CARTESIAN_POINT('Ctrl Pts',(-10.8787282346104,-31.7254814510871,
18.970758983208));
#33131=CARTESIAN_POINT('Ctrl Pts',(-10.9413883522577,-31.7429427563722,
18.9747896425663));
#33132=CARTESIAN_POINT('Ctrl Pts',(-11.1138394929039,-31.796391066361,18.9861335968407));
#33133=CARTESIAN_POINT('Ctrl Pts',(-11.2223508278271,-31.8362040814966,
18.9935569811521));
#33134=CARTESIAN_POINT('Ctrl Pts',(-11.563625161657,-31.9816002236887,19.0174613192039));
#33135=CARTESIAN_POINT('Ctrl Pts',(-11.7866056809594,-32.1079867292141,
19.0338700050418));
#33136=CARTESIAN_POINT('Ctrl Pts',(-12.0342478586321,-32.2880255862164,
19.0524707901725));
#33137=CARTESIAN_POINT('Ctrl Pts',(-12.0745372071784,-32.3187194548577,
19.0555138727141));
#33138=CARTESIAN_POINT('Ctrl Pts',(-12.1372938188597,-32.3687914018689,
19.0602831952697));
#33139=CARTESIAN_POINT('Ctrl Pts',(-12.1602193550271,-32.3875804363166,
19.0620319406714));
#33140=CARTESIAN_POINT('Ctrl Pts',(-12.2032181771113,-32.4237740154303,
19.0653252976279));
#33141=CARTESIAN_POINT('Ctrl Pts',(-12.2233389244651,-32.4411184580734,
19.0668721369762));
#33142=CARTESIAN_POINT('Ctrl Pts',(-12.2689709539587,-32.4813986920384,
19.0703947754584));
#33143=CARTESIAN_POINT('Ctrl Pts',(-12.294342333644,-32.5044890068333,19.0723640439074));
#33144=CARTESIAN_POINT('Ctrl Pts',(-12.3744593674015,-32.5796578095867,
19.0786219805554));
#33145=CARTESIAN_POINT('Ctrl Pts',(-12.4278178244577,-32.6331845522344,
19.0828498272079));
#33146=CARTESIAN_POINT('Ctrl Pts',(-12.5534346986981,-32.7679201282267,
19.0930080478961));
#33147=CARTESIAN_POINT('Ctrl Pts',(-12.6236634372342,-32.8509067920648,
19.0988658796263));
#33148=CARTESIAN_POINT('Ctrl Pts',(-12.81405373795,-33.0991574364479,19.1155633335551));
#33149=CARTESIAN_POINT('Ctrl Pts',(-12.923416834321,-33.2720746587202,19.1262019620166));
#33150=CARTESIAN_POINT('Ctrl Pts',(-13.0523092494715,-33.5235316630535,
19.1416406721746));
#33151=CARTESIAN_POINT('Ctrl Pts',(-13.0856347582639,-33.5945083183905,
19.1459984642093));
#33152=CARTESIAN_POINT('Ctrl Pts',(-13.1262158566297,-33.6893537579689,
19.1519013883363));
#33153=CARTESIAN_POINT('Ctrl Pts',(-13.1357135010849,-33.7122422912396,
19.153331886331));
#33154=CARTESIAN_POINT('Ctrl Pts',(-13.1502593583121,-33.7484118745938,
19.1556048590737));
#33155=CARTESIAN_POINT('Ctrl Pts',(-13.155476662514,-33.761624500976,19.156437753559));
#33156=CARTESIAN_POINT('Ctrl Pts',(-13.1662316670458,-33.7893704231475,
19.1581929677179));
#33157=CARTESIAN_POINT('Ctrl Pts',(-13.1717526174749,-33.803909600387,19.1591163004037));
#33158=CARTESIAN_POINT('Ctrl Pts',(-13.1776997615675,-33.8199018810217,
19.1601354427775));
#33159=CARTESIAN_POINT('Ctrl Pts',(-13.1782254172952,-33.8213183033965,
19.1602257375613));
#33160=CARTESIAN_POINT('Ctrl Pts',(-13.1787501240201,-33.8227350716418,
19.1603160842799));
#33161=CARTESIAN_POINT('Origin',(-10.,-35.,23.));
#33162=CARTESIAN_POINT('',(-13.1787501237351,-33.8227350708723,20.4156322019944));
#33163=CARTESIAN_POINT('',(-13.1787501240278,-33.8227350716626,20.0676097122989));
#33164=CARTESIAN_POINT('',(-13.1787501240207,-33.8227350716434,23.));
#33165=CARTESIAN_POINT('Ctrl Pts',(-13.1787501240278,-33.8227350716626,
20.0676097122989));
#33166=CARTESIAN_POINT('Ctrl Pts',(-13.1611853468585,-33.7753081618307,
20.0645358172842));
#33167=CARTESIAN_POINT('Ctrl Pts',(-13.1425606400635,-33.7282783450763,
20.0614952758765));
#33168=CARTESIAN_POINT('Ctrl Pts',(-13.1112568932655,-33.6541247221329,
20.0567113797675));
#33169=CARTESIAN_POINT('Ctrl Pts',(-13.099259690771,-33.6267231981489,20.0549458528331));
#33170=CARTESIAN_POINT('Ctrl Pts',(-13.0759469510001,-33.5753392155133,
20.0516382942934));
#33171=CARTESIAN_POINT('Ctrl Pts',(-13.0647097156829,-33.5513239100277,
20.0500937795061));
#33172=CARTESIAN_POINT('Ctrl Pts',(-13.0384948140615,-33.4969700983274,
20.046599939044));
#33173=CARTESIAN_POINT('Ctrl Pts',(-13.0233422630176,-33.4667187802419,
20.0446567445545));
#33174=CARTESIAN_POINT('Ctrl Pts',(-12.9741865859815,-33.3721449234778,
20.0385816191994));
#33175=CARTESIAN_POINT('Ctrl Pts',(-12.9385632426113,-33.308685392804,20.0345054032097));
#33176=CARTESIAN_POINT('Ctrl Pts',(-12.7492455449724,-32.9955000486554,
20.0142917830798));
#33177=CARTESIAN_POINT('Ctrl Pts',(-12.5656684892498,-32.765339734078,19.9992411396829));
#33178=CARTESIAN_POINT('Ctrl Pts',(-12.3059904598391,-32.5145598716652,
19.9797116865118));
#33179=CARTESIAN_POINT('Ctrl Pts',(-12.2558052955851,-32.4689239099351,
19.9759977495463));
#33180=CARTESIAN_POINT('Ctrl Pts',(-12.1695355872243,-32.3950790764823,
19.9696472301789));
#33181=CARTESIAN_POINT('Ctrl Pts',(-12.1341863687468,-32.3660399003952,
19.9670539915919));
#33182=CARTESIAN_POINT('Ctrl Pts',(-12.082659346815,-32.3254290472168,19.9632690030034));
#33183=CARTESIAN_POINT('Ctrl Pts',(-12.0669490907539,-32.3132694308581,
19.9621143428392));
#33184=CARTESIAN_POINT('Ctrl Pts',(-12.0392317543396,-32.2922034082524,
19.9600743146627));
#33185=CARTESIAN_POINT('Ctrl Pts',(-12.0272712214014,-32.2832372364144,
19.9591930115543));
#33186=CARTESIAN_POINT('Ctrl Pts',(-12.0007909774868,-32.2636586581814,
19.9572392635049));
#33187=CARTESIAN_POINT('Ctrl Pts',(-11.986246071251,-32.2530826391922,19.9561646006955));
#33188=CARTESIAN_POINT('Ctrl Pts',(-11.9428365403902,-32.2220433511747,
19.9529544518074));
#33189=CARTESIAN_POINT('Ctrl Pts',(-11.9137357601464,-32.2019163355518,
19.9507988211438));
#33190=CARTESIAN_POINT('Ctrl Pts',(-11.72870768896,-32.0781817134344,19.9370968595503));
#33191=CARTESIAN_POINT('Ctrl Pts',(-11.5647463020549,-31.9871920798866,
19.9249909928736));
#33192=CARTESIAN_POINT('Ctrl Pts',(-11.2506782001936,-31.8454832450127,
19.9027863463488));
#33193=CARTESIAN_POINT('Ctrl Pts',(-11.1028855288573,-31.7908220921335,
19.8926988712996));
#33194=CARTESIAN_POINT('Ctrl Pts',(-10.860121843555,-31.7197982307892,19.876920978072));
#33195=CARTESIAN_POINT('Ctrl Pts',(-10.7673250960579,-31.6968578472047,
19.8710644115977));
#33196=CARTESIAN_POINT('Ctrl Pts',(-10.6371360758448,-31.6704575776151,
19.8630908578149));
#33197=CARTESIAN_POINT('Ctrl Pts',(-10.6004754981986,-31.6636510278115,
19.8608716578841));
#33198=CARTESIAN_POINT('Ctrl Pts',(-10.5370934559862,-31.6529618743906,
19.8570783816861));
#33199=CARTESIAN_POINT('Ctrl Pts',(-10.5104247471574,-31.6487912277859,
19.8554954837629));
#33200=CARTESIAN_POINT('Ctrl Pts',(-10.4556145866066,-31.6408890933222,
19.8522682473569));
#33201=CARTESIAN_POINT('Ctrl Pts',(-10.4274703327131,-31.6371916616105,
19.8506250820894));
#33202=CARTESIAN_POINT('Ctrl Pts',(-10.3550419318484,-31.6286004332206,
19.8464304174761));
#33203=CARTESIAN_POINT('Ctrl Pts',(-10.3107010440653,-31.6242252840418,
19.8438949997539));
#33204=CARTESIAN_POINT('Ctrl Pts',(-10.0931031414894,-31.6070786695997,
19.8315938814629));
#33205=CARTESIAN_POINT('Ctrl Pts',(-9.91912016172872,-31.6067639673029,
19.8222131202546));
#33206=CARTESIAN_POINT('Ctrl Pts',(-9.56089029654409,-31.6336969049995,
19.8030834940875));
#33207=CARTESIAN_POINT('Ctrl Pts',(-9.377379939208,-31.6627628969024,19.7933834722086));
#33208=CARTESIAN_POINT('Ctrl Pts',(-9.11543702474463,-31.72661762402,19.7786880680003));
#33209=CARTESIAN_POINT('Ctrl Pts',(-9.03447156840141,-31.749579023568,19.7740203113382));
#33210=CARTESIAN_POINT('Ctrl Pts',(-8.93102322441993,-31.7831225913699,
19.7677962255488));
#33211=CARTESIAN_POINT('Ctrl Pts',(-8.90768008125241,-31.7909738660044,
19.7663742831878));
#33212=CARTESIAN_POINT('Ctrl Pts',(-8.86956932772088,-31.8042561015582,
19.7640208972209));
#33213=CARTESIAN_POINT('Ctrl Pts',(-8.8547498525729,-31.8095369220686,19.7630978068953));
#33214=CARTESIAN_POINT('Ctrl Pts',(-8.82677319264438,-31.8197262513598,
19.7613391071707));
#33215=CARTESIAN_POINT('Ctrl Pts',(-8.81360870219809,-31.8246137352099,
19.7605047871282));
#33216=CARTESIAN_POINT('Ctrl Pts',(-8.77811132179096,-31.8380441401931,
19.7582375120424));
#33217=CARTESIAN_POINT('Ctrl Pts',(-8.7558382593947,-31.846741638616,19.7567960001449));
#33218=CARTESIAN_POINT('Ctrl Pts',(-8.66859845564776,-31.8818764383098,
19.751080418585));
#33219=CARTESIAN_POINT('Ctrl Pts',(-8.60437037262096,-31.9100904206449,
19.7467201914259));
#33220=CARTESIAN_POINT('Ctrl Pts',(-8.37017146646221,-32.0217606199007,
19.7303664474104));
#33221=CARTESIAN_POINT('Ctrl Pts',(-8.20640599282022,-32.1174196323892,
19.7180428013634));
#33222=CARTESIAN_POINT('Ctrl Pts',(-7.89977225548018,-32.3328247178107,
19.6940168808215));
#33223=CARTESIAN_POINT('Ctrl Pts',(-7.75704118188679,-32.4516802642273,
19.6823490353678));
#33224=CARTESIAN_POINT('Ctrl Pts',(-7.59296174265422,-32.6128353619107,
19.6684468833062));
#33225=CARTESIAN_POINT('Ctrl Pts',(-7.56180779388541,-32.6446640938806,
19.6657812837434));
#33226=CARTESIAN_POINT('Ctrl Pts',(-7.51184066651742,-32.6977676839168,
19.6614608145589));
#33227=CARTESIAN_POINT('Ctrl Pts',(-7.49265232859032,-32.7186805936257,
19.6597902119846));
#33228=CARTESIAN_POINT('Ctrl Pts',(-7.45573060093968,-32.7599493538083,
19.6565520219705));
#33229=CARTESIAN_POINT('Ctrl Pts',(-7.43797331849109,-32.7802808696794,
19.6549835115507));
#33230=CARTESIAN_POINT('Ctrl Pts',(-7.39626501728809,-32.8292028996488,
19.6512711479091));
#33231=CARTESIAN_POINT('Ctrl Pts',(-7.37253899993583,-32.8579811485152,
19.6491364132991));
#33232=CARTESIAN_POINT('Ctrl Pts',(-7.29345492890884,-32.9571970752566,
19.6419345124926));
#33233=CARTESIAN_POINT('Ctrl Pts',(-7.24041394565002,-33.0294374841514,
19.6369559349648));
#33234=CARTESIAN_POINT('Ctrl Pts',(-7.04295711140645,-33.3220047531251,
19.6176508908766));
#33235=CARTESIAN_POINT('Ctrl Pts',(-6.92157235358177,-33.5567235724241,
19.6040656428064));
#33236=CARTESIAN_POINT('Ctrl Pts',(-6.80383465870549,-33.8686976563005,
19.5860516642116));
#33237=CARTESIAN_POINT('Ctrl Pts',(-6.78112733445468,-33.9350231730128,
19.5822189121504));
#33238=CARTESIAN_POINT('Ctrl Pts',(-6.74670955580571,-34.0467433695319,
19.5756874641138));
#33239=CARTESIAN_POINT('Ctrl Pts',(-6.73385488040754,-34.091764056572,19.5730353796341));
#33240=CARTESIAN_POINT('Ctrl Pts',(-6.71683463237456,-34.1564171818552,
19.5691796650591));
#33241=CARTESIAN_POINT('Ctrl Pts',(-6.71190410388051,-34.1758445912841,
19.5680150557355));
#33242=CARTESIAN_POINT('Ctrl Pts',(-6.70359403968709,-34.2098501885008,
19.5659642405519));
#33243=CARTESIAN_POINT('Ctrl Pts',(-6.70013828832138,-34.2244088363186,
19.5650822560961));
#33244=CARTESIAN_POINT('Ctrl Pts',(-6.69276971516678,-34.2563926978317,
19.5631354784728));
#33245=CARTESIAN_POINT('Ctrl Pts',(-6.68889817987596,-34.2738259972481,
19.5620685859996));
#33246=CARTESIAN_POINT('Ctrl Pts',(-6.67811567128542,-34.3242587156416,
19.558967148552));
#33247=CARTESIAN_POINT('Ctrl Pts',(-6.67155923932524,-34.3573308049227,
19.5569148203269));
#33248=CARTESIAN_POINT('Ctrl Pts',(-6.62035128375505,-34.6374806322714,
19.5394047114061));
#33249=CARTESIAN_POINT('Ctrl Pts',(-6.60278758370256,-34.888706792209,19.522948874795));
#33250=CARTESIAN_POINT('Ctrl Pts',(-6.61796212383946,-35.2569707242624,
19.4993579350556));
#33251=CARTESIAN_POINT('Ctrl Pts',(-6.62890263878737,-35.3740595957055,
19.4919248274958));
#33252=CARTESIAN_POINT('Ctrl Pts',(-6.65742461145622,-35.5691550810337,
19.4797226243928));
#33253=CARTESIAN_POINT('Ctrl Pts',(-6.67171945646803,-35.6475321798334,
19.4748699296963));
#33254=CARTESIAN_POINT('Ctrl Pts',(-6.69624504014244,-35.759493793627,19.4680083786439));
#33255=CARTESIAN_POINT('Ctrl Pts',(-6.70425520842962,-35.7935326481029,
19.4659316826203));
#33256=CARTESIAN_POINT('Ctrl Pts',(-6.71929456906651,-35.8532800341837,
19.4623018077232));
#33257=CARTESIAN_POINT('Ctrl Pts',(-6.72610282747604,-35.8790405594974,
19.4607418086034));
#33258=CARTESIAN_POINT('Ctrl Pts',(-6.74103385251855,-35.9329539583043,
19.457486558318));
#33259=CARTESIAN_POINT('Ctrl Pts',(-6.74921935847811,-35.961087268357,19.4557934525214));
#33260=CARTESIAN_POINT('Ctrl Pts',(-6.77206196209059,-36.0359635560181,
19.4512999845432));
#33261=CARTESIAN_POINT('Ctrl Pts',(-6.78736949485529,-36.0825017521497,
19.4485205595353));
#33262=CARTESIAN_POINT('Ctrl Pts',(-6.89296663141016,-36.3815396500134,
19.4307154226582));
#33263=CARTESIAN_POINT('Ctrl Pts',(-7.01193493440893,-36.6228942557022,
19.4166951656437));
#33264=CARTESIAN_POINT('Ctrl Pts',(-7.24502229282914,-36.9813949015625,
19.3939448329222));
#33265=CARTESIAN_POINT('Ctrl Pts',(-7.34124890867364,-37.1087578283937,
19.3853772865324));
#33266=CARTESIAN_POINT('Ctrl Pts',(-7.46475761880317,-37.2502798016761,
19.3746825590842));
#33267=CARTESIAN_POINT('Ctrl Pts',(-7.48371678793185,-37.2714602795498,
19.3730481757949));
#33268=CARTESIAN_POINT('Ctrl Pts',(-7.51413051543064,-37.3045892932183,
19.3704330879398));
#33269=CARTESIAN_POINT('Ctrl Pts',(-7.52541047499721,-37.3166971235827,
19.3694646179305));
#33270=CARTESIAN_POINT('Ctrl Pts',(-7.54720055073982,-37.3397457292179,
19.3675953660787));
#33271=CARTESIAN_POINT('Ctrl Pts',(-7.55769618130358,-37.350699308632,19.3666956103486));
#33272=CARTESIAN_POINT('Ctrl Pts',(-7.58143745514546,-37.3751458453699,
19.3646623692457));
#33273=CARTESIAN_POINT('Ctrl Pts',(-7.59472318478407,-37.3885991661621,
19.3635259687682));
#33274=CARTESIAN_POINT('Ctrl Pts',(-7.64232656506652,-37.4360031557601,
19.3594614917787));
#33275=CARTESIAN_POINT('Ctrl Pts',(-7.67725466493795,-37.46932966877,19.3564925850621));
#33276=CARTESIAN_POINT('Ctrl Pts',(-7.86577981016146,-37.6416706991776,
19.3405923055625));
#33277=CARTESIAN_POINT('Ctrl Pts',(-8.03116332555608,-37.7671278048527,
19.3270986645285));
#33278=CARTESIAN_POINT('Ctrl Pts',(-8.37276183680249,-37.9800458057855,
19.3012508776266));
#33279=CARTESIAN_POINT('Ctrl Pts',(-8.54721145733076,-38.0688763949976,
19.2889244251002));
#33280=CARTESIAN_POINT('Ctrl Pts',(-8.76996210152708,-38.1590228584702,
19.2743944193604));
#33281=CARTESIAN_POINT('Ctrl Pts',(-8.81188952445043,-38.1750295178659,
19.2717077962796));
#33282=CARTESIAN_POINT('Ctrl Pts',(-8.88090021395099,-38.199817213159,19.267362247924));
#33283=CARTESIAN_POINT('Ctrl Pts',(-8.90779706059852,-38.2090975899293,
19.2656872375211));
#33284=CARTESIAN_POINT('Ctrl Pts',(-8.96040147925873,-38.2265099971639,
19.2624464713426));
#33285=CARTESIAN_POINT('Ctrl Pts',(-8.98609544144652,-38.2346760972051,
19.2608797131301));
#33286=CARTESIAN_POINT('Ctrl Pts',(-9.04735744456869,-38.253344801224,19.2571809411306));
#33287=CARTESIAN_POINT('Ctrl Pts',(-9.08300617360643,-38.2635720782276,
19.2550578583474));
#33288=CARTESIAN_POINT('Ctrl Pts',(-9.20398881013651,-38.2961418823728,
19.2479444240423));
#33289=CARTESIAN_POINT('Ctrl Pts',(-9.29002760445747,-38.3157391417449,
19.2430396121035));
#33290=CARTESIAN_POINT('Ctrl Pts',(-9.64378970841421,-38.3819123559373,
19.223341819376));
#33291=CARTESIAN_POINT('Ctrl Pts',(-9.91585905934855,-38.3995775941096,
19.2093577381375));
#33292=CARTESIAN_POINT('Ctrl Pts',(-10.2533021625765,-38.3809226174505,
19.1910572017665));
#33293=CARTESIAN_POINT('Ctrl Pts',(-10.3193685896116,-38.3753225855994,
19.1874233018042));
#33294=CARTESIAN_POINT('Ctrl Pts',(-10.4299473272693,-38.362674029551,19.1811951147816));
#33295=CARTESIAN_POINT('Ctrl Pts',(-10.4745612976508,-38.3566683641654,
19.1786420343931));
#33296=CARTESIAN_POINT('Ctrl Pts',(-10.5385513147805,-38.3467532576821,
19.174905375416));
#33297=CARTESIAN_POINT('Ctrl Pts',(-10.5580351500368,-38.343559722372,19.1737575957409));
#33298=CARTESIAN_POINT('Ctrl Pts',(-10.5922100331009,-38.3376511968254,
19.1717249940317));
#33299=CARTESIAN_POINT('Ctrl Pts',(-10.6069127576297,-38.3350090145937,
19.1708441291067));
#33300=CARTESIAN_POINT('Ctrl Pts',(-10.6393637676653,-38.3289556381055,
19.1688854154355));
#33301=CARTESIAN_POINT('Ctrl Pts',(-10.6571023192061,-38.3254996884165,
19.1678052649529));
#33302=CARTESIAN_POINT('Ctrl Pts',(-10.7099331864079,-38.3147676142774,
19.1645616809863));
#33303=CARTESIAN_POINT('Ctrl Pts',(-10.744937598293,-38.3070768391787,19.1623774978116));
#33304=CARTESIAN_POINT('Ctrl Pts',(-10.9244070868059,-38.2646520009408,
19.151020528956));
#33305=CARTESIAN_POINT('Ctrl Pts',(-11.0665874787242,-38.2210037792346,
19.141498603022));
#33306=CARTESIAN_POINT('Ctrl Pts',(-11.3243046032701,-38.1229470467411,
19.1237370464006));
#33307=CARTESIAN_POINT('Ctrl Pts',(-11.4405398140531,-38.0710630035466,
19.1155228035228));
#33308=CARTESIAN_POINT('Ctrl Pts',(-11.6434641435263,-37.9664215234145,
19.1009929985612));
#33309=CARTESIAN_POINT('Ctrl Pts',(-11.7312278867476,-37.9160733361442,
19.0946392723619));
#33310=CARTESIAN_POINT('Ctrl Pts',(-11.8773329560114,-37.8233310446316,
19.0839755566213));
#33311=CARTESIAN_POINT('Ctrl Pts',(-11.93681223353,-37.7828648459176,19.0796075647189));
#33312=CARTESIAN_POINT('Ctrl Pts',(-12.022197371093,-37.7207090326118,19.0732951080739));
#33313=CARTESIAN_POINT('Ctrl Pts',(-12.0491358446431,-37.7004781541207,
19.071297043557));
#33314=CARTESIAN_POINT('Ctrl Pts',(-12.0967167044531,-37.6636227593792,
19.0677549023571));
#33315=CARTESIAN_POINT('Ctrl Pts',(-12.1174738447297,-37.6471516237341,
19.0662050832352));
#33316=CARTESIAN_POINT('Ctrl Pts',(-12.1613122314387,-37.6115195196296,
19.0629210718914));
#33317=CARTESIAN_POINT('Ctrl Pts',(-12.1843366701767,-37.5922920664684,
19.061189694256));
#33318=CARTESIAN_POINT('Ctrl Pts',(-12.2458296142369,-37.5395389026308,
19.056545175639));
#33319=CARTESIAN_POINT('Ctrl Pts',(-12.2838020755113,-37.5054454603878,
19.0536551283866));
#33320=CARTESIAN_POINT('Ctrl Pts',(-12.5009175032319,-37.3014698201752,
19.0369651388992));
#33321=CARTESIAN_POINT('Ctrl Pts',(-12.6618394362214,-37.1132850329462,
19.0239862285052));
#33322=CARTESIAN_POINT('Ctrl Pts',(-12.899684260763,-36.7643675571192,19.0015660251271));
#33323=CARTESIAN_POINT('Ctrl Pts',(-12.9870591560932,-36.6120252524541,
18.992199849269));
#33324=CARTESIAN_POINT('Ctrl Pts',(-13.074544533561,-36.4277265536526,18.9805880349539));
#33325=CARTESIAN_POINT('Ctrl Pts',(-13.0865108010922,-36.4016697758418,
18.9789398844224));
#33326=CARTESIAN_POINT('Ctrl Pts',(-13.1048804590286,-36.3602933345371,
18.9763078668655));
#33327=CARTESIAN_POINT('Ctrl Pts',(-13.1115045591466,-36.3450724790802,
18.9753365072467));
#33328=CARTESIAN_POINT('Ctrl Pts',(-13.1239572817365,-36.3158743448492,
18.9734660452761));
#33329=CARTESIAN_POINT('Ctrl Pts',(-13.1298044531037,-36.301905696061,18.9725680284185));
#33330=CARTESIAN_POINT('Ctrl Pts',(-13.14406548639,-36.2671853488605,18.9703288036037));
#33331=CARTESIAN_POINT('Ctrl Pts',(-13.1523676076886,-36.2463887427764,
18.9689813365523));
#33332=CARTESIAN_POINT('Ctrl Pts',(-13.1816270525135,-36.1709318029151,
18.9640737920417));
#33333=CARTESIAN_POINT('Ctrl Pts',(-13.2013725906665,-36.1158157043508,
18.9604544513983));
#33334=CARTESIAN_POINT('Ctrl Pts',(-13.2818106808362,-35.8715409242023,
18.9443435420874));
#33335=CARTESIAN_POINT('Ctrl Pts',(-13.3272339491523,-35.6777724713108,
18.9314074419919));
#33336=CARTESIAN_POINT('Ctrl Pts',(-13.3781944289231,-35.3223842453021,
18.9083686215589));
#33337=CARTESIAN_POINT('Ctrl Pts',(-13.3896657123435,-35.1621907236818,
18.8982236322739));
#33338=CARTESIAN_POINT('Ctrl Pts',(-13.389778607959,-34.9461372905748,18.8849939288848));
#33339=CARTESIAN_POINT('Ctrl Pts',(-13.388438049834,-34.8905087781159,18.8816264220252));
#33340=CARTESIAN_POINT('Ctrl Pts',(-13.3840803320592,-34.8011250038821,
18.8762764696107));
#33341=CARTESIAN_POINT('Ctrl Pts',(-13.381925533382,-34.7673397987074,18.8742682890804));
#33342=CARTESIAN_POINT('Ctrl Pts',(-13.377181046961,-34.7071582269766,18.8707148637787));
#33343=CARTESIAN_POINT('Ctrl Pts',(-13.3747870192056,-34.6807496871589,
18.8691637405984));
#33344=CARTESIAN_POINT('Ctrl Pts',(-13.3690346306615,-34.6246272115056,
18.8658837243108));
#33345=CARTESIAN_POINT('Ctrl Pts',(-13.3655924598424,-34.5949240197089,
18.8641575546559));
#33346=CARTESIAN_POINT('Ctrl Pts',(-13.3551001403706,-34.5137872241645,
18.859466777882));
#33347=CARTESIAN_POINT('Ctrl Pts',(-13.3472606761465,-34.4624628550752,
18.8565265836641));
#33348=CARTESIAN_POINT('Ctrl Pts',(-13.3091777776031,-34.2464988705079,
18.8442430615774));
#33349=CARTESIAN_POINT('Ctrl Pts',(-13.2679403249764,-34.0840332654547,
18.8352348849132));
#33350=CARTESIAN_POINT('Ctrl Pts',(-13.2033719792797,-33.8908891407193,
18.8244023837771));
#33351=CARTESIAN_POINT('Ctrl Pts',(-13.1913320735613,-33.856707778262,18.8224797537842));
#33352=CARTESIAN_POINT('Ctrl Pts',(-13.1787501466517,-33.8227351327498,
18.8205587414464));
#33353=CARTESIAN_POINT('',(-13.3897492734215,-34.9977805770088,19.2362441100456));
#33354=CARTESIAN_POINT('Ctrl Pts',(-13.1787501240201,-33.8227350716418,
19.1603160842799));
#33355=CARTESIAN_POINT('Ctrl Pts',(-13.1864743779049,-33.8435914416932,
19.161646086278));
#33356=CARTESIAN_POINT('Ctrl Pts',(-13.1939929729178,-33.8645227656139,
19.1629873410737));
#33357=CARTESIAN_POINT('Ctrl Pts',(-13.2259874889372,-33.9564263874323,
19.1688999912539));
#33358=CARTESIAN_POINT('Ctrl Pts',(-13.248306214562,-34.0281222976731,19.1735734052367));
#33359=CARTESIAN_POINT('Ctrl Pts',(-13.3486745287529,-34.3927961905211,
19.1974547585279));
#33360=CARTESIAN_POINT('Ctrl Pts',(-13.3895507473258,-34.6945694760009,
19.217413212814));
#33361=CARTESIAN_POINT('Ctrl Pts',(-13.3897492734215,-34.9977805770088,
19.2362441100456));
#33362=CARTESIAN_POINT('Ctrl Pts',(-13.3897492760003,-34.9977845192167,
19.236244354876));
#33363=CARTESIAN_POINT('Ctrl Pts',(-13.3897845749226,-35.0517928847712,
19.2395985377884));
#33364=CARTESIAN_POINT('Ctrl Pts',(-13.3885291145359,-35.1057969828223,
19.2429192167761));
#33365=CARTESIAN_POINT('Ctrl Pts',(-13.3840382928665,-35.2009817582665,
19.2487120744362));
#33366=CARTESIAN_POINT('Ctrl Pts',(-13.3813400213536,-35.2421749746294,
19.2511992241826));
#33367=CARTESIAN_POINT('Ctrl Pts',(-13.3756795764973,-35.3096641480058,
19.2552424422283));
#33368=CARTESIAN_POINT('Ctrl Pts',(-13.3731608174323,-35.3359920340823,
19.2568118173895));
#33369=CARTESIAN_POINT('Ctrl Pts',(-13.3676455837124,-35.3872997343317,
19.2598554009154));
#33370=CARTESIAN_POINT('Ctrl Pts',(-13.3646786396044,-35.4122809293162,
19.2613304166859));
#33371=CARTESIAN_POINT('Ctrl Pts',(-13.3577914067957,-35.4652304537003,
19.2644430440054));
#33372=CARTESIAN_POINT('Ctrl Pts',(-13.353799125562,-35.4931875932648,19.2660783040404));
#33373=CARTESIAN_POINT('Ctrl Pts',(-13.3427185322349,-35.5644110344104,
19.2702251560015));
#33374=CARTESIAN_POINT('Ctrl Pts',(-13.3351392672814,-35.6075963439119,
19.2727213995748));
#33375=CARTESIAN_POINT('Ctrl Pts',(-13.296058462672,-35.8074215452538,19.2842035962231));
#33376=CARTESIAN_POINT('Ctrl Pts',(-13.2543445292222,-35.9618628763027,
19.2928694811663));
#33377=CARTESIAN_POINT('Ctrl Pts',(-13.1383490953228,-36.2956197712006,
19.3117355404843));
#33378=CARTESIAN_POINT('Ctrl Pts',(-13.059272919385,-36.4726535645523,19.3218343031454));
#33379=CARTESIAN_POINT('Ctrl Pts',(-12.9217425693223,-36.7210451343814,
19.3372616502941));
#33380=CARTESIAN_POINT('Ctrl Pts',(-12.8748145766163,-36.798336603414,19.3422616321036));
#33381=CARTESIAN_POINT('Ctrl Pts',(-12.8109493466584,-36.8946245164247,
19.3488692801207));
#33382=CARTESIAN_POINT('Ctrl Pts',(-12.7968075449926,-36.9154387915058,
19.3503212366677));
#33383=CARTESIAN_POINT('Ctrl Pts',(-12.7733851514048,-36.9491000386322,
19.3527114435025));
#33384=CARTESIAN_POINT('Ctrl Pts',(-12.7642436310545,-36.9620431403915,
19.3536408211248));
#33385=CARTESIAN_POINT('Ctrl Pts',(-12.7457723506806,-36.9878105443928,
19.3555128129378));
#33386=CARTESIAN_POINT('Ctrl Pts',(-12.7364426676058,-37.0006344160155,
19.3564554125316));
#33387=CARTESIAN_POINT('Ctrl Pts',(-12.7120421745917,-37.0336834781207,
19.358912127531));
#33388=CARTESIAN_POINT('Ctrl Pts',(-12.6968352596872,-37.0538064041418,
19.3604349584379));
#33389=CARTESIAN_POINT('Ctrl Pts',(-12.6304483155188,-37.1396459325888,
19.367041392582));
#33390=CARTESIAN_POINT('Ctrl Pts',(-12.5770833450086,-37.2036293652792,
19.3722474779447));
#33391=CARTESIAN_POINT('Ctrl Pts',(-12.3879346911847,-37.4141378826565,
19.3901860990655));
#33392=CARTESIAN_POINT('Ctrl Pts',(-12.2415811064057,-37.5506096986927,
19.4032060297474));
#33393=CARTESIAN_POINT('Ctrl Pts',(-11.9566924007405,-37.7726957725488,
19.4262534029351));
#33394=CARTESIAN_POINT('Ctrl Pts',(-11.8223770407936,-37.8627680028019,
19.4363531739312));
#33395=CARTESIAN_POINT('Ctrl Pts',(-11.6444657816674,-37.9644594575813,
19.4487277933124));
#33396=CARTESIAN_POINT('Ctrl Pts',(-11.6063858318561,-37.9852658849396,
19.4513228272647));
#33397=CARTESIAN_POINT('Ctrl Pts',(-11.5429600089168,-38.0183558042834,
19.4555593685868));
#33398=CARTESIAN_POINT('Ctrl Pts',(-11.5178427355597,-38.0310643100842,
19.4572154406488));
#33399=CARTESIAN_POINT('Ctrl Pts',(-11.4684901122207,-38.0552677659962,
19.4604284252984));
#33400=CARTESIAN_POINT('Ctrl Pts',(-11.4442709384102,-38.0667908061405,
19.4619862113479));
#33401=CARTESIAN_POINT('Ctrl Pts',(-11.3855472598943,-38.0938804949821,
19.465719312078));
#33402=CARTESIAN_POINT('Ctrl Pts',(-11.3509134130815,-38.1091591853157,
19.4678848198425));
#33403=CARTESIAN_POINT('Ctrl Pts',(-11.2305431202365,-38.1598692547302,
19.4752943690897));
#33404=CARTESIAN_POINT('Ctrl Pts',(-11.143609868394,-38.1923609649953,19.4804426927704));
#33405=CARTESIAN_POINT('Ctrl Pts',(-10.8026758494185,-38.3040686270126,
19.5000333692691));
#33406=CARTESIAN_POINT('Ctrl Pts',(-10.5410520818374,-38.35684544356,19.5137354224122));
#33407=CARTESIAN_POINT('Ctrl Pts',(-10.210333311462,-38.3838587911433,19.5317087893995));
#33408=CARTESIAN_POINT('Ctrl Pts',(-10.144569352785,-38.3873056045895,19.5353191552091));
#33409=CARTESIAN_POINT('Ctrl Pts',(-10.0339647138807,-38.3898758513815,
19.5415112926484));
#33410=CARTESIAN_POINT('Ctrl Pts',(-9.9891651350432,-38.3900286281257,19.54405247508));
#33411=CARTESIAN_POINT('Ctrl Pts',(-9.92467337934728,-38.3889702474023,
19.5477747948146));
#33412=CARTESIAN_POINT('Ctrl Pts',(-9.90497250681671,-38.3884750511983,
19.548920510633));
#33413=CARTESIAN_POINT('Ctrl Pts',(-9.87034934580922,-38.3873025962247,
19.5509509327028));
#33414=CARTESIAN_POINT('Ctrl Pts',(-9.85542548127593,-38.3866984463618,
19.5518317148028));
#33415=CARTESIAN_POINT('Ctrl Pts',(-9.82242407454618,-38.3851439440076,
19.5537921348201));
#33416=CARTESIAN_POINT('Ctrl Pts',(-9.80435006495777,-38.3841474260754,
19.5548741014684));
#33417=CARTESIAN_POINT('Ctrl Pts',(-9.75037289045416,-38.3807375261865,
19.5581284079223));
#33418=CARTESIAN_POINT('Ctrl Pts',(-9.7145003391815,-38.3778972210151,19.5603216883914));
#33419=CARTESIAN_POINT('Ctrl Pts',(-9.52846418521909,-38.3601828585759,
19.571831760279));
#33420=CARTESIAN_POINT('Ctrl Pts',(-9.37938107206355,-38.3358656870698,
19.5815081576014));
#33421=CARTESIAN_POINT('Ctrl Pts',(-9.10374894855583,-38.2717872840282,
19.5997387997388));
#33422=CARTESIAN_POINT('Ctrl Pts',(-8.97692488673516,-38.2343743998584,
19.6082684906967));
#33423=CARTESIAN_POINT('Ctrl Pts',(-8.71638000743087,-38.1406501500173,
19.625857486038));
#33424=CARTESIAN_POINT('Ctrl Pts',(-8.58342192362891,-38.0829659163685,
19.6348694913263));
#33425=CARTESIAN_POINT('Ctrl Pts',(-8.41691090705096,-37.9976694432793,
19.646155627523));
#33426=CARTESIAN_POINT('Ctrl Pts',(-8.37963833479819,-37.9776872709997,
19.6486827369162));
#33427=CARTESIAN_POINT('Ctrl Pts',(-8.31838738648109,-37.9433592929094,
19.652838558637));
#33428=CARTESIAN_POINT('Ctrl Pts',(-8.29419579396036,-37.9294055692992,
19.6544807398343));
#33429=CARTESIAN_POINT('Ctrl Pts',(-8.24699091918078,-37.9013947038992,
19.6576876853369));
#33430=CARTESIAN_POINT('Ctrl Pts',(-8.22396751888269,-37.8873587848961,
19.6592530486379));
#33431=CARTESIAN_POINT('Ctrl Pts',(-8.17350936039638,-37.8557656979162,
19.6626877478857));
#33432=CARTESIAN_POINT('Ctrl Pts',(-8.14615506089277,-37.8380847104437,
19.6645524460385));
#33433=CARTESIAN_POINT('Ctrl Pts',(-8.05181835175569,-37.7751623597298,
19.6709972658533));
#33434=CARTESIAN_POINT('Ctrl Pts',(-7.98620010269377,-37.72792030648,19.6755044206689));
#33435=CARTESIAN_POINT('Ctrl Pts',(-7.70086023007183,-37.5065763306376,
19.695340422984));
#33436=CARTESIAN_POINT('Ctrl Pts',(-7.50156901498557,-37.3079864808002,
19.7097511677582));
#33437=CARTESIAN_POINT('Ctrl Pts',(-7.28778513431875,-37.0343981394582,
19.7285448794397));
#33438=CARTESIAN_POINT('Ctrl Pts',(-7.24814548197941,-36.9804497167778,
19.7322124223347));
#33439=CARTESIAN_POINT('Ctrl Pts',(-7.18438797133657,-36.8880646357383,
19.7384920718721));
#33440=CARTESIAN_POINT('Ctrl Pts',(-7.15939707648405,-36.8502523576473,
19.74106207898));
#33441=CARTESIAN_POINT('Ctrl Pts',(-7.12459150827332,-36.795222251874,19.7448191079696));
#33442=CARTESIAN_POINT('Ctrl Pts',(-7.11415703127194,-36.778400193081,19.7459697888211));
#33443=CARTESIAN_POINT('Ctrl Pts',(-7.09610551330263,-36.7487210102446,
19.7480055257937));
#33444=CARTESIAN_POINT('Ctrl Pts',(-7.08842521861717,-36.7359034080442,
19.7488865795069));
#33445=CARTESIAN_POINT('Ctrl Pts',(-7.07166225659191,-36.7075035553839,
19.750843221709));
#33446=CARTESIAN_POINT('Ctrl Pts',(-7.06261915196061,-36.6918995397369,
19.7519210767044));
#33447=CARTESIAN_POINT('Ctrl Pts',(-7.03607488908259,-36.6452427049893,
19.7551505023003));
#33448=CARTESIAN_POINT('Ctrl Pts',(-7.01893907605644,-36.6139861127826,
19.7573225634741));
#33449=CARTESIAN_POINT('Ctrl Pts',(-6.93476612076658,-36.4545354950783,
19.7684243122262));
#33450=CARTESIAN_POINT('Ctrl Pts',(-6.87549603906129,-36.322422248421,19.7776853448444));
#33451=CARTESIAN_POINT('Ctrl Pts',(-6.78140600123141,-36.0707245556632,
19.7949886816328));
#33452=CARTESIAN_POINT('Ctrl Pts',(-6.74437420746595,-35.9522083421974,
19.8030051329824));
#33453=CARTESIAN_POINT('Ctrl Pts',(-6.68806199929361,-35.7297773673681,
19.8176313335132));
#33454=CARTESIAN_POINT('Ctrl Pts',(-6.66697666990258,-35.6264716675134,
19.8242640758911));
#33455=CARTESIAN_POINT('Ctrl Pts',(-6.63933547000476,-35.4492367986342,
19.8353305846701));
#33456=CARTESIAN_POINT('Ctrl Pts',(-6.63032988216214,-35.3757716663386,
19.839828523691));
#33457=CARTESIAN_POINT('Ctrl Pts',(-6.62070214116034,-35.26816014551,19.8462890806219));
#33458=CARTESIAN_POINT('Ctrl Pts',(-6.61817949469435,-35.2342094769752,
19.8483089608516));
#33459=CARTESIAN_POINT('Ctrl Pts',(-6.6146012889051,-35.173737467794,19.8518752833638));
#33460=CARTESIAN_POINT('Ctrl Pts',(-6.61334499168027,-35.1472312970535,
19.8534277647332));
#33461=CARTESIAN_POINT('Ctrl Pts',(-6.61133929925244,-35.0909448175668,
19.8567027921618));
#33462=CARTESIAN_POINT('Ctrl Pts',(-6.61067095413299,-35.0611637572551,
19.8584227206753));
#33463=CARTESIAN_POINT('Ctrl Pts',(-6.60991982337146,-34.9800204922067,
19.8630762675357));
#33464=CARTESIAN_POINT('Ctrl Pts',(-6.61061163404398,-34.9286580179134,
19.8659861444027));
#33465=CARTESIAN_POINT('Ctrl Pts',(-6.62149561329613,-34.6280993142513,
19.8828396673708));
#33466=CARTESIAN_POINT('Ctrl Pts',(-6.65799596034638,-34.380627654014,19.895942516164));
#33467=CARTESIAN_POINT('Ctrl Pts',(-6.75149621644082,-34.0244203445412,
19.9154999551234));
#33468=CARTESIAN_POINT('Ctrl Pts',(-6.7876972036621,-33.9111289956048,19.9218440965742));
#33469=CARTESIAN_POINT('Ctrl Pts',(-6.85319494731223,-33.7380961440355,
19.9320338326522));
#33470=CARTESIAN_POINT('Ctrl Pts',(-6.87842514284344,-33.676915478525,19.9357387863629));
#33471=CARTESIAN_POINT('Ctrl Pts',(-6.91471662730229,-33.595738781596,19.9408425588553));
#33472=CARTESIAN_POINT('Ctrl Pts',(-6.92421440008435,-33.5750558108276,
19.9421597161659));
#33473=CARTESIAN_POINT('Ctrl Pts',(-6.94046996523299,-33.5405764884283,
19.9443862149576));
#33474=CARTESIAN_POINT('Ctrl Pts',(-6.94711477082101,-33.5267271840455,
19.9452889490864));
#33475=CARTESIAN_POINT('Ctrl Pts',(-6.96110150128007,-33.4980765853706,
19.9471748687212));
#33476=CARTESIAN_POINT('Ctrl Pts',(-6.96845781942039,-33.4832831473512,
19.9481588321655));
#33477=CARTESIAN_POINT('Ctrl Pts',(-6.98870892790336,-33.4432944357736,
19.9508451615955));
#33478=CARTESIAN_POINT('Ctrl Pts',(-7.00181133561802,-33.4182064757061,
19.9525593123731));
#33479=CARTESIAN_POINT('Ctrl Pts',(-7.08580668873753,-33.2621692315521,
19.9633885815555));
#33480=CARTESIAN_POINT('Ctrl Pts',(-7.16494440344835,-33.1358567381559,
19.972895562966));
#33481=CARTESIAN_POINT('Ctrl Pts',(-7.40016299556947,-32.8102107509234,
19.9987446931162));
#33482=CARTESIAN_POINT('Ctrl Pts',(-7.57069647243771,-32.6224281179145,
20.0150842408273));
#33483=CARTESIAN_POINT('Ctrl Pts',(-7.8087481616659,-32.4129276439528,20.0345333576256));
#33484=CARTESIAN_POINT('Ctrl Pts',(-7.85814783147684,-32.3718831614362,
20.038419588502));
#33485=CARTESIAN_POINT('Ctrl Pts',(-7.9341130578812,-32.3123318583815,20.0441781602691));
#33486=CARTESIAN_POINT('Ctrl Pts',(-7.95982411599474,-32.2927631489304,
20.0460914598109));
#33487=CARTESIAN_POINT('Ctrl Pts',(-8.00498997773149,-32.2593963042025,
20.0493921633121));
#33488=CARTESIAN_POINT('Ctrl Pts',(-8.02431756212809,-32.2454306045935,
20.0507859168318));
#33489=CARTESIAN_POINT('Ctrl Pts',(-8.06831482215952,-32.2143404470535,
20.0539175367482));
#33490=CARTESIAN_POINT('Ctrl Pts',(-8.09306810379204,-32.1973374091629,
20.0556507651515));
#33491=CARTESIAN_POINT('Ctrl Pts',(-8.16060552678165,-32.1522549975581,
20.0603054444828));
#33492=CARTESIAN_POINT('Ctrl Pts',(-8.20380571031646,-32.1248112957943,
20.0632036280528));
#33493=CARTESIAN_POINT('Ctrl Pts',(-8.45768393087942,-31.971486859662,20.0798180113542));
#33494=CARTESIAN_POINT('Ctrl Pts',(-8.68091048194822,-31.8678051342531,
20.0927250252142));
#33495=CARTESIAN_POINT('Ctrl Pts',(-9.08061482754219,-31.7325388330612,
20.1151269772694));
#33496=CARTESIAN_POINT('Ctrl Pts',(-9.25198638662764,-31.689103881127,20.1245512738168));
#33497=CARTESIAN_POINT('Ctrl Pts',(-9.45420982645986,-31.6543549080649,
20.1362299670203));
#33498=CARTESIAN_POINT('Ctrl Pts',(-9.4825418027632,-31.6498559891247,20.1378788917572));
#33499=CARTESIAN_POINT('Ctrl Pts',(-9.52735651853127,-31.6433217479596,
20.1405119133108));
#33500=CARTESIAN_POINT('Ctrl Pts',(-9.54380358260815,-31.6410469560046,
20.1414834893378));
#33501=CARTESIAN_POINT('Ctrl Pts',(-9.57528171350542,-31.6369286714489,
20.1433541519405));
#33502=CARTESIAN_POINT('Ctrl Pts',(-9.5903094631734,-31.6350649316252,20.1442521500799));
#33503=CARTESIAN_POINT('Ctrl Pts',(-9.6275844368058,-31.6306954826203,20.1464910671147));
#33504=CARTESIAN_POINT('Ctrl Pts',(-9.64984476244935,-31.6283093953852,
20.1478382400458));
#33505=CARTESIAN_POINT('Ctrl Pts',(-9.73035663857398,-31.6204851974397,
20.152743295928));
#33506=CARTESIAN_POINT('Ctrl Pts',(-9.78872015733889,-31.6163351474166,
20.1563603616714));
#33507=CARTESIAN_POINT('Ctrl Pts',(-10.0705548380071,-31.603614440014,20.1740333755053));
#33508=CARTESIAN_POINT('Ctrl Pts',(-10.2943960671935,-31.6156621029647,
20.1886517875108));
#33509=CARTESIAN_POINT('Ctrl Pts',(-10.6811901815642,-31.6751668178118,
20.2136564721994));
#33510=CARTESIAN_POINT('Ctrl Pts',(-10.8448576272418,-31.7129398609659,
20.2241628828816));
#33511=CARTESIAN_POINT('Ctrl Pts',(-11.0468404665663,-31.7756484944184,
20.2369381997889));
#33512=CARTESIAN_POINT('Ctrl Pts',(-11.0883529119116,-31.7894228242865,
20.2395544742172));
#33513=CARTESIAN_POINT('Ctrl Pts',(-11.156193277019,-31.8134001835384,20.2438162690791));
#33514=CARTESIAN_POINT('Ctrl Pts',(-11.1826799885321,-31.8231352876215,
20.2454767027279));
#33515=CARTESIAN_POINT('Ctrl Pts',(-11.2340599647061,-31.8427514893372,
20.2486918369664));
#33516=CARTESIAN_POINT('Ctrl Pts',(-11.258963708446,-31.8525990729377,20.2502474941414));
#33517=CARTESIAN_POINT('Ctrl Pts',(-11.3185582253842,-31.8769848125534,
20.2539650084044));
#33518=CARTESIAN_POINT('Ctrl Pts',(-11.353129221953,-31.8918074185857,20.2561172732135));
#33519=CARTESIAN_POINT('Ctrl Pts',(-11.4706727424195,-31.9445381461186,
20.263427379208));
#33520=CARTESIAN_POINT('Ctrl Pts',(-11.5523612280448,-31.9852194157938,
20.2684930426778));
#33521=CARTESIAN_POINT('Ctrl Pts',(-11.867082872848,-32.1581411203871,20.2881165580502));
#33522=CARTESIAN_POINT('Ctrl Pts',(-12.0857183711477,-32.3144963491286,
20.3019116597494));
#33523=CARTESIAN_POINT('Ctrl Pts',(-12.3324345241596,-32.5394087269167,
20.3199930828976));
#33524=CARTESIAN_POINT('Ctrl Pts',(-12.3798932094113,-32.5852810378745,
20.3236113222095));
#33525=CARTESIAN_POINT('Ctrl Pts',(-12.4573188271259,-32.6646193956947,
20.329815520593));
#33526=CARTESIAN_POINT('Ctrl Pts',(-12.4880150635659,-32.6973495638589,
20.3323606836019));
#33527=CARTESIAN_POINT('Ctrl Pts',(-12.5312525497046,-32.7453260885405,
20.336087794199));
#33528=CARTESIAN_POINT('Ctrl Pts',(-12.5443256021088,-32.7600890403227,
20.3372341936409));
#33529=CARTESIAN_POINT('Ctrl Pts',(-12.5670738128593,-32.7862339252988,
20.3392653421095));
#33530=CARTESIAN_POINT('Ctrl Pts',(-12.5768036963897,-32.7975670516342,
20.3401461561398));
#33531=CARTESIAN_POINT('Ctrl Pts',(-12.5981529378784,-32.8227692583367,
20.3421060354534));
#33532=CARTESIAN_POINT('Ctrl Pts',(-12.6097362277962,-32.8366671130018,
20.3431874207463));
#33533=CARTESIAN_POINT('Ctrl Pts',(-12.6432926523992,-32.8775904723364,
20.346371705913));
#33534=CARTESIAN_POINT('Ctrl Pts',(-12.664960536664,-32.9048619652437,20.348493789315));
#33535=CARTESIAN_POINT('Ctrl Pts',(-12.7979277733539,-33.0776166751844,
20.3619116875571));
#33536=CARTESIAN_POINT('Ctrl Pts',(-12.8976944995374,-33.2315785541648,
20.3737450059443));
#33537=CARTESIAN_POINT('Ctrl Pts',(-13.0591705866021,-33.5314413754368,
20.3956960454426));
#33538=CARTESIAN_POINT('Ctrl Pts',(-13.1240689965493,-33.6750897656337,
20.4057968251401));
#33539=CARTESIAN_POINT('Ctrl Pts',(-13.1787501237351,-33.8227350708723,
20.4156322019944));
#33540=CARTESIAN_POINT('Origin',(-10.,-35.,23.));
#33541=CARTESIAN_POINT('',(-13.1787500936073,-33.8227349895238,21.6644775413951));
#33542=CARTESIAN_POINT('',(-13.1787501333198,-33.8227350967521,21.3230163149173));
#33543=CARTESIAN_POINT('',(-13.1787501240207,-33.8227350716434,23.));
#33544=CARTESIAN_POINT('',(-13.3897498409715,-35.0010383320299,20.1438256239882));
#33545=CARTESIAN_POINT('Ctrl Pts',(-13.1787501333198,-33.8227350967521,
21.3230163149173));
#33546=CARTESIAN_POINT('Ctrl Pts',(-13.1402669858312,-33.7188261890181,
21.3160962228213));
#33547=CARTESIAN_POINT('Ctrl Pts',(-13.0967084745643,-33.6168571994136,
21.3090034474752));
#33548=CARTESIAN_POINT('Ctrl Pts',(-12.9319060910036,-33.2780694004307,
21.2847566361131));
#33549=CARTESIAN_POINT('Ctrl Pts',(-12.7878270355097,-33.0534180346275,
21.2675898966232));
#33550=CARTESIAN_POINT('Ctrl Pts',(-12.5843253798839,-32.8057708926119,
21.2480502979645));
#33551=CARTESIAN_POINT('Ctrl Pts',(-12.5486894025159,-32.7644772669941,
21.2447643123992));
#33552=CARTESIAN_POINT('Ctrl Pts',(-12.4914279145765,-32.7012748556937,
21.2396883190259));
#33553=CARTESIAN_POINT('Ctrl Pts',(-12.470475362046,-32.6787714628998,21.2378712795906));
#33554=CARTESIAN_POINT('Ctrl Pts',(-12.4309554134957,-32.6374677252693,
21.2345168297461));
#33555=CARTESIAN_POINT('Ctrl Pts',(-12.4124689287212,-32.6185935462785,
21.2329761820125));
#33556=CARTESIAN_POINT('Ctrl Pts',(-12.3706673022276,-32.5769016409987,
21.2295542213116));
#33557=CARTESIAN_POINT('Ctrl Pts',(-12.3472394637039,-32.554200310458,21.2276780149003));
#33558=CARTESIAN_POINT('Ctrl Pts',(-12.275504143539,-32.4866698058873,21.2220533878851));
#33559=CARTESIAN_POINT('Ctrl Pts',(-12.2262123506855,-32.442906508084,21.2183491001455));
#33560=CARTESIAN_POINT('Ctrl Pts',(-12.107161973885,-32.3432622192004,21.2097379492105));
#33561=CARTESIAN_POINT('Ctrl Pts',(-12.0364072414175,-32.2886471672074,
21.2048759668668));
#33562=CARTESIAN_POINT('Ctrl Pts',(-11.8490594979172,-32.1555105769936,
21.1925141486322));
#33563=CARTESIAN_POINT('Ctrl Pts',(-11.7295949226222,-32.0813284984821,
21.1851131518274));
#33564=CARTESIAN_POINT('Ctrl Pts',(-11.4575776911211,-31.9349995939614,
21.1687009623497));
#33565=CARTESIAN_POINT('Ctrl Pts',(-11.3035604610276,-31.8663953974293,
21.1596846456035));
#33566=CARTESIAN_POINT('Ctrl Pts',(-11.1180925343261,-31.7998284730845,
21.1484691655834));
#33567=CARTESIAN_POINT('Ctrl Pts',(-11.0909592120591,-31.7904772006969,
21.1468195383833));
#33568=CARTESIAN_POINT('Ctrl Pts',(-11.0479437416215,-31.7762607500315,
21.144185650614));
#33569=CARTESIAN_POINT('Ctrl Pts',(-11.0321383707925,-31.7711656599278,
21.1432139247373));
#33570=CARTESIAN_POINT('Ctrl Pts',(-11.0016828610239,-31.7615943488389,
21.141332802366));
#33571=CARTESIAN_POINT('Ctrl Pts',(-10.9870388245504,-31.7571009821792,
21.1404243639876));
#33572=CARTESIAN_POINT('Ctrl Pts',(-10.9507883214316,-31.7462461771116,
21.1381666232616));
#33573=CARTESIAN_POINT('Ctrl Pts',(-10.9291481272544,-31.7400006027872,
21.1368110558194));
#33574=CARTESIAN_POINT('Ctrl Pts',(-10.8455676430775,-31.7167782287938,
21.1315498580947));
#33575=CARTESIAN_POINT('Ctrl Pts',(-10.7832151156938,-31.7013483303259,
21.1275711494764));
#33576=CARTESIAN_POINT('Ctrl Pts',(-10.6098975805984,-31.6636496193188,
21.1164313952084));
#33577=CARTESIAN_POINT('Ctrl Pts',(-10.4981989458723,-31.6451521146798,
21.109164354599));
#33578=CARTESIAN_POINT('Ctrl Pts',(-10.1276219202218,-31.602700570786,21.0851320572966));
#33579=CARTESIAN_POINT('Ctrl Pts',(-9.86686416085046,-31.6029060269525,
21.0684276299297));
#33580=CARTESIAN_POINT('Ctrl Pts',(-9.55890117551041,-31.6386986539795,
21.049599996885));
#33581=CARTESIAN_POINT('Ctrl Pts',(-9.50927023819553,-31.6455850563841,
21.0465904952647));
#33582=CARTESIAN_POINT('Ctrl Pts',(-9.430657627776,-31.6582749635263,21.0418610150642));
#33583=CARTESIAN_POINT('Ctrl Pts',(-9.40156920191443,-31.6633613293175,
21.040119170246));
#33584=CARTESIAN_POINT('Ctrl Pts',(-9.34642253506713,-31.6737485909019,
21.0368314608407));
#33585=CARTESIAN_POINT('Ctrl Pts',(-9.32035310494966,-31.6789772514309,
21.0352834753672));
#33586=CARTESIAN_POINT('Ctrl Pts',(-9.26059311701581,-31.6916962833092,
21.0317480336775));
#33587=CARTESIAN_POINT('Ctrl Pts',(-9.22694974368161,-31.6993955937712,
21.0297672844043));
#33588=CARTESIAN_POINT('Ctrl Pts',(-9.11881987240803,-31.7258852755978,
21.0234273879753));
#33589=CARTESIAN_POINT('Ctrl Pts',(-9.04485035878773,-31.746694602652,21.0191314290186));
#33590=CARTESIAN_POINT('Ctrl Pts',(-8.86556078921875,-31.8037759822806,
21.008762965669));
#33591=CARTESIAN_POINT('Ctrl Pts',(-8.76119783629265,-31.8427588424619,
21.0027673901583));
#33592=CARTESIAN_POINT('Ctrl Pts',(-8.45706527544295,-31.9737693017101,
20.9851079822851));
#33593=CARTESIAN_POINT('Ctrl Pts',(-8.26414575489642,-32.0801514292994,
20.9736783224813));
#33594=CARTESIAN_POINT('Ctrl Pts',(-8.03157299617445,-32.2396425856585,
20.9581176603113));
#33595=CARTESIAN_POINT('Ctrl Pts',(-7.98123160821174,-32.2762431927009,
20.9546286238107));
#33596=CARTESIAN_POINT('Ctrl Pts',(-7.91377655284419,-32.3281838219972,
20.9497432595533));
#33597=CARTESIAN_POINT('Ctrl Pts',(-7.89576650758314,-32.3423447724907,
20.9484176227441));
#33598=CARTESIAN_POINT('Ctrl Pts',(-7.8660203626061,-32.3662254978074,20.9461898727932));
#33599=CARTESIAN_POINT('Ctrl Pts',(-7.85420339910283,-32.3758441050319,
20.9452946150572));
#33600=CARTESIAN_POINT('Ctrl Pts',(-7.82978833270833,-32.3959923286371,
20.943422612116));
#33601=CARTESIAN_POINT('Ctrl Pts',(-7.81720131000704,-32.4065342709862,
20.9424450650092));
#33602=CARTESIAN_POINT('Ctrl Pts',(-7.78349194359313,-32.4351859310051,
20.9397945169206));
#33603=CARTESIAN_POINT('Ctrl Pts',(-7.76251561109412,-32.4534645744628,
20.9381102320255));
#33604=CARTESIAN_POINT('Ctrl Pts',(-7.63914115920134,-32.5636734607895,
20.9280063637996));
#33605=CARTESIAN_POINT('Ctrl Pts',(-7.5422015101325,-32.6615045183677,20.9192503672406));
#33606=CARTESIAN_POINT('Ctrl Pts',(-7.26386237778455,-32.9788799457678,
20.8921258805095));
#33607=CARTESIAN_POINT('Ctrl Pts',(-7.10388848068874,-33.2156329374354,
20.8736960217714));
#33608=CARTESIAN_POINT('Ctrl Pts',(-6.95192399279683,-33.5159728107689,
20.8532167153632));
#33609=CARTESIAN_POINT('Ctrl Pts',(-6.92953703226849,-33.5628633835,20.8500909368474));
#33610=CARTESIAN_POINT('Ctrl Pts',(-6.89585595133953,-33.6377934887922,
20.845205852921));
#33611=CARTESIAN_POINT('Ctrl Pts',(-6.88384435354187,-33.665499745435,20.8434227181669));
#33612=CARTESIAN_POINT('Ctrl Pts',(-6.86302113163335,-33.715345884085,20.8402549143128));
#33613=CARTESIAN_POINT('Ctrl Pts',(-6.85406981794108,-33.7374248733243,
20.8388656687195));
#33614=CARTESIAN_POINT('Ctrl Pts',(-6.8336126228141,-33.7894525156608,20.835623627216));
#33615=CARTESIAN_POINT('Ctrl Pts',(-6.82229755519256,-33.8194740546552,
20.8337772126321));
#33616=CARTESIAN_POINT('Ctrl Pts',(-6.79003306443656,-33.9089063573563,
20.8283451548976));
#33617=CARTESIAN_POINT('Ctrl Pts',(-6.77031102225478,-33.9687469450605,
20.8247991167207));
#33618=CARTESIAN_POINT('Ctrl Pts',(-6.70769152097348,-34.1782149534663,
20.8126495899334));
#33619=CARTESIAN_POINT('Ctrl Pts',(-6.67343517303043,-34.3302255491785,
20.8043011876052));
#33620=CARTESIAN_POINT('Ctrl Pts',(-6.62018744111716,-34.6759896355574,
20.7857092651865));
#33621=CARTESIAN_POINT('Ctrl Pts',(-6.60717982923769,-34.8700901801265,
20.7755465852486));
#33622=CARTESIAN_POINT('Ctrl Pts',(-6.61207055170485,-35.1281897981063,
20.7613192373044));
#33623=CARTESIAN_POINT('Ctrl Pts',(-6.61509347986115,-35.192107749702,20.7577357147022));
#33624=CARTESIAN_POINT('Ctrl Pts',(-6.62167006993555,-35.2789760005041,
20.7527384990922));
#33625=CARTESIAN_POINT('Ctrl Pts',(-6.62365353953989,-35.3020351648611,
20.7513997481108));
#33626=CARTESIAN_POINT('Ctrl Pts',(-6.62733828003341,-35.3402814640963,
20.7491562971281));
#33627=CARTESIAN_POINT('Ctrl Pts',(-6.62890645244173,-35.3554811346509,
20.7482586673095));
#33628=CARTESIAN_POINT('Ctrl Pts',(-6.63236437584895,-35.3869139952379,
20.7463889541675));
#33629=CARTESIAN_POINT('Ctrl Pts',(-6.63426883061069,-35.403144896676,20.7454161534632));
#33630=CARTESIAN_POINT('Ctrl Pts',(-6.63968877441915,-35.4466184566698,
20.7427920121682));
#33631=CARTESIAN_POINT('Ctrl Pts',(-6.64341809397308,-35.4738326519488,
20.7411297518359));
#33632=CARTESIAN_POINT('Ctrl Pts',(-6.6664677706267,-35.6280740387228,20.7316086516929));
#33633=CARTESIAN_POINT('Ctrl Pts',(-6.69266619964882,-35.7539570652183,
20.7234557804387));
#33634=CARTESIAN_POINT('Ctrl Pts',(-6.8018451310795,-36.1610677375388,20.6964123240988));
#33635=CARTESIAN_POINT('Ctrl Pts',(-6.91414650493017,-36.4331215507197,
20.6773850848167));
#33636=CARTESIAN_POINT('Ctrl Pts',(-7.08628851226897,-36.7330512816328,
20.6563329025517));
#33637=CARTESIAN_POINT('Ctrl Pts',(-7.113579933122,-36.7781341461501,20.6531613022237));
#33638=CARTESIAN_POINT('Ctrl Pts',(-7.15823289906459,-36.8481575065837,
20.6482215381644));
#33639=CARTESIAN_POINT('Ctrl Pts',(-7.17489669645336,-36.8735308482042,
20.6464286460806));
#33640=CARTESIAN_POINT('Ctrl Pts',(-7.20657499486972,-36.9203823239639,
20.6431115129367));
#33641=CARTESIAN_POINT('Ctrl Pts',(-7.22150195426622,-36.9419166295661,
20.6415842007553));
#33642=CARTESIAN_POINT('Ctrl Pts',(-7.25580218730712,-36.9901944067439,
20.6381529187887));
#33643=CARTESIAN_POINT('Ctrl Pts',(-7.27531973466054,-37.0168324108284,
20.6362545656993));
#33644=CARTESIAN_POINT('Ctrl Pts',(-7.33627964198508,-37.0975315003419,
20.630483837977));
#33645=CARTESIAN_POINT('Ctrl Pts',(-7.37896590193656,-37.1506337805261,
20.6266591987111));
#33646=CARTESIAN_POINT('Ctrl Pts',(-7.58601327742642,-37.3928742705515,
20.6090082627623));
#33647=CARTESIAN_POINT('Ctrl Pts',(-7.76941000004373,-37.5646933635845,
20.5959518322867));
#33648=CARTESIAN_POINT('Ctrl Pts',(-8.08633919688312,-37.8016751161388,
20.5748438226631));
#33649=CARTESIAN_POINT('Ctrl Pts',(-8.20805936123526,-37.8810451562144,
20.5670006748164));
#33650=CARTESIAN_POINT('Ctrl Pts',(-8.35911326130663,-37.9662595784076,
20.5571243457608));
#33651=CARTESIAN_POINT('Ctrl Pts',(-8.383921828391,-37.9798483867735,20.5554977813112));
#33652=CARTESIAN_POINT('Ctrl Pts',(-8.42348200470763,-38.0008780247653,
20.5528923465613));
#33653=CARTESIAN_POINT('Ctrl Pts',(-8.43812348158442,-38.0085244930506,
20.5519255584112));
#33654=CARTESIAN_POINT('Ctrl Pts',(-8.46648955797091,-38.0230757213934,
20.5500466006328));
#33655=CARTESIAN_POINT('Ctrl Pts',(-8.48020614165381,-38.0299946678135,
20.5491352887193));
#33656=CARTESIAN_POINT('Ctrl Pts',(-8.51436810221523,-38.0469363956527,
20.5468596335747));
#33657=CARTESIAN_POINT('Ctrl Pts',(-8.53486816575161,-38.0568467709969,
20.5454888063523));
#33658=CARTESIAN_POINT('Ctrl Pts',(-8.61540468158909,-38.0947844405223,
20.5400874502244));
#33659=CARTESIAN_POINT('Ctrl Pts',(-8.67615454567597,-38.1212540694852,
20.5359789978298));
#33660=CARTESIAN_POINT('Ctrl Pts',(-8.84818660320149,-38.1902852711145,
20.5243247150522));
#33661=CARTESIAN_POINT('Ctrl Pts',(-8.96099324102022,-38.2287856282417,
20.5166624581554));
#33662=CARTESIAN_POINT('Ctrl Pts',(-9.31505042551913,-38.3291439555038,
20.4929438817597));
#33663=CARTESIAN_POINT('Ctrl Pts',(-9.56130054585836,-38.3704502663933,
20.4769745507221));
#33664=CARTESIAN_POINT('Ctrl Pts',(-9.86061079356185,-38.3872639936425,
20.4587511193313));
#33665=CARTESIAN_POINT('Ctrl Pts',(-9.91140033374375,-38.3889728872996,
20.455696094601));
#33666=CARTESIAN_POINT('Ctrl Pts',(-9.99215996494449,-38.3898732474655,
20.4508955534453));
#33667=CARTESIAN_POINT('Ctrl Pts',(-10.0221124866583,-38.389810204744,20.4491275693709));
#33668=CARTESIAN_POINT('Ctrl Pts',(-10.0785643457313,-38.3889430948752,
20.4458178786924));
#33669=CARTESIAN_POINT('Ctrl Pts',(-10.1050625594161,-38.3882251362819,
20.4442736520243));
#33670=CARTESIAN_POINT('Ctrl Pts',(-10.1652907692601,-38.3858860240237,
20.4407837667086));
#33671=CARTESIAN_POINT('Ctrl Pts',(-10.1990107043103,-38.384071521527,20.4388441839593));
#33672=CARTESIAN_POINT('Ctrl Pts',(-10.3048986162235,-38.3767853637381,
20.4327940403518));
#33673=CARTESIAN_POINT('Ctrl Pts',(-10.3769239266166,-38.3695061849631,
20.4287385149376));
#33674=CARTESIAN_POINT('Ctrl Pts',(-10.5498090115357,-38.3464201319128,
20.4191023404541));
#33675=CARTESIAN_POINT('Ctrl Pts',(-10.6502960138072,-38.3283531406261,
20.4135840059501));
#33676=CARTESIAN_POINT('Ctrl Pts',(-10.7967287142194,-38.295139165467,20.4055517842023));
#33677=CARTESIAN_POINT('Ctrl Pts',(-10.843406787834,-38.2835017663891,20.4029923955733));
#33678=CARTESIAN_POINT('Ctrl Pts',(-11.0919051537793,-38.2158992789203,
20.3893191280384));
#33679=CARTESIAN_POINT('Ctrl Pts',(-11.2884395632971,-38.142319548116,20.3783583074076));
#33680=CARTESIAN_POINT('Ctrl Pts',(-11.5181487604185,-38.0311266306934,
20.3641016456152));
#33681=CARTESIAN_POINT('Ctrl Pts',(-11.5589778005654,-38.0103308972074,
20.3615073647234));
#33682=CARTESIAN_POINT('Ctrl Pts',(-11.6156935357303,-37.9799802336969,
20.3578010037077));
#33683=CARTESIAN_POINT('Ctrl Pts',(-11.6319440950488,-37.9711119521423,
20.3567269650976));
#33684=CARTESIAN_POINT('Ctrl Pts',(-11.661296218146,-37.9547804098513,20.354763543297));
#33685=CARTESIAN_POINT('Ctrl Pts',(-11.6744223805344,-37.9473618849605,
20.3538768664203));
#33686=CARTESIAN_POINT('Ctrl Pts',(-11.702029753591,-37.9315150528478,20.3519928890465));
#33687=CARTESIAN_POINT('Ctrl Pts',(-11.7164984827113,-37.9230666635997,
20.3509944281097));
#33688=CARTESIAN_POINT('Ctrl Pts',(-11.7561780687489,-37.8995012946895,
20.3482268092283));
#33689=CARTESIAN_POINT('Ctrl Pts',(-11.7812552597969,-37.8841634384853,
20.346444696278));
#33690=CARTESIAN_POINT('Ctrl Pts',(-11.8376694057658,-37.8486427316393,
20.3423657172438));
#33691=CARTESIAN_POINT('Ctrl Pts',(-11.8688790736459,-37.8282653787377,
20.3400591758521));
#33692=CARTESIAN_POINT('Ctrl Pts',(-11.9712615007684,-37.7589834744033,
20.3323409508029));
#33693=CARTESIAN_POINT('Ctrl Pts',(-12.0408989220013,-37.7078758753492,
20.3268437335704));
#33694=CARTESIAN_POINT('Ctrl Pts',(-12.3326375227201,-37.4761150116692,
20.3029432463605));
#33695=CARTESIAN_POINT('Ctrl Pts',(-12.533357563899,-37.2703509316107,20.2843462311002));
#33696=CARTESIAN_POINT('Ctrl Pts',(-12.737328507536,-37.0000430749118,20.2636622936412));
#33697=CARTESIAN_POINT('Ctrl Pts',(-12.7678580124946,-36.9575755757717,
20.2605031129089));
#33698=CARTESIAN_POINT('Ctrl Pts',(-12.8159836261468,-36.8872532201749,
20.2554151089511));
#33699=CARTESIAN_POINT('Ctrl Pts',(-12.8341770862056,-36.8598195768509,
20.2534644572795));
#33700=CARTESIAN_POINT('Ctrl Pts',(-12.8662568969194,-36.8098826812721,
20.2499736942696));
#33701=CARTESIAN_POINT('Ctrl Pts',(-12.8802848339037,-36.7874739867632,
20.2484284903702));
#33702=CARTESIAN_POINT('Ctrl Pts',(-12.9099403627754,-36.7388454965389,
20.2451196653981));
#33703=CARTESIAN_POINT('Ctrl Pts',(-12.925478940079,-36.7125739792878,20.2433593357253));
#33704=CARTESIAN_POINT('Ctrl Pts',(-12.9680067176365,-36.6384027527018,
20.238462512425));
#33705=CARTESIAN_POINT('Ctrl Pts',(-12.9941891622714,-36.5900500584078,
20.2353543111342));
#33706=CARTESIAN_POINT('Ctrl Pts',(-13.0509083310789,-36.4789294992827,
20.2283823441658));
#33707=CARTESIAN_POINT('Ctrl Pts',(-13.0807062230327,-36.4158121555035,
20.2245422924027));
#33708=CARTESIAN_POINT('Ctrl Pts',(-13.2089862089231,-36.1208292940687,
20.2070443581614));
#33709=CARTESIAN_POINT('Ctrl Pts',(-13.2833725401939,-35.8793792505666,
20.1940356182472));
#33710=CARTESIAN_POINT('Ctrl Pts',(-13.3487487639202,-35.534838357255,20.1750619076463));
#33711=CARTESIAN_POINT('Ctrl Pts',(-13.3629151346599,-35.4369998758927,
20.1696206628712));
#33712=CARTESIAN_POINT('Ctrl Pts',(-13.3754286172593,-35.3123869531831,
20.1624712441341));
#33713=CARTESIAN_POINT('Ctrl Pts',(-13.3777621711456,-35.2860534602704,
20.1609480529267));
#33714=CARTESIAN_POINT('Ctrl Pts',(-13.381022401637,-35.2436235590546,20.1584701245838));
#33715=CARTESIAN_POINT('Ctrl Pts',(-13.3821427005456,-35.2275426304932,
20.1575255239153));
#33716=CARTESIAN_POINT('Ctrl Pts',(-13.3840196643209,-35.1975123351502,
20.1557503303104));
#33717=CARTESIAN_POINT('Ctrl Pts',(-13.3848048732879,-35.1835651354541,
20.154921322793));
#33718=CARTESIAN_POINT('Ctrl Pts',(-13.3862870557921,-35.1539806745553,
20.1531537799897));
#33719=CARTESIAN_POINT('Ctrl Pts',(-13.3869619695638,-35.1383425771513,
20.1522141047543));
#33720=CARTESIAN_POINT('Ctrl Pts',(-13.3889969388095,-35.0821610184463,
20.1488202887959));
#33721=CARTESIAN_POINT('Ctrl Pts',(-13.3897374162124,-35.0416003335705,
20.1463365969691));
#33722=CARTESIAN_POINT('Ctrl Pts',(-13.3897498409715,-35.0010383320299,
20.1438256239882));
#33723=CARTESIAN_POINT('Ctrl Pts',(-13.3897498397764,-35.0010422262792,
20.1438258650599));
#33724=CARTESIAN_POINT('Ctrl Pts',(-13.389821234382,-34.7688375145137,20.1294513438218));
#33725=CARTESIAN_POINT('Ctrl Pts',(-13.3660333076597,-34.5372390899468,
20.1142711274129));
#33726=CARTESIAN_POINT('Ctrl Pts',(-13.2845988396862,-34.1456188175152,
20.0886397868102));
#33727=CARTESIAN_POINT('Ctrl Pts',(-13.2382874513302,-33.9840947286066,
20.0780693460874));
#33728=CARTESIAN_POINT('Ctrl Pts',(-13.17971517951,-33.8253432955754,20.0677787655689));
#33729=CARTESIAN_POINT('Ctrl Pts',(-13.1792330523841,-33.8240390335285,
20.0676942263837));
#33730=CARTESIAN_POINT('Ctrl Pts',(-13.1787501240278,-33.8227350716626,
20.0676097122989));
#33731=CARTESIAN_POINT('Ctrl Pts',(-13.1787501237351,-33.8227350708723,
20.4156322019944));
#33732=CARTESIAN_POINT('Ctrl Pts',(-13.1797424235209,-33.8254143939277,
20.4158106848247));
#33733=CARTESIAN_POINT('Ctrl Pts',(-13.1807313585004,-33.8280950329722,
20.4159890846477));
#33734=CARTESIAN_POINT('Ctrl Pts',(-13.2150215335141,-33.921406256347,20.4221931120437));
#33735=CARTESIAN_POINT('Ctrl Pts',(-13.244440856324,-34.0134229941018,20.4281139314852));
#33736=CARTESIAN_POINT('Ctrl Pts',(-13.2797552385806,-34.1426723325319,
20.4361575738012));
#33737=CARTESIAN_POINT('Ctrl Pts',(-13.2890192513423,-34.1789289390912,
20.4383850332551));
#33738=CARTESIAN_POINT('Ctrl Pts',(-13.3039345352182,-34.2416126379442,
20.4421878980678));
#33739=CARTESIAN_POINT('Ctrl Pts',(-13.3098734955927,-34.2679670021105,
20.4437722436665));
#33740=CARTESIAN_POINT('Ctrl Pts',(-13.32139648777,-34.3221108660603,20.4469985481911));
#33741=CARTESIAN_POINT('Ctrl Pts',(-13.3269482992382,-34.3499050900237,
20.4486393834504));
#33742=CARTESIAN_POINT('Ctrl Pts',(-13.3402905217088,-34.4213546115755,
20.4528199944899));
#33743=CARTESIAN_POINT('Ctrl Pts',(-13.3475742324,-34.4650997574206,20.4553439052827));
#33744=CARTESIAN_POINT('Ctrl Pts',(-13.3779360975941,-34.6724903830181,
20.4671585580073));
#33745=CARTESIAN_POINT('Ctrl Pts',(-13.3898865545848,-34.8375436181589,
20.4761050069103));
#33746=CARTESIAN_POINT('Ctrl Pts',(-13.3895661459623,-35.2220415882748,
20.4966099349805));
#33747=CARTESIAN_POINT('Ctrl Pts',(-13.3681189732072,-35.4407059894748,
20.5080097651198));
#33748=CARTESIAN_POINT('Ctrl Pts',(-13.3135660392957,-35.7173776565305,
20.5235638768887));
#33749=CARTESIAN_POINT('Ctrl Pts',(-13.299704827826,-35.7786511828263,20.5270843393847));
#33750=CARTESIAN_POINT('Ctrl Pts',(-13.2784570121082,-35.8617732784254,
20.5320069342596));
#33751=CARTESIAN_POINT('Ctrl Pts',(-13.272537286335,-35.8839871102126,20.5333369757181));
#33752=CARTESIAN_POINT('Ctrl Pts',(-13.2623153201382,-35.9208346303501,
20.5355699921975));
#33753=CARTESIAN_POINT('Ctrl Pts',(-13.2581393019259,-35.9355030442002,
20.5364660398317));
#33754=CARTESIAN_POINT('Ctrl Pts',(-13.2492696351486,-35.9658781587236,
20.5383372406426));
#33755=CARTESIAN_POINT('Ctrl Pts',(-13.2445608352887,-35.9815797170145,
20.5393131670107));
#33756=CARTESIAN_POINT('Ctrl Pts',(-13.2315887423729,-36.0237219589988,
20.5419546928587));
#33757=CARTESIAN_POINT('Ctrl Pts',(-13.2231150762426,-36.0500959705038,
20.5436314513064));
#33758=CARTESIAN_POINT('Ctrl Pts',(-13.1716747087254,-36.2037113325952,
20.5535243483592));
#33759=CARTESIAN_POINT('Ctrl Pts',(-13.1215031014286,-36.3284025082254,
20.5620612116359));
#33760=CARTESIAN_POINT('Ctrl Pts',(-12.9399339258703,-36.7121453464489,
20.5893258653224));
#33761=CARTESIAN_POINT('Ctrl Pts',(-12.7825810609813,-36.9575371546396,
20.6081403924394));
#33762=CARTESIAN_POINT('Ctrl Pts',(-12.5628266413932,-37.2192258679611,
20.6289125791546));
#33763=CARTESIAN_POINT('Ctrl Pts',(-12.5289008953034,-37.257809677729,20.6320007408338));
#33764=CARTESIAN_POINT('Ctrl Pts',(-12.4739362530422,-37.3175270977966,
20.6368235108994));
#33765=CARTESIAN_POINT('Ctrl Pts',(-12.4534741776545,-37.3391786972222,
20.6385814941019));
#33766=CARTESIAN_POINT('Ctrl Pts',(-12.4142509870333,-37.3796010786396,
20.6418825939049));
#33767=CARTESIAN_POINT('Ctrl Pts',(-12.3955497982724,-37.3984266394473,
20.6434280795951));
#33768=CARTESIAN_POINT('Ctrl Pts',(-12.3523587219765,-37.4408957534412,
20.6469344879373));
#33769=CARTESIAN_POINT('Ctrl Pts',(-12.3277296834012,-37.4643940993537,
20.6488891045618));
#33770=CARTESIAN_POINT('Ctrl Pts',(-12.2484683858948,-37.5377680256003,
20.6550437536267));
#33771=CARTESIAN_POINT('Ctrl Pts',(-12.1925539232534,-37.5862298832706,
20.6591858792891));
#33772=CARTESIAN_POINT('Ctrl Pts',(-12.0532865343691,-37.6991690574091,
20.6690827226406));
#33773=CARTESIAN_POINT('Ctrl Pts',(-11.9684264437239,-37.7616658990211,
20.6747701365353));
#33774=CARTESIAN_POINT('Ctrl Pts',(-11.7775230978549,-37.8889832016795,
20.6870305484804));
#33775=CARTESIAN_POINT('Ctrl Pts',(-11.6705517284192,-37.9521296165816,
20.6935702853099));
#33776=CARTESIAN_POINT('Ctrl Pts',(-11.4319126876795,-38.0758681851275,
20.7078772969879));
#33777=CARTESIAN_POINT('Ctrl Pts',(-11.2993461803352,-38.1341714628078,
20.7156537544188));
#33778=CARTESIAN_POINT('Ctrl Pts',(-11.1299937593077,-38.1960584916601,
20.725834478796));
#33779=CARTESIAN_POINT('Ctrl Pts',(-11.0963226753759,-38.2077643552676,
20.7278705781836));
#33780=CARTESIAN_POINT('Ctrl Pts',(-11.04534786445,-38.2245896156921,20.7309796358504));
#33781=CARTESIAN_POINT('Ctrl Pts',(-11.0281766202933,-38.2301057495256,
20.7320314441309));
#33782=CARTESIAN_POINT('Ctrl Pts',(-10.9966993173681,-38.2399411779736,
20.7339691389511));
#33783=CARTESIAN_POINT('Ctrl Pts',(-10.9824075572206,-38.2443032735718,
20.7348526163829));
#33784=CARTESIAN_POINT('Ctrl Pts',(-10.9491168111755,-38.2542240528466,
20.736918975448));
#33785=CARTESIAN_POINT('Ctrl Pts',(-10.9300975247785,-38.2597109473222,
20.7381057197938));
#33786=CARTESIAN_POINT('Ctrl Pts',(-10.8673802098969,-38.2772107722701,
20.7420369952975));
#33787=CARTESIAN_POINT('Ctrl Pts',(-10.8234909448036,-38.2885135117182,
20.7448165165827));
#33788=CARTESIAN_POINT('Ctrl Pts',(-10.7142562356151,-38.314320803047,20.7517828237837));
#33789=CARTESIAN_POINT('Ctrl Pts',(-10.6486835175387,-38.327776005892,20.7560069176683));
#33790=CARTESIAN_POINT('Ctrl Pts',(-10.3067826126751,-38.3874433044256,
20.7781167557791));
#33791=CARTESIAN_POINT('Ctrl Pts',(-10.0258504827591,-38.4012138276423,
20.7964513705028));
#33792=CARTESIAN_POINT('Ctrl Pts',(-9.66575347564894,-38.3742004447113,
20.8188363146694));
#33793=CARTESIAN_POINT('Ctrl Pts',(-9.58532116182324,-38.3652626159723,
20.8237735646167));
#33794=CARTESIAN_POINT('Ctrl Pts',(-9.47304950182729,-38.3486996992343,
20.8305771750314));
#33795=CARTESIAN_POINT('Ctrl Pts',(-9.44088800875054,-38.3434802819212,
20.8325160494675));
#33796=CARTESIAN_POINT('Ctrl Pts',(-9.38225346324154,-38.33309487243,20.8360333705681));
#33797=CARTESIAN_POINT('Ctrl Pts',(-9.35575754640354,-38.3280751097144,
20.8376162176144));
#33798=CARTESIAN_POINT('Ctrl Pts',(-9.30195380167332,-38.3172151275187,
20.8408179705861));
#33799=CARTESIAN_POINT('Ctrl Pts',(-9.2746525696217,-38.3113525741656,20.8424360414151));
#33800=CARTESIAN_POINT('Ctrl Pts',(-9.20621416126245,-38.2957693488341,
20.8464773583752));
#33801=CARTESIAN_POINT('Ctrl Pts',(-9.16517995368286,-38.2856152044868,
20.8488868384231));
#33802=CARTESIAN_POINT('Ctrl Pts',(-8.98473369464489,-38.2373638059727,
20.8594356288459));
#33803=CARTESIAN_POINT('Ctrl Pts',(-8.84764516355096,-38.1911400024787,
20.8673170334236));
#33804=CARTESIAN_POINT('Ctrl Pts',(-8.59149612605775,-38.0861024177645,
20.8821582104425));
#33805=CARTESIAN_POINT('Ctrl Pts',(-8.47212062560268,-38.0287780253845,
20.8891284860037));
#33806=CARTESIAN_POINT('Ctrl Pts',(-8.224351938089,-37.8914141523077,20.9041912290463));
#33807=CARTESIAN_POINT('Ctrl Pts',(-8.09735267827896,-37.8094708373664,
20.912286788813));
#33808=CARTESIAN_POINT('Ctrl Pts',(-7.94737564428935,-37.6978572712773,
20.9228388833352));
#33809=CARTESIAN_POINT('Ctrl Pts',(-7.91884593000181,-37.6759107089597,
20.9248941885139));
#33810=CARTESIAN_POINT('Ctrl Pts',(-7.8765007992569,-37.6422497880646,20.9280267388225));
#33811=CARTESIAN_POINT('Ctrl Pts',(-7.862420122644,-37.6308715350572,20.9290823542122));
#33812=CARTESIAN_POINT('Ctrl Pts',(-7.83699970722492,-37.6099911226178,
20.9310150389804));
#33813=CARTESIAN_POINT('Ctrl Pts',(-7.82563006605457,-37.6005267335806,
20.9318895306533));
#33814=CARTESIAN_POINT('Ctrl Pts',(-7.799327871552,-37.5783390183394,20.9339359794902));
#33815=CARTESIAN_POINT('Ctrl Pts',(-7.78444349625642,-37.5655602211776,
20.9351117428707));
#33816=CARTESIAN_POINT('Ctrl Pts',(-7.73633303353773,-37.5235246861547,
20.9389677481076));
#33817=CARTESIAN_POINT('Ctrl Pts',(-7.70357027040226,-37.4937471961838,
20.9416812438432));
#33818=CARTESIAN_POINT('Ctrl Pts',(-7.62434280108415,-37.4188533207945,
20.9484424817542));
#33819=CARTESIAN_POINT('Ctrl Pts',(-7.57857052049581,-37.3730311736921,
20.9525249925178));
#33820=CARTESIAN_POINT('Ctrl Pts',(-7.3604677212843,-37.1418070952463,20.9727533046572));
#33821=CARTESIAN_POINT('Ctrl Pts',(-7.20794170573196,-36.9387879661309,
20.9893089686952));
#33822=CARTESIAN_POINT('Ctrl Pts',(-7.02672877305157,-36.6312102281304,
21.0116773367356));
#33823=CARTESIAN_POINT('Ctrl Pts',(-6.97815184977662,-36.5393588630552,
21.018067453703));
#33824=CARTESIAN_POINT('Ctrl Pts',(-6.91707256867729,-36.4097923364397,
21.0266843595967));
#33825=CARTESIAN_POINT('Ctrl Pts',(-6.90090148345945,-36.3738793832178,
21.0290326290667));
#33826=CARTESIAN_POINT('Ctrl Pts',(-6.87466876944409,-36.3127999263316,
21.0329607685183));
#33827=CARTESIAN_POINT('Ctrl Pts',(-6.8642767216079,-36.287780467368,21.0345515520571));
#33828=CARTESIAN_POINT('Ctrl Pts',(-6.8438458292439,-36.2368776995388,21.0377521993739));
#33829=CARTESIAN_POINT('Ctrl Pts',(-6.83382277271924,-36.2109902664664,
21.0393614437692));
#33830=CARTESIAN_POINT('Ctrl Pts',(-6.8096313074882,-36.1461544965799,21.043347608061));
#33831=CARTESIAN_POINT('Ctrl Pts',(-6.79585684569702,-36.1070634046308,
21.0457115686704));
#33832=CARTESIAN_POINT('Ctrl Pts',(-6.74055254072495,-35.9404246774226,
21.0556351117259));
#33833=CARTESIAN_POINT('Ctrl Pts',(-6.70589367841861,-35.8107188038258,
21.0629756613967));
#33834=CARTESIAN_POINT('Ctrl Pts',(-6.65116097682716,-35.5431351969952,
21.0776617444635));
#33835=CARTESIAN_POINT('Ctrl Pts',(-6.63171047904686,-35.4053950531635,
21.0849841031622));
#33836=CARTESIAN_POINT('Ctrl Pts',(-6.60843292257013,-35.1106220637268,
21.1006946879956));
#33837=CARTESIAN_POINT('Ctrl Pts',(-6.60694605196937,-34.9537408978524,
21.1090814540416));
#33838=CARTESIAN_POINT('Ctrl Pts',(-6.6184568825366,-34.7615546718182,21.1199501502817));
#33839=CARTESIAN_POINT('Ctrl Pts',(-6.62116740510742,-34.7258100813717,
21.1219972994564));
#33840=CARTESIAN_POINT('Ctrl Pts',(-6.62609648201241,-34.6721176903392,
21.125119874907));
#33841=CARTESIAN_POINT('Ctrl Pts',(-6.62789272521778,-34.6541326075708,
21.1261738757734));
#33842=CARTESIAN_POINT('Ctrl Pts',(-6.63143618344756,-34.6213100703901,
21.1281135060378));
#33843=CARTESIAN_POINT('Ctrl Pts',(-6.63313777459847,-34.6064685807681,
21.1289966895752));
#33844=CARTESIAN_POINT('Ctrl Pts',(-6.63731579869345,-34.5720399584068,
21.1310595589739));
#33845=CARTESIAN_POINT('Ctrl Pts',(-6.6398652989797,-34.5524627562589,21.1322430611186));
#33846=CARTESIAN_POINT('Ctrl Pts',(-6.6487874216445,-34.4883311560712,21.1361519951363));
#33847=CARTESIAN_POINT('Ctrl Pts',(-6.65587616557099,-34.4438830000727,
21.1389118971841));
#33848=CARTESIAN_POINT('Ctrl Pts',(-6.67558698498592,-34.3343603925951,
21.1458170409067));
#33849=CARTESIAN_POINT('Ctrl Pts',(-6.68923674053706,-34.2694907689832,
21.1499988242277));
#33850=CARTESIAN_POINT('Ctrl Pts',(-6.76844148015486,-33.9411649947635,
21.1715082441051));
#33851=CARTESIAN_POINT('Ctrl Pts',(-6.86358870626935,-33.6858247758495,
21.1892732232653));
#33852=CARTESIAN_POINT('Ctrl Pts',(-7.02872066587874,-33.3660755931273,
21.2116608912612));
#33853=CARTESIAN_POINT('Ctrl Pts',(-7.07231429488231,-33.2891907265559,
21.2170667399001));
#33854=CARTESIAN_POINT('Ctrl Pts',(-7.13841167655764,-33.1825584685678,
21.2245956565906));
#33855=CARTESIAN_POINT('Ctrl Pts',(-7.15847479032698,-33.1513474907533,
21.2268035569805));
#33856=CARTESIAN_POINT('Ctrl Pts',(-7.19399589927461,-33.098034455884,21.2305837155766));
#33857=CARTESIAN_POINT('Ctrl Pts',(-7.20921239205201,-33.0757763814661,
21.2321646340288));
#33858=CARTESIAN_POINT('Ctrl Pts',(-7.24102482853563,-33.03041371838,21.2353931999895));
#33859=CARTESIAN_POINT('Ctrl Pts',(-7.25764932291308,-33.007331700204,21.2370396057097));
#33860=CARTESIAN_POINT('Ctrl Pts',(-7.30122555589158,-32.9484073644773,
21.2412538616494));
#33861=CARTESIAN_POINT('Ctrl Pts',(-7.32860195801543,-32.9128850994988,
21.2438053259418));
#33862=CARTESIAN_POINT('Ctrl Pts',(-7.47836403436166,-32.7263375614643,
21.2572837640717));
#33863=CARTESIAN_POINT('Ctrl Pts',(-7.61286865388196,-32.5855013357581,
21.2677155456504));
#33864=CARTESIAN_POINT('Ctrl Pts',(-7.91274481328573,-32.3212085415871,
21.2889430882737));
#33865=CARTESIAN_POINT('Ctrl Pts',(-8.07877354977005,-32.1997442559754,
21.2996877185417));
#33866=CARTESIAN_POINT('Ctrl Pts',(-8.29808102172875,-32.0680328262602,
21.3139243093506));
#33867=CARTESIAN_POINT('Ctrl Pts',(-8.34198504788414,-32.0429836677071,
21.3167776545881));
#33868=CARTESIAN_POINT('Ctrl Pts',(-8.40512137217996,-32.0088097791362,
21.3209087969181));
#33869=CARTESIAN_POINT('Ctrl Pts',(-8.42390673970332,-31.998869086536,21.3221413959815));
#33870=CARTESIAN_POINT('Ctrl Pts',(-8.4562049603431,-31.9821646421291,21.3242685907873));
#33871=CARTESIAN_POINT('Ctrl Pts',(-8.46967166931177,-31.9753134764087,
21.3251578984764));
#33872=CARTESIAN_POINT('Ctrl Pts',(-8.49852202645079,-31.9608779061521,
21.3270688328802));
#33873=CARTESIAN_POINT('Ctrl Pts',(-8.5139174609892,-31.9533201898323,21.3280918680074));
#33874=CARTESIAN_POINT('Ctrl Pts',(-8.55754828394438,-31.9323109212226,
21.3309990539693));
#33875=CARTESIAN_POINT('Ctrl Pts',(-8.58591273040245,-31.9191331933119,
21.3328982757617));
#33876=CARTESIAN_POINT('Ctrl Pts',(-8.76875066305002,-31.8372459939738,
21.3451809033527));
#33877=CARTESIAN_POINT('Ctrl Pts',(-8.9279881005379,-31.7797874663349,21.3560484720248));
#33878=CARTESIAN_POINT('Ctrl Pts',(-9.33064306543395,-31.667683375062,21.3829872596265));
#33879=CARTESIAN_POINT('Ctrl Pts',(-9.57711889399226,-31.6275259536363,
21.3989589344847));
#33880=CARTESIAN_POINT('Ctrl Pts',(-9.8765360968515,-31.6121182134518,21.4171842130132));
#33881=CARTESIAN_POINT('Ctrl Pts',(-9.92732938377889,-31.6106481836983,
21.4202390070607));
#33882=CARTESIAN_POINT('Ctrl Pts',(-10.008087806878,-31.610127341894,21.4250392711657));
#33883=CARTESIAN_POINT('Ctrl Pts',(-10.0380388796514,-31.6103311104707,
21.4268072045195));
#33884=CARTESIAN_POINT('Ctrl Pts',(-10.0944853168803,-31.6114634151667,
21.4301168491632));
#33885=CARTESIAN_POINT('Ctrl Pts',(-10.1209799618856,-31.6123058624658,
21.4316610797822));
#33886=CARTESIAN_POINT('Ctrl Pts',(-10.1811978643435,-31.6149279735065,
21.4351510392527));
#33887=CARTESIAN_POINT('Ctrl Pts',(-10.214910150706,-31.6169009717589,21.4370906911254));
#33888=CARTESIAN_POINT('Ctrl Pts',(-10.3207713096603,-31.624685288591,21.4431413193169));
#33889=CARTESIAN_POINT('Ctrl Pts',(-10.3927689855877,-31.6323038770644,
21.4471972469665));
#33890=CARTESIAN_POINT('Ctrl Pts',(-10.5655658827432,-31.6562063501155,
21.4568346261945));
#33891=CARTESIAN_POINT('Ctrl Pts',(-10.6659815489268,-31.6747494525009,
21.4623537406012));
#33892=CARTESIAN_POINT('Ctrl Pts',(-10.8123115190576,-31.7086670178691,
21.4703889722032));
#33893=CARTESIAN_POINT('Ctrl Pts',(-10.8589746217431,-31.720535790954,21.4729505707608));
#33894=CARTESIAN_POINT('Ctrl Pts',(-11.1073057613315,-31.7893630352085,
21.486632408585));
#33895=CARTESIAN_POINT('Ctrl Pts',(-11.3035978550968,-31.863930491877,21.4975995931196));
#33896=CARTESIAN_POINT('Ctrl Pts',(-11.5327556708386,-31.9762353780533,
21.5118573801948));
#33897=CARTESIAN_POINT('Ctrl Pts',(-11.5733689209364,-31.9971676269638,
21.5144445463399));
#33898=CARTESIAN_POINT('Ctrl Pts',(-11.6298068361418,-32.0277152434651,
21.5181423536427));
#33899=CARTESIAN_POINT('Ctrl Pts',(-11.6459963162013,-32.0366500221665,
21.5192151827082));
#33900=CARTESIAN_POINT('Ctrl Pts',(-11.675378410593,-32.0531807032142,21.5211858768225));
#33901=CARTESIAN_POINT('Ctrl Pts',(-11.6885946907965,-32.060733977467,21.5220811588593));
#33902=CARTESIAN_POINT('Ctrl Pts',(-11.7163085137288,-32.0768213978027,
21.5239779974719));
#33903=CARTESIAN_POINT('Ctrl Pts',(-11.7307939268888,-32.0853747392143,
21.5249806542448));
#33904=CARTESIAN_POINT('Ctrl Pts',(-11.7706878609703,-32.1093335582906,
21.5277719296868));
#33905=CARTESIAN_POINT('Ctrl Pts',(-11.7959578097172,-32.1249654970002,
21.5295738524112));
#33906=CARTESIAN_POINT('Ctrl Pts',(-11.9731265290204,-32.2378088681751,
21.5424306498272));
#33907=CARTESIAN_POINT('Ctrl Pts',(-12.1172483973595,-32.3466669134747,
21.5540478761972));
#33908=CARTESIAN_POINT('Ctrl Pts',(-12.4303626577193,-32.6249880504184,
21.5810525332624));
#33909=CARTESIAN_POINT('Ctrl Pts',(-12.5914987687936,-32.8019301407458,
21.5963332882119));
#33910=CARTESIAN_POINT('Ctrl Pts',(-12.7633592544891,-33.036092859493,21.6140032734572));
#33911=CARTESIAN_POINT('Ctrl Pts',(-12.7930338605456,-33.0785297499357,
21.6171180454524));
#33912=CARTESIAN_POINT('Ctrl Pts',(-12.8384373410203,-33.1467358479106,
21.6219899861644));
#33913=CARTESIAN_POINT('Ctrl Pts',(-12.8548133696525,-33.1720625643064,
21.6237707702938));
#33914=CARTESIAN_POINT('Ctrl Pts',(-12.8835193579078,-33.2177853828403,
21.6269364457863));
#33915=CARTESIAN_POINT('Ctrl Pts',(-12.8959761784949,-33.2380990818352,
21.628325879629));
#33916=CARTESIAN_POINT('Ctrl Pts',(-12.9247252436309,-33.2861097653666,
21.6315709493723));
#33917=CARTESIAN_POINT('Ctrl Pts',(-12.9408400705193,-33.3139106582638,
21.6334201626978));
#33918=CARTESIAN_POINT('Ctrl Pts',(-12.9875015230559,-33.3971145452151,
21.6388701299844));
#33919=CARTESIAN_POINT('Ctrl Pts',(-13.0168959875074,-33.4531495120161,
21.6424308683072));
#33920=CARTESIAN_POINT('Ctrl Pts',(-13.09460618968,-33.611942182526,21.6522535415147));
#33921=CARTESIAN_POINT('Ctrl Pts',(-13.1393414202323,-33.7163270668683,
21.6584041337633));
#33922=CARTESIAN_POINT('Ctrl Pts',(-13.1787500936073,-33.8227349895238,
21.6644775413951));
#33923=CARTESIAN_POINT('Origin',(-10.,-35.,23.));
#33924=CARTESIAN_POINT('',(-13.1787501240204,-33.8227350716428,22.9104831197053));
#33925=CARTESIAN_POINT('',(-13.1787501379842,-33.8227351093465,22.5700367124769));
#33926=CARTESIAN_POINT('',(-13.1787501240207,-33.8227350716434,23.));
#33927=CARTESIAN_POINT('Ctrl Pts',(-13.1787501379842,-33.8227351093465,
22.5700367124769));
#33928=CARTESIAN_POINT('Ctrl Pts',(-13.1376176986524,-33.711672808721,22.563741246396));
#33929=CARTESIAN_POINT('Ctrl Pts',(-13.0906853862704,-33.6028221111455,
22.5574976443462));
#33930=CARTESIAN_POINT('Ctrl Pts',(-12.9793754110903,-33.3778768480948,
22.5440690148351));
#33931=CARTESIAN_POINT('Ctrl Pts',(-12.9137041264173,-33.2626794508871,
22.5368727854472));
#33932=CARTESIAN_POINT('Ctrl Pts',(-12.8264011327451,-33.128469811955,22.5277475901435));
#33933=CARTESIAN_POINT('Ctrl Pts',(-12.8110515889448,-33.1054928164769,
22.5261575527729));
#33934=CARTESIAN_POINT('Ctrl Pts',(-12.7861599442011,-33.0692006692235,
22.5235971835025));
#33935=CARTESIAN_POINT('Ctrl Pts',(-12.7767989417492,-33.0557621279459,
22.5226382308669));
#33936=CARTESIAN_POINT('Ctrl Pts',(-12.7585282543424,-33.0299340604824,
22.5207729722818));
#33937=CARTESIAN_POINT('Ctrl Pts',(-12.749631677789,-33.0175359926719,22.5198674993266));
#33938=CARTESIAN_POINT('Ctrl Pts',(-12.7270964442602,-32.9865748962383,
22.5175816295615));
#33939=CARTESIAN_POINT('Ctrl Pts',(-12.7133518333218,-32.968090201426,22.5161944028187));
#33940=CARTESIAN_POINT('Ctrl Pts',(-12.6612222251301,-32.8994548846264,
22.5109631377593));
#33941=CARTESIAN_POINT('Ctrl Pts',(-12.6216284478103,-32.8502426255418,
22.5070497055591));
#33942=CARTESIAN_POINT('Ctrl Pts',(-12.3878900997955,-32.575787906325,22.484408035944));
#33943=CARTESIAN_POINT('Ctrl Pts',(-12.1661413279739,-32.3757504411427,
22.4648031407634));
#33944=CARTESIAN_POINT('Ctrl Pts',(-11.8647312001848,-32.1684164322998,
22.4419289575259));
#33945=CARTESIAN_POINT('Ctrl Pts',(-11.8071866185858,-32.1313478058999,
22.4377009266429));
#33946=CARTESIAN_POINT('Ctrl Pts',(-11.7021411727101,-32.0680968746584,
22.4302316393656));
#33947=CARTESIAN_POINT('Ctrl Pts',(-11.6550608448305,-32.0412646934652,
22.4269692887427));
#33948=CARTESIAN_POINT('Ctrl Pts',(-11.5806252426908,-32.0011751200555,
22.4219405041543));
#33949=CARTESIAN_POINT('Ctrl Pts',(-11.5537022595429,-31.9871382048065,
22.4201472123033));
#33950=CARTESIAN_POINT('Ctrl Pts',(-11.5029760807918,-31.9615517666286,
22.4168149269598));
#33951=CARTESIAN_POINT('Ctrl Pts',(-11.4792194034459,-31.9499156107942,
22.4152730391401));
#33952=CARTESIAN_POINT('Ctrl Pts',(-11.4253987337083,-31.9243306858185,
22.4118206763353));
#33953=CARTESIAN_POINT('Ctrl Pts',(-11.3952612695439,-31.9105422189353,
22.4099157474859));
#33954=CARTESIAN_POINT('Ctrl Pts',(-11.3019674795773,-31.8695021943585,
22.4041011236112));
#33955=CARTESIAN_POINT('Ctrl Pts',(-11.2381783226978,-31.843728282554,22.4002402748824));
#33956=CARTESIAN_POINT('Ctrl Pts',(-10.893496879008,-31.7165198661492,22.3798981167027));
#33957=CARTESIAN_POINT('Ctrl Pts',(-10.6009377597614,-31.6506056722566,
22.3645787437914));
#33958=CARTESIAN_POINT('Ctrl Pts',(-10.2356426849547,-31.6177634356753,
22.344741667329));
#33959=CARTESIAN_POINT('Ctrl Pts',(-10.1675852748959,-31.6137091251308,
22.3410096298109));
#33960=CARTESIAN_POINT('Ctrl Pts',(-10.053565861396,-31.6103623432665,22.3346314948549));
#33961=CARTESIAN_POINT('Ctrl Pts',(-10.0076557669188,-31.6099478305808,
22.3320292315965));
#33962=CARTESIAN_POINT('Ctrl Pts',(-9.94186130276043,-31.6106902301714,
22.3282333881118));
#33963=CARTESIAN_POINT('Ctrl Pts',(-9.92197169764219,-31.6110897966416,
22.3270771907272));
#33964=CARTESIAN_POINT('Ctrl Pts',(-9.88714251583776,-31.6120962552786,
22.3250355048485));
#33965=CARTESIAN_POINT('Ctrl Pts',(-9.87220163151213,-31.612626952792,22.3241541054779));
#33966=CARTESIAN_POINT('Ctrl Pts',(-9.83931643290485,-31.6140129134367,
22.3222014745032));
#33967=CARTESIAN_POINT('Ctrl Pts',(-9.82137534201628,-31.6149119717656,
22.3211280437448));
#33968=CARTESIAN_POINT('Ctrl Pts',(-9.76928420541067,-31.6179376080129,
22.317989383098));
#33969=CARTESIAN_POINT('Ctrl Pts',(-9.73515909739502,-31.6204386520451,
22.3159057471138));
#33970=CARTESIAN_POINT('Ctrl Pts',(-9.45373903072422,-31.6453523862283,
22.2985268603149));
#33971=CARTESIAN_POINT('Ctrl Pts',(-9.20956567706115,-31.6943582004883,
22.2822605001604));
#33972=CARTESIAN_POINT('Ctrl Pts',(-8.85983550571905,-31.8055490534237,
22.258763718696));
#33973=CARTESIAN_POINT('Ctrl Pts',(-8.74868598711848,-31.8474281753225,
22.251252866723));
#33974=CARTESIAN_POINT('Ctrl Pts',(-8.56652355707648,-31.9272199770638,
22.2389418655143));
#33975=CARTESIAN_POINT('Ctrl Pts',(-8.49425235966925,-31.9619813328979,
22.2340560959784));
#33976=CARTESIAN_POINT('Ctrl Pts',(-8.39225059753278,-32.0155778876293,
22.227157380898));
#33977=CARTESIAN_POINT('Ctrl Pts',(-8.36147799758298,-32.032361330629,22.2250755680216));
#33978=CARTESIAN_POINT('Ctrl Pts',(-8.30777079576461,-32.0627434840589,
22.221439913661));
#33979=CARTESIAN_POINT('Ctrl Pts',(-8.284726381506,-32.0761409072782,22.2198791812572));
#33980=CARTESIAN_POINT('Ctrl Pts',(-8.23672289347574,-32.1048117585278,
22.2166254201802));
#33981=CARTESIAN_POINT('Ctrl Pts',(-8.21179864953554,-32.1201393929929,
22.2149344972395));
#33982=CARTESIAN_POINT('Ctrl Pts',(-8.14584906974524,-32.1618826795923,
22.2104540432144));
#33983=CARTESIAN_POINT('Ctrl Pts',(-8.10518958857028,-32.1888650979512,
22.2076852277565));
#33984=CARTESIAN_POINT('Ctrl Pts',(-7.84382399588872,-32.3705604753737,
22.1898109435594));
#33985=CARTESIAN_POINT('Ctrl Pts',(-7.64166368014102,-32.5502434123526,
22.175723802859));
#33986=CARTESIAN_POINT('Ctrl Pts',(-7.3578104031017,-32.8705977040419,22.1529484125132));
#33987=CARTESIAN_POINT('Ctrl Pts',(-7.26116989790374,-32.9964234827058,
22.1444297194764));
#33988=CARTESIAN_POINT('Ctrl Pts',(-7.15801121976463,-33.1522143681483,
22.1337909986669));
#33989=CARTESIAN_POINT('Ctrl Pts',(-7.14262718598728,-33.1760941751605,
22.1321577443594));
#33990=CARTESIAN_POINT('Ctrl Pts',(-7.11876148391041,-33.2141827162502,
22.1295440559974));
#33991=CARTESIAN_POINT('Ctrl Pts',(-7.11008030176965,-33.2282655756924,
22.1285758346648));
#33992=CARTESIAN_POINT('Ctrl Pts',(-7.09363604649763,-33.2553843339179,
22.1267067536304));
#33993=CARTESIAN_POINT('Ctrl Pts',(-7.08585685595849,-33.268409703383,22.1258069157041));
#33994=CARTESIAN_POINT('Ctrl Pts',(-7.06857617134252,-33.2977905010256,
22.1237731504447));
#33995=CARTESIAN_POINT('Ctrl Pts',(-7.05912361379391,-33.3141741231999,
22.1226363025139));
#33996=CARTESIAN_POINT('Ctrl Pts',(-7.02601084463858,-33.3726927998073,
22.1185683067489));
#33997=CARTESIAN_POINT('Ctrl Pts',(-7.00311607546772,-33.4152519236794,
22.115596236862));
#33998=CARTESIAN_POINT('Ctrl Pts',(-6.88693653507092,-33.642744952137,22.0996944143998));
#33999=CARTESIAN_POINT('Ctrl Pts',(-6.80984180491637,-33.8354441446983,
22.0862029319513));
#34000=CARTESIAN_POINT('Ctrl Pts',(-6.70449611617657,-34.1897662310774,
22.0624657948694));
#34001=CARTESIAN_POINT('Ctrl Pts',(-6.6694358220799,-34.3487109761724,22.0521706120813));
#34002=CARTESIAN_POINT('Ctrl Pts',(-6.63673133105342,-34.5723810005353,
22.0383130559082));
#34003=CARTESIAN_POINT('Ctrl Pts',(-6.62931334434065,-34.6354366661849,
22.0344726589624));
#34004=CARTESIAN_POINT('Ctrl Pts',(-6.62081025148256,-34.7307107481719,
22.0287672340598));
#34005=CARTESIAN_POINT('Ctrl Pts',(-6.61840662364092,-34.7627946004006,
22.0268623701878));
#34006=CARTESIAN_POINT('Ctrl Pts',(-6.61501816603948,-34.8186964332337,
22.0235709215679));
#34007=CARTESIAN_POINT('Ctrl Pts',(-6.61382715518108,-34.8424991823737,
22.0221780984308));
#34008=CARTESIAN_POINT('Ctrl Pts',(-6.61169902960354,-34.8964176622354,
22.0190418353438));
#34009=CARTESIAN_POINT('Ctrl Pts',(-6.6109122000578,-34.9265375237965,22.0173031230613));
#34010=CARTESIAN_POINT('Ctrl Pts',(-6.60986689105551,-35.0082962245054,
22.012616958412));
#34011=CARTESIAN_POINT('Ctrl Pts',(-6.61038657672287,-35.0599379549259,
22.0096933305404));
#34012=CARTESIAN_POINT('Ctrl Pts',(-6.61999523229314,-35.3517658402121,
21.9933425233035));
#34013=CARTESIAN_POINT('Ctrl Pts',(-6.6534287301087,-35.5904602623956,21.9806847615013));
#34014=CARTESIAN_POINT('Ctrl Pts',(-6.75573419163348,-35.9988947511982,
21.95833983974));
#34015=CARTESIAN_POINT('Ctrl Pts',(-6.81357409613821,-36.1703531082455,
21.9487094528061));
#34016=CARTESIAN_POINT('Ctrl Pts',(-6.89611400993883,-36.362762611134,21.9367934717562));
#34017=CARTESIAN_POINT('Ctrl Pts',(-6.90777305965901,-36.3890149773763,
21.9351424287581));
#34018=CARTESIAN_POINT('Ctrl Pts',(-6.92669885405144,-36.4302101536988,
21.9325067943769));
#34019=CARTESIAN_POINT('Ctrl Pts',(-6.93374451162188,-36.4452537050986,
21.9315347656889));
#34020=CARTESIAN_POINT('Ctrl Pts',(-6.94742216941084,-36.4739073439134,
21.9296638825868));
#34021=CARTESIAN_POINT('Ctrl Pts',(-6.95403522431336,-36.487525738278,21.9287661255488));
#34022=CARTESIAN_POINT('Ctrl Pts',(-6.97064368655332,-36.5211527350863,
21.9265287657307));
#34023=CARTESIAN_POINT('Ctrl Pts',(-6.98074624347804,-36.5411073980275,
21.9251829280307));
#34024=CARTESIAN_POINT('Ctrl Pts',(-7.0179176497323,-36.6127601490116,21.9202883697684));
#34025=CARTESIAN_POINT('Ctrl Pts',(-7.04612164722486,-36.6638546475441,
21.9166807809232));
#34026=CARTESIAN_POINT('Ctrl Pts',(-7.17614792112779,-36.8856763746233,
21.9005752241649));
#34027=CARTESIAN_POINT('Ctrl Pts',(-7.29155253324919,-37.04798061258,21.8876309094508));
#34028=CARTESIAN_POINT('Ctrl Pts',(-7.44847768085481,-37.2320388334943,
21.872109708858));
#34029=CARTESIAN_POINT('Ctrl Pts',(-7.47707043848378,-37.2643078529894,
21.8693523126196));
#34030=CARTESIAN_POINT('Ctrl Pts',(-7.57490351605026,-37.3705651144733,
21.8601598026941));
#34031=CARTESIAN_POINT('Ctrl Pts',(-7.64684738181105,-37.4419965886759,
21.8537928539741));
#34032=CARTESIAN_POINT('Ctrl Pts',(-7.77521767097204,-37.5585025426337,
21.8431099084415));
#34033=CARTESIAN_POINT('Ctrl Pts',(-7.83007854770229,-37.6051936072031,
21.8387356304577));
#34034=CARTESIAN_POINT('Ctrl Pts',(-7.91273957331627,-37.6711205583938,
21.8324158928297));
#34035=CARTESIAN_POINT('Ctrl Pts',(-7.93940321835026,-37.6917433296695,
21.8304166645453));
#34036=CARTESIAN_POINT('Ctrl Pts',(-7.98757256395356,-37.727864212312,21.8268731254822));
#34037=CARTESIAN_POINT('Ctrl Pts',(-8.00896050673847,-37.7435140133772,
21.8253230582709));
#34038=CARTESIAN_POINT('Ctrl Pts',(-8.05493723459717,-37.7763348443081,
21.8220391954535));
#34039=CARTESIAN_POINT('Ctrl Pts',(-8.07957490053254,-37.7934337024044,
21.8203082055762));
#34040=CARTESIAN_POINT('Ctrl Pts',(-8.14670308686897,-37.8387135928312,
21.8156663631566));
#34041=CARTESIAN_POINT('Ctrl Pts',(-8.18960859901228,-37.8662672006653,
21.812778552512));
#34042=CARTESIAN_POINT('Ctrl Pts',(-8.44415559762776,-38.0217383655734,
21.796067227445));
#34043=CARTESIAN_POINT('Ctrl Pts',(-8.66865943771152,-38.1271549339003,
21.7830680071628));
#34044=CARTESIAN_POINT('Ctrl Pts',(-9.0162365776545,-38.2460787385525,21.7635625263914));
#34045=CARTESIAN_POINT('Ctrl Pts',(-9.13180257655126,-38.2788790223566,
21.757157668853));
#34046=CARTESIAN_POINT('Ctrl Pts',(-9.31376882354845,-38.3202293482322,
21.746882945748));
#34047=CARTESIAN_POINT('Ctrl Pts',(-9.37909662960953,-38.3330637553211,
21.7431565387111));
#34048=CARTESIAN_POINT('Ctrl Pts',(-9.46725425752513,-38.3477017776507,
21.7380276239211));
#34049=CARTESIAN_POINT('Ctrl Pts',(-9.48978960961286,-38.351210305986,21.73670780782));
#34050=CARTESIAN_POINT('Ctrl Pts',(-9.5275677849971,-38.3567021153977,21.7344781314196));
#34051=CARTESIAN_POINT('Ctrl Pts',(-9.54279225449063,-38.3588096640907,
21.733574921589));
#34052=CARTESIAN_POINT('Ctrl Pts',(-9.57439480773207,-38.3629656115988,
21.7316895338593));
#34053=CARTESIAN_POINT('Ctrl Pts',(-9.59077424765902,-38.3649980301599,
21.7307065962187));
#34054=CARTESIAN_POINT('Ctrl Pts',(-9.63520362093801,-38.3701818035246,
21.7280259940869));
#34055=CARTESIAN_POINT('Ctrl Pts',(-9.66327853207224,-38.3731024779914,
21.7263166255495));
#34056=CARTESIAN_POINT('Ctrl Pts',(-9.83078526454199,-38.3884164612281,
21.7160384550533));
#34057=CARTESIAN_POINT('Ctrl Pts',(-9.97082841551456,-38.3925125819555,
21.7071234683187));
#34058=CARTESIAN_POINT('Ctrl Pts',(-10.3105953595599,-38.3814098703585,
21.6852711138366));
#34059=CARTESIAN_POINT('Ctrl Pts',(-10.5095286513717,-38.3572003441564,
21.6723096346984));
#34060=CARTESIAN_POINT('Ctrl Pts',(-10.8113704460571,-38.293003325,21.6529509665439));
#34061=CARTESIAN_POINT('Ctrl Pts',(-10.916428042639,-38.2653263801649,21.6462660008175));
#34062=CARTESIAN_POINT('Ctrl Pts',(-11.0570823376647,-38.2209463248077,
21.6373978945339));
#34063=CARTESIAN_POINT('Ctrl Pts',(-11.0939766533955,-38.2086030553521,
21.6350792451096));
#34064=CARTESIAN_POINT('Ctrl Pts',(-11.1563640427418,-38.1865296420804,
21.6311698040555));
#34065=CARTESIAN_POINT('Ctrl Pts',(-11.1819663706516,-38.1771220503234,
21.6295687435354));
#34066=CARTESIAN_POINT('Ctrl Pts',(-11.2304956242356,-38.1586221217308,
21.626539285772));
#34067=CARTESIAN_POINT('Ctrl Pts',(-11.2534421970858,-38.149586622816,21.6251091443025));
#34068=CARTESIAN_POINT('Ctrl Pts',(-11.3070591443628,-38.1277954983539,
21.6217718261546));
#34069=CARTESIAN_POINT('Ctrl Pts',(-11.3376449672406,-38.1148377707331,
21.6198714395194));
#34070=CARTESIAN_POINT('Ctrl Pts',(-11.4468684890122,-38.0666594719413,
21.6130922200153));
#34071=CARTESIAN_POINT('Ctrl Pts',(-11.5243500729054,-38.0288920786886,
21.6082976337194));
#34072=CARTESIAN_POINT('Ctrl Pts',(-11.8417914851368,-37.8588888231763,
21.5885707029542));
#34073=CARTESIAN_POINT('Ctrl Pts',(-12.0666877467752,-37.7007838589456,
21.5744754338813));
#34074=CARTESIAN_POINT('Ctrl Pts',(-12.3194609763066,-37.4728370824409,
21.5560461746748));
#34075=CARTESIAN_POINT('Ctrl Pts',(-12.3674969355891,-37.4268868604747,
21.5524033050401));
#34076=CARTESIAN_POINT('Ctrl Pts',(-12.4458056605234,-37.347439756066,21.5461613960323));
#34077=CARTESIAN_POINT('Ctrl Pts',(-12.4768169988418,-37.3146956362789,
21.5436038013213));
#34078=CARTESIAN_POINT('Ctrl Pts',(-12.520461477466,-37.2667309867488,21.5398617162945));
#34079=CARTESIAN_POINT('Ctrl Pts',(-12.5336302327839,-37.2520020489353,
21.5387131697554));
#34080=CARTESIAN_POINT('Ctrl Pts',(-12.5565294444878,-37.2259347422351,
21.536679722016));
#34081=CARTESIAN_POINT('Ctrl Pts',(-12.5663148680068,-37.2146458550585,
21.5357987896089));
#34082=CARTESIAN_POINT('Ctrl Pts',(-12.5877666903053,-37.1895650046557,
21.533840542503));
#34083=CARTESIAN_POINT('Ctrl Pts',(-12.5993975323103,-37.1757444219897,
21.5327609347309));
#34084=CARTESIAN_POINT('Ctrl Pts',(-12.6330427024561,-37.135110018607,21.529586875146));
#34085=CARTESIAN_POINT('Ctrl Pts',(-12.6547558930936,-37.1080511407784,
21.5274734153496));
#34086=CARTESIAN_POINT('Ctrl Pts',(-12.7903099733162,-36.9337081422798,
21.5138825438768));
#34087=CARTESIAN_POINT('Ctrl Pts',(-12.8922632108645,-36.7775996746517,
21.501849193541));
#34088=CARTESIAN_POINT('Ctrl Pts',(-13.0562987579485,-36.4746302106539,
21.4796454067493));
#34089=CARTESIAN_POINT('Ctrl Pts',(-13.1218661346566,-36.3302088964952,
21.4694890464365));
#34090=CARTESIAN_POINT('Ctrl Pts',(-13.2105287638497,-36.0918366105283,
21.4536219736481));
#34091=CARTESIAN_POINT('Ctrl Pts',(-13.2401341735268,-36.000567512039,21.4477425953186));
#34092=CARTESIAN_POINT('Ctrl Pts',(-13.275832687443,-35.8721920037655,21.4397441484479));
#34093=CARTESIAN_POINT('Ctrl Pts',(-13.2852396834973,-35.8360616464855,
21.4375220092756));
#34094=CARTESIAN_POINT('Ctrl Pts',(-13.30041843446,-35.7735452004135,21.4337253265084));
#34095=CARTESIAN_POINT('Ctrl Pts',(-13.3064751037301,-35.7472325413186,
21.4321419190067));
#34096=CARTESIAN_POINT('Ctrl Pts',(-13.3182496912756,-35.6931297441005,
21.4289150345263));
#34097=CARTESIAN_POINT('Ctrl Pts',(-13.3239344023829,-35.6653345140264,
21.4272727130019));
#34098=CARTESIAN_POINT('Ctrl Pts',(-13.3376335982534,-35.5937887527209,
21.4230831144521));
#34099=CARTESIAN_POINT('Ctrl Pts',(-13.3451373092684,-35.5499452330688,
21.4205518410088));
#34100=CARTESIAN_POINT('Ctrl Pts',(-13.3771969771401,-35.3375653629982,
21.4084463936505));
#34101=CARTESIAN_POINT('Ctrl Pts',(-13.3898921009111,-35.1674812302973,
21.3992404617354));
#34102=CARTESIAN_POINT('Ctrl Pts',(-13.3895475950888,-34.7579871130917,
21.3774224061149));
#34103=CARTESIAN_POINT('Ctrl Pts',(-13.3640366909492,-34.5195447800139,
21.365014017526));
#34104=CARTESIAN_POINT('Ctrl Pts',(-13.3041286563306,-34.2415911078333,
21.3491058622142));
#34105=CARTESIAN_POINT('Ctrl Pts',(-13.293717064086,-34.1975800844463,21.3465412789965));
#34106=CARTESIAN_POINT('Ctrl Pts',(-13.2775434534815,-34.1348428241764,
21.3428028679112));
#34107=CARTESIAN_POINT('Ctrl Pts',(-13.272494294406,-34.1159360420124,21.3416653853085));
#34108=CARTESIAN_POINT('Ctrl Pts',(-13.2632990015683,-34.0826624060655,
21.3396426608231));
#34109=CARTESIAN_POINT('Ctrl Pts',(-13.259221079058,-34.0682776263751,21.3387612019157));
#34110=CARTESIAN_POINT('Ctrl Pts',(-13.2500374926068,-34.0366809231078,
21.3368092106831));
#34111=CARTESIAN_POINT('Ctrl Pts',(-13.2448902572386,-34.0194825172306,
21.3357364900349));
#34112=CARTESIAN_POINT('Ctrl Pts',(-13.2292397424989,-33.9686627847612,
21.3325379953537));
#34113=CARTESIAN_POINT('Ctrl Pts',(-13.2183490524295,-33.9351643634232,
21.3303922840306));
#34114=CARTESIAN_POINT('Ctrl Pts',(-13.1978680991166,-33.8753539939704,
21.3265012087214));
#34115=CARTESIAN_POINT('Ctrl Pts',(-13.1884710371189,-33.84898265086,21.3247643411037));
#34116=CARTESIAN_POINT('Ctrl Pts',(-13.1787501333198,-33.8227350967521,
21.3230163149173));
#34117=CARTESIAN_POINT('',(-13.389749867084,-34.9990507350945,21.7311301749608));
#34118=CARTESIAN_POINT('Ctrl Pts',(-13.1787500936073,-33.8227349895238,
21.6644775413951));
#34119=CARTESIAN_POINT('Ctrl Pts',(-13.1948737496338,-33.8662707037832,
21.6669624140685));
#34120=CARTESIAN_POINT('Ctrl Pts',(-13.2101057520662,-33.9101450433166,
21.6694348331333));
#34121=CARTESIAN_POINT('Ctrl Pts',(-13.2712235710965,-34.0986084927412,
21.6799584931992));
#34122=CARTESIAN_POINT('Ctrl Pts',(-13.3082740429438,-34.2458582370596,
21.6879338889851));
#34123=CARTESIAN_POINT('Ctrl Pts',(-13.3523689409156,-34.4889866704007,
21.70132228591));
#34124=CARTESIAN_POINT('Ctrl Pts',(-13.3654246881183,-34.5835557279141,
21.7065849537685));
#34125=CARTESIAN_POINT('Ctrl Pts',(-13.376957464737,-34.7046195661836,21.7135295727455));
#34126=CARTESIAN_POINT('Ctrl Pts',(-13.3791392763981,-34.7307250836849,
21.715039329318));
#34127=CARTESIAN_POINT('Ctrl Pts',(-13.3821708185903,-34.7728793126426,
21.717500700615));
#34128=CARTESIAN_POINT('Ctrl Pts',(-13.3832094036412,-34.7889138547634,
21.7184424219694));
#34129=CARTESIAN_POINT('Ctrl Pts',(-13.3849363291718,-34.8188768975796,
21.7202133817078));
#34130=CARTESIAN_POINT('Ctrl Pts',(-13.3856527898447,-34.8328034192798,
21.7210410532929));
#34131=CARTESIAN_POINT('Ctrl Pts',(-13.3869928569964,-34.8624109981548,
21.7228097754308));
#34132=CARTESIAN_POINT('Ctrl Pts',(-13.3875935356735,-34.8780928088416,
21.7237520103063));
#34133=CARTESIAN_POINT('Ctrl Pts',(-13.3891851625189,-34.9288597128656,
21.7268186450154));
#34134=CARTESIAN_POINT('Ctrl Pts',(-13.3897400388564,-34.9639549119412,
21.7289638292364));
#34135=CARTESIAN_POINT('Ctrl Pts',(-13.389749867084,-34.9990507350945,21.7311301749608));
#34136=CARTESIAN_POINT('Ctrl Pts',(-13.3897498660442,-34.9990470292048,
21.7311299462089));
#34137=CARTESIAN_POINT('Ctrl Pts',(-13.3898014297935,-35.1824610573557,
21.7424514621912));
#34138=CARTESIAN_POINT('Ctrl Pts',(-13.374966596757,-35.3655710725717,21.75431371688));
#34139=CARTESIAN_POINT('Ctrl Pts',(-13.3201353354254,-35.7011744871535,
21.7762271822552));
#34140=CARTESIAN_POINT('Ctrl Pts',(-13.2841883531142,-35.8538492343368,
21.7862660856627));
#34141=CARTESIAN_POINT('Ctrl Pts',(-13.2095983064274,-36.0945150714575,
21.8019809951908));
#34142=CARTESIAN_POINT('Ctrl Pts',(-13.1775629265222,-36.1843061302093,
21.8078213884003));
#34143=CARTESIAN_POINT('Ctrl Pts',(-13.127799109752,-36.3071592484198,21.8157772703349));
#34144=CARTESIAN_POINT('Ctrl Pts',(-13.1132458624233,-36.3414518023022,
21.8179943667585));
#34145=CARTESIAN_POINT('Ctrl Pts',(-13.0871796535606,-36.4001625144136,
21.8217851933286));
#34146=CARTESIAN_POINT('Ctrl Pts',(-13.0759350710889,-36.4246953292758,
21.8233677151569));
#34147=CARTESIAN_POINT('Ctrl Pts',(-13.0522597927309,-36.4747615068826,
21.8265951718281));
#34148=CARTESIAN_POINT('Ctrl Pts',(-13.0397987851075,-36.5002782281438,
21.8282389208609));
#34149=CARTESIAN_POINT('Ctrl Pts',(-13.0069434719252,-36.5654665427469,
21.8324371465003));
#34150=CARTESIAN_POINT('Ctrl Pts',(-12.9860837897947,-36.6048982523692,
21.8349754860888));
#34151=CARTESIAN_POINT('Ctrl Pts',(-12.8789622783248,-36.7980699339472,
21.8474232633832));
#34152=CARTESIAN_POINT('Ctrl Pts',(-12.7815747146027,-36.9453356086829,
21.856934959789));
#34153=CARTESIAN_POINT('Ctrl Pts',(-12.5604090539148,-37.2289762607998,
21.8760799413469));
#34154=CARTESIAN_POINT('Ctrl Pts',(-12.4361123461674,-37.3641869203607,
21.8856737265604));
#34155=CARTESIAN_POINT('Ctrl Pts',(-12.2400646918167,-37.545489596148,21.9002317856925));
#34156=CARTESIAN_POINT('Ctrl Pts',(-12.1765519452948,-37.600005116813,21.9048752055764));
#34157=CARTESIAN_POINT('Ctrl Pts',(-12.0918562634241,-37.667423278751,21.9110711413184));
#34158=CARTESIAN_POINT('Ctrl Pts',(-12.0724543058802,-37.6825254239083,
21.9124907678182));
#34159=CARTESIAN_POINT('Ctrl Pts',(-12.0403782051454,-37.7069372130646,
21.9148413176081));
#34160=CARTESIAN_POINT('Ctrl Pts',(-12.0278001317851,-37.7163723794699,
21.9157639272681));
#34161=CARTESIAN_POINT('Ctrl Pts',(-12.003859659853,-37.7340718570004,21.917522580629));
#34162=CARTESIAN_POINT('Ctrl Pts',(-11.9925106385795,-37.7423536962041,
21.9183573447529));
#34163=CARTESIAN_POINT('Ctrl Pts',(-11.9616775860849,-37.7645613877999,
21.9206273817551));
#34164=CARTESIAN_POINT('Ctrl Pts',(-11.9420972906718,-37.7783514286413,
21.9220712465145));
#34165=CARTESIAN_POINT('Ctrl Pts',(-11.8643354689945,-37.8318939990843,
21.9278092094343));
#34166=CARTESIAN_POINT('Ctrl Pts',(-11.8050696840158,-37.8700335241079,
21.9321902869708));
#34167=CARTESIAN_POINT('Ctrl Pts',(-11.5825515252263,-38.0036122115057,
21.9485512081874));
#34168=CARTESIAN_POINT('Ctrl Pts',(-11.4125858551877,-38.0871921023347,
21.9608582823783));
#34169=CARTESIAN_POINT('Ctrl Pts',(-11.0778030109755,-38.2183553781346,
21.9839109068227));
#34170=CARTESIAN_POINT('Ctrl Pts',(-10.9145832554482,-38.2684891111561,
21.9946603017103));
#34171=CARTESIAN_POINT('Ctrl Pts',(-10.6972330757303,-38.3176812395879,
22.0082163571504));
#34172=CARTESIAN_POINT('Ctrl Pts',(-10.6459381339013,-38.3280485502794,
22.0113636114434));
#34173=CARTESIAN_POINT('Ctrl Pts',(-10.5649023637633,-38.3424825215882,
22.0162563644988));
#34174=CARTESIAN_POINT('Ctrl Pts',(-10.535314081407,-38.3473486535563,22.0180263976449));
#34175=CARTESIAN_POINT('Ctrl Pts',(-10.4794596757818,-38.355774992147,22.0213378715053));
#34176=CARTESIAN_POINT('Ctrl Pts',(-10.453208967522,-38.3594209425359,22.0228818630104));
#34177=CARTESIAN_POINT('Ctrl Pts',(-10.3934740504008,-38.3670045641113,
22.0263684815111));
#34178=CARTESIAN_POINT('Ctrl Pts',(-10.3599681695719,-38.3707513400725,
22.0283050782568));
#34179=CARTESIAN_POINT('Ctrl Pts',(-10.2715337675651,-38.3793067604117,
22.0333699483863));
#34180=CARTESIAN_POINT('Ctrl Pts',(-10.2165331813105,-38.3832763134464,
22.0364727101992));
#34181=CARTESIAN_POINT('Ctrl Pts',(-9.90312068228571,-38.3982215058787,
22.0539308080207));
#34182=CARTESIAN_POINT('Ctrl Pts',(-9.64422867801832,-38.3809359490208,
22.0674124687924));
#34183=CARTESIAN_POINT('Ctrl Pts',(-9.25546531681056,-38.3097924925162,
22.0884811352638));
#34184=CARTESIAN_POINT('Ctrl Pts',(-9.12273998932656,-38.2771124984082,
22.0958458289397));
#34185=CARTESIAN_POINT('Ctrl Pts',(-8.95896723938749,-38.2261244666974,
22.1055377358029));
#34186=CARTESIAN_POINT('Ctrl Pts',(-8.92573790191977,-38.2152121280007,
22.107536540246));
#34187=CARTESIAN_POINT('Ctrl Pts',(-8.87576387900573,-38.1979397625401,
22.1105999404111));
#34188=CARTESIAN_POINT('Ctrl Pts',(-8.85889002823405,-38.1919576409867,
22.1116443036231));
#34189=CARTESIAN_POINT('Ctrl Pts',(-8.82800610899173,-38.1807324844832,
22.1135755383714));
#34190=CARTESIAN_POINT('Ctrl Pts',(-8.81398223913815,-38.1755299812052,
22.1144601263776));
#34191=CARTESIAN_POINT('Ctrl Pts',(-8.78162832270628,-38.1632832810413,
22.1165184405307));
#34192=CARTESIAN_POINT('Ctrl Pts',(-8.76332455319008,-38.1561724380565,
22.1176958732035));
#34193=CARTESIAN_POINT('Ctrl Pts',(-8.70269691962236,-38.1320108242399,
22.1216366890609));
#34194=CARTESIAN_POINT('Ctrl Pts',(-8.6606572828943,-38.1142652010072,22.1244357608061));
#34195=CARTESIAN_POINT('Ctrl Pts',(-8.42660583762881,-38.0098527789951,
22.140345773963));
#34196=CARTESIAN_POINT('Ctrl Pts',(-8.24264930127822,-37.9062853810792,
22.1540685466479));
#34197=CARTESIAN_POINT('Ctrl Pts',(-7.90736028029149,-37.673981032209,22.1802689251291));
#34198=CARTESIAN_POINT('Ctrl Pts',(-7.75531358766897,-37.5476889197956,
22.1927199908908));
#34199=CARTESIAN_POINT('Ctrl Pts',(-7.58317184072951,-37.3772600271542,
22.207367828932));
#34200=CARTESIAN_POINT('Ctrl Pts',(-7.55187501122673,-37.3450176796722,
22.2100578466236));
#34201=CARTESIAN_POINT('Ctrl Pts',(-7.501813478758,-37.29134877964,22.2144073871783));
#34202=CARTESIAN_POINT('Ctrl Pts',(-7.48266218809584,-37.2702919502743,
22.2160830538561));
#34203=CARTESIAN_POINT('Ctrl Pts',(-7.44589610966172,-37.2288303634244,
22.2193240945206));
#34204=CARTESIAN_POINT('Ctrl Pts',(-7.42825507096532,-37.2084518453126,
22.2208904842015));
#34205=CARTESIAN_POINT('Ctrl Pts',(-7.38694751422866,-37.1595680598413,
22.2245868114883));
#34206=CARTESIAN_POINT('Ctrl Pts',(-7.36350130915709,-37.1308806406257,
22.2267078497248));
#34207=CARTESIAN_POINT('Ctrl Pts',(-7.28602816096082,-37.0328521861737,
22.2338020674531));
#34208=CARTESIAN_POINT('Ctrl Pts',(-7.23422722925325,-36.9617935298267,
22.2386903889364));
#34209=CARTESIAN_POINT('Ctrl Pts',(-7.03366624091163,-36.6629100794874,
22.2583932251581));
#34210=CARTESIAN_POINT('Ctrl Pts',(-6.90983989402039,-36.4196150802825,
22.272394499527));
#34211=CARTESIAN_POINT('Ctrl Pts',(-6.79364603208641,-36.1018609088283,
22.2907149503242));
#34212=CARTESIAN_POINT('Ctrl Pts',(-6.77270400059847,-36.0389239064928,
22.2943502301844));
#34213=CARTESIAN_POINT('Ctrl Pts',(-6.74066576285426,-35.9322943698348,
22.3005805224513));
#34214=CARTESIAN_POINT('Ctrl Pts',(-6.72857025323899,-35.888920396955,22.3031342905904));
#34215=CARTESIAN_POINT('Ctrl Pts',(-6.71241868753829,-35.8261985690928,
22.3068717668717));
#34216=CARTESIAN_POINT('Ctrl Pts',(-6.70766185898986,-35.8070343772999,
22.3080196532421));
#34217=CARTESIAN_POINT('Ctrl Pts',(-6.69960068354594,-35.7732998146078,
22.3100523932856));
#34218=CARTESIAN_POINT('Ctrl Pts',(-6.69622480620727,-35.7587474599528,
22.310933288554));
#34219=CARTESIAN_POINT('Ctrl Pts',(-6.68897760945146,-35.726541395849,22.3128920343417));
#34220=CARTESIAN_POINT('Ctrl Pts',(-6.68515124754349,-35.7088789647203,
22.3139721861852));
#34221=CARTESIAN_POINT('Ctrl Pts',(-6.67438372353001,-35.6571818427568,
22.3171493743282));
#34222=CARTESIAN_POINT('Ctrl Pts',(-6.66782444519026,-35.6230709939965,
22.319265472243));
#34223=CARTESIAN_POINT('Ctrl Pts',(-6.62960161763157,-35.4063907765405,
22.3328067584454));
#34224=CARTESIAN_POINT('Ctrl Pts',(-6.61243092858146,-35.2215958436088,
22.3447825320378));
#34225=CARTESIAN_POINT('Ctrl Pts',(-6.60874088432275,-34.8774078561114,
22.3669663739473));
#34226=CARTESIAN_POINT('Ctrl Pts',(-6.61821705820595,-34.7185414332373,
22.3771588389397));
#34227=CARTESIAN_POINT('Ctrl Pts',(-6.65125485446441,-34.4656367369562,
22.3930725831109));
#34228=CARTESIAN_POINT('Ctrl Pts',(-6.66774796781935,-34.3709235048089,
22.3989638545905));
#34229=CARTESIAN_POINT('Ctrl Pts',(-6.69621222701085,-34.2405351241062,
22.4069752770926));
#34230=CARTESIAN_POINT('Ctrl Pts',(-6.70478256745449,-34.204171635057,22.4091989470177));
#34231=CARTESIAN_POINT('Ctrl Pts',(-6.72058073435574,-34.1417788602738,
22.4129974078084));
#34232=CARTESIAN_POINT('Ctrl Pts',(-6.72752164809753,-34.1156811979278,
22.4145810845332));
#34233=CARTESIAN_POINT('Ctrl Pts',(-6.7423902829352,-34.0623495648298,22.4178077987725));
#34234=CARTESIAN_POINT('Ctrl Pts',(-6.75034945539181,-34.0351265283714,
22.4194496900079));
#34235=CARTESIAN_POINT('Ctrl Pts',(-6.77165371380438,-33.9655146496115,
22.4236366885944));
#34236=CARTESIAN_POINT('Ctrl Pts',(-6.78549257598768,-33.923281855694,22.4261658324929));
#34237=CARTESIAN_POINT('Ctrl Pts',(-6.85583670590559,-33.7220692811147,
22.4381797374926));
#34238=CARTESIAN_POINT('Ctrl Pts',(-6.92332986983456,-33.5671779217981,
22.4473039103074));
#34239=CARTESIAN_POINT('Ctrl Pts',(-7.07971194799279,-33.2708419029367,
22.465161458087));
#34240=CARTESIAN_POINT('Ctrl Pts',(-7.16805894470149,-33.129658681684,22.4738770472087));
#34241=CARTESIAN_POINT('Ctrl Pts',(-7.30855850616282,-32.9380522139871,
22.4867038150892));
#34242=CARTESIAN_POINT('Ctrl Pts',(-7.35250952116893,-32.8819161706727,
22.4905986910988));
#34243=CARTESIAN_POINT('Ctrl Pts',(-7.42855954470036,-32.7908501354757,
22.4972244262691));
#34244=CARTESIAN_POINT('Ctrl Pts',(-7.45968155666443,-32.7551323236651,
22.4999069213872));
#34245=CARTESIAN_POINT('Ctrl Pts',(-7.50508206894105,-32.7051808444429,
22.503799149493));
#34246=CARTESIAN_POINT('Ctrl Pts',(-7.51875614414188,-32.6904027787917,
22.5049688462187));
#34247=CARTESIAN_POINT('Ctrl Pts',(-7.54273544682032,-32.6649462151685,
22.5070174223472));
#34248=CARTESIAN_POINT('Ctrl Pts',(-7.55298044535729,-32.6542121681171,
22.5078919043169));
#34249=CARTESIAN_POINT('Ctrl Pts',(-7.57562548140609,-32.6307959520671,
22.5098236188996));
#34250=CARTESIAN_POINT('Ctrl Pts',(-7.58805458115482,-32.6181438135356,
22.5108829411165));
#34251=CARTESIAN_POINT('Ctrl Pts',(-7.62399014855268,-32.5821330852437,
22.5139414881966));
#34252=CARTESIAN_POINT('Ctrl Pts',(-7.64774000680703,-32.5590215118438,
22.5159577899144));
#34253=CARTESIAN_POINT('Ctrl Pts',(-7.85656091948985,-32.3616904577138,
22.5336126020715));
#34254=CARTESIAN_POINT('Ctrl Pts',(-8.0603371460303,-32.2084575586157,22.5502799925132));
#34255=CARTESIAN_POINT('Ctrl Pts',(-8.42181563377445,-31.9954877196059,
22.5771231250587));
#34256=CARTESIAN_POINT('Ctrl Pts',(-8.57028324371348,-31.9220652871872,
22.5875139429465));
#34257=CARTESIAN_POINT('Ctrl Pts',(-8.76847037169948,-31.841504697235,22.6004891765195));
#34258=CARTESIAN_POINT('Ctrl Pts',(-8.81379345509957,-31.8242052647429,
22.6034001258894));
#34259=CARTESIAN_POINT('Ctrl Pts',(-8.88697090826083,-31.7980593538467,
22.6080125397807));
#34260=CARTESIAN_POINT('Ctrl Pts',(-8.91459418364839,-31.7885903478059,
22.6097340364942));
#34261=CARTESIAN_POINT('Ctrl Pts',(-8.96767651560219,-31.7711573855649,
22.6130058119521));
#34262=CARTESIAN_POINT('Ctrl Pts',(-8.9931138511195,-31.7631347343151,22.6145578890372));
#34263=CARTESIAN_POINT('Ctrl Pts',(-9.05173785083539,-31.7454033476397,
22.6181000459552));
#34264=CARTESIAN_POINT('Ctrl Pts',(-9.08498395861011,-31.7359003933252,
22.6200834231012));
#34265=CARTESIAN_POINT('Ctrl Pts',(-9.1920558845101,-31.707059850489,22.6263948678563));
#34266=CARTESIAN_POINT('Ctrl Pts',(-9.26639369848994,-31.6897052261789,
22.6306609566973));
#34267=CARTESIAN_POINT('Ctrl Pts',(-9.57747557085968,-31.6280766783013,
22.6481317161137));
#34268=CARTESIAN_POINT('Ctrl Pts',(-9.81800128341718,-31.6065838420149,
22.6606773170699));
#34269=CARTESIAN_POINT('Ctrl Pts',(-10.2005904220841,-31.6132190992123,
22.6811039488407));
#34270=CARTESIAN_POINT('Ctrl Pts',(-10.3420931772,-31.6245762595113,22.6887780304506));
#34271=CARTESIAN_POINT('Ctrl Pts',(-10.510133267236,-31.648738868499,22.6984497112034));
#34272=CARTESIAN_POINT('Ctrl Pts',(-10.5377626351861,-31.6530613446452,
22.7000583515354));
#34273=CARTESIAN_POINT('Ctrl Pts',(-10.5815532377616,-31.6604683755219,
22.7026416717853));
#34274=CARTESIAN_POINT('Ctrl Pts',(-10.5977515228169,-31.6633296939084,
22.7036046165762));
#34275=CARTESIAN_POINT('Ctrl Pts',(-10.6288967639686,-31.669065358405,22.7054714176766));
#34276=CARTESIAN_POINT('Ctrl Pts',(-10.6438462278285,-31.6719226678952,
22.7063743588041));
#34277=CARTESIAN_POINT('Ctrl Pts',(-10.6811603653796,-31.6793153761943,
22.7086445849749));
#34278=CARTESIAN_POINT('Ctrl Pts',(-10.7034992376547,-31.6839760895616,
22.7100185081185));
#34279=CARTESIAN_POINT('Ctrl Pts',(-10.7859292328761,-31.7020444255662,
22.7151388644035));
#34280=CARTESIAN_POINT('Ctrl Pts',(-10.8456958063665,-31.7168622669218,
22.7189511238833));
#34281=CARTESIAN_POINT('Ctrl Pts',(-11.1174858838226,-31.7921602125352,
22.7366490045419));
#34282=CARTESIAN_POINT('Ctrl Pts',(-11.3236965972872,-31.8716077971768,
22.7510560753466));
#34283=CARTESIAN_POINT('Ctrl Pts',(-11.6203312529385,-32.0205115446803,
22.7722595594451));
#34284=CARTESIAN_POINT('Ctrl Pts',(-11.7174108754945,-32.0753926600818,
22.7792920733027));
#34285=CARTESIAN_POINT('Ctrl Pts',(-11.8765853574774,-32.1760416102348,
22.7909294053451));
#34286=CARTESIAN_POINT('Ctrl Pts',(-11.940141184754,-32.2193225309812,22.7956077829984));
#34287=CARTESIAN_POINT('Ctrl Pts',(-12.030028391597,-32.2851185409094,22.8022728460976));
#34288=CARTESIAN_POINT('Ctrl Pts',(-12.0575700804559,-32.3059320528537,
22.8043220708423));
#34289=CARTESIAN_POINT('Ctrl Pts',(-12.1057547361529,-32.3435156722515,
22.8079210725417));
#34290=CARTESIAN_POINT('Ctrl Pts',(-12.1265269486587,-32.3601145500539,
22.8094772911971));
#34291=CARTESIAN_POINT('Ctrl Pts',(-12.1699478058771,-32.3956568563033,
22.8127413424798));
#34292=CARTESIAN_POINT('Ctrl Pts',(-12.1925486637182,-32.4146553175153,
22.8144468090642));
#34293=CARTESIAN_POINT('Ctrl Pts',(-12.2528071535975,-32.4666676766893,
22.819013963924));
#34294=CARTESIAN_POINT('Ctrl Pts',(-12.2899868851227,-32.5002253782329,
22.8218534424652));
#34295=CARTESIAN_POINT('Ctrl Pts',(-12.5155548551991,-32.7130763878839,
22.8392504509205));
#34296=CARTESIAN_POINT('Ctrl Pts',(-12.6835305718693,-32.9127265797917,
22.852876034994));
#34297=CARTESIAN_POINT('Ctrl Pts',(-12.8894232342055,-33.223930495808,22.8727117155986));
#34298=CARTESIAN_POINT('Ctrl Pts',(-12.9470505615618,-33.3212863198408,
22.878760878303));
#34299=CARTESIAN_POINT('Ctrl Pts',(-13.0295989251202,-33.4781405116842,
22.888535624039));
#34300=CARTESIAN_POINT('Ctrl Pts',(-13.0578736639977,-33.5357822730399,
22.8921339168106));
#34301=CARTESIAN_POINT('Ctrl Pts',(-13.0938326434641,-33.6146799005638,
22.8971125471099));
#34302=CARTESIAN_POINT('Ctrl Pts',(-13.1029674435577,-33.6352636924332,
22.8984162489877));
#34303=CARTESIAN_POINT('Ctrl Pts',(-13.1179696269838,-33.669998087967,22.9006267133852));
#34304=CARTESIAN_POINT('Ctrl Pts',(-13.1239475829133,-33.6841006217632,
22.9015270859914));
#34305=CARTESIAN_POINT('Ctrl Pts',(-13.1362076135993,-33.7135775626803,
22.9034159088437));
#34306=CARTESIAN_POINT('Ctrl Pts',(-13.1424725514251,-33.728958253706,22.9044052311375));
#34307=CARTESIAN_POINT('Ctrl Pts',(-13.1589894645888,-33.7703766095457,
22.9070782124231));
#34308=CARTESIAN_POINT('Ctrl Pts',(-13.1690322333133,-33.7964956538649,
22.9087731676124));
#34309=CARTESIAN_POINT('Ctrl Pts',(-13.1787501240202,-33.8227350716421,
22.9104831197053));
#34310=CARTESIAN_POINT('Origin',(-10.,-35.,23.));
#34311=CARTESIAN_POINT('',(-13.1787501240175,-33.8227350716349,24.1659533822777));
#34312=CARTESIAN_POINT('',(-13.1787501550516,-33.8227351554304,23.8178420415151));
#34313=CARTESIAN_POINT('',(-13.1787501240207,-33.8227350716434,23.));
#34314=CARTESIAN_POINT('',(-13.3897493118742,-35.0021598954043,22.6386988750799));
#34315=CARTESIAN_POINT('Ctrl Pts',(-13.1787501550516,-33.8227351554304,
23.8178420415151));
#34316=CARTESIAN_POINT('Ctrl Pts',(-13.1694440940813,-33.79760772307,23.8161925519317));
#34317=CARTESIAN_POINT('Ctrl Pts',(-13.1598381340822,-33.7725853491873,
23.8145514041043));
#34318=CARTESIAN_POINT('Ctrl Pts',(-13.130346019916,-33.698404848225,23.8096905622592));
#34319=CARTESIAN_POINT('Ctrl Pts',(-13.10960418551,-33.6496006415447,23.8064985649223));
#34320=CARTESIAN_POINT('Ctrl Pts',(-13.0751712864305,-33.5735876306355,
23.8015344797837));
#34321=CARTESIAN_POINT('Ctrl Pts',(-13.062244683633,-33.5460439221437,23.7997372591049));
#34322=CARTESIAN_POINT('Ctrl Pts',(-13.0373921036912,-33.4948908274866,
23.7964013663375));
#34323=CARTESIAN_POINT('Ctrl Pts',(-13.0255573302067,-33.4712399426843,
23.7948597426906));
#34324=CARTESIAN_POINT('Ctrl Pts',(-12.9983125042682,-33.4183491415447,
23.7914127065048));
#34325=CARTESIAN_POINT('Ctrl Pts',(-12.9827490387604,-33.3891910128053,
23.7895127638632));
#34326=CARTESIAN_POINT('Ctrl Pts',(-12.9337345732362,-33.3005095107186,
23.7837314481919));
#34327=CARTESIAN_POINT('Ctrl Pts',(-12.8989087696405,-33.2417635878976,
23.7798980772683));
#34328=CARTESIAN_POINT('Ctrl Pts',(-12.7279484206883,-32.9722846198199,
23.7622230869209));
#34329=CARTESIAN_POINT('Ctrl Pts',(-12.5704730652143,-32.7760384464127,
23.7491527600519));
#34330=CARTESIAN_POINT('Ctrl Pts',(-12.2903356675787,-32.4968648057453,
23.7280551933204));
#34331=CARTESIAN_POINT('Ctrl Pts',(-12.1814707797683,-32.4014427254085,
23.7202398678366));
#34332=CARTESIAN_POINT('Ctrl Pts',(-12.044442129159,-32.2960285951779,23.7103947022976));
#34333=CARTESIAN_POINT('Ctrl Pts',(-12.0218109396094,-32.2790653460101,
23.7087683334301));
#34334=CARTESIAN_POINT('Ctrl Pts',(-11.9856313116043,-32.2526474236907,
23.7061631400269));
#34335=CARTESIAN_POINT('Ctrl Pts',(-11.9722209738447,-32.2430048441155,
23.7051963938343));
#34336=CARTESIAN_POINT('Ctrl Pts',(-11.9462019749968,-32.2245830984589,
23.7033174543664));
#34337=CARTESIAN_POINT('Ctrl Pts',(-11.9336032485929,-32.2157910373626,
23.7024061179539));
#34338=CARTESIAN_POINT('Ctrl Pts',(-11.9021829762087,-32.1941804127002,
23.7001303088349));
#34339=CARTESIAN_POINT('Ctrl Pts',(-11.8832913539988,-32.1814654081235,
23.6987593502386));
#34340=CARTESIAN_POINT('Ctrl Pts',(-11.8089228310228,-32.1324931578094,
23.6933567634038));
#34341=CARTESIAN_POINT('Ctrl Pts',(-11.7525185632101,-32.097677687176,23.6892471682913));
#34342=CARTESIAN_POINT('Ctrl Pts',(-11.5919337201054,-32.0049450740948,
23.677588285181));
#34343=CARTESIAN_POINT('Ctrl Pts',(-11.485666761563,-31.9508363905632,23.6699224755694));
#34344=CARTESIAN_POINT('Ctrl Pts',(-11.1494196489394,-31.8013842420114,
23.6462064915628));
#34345=CARTESIAN_POINT('Ctrl Pts',(-10.9115910377708,-31.7256532180256,
23.6302435018371));
#34346=CARTESIAN_POINT('Ctrl Pts',(-10.6177630574535,-31.6666298512308,
23.6120250663025));
#34347=CARTESIAN_POINT('Ctrl Pts',(-10.5677176320278,-31.6577425514174,
23.6089694134727));
#34348=CARTESIAN_POINT('Ctrl Pts',(-10.4878875144455,-31.6454109039628,
23.6041681220882));
#34349=CARTESIAN_POINT('Ctrl Pts',(-10.4582258686399,-31.641230676341,23.6024000039088));
#34350=CARTESIAN_POINT('Ctrl Pts',(-10.4022184996779,-31.634093299625,23.5990901980501));
#34351=CARTESIAN_POINT('Ctrl Pts',(-10.375886093528,-31.6310510035616,23.597545988276));
#34352=CARTESIAN_POINT('Ctrl Pts',(-10.3159377033617,-31.6248365476773,
23.594056322629));
#34353=CARTESIAN_POINT('Ctrl Pts',(-10.2823043038806,-31.6218571138223,
23.5921169396167));
#34354=CARTESIAN_POINT('Ctrl Pts',(-10.176476420174,-31.6140738938347,23.5860681692523));
#34355=CARTESIAN_POINT('Ctrl Pts',(-10.1041672257485,-31.6110783824963,
23.5820137802031));
#34356=CARTESIAN_POINT('Ctrl Pts',(-9.92981888811991,-31.6094419995471,
23.5723810027352));
#34357=CARTESIAN_POINT('Ctrl Pts',(-9.82782854056136,-31.6130887499518,
23.5668648654558));
#34358=CARTESIAN_POINT('Ctrl Pts',(-9.67834119998528,-31.6252049403332,
23.5588418623242));
#34359=CARTESIAN_POINT('Ctrl Pts',(-9.63061625344907,-31.6300946865812,
23.5562894306932));
#34360=CARTESIAN_POINT('Ctrl Pts',(-9.37553546434112,-31.6617135406022,
23.5426422736755));
#34361=CARTESIAN_POINT('Ctrl Pts',(-9.17090401804028,-31.7065677367936,
23.5317006181288));
#34362=CARTESIAN_POINT('Ctrl Pts',(-8.92769650464525,-31.7839922848569,
23.5174472563382));
#34363=CARTESIAN_POINT('Ctrl Pts',(-8.88395749993603,-31.7989081360397,
23.5148314732064));
#34364=CARTESIAN_POINT('Ctrl Pts',(-8.82308213222965,-31.8210670772726,
23.5110992809424));
#34365=CARTESIAN_POINT('Ctrl Pts',(-8.80567792500265,-31.8275648245501,
23.5100216110964));
#34366=CARTESIAN_POINT('Ctrl Pts',(-8.77423336622413,-31.8395998677479,
23.5080537301525));
#34367=CARTESIAN_POINT('Ctrl Pts',(-8.76017468979705,-31.8450885858741,
23.5071662710338));
#34368=CARTESIAN_POINT('Ctrl Pts',(-8.73061981882877,-31.8568553092986,
23.5052836951311));
#34369=CARTESIAN_POINT('Ctrl Pts',(-8.71513285466987,-31.8631542939036,
23.5042874550362));
#34370=CARTESIAN_POINT('Ctrl Pts',(-8.67270184314376,-31.8807791171718,
23.5015323352365));
#34371=CARTESIAN_POINT('Ctrl Pts',(-8.64585730445979,-31.8923390229004,
23.4997606834218));
#34372=CARTESIAN_POINT('Ctrl Pts',(-8.58538190791726,-31.9193135169226,
23.495709802704));
#34373=CARTESIAN_POINT('Ctrl Pts',(-8.55184741881983,-31.9349343487788,
23.4934210799052));
#34374=CARTESIAN_POINT('Ctrl Pts',(-8.44183160161243,-31.9883896988216,
23.4857864734567));
#34375=CARTESIAN_POINT('Ctrl Pts',(-8.36652570751825,-32.0285616975968,
23.4803568245721));
#34376=CARTESIAN_POINT('Ctrl Pts',(-8.05252377068077,-32.2116121589933,
23.4570484137369));
#34377=CARTESIAN_POINT('Ctrl Pts',(-7.83033880105019,-32.3807663672527,
23.4389671628804));
#34378=CARTESIAN_POINT('Ctrl Pts',(-7.58611001355821,-32.619341809599,23.4180304098819));
#34379=CARTESIAN_POINT('Ctrl Pts',(-7.54214797958754,-32.6647564308409,
23.4142055918965));
#34380=CARTESIAN_POINT('Ctrl Pts',(-7.47752579955761,-32.7353617871283,
23.4084937506741));
#34381=CARTESIAN_POINT('Ctrl Pts',(-7.4559182686312,-32.7596628419597,23.4065677043994));
#34382=CARTESIAN_POINT('Ctrl Pts',(-7.41739843860323,-32.8042605205775,
23.4031031527287));
#34383=CARTESIAN_POINT('Ctrl Pts',(-7.40036758741181,-32.8244508591349,
23.4015598915683));
#34384=CARTESIAN_POINT('Ctrl Pts',(-7.36397387653125,-32.8686338372851,
23.3982357845438));
#34385=CARTESIAN_POINT('Ctrl Pts',(-7.34469873556579,-32.892695862372,23.3964585036294));
#34386=CARTESIAN_POINT('Ctrl Pts',(-7.29102497250578,-32.9616051704085,
23.3914583848634));
#34387=CARTESIAN_POINT('Ctrl Pts',(-7.25741513543777,-33.0070554569765,
23.3882658807429));
#34388=CARTESIAN_POINT('Ctrl Pts',(-7.18337160049578,-33.1126068471707,
23.381068797031));
#34389=CARTESIAN_POINT('Ctrl Pts',(-7.14369575630167,-33.1732062564826,
23.3770903832142));
#34390=CARTESIAN_POINT('Ctrl Pts',(-7.00485319900036,-33.4008658753611,
23.3626102640712));
#34391=CARTESIAN_POINT('Ctrl Pts',(-6.91815847123986,-33.5750830210797,
23.3524430407306));
#34392=CARTESIAN_POINT('Ctrl Pts',(-6.79268960287007,-33.893046966402,23.3342191521376));
#34393=CARTESIAN_POINT('Ctrl Pts',(-6.74754754833187,-34.0337034603451,
23.3262533069705));
#34394=CARTESIAN_POINT('Ctrl Pts',(-6.70484501038276,-34.2042868580791,
23.3162396105382));
#34395=CARTESIAN_POINT('Ctrl Pts',(-6.69831751718405,-34.2318213218514,
23.3146124203341));
#34396=CARTESIAN_POINT('Ctrl Pts',(-6.68852646295664,-34.2755546937307,
23.3120062135951));
#34397=CARTESIAN_POINT('Ctrl Pts',(-6.68503518335092,-34.2917018793287,
23.311039291401));
#34398=CARTESIAN_POINT('Ctrl Pts',(-6.67852550614222,-34.3229119404873,
23.3091602787077));
#34399=CARTESIAN_POINT('Ctrl Pts',(-6.67549125330258,-34.3379708370795,
23.3082490486839));
#34400=CARTESIAN_POINT('Ctrl Pts',(-6.6682151032405,-34.3753940263804,23.3059738966956));
#34401=CARTESIAN_POINT('Ctrl Pts',(-6.66409596913806,-34.3977812227259,
23.3046034968694));
#34402=CARTESIAN_POINT('Ctrl Pts',(-6.64887998274017,-34.4854303592358,
23.2992061160042));
#34403=CARTESIAN_POINT('Ctrl Pts',(-6.63947099576578,-34.5509666784846,
23.2951013509861));
#34404=CARTESIAN_POINT('Ctrl Pts',(-6.61853837241558,-34.7349144495417,
23.2834619016546));
#34405=CARTESIAN_POINT('Ctrl Pts',(-6.61132000297716,-34.8537179595692,
23.275811096451));
#34406=CARTESIAN_POINT('Ctrl Pts',(-6.6083495691758,-35.2218460701567,23.2520840295923));
#34407=CARTESIAN_POINT('Ctrl Pts',(-6.63382522673741,-35.4705450740019,
23.2360941190474));
#34408=CARTESIAN_POINT('Ctrl Pts',(-6.69717401394581,-35.7644508238692,
23.2178180705981));
#34409=CARTESIAN_POINT('Ctrl Pts',(-6.70913984768951,-35.8144227689762,
23.214729481356));
#34410=CARTESIAN_POINT('Ctrl Pts',(-6.72983157683658,-35.8929115307665,
23.2099062043782));
#34411=CARTESIAN_POINT('Ctrl Pts',(-6.73780518433496,-35.9216168331301,
23.208148133519));
#34412=CARTESIAN_POINT('Ctrl Pts',(-6.75359432906417,-35.9756840309177,
23.2048469589763));
#34413=CARTESIAN_POINT('Ctrl Pts',(-6.76133124597041,-36.0010663659831,
23.2033014848752));
#34414=CARTESIAN_POINT('Ctrl Pts',(-6.77967087247175,-36.0587935497158,
23.1997952246571));
#34415=CARTESIAN_POINT('Ctrl Pts',(-6.79046439546347,-36.0910750632311,
23.197840742505));
#34416=CARTESIAN_POINT('Ctrl Pts',(-6.82624766654928,-36.1929671506637,
23.1916870361398));
#34417=CARTESIAN_POINT('Ctrl Pts',(-6.85303081167555,-36.2619272978937,
23.1875456924529));
#34418=CARTESIAN_POINT('Ctrl Pts',(-6.92336364909026,-36.4268152097634,
23.177651218374));
#34419=CARTESIAN_POINT('Ctrl Pts',(-6.96916961968725,-36.5216971093717,
23.1719653453803));
#34420=CARTESIAN_POINT('Ctrl Pts',(-7.07844932709289,-36.7234739894091,
23.1597045524583));
#34421=CARTESIAN_POINT('Ctrl Pts',(-7.14353171380071,-36.8293195196082,
23.1531629979742));
#34422=CARTESIAN_POINT('Ctrl Pts',(-7.2967195397611,-37.050272731669,23.1388533510533));
#34423=CARTESIAN_POINT('Ctrl Pts',(-7.3866876373612,-37.1637777684862,23.1310761063742));
#34424=CARTESIAN_POINT('Ctrl Pts',(-7.50750583466518,-37.2976398027246,
23.1208944759729));
#34425=CARTESIAN_POINT('Ctrl Pts',(-7.53180529102275,-37.3237234119275,
23.1188583384088));
#34426=CARTESIAN_POINT('Ctrl Pts',(-7.56901104871671,-37.3624189025289,
23.1157492339123));
#34427=CARTESIAN_POINT('Ctrl Pts',(-7.58161481919966,-37.3753196496195,
23.114697417928));
#34428=CARTESIAN_POINT('Ctrl Pts',(-7.60484838214149,-37.3987240552316,
23.1127597160731));
#34429=CARTESIAN_POINT('Ctrl Pts',(-7.61544553135115,-37.409258874664,23.1118762394365));
#34430=CARTESIAN_POINT('Ctrl Pts',(-7.64024227225387,-37.4335859070175,
23.1098098917815));
#34431=CARTESIAN_POINT('Ctrl Pts',(-7.65449335541902,-37.4473241385295,
23.108623158207));
#34432=CARTESIAN_POINT('Ctrl Pts',(-7.70176408991363,-37.4921016191482,
23.1046919583316));
#34433=CARTESIAN_POINT('Ctrl Pts',(-7.73528464685746,-37.5226023718299,
23.101912503679));
#34434=CARTESIAN_POINT('Ctrl Pts',(-7.81979828322199,-37.5964600003939,
23.0949464048634));
#34435=CARTESIAN_POINT('Ctrl Pts',(-7.87148258168086,-37.63899540643,23.0907224553632));
#34436=CARTESIAN_POINT('Ctrl Pts',(-8.1458523419351,-37.8514920644522,23.0686147340667));
#34437=CARTESIAN_POINT('Ctrl Pts',(-8.38776326914076,-37.9949289257836,
23.0502821308231));
#34438=CARTESIAN_POINT('Ctrl Pts',(-8.71874056877548,-38.1393195935546,
23.0278973259944));
#34439=CARTESIAN_POINT('Ctrl Pts',(-8.79404962947304,-38.1690122402669,
23.0229585723145));
#34440=CARTESIAN_POINT('Ctrl Pts',(-8.90107521646151,-38.2068412908393,
23.0161532775115));
#34441=CARTESIAN_POINT('Ctrl Pts',(-8.93195185394021,-38.2172565973856,
23.0142141750579));
#34442=CARTESIAN_POINT('Ctrl Pts',(-8.98864838219097,-38.2354752612977,
23.0106965705255));
#34443=CARTESIAN_POINT('Ctrl Pts',(-9.01442012981425,-38.2434186660722,
23.0091136654869));
#34444=CARTESIAN_POINT('Ctrl Pts',(-9.0670627654046,-38.2589588434761,23.0059119239557));
#34445=CARTESIAN_POINT('Ctrl Pts',(-9.09393824325474,-38.2665328389706,
23.0042939209376));
#34446=CARTESIAN_POINT('Ctrl Pts',(-9.16171958338777,-38.2847339264534,
23.0002530266599));
#34447=CARTESIAN_POINT('Ctrl Pts',(-9.20273691397202,-38.2949298656002,
22.9978438952389));
#34448=CARTESIAN_POINT('Ctrl Pts',(-9.38472826244784,-38.3365710134546,
22.9873002152675));
#34449=CARTESIAN_POINT('Ctrl Pts',(-9.52744338117719,-38.3597562075392,
22.9794232391571));
#34450=CARTESIAN_POINT('Ctrl Pts',(-9.80296663439148,-38.3866069115911,
22.9645827992421));
#34451=CARTESIAN_POINT('Ctrl Pts',(-9.93535907813262,-38.3917179258534,
22.9576091044348));
#34452=CARTESIAN_POINT('Ctrl Pts',(-10.2186965811993,-38.3860571144902,
22.942541361258));
#34453=CARTESIAN_POINT('Ctrl Pts',(-10.3692987441442,-38.3729543115252,
22.9344442747116));
#34454=CARTESIAN_POINT('Ctrl Pts',(-10.5540816896695,-38.3443525882184,
22.9238903774055));
#34455=CARTESIAN_POINT('Ctrl Pts',(-10.5895623520611,-38.3382805109371,
22.9218349557408));
#34456=CARTESIAN_POINT('Ctrl Pts',(-10.6427316386463,-38.3283072054364,
22.9187022627679));
#34457=CARTESIAN_POINT('Ctrl Pts',(-10.6604977367765,-38.324827141485,22.9176466241199));
#34458=CARTESIAN_POINT('Ctrl Pts',(-10.6927295424391,-38.3182449738906,
22.9157139182871));
#34459=CARTESIAN_POINT('Ctrl Pts',(-10.707204038937,-38.3151902431169,22.9148394291914));
#34460=CARTESIAN_POINT('Ctrl Pts',(-10.7408253945437,-38.3078645112366,
22.9127930148259));
#34461=CARTESIAN_POINT('Ctrl Pts',(-10.7599555812798,-38.3035219635617,
22.9116172838046));
#34462=CARTESIAN_POINT('Ctrl Pts',(-10.8221293671421,-38.2888399181798,
22.9077615000137));
#34463=CARTESIAN_POINT('Ctrl Pts',(-10.8650067016278,-38.2778236247112,
22.9050481984178));
#34464=CARTESIAN_POINT('Ctrl Pts',(-10.9700398998716,-38.2486336029008,
22.8982875606185));
#34465=CARTESIAN_POINT('Ctrl Pts',(-11.0319134454529,-38.2295125786671,
22.8942054631409));
#34466=CARTESIAN_POINT('Ctrl Pts',(-11.3327138817197,-38.1270282713596,
22.8739821659142));
#34467=CARTESIAN_POINT('Ctrl Pts',(-11.5623694805042,-38.0188497286454,
22.8574312179954));
#34468=CARTESIAN_POINT('Ctrl Pts',(-11.866314326056,-37.8316201889597,22.8350626703784));
#34469=CARTESIAN_POINT('Ctrl Pts',(-11.9522381613845,-37.7730798005677,
22.8286684304963));
#34470=CARTESIAN_POINT('Ctrl Pts',(-12.0668419958852,-37.6870282359272,
22.8200471030434));
#34471=CARTESIAN_POINT('Ctrl Pts',(-12.0979266917168,-37.6628293916601,
22.8176983664549));
#34472=CARTESIAN_POINT('Ctrl Pts',(-12.1496678465436,-37.6210812983317,
22.813769678177));
#34473=CARTESIAN_POINT('Ctrl Pts',(-12.170547861932,-37.6038166343889,22.812178805928));
#34474=CARTESIAN_POINT('Ctrl Pts',(-12.212396890734,-37.5683604687079,22.8089781632739));
#34475=CARTESIAN_POINT('Ctrl Pts',(-12.2333539214903,-37.5501580005037,
22.8073690099432));
#34476=CARTESIAN_POINT('Ctrl Pts',(-12.285030989637,-37.504147596669,22.8033834211524));
#34477=CARTESIAN_POINT('Ctrl Pts',(-12.3154696284277,-37.4760295677066,
22.8010199366185));
#34478=CARTESIAN_POINT('Ctrl Pts',(-12.4421539997109,-37.3546237252692,
22.791102545365));
#34479=CARTESIAN_POINT('Ctrl Pts',(-12.5333419419097,-37.2562253356138,
22.7837673076984));
#34480=CARTESIAN_POINT('Ctrl Pts',(-12.706761857214,-37.045281055661,22.7690831906271));
#34481=CARTESIAN_POINT('Ctrl Pts',(-12.7883638456398,-36.9325532897672,
22.7617578250463));
#34482=CARTESIAN_POINT('Ctrl Pts',(-12.9467634478842,-36.6827267903299,
22.7460410038403));
#34483=CARTESIAN_POINT('Ctrl Pts',(-13.0214195153088,-36.5446678894903,
22.7376510464476));
#34484=CARTESIAN_POINT('Ctrl Pts',(-13.10107390006,-36.3693176155241,22.7267787654395));
#34485=CARTESIAN_POINT('Ctrl Pts',(-13.1153804520665,-36.3364484616631,
22.7247315884129));
#34486=CARTESIAN_POINT('Ctrl Pts',(-13.1361122373471,-36.2866747048548,
22.7216089787021));
#34487=CARTESIAN_POINT('Ctrl Pts',(-13.1429282742043,-36.2699344836114,
22.7205549721204));
#34488=CARTESIAN_POINT('Ctrl Pts',(-13.1551328274853,-36.2392598959705,
22.7186153364739));
#34489=CARTESIAN_POINT('Ctrl Pts',(-13.1605635675376,-36.2253432817686,
22.7177321533613));
#34490=CARTESIAN_POINT('Ctrl Pts',(-13.1729575065669,-36.1929524264085,
22.7156692917471));
#34491=CARTESIAN_POINT('Ctrl Pts',(-13.1798514675643,-36.1744528228081,
22.7144857970722));
#34492=CARTESIAN_POINT('Ctrl Pts',(-13.2019304779914,-36.1135851557525,
22.7105769156143));
#34493=CARTESIAN_POINT('Ctrl Pts',(-13.2164327785833,-36.0709764013763,
22.7078170598837));
#34494=CARTESIAN_POINT('Ctrl Pts',(-13.2501833991684,-35.9649381586313,
22.7009120606399));
#34495=CARTESIAN_POINT('Ctrl Pts',(-13.2684274840359,-35.9012095623811,
22.6967303772893));
#34496=CARTESIAN_POINT('Ctrl Pts',(-13.3543056274298,-35.564178620736,22.6745805635256));
#34497=CARTESIAN_POINT('Ctrl Pts',(-13.3895698991912,-35.2837309463288,
22.6561515965784));
#34498=CARTESIAN_POINT('Ctrl Pts',(-13.3897493118742,-35.0021598954043,
22.6386988750799));
#34499=CARTESIAN_POINT('Ctrl Pts',(-13.3897493143655,-35.0021559820986,
22.6386986325201));
#34500=CARTESIAN_POINT('Ctrl Pts',(-13.3897813530779,-34.9517830205386,
22.6355763483221));
#34501=CARTESIAN_POINT('Ctrl Pts',(-13.3886905509555,-34.9014133179565,
22.6324836405767));
#34502=CARTESIAN_POINT('Ctrl Pts',(-13.3847480855858,-34.8117581780564,
22.6270320201307));
#34503=CARTESIAN_POINT('Ctrl Pts',(-13.3823338406184,-34.7724641323813,
22.6246609047137));
#34504=CARTESIAN_POINT('Ctrl Pts',(-13.3771513033993,-34.70681828144,22.6207292907024));
#34505=CARTESIAN_POINT('Ctrl Pts',(-13.3747576087104,-34.6804415728901,
22.6191575733152));
#34506=CARTESIAN_POINT('Ctrl Pts',(-13.3694901319793,-34.6290915669839,
22.616112774202));
#34507=CARTESIAN_POINT('Ctrl Pts',(-13.3666472101612,-34.6041169008927,
22.6146388442416));
#34508=CARTESIAN_POINT('Ctrl Pts',(-13.360026987176,-34.5512033824149,22.6115299700426));
#34509=CARTESIAN_POINT('Ctrl Pts',(-13.3561783860098,-34.5232752685115,
22.6098973538604));
#34510=CARTESIAN_POINT('Ctrl Pts',(-13.3454914997547,-34.4522842053785,
22.605766655022));
#34511=CARTESIAN_POINT('Ctrl Pts',(-13.3381698616087,-34.4092985647781,
22.6032836747446));
#34512=CARTESIAN_POINT('Ctrl Pts',(-13.3010067134662,-34.2139597188259,
22.5920679108909));
#34513=CARTESIAN_POINT('Ctrl Pts',(-13.261549413046,-34.0636201719023,22.5836355080249));
#34514=CARTESIAN_POINT('Ctrl Pts',(-13.201321222039,-33.8850797250537,22.5735646774699));
#34515=CARTESIAN_POINT('Ctrl Pts',(-13.1902628614254,-33.8538207821783,
22.5717987757316));
#34516=CARTESIAN_POINT('Ctrl Pts',(-13.1787501379842,-33.8227351093465,
22.5700367124769));
#34517=CARTESIAN_POINT('Ctrl Pts',(-13.1787501240202,-33.8227350716421,
22.9104831197053));
#34518=CARTESIAN_POINT('Ctrl Pts',(-13.1790010828795,-33.8234126893014,
22.9105272782207));
#34519=CARTESIAN_POINT('Ctrl Pts',(-13.1792518250776,-33.8240903872375,
22.9105714467413));
#34520=CARTESIAN_POINT('Ctrl Pts',(-13.2379593845312,-33.9829193244527,
22.9209241292555));
#34521=CARTESIAN_POINT('Ctrl Pts',(-13.2845300383789,-34.1451980259089,
22.931747794009));
#34522=CARTESIAN_POINT('Ctrl Pts',(-13.3479888900709,-34.4505396763261,
22.9518445278896));
#34523=CARTESIAN_POINT('Ctrl Pts',(-13.3682219700549,-34.5925434889456,
22.9610882235064));
#34524=CARTESIAN_POINT('Ctrl Pts',(-13.3862516589892,-34.8228200820771,
22.9756971533644));
#34525=CARTESIAN_POINT('Ctrl Pts',(-13.3897019623642,-34.9104709072447,
22.9811718835349));
#34526=CARTESIAN_POINT('Ctrl Pts',(-13.3897847493606,-35.0631798689789,
22.9905426671675));
#34527=CARTESIAN_POINT('Ctrl Pts',(-13.3879493868013,-35.1281879909346,
22.994479274308));
#34528=CARTESIAN_POINT('Ctrl Pts',(-13.3823960453813,-35.2255117986716,
23.0002961702296));
#34529=CARTESIAN_POINT('Ctrl Pts',(-13.3800816042195,-35.2578895846344,
23.0022186676488));
#34530=CARTESIAN_POINT('Ctrl Pts',(-13.3750412122609,-35.3165428174658,
23.0056794712165));
#34531=CARTESIAN_POINT('Ctrl Pts',(-13.3724725330889,-35.3428288374107,
23.0072224844828));
#34532=CARTESIAN_POINT('Ctrl Pts',(-13.366235136149,-35.399774102426,23.0105489599472));
#34533=CARTESIAN_POINT('Ctrl Pts',(-13.3624541712792,-35.4304188209739,
23.0123288159882));
#34534=CARTESIAN_POINT('Ctrl Pts',(-13.3505366499884,-35.5172330286673,
23.0173447067182));
#34535=CARTESIAN_POINT('Ctrl Pts',(-13.3414072947925,-35.5732570585567,
23.0205500901092));
#34536=CARTESIAN_POINT('Ctrl Pts',(-13.3173626238281,-35.7005802010372,
23.0277817467983));
#34537=CARTESIAN_POINT('Ctrl Pts',(-13.3015475742769,-35.771681205236,23.0317814653936));
#34538=CARTESIAN_POINT('Ctrl Pts',(-13.2346130159345,-36.03263006282,23.0464064850513));
#34539=CARTESIAN_POINT('Ctrl Pts',(-13.1693029993633,-36.2184275686629,
23.056689182484));
#34540=CARTESIAN_POINT('Ctrl Pts',(-13.0286963490147,-36.5291421174995,
23.0748829678814));
#34541=CARTESIAN_POINT('Ctrl Pts',(-12.9607857935857,-36.656809011298,23.0826901502761));
#34542=CARTESIAN_POINT('Ctrl Pts',(-12.8700995577321,-36.803810810818,23.0925261908049));
#34543=CARTESIAN_POINT('Ctrl Pts',(-12.8549505486745,-36.827693126973,23.0941524954441));
#34544=CARTESIAN_POINT('Ctrl Pts',(-12.8304838875117,-36.8652181744952,
23.0967576094203));
#34545=CARTESIAN_POINT('Ctrl Pts',(-12.8213619502363,-36.8789876521033,
23.0977243416623));
#34546=CARTESIAN_POINT('Ctrl Pts',(-12.803561480858,-36.9054354178798,23.0996032748626));
#34547=CARTESIAN_POINT('Ctrl Pts',(-12.7948968044657,-36.9181222397981,
23.1005146192387));
#34548=CARTESIAN_POINT('Ctrl Pts',(-12.7731754228395,-36.9494670392508,
23.1027904785544));
#34549=CARTESIAN_POINT('Ctrl Pts',(-12.7600164756916,-36.9680530112449,
23.104161480002));
#34550=CARTESIAN_POINT('Ctrl Pts',(-12.7078295433343,-37.040210096098,23.1095644683791));
#34551=CARTESIAN_POINT('Ctrl Pts',(-12.6674231164322,-37.0927615279647,
23.1136744363155));
#34552=CARTESIAN_POINT('Ctrl Pts',(-12.550115483698,-37.2364083187136,23.1253348210549));
#34553=CARTESIAN_POINT('Ctrl Pts',(-12.4699123664173,-37.3246809491208,
23.1330017904794));
#34554=CARTESIAN_POINT('Ctrl Pts',(-12.208469436395,-37.5835935496903,23.1567169218281));
#34555=CARTESIAN_POINT('Ctrl Pts',(-12.0129456059501,-37.738682096861,23.1726778351449));
#34556=CARTESIAN_POINT('Ctrl Pts',(-11.7591371750142,-37.8980035332952,
23.1908946337718));
#34557=CARTESIAN_POINT('Ctrl Pts',(-11.7154879285399,-37.9240536358084,
23.1939504911727));
#34558=CARTESIAN_POINT('Ctrl Pts',(-11.6452077499257,-37.9638815313459,
23.198752026844));
#34559=CARTESIAN_POINT('Ctrl Pts',(-11.6189527653518,-37.9783039304401,
23.2005201886356));
#34560=CARTESIAN_POINT('Ctrl Pts',(-11.5691106555619,-38.0048293431154,
23.2038300318621));
#34561=CARTESIAN_POINT('Ctrl Pts',(-11.5455661723416,-38.0170072748266,
23.2053742360527));
#34562=CARTESIAN_POINT('Ctrl Pts',(-11.4917134558521,-38.0440656774081,
23.208863829948));
#34563=CARTESIAN_POINT('Ctrl Pts',(-11.4613206427465,-38.0587721358313,
23.2108031477835));
#34564=CARTESIAN_POINT('Ctrl Pts',(-11.3651291295619,-38.1035561850087,
23.2168514704541));
#34565=CARTESIAN_POINT('Ctrl Pts',(-11.2985824090147,-38.1319839204299,
23.2209054890995));
#34566=CARTESIAN_POINT('Ctrl Pts',(-11.1361526102051,-38.1953033271573,
23.2305371594068));
#34567=CARTESIAN_POINT('Ctrl Pts',(-11.0395045968132,-38.228039371375,23.2360525806019));
#34568=CARTESIAN_POINT('Ctrl Pts',(-10.8954870939265,-38.2696795590069,
23.2440723574039));
#34569=CARTESIAN_POINT('Ctrl Pts',(-10.8491734664789,-38.2820125034578,
23.2466223021425));
#34570=CARTESIAN_POINT('Ctrl Pts',(-10.5996175873226,-38.3428309209478,
23.2602603601131));
#34571=CARTESIAN_POINT('Ctrl Pts',(-10.3925017358387,-38.3734234894795,
23.2711953993331));
#34572=CARTESIAN_POINT('Ctrl Pts',(-10.1376333653962,-38.3872717712888,
23.2854476542762));
#34573=CARTESIAN_POINT('Ctrl Pts',(-10.0913114128663,-38.3888367903651,
23.2880708896157));
#34574=CARTESIAN_POINT('Ctrl Pts',(-10.0263759546072,-38.3896984131283,
23.291812027625));
#34575=CARTESIAN_POINT('Ctrl Pts',(-10.0077763137609,-38.3897921054777,
23.2928909476672));
#34576=CARTESIAN_POINT('Ctrl Pts',(-9.97408011176945,-38.3896845206079,
23.2948603665365));
#34577=CARTESIAN_POINT('Ctrl Pts',(-9.95898363218618,-38.3895354610581,
23.2957480976578));
#34578=CARTESIAN_POINT('Ctrl Pts',(-9.92718395915454,-38.3890090010259,
23.2976302029118));
#34579=CARTESIAN_POINT('Ctrl Pts',(-9.91048195208024,-38.388608959139,23.2986256876876));
#34580=CARTESIAN_POINT('Ctrl Pts',(-9.86462781526631,-38.387171438149,23.3013765621024));
#34581=CARTESIAN_POINT('Ctrl Pts',(-9.83548571069105,-38.3858811119874,
23.303144661988));
#34582=CARTESIAN_POINT('Ctrl Pts',(-9.6252057363491,-38.3738494978915,23.3160286331056));
#34583=CARTESIAN_POINT('Ctrl Pts',(-9.44518642037493,-38.3489553476491,
23.3277180509822));
#34584=CARTESIAN_POINT('Ctrl Pts',(-9.03521032534632,-38.2582890758964,
23.3547840198888));
#34585=CARTESIAN_POINT('Ctrl Pts',(-8.80842727543235,-38.1823660636285,
23.3700538834943));
#34586=CARTESIAN_POINT('Ctrl Pts',(-8.54436482382719,-38.0617336899138,
23.387714922686));
#34587=CARTESIAN_POINT('Ctrl Pts',(-8.49775787613767,-38.0391373772526,
23.390830489602));
#34588=CARTESIAN_POINT('Ctrl Pts',(-8.42485451841121,-38.0017047546445,
23.3957033796484));
#34589=CARTESIAN_POINT('Ctrl Pts',(-8.39820847715695,-37.9875707067175,
23.3974843336162));
#34590=CARTESIAN_POINT('Ctrl Pts',(-8.35085531054139,-37.9616371497472,
23.4006501625686));
#34591=CARTESIAN_POINT('Ctrl Pts',(-8.33007753945989,-37.9499714968297,
23.4020395824929));
#34592=CARTESIAN_POINT('Ctrl Pts',(-8.28157722534894,-37.9220644103186,
23.4052844318827));
#34593=CARTESIAN_POINT('Ctrl Pts',(-8.25395890360866,-37.9056458562175,
23.4071334417713));
#34594=CARTESIAN_POINT('Ctrl Pts',(-8.17268069860289,-37.8557501323348,
23.4125821060863));
#34595=CARTESIAN_POINT('Ctrl Pts',(-8.11971828912701,-37.8211604057424,
23.416141774823));
#34596=CARTESIAN_POINT('Ctrl Pts',(-7.93654824841711,-37.6940809644331,
23.4285286780925));
#34597=CARTESIAN_POINT('Ctrl Pts',(-7.81193341496044,-37.5938920255088,
23.4370847052617));
#34598=CARTESIAN_POINT('Ctrl Pts',(-7.54701195905143,-37.3481712643646,
23.4562779408289));
#34599=CARTESIAN_POINT('Ctrl Pts',(-7.41172423186079,-37.1981524233418,
23.4668293920215));
#34600=CARTESIAN_POINT('Ctrl Pts',(-7.25753326725108,-36.9930642822274,
23.4810612625621));
#34601=CARTESIAN_POINT('Ctrl Pts',(-7.22556390326457,-36.9483153418577,
23.4841575152034));
#34602=CARTESIAN_POINT('Ctrl Pts',(-7.18243226498748,-36.8847266767542,
23.4885743706552));
#34603=CARTESIAN_POINT('Ctrl Pts',(-7.17034112097579,-36.8665243533994,
23.4898406012223));
#34604=CARTESIAN_POINT('Ctrl Pts',(-7.15013825211101,-36.8354629376268,
23.4920068378794));
#34605=CARTESIAN_POINT('Ctrl Pts',(-7.14193531276381,-36.822663549731,23.492901052687));
#34606=CARTESIAN_POINT('Ctrl Pts',(-7.12480973069822,-36.7955418959299,
23.4947999599309));
#34607=CARTESIAN_POINT('Ctrl Pts',(-7.11590761350785,-36.7812076982218,
23.4958058059921));
#34608=CARTESIAN_POINT('Ctrl Pts',(-7.09149913517007,-36.7412424228365,
23.4986151084747));
#34609=CARTESIAN_POINT('Ctrl Pts',(-7.07622533069247,-36.715471948305,23.5004321375612));
#34610=CARTESIAN_POINT('Ctrl Pts',(-6.97673175715375,-36.5424138805786,
23.5126535679864));
#34611=CARTESIAN_POINT('Ctrl Pts',(-6.90333759894026,-36.3891952764166,
23.5235547410299));
#34612=CARTESIAN_POINT('Ctrl Pts',(-6.75053742216397,-35.9972141772379,
23.5506687645879));
#34613=CARTESIAN_POINT('Ctrl Pts',(-6.68560622531708,-35.7538400602735,
23.5667839378455));
#34614=CARTESIAN_POINT('Ctrl Pts',(-6.64052294392229,-35.4549034333119,
23.5851580632396));
#34615=CARTESIAN_POINT('Ctrl Pts',(-6.63403877164963,-35.4041394072019,
23.5882337708725));
#34616=CARTESIAN_POINT('Ctrl Pts',(-6.62560612918472,-35.3236602908664,
23.5930417801839));
#34617=CARTESIAN_POINT('Ctrl Pts',(-6.6228956525964,-35.2940345056107,23.5947972151775));
#34618=CARTESIAN_POINT('Ctrl Pts',(-6.61850537903817,-35.2379152297356,
23.5980961604659));
#34619=CARTESIAN_POINT('Ctrl Pts',(-6.61674612479648,-35.2114303740201,
23.5996420010538));
#34620=CARTESIAN_POINT('Ctrl Pts',(-6.61343724596228,-35.1508682745644,
23.6031527918713));
#34621=CARTESIAN_POINT('Ctrl Pts',(-6.61209054415758,-35.1167825455154,
23.6051113752996));
#34622=CARTESIAN_POINT('Ctrl Pts',(-6.60944386494779,-35.0083069601176,
23.6112938448838));
#34623=CARTESIAN_POINT('Ctrl Pts',(-6.6100781074341,-34.9338897022159,23.6154590467951));
#34624=CARTESIAN_POINT('Ctrl Pts',(-6.61756186888467,-34.753425244386,23.6254259231571));
#34625=CARTESIAN_POINT('Ctrl Pts',(-6.62694851964493,-34.6475619564078,
23.6311589136535));
#34626=CARTESIAN_POINT('Ctrl Pts',(-6.65796802398009,-34.4199289329964,
23.6434301671122));
#34627=CARTESIAN_POINT('Ctrl Pts',(-6.68132093506506,-34.2985518921759,
23.6499375610396));
#34628=CARTESIAN_POINT('Ctrl Pts',(-6.74609655649723,-34.0391626945003,
23.6641690918936));
#34629=CARTESIAN_POINT('Ctrl Pts',(-6.78979213682082,-33.901977345488,23.6719027159648));
#34630=CARTESIAN_POINT('Ctrl Pts',(-6.85500491518204,-33.7348205297763,
23.6820342088643));
#34631=CARTESIAN_POINT('Ctrl Pts',(-6.86846901528448,-33.7018526058065,
23.6840682832975));
#34632=CARTESIAN_POINT('Ctrl Pts',(-6.88952781414028,-33.6525235179322,
23.6871748631689));
#34633=CARTESIAN_POINT('Ctrl Pts',(-6.89673821474192,-33.6359998719865,
23.6882262688977));
#34634=CARTESIAN_POINT('Ctrl Pts',(-6.91016583274607,-33.6058862287929,
23.6901636098934));
#34635=CARTESIAN_POINT('Ctrl Pts',(-6.91634159756907,-33.5922787141369,
23.6910471428099));
#34636=CARTESIAN_POINT('Ctrl Pts',(-6.93091106840179,-33.5607326788209,
23.6931141493239));
#34637=CARTESIAN_POINT('Ctrl Pts',(-6.93937220442957,-33.5428264526464,
23.694301494231));
#34638=CARTESIAN_POINT('Ctrl Pts',(-6.96773465624343,-33.4841401759713,
23.6982369190404));
#34639=CARTESIAN_POINT('Ctrl Pts',(-6.9882971767302,-33.443687112948,23.7010200860654));
#34640=CARTESIAN_POINT('Ctrl Pts',(-7.04123950430119,-33.3445131015472,
23.707997780355));
#34641=CARTESIAN_POINT('Ctrl Pts',(-7.07456107777427,-33.2863177814506,
23.7122297590936));
#34642=CARTESIAN_POINT('Ctrl Pts',(-7.25681623951452,-32.9888370647024,
23.7344557312121));
#34643=CARTESIAN_POINT('Ctrl Pts',(-7.43347240524709,-32.7677798443104,
23.7529007125881));
#34644=CARTESIAN_POINT('Ctrl Pts',(-7.69267842377447,-32.5154378570647,
23.7753098168571));
#34645=CARTESIAN_POINT('Ctrl Pts',(-7.75185067938511,-32.4617706754214,
23.7801806313066));
#34646=CARTESIAN_POINT('Ctrl Pts',(-7.83753258748941,-32.3894096367838,
23.7869015435543));
#34647=CARTESIAN_POINT('Ctrl Pts',(-7.86249483829816,-32.3689319380587,
23.7888222420256));
#34648=CARTESIAN_POINT('Ctrl Pts',(-7.90878120517758,-32.3320546613213,
23.7923170393959));
#34649=CARTESIAN_POINT('Ctrl Pts',(-7.93001505060156,-32.3155464709985,
23.7938953333241));
#34650=CARTESIAN_POINT('Ctrl Pts',(-7.97377293734329,-32.282354984855,23.7970983145203));
#34651=CARTESIAN_POINT('Ctrl Pts',(-7.99631195689883,-32.2656948172535,
23.7987220349153));
#34652=CARTESIAN_POINT('Ctrl Pts',(-8.05377661773693,-32.224310822668,23.80279825973));
#34653=CARTESIAN_POINT('Ctrl Pts',(-8.08896908041864,-32.1999648362236,
23.8052364805353));
#34654=CARTESIAN_POINT('Ctrl Pts',(-8.25115199474961,-32.0922499406877,
23.8162264931445));
#34655=CARTESIAN_POINT('Ctrl Pts',(-8.38320221879958,-32.0168051495611,
23.8244906097043));
#34656=CARTESIAN_POINT('Ctrl Pts',(-8.56042531927445,-31.9307882131128,
23.8350306602775));
#34657=CARTESIAN_POINT('Ctrl Pts',(-8.60135950282255,-31.911919512682,23.837429898961));
#34658=CARTESIAN_POINT('Ctrl Pts',(-8.82835529851998,-31.8127249721091,
23.8505875494917));
#34659=CARTESIAN_POINT('Ctrl Pts',(-9.02093949721846,-31.7484003248942,
23.8611927633129));
#34660=CARTESIAN_POINT('Ctrl Pts',(-9.270449647207,-31.6892513907292,23.8754287775475));
#34661=CARTESIAN_POINT('Ctrl Pts',(-9.32308914197298,-31.6780892375746,
23.8784605562108));
#34662=CARTESIAN_POINT('Ctrl Pts',(-9.39725792566655,-31.6641978213119,
23.8827996267804));
#34663=CARTESIAN_POINT('Ctrl Pts',(-9.41858407477265,-31.6604147483941,
23.8840550111149));
#34664=CARTESIAN_POINT('Ctrl Pts',(-9.45490728261951,-31.6543297887092,
23.8862085799005));
#34665=CARTESIAN_POINT('Ctrl Pts',(-9.46988654740198,-31.6519236933609,
23.8871011446386));
#34666=CARTESIAN_POINT('Ctrl Pts',(-9.50164327201351,-31.6470411229716,
23.889003590587));
#34667=CARTESIAN_POINT('Ctrl Pts',(-9.51842370899059,-31.6445899046113,
23.8900147129457));
#34668=CARTESIAN_POINT('Ctrl Pts',(-9.56529403486736,-31.6381021021548,
23.8928539274645));
#34669=CARTESIAN_POINT('Ctrl Pts',(-9.59542009108317,-31.634343792011,23.8946960429954));
#34670=CARTESIAN_POINT('Ctrl Pts',(-9.79981789317652,-31.611628420839,23.9072925210599));
#34671=CARTESIAN_POINT('Ctrl Pts',(-9.97526950691085,-31.6058118904308,
23.9185738642919));
#34672=CARTESIAN_POINT('Ctrl Pts',(-10.3933747781349,-31.6243769869812,
23.9455507285583));
#34673=CARTESIAN_POINT('Ctrl Pts',(-10.6345530369694,-31.6612949652629,
23.961141443297));
#34674=CARTESIAN_POINT('Ctrl Pts',(-10.9193819838988,-31.7369061772017,
23.9790634071563));
#34675=CARTESIAN_POINT('Ctrl Pts',(-10.9687336709589,-31.7512156064774,
23.9821534868314));
#34676=CARTESIAN_POINT('Ctrl Pts',(-11.0464279570525,-31.7756709325043,
23.9869959303421));
#34677=CARTESIAN_POINT('Ctrl Pts',(-11.0749920456646,-31.7850814016771,
23.9887714324808));
#34678=CARTESIAN_POINT('Ctrl Pts',(-11.125967887394,-31.8026308238658,23.9919323590753));
#34679=CARTESIAN_POINT('Ctrl Pts',(-11.1484258698202,-31.8106283696777,
23.9933222493374));
#34680=CARTESIAN_POINT('Ctrl Pts',(-11.2010610211555,-31.8300004115753,
23.9965742897645));
#34681=CARTESIAN_POINT('Ctrl Pts',(-11.2311642225951,-31.8415700535238,
23.998429922751));
#34682=CARTESIAN_POINT('Ctrl Pts',(-11.3203962394804,-31.8773344864136,
24.0039211067087));
#34683=CARTESIAN_POINT('Ctrl Pts',(-11.3790126147566,-31.9027736493883,
24.0075156888564));
#34684=CARTESIAN_POINT('Ctrl Pts',(-11.5858996660041,-31.9996001644871,
24.0202021968438));
#34685=CARTESIAN_POINT('Ctrl Pts',(-11.7296538869797,-32.0801060843263,
24.0290039686395));
#34686=CARTESIAN_POINT('Ctrl Pts',(-12.0438125389283,-32.2874160022344,
24.048985853139));
#34687=CARTESIAN_POINT('Ctrl Pts',(-12.2092816530836,-32.4203995041232,
24.0600735199346));
#34688=CARTESIAN_POINT('Ctrl Pts',(-12.393087090061,-32.5988525326871,24.0744171755984));
#34689=CARTESIAN_POINT('Ctrl Pts',(-12.4243195403229,-32.6303904623322,
24.0769356056674));
#34690=CARTESIAN_POINT('Ctrl Pts',(-12.4683199746456,-32.6766018300751,
24.0806185107391));
#34691=CARTESIAN_POINT('Ctrl Pts',(-12.4815961412126,-32.6907873405985,
24.0817481056172));
#34692=CARTESIAN_POINT('Ctrl Pts',(-12.5048644784994,-32.7160818237243,
24.0837623146084));
#34693=CARTESIAN_POINT('Ctrl Pts',(-12.5149062735316,-32.7271439300249,
24.084643267543));
#34694=CARTESIAN_POINT('Ctrl Pts',(-12.5369240889633,-32.7517234727664,
24.0866012363964));
#34695=CARTESIAN_POINT('Ctrl Pts',(-12.548865280149,-32.7652702786513,24.0876805407923));
#34696=CARTESIAN_POINT('Ctrl Pts',(-12.584131396493,-32.805928654695,24.0909187230498));
#34697=CARTESIAN_POINT('Ctrl Pts',(-12.6071354052805,-32.8333138431699,
24.093098249348));
#34698=CARTESIAN_POINT('Ctrl Pts',(-12.7204882791658,-32.9726743106362,
24.104160264052));
#34699=CARTESIAN_POINT('Ctrl Pts',(-12.8040703056619,-33.0899504987808,
24.1133698032258));
#34700=CARTESIAN_POINT('Ctrl Pts',(-12.9994144334242,-33.4046224791904,
24.1372187559737));
#34701=CARTESIAN_POINT('Ctrl Pts',(-13.0993092042049,-33.6085900380416,
24.1518424645592));
#34702=CARTESIAN_POINT('Ctrl Pts',(-13.1783251486862,-33.8215880661724,
24.1658778257468));
#34703=CARTESIAN_POINT('Ctrl Pts',(-13.1785377141563,-33.822161540685,24.1659156062566));
#34704=CARTESIAN_POINT('Ctrl Pts',(-13.1787501240175,-33.8227350716349,
24.1659533822777));
#34705=CARTESIAN_POINT('Origin',(-10.,-35.,23.));
#34706=CARTESIAN_POINT('',(-13.1787501041971,-33.8227350181174,25.4139789249709));
#34707=CARTESIAN_POINT('',(-13.1787501240264,-33.8227350716589,25.0733224007726));
#34708=CARTESIAN_POINT('',(-13.1787501240207,-33.8227350716434,23.));
#34709=CARTESIAN_POINT('Ctrl Pts',(-13.1787501240264,-33.8227350716589,
25.0733224007726));
#34710=CARTESIAN_POINT('Ctrl Pts',(-13.1777037596094,-33.8199097679058,
25.0731373103509));
#34711=CARTESIAN_POINT('Ctrl Pts',(-13.1766536278777,-33.8170858576181,
25.0729520551845));
#34712=CARTESIAN_POINT('Ctrl Pts',(-13.1105312555146,-33.6399991599586,
25.061318838559));
#34713=CARTESIAN_POINT('Ctrl Pts',(-13.03123358399,-33.4713992994131,25.0492945094602));
#34714=CARTESIAN_POINT('Ctrl Pts',(-12.859508122886,-33.1727790714007,25.0270938575118));
#34715=CARTESIAN_POINT('Ctrl Pts',(-12.7709567695585,-33.0410898103502,
25.0169318539089));
#34716=CARTESIAN_POINT('Ctrl Pts',(-12.6145332893973,-32.8404112798225,
25.0010574830173));
#34717=CARTESIAN_POINT('Ctrl Pts',(-12.552368643226,-32.7672831003161,24.9951762428979));
#34718=CARTESIAN_POINT('Ctrl Pts',(-12.4618136261793,-32.6694909035106,
24.9871757644255));
#34719=CARTESIAN_POINT('Ctrl Pts',(-12.4359952175913,-32.642516925621,24.9849533853306));
#34720=CARTESIAN_POINT('Ctrl Pts',(-12.3907465244094,-32.5967802616235,
24.9811564238413));
#34721=CARTESIAN_POINT('Ctrl Pts',(-12.3715283686053,-32.5778135260492,
24.9795729741009));
#34722=CARTESIAN_POINT('Ctrl Pts',(-12.3316579991339,-32.5393942289379,
24.976346116251));
#34723=CARTESIAN_POINT('Ctrl Pts',(-12.3109840539793,-32.5199672262558,
24.9747038621571));
#34724=CARTESIAN_POINT('Ctrl Pts',(-12.2572818440721,-32.4707587587375,
24.9705146713141));
#34725=CARTESIAN_POINT('Ctrl Pts',(-12.2239064735533,-32.441363090422,24.9679837318499));
#34726=CARTESIAN_POINT('Ctrl Pts',(-12.051759736685,-32.2956572505476,24.9552725652429));
#34727=CARTESIAN_POINT('Ctrl Pts',(-11.9044025749955,-32.1899380234172,
24.9455152308359));
#34728=CARTESIAN_POINT('Ctrl Pts',(-11.5952888492264,-32.0037049552123,
24.9263185053184));
#34729=CARTESIAN_POINT('Ctrl Pts',(-11.4341568436961,-31.9233267497013,
24.9169035832575));
#34730=CARTESIAN_POINT('Ctrl Pts',(-11.190539411228,-31.8251153799393,24.9025774546773));
#34731=CARTESIAN_POINT('Ctrl Pts',(-11.112552554242,-31.7969543904365,24.8979758074541));
#34732=CARTESIAN_POINT('Ctrl Pts',(-11.0102705949371,-31.7642065287768,
24.8918282026853));
#34733=CARTESIAN_POINT('Ctrl Pts',(-10.9868430939097,-31.7569849372781,
24.890412583451));
#34734=CARTESIAN_POINT('Ctrl Pts',(-10.9482790901677,-31.7455540268332,
24.8880669355799));
#34735=CARTESIAN_POINT('Ctrl Pts',(-10.9331875284635,-31.7411945677443,
24.8871451520212));
#34736=CARTESIAN_POINT('Ctrl Pts',(-10.9045301716943,-31.7331317800673,
24.8853865735951));
#34737=CARTESIAN_POINT('Ctrl Pts',(-10.8909705841274,-31.7294076682649,
24.8845510413255));
#34738=CARTESIAN_POINT('Ctrl Pts',(-10.8541917129508,-31.7195521176187,
24.8822761980079));
#34739=CARTESIAN_POINT('Ctrl Pts',(-10.830930246086,-31.713583007912,24.8808282337519));
#34740=CARTESIAN_POINT('Ctrl Pts',(-10.7386138374729,-31.6909364876734,
24.8750507733567));
#34741=CARTESIAN_POINT('Ctrl Pts',(-10.6691091929677,-31.6761854416009,
24.8706328341077));
#34742=CARTESIAN_POINT('Ctrl Pts',(-10.3914354597829,-31.6263164408925,
24.8528434475071));
#34743=CARTESIAN_POINT('Ctrl Pts',(-10.1806449343159,-31.6084913805317,
24.8390639713098));
#34744=CARTESIAN_POINT('Ctrl Pts',(-9.8050428765181,-31.6118638516153,24.8150813786961));
#34745=CARTESIAN_POINT('Ctrl Pts',(-9.64082993207185,-31.6253171939246,
24.8047837523791));
#34746=CARTESIAN_POINT('Ctrl Pts',(-9.43518396737897,-31.6573535366117,
24.7922137639916));
#34747=CARTESIAN_POINT('Ctrl Pts',(-9.39227501204829,-31.6648878378857,
24.7896081305403));
#34748=CARTESIAN_POINT('Ctrl Pts',(-9.32186304665412,-31.6786554559428,
24.7853589910096));
#34749=CARTESIAN_POINT('Ctrl Pts',(-9.2942723693428,-31.6844083648889,24.7837007465797));
#34750=CARTESIAN_POINT('Ctrl Pts',(-9.2405918998506,-31.6963016838651,24.7804867126448));
#34751=CARTESIAN_POINT('Ctrl Pts',(-9.2144969265699,-31.7024087262599,24.7789300080147));
#34752=CARTESIAN_POINT('Ctrl Pts',(-9.15184397193125,-31.7178574146537,
24.7752047757453));
#34753=CARTESIAN_POINT('Ctrl Pts',(-9.11536377024632,-31.7275013367975,
24.7730459467168));
#34754=CARTESIAN_POINT('Ctrl Pts',(-8.99053105994283,-31.7627422400702,
24.7656867285968));
#34755=CARTESIAN_POINT('Ctrl Pts',(-8.90306050369842,-31.7913256589993,
24.7605802564749));
#34756=CARTESIAN_POINT('Ctrl Pts',(-8.56669974555132,-31.916606648316,24.7409730465801));
#34757=CARTESIAN_POINT('Ctrl Pts',(-8.32844245781738,-32.0389950659119,
24.7272239332942));
#34758=CARTESIAN_POINT('Ctrl Pts',(-8.05233236780887,-32.2248709460987,
24.7091958965059));
#34759=CARTESIAN_POINT('Ctrl Pts',(-7.99873727330996,-32.263268901778,24.7055815331206));
#34760=CARTESIAN_POINT('Ctrl Pts',(-7.91062939412495,-32.3303660067952,
24.6993832720935));
#34761=CARTESIAN_POINT('Ctrl Pts',(-7.87550446549777,-32.3582328805144,
24.6968400688663));
#34762=CARTESIAN_POINT('Ctrl Pts',(-7.82574694359087,-32.3993429048742,
24.6931153189437));
#34763=CARTESIAN_POINT('Ctrl Pts',(-7.81065979865678,-32.4120310817214,
24.6919692581946));
#34764=CARTESIAN_POINT('Ctrl Pts',(-7.7843369962257,-32.4345632661665,24.6899384713474));
#34765=CARTESIAN_POINT('Ctrl Pts',(-7.77305440585038,-32.4443510628681,
24.6890576749047));
#34766=CARTESIAN_POINT('Ctrl Pts',(-7.74824537923675,-32.4661622615566,
24.6870975337613));
#34767=CARTESIAN_POINT('Ctrl Pts',(-7.73475046598716,-32.4782194637301,
24.6860158647647));
#34768=CARTESIAN_POINT('Ctrl Pts',(-7.6947303294352,-32.5145563993446,24.682763361456));
#34769=CARTESIAN_POINT('Ctrl Pts',(-7.66849503062537,-32.5391500448926,
24.6805716192283));
#34770=CARTESIAN_POINT('Ctrl Pts',(-7.53448594092292,-32.6688403226377,
24.6690857645331));
#34771=CARTESIAN_POINT('Ctrl Pts',(-7.43341640947634,-32.7806067077771,
24.6594336963436));
#34772=CARTESIAN_POINT('Ctrl Pts',(-7.25870959952693,-33.0017562762593,
24.6412775559854));
#34773=CARTESIAN_POINT('Ctrl Pts',(-7.18335653062317,-33.1094516690399,
24.6327981474552));
#34774=CARTESIAN_POINT('Ctrl Pts',(-7.03793256607087,-33.3453642949642,
24.6151884792975));
#34775=CARTESIAN_POINT('Ctrl Pts',(-6.969505030181,-33.4742962776749,24.606109752659));
#34776=CARTESIAN_POINT('Ctrl Pts',(-6.89218229929252,-33.6458697615538,
24.5947561331348));
#34777=CARTESIAN_POINT('Ctrl Pts',(-6.87550208800552,-33.6848146118189,
24.5922243676755));
#34778=CARTESIAN_POINT('Ctrl Pts',(-6.84903845778761,-33.7499491557499,
24.5880630162852));
#34779=CARTESIAN_POINT('Ctrl Pts',(-6.83884146638376,-33.7759646455863,
24.5864198872428));
#34780=CARTESIAN_POINT('Ctrl Pts',(-6.81944242775695,-33.8273171685963,
24.5832125741429));
#34781=CARTESIAN_POINT('Ctrl Pts',(-6.81021864308454,-33.8526437127554,
24.5816477718171));
#34782=CARTESIAN_POINT('Ctrl Pts',(-6.79053277593163,-33.9087699276644,
24.5782160781016));
#34783=CARTESIAN_POINT('Ctrl Pts',(-6.78020988729705,-33.939615792822,24.5763537937888));
#34784=CARTESIAN_POINT('Ctrl Pts',(-6.74587268238143,-34.0473469306297,
24.5699270820992));
#34785=CARTESIAN_POINT('Ctrl Pts',(-6.72415488617519,-34.1249385080632,
24.5654350586408));
#34786=CARTESIAN_POINT('Ctrl Pts',(-6.63925294291248,-34.4760244381511,
24.5455916288613));
#34787=CARTESIAN_POINT('Ctrl Pts',(-6.60742110607607,-34.7559303116643,
24.5311629748319));
#34788=CARTESIAN_POINT('Ctrl Pts',(-6.61116905249123,-35.103506303396,24.5123486145624));
#34789=CARTESIAN_POINT('Ctrl Pts',(-6.61387482203468,-35.1704233714469,
24.5086797101106));
#34790=CARTESIAN_POINT('Ctrl Pts',(-6.62173269143315,-35.2824363383509,
24.5023979788015));
#34791=CARTESIAN_POINT('Ctrl Pts',(-6.62581194236091,-35.3275894322445,
24.4998272876006));
#34792=CARTESIAN_POINT('Ctrl Pts',(-6.63297163165144,-35.3923225438618,
24.4960694337222));
#34793=CARTESIAN_POINT('Ctrl Pts',(-6.63532034145911,-35.4119802981523,
24.4949186339168));
#34794=CARTESIAN_POINT('Ctrl Pts',(-6.63974378192479,-35.4464375836497,
24.4928827674385));
#34795=CARTESIAN_POINT('Ctrl Pts',(-6.64174439099302,-35.461245726155,24.4920017050168));
#34796=CARTESIAN_POINT('Ctrl Pts',(-6.64637548459245,-35.4938956236464,
24.4900451449926));
#34797=CARTESIAN_POINT('Ctrl Pts',(-6.64905043774846,-35.5117296908787,
24.4889673823148));
#34798=CARTESIAN_POINT('Ctrl Pts',(-6.65743468330857,-35.5647408057601,
24.485738519422));
#34799=CARTESIAN_POINT('Ctrl Pts',(-6.66355638595195,-35.5998490372737,
24.4835669388163));
#34800=CARTESIAN_POINT('Ctrl Pts',(-6.69729039371144,-35.7767821809214,
24.4724765897741));
#34801=CARTESIAN_POINT('Ctrl Pts',(-6.73339539780418,-35.9168255296127,
24.4632272721264));
#34802=CARTESIAN_POINT('Ctrl Pts',(-6.81678009774279,-36.1716706251502,
24.4459608456862));
#34803=CARTESIAN_POINT('Ctrl Pts',(-6.86164576670486,-36.2870257574511,
24.4379696851665));
#34804=CARTESIAN_POINT('Ctrl Pts',(-6.9563661274185,-36.4959521922733,24.4233450031194));
#34805=CARTESIAN_POINT('Ctrl Pts',(-7.00449857195458,-36.5901428467637,
24.4166898999895));
#34806=CARTESIAN_POINT('Ctrl Pts',(-7.09375258837058,-36.7463189936019,
24.4055912703018));
#34807=CARTESIAN_POINT('Ctrl Pts',(-7.13265177899439,-36.8094804493413,
24.4010830628702));
#34808=CARTESIAN_POINT('Ctrl Pts',(-7.19240189958801,-36.8997259456667,
24.3946108353764));
#34809=CARTESIAN_POINT('Ctrl Pts',(-7.21163747058635,-36.9278486179572,
24.3925892584952));
#34810=CARTESIAN_POINT('Ctrl Pts',(-7.24660475850377,-36.9773527611934,
24.3890210540228));
#34811=CARTESIAN_POINT('Ctrl Pts',(-7.26216954724209,-36.9988481106571,
24.3874683641327));
#34812=CARTESIAN_POINT('Ctrl Pts',(-7.295727707954,-37.0440652463354,24.3841940140367));
#34813=CARTESIAN_POINT('Ctrl Pts',(-7.31378448124538,-37.0677373211333,
24.3824749563784));
#34814=CARTESIAN_POINT('Ctrl Pts',(-7.36378710284971,-37.1315291208781,
24.3778266265635));
#34815=CARTESIAN_POINT('Ctrl Pts',(-7.39633588030019,-37.1711675134272,
24.3749210020832));
#34816=CARTESIAN_POINT('Ctrl Pts',(-7.59283026622022,-37.3996846906618,
24.3580314469152));
#34817=CARTESIAN_POINT('Ctrl Pts',(-7.77637103877369,-37.5706882477391,
24.3448941107025));
#34818=CARTESIAN_POINT('Ctrl Pts',(-8.11353617574474,-37.8214508688737,
24.3225781722141));
#34819=CARTESIAN_POINT('Ctrl Pts',(-8.25743678234348,-37.9125232396933,
24.3134867302454));
#34820=CARTESIAN_POINT('Ctrl Pts',(-8.43418665700761,-38.0065835303801,
24.3021118298687));
#34821=CARTESIAN_POINT('Ctrl Pts',(-8.46101698582948,-38.0204051217703,
24.3003795694543));
#34822=CARTESIAN_POINT('Ctrl Pts',(-8.50317187264601,-38.0414136422275,
24.2976437774197));
#34823=CARTESIAN_POINT('Ctrl Pts',(-8.51837240181083,-38.0488474903851,
24.2966544580675));
#34824=CARTESIAN_POINT('Ctrl Pts',(-8.54731852613893,-38.0627360629923,
24.2947639889825));
#34825=CARTESIAN_POINT('Ctrl Pts',(-8.56105277922902,-38.0692126868888,
24.2938641411524));
#34826=CARTESIAN_POINT('Ctrl Pts',(-8.59455814967905,-38.0847384087863,
24.2916625817283));
#34827=CARTESIAN_POINT('Ctrl Pts',(-8.61437352309773,-38.0936898773976,
24.2903552937946));
#34828=CARTESIAN_POINT('Ctrl Pts',(-8.68398513447013,-38.1243335486597,
24.2857479243447));
#34829=CARTESIAN_POINT('Ctrl Pts',(-8.7342132110815,-38.1450180236902,24.282397184276));
#34830=CARTESIAN_POINT('Ctrl Pts',(-8.97367527450129,-38.236965710208,24.2663695794947));
#34831=CARTESIAN_POINT('Ctrl Pts',(-9.16853643458028,-38.2924084356933,
24.2532006209466));
#34832=CARTESIAN_POINT('Ctrl Pts',(-9.55643201873365,-38.3661203646877,
24.2278562357609));
#34833=CARTESIAN_POINT('Ctrl Pts',(-9.74843809505455,-38.3858905111979,
24.2157101759797));
#34834=CARTESIAN_POINT('Ctrl Pts',(-9.98588834605419,-38.3900164914881,
24.2013513859106));
#34835=CARTESIAN_POINT('Ctrl Pts',(-10.0306812641088,-38.3899070634982,
24.1986700591061));
#34836=CARTESIAN_POINT('Ctrl Pts',(-10.1038862041232,-38.3882770162454,
24.1943308617843));
#34837=CARTESIAN_POINT('Ctrl Pts',(-10.1323034122903,-38.3872864306022,
24.1926569942099));
#34838=CARTESIAN_POINT('Ctrl Pts',(-10.1876414829368,-38.3846599416066,
24.1894169729571));
#34839=CARTESIAN_POINT('Ctrl Pts',(-10.2145618418345,-38.383060082835,24.1878498364535));
#34840=CARTESIAN_POINT('Ctrl Pts',(-10.2785001973706,-38.3784939861124,
24.1841478573401));
#34841=CARTESIAN_POINT('Ctrl Pts',(-10.3154945775324,-38.3752403321314,
24.1820219911742));
#34842=CARTESIAN_POINT('Ctrl Pts',(-10.440554876662,-38.3621670813373,24.1748833247072));
#34843=CARTESIAN_POINT('Ctrl Pts',(-10.5282897841573,-38.3495026112845,
24.1699569627529));
#34844=CARTESIAN_POINT('Ctrl Pts',(-10.8821379423599,-38.2841732464141,
24.1502667923338));
#34845=CARTESIAN_POINT('Ctrl Pts',(-11.1419510929791,-38.2031077929201,
24.1363060898995));
#34846=CARTESIAN_POINT('Ctrl Pts',(-11.4497562110455,-38.064800448062,24.1180326370402));
#34847=CARTESIAN_POINT('Ctrl Pts',(-11.5093790202929,-38.0358802602029,
24.1144006674799));
#34848=CARTESIAN_POINT('Ctrl Pts',(-11.6080050806346,-37.9844177633764,
24.1081754427482));
#34849=CARTESIAN_POINT('Ctrl Pts',(-11.6474768113919,-37.9628110775127,
24.1056233445802));
#34850=CARTESIAN_POINT('Ctrl Pts',(-11.7036288203203,-37.9306046478162,
24.1018878794908));
#34851=CARTESIAN_POINT('Ctrl Pts',(-11.7206662814277,-37.9206338809392,
24.100740281153));
#34852=CARTESIAN_POINT('Ctrl Pts',(-11.7504423115027,-37.9028572053049,
24.0987078493396));
#34853=CARTESIAN_POINT('Ctrl Pts',(-11.7632178752809,-37.8951150153885,
24.0978269697308));
#34854=CARTESIAN_POINT('Ctrl Pts',(-11.7913389761971,-37.8778180071843,
24.0958680042558));
#34855=CARTESIAN_POINT('Ctrl Pts',(-11.80665933728,-37.8682248546455,24.0947876134484));
#34856=CARTESIAN_POINT('Ctrl Pts',(-11.8512089351539,-37.8398306917014,
24.091609051988));
#34857=CARTESIAN_POINT('Ctrl Pts',(-11.8802258171739,-37.8207026702786,
24.0894917961642));
#34858=CARTESIAN_POINT('Ctrl Pts',(-12.0617385625394,-37.6970036602281,
24.0759730861485));
#34859=CARTESIAN_POINT('Ctrl Pts',(-12.2057476118327,-37.5805546601346,
24.0640234658594));
#34860=CARTESIAN_POINT('Ctrl Pts',(-12.4547259282142,-37.3430889791939,
24.0418486337316));
#34861=CARTESIAN_POINT('Ctrl Pts',(-12.5620456576854,-37.225235939274,24.0316396997669));
#34862=CARTESIAN_POINT('Ctrl Pts',(-12.720280298216,-37.0247789155064,24.0157046819958));
#34863=CARTESIAN_POINT('Ctrl Pts',(-12.7766335035764,-36.9467828968309,
24.0098079991194));
#34864=CARTESIAN_POINT('Ctrl Pts',(-12.8501730243033,-36.8352970124455,
24.0017906735044));
#34865=CARTESIAN_POINT('Ctrl Pts',(-12.8702319900878,-36.803765473424,23.9995663076097));
#34866=CARTESIAN_POINT('Ctrl Pts',(-12.903882433553,-36.7488856908229,23.9957670377681));
#34867=CARTESIAN_POINT('Ctrl Pts',(-12.9177234441872,-36.725695313065,23.9941832379845));
#34868=CARTESIAN_POINT('Ctrl Pts',(-12.9455273160126,-36.6778194288057,
23.9909565988483));
#34869=CARTESIAN_POINT('Ctrl Pts',(-12.959460508519,-36.6531191047775,23.9893149016175));
#34870=CARTESIAN_POINT('Ctrl Pts',(-12.994418941029,-36.5892870530843,23.9851290780429));
#34871=CARTESIAN_POINT('Ctrl Pts',(-13.0149882672211,-36.5499110094683,
23.9826008970126));
#34872=CARTESIAN_POINT('Ctrl Pts',(-13.1096368043195,-36.3597053322764,
23.9706263010761));
#34873=CARTESIAN_POINT('Ctrl Pts',(-13.1732098537437,-36.2039050022012,
23.9615372197958));
#34874=CARTESIAN_POINT('Ctrl Pts',(-13.2835703195063,-35.8630016912642,
23.9424380108322));
#34875=CARTESIAN_POINT('Ctrl Pts',(-13.3268230420832,-35.6773828705033,
23.9324998099822));
#34876=CARTESIAN_POINT('Ctrl Pts',(-13.3665598520118,-35.4048804225185,
23.9174975833685));
#34877=CARTESIAN_POINT('Ctrl Pts',(-13.3756655976754,-35.3202076480346,
23.9127765415568));
#34878=CARTESIAN_POINT('Ctrl Pts',(-13.383289906604,-35.2106310184132,23.9064908535421));
#34879=CARTESIAN_POINT('Ctrl Pts',(-13.3847357889658,-35.1859558572627,
23.9050639048499));
#34880=CARTESIAN_POINT('Ctrl Pts',(-13.3866610174315,-35.1455345782663,
23.9027043891909));
#34881=CARTESIAN_POINT('Ctrl Pts',(-13.3873006950602,-35.1297965467947,
23.9017802615147));
#34882=CARTESIAN_POINT('Ctrl Pts',(-13.3883026527301,-35.1000348929821,
23.9000214294544));
#34883=CARTESIAN_POINT('Ctrl Pts',(-13.3886876081946,-35.0860123523354,
23.8991880353236));
#34884=CARTESIAN_POINT('Ctrl Pts',(-13.3894915958565,-35.0481630098936,
23.8969266057667));
#34885=CARTESIAN_POINT('Ctrl Pts',(-13.3897464126101,-35.0243339654891,
23.8954900880576));
#34886=CARTESIAN_POINT('Ctrl Pts',(-13.3897612595208,-34.9246694112491,
23.8894339278107));
#34887=CARTESIAN_POINT('Ctrl Pts',(-13.3872276505839,-34.8488601237088,
23.8847115859043));
#34888=CARTESIAN_POINT('Ctrl Pts',(-13.3720525628155,-34.6225561572871,
23.8703860111663));
#34889=CARTESIAN_POINT('Ctrl Pts',(-13.3518968174119,-34.4727547277818,
23.8606071038608));
#34890=CARTESIAN_POINT('Ctrl Pts',(-13.2871052863501,-34.1539954505898,
23.8396687482438));
#34891=CARTESIAN_POINT('Ctrl Pts',(-13.2392695055602,-33.9861443455545,
23.8285690331584));
#34892=CARTESIAN_POINT('Ctrl Pts',(-13.1787501550516,-33.8227351554304,
23.8178420415151));
#34893=CARTESIAN_POINT('',(-13.3897487153538,-35.0029511451049,24.2344127503854));
#34894=CARTESIAN_POINT('Ctrl Pts',(-13.1787501240175,-33.8227350716349,
24.1659533822777));
#34895=CARTESIAN_POINT('Ctrl Pts',(-13.2050987685498,-33.8938794292528,
24.1706393556419));
#34896=CARTESIAN_POINT('Ctrl Pts',(-13.2290530202204,-33.965892250316,24.1752555057));
#34897=CARTESIAN_POINT('Ctrl Pts',(-13.2602388283821,-34.0713398226487,
24.1818343453727));
#34898=CARTESIAN_POINT('Ctrl Pts',(-13.2694125310574,-34.1041714605046,
24.1838579400893));
#34899=CARTESIAN_POINT('Ctrl Pts',(-13.28486230881,-34.1628664636576,24.1874329555466));
#34900=CARTESIAN_POINT('Ctrl Pts',(-13.2913318785798,-34.1886754838599,
24.1889904038047));
#34901=CARTESIAN_POINT('Ctrl Pts',(-13.3043200618768,-34.243203414143,24.1922513776549));
#34902=CARTESIAN_POINT('Ctrl Pts',(-13.3107696814499,-34.2719365830112,
24.1939526121165));
#34903=CARTESIAN_POINT('Ctrl Pts',(-13.3231506591771,-34.3306649670845,
24.1973967439237));
#34904=CARTESIAN_POINT('Ctrl Pts',(-13.3290522492268,-34.3606637065046,
24.1991385882913));
#34905=CARTESIAN_POINT('Ctrl Pts',(-13.3467253257844,-34.4573902297874,
24.2047027675562));
#34906=CARTESIAN_POINT('Ctrl Pts',(-13.356902710259,-34.5243943175358,24.2084773853082));
#34907=CARTESIAN_POINT('Ctrl Pts',(-13.3816250256084,-34.7281277796348,
24.2197649678847));
#34908=CARTESIAN_POINT('Ctrl Pts',(-13.3898684009191,-34.8654777316019,
24.2271128972712));
#34909=CARTESIAN_POINT('Ctrl Pts',(-13.3897487153538,-35.0029511451049,
24.2344127503854));
#34910=CARTESIAN_POINT('Ctrl Pts',(-13.3897487163515,-35.002949998855,24.2344126895194));
#34911=CARTESIAN_POINT('Ctrl Pts',(-13.389557470868,-35.2227040272623,24.2460816526017));
#34912=CARTESIAN_POINT('Ctrl Pts',(-13.3679972012171,-35.4419036878591,
24.2575682627097));
#34913=CARTESIAN_POINT('Ctrl Pts',(-13.3198065562547,-35.6856496526208,
24.2715260273842));
#34914=CARTESIAN_POINT('Ctrl Pts',(-13.3138742712255,-35.7137704312125,
24.2731550001771));
#34915=CARTESIAN_POINT('Ctrl Pts',(-13.302317964461,-35.765297633892,24.2761798111977));
#34916=CARTESIAN_POINT('Ctrl Pts',(-13.2968007467721,-35.7887262974359,
24.2775704471149));
#34917=CARTESIAN_POINT('Ctrl Pts',(-13.2872933619645,-35.8272552760768,
24.2798856118402));
#34918=CARTESIAN_POINT('Ctrl Pts',(-13.2834473764778,-35.8423907952853,
24.280802319444));
#34919=CARTESIAN_POINT('Ctrl Pts',(-13.2754188054373,-35.8730959907211,
24.2826777256283));
#34920=CARTESIAN_POINT('Ctrl Pts',(-13.2712294963358,-35.8886633326383,
24.2836367407879));
#34921=CARTESIAN_POINT('Ctrl Pts',(-13.2598759827137,-35.929684272583,24.286184399295));
#34922=CARTESIAN_POINT('Ctrl Pts',(-13.2525248446699,-35.9550844518139,
24.287782933385));
#34923=CARTESIAN_POINT('Ctrl Pts',(-13.2165368732437,-36.0741961793681,
24.2953699858009));
#34924=CARTESIAN_POINT('Ctrl Pts',(-13.1841443911628,-36.166716855223,24.3015283282721));
#34925=CARTESIAN_POINT('Ctrl Pts',(-13.0713591454305,-36.4489985478191,
24.3208951226771));
#34926=CARTESIAN_POINT('Ctrl Pts',(-12.977644349327,-36.6329371806667,24.3343226006404));
#34927=CARTESIAN_POINT('Ctrl Pts',(-12.817473713754,-36.8871033407532,24.3533856702217));
#34928=CARTESIAN_POINT('Ctrl Pts',(-12.7638252912858,-36.964838193712,24.3592992059404));
#34929=CARTESIAN_POINT('Ctrl Pts',(-12.6657480381098,-37.0949676548479,
24.3693201602546));
#34930=CARTESIAN_POINT('Ctrl Pts',(-12.6228456871337,-37.148437476239,24.3734764560856));
#34931=CARTESIAN_POINT('Ctrl Pts',(-12.5568640109711,-37.2257463500624,
24.3795466231905));
#34932=CARTESIAN_POINT('Ctrl Pts',(-12.5350107605126,-37.2506045734466,
24.3815083486727));
#34933=CARTESIAN_POINT('Ctrl Pts',(-12.4950445170227,-37.2947456178366,
24.3850110316012));
#34934=CARTESIAN_POINT('Ctrl Pts',(-12.4770634542439,-37.3141437498389,
24.3865572329557));
#34935=CARTESIAN_POINT('Ctrl Pts',(-12.4379371296702,-37.3553749667458,
24.3898598001322));
#34936=CARTESIAN_POINT('Ctrl Pts',(-12.4167214558623,-37.3771382318965,
24.3916129911705));
#34937=CARTESIAN_POINT('Ctrl Pts',(-12.3578077616813,-37.4359684584709,
24.3963825126837));
#34938=CARTESIAN_POINT('Ctrl Pts',(-12.3195300432494,-37.4724442503966,
24.3993735159308));
#34939=CARTESIAN_POINT('Ctrl Pts',(-12.1154255111954,-37.6580266281995,
24.4148066693152));
#34940=CARTESIAN_POINT('Ctrl Pts',(-11.9360338293216,-37.79140053632,24.4266058166952));
#34941=CARTESIAN_POINT('Ctrl Pts',(-11.577078147921,-38.0069111006793,24.4488059708313));
#34942=CARTESIAN_POINT('Ctrl Pts',(-11.4009444952813,-38.0928989344067,
24.4591763062561));
#34943=CARTESIAN_POINT('Ctrl Pts',(-11.1915248128081,-38.1735632068501,
24.4719476335477));
#34944=CARTESIAN_POINT('Ctrl Pts',(-11.1645146641302,-38.1835735091049,
24.473603172001));
#34945=CARTESIAN_POINT('Ctrl Pts',(-11.1217161260763,-38.198817675594,24.4762443519741));
#34946=CARTESIAN_POINT('Ctrl Pts',(-11.1060105763349,-38.2042818491567,
24.4772173417119));
#34947=CARTESIAN_POINT('Ctrl Pts',(-11.0759381263507,-38.2144970338249,
24.4790886989367));
#34948=CARTESIAN_POINT('Ctrl Pts',(-11.061578624952,-38.2192677462002,24.479985950123));
#34949=CARTESIAN_POINT('Ctrl Pts',(-11.025958939709,-38.2308375914742,24.4822200337298));
#34950=CARTESIAN_POINT('Ctrl Pts',(-11.0046628076571,-38.2375231077081,
24.4835630608457));
#34951=CARTESIAN_POINT('Ctrl Pts',(-10.9277882803292,-38.2608248945439,
24.4884335003926));
#34952=CARTESIAN_POINT('Ctrl Pts',(-10.8718541780812,-38.2762233685315,
24.4920190430788));
#34953=CARTESIAN_POINT('Ctrl Pts',(-10.6223486242638,-38.3380698021468,
24.5081173038665));
#34954=CARTESIAN_POINT('Ctrl Pts',(-10.4253048259013,-38.368848449039,24.5210800690393));
#34955=CARTESIAN_POINT('Ctrl Pts',(-10.0687596977649,-38.3927475661615,
24.5440117078395));
#34956=CARTESIAN_POINT('Ctrl Pts',(-9.91025244986144,-38.3922587063558,
24.5540277623386));
#34957=CARTESIAN_POINT('Ctrl Pts',(-9.68936331675368,-38.3760772867058,
24.5676024860253));
#34958=CARTESIAN_POINT('Ctrl Pts',(-9.62652036301723,-38.3697042526392,
24.5714226215228));
#34959=CARTESIAN_POINT('Ctrl Pts',(-9.53204530914583,-38.3574476241247,
24.5771045277702));
#34960=CARTESIAN_POINT('Ctrl Pts',(-9.50026127651868,-38.3528640676407,
24.5790056425006));
#34961=CARTESIAN_POINT('Ctrl Pts',(-9.44501497096434,-38.3440939518448,
24.5822929907971));
#34962=CARTESIAN_POINT('Ctrl Pts',(-9.42152322346232,-38.3401103878718,
24.5836854133492));
#34963=CARTESIAN_POINT('Ctrl Pts',(-9.36838100463392,-38.3305214226798,
24.5868238132335));
#34964=CARTESIAN_POINT('Ctrl Pts',(-9.33875923745743,-38.3247670957518,
24.5885650222385));
#34965=CARTESIAN_POINT('Ctrl Pts',(-9.25845816925667,-38.3080521345346,
24.5932655370562));
#34966=CARTESIAN_POINT('Ctrl Pts',(-9.20794615505068,-38.2963228477853,
24.5962007625502));
#34967=CARTESIAN_POINT('Ctrl Pts',(-8.92746188475293,-38.2243720739452,
24.6124133615817));
#34968=CARTESIAN_POINT('Ctrl Pts',(-8.70405324593885,-38.141249183347,24.624941401881));
#34969=CARTESIAN_POINT('Ctrl Pts',(-8.32790229774715,-37.9542740463019,
24.6472297425558));
#34970=CARTESIAN_POINT('Ctrl Pts',(-8.17147062457748,-37.8600893357387,
24.6569393433433));
#34971=CARTESIAN_POINT('Ctrl Pts',(-7.99978149385415,-37.736855025669,24.6689624963716));
#34972=CARTESIAN_POINT('Ctrl Pts',(-7.97639372514418,-37.7196078814374,
24.6706322077397));
#34973=CARTESIAN_POINT('Ctrl Pts',(-7.93993272728111,-37.6919892692622,
24.673290870923));
#34974=CARTESIAN_POINT('Ctrl Pts',(-7.92670889104122,-37.6818179181006,
24.674266888401));
#34975=CARTESIAN_POINT('Ctrl Pts',(-7.90165412414407,-37.6622505317391,
24.6761397904135));
#34976=CARTESIAN_POINT('Ctrl Pts',(-7.8898100958466,-37.6528723759848,24.6770354994564));
#34977=CARTESIAN_POINT('Ctrl Pts',(-7.8634904877021,-37.6317446232106,24.6790485325802));
#34978=CARTESIAN_POINT('Ctrl Pts',(-7.84904836924341,-37.6199541419106,
24.6801685879334));
#34979=CARTESIAN_POINT('Ctrl Pts',(-7.79883931084995,-37.5782687319091,
24.6841148188025));
#34980=CARTESIAN_POINT('Ctrl Pts',(-7.76359386597663,-37.547756893067,24.6869789411453));
#34981=CARTESIAN_POINT('Ctrl Pts',(-7.57406914437529,-37.3767227843365,
24.7028519654682));
#34982=CARTESIAN_POINT('Ctrl Pts',(-7.43239553345001,-37.2229153903095,
24.7164451304174));
#34983=CARTESIAN_POINT('Ctrl Pts',(-7.18670198487238,-36.9011195230579,
24.7424468042141));
#34984=CARTESIAN_POINT('Ctrl Pts',(-7.08138567914864,-36.7351114304078,
24.7548281053633));
#34985=CARTESIAN_POINT('Ctrl Pts',(-6.97034051022602,-36.5210470738262,
24.7694099776128));
#34986=CARTESIAN_POINT('Ctrl Pts',(-6.95045951579454,-36.4807849100586,
24.7720980970854));
#34987=CARTESIAN_POINT('Ctrl Pts',(-6.9192942610958,-36.4143786324943,24.7764453784158));
#34988=CARTESIAN_POINT('Ctrl Pts',(-6.90752958165394,-36.388467338913,24.7781206519957));
#34989=CARTESIAN_POINT('Ctrl Pts',(-6.88525848933116,-36.3377282837044,
24.7813614683322));
#34990=CARTESIAN_POINT('Ctrl Pts',(-6.87471925435066,-36.3129173476333,
24.7829280196204));
#34991=CARTESIAN_POINT('Ctrl Pts',(-6.85039335736396,-36.2536972920977,
24.7866255737663));
#34992=CARTESIAN_POINT('Ctrl Pts',(-6.8368727761614,-36.2191821941423,24.7887476605256));
#34993=CARTESIAN_POINT('Ctrl Pts',(-6.79314956497395,-36.1019393907378,
24.7958521552615));
#34994=CARTESIAN_POINT('Ctrl Pts',(-6.76560407892482,-36.0182558063276,
24.8007493369715));
#34995=CARTESIAN_POINT('Ctrl Pts',(-6.6664776636023,-35.672259401858,24.8204494026849));
#34996=CARTESIAN_POINT('Ctrl Pts',(-6.62331920405078,-35.4028910901985,
24.8344413777944));
#34997=CARTESIAN_POINT('Ctrl Pts',(-6.61022501780199,-35.0650144979142,
24.8527510581505));
#34998=CARTESIAN_POINT('Ctrl Pts',(-6.60960197732753,-34.9987021291413,
24.856385581082));
#34999=CARTESIAN_POINT('Ctrl Pts',(-6.61182133907472,-34.8874069387649,
24.8626147146398));
#35000=CARTESIAN_POINT('Ctrl Pts',(-6.61361546613743,-34.8424207392027,
24.8651681009589));
#35001=CARTESIAN_POINT('Ctrl Pts',(-6.61748442389753,-34.7777764802262,
24.8689051173671));
#35002=CARTESIAN_POINT('Ctrl Pts',(-6.61883618504558,-34.758078254302,24.8700529378478));
#35003=CARTESIAN_POINT('Ctrl Pts',(-6.62151287794324,-34.7234986168888,
24.8720856073144));
#35004=CARTESIAN_POINT('Ctrl Pts',(-6.62276422071056,-34.7086124099631,
24.872966498933));
#35005=CARTESIAN_POINT('Ctrl Pts',(-6.62574688776563,-34.6757352363023,
24.8749252947229));
#35006=CARTESIAN_POINT('Ctrl Pts',(-6.62752369249953,-34.6577497619699,
24.876005501044));
#35007=CARTESIAN_POINT('Ctrl Pts',(-6.63325267066989,-34.6041441034158,
24.8792491418261));
#35008=CARTESIAN_POINT('Ctrl Pts',(-6.63762589911724,-34.5685725369179,
24.8814333234479));
#35009=CARTESIAN_POINT('Ctrl Pts',(-6.66302676493493,-34.3859254697169,
24.8927895837874));
#35010=CARTESIAN_POINT('Ctrl Pts',(-6.69314215077066,-34.240288137942,24.9023107148573));
#35011=CARTESIAN_POINT('Ctrl Pts',(-6.76658094138884,-33.9745353272757,
24.9200703050858));
#35012=CARTESIAN_POINT('Ctrl Pts',(-6.80732503891533,-33.8539610898808,
24.9282833771205));
#35013=CARTESIAN_POINT('Ctrl Pts',(-6.91116848139234,-33.5955725659471,
24.9460051862209));
#35014=CARTESIAN_POINT('Ctrl Pts',(-6.97692902598639,-33.4591079773554,
24.9554407948336));
#35015=CARTESIAN_POINT('Ctrl Pts',(-7.07268868593591,-33.29029801448,24.9671537458906));
#35016=CARTESIAN_POINT('Ctrl Pts',(-7.09448263704099,-33.25351738835,24.9697092945455));
#35017=CARTESIAN_POINT('Ctrl Pts',(-7.13170346490561,-33.1933276251907,
24.9738988956297));
#35018=CARTESIAN_POINT('Ctrl Pts',(-7.14673487782694,-33.1696808212458,
24.9755468724839));
#35019=CARTESIAN_POINT('Ctrl Pts',(-7.17676900970466,-33.1237016656158,
24.9787561612413));
#35020=CARTESIAN_POINT('Ctrl Pts',(-7.19174777841637,-33.1013562247761,
24.9803181888145));
#35021=CARTESIAN_POINT('Ctrl Pts',(-7.22529801605274,-33.0525715174157,
24.9837349091707));
#35022=CARTESIAN_POINT('Ctrl Pts',(-7.24398479870379,-33.0262145237367,
24.9855851477254));
#35023=CARTESIAN_POINT('Ctrl Pts',(-7.31024396435616,-32.9355345737865,
24.991970307384));
#35024=CARTESIAN_POINT('Ctrl Pts',(-7.35971591371658,-32.8726292512907,
24.9964337567691));
#35025=CARTESIAN_POINT('Ctrl Pts',(-7.59323727156486,-32.5964087329697,
25.0163133572538));
#35026=CARTESIAN_POINT('Ctrl Pts',(-7.80119511333199,-32.4048111331099,
25.0307937211409));
#35027=CARTESIAN_POINT('Ctrl Pts',(-8.08500697919784,-32.2021972025712,
25.0496676982648));
#35028=CARTESIAN_POINT('Ctrl Pts',(-8.14070628208018,-32.1648765931853,
25.0533405193687));
#35029=CARTESIAN_POINT('Ctrl Pts',(-8.23589638556857,-32.1051076052235,
25.0596282379565));
#35030=CARTESIAN_POINT('Ctrl Pts',(-8.27479905542806,-32.0817565504525,
25.0622008953476));
#35031=CARTESIAN_POINT('Ctrl Pts',(-8.33133751215488,-32.0493453690614,
25.0659611158944));
#35032=CARTESIAN_POINT('Ctrl Pts',(-8.34860391579449,-32.0396472876639,
25.0671122530522));
#35033=CARTESIAN_POINT('Ctrl Pts',(-8.37904675691685,-32.0228975555821,
25.0691484819474));
#35034=CARTESIAN_POINT('Ctrl Pts',(-8.39218639271998,-32.0157808771441,
25.070029564123));
#35035=CARTESIAN_POINT('Ctrl Pts',(-8.42128281592764,-32.000269650466,25.0719858730274));
#35036=CARTESIAN_POINT('Ctrl Pts',(-8.43725958041177,-31.991915482223,25.073063360658));
#35037=CARTESIAN_POINT('Ctrl Pts',(-8.48402679719789,-31.9679342755029,
25.0762252483454));
#35038=CARTESIAN_POINT('Ctrl Pts',(-8.51498945259423,-31.952650202956,25.0783284484239));
#35039=CARTESIAN_POINT('Ctrl Pts',(-8.71712084217275,-31.8566842438053,
25.0920965934837));
#35040=CARTESIAN_POINT('Ctrl Pts',(-8.89454619189799,-31.7899883613176,
25.1043370156309));
#35041=CARTESIAN_POINT('Ctrl Pts',(-9.22716259565232,-31.6958184650572,
25.1266135216758));
#35042=CARTESIAN_POINT('Ctrl Pts',(-9.38051372151334,-31.6636640829672,
25.136641502814));
#35043=CARTESIAN_POINT('Ctrl Pts',(-9.62987868787729,-31.6291716481908,
25.1523422370958));
#35044=CARTESIAN_POINT('Ctrl Pts',(-9.72472321203555,-31.6201037175278,
25.1581789822731));
#35045=CARTESIAN_POINT('Ctrl Pts',(-9.85701999312256,-31.6130620443345,
25.1661308788803));
#35046=CARTESIAN_POINT('Ctrl Pts',(-9.89424008132489,-31.6116955562562,
25.1683475016195));
#35047=CARTESIAN_POINT('Ctrl Pts',(-9.95845499241266,-31.6103971879772,
25.1721377783345));
#35048=CARTESIAN_POINT('Ctrl Pts',(-9.98543981315512,-31.6101738577671,
25.1737202172129));
#35049=CARTESIAN_POINT('Ctrl Pts',(-10.0408224162439,-31.6103768622678,
25.1769477289714));
#35050=CARTESIAN_POINT('Ctrl Pts',(-10.0692179855594,-31.6108377986161,
25.1785916131774));
#35051=CARTESIAN_POINT('Ctrl Pts',(-10.1422022420484,-31.6129401917839,
25.1827906551621));
#35052=CARTESIAN_POINT('Ctrl Pts',(-10.1867710803497,-31.6151052533139,
25.1853296632776));
#35053=CARTESIAN_POINT('Ctrl Pts',(-10.4077268521521,-31.6302164811966,
25.1978103623513));
#35054=CARTESIAN_POINT('Ctrl Pts',(-10.5829611608843,-31.6560730077891,
25.2073514090393));
#35055=CARTESIAN_POINT('Ctrl Pts',(-10.9107081500622,-31.7309941693607,
25.2252453198962));
#35056=CARTESIAN_POINT('Ctrl Pts',(-11.063321650142,-31.777402845856,25.2336047440714));
#35057=CARTESIAN_POINT('Ctrl Pts',(-11.2778284180127,-31.8595361580688,
25.2460112859812));
#35058=CARTESIAN_POINT('Ctrl Pts',(-11.3427534508646,-31.8867427401561,
25.2498591920003));
#35059=CARTESIAN_POINT('Ctrl Pts',(-11.4494996777622,-31.9354347249306,
25.2564136621465));
#35060=CARTESIAN_POINT('Ctrl Pts',(-11.4918066171576,-31.9558051626408,
25.2590731907785));
#35061=CARTESIAN_POINT('Ctrl Pts',(-11.5515691203872,-31.986125257689,25.2629378511485));
#35062=CARTESIAN_POINT('Ctrl Pts',(-11.569382185958,-31.9953623829993,25.2641037151851));
#35063=CARTESIAN_POINT('Ctrl Pts',(-11.6003359971998,-32.0117641087771,
25.2661559086322));
#35064=CARTESIAN_POINT('Ctrl Pts',(-11.6135129667573,-32.018858449966,25.2670379971065));
#35065=CARTESIAN_POINT('Ctrl Pts',(-11.642297569464,-32.0346025328819,25.2689839691578));
#35066=CARTESIAN_POINT('Ctrl Pts',(-11.6578839313121,-32.0432882650192,
25.2700499376898));
#35067=CARTESIAN_POINT('Ctrl Pts',(-11.7026593526718,-32.0687053844993,
25.2731461002313));
#35068=CARTESIAN_POINT('Ctrl Pts',(-11.7316680360506,-32.0857483597004,
25.2751939895415));
#35069=CARTESIAN_POINT('Ctrl Pts',(-11.9753072010917,-32.2338115438166,
25.2927219189394));
#35070=CARTESIAN_POINT('Ctrl Pts',(-12.1749888619193,-32.3879025223372,
25.3092037589841));
#35071=CARTESIAN_POINT('Ctrl Pts',(-12.4401638581022,-32.6442037764079,
25.332807356536));
#35072=CARTESIAN_POINT('Ctrl Pts',(-12.5202544506499,-32.7300888027633,
25.3402295786459));
#35073=CARTESIAN_POINT('Ctrl Pts',(-12.6469057588669,-32.8808903219142,
25.3524165107193));
#35074=CARTESIAN_POINT('Ctrl Pts',(-12.6959189647463,-32.9436054801293,
25.3572645381508));
#35075=CARTESIAN_POINT('Ctrl Pts',(-12.7632234716228,-33.0362732166188,
25.3641208420278));
#35076=CARTESIAN_POINT('Ctrl Pts',(-12.783326200648,-33.0648715205522,25.366196813312));
#35077=CARTESIAN_POINT('Ctrl Pts',(-12.8179657177998,-33.1158067840632,
25.3698258716006));
#35078=CARTESIAN_POINT('Ctrl Pts',(-12.8326879204357,-33.1380134084014,
25.3713857688134));
#35079=CARTESIAN_POINT('Ctrl Pts',(-12.8630502057364,-33.1850048773397,
25.374641237903));
#35080=CARTESIAN_POINT('Ctrl Pts',(-12.8786338183571,-33.2098236976073,
25.3763346587354));
#35081=CARTESIAN_POINT('Ctrl Pts',(-12.919415939758,-33.2766840806945,25.3808299991001));
#35082=CARTESIAN_POINT('Ctrl Pts',(-12.944028242768,-33.3190760774526,25.3836109494865));
#35083=CARTESIAN_POINT('Ctrl Pts',(-13.0495237701613,-33.5102105692971,
25.3958677269295));
#35084=CARTESIAN_POINT('Ctrl Pts',(-13.1200463218647,-33.6642280914039,
25.4049836951215));
#35085=CARTESIAN_POINT('Ctrl Pts',(-13.1787501041971,-33.8227350181174,
25.4139789249709));
#35086=CARTESIAN_POINT('Origin',(-10.,-35.,23.));
#35087=CARTESIAN_POINT('',(-13.1787501100144,-33.8227350338248,26.6607619345813));
#35088=CARTESIAN_POINT('',(-13.1787501930238,-33.8227352579598,26.3195306104224));
#35089=CARTESIAN_POINT('',(-13.1787501240207,-33.8227350716434,23.));
#35090=CARTESIAN_POINT('',(-13.3897489515553,-34.9973339299542,25.1396837753564));
#35091=CARTESIAN_POINT('Ctrl Pts',(-13.1787501930238,-33.8227352579598,
26.3195306104224));
#35092=CARTESIAN_POINT('Ctrl Pts',(-13.1275287934103,-33.6844315883653,
26.3116511514972));
#35093=CARTESIAN_POINT('Ctrl Pts',(-13.0673147987542,-33.5495611216508,
26.3039018275174));
#35094=CARTESIAN_POINT('Ctrl Pts',(-12.9360680687594,-33.3006443959325,
26.2888533570821));
#35095=CARTESIAN_POINT('Ctrl Pts',(-12.8667205839725,-33.1861060663972,
26.2815933404214));
#35096=CARTESIAN_POINT('Ctrl Pts',(-12.7748581417378,-33.0528595926025,
26.2723744883258));
#35097=CARTESIAN_POINT('Ctrl Pts',(-12.7586346206402,-33.0299420327976,
26.2707595185889));
#35098=CARTESIAN_POINT('Ctrl Pts',(-12.7324443584637,-32.9939032256492,
26.2681683890439));
#35099=CARTESIAN_POINT('Ctrl Pts',(-12.7226630753473,-32.9806480758556,
26.2672040864343));
#35100=CARTESIAN_POINT('Ctrl Pts',(-12.703559380756,-32.9551507375422,26.2653261325253));
#35101=CARTESIAN_POINT('Ctrl Pts',(-12.6942496035125,-32.9428998878466,
26.264413287662));
#35102=CARTESIAN_POINT('Ctrl Pts',(-12.6708780749975,-32.9125758101539,
26.2621282078519));
#35103=CARTESIAN_POINT('Ctrl Pts',(-12.6567160940558,-32.8945810458098,
26.2607493737556));
#35104=CARTESIAN_POINT('Ctrl Pts',(-12.6001872699501,-32.8242318317679,
26.2552728093567));
#35105=CARTESIAN_POINT('Ctrl Pts',(-12.5564486954784,-32.7730043106772,
26.2510944892195));
#35106=CARTESIAN_POINT('Ctrl Pts',(-12.4289817699211,-32.6324186583855,
26.2391567064824));
#35107=CARTESIAN_POINT('Ctrl Pts',(-12.3418970711533,-32.5462458637701,
26.2312749164038));
#35108=CARTESIAN_POINT('Ctrl Pts',(-12.0685078467215,-32.3035575717819,
26.2077110947291));
#35109=CARTESIAN_POINT('Ctrl Pts',(-11.8698006332764,-32.1621475627646,
26.1921269852289));
#35110=CARTESIAN_POINT('Ctrl Pts',(-11.612824737059,-32.0180808469371,26.1742103397903));
#35111=CARTESIAN_POINT('Ctrl Pts',(-11.5674357647263,-31.9939742143985,
26.1711196937653));
#35112=CARTESIAN_POINT('Ctrl Pts',(-11.4946398504755,-31.9574087950245,
26.1662765732097));
#35113=CARTESIAN_POINT('Ctrl Pts',(-11.4675863175996,-31.9442676800934,
26.1645009494808));
#35114=CARTESIAN_POINT('Ctrl Pts',(-11.41878173469,-31.9213587884274,26.1613399136456));
#35115=CARTESIAN_POINT('Ctrl Pts',(-11.3970960169682,-31.9114572882191,
26.1599500339689));
#35116=CARTESIAN_POINT('Ctrl Pts',(-11.3458355913086,-31.8887026251433,
26.1566981549842));
#35117=CARTESIAN_POINT('Ctrl Pts',(-11.3161780838081,-31.8760409497009,
26.15484267066));
#35118=CARTESIAN_POINT('Ctrl Pts',(-11.2272522331854,-31.8395670790632,
26.1493524451096));
#35119=CARTESIAN_POINT('Ctrl Pts',(-11.1674852575761,-31.8170040552819,
26.1457586504029));
#35120=CARTESIAN_POINT('Ctrl Pts',(-10.9515867180849,-31.7423989277845,
26.1330719643843));
#35121=CARTESIAN_POINT('Ctrl Pts',(-10.7923445334855,-31.7000487436451,
26.1242693340018));
#35122=CARTESIAN_POINT('Ctrl Pts',(-10.4225491747609,-31.630027421544,26.1042889504311));
#35123=CARTESIAN_POINT('Ctrl Pts',(-10.2112356651129,-31.6102175589044,
26.0932035591212));
#35124=CARTESIAN_POINT('Ctrl Pts',(-9.95506088281142,-31.610256853287,26.0788608354605));
#35125=CARTESIAN_POINT('Ctrl Pts',(-9.91064829397407,-31.6111367671557,
26.0763404584383));
#35126=CARTESIAN_POINT('Ctrl Pts',(-9.84684810430115,-31.6136557644243,
26.0726552101951));
#35127=CARTESIAN_POINT('Ctrl Pts',(-9.82743560367628,-31.6145894967909,
26.0715252803161));
#35128=CARTESIAN_POINT('Ctrl Pts',(-9.79311537120632,-31.6165362340046,
26.0695107111265));
#35129=CARTESIAN_POINT('Ctrl Pts',(-9.77820466278739,-31.6174809502731,
26.0686297381704));
#35130=CARTESIAN_POINT('Ctrl Pts',(-9.74529027420171,-31.6197849231823,
26.0666720297836));
#35131=CARTESIAN_POINT('Ctrl Pts',(-9.72729112865333,-31.6211894327692,
26.0655930101992));
#35132=CARTESIAN_POINT('Ctrl Pts',(-9.67369544307343,-31.625802643764,26.0623565514663));
#35133=CARTESIAN_POINT('Ctrl Pts',(-9.63813856958889,-31.629430530412,26.0601784950129));
#35134=CARTESIAN_POINT('Ctrl Pts',(-9.45998187875568,-31.6504593630266,
26.0491318455236));
#35135=CARTESIAN_POINT('Ctrl Pts',(-9.31854207937637,-31.6763498051946,
26.039937130674));
#35136=CARTESIAN_POINT('Ctrl Pts',(-8.914660216476,-31.7771482142732,26.0131334800925));
#35137=CARTESIAN_POINT('Ctrl Pts',(-8.65901798882663,-31.8748517235715,
25.9955698331783));
#35138=CARTESIAN_POINT('Ctrl Pts',(-8.37507263254275,-32.0247096409041,
25.9760997762504));
#35139=CARTESIAN_POINT('Ctrl Pts',(-8.33280865278018,-32.048184449669,25.9731991254146));
#35140=CARTESIAN_POINT('Ctrl Pts',(-8.26587225564731,-32.0872596031988,
25.9685989542391));
#35141=CARTESIAN_POINT('Ctrl Pts',(-8.24087522746037,-32.1022878391613,
25.9668795897919));
#35142=CARTESIAN_POINT('Ctrl Pts',(-8.19338731153039,-32.1316786207549,
25.9636094140972));
#35143=CARTESIAN_POINT('Ctrl Pts',(-8.17086607256977,-32.1459877231989,
25.9620568390419));
#35144=CARTESIAN_POINT('Ctrl Pts',(-8.11898913144285,-32.1798146036373,
25.9584753084798));
#35145=CARTESIAN_POINT('Ctrl Pts',(-8.08976398221491,-32.1995275315742,
25.9564536905079));
#35146=CARTESIAN_POINT('Ctrl Pts',(-7.99404942229286,-32.2662844860209,
25.9498141380747));
#35147=CARTESIAN_POINT('Ctrl Pts',(-7.92894577255225,-32.3152702134998,
25.9452684634052));
#35148=CARTESIAN_POINT('Ctrl Pts',(-7.77121350786264,-32.4431078872044,
25.934108786597));
#35149=CARTESIAN_POINT('Ctrl Pts',(-7.68094372798789,-32.5246884829679,
25.927589658665));
#35150=CARTESIAN_POINT('Ctrl Pts',(-7.46575488408208,-32.741291247819,25.9113503186686));
#35151=CARTESIAN_POINT('Ctrl Pts',(-7.34708032452994,-32.8819410982023,
25.9017322140363));
#35152=CARTESIAN_POINT('Ctrl Pts',(-7.19533725223829,-33.0946675905303,
25.8874490695594));
#35153=CARTESIAN_POINT('Ctrl Pts',(-7.15246625819151,-33.1593548466305,
25.8831343939313));
#35154=CARTESIAN_POINT('Ctrl Pts',(-7.09892266121463,-33.2464990398643,
25.8772813469308));
#35155=CARTESIAN_POINT('Ctrl Pts',(-7.08622096590751,-33.2676873817578,
25.8758551637343));
#35156=CARTESIAN_POINT('Ctrl Pts',(-7.06658944382127,-33.3012625408345,
25.8735873867013));
#35157=CARTESIAN_POINT('Ctrl Pts',(-7.05950364228452,-33.3135577090986,
25.8727552975367));
#35158=CARTESIAN_POINT('Ctrl Pts',(-7.04480723162945,-33.3394328983479,
25.8709999839324));
#35159=CARTESIAN_POINT('Ctrl Pts',(-7.03721266316546,-33.3530213835385,
25.8700757267377));
#35160=CARTESIAN_POINT('Ctrl Pts',(-7.01823261251563,-33.3875373185417,
25.8677227740536));
#35161=CARTESIAN_POINT('Ctrl Pts',(-7.00697379096015,-33.4085331627742,
25.8662866487066));
#35162=CARTESIAN_POINT('Ctrl Pts',(-6.96083415653091,-33.4967975148889,
25.8602346779064));
#35163=CARTESIAN_POINT('Ctrl Pts',(-6.92799473476246,-33.5651032391929,
25.8555163028674));
#35164=CARTESIAN_POINT('Ctrl Pts',(-6.83674094832738,-33.7724310680922,
25.8412094669498));
#35165=CARTESIAN_POINT('Ctrl Pts',(-6.78528281092349,-33.9143093400934,
25.8314457715305));
#35166=CARTESIAN_POINT('Ctrl Pts',(-6.68753696179293,-34.2526317979794,
25.80877642403));
#35167=CARTESIAN_POINT('Ctrl Pts',(-6.64898337271048,-34.4507473405117,
25.7959797191622));
#35168=CARTESIAN_POINT('Ctrl Pts',(-6.62279343430231,-34.7038722220211,
25.7804843580662));
#35169=CARTESIAN_POINT('Ctrl Pts',(-6.61857482675904,-34.756730354728,25.7772925334374));
#35170=CARTESIAN_POINT('Ctrl Pts',(-6.61388946112314,-34.8400435347316,
25.7723286541669));
#35171=CARTESIAN_POINT('Ctrl Pts',(-6.61259017752397,-34.8704413751505,
25.7705314700851));
#35172=CARTESIAN_POINT('Ctrl Pts',(-6.61092678106691,-34.9272873280363,
25.7671956110137));
#35173=CARTESIAN_POINT('Ctrl Pts',(-6.61046263334993,-34.9537299827227,
25.7656539849983));
#35174=CARTESIAN_POINT('Ctrl Pts',(-6.61011468400408,-35.0132253827938,
25.7622068996898));
#35175=CARTESIAN_POINT('Ctrl Pts',(-6.61040475210597,-35.0462766892399,
25.7603069109981));
#35176=CARTESIAN_POINT('Ctrl Pts',(-6.61277586923587,-35.1475797878267,
25.754525288429));
#35177=CARTESIAN_POINT('Ctrl Pts',(-6.61643571069143,-35.2157792211217,
25.7506916644));
#35178=CARTESIAN_POINT('Ctrl Pts',(-6.64315802820328,-35.5338058696532,
25.7330159722488));
#35179=CARTESIAN_POINT('Ctrl Pts',(-6.6918456095314,-35.7806764872546,25.7199452386104));
#35180=CARTESIAN_POINT('Ctrl Pts',(-6.81084117792656,-36.1578362115865,
25.6988479729883));
#35181=CARTESIAN_POINT('Ctrl Pts',(-6.86313051908764,-36.2928108712379,
25.6910334574032));
#35182=CARTESIAN_POINT('Ctrl Pts',(-6.93575178011109,-36.4496854204239,
25.6811891993183));
#35183=CARTESIAN_POINT('Ctrl Pts',(-6.94795354802824,-36.4752007712583,
25.679562836663));
#35184=CARTESIAN_POINT('Ctrl Pts',(-6.96778452493482,-36.5153703165132,
25.6769576509158));
#35185=CARTESIAN_POINT('Ctrl Pts',(-6.97520431449757,-36.5301270925732,
25.6759909060457));
#35186=CARTESIAN_POINT('Ctrl Pts',(-6.98973325513308,-36.5585041642485,
25.6741119671164));
#35187=CARTESIAN_POINT('Ctrl Pts',(-6.9968276296409,-36.5721312874253,25.6732006298927));
#35188=CARTESIAN_POINT('Ctrl Pts',(-7.01466688631889,-36.6058361793591,
25.6709248157731));
#35189=CARTESIAN_POINT('Ctrl Pts',(-7.0255218382554,-36.6258546177568,25.6695538529262));
#35190=CARTESIAN_POINT('Ctrl Pts',(-7.06875434913484,-36.7037007686679,
25.6641512264641));
#35191=CARTESIAN_POINT('Ctrl Pts',(-7.10262157527926,-36.7606801135123,
25.6600415945817));
#35192=CARTESIAN_POINT('Ctrl Pts',(-7.20200166040816,-36.917240903225,25.648382563442));
#35193=CARTESIAN_POINT('Ctrl Pts',(-7.27112757513383,-37.014413101441,25.6407166395166));
#35194=CARTESIAN_POINT('Ctrl Pts',(-7.49992639763282,-37.3025939195883,
25.6170007397345));
#35195=CARTESIAN_POINT('Ctrl Pts',(-7.67563763592788,-37.479855468991,25.6010379548524));
#35196=CARTESIAN_POINT('Ctrl Pts',(-7.90871828068696,-37.6682444692122,
25.5828196807745));
#35197=CARTESIAN_POINT('Ctrl Pts',(-7.94895756980383,-37.6992986394652,
25.5797640077375));
#35198=CARTESIAN_POINT('Ctrl Pts',(-8.01399975508353,-37.7471995306856,
25.574962692194));
#35199=CARTESIAN_POINT('Ctrl Pts',(-8.03835278508185,-37.7646414821188,
25.5731945696784));
#35200=CARTESIAN_POINT('Ctrl Pts',(-8.08468633467785,-37.796905647308,25.5698847600573));
#35201=CARTESIAN_POINT('Ctrl Pts',(-8.10661561672311,-37.8117971606208,
25.568340550792));
#35202=CARTESIAN_POINT('Ctrl Pts',(-8.15686934140836,-37.8450684227092,
25.5648508921096));
#35203=CARTESIAN_POINT('Ctrl Pts',(-8.185298473421,-37.8632854278068,25.562911515456));
#35204=CARTESIAN_POINT('Ctrl Pts',(-8.27548781193689,-37.9191946045994,
25.5568627889473));
#35205=CARTESIAN_POINT('Ctrl Pts',(-8.33818711939478,-37.9553372723505,
25.5528084362073));
#35206=CARTESIAN_POINT('Ctrl Pts',(-8.49195128019705,-38.037531518084,25.5431757673161));
#35207=CARTESIAN_POINT('Ctrl Pts',(-8.58403230329462,-38.0815330650078,
25.5376597002759));
#35208=CARTESIAN_POINT('Ctrl Pts',(-8.72212775165444,-38.1400235921513,
25.5296370091679));
#35209=CARTESIAN_POINT('Ctrl Pts',(-8.7666863409551,-38.1577908664127,25.5270848170772));
#35210=CARTESIAN_POINT('Ctrl Pts',(-9.00739007930714,-38.2478966858258,
25.5134385408668));
#35211=CARTESIAN_POINT('Ctrl Pts',(-9.20951422219543,-38.3029113453702,
25.502497526991));
#35212=CARTESIAN_POINT('Ctrl Pts',(-9.46092488778908,-38.3469298844386,
25.4882442732159));
#35213=CARTESIAN_POINT('Ctrl Pts',(-9.5066113265404,-38.353969114046,25.4856277679349));
#35214=CARTESIAN_POINT('Ctrl Pts',(-9.57084227228276,-38.3625249322152,
25.4818947086259));
#35215=CARTESIAN_POINT('Ctrl Pts',(-9.58927890880338,-38.3648266562847,
25.4808169174309));
#35216=CARTESIAN_POINT('Ctrl Pts',(-9.62272436181845,-38.3687231919704,
25.4788488872577));
#35217=CARTESIAN_POINT('Ctrl Pts',(-9.63772691868671,-38.3703695732399,
25.4779614017852));
#35218=CARTESIAN_POINT('Ctrl Pts',(-9.66936996797806,-38.3736283632646,
25.4760788717889));
#35219=CARTESIAN_POINT('Ctrl Pts',(-9.68601199357414,-38.375217927378,25.4750827051862));
#35220=CARTESIAN_POINT('Ctrl Pts',(-9.73177407710077,-38.37924752609,25.4723279986244));
#35221=CARTESIAN_POINT('Ctrl Pts',(-9.76091433394061,-38.3814341495968,
25.4705566925829));
#35222=CARTESIAN_POINT('Ctrl Pts',(-9.82699105636127,-38.3855340462016,
25.4665067398777));
#35223=CARTESIAN_POINT('Ctrl Pts',(-9.8639376220256,-38.3872200538519,25.4642186052806));
#35224=CARTESIAN_POINT('Ctrl Pts',(-9.98615734372112,-38.3907945940137,
25.4565867515744));
#35225=CARTESIAN_POINT('Ctrl Pts',(-10.07147127874,-38.3900693120792,25.4511593252153));
#35226=CARTESIAN_POINT('Ctrl Pts',(-10.4342491945548,-38.3732850748911,
25.4278701189639));
#35227=CARTESIAN_POINT('Ctrl Pts',(-10.7092555860482,-38.3263531081236,
25.4098055995211));
#35228=CARTESIAN_POINT('Ctrl Pts',(-11.0361673540544,-38.2281233395888,
25.3888702850396));
#35229=CARTESIAN_POINT('Ctrl Pts',(-11.0963530811589,-38.2081823210776,
25.385033244961));
#35230=CARTESIAN_POINT('Ctrl Pts',(-11.1865501928067,-38.1754627188258,
25.3793071009394));
#35231=CARTESIAN_POINT('Ctrl Pts',(-11.2169923098703,-38.1639207744977,
25.3773786800668));
#35232=CARTESIAN_POINT('Ctrl Pts',(-11.2718256535501,-38.1422225089752,
25.3739116159283));
#35233=CARTESIAN_POINT('Ctrl Pts',(-11.2962731030927,-38.132216290365,25.3723681843576));
#35234=CARTESIAN_POINT('Ctrl Pts',(-11.3489656455862,-38.1099268842096,
25.3690456386899));
#35235=CARTESIAN_POINT('Ctrl Pts',(-11.3771654836561,-38.0975423901317,
25.3672700622237));
#35236=CARTESIAN_POINT('Ctrl Pts',(-11.4564834654865,-38.0614110360573,
25.3622803699208));
#35237=CARTESIAN_POINT('Ctrl Pts',(-11.5071848006246,-38.0367706696,25.3590963787428));
#35238=CARTESIAN_POINT('Ctrl Pts',(-11.6213302696875,-37.9777336868732,
25.3519221203194));
#35239=CARTESIAN_POINT('Ctrl Pts',(-11.6843382284646,-37.9425525207368,
25.347957763896));
#35240=CARTESIAN_POINT('Ctrl Pts',(-11.9113616681144,-37.8061082065748,
25.3335721351127));
#35241=CARTESIAN_POINT('Ctrl Pts',(-12.0677762878915,-37.6929258019597,
25.3234801161834));
#35242=CARTESIAN_POINT('Ctrl Pts',(-12.3270309109062,-37.4693555238239,
25.3052357620447));
#35243=CARTESIAN_POINT('Ctrl Pts',(-12.4337297570218,-37.3642630279971,
25.2971662790281));
#35244=CARTESIAN_POINT('Ctrl Pts',(-12.5519368459782,-37.2313279986519,
25.2870363961496));
#35245=CARTESIAN_POINT('Ctrl Pts',(-12.5704799050936,-37.2099410059806,
25.285408719021));
#35246=CARTESIAN_POINT('Ctrl Pts',(-12.5994186509405,-37.1757069488328,
25.2828019115322));
#35247=CARTESIAN_POINT('Ctrl Pts',(-12.6099923539027,-37.1630113124236,
25.2818348850014));
#35248=CARTESIAN_POINT('Ctrl Pts',(-12.6302166226172,-37.1383642209727,
25.2799558287584));
#35249=CARTESIAN_POINT('Ctrl Pts',(-12.6398794290999,-37.1264236616857,
25.2790446616619));
#35250=CARTESIAN_POINT('Ctrl Pts',(-12.6636560058445,-37.0966305492294,
25.2767698985695));
#35251=CARTESIAN_POINT('Ctrl Pts',(-12.6776716534895,-37.078700900043,25.2753998294631));
#35252=CARTESIAN_POINT('Ctrl Pts',(-12.7317201533232,-37.0081051699611,
25.27000552723));
#35253=CARTESIAN_POINT('Ctrl Pts',(-12.7703861561577,-36.9544157040958,
25.265903618178));
#35254=CARTESIAN_POINT('Ctrl Pts',(-12.8788188305548,-36.7941638573607,
25.253739180942));
#35255=CARTESIAN_POINT('Ctrl Pts',(-12.9441804497685,-36.6847612420923,
25.2455361145666));
#35256=CARTESIAN_POINT('Ctrl Pts',(-13.1084485628498,-36.3709243740313,
25.2227023152081));
#35257=CARTESIAN_POINT('Ctrl Pts',(-13.1932326572253,-36.15981814523,25.2081578691538));
#35258=CARTESIAN_POINT('Ctrl Pts',(-13.2711802378338,-35.8903131964984,
25.1910045978432));
#35259=CARTESIAN_POINT('Ctrl Pts',(-13.2848489513258,-35.838478139077,25.1877641573827));
#35260=CARTESIAN_POINT('Ctrl Pts',(-13.3050041925644,-35.7539629530655,
25.1825737660494));
#35261=CARTESIAN_POINT('Ctrl Pts',(-13.312248065908,-35.7214746813781,25.1806004950809));
#35262=CARTESIAN_POINT('Ctrl Pts',(-13.324390475741,-35.6629730989752,25.1770853115999));
#35263=CARTESIAN_POINT('Ctrl Pts',(-13.3294649830156,-35.6369994905114,
25.1755379974232));
#35264=CARTESIAN_POINT('Ctrl Pts',(-13.3387175443593,-35.5865055452396,
25.1725548612563));
#35265=CARTESIAN_POINT('Ctrl Pts',(-13.3429308949007,-35.5619934832242,
25.1711180294128));
#35266=CARTESIAN_POINT('Ctrl Pts',(-13.3516007611882,-35.5080021073847,
25.1679769160015));
#35267=CARTESIAN_POINT('Ctrl Pts',(-13.355938936534,-35.4785057328764,25.1662763497801));
#35268=CARTESIAN_POINT('Ctrl Pts',(-13.3674688356676,-35.3922183796251,
25.161343561259));
#35269=CARTESIAN_POINT('Ctrl Pts',(-13.3736120590693,-35.3352965699076,
25.158142570588));
#35270=CARTESIAN_POINT('Ctrl Pts',(-13.3860065529804,-35.1848084218353,
25.1497937535001));
#35271=CARTESIAN_POINT('Ctrl Pts',(-13.3898226926569,-35.0910913397411,
25.1447109691293));
#35272=CARTESIAN_POINT('Ctrl Pts',(-13.3897489515553,-34.9973339299542,
25.1396837753564));
#35273=CARTESIAN_POINT('Ctrl Pts',(-13.389748954038,-34.9973370883974,25.1396839447095));
#35274=CARTESIAN_POINT('Ctrl Pts',(-13.3895886446596,-34.7932715281918,
25.1287421175687));
#35275=CARTESIAN_POINT('Ctrl Pts',(-13.371001697134,-34.5896392054684,25.1181177862061));
#35276=CARTESIAN_POINT('Ctrl Pts',(-13.3222361968378,-34.3235637280122,
25.1034711517141));
#35277=CARTESIAN_POINT('Ctrl Pts',(-13.3083405108317,-34.258581387182,25.0998294964393));
#35278=CARTESIAN_POINT('Ctrl Pts',(-13.2818257879657,-34.1502604925755,
25.0935894458589));
#35279=CARTESIAN_POINT('Ctrl Pts',(-13.2702342466418,-34.1066885748227,
25.0910324631202));
#35280=CARTESIAN_POINT('Ctrl Pts',(-13.2523190069828,-34.0443764191298,
25.0872911150932));
#35281=CARTESIAN_POINT('Ctrl Pts',(-13.2466944756061,-34.0254384099583,
25.086142674056));
#35282=CARTESIAN_POINT('Ctrl Pts',(-13.2365262793365,-33.992266941969,25.0841093394122));
#35283=CARTESIAN_POINT('Ctrl Pts',(-13.2320535534741,-33.9780126769839,
25.0832284129384));
#35284=CARTESIAN_POINT('Ctrl Pts',(-13.2219643393755,-33.9465878301534,
25.0812700861574));
#35285=CARTESIAN_POINT('Ctrl Pts',(-13.2163048048448,-33.9294324991637,
25.0801903914591));
#35286=CARTESIAN_POINT('Ctrl Pts',(-13.2003412141904,-33.8823125588762,
25.0771971170973));
#35287=CARTESIAN_POINT('Ctrl Pts',(-13.1897539871707,-33.8524467622835,
25.0752688638173));
#35288=CARTESIAN_POINT('Ctrl Pts',(-13.1787501240264,-33.8227350716589,
25.0733224007726));
#35289=CARTESIAN_POINT('Ctrl Pts',(-13.1787501041971,-33.8227350181174,
25.4139789249709));
#35290=CARTESIAN_POINT('Ctrl Pts',(-13.2129572634916,-33.9150982607561,
25.419220516707));
#35291=CARTESIAN_POINT('Ctrl Pts',(-13.2431511806743,-34.0089857317186,
25.4244249055303));
#35292=CARTESIAN_POINT('Ctrl Pts',(-13.3114018017695,-34.2580493560975,
25.4381640698729));
#35293=CARTESIAN_POINT('Ctrl Pts',(-13.3426519766591,-34.4147313341876,
25.4467386760083));
#35294=CARTESIAN_POINT('Ctrl Pts',(-13.3663308146369,-34.6012141985136,
25.4574414958164));
#35295=CARTESIAN_POINT('Ctrl Pts',(-13.3695568005663,-34.6294596858261,
25.459076027929));
#35296=CARTESIAN_POINT('Ctrl Pts',(-13.3740979302152,-34.6742054682466,
25.4616912925964));
#35297=CARTESIAN_POINT('Ctrl Pts',(-13.3756481974522,-34.6906811651713,
25.4626597874223));
#35298=CARTESIAN_POINT('Ctrl Pts',(-13.3783881988411,-34.7222800736297,
25.4645289931918));
#35299=CARTESIAN_POINT('Ctrl Pts',(-13.3795971498082,-34.7374009685751,
25.4654286768883));
#35300=CARTESIAN_POINT('Ctrl Pts',(-13.3823498932698,-34.7750062334487,
25.4676783979022));
#35301=CARTESIAN_POINT('Ctrl Pts',(-13.3837709941551,-34.7974986553637,
25.4690348218451));
#35302=CARTESIAN_POINT('Ctrl Pts',(-13.3881296072056,-34.8794653319769,
25.4740132425915));
#35303=CARTESIAN_POINT('Ctrl Pts',(-13.3897239753482,-34.9389972047508,
25.4776966446478));
#35304=CARTESIAN_POINT('Ctrl Pts',(-13.389794204562,-35.1016409861366,25.4878913106812));
#35305=CARTESIAN_POINT('Ctrl Pts',(-13.3851345470166,-35.204689100525,25.4944934049557));
#35306=CARTESIAN_POINT('Ctrl Pts',(-13.3515711786711,-35.5733225716754,
25.5183172007609));
#35307=CARTESIAN_POINT('Ctrl Pts',(-13.2960042769614,-35.8355401828051,
25.5355547403311));
#35308=CARTESIAN_POINT('Ctrl Pts',(-13.1929877658504,-36.1393475372853,
25.5550977597033));
#35309=CARTESIAN_POINT('Ctrl Pts',(-13.1745538687943,-36.1897444721278,
25.5583290371695));
#35310=CARTESIAN_POINT('Ctrl Pts',(-13.1437547084232,-36.2681266632395,
25.5633399240688));
#35311=CARTESIAN_POINT('Ctrl Pts',(-13.1321945298213,-36.2964167615916,
25.565145452981));
#35312=CARTESIAN_POINT('Ctrl Pts',(-13.1099245549794,-36.3488784241009,
25.5684890536845));
#35313=CARTESIAN_POINT('Ctrl Pts',(-13.0993115814652,-36.3730883147344,
25.5700301974044));
#35314=CARTESIAN_POINT('Ctrl Pts',(-13.0748704925588,-36.427114770452,25.5734663663822));
#35315=CARTESIAN_POINT('Ctrl Pts',(-13.0608896441662,-36.4568595706773,
25.5753560782388));
#35316=CARTESIAN_POINT('Ctrl Pts',(-13.0169917442215,-36.5468314821119,
25.5810694871647));
#35317=CARTESIAN_POINT('Ctrl Pts',(-12.9857124468639,-36.6063775501698,
25.5848468795753));
#35318=CARTESIAN_POINT('Ctrl Pts',(-12.8303869168392,-36.8818362195399,
25.6023724886231));
#35319=CARTESIAN_POINT('Ctrl Pts',(-12.6845741895147,-37.0845777120648,
25.6153579235765));
#35320=CARTESIAN_POINT('Ctrl Pts',(-12.4187419946939,-37.3794981642517,
25.6365239427438));
#35321=CARTESIAN_POINT('Ctrl Pts',(-12.3125290895914,-37.4828460358857,
25.6445138166512));
#35322=CARTESIAN_POINT('Ctrl Pts',(-12.1783851838074,-37.5972762493921,
25.6545544356736));
#35323=CARTESIAN_POINT('Ctrl Pts',(-12.1566266061187,-37.6153713876843,
25.6561817391956));
#35324=CARTESIAN_POINT('Ctrl Pts',(-12.1218111934531,-37.6435951395608,
25.6587880855468));
#35325=CARTESIAN_POINT('Ctrl Pts',(-12.1089020023421,-37.6539047311729,
25.6597550318242));
#35326=CARTESIAN_POINT('Ctrl Pts',(-12.0838449286878,-37.6736176539674,
25.6616340540304));
#35327=CARTESIAN_POINT('Ctrl Pts',(-12.0717076683729,-37.6830334230064,
25.6625452689832));
#35328=CARTESIAN_POINT('Ctrl Pts',(-12.0414282470533,-37.7061954614059,
25.6648203290142));
#35329=CARTESIAN_POINT('Ctrl Pts',(-12.0232109799637,-37.7198419865925,
25.6661906508364));
#35330=CARTESIAN_POINT('Ctrl Pts',(-11.9514880592596,-37.7724502247904,
25.6715873077567));
#35331=CARTESIAN_POINT('Ctrl Pts',(-11.8969862249369,-37.8100227728828,
25.675691401441));
#35332=CARTESIAN_POINT('Ctrl Pts',(-11.7415854188545,-37.9105713946347,
25.6873281520633));
#35333=CARTESIAN_POINT('Ctrl Pts',(-11.6384216439193,-37.9698682801586,
25.6949768743176));
#35334=CARTESIAN_POINT('Ctrl Pts',(-11.3100229291648,-38.1362997480817,
25.7187054880072));
#35335=CARTESIAN_POINT('Ctrl Pts',(-11.0758985346293,-38.2241301926879,
25.7346991449924));
#35336=CARTESIAN_POINT('Ctrl Pts',(-10.7844420210448,-38.2981350251136,
25.7529781359782));
#35337=CARTESIAN_POINT('Ctrl Pts',(-10.7343692539989,-38.309644415842,25.7560663467279));
#35338=CARTESIAN_POINT('Ctrl Pts',(-10.6548760180456,-38.3260231273484,
25.7608891748018));
#35339=CARTESIAN_POINT('Ctrl Pts',(-10.6256213060734,-38.331649817864,25.7626471679003));
#35340=CARTESIAN_POINT('Ctrl Pts',(-10.5701751945687,-38.3415579252178,
25.765948275864));
#35341=CARTESIAN_POINT('Ctrl Pts',(-10.5440004526708,-38.3459188105124,
25.7674937599726));
#35342=CARTESIAN_POINT('Ctrl Pts',(-10.4841385288724,-38.3551711582749,
25.7710001505805));
#35343=CARTESIAN_POINT('Ctrl Pts',(-10.4504231877382,-38.3598634925088,
25.772954751293));
#35344=CARTESIAN_POINT('Ctrl Pts',(-10.3432344720431,-38.3731389655881,
25.7791092898475));
#35345=CARTESIAN_POINT('Ctrl Pts',(-10.2695458403651,-38.3798258098917,
25.7832513239744));
#35346=CARTESIAN_POINT('Ctrl Pts',(-10.0905440204856,-38.3901770211333,
25.7931478901322));
#35347=CARTESIAN_POINT('Ctrl Pts',(-9.9851639209605,-38.3913537642606,25.7988351237834));
#35348=CARTESIAN_POINT('Ctrl Pts',(-9.75584331201983,-38.3832234372192,
25.8110955807886));
#35349=CARTESIAN_POINT('Ctrl Pts',(-9.63212701842956,-38.3720146546837,
25.8176355307134));
#35350=CARTESIAN_POINT('Ctrl Pts',(-9.36614070135747,-38.3331009518414,
25.8319428517003));
#35351=CARTESIAN_POINT('Ctrl Pts',(-9.2244776685438,-38.3030133054572,25.8397194017971));
#35352=CARTESIAN_POINT('Ctrl Pts',(-9.05086013906078,-38.254352363876,25.849900232811));
#35353=CARTESIAN_POINT('Ctrl Pts',(-9.01669095744491,-38.2441915633943,
25.8519363366232));
#35354=CARTESIAN_POINT('Ctrl Pts',(-8.96548552225046,-38.2280814957475,
25.8550453996338));
#35355=CARTESIAN_POINT('Ctrl Pts',(-8.94832512701744,-38.2225316565853,
25.8560972087198));
#35356=CARTESIAN_POINT('Ctrl Pts',(-8.91702914806747,-38.2121336366651,
25.8580349042542));
#35357=CARTESIAN_POINT('Ctrl Pts',(-8.9028801765355,-38.2073285507279,25.8589183815811));
#35358=CARTESIAN_POINT('Ctrl Pts',(-8.87006229146392,-38.1959408131902,
25.8609847393125));
#35359=CARTESIAN_POINT('Ctrl Pts',(-8.85141882194449,-38.189288030629,25.8621714824119));
#35360=CARTESIAN_POINT('Ctrl Pts',(-8.79028749083757,-38.1668682492365,
25.8661027488397));
#35361=CARTESIAN_POINT('Ctrl Pts',(-8.74805912484931,-38.150413066012,25.868882262076));
#35362=CARTESIAN_POINT('Ctrl Pts',(-8.64431527820294,-38.1075719227212,
25.8758485440499));
#35363=CARTESIAN_POINT('Ctrl Pts',(-8.58322809779685,-38.0802014207884,
25.8800726204313));
#35364=CARTESIAN_POINT('Ctrl Pts',(-8.27084281022892,-37.9289761100363,
25.9021822029667));
#35365=CARTESIAN_POINT('Ctrl Pts',(-8.03475214678143,-37.7760984401869,
25.9205165747857));
#35366=CARTESIAN_POINT('Ctrl Pts',(-7.75821188526995,-37.5438820513353,
25.9429015005832));
#35367=CARTESIAN_POINT('Ctrl Pts',(-7.69813674202134,-37.4896539955077,
25.947838930622));
#35368=CARTESIAN_POINT('Ctrl Pts',(-7.61666811687911,-37.410642169025,25.9546427428696));
#35369=CARTESIAN_POINT('Ctrl Pts',(-7.59360813427828,-37.3876232600545,
25.9565816447087));
#35370=CARTESIAN_POINT('Ctrl Pts',(-7.55207491946181,-37.3449509628874,
25.9600989999674));
#35371=CARTESIAN_POINT('Ctrl Pts',(-7.53349772445642,-37.3254029340383,
25.961681854077));
#35372=CARTESIAN_POINT('Ctrl Pts',(-7.49616355970659,-37.2851669018394,
25.9648836059633));
#35373=CARTESIAN_POINT('Ctrl Pts',(-7.4774249821693,-37.2644646246677,25.9665016688372));
#35374=CARTESIAN_POINT('Ctrl Pts',(-7.43096969455841,-37.2118487255616,
25.9705429356919));
#35375=CARTESIAN_POINT('Ctrl Pts',(-7.40358969162847,-37.1796433719326,
25.9729523743342));
#35376=CARTESIAN_POINT('Ctrl Pts',(-7.28529368550675,-37.0351060836231,
25.9835005559506));
#35377=CARTESIAN_POINT('Ctrl Pts',(-7.20100857082505,-36.9175349346139,
25.991381432895));
#35378=CARTESIAN_POINT('Ctrl Pts',(-7.05441355906147,-36.6826865021368,
26.0062225217367));
#35379=CARTESIAN_POINT('Ctrl Pts',(-6.99098006290977,-36.5664331386744,
26.0131932043671));
#35380=CARTESIAN_POINT('Ctrl Pts',(-6.87006125878939,-36.3102237985343,
26.0282565425033));
#35381=CARTESIAN_POINT('Ctrl Pts',(-6.81481892294492,-36.1695365786471,
26.0363522838461));
#35382=CARTESIAN_POINT('Ctrl Pts',(-6.75825114706546,-35.9913450430184,
26.0469045926988));
#35383=CARTESIAN_POINT('Ctrl Pts',(-6.74790789526704,-35.9568685101434,
26.0489599117236));
#35384=CARTESIAN_POINT('Ctrl Pts',(-6.73319066519045,-35.9048146605224,
26.0520924790329));
#35385=CARTESIAN_POINT('Ctrl Pts',(-6.72840507145545,-35.887355279121,26.0531480972335));
#35386=CARTESIAN_POINT('Ctrl Pts',(-6.71996330565019,-35.8555601733856,
26.055080784534));
#35387=CARTESIAN_POINT('Ctrl Pts',(-6.71626080182107,-35.8412376477149,
26.0559552758819));
#35388=CARTESIAN_POINT('Ctrl Pts',(-6.70786670185911,-35.8078664835325,
26.058001720546));
#35389=CARTESIAN_POINT('Ctrl Pts',(-6.7032466080321,-35.7888009507106,26.0591774800221));
#35390=CARTESIAN_POINT('Ctrl Pts',(-6.68874004512308,-35.7265827244959,
26.0630334589216));
#35391=CARTESIAN_POINT('Ctrl Pts',(-6.67953378370474,-35.6832778757785,
26.0657469316272));
#35392=CARTESIAN_POINT('Ctrl Pts',(-6.65895609562506,-35.5762152776175,
26.072508098465));
#35393=CARTESIAN_POINT('Ctrl Pts',(-6.64855888022745,-35.5122889800574,
26.0765905603229));
#35394=CARTESIAN_POINT('Ctrl Pts',(-6.60654095726604,-35.1972301629496,
26.0968182803444));
#35395=CARTESIAN_POINT('Ctrl Pts',(-6.60128315806256,-34.9433621271681,
26.1133733876838));
#35396=CARTESIAN_POINT('Ctrl Pts',(-6.63379626043595,-34.58785613312,26.1357417760478));
#35397=CARTESIAN_POINT('Ctrl Pts',(-6.64800289240874,-34.4849185214098,
26.1421323788901));
#35398=CARTESIAN_POINT('Ctrl Pts',(-6.67408617961277,-34.3440630302138,
26.1507498057135));
#35399=CARTESIAN_POINT('Ctrl Pts',(-6.68193156180881,-34.3054655626707,
26.1530981300991));
#35400=CARTESIAN_POINT('Ctrl Pts',(-6.6963059968704,-34.240562780938,26.1570263339079));
#35401=CARTESIAN_POINT('Ctrl Pts',(-6.70248092819276,-34.2141838697252,
26.1586171277142));
#35402=CARTESIAN_POINT('Ctrl Pts',(-6.71562190038833,-34.1609314207618,
26.1618177740163));
#35403=CARTESIAN_POINT('Ctrl Pts',(-6.7226031572945,-34.134063752851,26.1634270074025));
#35404=CARTESIAN_POINT('Ctrl Pts',(-6.74082766727707,-34.0673059747721,
26.1674131029878));
#35405=CARTESIAN_POINT('Ctrl Pts',(-6.75247404875212,-34.027530028233,26.1697770068922));
#35406=CARTESIAN_POINT('Ctrl Pts',(-6.80488914833904,-33.859973807664,26.1796998190131));
#35407=CARTESIAN_POINT('Ctrl Pts',(-6.85249455974218,-33.7344535966079,
26.1870397376459));
#35408=CARTESIAN_POINT('Ctrl Pts',(-6.96432232106842,-33.4852783937836,
26.2017255878084));
#35409=CARTESIAN_POINT('Ctrl Pts',(-7.02897240599284,-33.3621000178203,
26.2090483043451));
#35410=CARTESIAN_POINT('Ctrl Pts',(-7.18222353086735,-33.109205826839,26.2247596311003));
#35411=CARTESIAN_POINT('Ctrl Pts',(-7.27263585152958,-32.9809799028101,
26.233146776698));
#35412=CARTESIAN_POINT('Ctrl Pts',(-7.39421758924553,-32.8316854329314,
26.2440158992788));
#35413=CARTESIAN_POINT('Ctrl Pts',(-7.4172920549161,-32.8042519519879,26.246063051668));
#35414=CARTESIAN_POINT('Ctrl Pts',(-7.45264863034253,-32.7635445997001,
26.2491856309586));
#35415=CARTESIAN_POINT('Ctrl Pts',(-7.46460969206261,-32.7499938416638,
26.2502396323647));
#35416=CARTESIAN_POINT('Ctrl Pts',(-7.48665385528628,-32.725418850499,26.2521792628443));
#35417=CARTESIAN_POINT('Ctrl Pts',(-7.49670227708665,-32.714364698152,26.2530624460443));
#35418=CARTESIAN_POINT('Ctrl Pts',(-7.52019945817633,-32.6888565369721,
26.2551253135916));
#35419=CARTESIAN_POINT('Ctrl Pts',(-7.53370173168165,-32.6744532590733,
26.2563088142036));
#35420=CARTESIAN_POINT('Ctrl Pts',(-7.57839587030927,-32.6276037053638,
26.2602177389312));
#35421=CARTESIAN_POINT('Ctrl Pts',(-7.61010701372241,-32.5956618706364,
26.2629776330275));
#35422=CARTESIAN_POINT('Ctrl Pts',(-7.69006631473472,-32.5182658650929,
26.2698827521669));
#35423=CARTESIAN_POINT('Ctrl Pts',(-7.73902908824637,-32.473578103648,26.2740645185709));
#35424=CARTESIAN_POINT('Ctrl Pts',(-7.99505764738329,-32.2533099340334,
26.2955736995837));
#35425=CARTESIAN_POINT('Ctrl Pts',(-8.22140544168132,-32.1015983993868,
26.3133384524663));
#35426=CARTESIAN_POINT('Ctrl Pts',(-8.5421804687877,-31.9384689103824,26.3357261314496));
#35427=CARTESIAN_POINT('Ctrl Pts',(-8.62247034456128,-31.9015125373524,
26.341132176333));
#35428=CARTESIAN_POINT('Ctrl Pts',(-8.73840037337257,-31.853549958443,26.3486613063678));
#35429=CARTESIAN_POINT('Ctrl Pts',(-8.77291390409971,-31.8399301654411,
26.3508692307131));
#35430=CARTESIAN_POINT('Ctrl Pts',(-8.83288295510866,-31.8173957595879,
26.3546494168831));
#35431=CARTESIAN_POINT('Ctrl Pts',(-8.85823353818087,-31.8082134537633,
26.3562303392996));
#35432=CARTESIAN_POINT('Ctrl Pts',(-8.91054866164516,-31.7899673068413,
26.3594589016785));
#35433=CARTESIAN_POINT('Ctrl Pts',(-8.93752319627041,-31.7809384561716,
26.3611053000019));
#35434=CARTESIAN_POINT('Ctrl Pts',(-9.00730686013322,-31.7585533917055,
26.3653195122652));
#35435=CARTESIAN_POINT('Ctrl Pts',(-9.05027380715635,-31.7457049600124,
26.3678709409509));
#35436=CARTESIAN_POINT('Ctrl Pts',(-9.28076529627067,-31.6817350555673,
26.3813481869752));
#35437=CARTESIAN_POINT('Ctrl Pts',(-9.47217660170899,-31.645958513302,26.3917789287601));
#35438=CARTESIAN_POINT('Ctrl Pts',(-9.86988956466424,-31.6065336636191,
26.4130034303189));
#35439=CARTESIAN_POINT('Ctrl Pts',(-10.0755613419869,-31.6048831516737,
26.4237460936282));
#35440=CARTESIAN_POINT('Ctrl Pts',(-10.3305179848077,-31.6260227368063,
26.4379828610382));
#35441=CARTESIAN_POINT('Ctrl Pts',(-10.3808353652946,-31.631331332962,26.4408389212348));
#35442=CARTESIAN_POINT('Ctrl Pts',(-10.4520974594067,-31.6404665742537,
26.4449731134135));
#35443=CARTESIAN_POINT('Ctrl Pts',(-10.473156123429,-31.6433677317321,26.446205945882));
#35444=CARTESIAN_POINT('Ctrl Pts',(-10.5091345892581,-31.6486696134076,
26.4483334095148));
#35445=CARTESIAN_POINT('Ctrl Pts',(-10.5240679906151,-31.6509723612199,
26.4492227489572));
#35446=CARTESIAN_POINT('Ctrl Pts',(-10.5559164797611,-31.6561016756259,
26.4511335902493));
#35447=CARTESIAN_POINT('Ctrl Pts',(-10.5728255565746,-31.6589567512475,
26.4521564984432));
#35448=CARTESIAN_POINT('Ctrl Pts',(-10.6205009856308,-31.6673792374303,
26.4550629539747));
#35449=CARTESIAN_POINT('Ctrl Pts',(-10.6512122412304,-31.6732440596472,
26.4569615608066));
#35450=CARTESIAN_POINT('Ctrl Pts',(-10.836672362302,-31.7113271106378,26.4685691744811));
#35451=CARTESIAN_POINT('Ctrl Pts',(-10.9890816830527,-31.7539102136194,
26.4787014293021));
#35452=CARTESIAN_POINT('Ctrl Pts',(-11.3858389876231,-31.8953085214995,
26.5058354895143));
#35453=CARTESIAN_POINT('Ctrl Pts',(-11.6226409072967,-32.0122351439981,
26.5227618272676));
#35454=CARTESIAN_POINT('Ctrl Pts',(-11.8852248964148,-32.1824126316501,
26.5417572993969));
#35455=CARTESIAN_POINT('Ctrl Pts',(-11.9263039295433,-32.2103360326956,
26.5447398694716));
#35456=CARTESIAN_POINT('Ctrl Pts',(-11.9907327384722,-32.2562334583408,
26.5494373778344));
#35457=CARTESIAN_POINT('Ctrl Pts',(-12.0144862833857,-32.2736257103926,
26.5511736749775));
#35458=CARTESIAN_POINT('Ctrl Pts',(-12.0592727073015,-32.3073230854144,
26.5544569288129));
#35459=CARTESIAN_POINT('Ctrl Pts',(-12.0803459229166,-32.3235706716264,
26.5560059195984));
#35460=CARTESIAN_POINT('Ctrl Pts',(-12.1284420332533,-32.3615643835789,
26.5595520838058));
#35461=CARTESIAN_POINT('Ctrl Pts',(-12.1553270775538,-32.3834806887348,
26.5615424030793));
#35462=CARTESIAN_POINT('Ctrl Pts',(-12.2414728540983,-32.4559344303847,
26.5679513397322));
#35463=CARTESIAN_POINT('Ctrl Pts',(-12.2993314179036,-32.5081038435288,
26.5723047372074));
#35464=CARTESIAN_POINT('Ctrl Pts',(-12.4370656755033,-32.641180676283,26.5828522676746));
#35465=CARTESIAN_POINT('Ctrl Pts',(-12.5147680926914,-32.7242009170442,
26.5889656108552));
#35466=CARTESIAN_POINT('Ctrl Pts',(-12.7392859507738,-32.9896553456035,
26.6074936889142));
#35467=CARTESIAN_POINT('Ctrl Pts',(-12.871489288313,-33.1834918118743,26.6196426154485));
#35468=CARTESIAN_POINT('Ctrl Pts',(-13.0057340614978,-33.4320953232967,
26.6353892693375));
#35469=CARTESIAN_POINT('Ctrl Pts',(-13.0278814834501,-33.475304765655,26.6381332859469));
#35470=CARTESIAN_POINT('Ctrl Pts',(-13.0573717272145,-33.5360183428181,
26.6420189060492));
#35471=CARTESIAN_POINT('Ctrl Pts',(-13.0655080173236,-33.553132787245,26.6431174733388));
#35472=CARTESIAN_POINT('Ctrl Pts',(-13.0799026601356,-33.5840780026437,
26.6451112449979));
#35473=CARTESIAN_POINT('Ctrl Pts',(-13.0862125285197,-33.5978845551625,
26.6460034342897));
#35474=CARTESIAN_POINT('Ctrl Pts',(-13.0991978172164,-33.6268098908368,
26.6478789637757));
#35475=CARTESIAN_POINT('Ctrl Pts',(-13.1058556962028,-33.6419357322663,
26.6488632232741));
#35476=CARTESIAN_POINT('Ctrl Pts',(-13.1236240344906,-33.6831172084403,
26.6515512100539));
#35477=CARTESIAN_POINT('Ctrl Pts',(-13.1345186940054,-33.7092638385882,
26.6532667455711));
#35478=CARTESIAN_POINT('Ctrl Pts',(-13.1567086308783,-33.7644568695072,
26.6569020894987));
#35479=CARTESIAN_POINT('Ctrl Pts',(-13.1679315584425,-33.793523706734,26.6588246380766));
#35480=CARTESIAN_POINT('Ctrl Pts',(-13.1787501100144,-33.8227350338248,
26.6607619345813));
#35481=CARTESIAN_POINT('Origin',(-10.,-35.,23.));
#35482=CARTESIAN_POINT('',(-13.1787501240207,-33.8227350716434,27.9134187994658));
#35483=CARTESIAN_POINT('',(-13.1787501609633,-33.8227351713926,27.5681448070208));
#35484=CARTESIAN_POINT('',(-13.1787501240207,-33.8227350716434,23.));
#35485=CARTESIAN_POINT('Ctrl Pts',(-13.1787501609633,-33.8227351713926,
27.5681448070208));
#35486=CARTESIAN_POINT('Ctrl Pts',(-13.1643813608665,-33.7839377619137,
27.5655680901549));
#35487=CARTESIAN_POINT('Ctrl Pts',(-13.1492995268026,-33.7453960250088,
27.5630098028168));
#35488=CARTESIAN_POINT('Ctrl Pts',(-13.1092449476349,-33.6483163142835,
27.5565712050213));
#35489=CARTESIAN_POINT('Ctrl Pts',(-13.0833267073364,-33.5901949926469,
27.5527215942986));
#35490=CARTESIAN_POINT('Ctrl Pts',(-13.0418498987587,-33.5038078207362,
27.5470054725543));
#35491=CARTESIAN_POINT('Ctrl Pts',(-13.0275001359323,-33.4749803679706,
27.5450989013236));
#35492=CARTESIAN_POINT('Ctrl Pts',(-13.0018174493583,-33.4251777478082,
27.541805575749));
#35493=CARTESIAN_POINT('Ctrl Pts',(-12.9906701651826,-33.4041099250419,
27.5404125606289));
#35494=CARTESIAN_POINT('Ctrl Pts',(-12.964940509539,-33.3566986492947,27.5372772306927));
#35495=CARTESIAN_POINT('Ctrl Pts',(-12.950227387756,-33.3304281988641,27.5355396253448));
#35496=CARTESIAN_POINT('Ctrl Pts',(-12.9093833772063,-33.2597270433301,
27.5308598489441));
#35497=CARTESIAN_POINT('Ctrl Pts',(-12.8825854768214,-33.2156897803185,
27.5279413885189));
#35498=CARTESIAN_POINT('Ctrl Pts',(-12.7246105800999,-32.9689422747003,
27.5115334046535));
#35499=CARTESIAN_POINT('Ctrl Pts',(-12.573077890682,-32.7800946832824,27.4988217574958));
#35500=CARTESIAN_POINT('Ctrl Pts',(-12.2771947268719,-32.4827645222447,
27.4765592928455));
#35501=CARTESIAN_POINT('Ctrl Pts',(-12.141904666696,-32.3666902011078,27.4670685685695));
#35502=CARTESIAN_POINT('Ctrl Pts',(-11.9741568379915,-32.2442801585959,
27.455263900406));
#35503=CARTESIAN_POINT('Ctrl Pts',(-11.949938424716,-32.227090503062,27.4535585315313));
#35504=CARTESIAN_POINT('Ctrl Pts',(-11.9116558996629,-32.2006679958829,
27.4508558875668));
#35505=CARTESIAN_POINT('Ctrl Pts',(-11.897743034697,-32.1912174708495,27.4498722689473));
#35506=CARTESIAN_POINT('Ctrl Pts',(-11.8711037197195,-32.173410586427,27.4479850771965));
#35507=CARTESIAN_POINT('Ctrl Pts',(-11.8583904396998,-32.1650358411843,
27.447082696634));
#35508=CARTESIAN_POINT('Ctrl Pts',(-11.8301063356236,-32.14667597092,27.4450718566857));
#35509=CARTESIAN_POINT('Ctrl Pts',(-11.8145093358306,-32.1367321027922,
27.4439608775482));
#35510=CARTESIAN_POINT('Ctrl Pts',(-11.760078219655,-32.1026528827749,27.4400785412877));
#35511=CARTESIAN_POINT('Ctrl Pts',(-11.7208392858743,-32.0791769342427,
27.4372707474602));
#35512=CARTESIAN_POINT('Ctrl Pts',(-11.4992150140852,-31.9525991408178,
27.4214120803381));
#35513=CARTESIAN_POINT('Ctrl Pts',(-11.3080580221233,-31.8657895011142,
27.4077648192133));
#35514=CARTESIAN_POINT('Ctrl Pts',(-11.0645877792841,-31.7814008929861,
27.3912148823381));
#35515=CARTESIAN_POINT('Ctrl Pts',(-11.0187229994492,-31.7665914313692,
27.3881300362067));
#35516=CARTESIAN_POINT('Ctrl Pts',(-10.8748300020872,-31.7234950250931,
27.3785675276167));
#35517=CARTESIAN_POINT('Ctrl Pts',(-10.775825532725,-31.6986503006313,27.3721552421899));
#35518=CARTESIAN_POINT('Ctrl Pts',(-10.6049390277344,-31.6638810653378,
27.3614066409619));
#35519=CARTESIAN_POINT('Ctrl Pts',(-10.53358621181,-31.6517276526281,27.357011058869));
#35520=CARTESIAN_POINT('Ctrl Pts',(-10.4284457954929,-31.637266102549,27.3506670227089));
#35521=CARTESIAN_POINT('Ctrl Pts',(-10.3949290634287,-31.6331652515554,
27.3486642052471));
#35522=CARTESIAN_POINT('Ctrl Pts',(-10.335000502167,-31.6267401067101,27.3451167207868));
#35523=CARTESIAN_POINT('Ctrl Pts',(-10.3086125162228,-31.6242236421584,
27.3435662482546));
#35524=CARTESIAN_POINT('Ctrl Pts',(-10.2523493454763,-31.6195234093727,
27.3402839930804));
#35525=CARTESIAN_POINT('Ctrl Pts',(-10.2224691350522,-31.6174255752575,
27.3385549827382));
#35526=CARTESIAN_POINT('Ctrl Pts',(-10.1418306684677,-31.6128372696264,
27.3339244854419));
#35527=CARTESIAN_POINT('Ctrl Pts',(-10.0910368006633,-31.6110916244331,
27.3310458419315));
#35528=CARTESIAN_POINT('Ctrl Pts',(-9.79136223960751,-31.6075355972096,
27.314252463339));
#35529=CARTESIAN_POINT('Ctrl Pts',(-9.54293614804405,-31.6319964111137,
27.3011750101278));
#35530=CARTESIAN_POINT('Ctrl Pts',(-9.18283369375264,-31.7080642270481,
27.2816303785854));
#35531=CARTESIAN_POINT('Ctrl Pts',(-9.06764156705829,-31.7388182408458,
27.2752714006471));
#35532=CARTESIAN_POINT('Ctrl Pts',(-8.89128037632563,-31.7960123153208,
27.2650608821389));
#35533=CARTESIAN_POINT('Ctrl Pts',(-8.82886292459748,-31.8182971395685,
27.2613506692065));
#35534=CARTESIAN_POINT('Ctrl Pts',(-8.74593117112914,-31.8506770630332,
27.2562407327734));
#35535=CARTESIAN_POINT('Ctrl Pts',(-8.72480407748053,-31.8591722607726,
27.2549229228342));
#35536=CARTESIAN_POINT('Ctrl Pts',(-8.68956939028939,-31.8737542159128,
27.2526956450542));
#35537=CARTESIAN_POINT('Ctrl Pts',(-8.67541426678867,-31.8797253784759,
27.2517927951618));
#35538=CARTESIAN_POINT('Ctrl Pts',(-8.64612532627924,-31.8923157719466,
27.2499070103446));
#35539=CARTESIAN_POINT('Ctrl Pts',(-8.63099862683602,-31.8989496765556,
27.2489233019772));
#35540=CARTESIAN_POINT('Ctrl Pts',(-8.59010240544302,-31.9172424959816,
27.2462383929969));
#35541=CARTESIAN_POINT('Ctrl Pts',(-8.56442990275235,-31.9291135745576,
27.2445254276006));
#35542=CARTESIAN_POINT('Ctrl Pts',(-8.40824763206342,-32.0037193468699,
27.2339482870017));
#35543=CARTESIAN_POINT('Ctrl Pts',(-8.28173042756514,-32.074437597072,27.2247136372165));
#35544=CARTESIAN_POINT('Ctrl Pts',(-7.94955891696659,-32.2891039192817,
27.1992754665067));
#35545=CARTESIAN_POINT('Ctrl Pts',(-7.75469953489457,-32.4481527733674,
27.1830534737424));
#35546=CARTESIAN_POINT('Ctrl Pts',(-7.53140141296439,-32.6759775391306,
27.1634391483731));
#35547=CARTESIAN_POINT('Ctrl Pts',(-7.48512666091504,-32.7261327066511,
27.159302369321));
#35548=CARTESIAN_POINT('Ctrl Pts',(-7.41873337237048,-32.80260169821,27.1532546321753));
#35549=CARTESIAN_POINT('Ctrl Pts',(-7.39743750208104,-32.8278661965755,
27.1512963341591));
#35550=CARTESIAN_POINT('Ctrl Pts',(-7.35976781351184,-32.8739053695781,
27.1477973489305));
#35551=CARTESIAN_POINT('Ctrl Pts',(-7.3432615293839,-32.8945677086267,27.1462514646324));
#35552=CARTESIAN_POINT('Ctrl Pts',(-7.3082845860345,-32.9394177481084,27.1429470015176));
#35553=CARTESIAN_POINT('Ctrl Pts',(-7.28989435650107,-32.9636654070215,
27.1411916331636));
#35554=CARTESIAN_POINT('Ctrl Pts',(-7.2403468065514,-33.0308545829959,27.1364095396556));
#35555=CARTESIAN_POINT('Ctrl Pts',(-7.20986648157781,-33.0742858996902,
27.1334083719637));
#35556=CARTESIAN_POINT('Ctrl Pts',(-7.07285580709606,-33.2795985920008,
27.119601327904));
#35557=CARTESIAN_POINT('Ctrl Pts',(-6.97930978398156,-33.4497115805019,
27.1092606810493));
#35558=CARTESIAN_POINT('Ctrl Pts',(-6.83741220874823,-33.7699854450732,
27.0906803702884));
#35559=CARTESIAN_POINT('Ctrl Pts',(-6.78400664131824,-33.9172817198232,
27.0824332969634));
#35560=CARTESIAN_POINT('Ctrl Pts',(-6.71971189664959,-34.1420435312312,
27.0696441038781));
#35561=CARTESIAN_POINT('Ctrl Pts',(-6.70100364014649,-34.217056430038,27.0653414095174));
#35562=CARTESIAN_POINT('Ctrl Pts',(-6.67987290411002,-34.3160876629172,
27.0595403772934));
#35563=CARTESIAN_POINT('Ctrl Pts',(-6.67511831688643,-34.3395897176305,
27.05815486262));
#35564=CARTESIAN_POINT('Ctrl Pts',(-6.66768308675801,-34.3784596970306,
27.0558459286593));
#35565=CARTESIAN_POINT('Ctrl Pts',(-6.66485839126151,-34.3937997068489,
27.0549302444276));
#35566=CARTESIAN_POINT('Ctrl Pts',(-6.6596715321306,-34.4231019996741,27.0531716989397));
#35567=CARTESIAN_POINT('Ctrl Pts',(-6.65729080581259,-34.43706056888,27.0523299681995));
#35568=CARTESIAN_POINT('Ctrl Pts',(-6.65102308935945,-34.4752514621302,
27.0500167595333));
#35569=CARTESIAN_POINT('Ctrl Pts',(-6.64731177780774,-34.4995112543806,
27.0485361352145));
#35570=CARTESIAN_POINT('Ctrl Pts',(-6.63319544764557,-34.5990012943337,
27.0424240480923));
#35571=CARTESIAN_POINT('Ctrl Pts',(-6.6250573262537,-34.6745262833766,27.0376911637111));
#35572=CARTESIAN_POINT('Ctrl Pts',(-6.60425265632037,-34.9561373062805,
27.0198457310312));
#35573=CARTESIAN_POINT('Ctrl Pts',(-6.60788209419339,-35.162976625266,27.0063766598641));
#35574=CARTESIAN_POINT('Ctrl Pts',(-6.648045311981,-35.5305406980391,26.9827752344443));
#35575=CARTESIAN_POINT('Ctrl Pts',(-6.67749351563748,-35.6914017720423,
26.97255754757));
#35576=CARTESIAN_POINT('Ctrl Pts',(-6.72932968277317,-35.8916345909871,
26.9600664028032));
#35577=CARTESIAN_POINT('Ctrl Pts',(-6.74103904799746,-35.9335257601553,
26.9574649922675));
#35578=CARTESIAN_POINT('Ctrl Pts',(-6.76165543098856,-36.0021591580661,
26.9532208738375));
#35579=CARTESIAN_POINT('Ctrl Pts',(-6.77009522292039,-36.0290353386993,
26.9515634968187));
#35580=CARTESIAN_POINT('Ctrl Pts',(-6.78721870717594,-36.0812770345316,
26.9483498890499));
#35581=CARTESIAN_POINT('Ctrl Pts',(-6.7958702169174,-36.1066508277452,26.9467927597209));
#35582=CARTESIAN_POINT('Ctrl Pts',(-6.81743683136609,-36.1675289639846,
26.9430644194347));
#35583=CARTESIAN_POINT('Ctrl Pts',(-6.83064639531074,-36.2029256395468,
26.9409029499154));
#35584=CARTESIAN_POINT('Ctrl Pts',(-6.87815348722067,-36.3240077944213,
26.9335238726485));
#35585=CARTESIAN_POINT('Ctrl Pts',(-6.9153577825169,-36.40851220673,26.9284008903459));
#35586=CARTESIAN_POINT('Ctrl Pts',(-7.07325039934854,-36.7307805053421,
26.9088002061576));
#35587=CARTESIAN_POINT('Ctrl Pts',(-7.21835204256103,-36.9554768439312,
26.8950696547273));
#35588=CARTESIAN_POINT('Ctrl Pts',(-7.43027226994807,-37.2116161311006,
26.8770631742104));
#35589=CARTESIAN_POINT('Ctrl Pts',(-7.47374395077426,-37.261144848647,26.8734503832279));
#35590=CARTESIAN_POINT('Ctrl Pts',(-7.54916387998048,-37.3421819318584,
26.8672545310238));
#35591=CARTESIAN_POINT('Ctrl Pts',(-7.58034507818804,-37.3743806670719,
26.8647121229581));
#35592=CARTESIAN_POINT('Ctrl Pts',(-7.62614415678353,-37.4198351223223,
26.8609883304553));
#35593=CARTESIAN_POINT('Ctrl Pts',(-7.6402549104934,-37.4335974719789,26.8598424066997));
#35594=CARTESIAN_POINT('Ctrl Pts',(-7.66526830996823,-37.4575711815212,
26.8578117657721));
#35595=CARTESIAN_POINT('Ctrl Pts',(-7.67611966867757,-37.4678347533675,
26.8569309760888));
#35596=CARTESIAN_POINT('Ctrl Pts',(-7.7002696094403,-37.49037602687,26.8549707278462));
#35597=CARTESIAN_POINT('Ctrl Pts',(-7.71359874458483,-37.5026190064143,
26.8538889432502));
#35598=CARTESIAN_POINT('Ctrl Pts',(-7.75370929357483,-37.5388731547109,
26.8506357390741));
#35599=CARTESIAN_POINT('Ctrl Pts',(-7.7807747187098,-37.562564684434,26.8484433988428));
#35600=CARTESIAN_POINT('Ctrl Pts',(-7.92315109332242,-37.6832455514444,
26.8369480518014));
#35601=CARTESIAN_POINT('Ctrl Pts',(-8.04445070891223,-37.7728916180789,
26.8272864418007));
#35602=CARTESIAN_POINT('Ctrl Pts',(-8.28213386071937,-37.9251783213993,
26.8091010239399));
#35603=CARTESIAN_POINT('Ctrl Pts',(-8.39701516869686,-37.989677964705,26.8006018354876));
#35604=CARTESIAN_POINT('Ctrl Pts',(-8.64606803263779,-38.1110148204502,
26.7830002692553));
#35605=CARTESIAN_POINT('Ctrl Pts',(-8.78075004027341,-38.166225396847,26.7739477666337));
#35606=CARTESIAN_POINT('Ctrl Pts',(-8.9586966417522,-38.2261252883098,26.762620658718));
#35607=CARTESIAN_POINT('Ctrl Pts',(-8.99906733322436,-38.2388780618731,
26.7600907149053));
#35608=CARTESIAN_POINT('Ctrl Pts',(-9.06645817759303,-38.2587858305177,
26.7559315267622));
#35609=CARTESIAN_POINT('Ctrl Pts',(-9.09334600186111,-38.26636862904,26.7542887683861));
#35610=CARTESIAN_POINT('Ctrl Pts',(-9.14635811110742,-38.2806138514496,
26.7510815992656));
#35611=CARTESIAN_POINT('Ctrl Pts',(-9.17247416380091,-38.2872987038947,
26.7495165777871));
#35612=CARTESIAN_POINT('Ctrl Pts',(-9.23028737403051,-38.3013643417998,
26.7460837100557));
#35613=CARTESIAN_POINT('Ctrl Pts',(-9.26201687841528,-38.3086016774235,
26.7442204828709));
#35614=CARTESIAN_POINT('Ctrl Pts',(-9.37273114119309,-38.3321830583544,
26.73778670631));
#35615=CARTESIAN_POINT('Ctrl Pts',(-9.45219391236756,-38.3461649698683,
26.7332887801457));
#35616=CARTESIAN_POINT('Ctrl Pts',(-9.8099106929276,-38.3960209019083,26.7134482685919));
#35617=CARTESIAN_POINT('Ctrl Pts',(-10.0914482915887,-38.4001058095978,
26.6990266168772));
#35618=CARTESIAN_POINT('Ctrl Pts',(-10.4368141211214,-38.3621541916367,
26.6802203311006));
#35619=CARTESIAN_POINT('Ctrl Pts',(-10.5031291686947,-38.3528715342877,
26.676551959183));
#35620=CARTESIAN_POINT('Ctrl Pts',(-10.6138086552864,-38.3340214136477,
26.6702710420488));
#35621=CARTESIAN_POINT('Ctrl Pts',(-10.6583356234607,-38.3255155465053,
26.6677006183227));
#35622=CARTESIAN_POINT('Ctrl Pts',(-10.7220432405637,-38.3120160835871,
26.6639430866258));
#35623=CARTESIAN_POINT('Ctrl Pts',(-10.7413732819027,-38.3077428248048,
26.6627923329609));
#35624=CARTESIAN_POINT('Ctrl Pts',(-10.7752264897846,-38.2999473109075,
26.6607565162829));
#35625=CARTESIAN_POINT('Ctrl Pts',(-10.7897655231144,-38.2964979556856,
26.6598754567988));
#35626=CARTESIAN_POINT('Ctrl Pts',(-10.8218010594089,-38.2886734890689,
26.6579188632706));
#35627=CARTESIAN_POINT('Ctrl Pts',(-10.8392855297969,-38.2842548723115,
26.6568410635853));
#35628=CARTESIAN_POINT('Ctrl Pts',(-10.8912166359325,-38.2706892545022,
26.6536119766901));
#35629=CARTESIAN_POINT('Ctrl Pts',(-10.925554147983,-38.2611385425921,26.6514402050523));
#35630=CARTESIAN_POINT('Ctrl Pts',(-11.0983744421087,-38.210120736119,26.6403453218782));
#35631=CARTESIAN_POINT('Ctrl Pts',(-11.2342451086578,-38.1603692727695,
26.631091344763));
#35632=CARTESIAN_POINT('Ctrl Pts',(-11.4798383103547,-38.0521825339116,
26.6138102530762));
#35633=CARTESIAN_POINT('Ctrl Pts',(-11.5903456795482,-37.996087760883,26.6058090486547));
#35634=CARTESIAN_POINT('Ctrl Pts',(-11.7889218549526,-37.8811994277568,
26.591183772273));
#35635=CARTESIAN_POINT('Ctrl Pts',(-11.8777917220539,-37.8240844093866,
26.5845375592733));
#35636=CARTESIAN_POINT('Ctrl Pts',(-12.0242457051605,-37.7199859788669,
26.5734516970385));
#35637=CARTESIAN_POINT('Ctrl Pts',(-12.0832145070974,-37.6750912108364,
26.5689475692721));
#35638=CARTESIAN_POINT('Ctrl Pts',(-12.1670755527956,-37.6067889374803,
26.5624799775202));
#35639=CARTESIAN_POINT('Ctrl Pts',(-12.1931580784501,-37.5848835149813,
26.5604590738322));
#35640=CARTESIAN_POINT('Ctrl Pts',(-12.2389677001923,-37.5452176475842,
26.5568916156273));
#35641=CARTESIAN_POINT('Ctrl Pts',(-12.2588243685801,-37.5276118704048,
26.5553390080314));
#35642=CARTESIAN_POINT('Ctrl Pts',(-12.3005196453697,-37.4897592448251,
26.5520643880616));
#35643=CARTESIAN_POINT('Ctrl Pts',(-12.3223024083116,-37.4694540574639,
26.5503449841888));
#35644=CARTESIAN_POINT('Ctrl Pts',(-12.3808847611805,-37.4133847064915,
26.5456945828851));
#35645=CARTESIAN_POINT('Ctrl Pts',(-12.4171451048612,-37.3770670831036,
26.5427872703335));
#35646=CARTESIAN_POINT('Ctrl Pts',(-12.6250171846187,-37.1591893865509,
26.5259119482922));
#35647=CARTESIAN_POINT('Ctrl Pts',(-12.7769569875033,-36.959932397515,26.5127882387389));
#35648=CARTESIAN_POINT('Ctrl Pts',(-12.9667199856531,-36.6440950197546,
26.4932202044339));
#35649=CARTESIAN_POINT('Ctrl Pts',(-13.022428787916,-36.5392845628019,26.4868881874643));
#35650=CARTESIAN_POINT('Ctrl Pts',(-13.1004416261757,-36.3718726463021,
26.4767154394661));
#35651=CARTESIAN_POINT('Ctrl Pts',(-13.1265969675572,-36.3111686007616,
26.4730147892819));
#35652=CARTESIAN_POINT('Ctrl Pts',(-13.159347275358,-36.2285957104624,26.4679160605329));
#35653=CARTESIAN_POINT('Ctrl Pts',(-13.1675214715775,-36.2073650205264,
26.4665994374467));
#35654=CARTESIAN_POINT('Ctrl Pts',(-13.1808551926849,-36.1716659973395,
26.4643735760864));
#35655=CARTESIAN_POINT('Ctrl Pts',(-13.186131352381,-36.1572415325053,26.4634709364931));
#35656=CARTESIAN_POINT('Ctrl Pts',(-13.1968803503905,-36.1272240969356,
26.4615849070096));
#35657=CARTESIAN_POINT('Ctrl Pts',(-13.2023374466621,-36.1116262824911,
26.4606007355055));
#35658=CARTESIAN_POINT('Ctrl Pts',(-13.2168363248903,-36.0691917869529,
26.4579132437476));
#35659=CARTESIAN_POINT('Ctrl Pts',(-13.2256560046555,-36.042281269149,26.456198122282));
#35660=CARTESIAN_POINT('Ctrl Pts',(-13.2797922504546,-35.8698295941028,
26.4451522720509));
#35661=CARTESIAN_POINT('Ctrl Pts',(-13.3155812996538,-35.7214935176125,
26.4354108845216));
#35662=CARTESIAN_POINT('Ctrl Pts',(-13.3733890042827,-35.3833848395515,
26.4133313788544));
#35663=CARTESIAN_POINT('Ctrl Pts',(-13.3896100394668,-35.1931105210115,
26.4010055067278));
#35664=CARTESIAN_POINT('Ctrl Pts',(-13.3898250629205,-34.8983315803273,
26.3825329145607));
#35665=CARTESIAN_POINT('Ctrl Pts',(-13.3851018685923,-34.7942352126983,
26.3761238809521));
#35666=CARTESIAN_POINT('Ctrl Pts',(-13.3719934748467,-34.6512612540976,
26.3674867017218));
#35667=CARTESIAN_POINT('Ctrl Pts',(-13.3677102680831,-34.6120741640032,
26.365136301304));
#35668=CARTESIAN_POINT('Ctrl Pts',(-13.3596408897165,-34.5485301049426,
26.3613510938373));
#35669=CARTESIAN_POINT('Ctrl Pts',(-13.3562709821072,-34.5241248940409,
26.3599035917135));
#35670=CARTESIAN_POINT('Ctrl Pts',(-13.3486063365844,-34.4727562249109,
26.3568693632134));
#35671=CARTESIAN_POINT('Ctrl Pts',(-13.3442512838865,-34.445803455646,26.3552846252909));
#35672=CARTESIAN_POINT('Ctrl Pts',(-13.3328777702249,-34.3804394466201,
26.3514576980142));
#35673=CARTESIAN_POINT('Ctrl Pts',(-13.3255202663303,-34.3420907003197,
26.3492262057105));
#35674=CARTESIAN_POINT('Ctrl Pts',(-13.2949464803174,-34.1963858352286,
26.3407913880578));
#35675=CARTESIAN_POINT('Ctrl Pts',(-13.2671793421232,-34.0900492891848,
26.3347292253266));
#35676=CARTESIAN_POINT('Ctrl Pts',(-13.2171487806147,-33.9305891135584,
26.325664421708));
#35677=CARTESIAN_POINT('Ctrl Pts',(-13.1986265369331,-33.8764036723632,
26.3225882159661));
#35678=CARTESIAN_POINT('Ctrl Pts',(-13.1787501930238,-33.8227352579598,
26.3195306104224));
#35679=CARTESIAN_POINT('',(-13.3897497681227,-34.9987462009367,26.7339821967504));
#35680=CARTESIAN_POINT('Ctrl Pts',(-13.1787501100144,-33.8227350338248,
26.6607619345813));
#35681=CARTESIAN_POINT('Ctrl Pts',(-13.2216841843832,-33.9386619470895,
26.6684502125966));
#35682=CARTESIAN_POINT('Ctrl Pts',(-13.258249581665,-34.0568647109076,26.6763673997128));
#35683=CARTESIAN_POINT('Ctrl Pts',(-13.3167604124846,-34.2905904905764,
26.6918795664257));
#35684=CARTESIAN_POINT('Ctrl Pts',(-13.3393195908669,-34.4057716545837,
26.6994587083872));
#35685=CARTESIAN_POINT('Ctrl Pts',(-13.3783572706517,-34.6797789408598,
26.7171358122187));
#35686=CARTESIAN_POINT('Ctrl Pts',(-13.3896826954089,-34.8390678269662,
26.7271303610769));
#35687=CARTESIAN_POINT('Ctrl Pts',(-13.3897497009165,-34.9985760489549,
26.7367914542175));
#35688=CARTESIAN_POINT('Ctrl Pts',(-13.3897497681227,-34.9987462009367,
26.7339821967504));
#35689=CARTESIAN_POINT('Ctrl Pts',(-13.3897890807776,-35.1050312244497,
26.7401898647502));
#35690=CARTESIAN_POINT('Ctrl Pts',(-13.384825222301,-35.2112871201384,26.7463975327499));
#35691=CARTESIAN_POINT('Ctrl Pts',(-13.3748927040034,-35.3170241299407,
26.7526052007497));
#35692=CARTESIAN_POINT('Ctrl Pts',(-13.3649548482649,-35.4228179596774,
26.7588162045662));
#35693=CARTESIAN_POINT('Ctrl Pts',(-13.3500430540965,-35.5280919481609,
26.7650272083827));
#35694=CARTESIAN_POINT('Ctrl Pts',(-13.3302435188097,-35.6323631614237,
26.7712382121992));
#35695=CARTESIAN_POINT('Ctrl Pts',(-13.3101893565053,-35.7379753287885,
26.7775290910914));
#35696=CARTESIAN_POINT('Ctrl Pts',(-13.2851209398701,-35.8425583312712,
26.7838199699835));
#35697=CARTESIAN_POINT('Ctrl Pts',(-13.2551803933349,-35.9456244864363,
26.7901108488757));
#35698=CARTESIAN_POINT('Ctrl Pts',(-13.2255498660117,-36.0476234437076,
26.7963365888995));
#35699=CARTESIAN_POINT('Ctrl Pts',(-13.1911478356904,-36.1481364617781,
26.8025623289234));
#35700=CARTESIAN_POINT('Ctrl Pts',(-13.1521609226748,-36.2467103031827,
26.8087880689473));
#35701=CARTESIAN_POINT('Ctrl Pts',(-13.1125621394122,-36.3468311868132,
26.8151115172736));
#35702=CARTESIAN_POINT('Ctrl Pts',(-13.0682335273692,-36.4449511173892,
26.8214349655998));
#35703=CARTESIAN_POINT('Ctrl Pts',(-13.0194189846595,-36.5406213219276,
26.8277584139261));
#35704=CARTESIAN_POINT('Ctrl Pts',(-12.9706044419497,-36.6362915264661,
26.8340818622524));
#35705=CARTESIAN_POINT('Ctrl Pts',(-12.9173042373172,-36.7295116662979,
26.8404053105786));
#35706=CARTESIAN_POINT('Ctrl Pts',(-12.8598073032938,-36.819864624231,26.8467287589049));
#35707=CARTESIAN_POINT('Ctrl Pts',(-12.8043271157924,-36.9070483868538,
26.8528304077103));
#35708=CARTESIAN_POINT('Ctrl Pts',(-12.7447627250912,-36.9918401274393,
26.8589320565157));
#35709=CARTESIAN_POINT('Ctrl Pts',(-12.6813468174827,-37.0738332398906,
26.8650337053211));
#35710=CARTESIAN_POINT('Ctrl Pts',(-12.6180143251107,-37.1557185012503,
26.8711273282147));
#35711=CARTESIAN_POINT('Ctrl Pts',(-12.5508406470472,-37.2348121173873,
26.8772209511084));
#35712=CARTESIAN_POINT('Ctrl Pts',(-12.4801026278758,-37.3107349518505,
26.883314574002));
#35713=CARTESIAN_POINT('Ctrl Pts',(-12.4094374149536,-37.3865796436562,
26.8894019251081));
#35714=CARTESIAN_POINT('Ctrl Pts',(-12.3352154459125,-37.4592597319462,
26.8954892762142));
#35715=CARTESIAN_POINT('Ctrl Pts',(-12.257754298081,-37.5284284826739,26.9015766273203));
#35716=CARTESIAN_POINT('Ctrl Pts',(-12.1803482539649,-37.5975480286678,
26.9076596480534));
#35717=CARTESIAN_POINT('Ctrl Pts',(-12.0997079314097,-37.6631609202428,
26.9137426687865));
#35718=CARTESIAN_POINT('Ctrl Pts',(-12.0161876933331,-37.7249572928309,
26.9198256895197));
#35719=CARTESIAN_POINT('Ctrl Pts',(-11.9326983778213,-37.7867307859064,
26.9259064580729));
#35720=CARTESIAN_POINT('Ctrl Pts',(-11.8463316094067,-37.8446903141597,
26.931987226626));
#35721=CARTESIAN_POINT('Ctrl Pts',(-11.7574741265705,-37.8985668453453,
26.9380679951792));
#35722=CARTESIAN_POINT('Ctrl Pts',(-11.6686265213079,-37.9524373875091,
26.9441480877822));
#35723=CARTESIAN_POINT('Ctrl Pts',(-11.5772891179516,-38.0022256133608,
26.9502281803851));
#35724=CARTESIAN_POINT('Ctrl Pts',(-11.4838760925702,-38.0477068107675,
26.956308272988));
#35725=CARTESIAN_POINT('Ctrl Pts',(-11.390449250198,-38.0931947354296,26.9623892649151));
#35726=CARTESIAN_POINT('Ctrl Pts',(-11.2949465604751,-38.1343741786936,
26.9684702568421));
#35727=CARTESIAN_POINT('Ctrl Pts',(-11.1978043188133,-38.1710676240554,
26.9745512487691));
#35728=CARTESIAN_POINT('Ctrl Pts',(-11.100561247805,-38.207799155589,26.9806385524965));
#35729=CARTESIAN_POINT('Ctrl Pts',(-11.0016756271896,-38.2400352388196,
26.986725856224));
#35730=CARTESIAN_POINT('Ctrl Pts',(-10.9016011110949,-38.2676475481564,
26.9928131599514));
#35731=CARTESIAN_POINT('Ctrl Pts',(-10.8014728281809,-38.295274692699,26.9989037341914));
#35732=CARTESIAN_POINT('Ctrl Pts',(-10.700154794652,-38.3182730203065,27.0049943084314));
#35733=CARTESIAN_POINT('Ctrl Pts',(-10.5981111607529,-38.3365653150932,
27.0110848826714));
#35734=CARTESIAN_POINT('Ctrl Pts',(-10.4959009340921,-38.3548874732216,
27.0171854001635));
#35735=CARTESIAN_POINT('Ctrl Pts',(-10.3929631649858,-38.3684881943241,
27.0232859176557));
#35736=CARTESIAN_POINT('Ctrl Pts',(-10.2897676712297,-38.3773421146236,
27.0293864351478));
#35737=CARTESIAN_POINT('Ctrl Pts',(-10.2084487595871,-38.3843190778254,
27.034193693923));
#35738=CARTESIAN_POINT('Ctrl Pts',(-10.1269699497257,-38.3883495208024,
27.0390009526982));
#35739=CARTESIAN_POINT('Ctrl Pts',(-10.045559979307,-38.3894438114218,27.0438082114734));
#35740=CARTESIAN_POINT('Ctrl Pts',(-9.94222969266637,-38.3908327489535,
27.0499098649274));
#35741=CARTESIAN_POINT('Ctrl Pts',(-9.8386612147156,-38.3874945496007,27.0560115183814));
#35742=CARTESIAN_POINT('Ctrl Pts',(-9.73532216989635,-38.3794009393311,
27.0621131718354));
#35743=CARTESIAN_POINT('Ctrl Pts',(-9.63211905313828,-38.3713179750738,
27.0682067994176));
#35744=CARTESIAN_POINT('Ctrl Pts',(-9.52914519239832,-38.3584920683563,
27.0743004269998));
#35745=CARTESIAN_POINT('Ctrl Pts',(-9.42686944319496,-38.3409469357289,
27.0803940545821));
#35746=CARTESIAN_POINT('Ctrl Pts',(-9.32469895942654,-38.3234198611067,
27.0864814104101));
#35747=CARTESIAN_POINT('Ctrl Pts',(-9.22322557777763,-38.3011832910373,
27.0925687662381));
#35748=CARTESIAN_POINT('Ctrl Pts',(-9.12291338147732,-38.2743127715764,
27.0986561220662));
#35749=CARTESIAN_POINT('Ctrl Pts',(-9.0226725439398,-38.2474613669101,27.1047391475516));
#35750=CARTESIAN_POINT('Ctrl Pts',(-8.92359166110563,-38.2159826784515,
27.110822173037));
#35751=CARTESIAN_POINT('Ctrl Pts',(-8.82612414410728,-38.1800032291575,
27.1169051985224));
#35752=CARTESIAN_POINT('Ctrl Pts',(-8.72869271321997,-38.1440371007979,
27.1229859718448));
#35753=CARTESIAN_POINT('Ctrl Pts',(-8.63287386186256,-38.1035736713432,
27.1290667451673));
#35754=CARTESIAN_POINT('Ctrl Pts',(-8.53910459725674,-38.0587889245163,
27.1351475184897));
#35755=CARTESIAN_POINT('Ctrl Pts',(-8.44534575604772,-38.0140091559645,
27.141227615873));
#35756=CARTESIAN_POINT('Ctrl Pts',(-8.35363643452957,-37.9649092095808,
27.1473077132563));
#35757=CARTESIAN_POINT('Ctrl Pts',(-8.26439161211884,-37.9117123117534,
27.1533878106396));
#35758=CARTESIAN_POINT('Ctrl Pts',(-8.17513358917933,-37.8585075453779,
27.1594688073524));
#35759=CARTESIAN_POINT('Ctrl Pts',(-8.08834115704462,-37.8012048426389,
27.1655498040653));
#35760=CARTESIAN_POINT('Ctrl Pts',(-8.0044019470703,-37.7400718008189,27.1716308007781));
#35761=CARTESIAN_POINT('Ctrl Pts',(-7.92037561227555,-37.6788753058727,
27.1777181092699));
#35762=CARTESIAN_POINT('Ctrl Pts',(-7.83920876045743,-37.6138407843401,
27.1838054177618));
#35763=CARTESIAN_POINT('Ctrl Pts',(-7.76125739651567,-37.5452773164911,
27.1898927262536));
#35764=CARTESIAN_POINT('Ctrl Pts',(-7.68326415190567,-37.4766770117773,
27.1959833052533));
#35765=CARTESIAN_POINT('Ctrl Pts',(-7.60849014427039,-37.4045442811282,
27.202073884253));
#35766=CARTESIAN_POINT('Ctrl Pts',(-7.53725438541685,-37.3292249999413,
27.2081644632527));
#35767=CARTESIAN_POINT('Ctrl Pts',(-7.46590233038794,-37.2537827560111,
27.2142649854474));
#35768=CARTESIAN_POINT('Ctrl Pts',(-7.39810034314356,-37.1751438932789,
27.2203655076422));
#35769=CARTESIAN_POINT('Ctrl Pts',(-7.33412717462984,-37.0936874507559,
27.2264660298369));
#35770=CARTESIAN_POINT('Ctrl Pts',(-7.28371631876174,-37.0294997752202,
27.2312732412386));
#35771=CARTESIAN_POINT('Ctrl Pts',(-7.23568215067551,-36.9635632256665,
27.2360804526402));
#35772=CARTESIAN_POINT('Ctrl Pts',(-7.19014138122318,-36.8960747888693,
27.2408876640418));
#35773=CARTESIAN_POINT('Ctrl Pts',(-7.13233799060928,-36.8104139508768,
27.2469892982864));
#35774=CARTESIAN_POINT('Ctrl Pts',(-7.0783576454435,-36.7219626636669,27.2530909325309));
#35775=CARTESIAN_POINT('Ctrl Pts',(-7.02848032780385,-36.6310965330879,
27.2591925667755));
#35776=CARTESIAN_POINT('Ctrl Pts',(-6.97866861725399,-36.5403499250227,
27.265286175118));
#35777=CARTESIAN_POINT('Ctrl Pts',(-6.93294940888755,-36.4471951602325,
27.2713797834605));
#35778=CARTESIAN_POINT('Ctrl Pts',(-6.89155987630513,-36.3520373737082,
27.2774733918029));
#35779=CARTESIAN_POINT('Ctrl Pts',(-6.85021294330727,-36.256977526975,27.2835607283862));
#35780=CARTESIAN_POINT('Ctrl Pts',(-6.81318699451426,-36.1599191481521,
27.2896480649694));
#35781=CARTESIAN_POINT('Ctrl Pts',(-6.78067323890418,-36.0612917920121,
27.2957354015527));
#35782=CARTESIAN_POINT('Ctrl Pts',(-6.7481826121946,-35.9627345951713,27.301818407864));
#35783=CARTESIAN_POINT('Ctrl Pts',(-6.72019792928452,-35.8626110455444,
27.3079014141754));
#35784=CARTESIAN_POINT('Ctrl Pts',(-6.69686191353556,-35.7613697158727,
27.3139844204867));
#35785=CARTESIAN_POINT('Ctrl Pts',(-6.6735345374864,-35.6601658688075,27.3200651746849));
#35786=CARTESIAN_POINT('Ctrl Pts',(-6.65485250403436,-35.5578454805441,
27.326145928883));
#35787=CARTESIAN_POINT('Ctrl Pts',(-6.64090817697617,-35.4548705167346,
27.3322266830812));
#35788=CARTESIAN_POINT('Ctrl Pts',(-6.62696539980954,-35.3519069984418,
27.3383067614124));
#35789=CARTESIAN_POINT('Ctrl Pts',(-6.61775933931373,-35.248289473158,27.3443868397437));
#35790=CARTESIAN_POINT('Ctrl Pts',(-6.61333077204748,-35.1444873798624,
27.3504669180749));
#35791=CARTESIAN_POINT('Ctrl Pts',(-6.60890154966468,-35.0406699311559,
27.3565478958302));
#35792=CARTESIAN_POINT('Ctrl Pts',(-6.60925124284346,-34.9366682876005,
27.3626288735855));
#35793=CARTESIAN_POINT('Ctrl Pts',(-6.61436852639487,-34.832953337554,27.3687098513408));
#35794=CARTESIAN_POINT('Ctrl Pts',(-6.6194911216758,-34.7291307316084,27.3747971411382));
#35795=CARTESIAN_POINT('Ctrl Pts',(-6.62939116927492,-34.6255958415428,
27.3808844309356));
#35796=CARTESIAN_POINT('Ctrl Pts',(-6.64400531235691,-34.522815843713,27.386971720733));
#35797=CARTESIAN_POINT('Ctrl Pts',(-6.65862730743689,-34.4199806234639,
27.3930622811557));
#35798=CARTESIAN_POINT('Ctrl Pts',(-6.6779683635389,-34.3179015237124,27.3991528415785));
#35799=CARTESIAN_POINT('Ctrl Pts',(-6.70191407119283,-34.2170349505219,
27.4052434020012));
#35800=CARTESIAN_POINT('Ctrl Pts',(-6.72589887312402,-34.116003700395,27.4113439060039));
#35801=CARTESIAN_POINT('Ctrl Pts',(-6.75450322669983,-34.0161893429761,
27.4174444100066));
#35802=CARTESIAN_POINT('Ctrl Pts',(-6.78756291584155,-33.9180327903196,
27.4235449140092));
#35803=CARTESIAN_POINT('Ctrl Pts',(-6.81361505484069,-33.8406821491045,
27.4283523148762));
#35804=CARTESIAN_POINT('Ctrl Pts',(-6.84243293384911,-33.7643607104903,
27.4331597157432));
#35805=CARTESIAN_POINT('Ctrl Pts',(-6.87391576234909,-33.6892740936372,
27.4379671166102));
#35806=CARTESIAN_POINT('Ctrl Pts',(-6.9138744530809,-33.5939725262786,27.4440687743589));
#35807=CARTESIAN_POINT('Ctrl Pts',(-6.95826267774881,-33.500338838719,27.4501704321076));
#35808=CARTESIAN_POINT('Ctrl Pts',(-7.00691976425638,-33.4088130955476,
27.4562720898564));
#35809=CARTESIAN_POINT('Ctrl Pts',(-7.05551284823835,-33.3174077434464,
27.4623657216106));
#35810=CARTESIAN_POINT('Ctrl Pts',(-7.10836343177939,-33.2281051979174,
27.4684593533649));
#35811=CARTESIAN_POINT('Ctrl Pts',(-7.16526267946933,-33.1413259064347,
27.4745529851191));
#35812=CARTESIAN_POINT('Ctrl Pts',(-7.22210336351543,-33.0546359326799,
27.4806403449929));
#35813=CARTESIAN_POINT('Ctrl Pts',(-7.28298419211704,-32.9704644045166,
27.4867277048667));
#35814=CARTESIAN_POINT('Ctrl Pts',(-7.34765070978279,-32.8892067118772,
27.4928150647405));
#35815=CARTESIAN_POINT('Ctrl Pts',(-7.41227122369864,-32.8080068259468,
27.4988980940675));
#35816=CARTESIAN_POINT('Ctrl Pts',(-7.48067180556188,-32.7297169871251,
27.5049811233945));
#35817=CARTESIAN_POINT('Ctrl Pts',(-7.5525555158057,-32.654702458261,27.5110641527215));
#35818=CARTESIAN_POINT('Ctrl Pts',(-7.62441261054486,-32.5797157041116,
27.5171449297594));
#35819=CARTESIAN_POINT('Ctrl Pts',(-7.69974997492076,-32.5080021582398,
27.5232257067974));
#35820=CARTESIAN_POINT('Ctrl Pts',(-7.77823186265473,-32.4398923057072,
27.5293064838353));
#35821=CARTESIAN_POINT('Ctrl Pts',(-7.85670502466954,-32.3717900257172,
27.5353865848045));
#35822=CARTESIAN_POINT('Ctrl Pts',(-7.93832169178252,-32.3072909227079,
27.5414666857736));
#35823=CARTESIAN_POINT('Ctrl Pts',(-8.02271158897098,-32.2466864322947,
27.5475467867428));
#35824=CARTESIAN_POINT('Ctrl Pts',(-8.10711396672057,-32.1860729789833,
27.5536277869081));
#35825=CARTESIAN_POINT('Ctrl Pts',(-8.19429004191073,-32.129355532131,27.5597087870734));
#35826=CARTESIAN_POINT('Ctrl Pts',(-8.28383976695354,-32.0767827454994,
27.5657897872387));
#35827=CARTESIAN_POINT('Ctrl Pts',(-8.37348243687032,-32.0241553928596,
27.5718770989566));
#35828=CARTESIAN_POINT('Ctrl Pts',(-8.46550330714674,-31.9756815084767,
27.5779644106745));
#35829=CARTESIAN_POINT('Ctrl Pts',(-8.55947691288674,-31.9315641936006,
27.5840517223923));
#35830=CARTESIAN_POINT('Ctrl Pts',(-8.65350100562476,-31.8874231768482,
27.5901423044976));
#35831=CARTESIAN_POINT('Ctrl Pts',(-8.74947952832602,-31.8476435556022,
27.5962328866028));
#35832=CARTESIAN_POINT('Ctrl Pts',(-8.84696803868841,-31.8123798283525,
27.602323468708));
#35833=CARTESIAN_POINT('Ctrl Pts',(-8.94461570049785,-31.7770585325422,
27.6084239937794));
#35834=CARTESIAN_POINT('Ctrl Pts',(-9.04377786564368,-31.7462679852451,
27.6145245188508));
#35835=CARTESIAN_POINT('Ctrl Pts',(-9.14399574824647,-31.7201125349366,
27.6206250439221));
#35836=CARTESIAN_POINT('Ctrl Pts',(-9.22296680446462,-31.6995022058908,
27.6254322190076));
#35837=CARTESIAN_POINT('Ctrl Pts',(-9.30259308017987,-31.6817689645993,
27.6302393940932));
#35838=CARTESIAN_POINT('Ctrl Pts',(-9.38264738479791,-31.66694122299,27.6350465691787));
#35839=CARTESIAN_POINT('Ctrl Pts',(-9.4842592359165,-31.6481205701842,27.641148251798));
#35840=CARTESIAN_POINT('Ctrl Pts',(-9.58690422524929,-31.6339189683107,
27.6472499344173));
#35841=CARTESIAN_POINT('Ctrl Pts',(-9.69012621650684,-31.6244432606156,
27.6533516170366));
#35842=CARTESIAN_POINT('Ctrl Pts',(-9.7932124376878,-31.61498001652,27.6594452739833));
#35843=CARTESIAN_POINT('Ctrl Pts',(-9.89687372961916,-31.6102303475855,
27.6655389309299));
#35844=CARTESIAN_POINT('Ctrl Pts',(-10.0006439622708,-31.6102500611678,
27.6716325878765));
#35845=CARTESIAN_POINT('Ctrl Pts',(-10.1043073945313,-31.610269754461,27.6777199732275));
#35846=CARTESIAN_POINT('Ctrl Pts',(-10.208079119075,-31.6150490693068,27.6838073585784));
#35847=CARTESIAN_POINT('Ctrl Pts',(-10.3114889564063,-31.6245919220727,
27.6898947439293));
#35848=CARTESIAN_POINT('Ctrl Pts',(-10.4148252337353,-31.6341279865843,
27.6959777990532));
#35849=CARTESIAN_POINT('Ctrl Pts',(-10.5177997110688,-31.6484208114754,
27.702060854177));
#35850=CARTESIAN_POINT('Ctrl Pts',(-10.6199441184374,-31.6674222660957,
27.7081439093008));
#35851=CARTESIAN_POINT('Ctrl Pts',(-10.7220507093345,-31.6864166858916,
27.7142247123221));
#35852=CARTESIAN_POINT('Ctrl Pts',(-10.8233274209573,-31.7101161926559,
27.7203055153434));
#35853=CARTESIAN_POINT('Ctrl Pts',(-10.9233137983367,-31.7384211350481,
27.7263863183646));
#35854=CARTESIAN_POINT('Ctrl Pts',(-11.0232890616861,-31.7667229311919,
27.7324664454716));
#35855=CARTESIAN_POINT('Ctrl Pts',(-11.1219738644293,-31.7996290285011,
27.7385465725785));
#35856=CARTESIAN_POINT('Ctrl Pts',(-11.2189214842533,-31.8369894913665,
27.7446266996854));
#35857=CARTESIAN_POINT('Ctrl Pts',(-11.3158834437109,-31.8743554802609,
27.7507077261109));
#35858=CARTESIAN_POINT('Ctrl Pts',(-11.4111073105846,-31.9161769898498,
27.7567887525364));
#35859=CARTESIAN_POINT('Ctrl Pts',(-11.5041658239971,-31.9622557322218,
27.7628697789619));
#35860=CARTESIAN_POINT('Ctrl Pts',(-11.597320924078,-32.0083823003332,27.7689571169656));
#35861=CARTESIAN_POINT('Ctrl Pts',(-11.6883057982808,-32.0587747354434,
27.7750444549693));
#35862=CARTESIAN_POINT('Ctrl Pts',(-11.7767173518078,-32.1131885211734,
27.781131792973));
#35863=CARTESIAN_POINT('Ctrl Pts',(-11.8651764047115,-32.1676315408756,
27.7872224014176));
#35864=CARTESIAN_POINT('Ctrl Pts',(-11.9510590294139,-32.2260999739477,
27.7933130098621));
#35865=CARTESIAN_POINT('Ctrl Pts',(-12.0339923783905,-32.2883067896332,
27.7994036183067));
#35866=CARTESIAN_POINT('Ctrl Pts',(-12.1170611141713,-32.3506151565291,
27.8055041695309));
#35867=CARTESIAN_POINT('Ctrl Pts',(-12.1971706257857,-32.4166738253225,
27.8116047207551));
#35868=CARTESIAN_POINT('Ctrl Pts',(-12.273982147142,-32.48615627833,27.8177052719793));
#35869=CARTESIAN_POINT('Ctrl Pts',(-12.3345056248876,-32.5409048319852,
27.8225121885686));
#35870=CARTESIAN_POINT('Ctrl Pts',(-12.3929821732118,-32.5977782733554,
27.8273191051579));
#35871=CARTESIAN_POINT('Ctrl Pts',(-12.4492635157942,-32.6566021906857,
27.8321260217471));
#35872=CARTESIAN_POINT('Ctrl Pts',(-12.5197884220859,-32.7303131411903,
27.8381494626683));
#35873=CARTESIAN_POINT('Ctrl Pts',(-12.5871173119216,-32.8073514381577,
27.8441729035895));
#35874=CARTESIAN_POINT('Ctrl Pts',(-12.6509144243622,-32.887404966112,27.8501963445107));
#35875=CARTESIAN_POINT('Ctrl Pts',(-12.7146125210988,-32.9673342477465,
27.8562104368074));
#35876=CARTESIAN_POINT('Ctrl Pts',(-12.7747894695597,-33.0502691130629,
27.8622245291042));
#35877=CARTESIAN_POINT('Ctrl Pts',(-12.8311464980834,-33.1358609040927,
27.8682386214009));
#35878=CARTESIAN_POINT('Ctrl Pts',(-12.8874529871053,-33.221375938654,27.8742473204178));
#35879=CARTESIAN_POINT('Ctrl Pts',(-12.9399461180647,-33.309542802434,27.8802560194346));
#35880=CARTESIAN_POINT('Ctrl Pts',(-12.9883679065639,-33.3999805258939,
27.8862647184515));
#35881=CARTESIAN_POINT('Ctrl Pts',(-13.0367575515633,-33.4903582147073,
27.8922694287554));
#35882=CARTESIAN_POINT('Ctrl Pts',(-13.0810810178945,-33.5830033808398,
27.8982741390593));
#35883=CARTESIAN_POINT('Ctrl Pts',(-13.1211247321806,-33.6775078568586,
27.9042788493632));
#35884=CARTESIAN_POINT('Ctrl Pts',(-13.1414419793625,-33.7254572250255,
27.9073254993974));
#35885=CARTESIAN_POINT('Ctrl Pts',(-13.1606582077987,-33.7738848260026,
27.9103721494316));
#35886=CARTESIAN_POINT('Ctrl Pts',(-13.1787501240207,-33.8227350716434,
27.9134187994658));
#35887=CARTESIAN_POINT('Origin',(-10.,-35.,23.));
#35888=CARTESIAN_POINT('',(-13.1787501097524,-33.8227350331175,29.1634929519179));
#35889=CARTESIAN_POINT('',(-13.1787501240208,-33.8227350716437,28.823527842849));
#35890=CARTESIAN_POINT('',(-13.1787501240207,-33.8227350716434,23.));
#35891=CARTESIAN_POINT('',(-7.42676557298528,-32.7934484719078,30.));
#35892=CARTESIAN_POINT('Ctrl Pts',(-7.42676557298526,-32.7934484719078,
30.));
#35893=CARTESIAN_POINT('Ctrl Pts',(-7.42045295623278,-32.8008101140653,
29.9994308516325));
#35894=CARTESIAN_POINT('Ctrl Pts',(-7.41417188875379,-32.8081988938986,
29.9988635376667));
#35895=CARTESIAN_POINT('Ctrl Pts',(-7.40029705405223,-32.82466331742,29.9976078642351));
#35896=CARTESIAN_POINT('Ctrl Pts',(-7.3927189018354,-32.8337520059171,29.9969203688605));
#35897=CARTESIAN_POINT('Ctrl Pts',(-7.36365296757774,-32.8689850725241,
29.9942762747548));
#35898=CARTESIAN_POINT('Ctrl Pts',(-7.34250898726559,-32.8954116895691,
29.9923374526965));
#35899=CARTESIAN_POINT('Ctrl Pts',(-7.23066464143884,-33.0395730979113,
29.981973894332));
#35900=CARTESIAN_POINT('Ctrl Pts',(-7.14737974006372,-33.1628674953582,
29.97386011666));
#35901=CARTESIAN_POINT('Ctrl Pts',(-6.99559951859121,-33.4229059648852,
29.9574884969299));
#35902=CARTESIAN_POINT('Ctrl Pts',(-6.92771857518107,-33.559606692338,29.9492480664531));
#35903=CARTESIAN_POINT('Ctrl Pts',(-6.8342281892156,-33.784825790337,29.9357546417517));
#35904=CARTESIAN_POINT('Ctrl Pts',(-6.8026160581166,-33.8706223604427,29.9306341923334));
#35905=CARTESIAN_POINT('Ctrl Pts',(-6.76258063009137,-33.9945021639557,
29.923203264082));
#35906=CARTESIAN_POINT('Ctrl Pts',(-6.7512855014978,-34.0316178299341,29.920972378891));
#35907=CARTESIAN_POINT('Ctrl Pts',(-6.73249217375053,-34.0974062589309,
29.9170055373366));
#35908=CARTESIAN_POINT('Ctrl Pts',(-6.72472821916191,-34.1259991168292,
29.9152773583261));
#35909=CARTESIAN_POINT('Ctrl Pts',(-6.70914932295406,-34.1864978506844,
29.9116100895573));
#35910=CARTESIAN_POINT('Ctrl Pts',(-6.70142138553885,-34.2184227836219,
29.909668684328));
#35911=CARTESIAN_POINT('Ctrl Pts',(-6.68178351044353,-34.3050348342957,
29.9043821702176));
#35912=CARTESIAN_POINT('Ctrl Pts',(-6.67076241279652,-34.3599110889422,
29.9010116993012));
#35913=CARTESIAN_POINT('Ctrl Pts',(-6.60789009691365,-34.7187757307886,
29.8788139171087));
#35914=CARTESIAN_POINT('Ctrl Pts',(-6.59638019761221,-35.0283172761005,
29.8587607128677));
#35915=CARTESIAN_POINT('Ctrl Pts',(-6.64201860350012,-35.4877615589473,
29.8288687764698));
#35916=CARTESIAN_POINT('Ctrl Pts',(-6.66753844244158,-35.6392650389571,
29.8190273788908));
#35917=CARTESIAN_POINT('Ctrl Pts',(-6.70994576996796,-35.8165654634065,
29.8078585840293));
#35918=CARTESIAN_POINT('Ctrl Pts',(-6.71700888275631,-35.844514913058,29.8061086866409));
#35919=CARTESIAN_POINT('Ctrl Pts',(-6.72873079523429,-35.8885282184635,
29.8033734263145));
#35920=CARTESIAN_POINT('Ctrl Pts',(-6.73315323901014,-35.9046529011187,
29.8023756938387));
#35921=CARTESIAN_POINT('Ctrl Pts',(-6.74175642433794,-35.9351349870315,
29.8004986507799));
#35922=CARTESIAN_POINT('Ctrl Pts',(-6.74591303029129,-35.9494981069945,
29.7996181225295));
#35923=CARTESIAN_POINT('Ctrl Pts',(-6.75628299928376,-35.9844633455038,
29.7974840067185));
#35924=CARTESIAN_POINT('Ctrl Pts',(-6.76259766332361,-36.0050344390657,
29.7962362630186));
#35925=CARTESIAN_POINT('Ctrl Pts',(-6.78590624680633,-36.0784661715619,
29.791805548616));
#35926=CARTESIAN_POINT('Ctrl Pts',(-6.80400329066443,-36.1309702509515,
29.7886809796411));
#35927=CARTESIAN_POINT('Ctrl Pts',(-6.89313402640073,-36.3703041807197,
29.7745352753796));
#35928=CARTESIAN_POINT('Ctrl Pts',(-6.97931842156187,-36.5510789630564,
29.7641071426166));
#35929=CARTESIAN_POINT('Ctrl Pts',(-7.14584504109605,-36.8331685036441,
29.7467579644264));
#35930=CARTESIAN_POINT('Ctrl Pts',(-7.21691002322565,-36.939359338186,29.7399497211604));
#35931=CARTESIAN_POINT('Ctrl Pts',(-7.3439289923636,-37.1077532575538,29.7283971177205));
#35932=CARTESIAN_POINT('Ctrl Pts',(-7.39649518087785,-37.1723485236772,
29.7237639846271));
#35933=CARTESIAN_POINT('Ctrl Pts',(-7.47416806215517,-37.2609228966324,
29.7170722531329));
#35934=CARTESIAN_POINT('Ctrl Pts',(-7.4973483452594,-37.2865550262831,29.715093352464));
#35935=CARTESIAN_POINT('Ctrl Pts',(-7.53836442036808,-37.3305385401572,
29.7116200047846));
#35936=CARTESIAN_POINT('Ctrl Pts',(-7.55602387716367,-37.3490509296667,
29.710133298304));
#35937=CARTESIAN_POINT('Ctrl Pts',(-7.59300842837803,-37.3869532810686,
29.7070364537089));
#35938=CARTESIAN_POINT('Ctrl Pts',(-7.61236218715025,-37.4063125311953,
29.7054250756153));
#35939=CARTESIAN_POINT('Ctrl Pts',(-7.66332897322519,-37.4560735083499,
29.7012039386291));
#35940=CARTESIAN_POINT('Ctrl Pts',(-7.6953005197271,-37.4860990702586,29.6985777143103));
#35941=CARTESIAN_POINT('Ctrl Pts',(-7.85830967512745,-37.6333393469694,
29.6852885042185));
#35942=CARTESIAN_POINT('Ctrl Pts',(-7.99772571991931,-37.7408384349338,
29.6742196531397));
#35943=CARTESIAN_POINT('Ctrl Pts',(-8.31020344983826,-37.9451715705292,
29.6501926681347));
#35944=CARTESIAN_POINT('Ctrl Pts',(-8.48471222671159,-38.0386427793486,
29.6372125479186));
#35945=CARTESIAN_POINT('Ctrl Pts',(-8.72023422058169,-38.1394326880846,
29.6208818902536));
#35946=CARTESIAN_POINT('Ctrl Pts',(-8.77469235248713,-38.1610852485021,
29.6171856118582));
#35947=CARTESIAN_POINT('Ctrl Pts',(-8.86803820943254,-38.1954244499402,
29.6110150118393));
#35948=CARTESIAN_POINT('Ctrl Pts',(-8.90664327070889,-38.208838779557,29.6085099334164));
#35949=CARTESIAN_POINT('Ctrl Pts',(-8.96295821420876,-38.2272724531387,
29.6049329637538));
#35950=CARTESIAN_POINT('Ctrl Pts',(-8.98047978690964,-38.2328504022311,
29.6038307732371));
#35951=CARTESIAN_POINT('Ctrl Pts',(-9.01198313323975,-38.2425978107858,
29.601869389844));
#35952=CARTESIAN_POINT('Ctrl Pts',(-9.02594765867314,-38.2468199725771,
29.6010071538164));
#35953=CARTESIAN_POINT('Ctrl Pts',(-9.05729624435203,-38.2560777376331,
29.5990868037388));
#35954=CARTESIAN_POINT('Ctrl Pts',(-9.07469450810737,-38.2610646088578,
29.598031466103));
#35955=CARTESIAN_POINT('Ctrl Pts',(-9.12576449401288,-38.2752611917336,
29.5949619708963));
#35956=CARTESIAN_POINT('Ctrl Pts',(-9.15954047621683,-38.2840906779917,
29.5929677561252));
#35957=CARTESIAN_POINT('Ctrl Pts',(-9.33012177461731,-38.3258786672071,
29.583048483904));
#35958=CARTESIAN_POINT('Ctrl Pts',(-9.46876093541178,-38.3508205140381,
29.5754730698707));
#35959=CARTESIAN_POINT('Ctrl Pts',(-9.85799846387174,-38.3960713984852,
29.5546071660816));
#35960=CARTESIAN_POINT('Ctrl Pts',(-10.1098689701902,-38.3972618388653,
29.5415030110932));
#35961=CARTESIAN_POINT('Ctrl Pts',(-10.4241018902344,-38.3637413616659,
29.5239587946753));
#35962=CARTESIAN_POINT('Ctrl Pts',(-10.4884313808481,-38.3550040832986,
29.5203077919428));
#35963=CARTESIAN_POINT('Ctrl Pts',(-10.5847276879626,-38.3390968386799,
29.5147335958256));
#35964=CARTESIAN_POINT('Ctrl Pts',(-10.6169080298704,-38.333301448101,29.5128524144307));
#35965=CARTESIAN_POINT('Ctrl Pts',(-10.6727136531311,-38.3224155671968,
29.5095560193829));
#35966=CARTESIAN_POINT('Ctrl Pts',(-10.6963779766777,-38.3175362137878,
29.5081474412235));
#35967=CARTESIAN_POINT('Ctrl Pts',(-10.7497802973275,-38.3059286295644,
29.5049435614938));
#35968=CARTESIAN_POINT('Ctrl Pts',(-10.7794834432576,-38.2990513894333,
29.5031437292096));
#35969=CARTESIAN_POINT('Ctrl Pts',(-10.8597870652118,-38.2793134692414,
29.4982279594976));
#35970=CARTESIAN_POINT('Ctrl Pts',(-10.9101881843626,-38.2656833361335,
29.4950884796461));
#35971=CARTESIAN_POINT('Ctrl Pts',(-11.166831840013,-38.1898756936946,29.4788171915766));
#35972=CARTESIAN_POINT('Ctrl Pts',(-11.3670978527846,-38.1093123705836,
29.4651224033587));
#35973=CARTESIAN_POINT('Ctrl Pts',(-11.6765486482266,-37.9491197511119,
29.4427547224856));
#35974=CARTESIAN_POINT('Ctrl Pts',(-11.7910535477669,-37.8810158421817,
29.4341920092372));
#35975=CARTESIAN_POINT('Ctrl Pts',(-11.9597415219069,-37.7667323860013,
29.4213816558017));
#35976=CARTESIAN_POINT('Ctrl Pts',(-12.0169744152259,-37.7252908972784,
29.4169991055172));
#35977=CARTESIAN_POINT('Ctrl Pts',(-12.0915250879281,-37.6676738027531,
29.41128335649));
#35978=CARTESIAN_POINT('Ctrl Pts',(-12.1100259357576,-37.6530645163738,
29.4098643319993));
#35979=CARTESIAN_POINT('Ctrl Pts',(-12.1406371129868,-37.628369474216,29.4075175666014));
#35980=CARTESIAN_POINT('Ctrl Pts',(-12.1528319999229,-37.6183902973371,
29.4065829678717));
#35981=CARTESIAN_POINT('Ctrl Pts',(-12.1777684613347,-37.5976925902304,
29.4046732883358));
#35982=CARTESIAN_POINT('Ctrl Pts',(-12.1905015132489,-37.5869645166162,
29.4036989108514));
#35983=CARTESIAN_POINT('Ctrl Pts',(-12.2247779792527,-37.5576507778983,
29.4010763884273));
#35984=CARTESIAN_POINT('Ctrl Pts',(-12.2461677389903,-37.5388865981802,
29.3994403068191));
#35985=CARTESIAN_POINT('Ctrl Pts',(-12.3796144082921,-37.4188137116368,
29.3892176200321));
#35986=CARTESIAN_POINT('Ctrl Pts',(-12.485041879298,-37.3103681156634,29.3810672753795));
#35987=CARTESIAN_POINT('Ctrl Pts',(-12.7062679107487,-37.050076439927,29.3628493400805));
#35988=CARTESIAN_POINT('Ctrl Pts',(-12.8171840470334,-36.8947748789666,
29.3528560813828));
#35989=CARTESIAN_POINT('Ctrl Pts',(-12.9511049416009,-36.6692910333153,
29.3385984195455));
#35990=CARTESIAN_POINT('Ctrl Pts',(-12.985773997062,-36.6064575111552,29.3346527340544));
#35991=CARTESIAN_POINT('Ctrl Pts',(-13.0439797208477,-36.4925638035981,
29.3275075439075));
#35992=CARTESIAN_POINT('Ctrl Pts',(-13.068289527896,-36.4419286125954,29.3243333587413));
#35993=CARTESIAN_POINT('Ctrl Pts',(-13.1039883720903,-36.3625759767692,
29.3193500754838));
#35994=CARTESIAN_POINT('Ctrl Pts',(-13.1162622550995,-36.3342663054993,
29.3175705856089));
#35995=CARTESIAN_POINT('Ctrl Pts',(-13.1383795284386,-36.2812823627509,
29.314235155466));
#35996=CARTESIAN_POINT('Ctrl Pts',(-13.1483226999809,-36.2566521695357,
29.3126826805156));
#35997=CARTESIAN_POINT('Ctrl Pts',(-13.1699193630262,-36.2012894991984,
29.3091876036033));
#35998=CARTESIAN_POINT('Ctrl Pts',(-13.1814172712542,-36.1704995777464,
29.3072400680654));
#35999=CARTESIAN_POINT('Ctrl Pts',(-13.2148807886321,-36.0767509084875,
29.301296931113));
#36000=CARTESIAN_POINT('Ctrl Pts',(-13.2354371883807,-36.0133095651879,
29.2972567709006));
#36001=CARTESIAN_POINT('Ctrl Pts',(-13.3389873981864,-35.6583518947158,
29.2745426702211));
#36002=CARTESIAN_POINT('Ctrl Pts',(-13.3844514449687,-35.3573497967771,
29.2547082041147));
#36003=CARTESIAN_POINT('Ctrl Pts',(-13.3904139851082,-34.9858265034264,
29.2310162355354));
#36004=CARTESIAN_POINT('Ctrl Pts',(-13.3894334515727,-34.9172370072722,
29.2266834672566));
#36005=CARTESIAN_POINT('Ctrl Pts',(-13.384313564574,-34.802628385905,29.2195581642237));
#36006=CARTESIAN_POINT('Ctrl Pts',(-13.3813134937036,-34.7565798745864,
29.2167263888309));
#36007=CARTESIAN_POINT('Ctrl Pts',(-13.3756699803911,-34.6907175259261,
29.2127338454318));
#36008=CARTESIAN_POINT('Ctrl Pts',(-13.3737902532577,-34.6708452720184,
29.211536753869));
#36009=CARTESIAN_POINT('Ctrl Pts',(-13.3701959708319,-34.636121404494,29.209459579159));
#36010=CARTESIAN_POINT('Ctrl Pts',(-13.3685585365772,-34.6212627164359,
29.2085754659808));
#36011=CARTESIAN_POINT('Ctrl Pts',(-13.3647497753424,-34.5886816769454,
29.2066475378164));
#36012=CARTESIAN_POINT('Ctrl Pts',(-13.362536670606,-34.5709650557845,29.2056059802193));
#36013=CARTESIAN_POINT('Ctrl Pts',(-13.3555736289156,-34.5185913490761,
29.2025448884499));
#36014=CARTESIAN_POINT('Ctrl Pts',(-13.3504269693134,-34.4839883793366,
29.2005457490284));
#36015=CARTESIAN_POINT('Ctrl Pts',(-13.3143128154574,-34.2645768592071,
29.1879830638303));
#36016=CARTESIAN_POINT('Ctrl Pts',(-13.268598232159,-34.0825049102161,29.1780597520728));
#36017=CARTESIAN_POINT('Ctrl Pts',(-13.1986445260763,-33.8775346613848,
29.166582597997));
#36018=CARTESIAN_POINT('Ctrl Pts',(-13.1888728361093,-33.8500675524935,
29.1650383635687));
#36019=CARTESIAN_POINT('Ctrl Pts',(-13.1787501097524,-33.8227350331175,
29.1634929519179));
#36020=CARTESIAN_POINT('',(-12.5373010662035,-32.7522214606544,30.));
#36021=CARTESIAN_POINT('Origin',(-10.,-35.,30.));
#36022=CARTESIAN_POINT('Ctrl Pts',(-12.5373010662035,-32.7522214606544,
30.));
#36023=CARTESIAN_POINT('Ctrl Pts',(-12.5306561517406,-32.7447206556345,
29.9993854250735));
#36024=CARTESIAN_POINT('Ctrl Pts',(-12.5239780167117,-32.7372493619221,
29.9987689954815));
#36025=CARTESIAN_POINT('Ctrl Pts',(-12.3346109279579,-32.5272726485279,
29.9813261713196));
#36026=CARTESIAN_POINT('Ctrl Pts',(-12.1281855390359,-32.3475265511935,
29.9633698274277));
#36027=CARTESIAN_POINT('Ctrl Pts',(-11.8172905516303,-32.1367067220662,
29.9394502167781));
#36028=CARTESIAN_POINT('Ctrl Pts',(-11.7295349331529,-32.0828601282193,
29.9329812956598));
#36029=CARTESIAN_POINT('Ctrl Pts',(-11.5754986281841,-31.9977426364613,
29.9221327305273));
#36030=CARTESIAN_POINT('Ctrl Pts',(-11.5104084178899,-31.9644748681779,
29.9176933147489));
#36031=CARTESIAN_POINT('Ctrl Pts',(-11.4133909228341,-31.9187830869011,
29.9112827185171));
#36032=CARTESIAN_POINT('Ctrl Pts',(-11.3822731483448,-31.9046982963963,
29.9092566876991));
#36033=CARTESIAN_POINT('Ctrl Pts',(-11.3263160351192,-31.8803827036066,
29.9056655026499));
#36034=CARTESIAN_POINT('Ctrl Pts',(-11.3015582984652,-31.8699724669921,
29.9040945175085));
#36035=CARTESIAN_POINT('Ctrl Pts',(-11.2485040519356,-31.8484023520084,
29.9007648567265));
#36036=CARTESIAN_POINT('Ctrl Pts',(-11.2201756644919,-31.8373268370343,
29.8990090431216));
#36037=CARTESIAN_POINT('Ctrl Pts',(-11.1431474279658,-31.808400249115,29.8942914827256));
#36038=CARTESIAN_POINT('Ctrl Pts',(-11.0941797798121,-31.791282808994,29.8913532204723));
#36039=CARTESIAN_POINT('Ctrl Pts',(-10.8312114803665,-31.7060784396256,
29.8758609008324));
#36040=CARTESIAN_POINT('Ctrl Pts',(-10.611235019576,-31.6582588968864,29.8639495621657));
#36041=CARTESIAN_POINT('Ctrl Pts',(-10.2620345608516,-31.6180102868005,
29.8452229819141));
#36042=CARTESIAN_POINT('Ctrl Pts',(-10.135228081649,-31.6105713624658,29.8384474161599));
#36043=CARTESIAN_POINT('Ctrl Pts',(-9.93956104973214,-31.6100916280698,
29.8276695400054));
#36044=CARTESIAN_POINT('Ctrl Pts',(-9.8708263071449,-31.6120146741786,29.8238212778998));
#36045=CARTESIAN_POINT('Ctrl Pts',(-9.77888496054104,-31.6173887666256,
29.8185357394441));
#36046=CARTESIAN_POINT('Ctrl Pts',(-9.75558304095288,-31.618992620027,29.8171842305274));
#36047=CARTESIAN_POINT('Ctrl Pts',(-9.71663497216785,-31.6220781145327,
29.814902557778));
#36048=CARTESIAN_POINT('Ctrl Pts',(-9.70097876753382,-31.623428026694,29.8139792321263));
#36049=CARTESIAN_POINT('Ctrl Pts',(-9.66868136025601,-31.6264391660914,
29.8120607777874));
#36050=CARTESIAN_POINT('Ctrl Pts',(-9.65204207586059,-31.6281147708921,
29.8110649239935));
#36051=CARTESIAN_POINT('Ctrl Pts',(-9.60678639400856,-31.6330106348878,
29.8083372352713));
#36052=CARTESIAN_POINT('Ctrl Pts',(-9.57819816527388,-31.6364724739644,
29.8065932601901));
#36053=CARTESIAN_POINT('Ctrl Pts',(-9.38983715711678,-31.6617207750094,
29.7949795702531));
#36054=CARTESIAN_POINT('Ctrl Pts',(-9.23176180625438,-31.6945185390058,
29.7846569208221));
#36055=CARTESIAN_POINT('Ctrl Pts',(-8.9521123635773,-31.7736885440693,29.7659520500969));
#36056=CARTESIAN_POINT('Ctrl Pts',(-8.82970498088461,-31.8160455659469,
29.7576020183712));
#36057=CARTESIAN_POINT('Ctrl Pts',(-8.57359015920598,-31.9214412213651,
29.7400043071661));
#36058=CARTESIAN_POINT('Ctrl Pts',(-8.44096175182365,-31.9864343477039,
29.7308156751714));
#36059=CARTESIAN_POINT('Ctrl Pts',(-8.27603078891577,-32.0810704645365,
29.7193422150339));
#36060=CARTESIAN_POINT('Ctrl Pts',(-8.23948655403542,-32.1029649421173,
29.7167960502857));
#36061=CARTESIAN_POINT('Ctrl Pts',(-8.17954572580588,-32.1404300672805,
29.7126114739265));
#36062=CARTESIAN_POINT('Ctrl Pts',(-8.15591347260316,-32.1556127347825,
29.7109594486569));
#36063=CARTESIAN_POINT('Ctrl Pts',(-8.10986093556611,-32.1860146662392,
29.7077347563357));
#36064=CARTESIAN_POINT('Ctrl Pts',(-8.08742907389436,-32.2012124667646,
29.706161469149));
#36065=CARTESIAN_POINT('Ctrl Pts',(-8.03833119757791,-32.235342719613,29.7027109130018));
#36066=CARTESIAN_POINT('Ctrl Pts',(-8.0117519070617,-32.2543955138952,29.7008382837032));
#36067=CARTESIAN_POINT('Ctrl Pts',(-7.92028176962833,-32.3219888878312,
29.6943728225227));
#36068=CARTESIAN_POINT('Ctrl Pts',(-7.85685658006084,-32.3724709153663,
29.689853022791));
#36069=CARTESIAN_POINT('Ctrl Pts',(-7.58150804141698,-32.6082394598178,
29.6699370741624));
#36070=CARTESIAN_POINT('Ctrl Pts',(-7.39136364075251,-32.8171970863654,
29.6554659459212));
#36071=CARTESIAN_POINT('Ctrl Pts',(-7.19054858480866,-33.1021334788801,
29.6365956262216));
#36072=CARTESIAN_POINT('Ctrl Pts',(-7.15350484188685,-33.1581588026217,
29.6329157366886));
#36073=CARTESIAN_POINT('Ctrl Pts',(-7.09421495757469,-33.2538942970608,
29.6266153441988));
#36074=CARTESIAN_POINT('Ctrl Pts',(-7.07105974920675,-33.2930200837212,
29.6240371239073));
#36075=CARTESIAN_POINT('Ctrl Pts',(-7.03893671154437,-33.3498778285416,
29.6202686032285));
#36076=CARTESIAN_POINT('Ctrl Pts',(-7.02932611122453,-33.3672429500064,
29.6191147785978));
#36077=CARTESIAN_POINT('Ctrl Pts',(-7.01275010019831,-33.3978245215162,
29.6170760364678));
#36078=CARTESIAN_POINT('Ctrl Pts',(-7.0057186838236,-33.4110042106843,29.6161951738241));
#36079=CARTESIAN_POINT('Ctrl Pts',(-6.9904364187531,-33.4401109573056,29.6142444460281));
#36080=CARTESIAN_POINT('Ctrl Pts',(-6.98222485247605,-33.4560570275034,
29.6131723923681));
#36081=CARTESIAN_POINT('Ctrl Pts',(-6.95867039359623,-33.5027033727614,
29.6100282889433));
#36082=CARTESIAN_POINT('Ctrl Pts',(-6.94366716234826,-33.533571565035,29.6079375869728));
#36083=CARTESIAN_POINT('Ctrl Pts',(-6.82431268162507,-33.7889268329935,
29.5905918399206));
#36084=CARTESIAN_POINT('Ctrl Pts',(-6.74437654767733,-34.0239894615909,
29.5743687130192));
#36085=CARTESIAN_POINT('Ctrl Pts',(-6.66495266076797,-34.3819025280143,
29.5508843058554));
#36086=CARTESIAN_POINT('Ctrl Pts',(-6.64529730870072,-34.499441216909,29.5433454835769));
#36087=CARTESIAN_POINT('Ctrl Pts',(-6.62281878658863,-34.6975219916843,
29.5310018882551));
#36088=CARTESIAN_POINT('Ctrl Pts',(-6.616603708912,-34.7775656458223,29.5261100967243));
#36089=CARTESIAN_POINT('Ctrl Pts',(-6.61176946195864,-34.8926699005481,
29.5192124964783));
#36090=CARTESIAN_POINT('Ctrl Pts',(-6.61084309435512,-34.9276015467316,
29.5171371173606));
#36091=CARTESIAN_POINT('Ctrl Pts',(-6.6101640395619,-34.9890491212673,29.5135165502415));
#36092=CARTESIAN_POINT('Ctrl Pts',(-6.61018204956866,-35.0155590176464,
29.5119644235955));
#36093=CARTESIAN_POINT('Ctrl Pts',(-6.61087126471377,-35.0710921438624,
29.508732709748));
#36094=CARTESIAN_POINT('Ctrl Pts',(-6.6116043275727,-35.1001125400493,29.507055160839));
#36095=CARTESIAN_POINT('Ctrl Pts',(-6.6145465589619,-35.1772976644314,29.5026212854126));
#36096=CARTESIAN_POINT('Ctrl Pts',(-6.61741069967402,-35.2254316209416,
29.4998852315949));
#36097=CARTESIAN_POINT('Ctrl Pts',(-6.64345057301039,-35.5471287286141,
29.4817611065749));
#36098=CARTESIAN_POINT('Ctrl Pts',(-6.69875750342126,-35.817056970931,29.4674454397777));
#36099=CARTESIAN_POINT('Ctrl Pts',(-6.83574493718743,-36.2257129992017,
29.4445267462644));
#36100=CARTESIAN_POINT('Ctrl Pts',(-6.89567578940038,-36.3704171157163,
29.4361163223826));
#36101=CARTESIAN_POINT('Ctrl Pts',(-6.97796816957431,-36.5357497886958,
29.4256026530395));
#36102=CARTESIAN_POINT('Ctrl Pts',(-6.99087696428638,-36.5608914895648,
29.4239778696222));
#36103=CARTESIAN_POINT('Ctrl Pts',(-7.01179025491488,-36.6003992970988,
29.4213787117641));
#36104=CARTESIAN_POINT('Ctrl Pts',(-7.01958780436487,-36.6148741468381,
29.4204165322531));
#36105=CARTESIAN_POINT('Ctrl Pts',(-7.03477106425126,-36.6425747719546,
29.418555006081));
#36106=CARTESIAN_POINT('Ctrl Pts',(-7.04214065894238,-36.655808748256,29.4176566397267));
#36107=CARTESIAN_POINT('Ctrl Pts',(-7.05888871716779,-36.685415530278,29.4156272194948));
#36108=CARTESIAN_POINT('Ctrl Pts',(-7.06831569410279,-36.701760318824,29.4144932598419));
#36109=CARTESIAN_POINT('Ctrl Pts',(-7.10225250751533,-36.7594821142495,
29.4104425147323));
#36110=CARTESIAN_POINT('Ctrl Pts',(-7.12750484700645,-36.8004135484821,
29.4074852082441));
#36111=CARTESIAN_POINT('Ctrl Pts',(-7.26628139098329,-37.01500114668,29.391579572438));
#36112=CARTESIAN_POINT('Ctrl Pts',(-7.39469513943745,-37.1784920962804,
29.3780656527411));
#36113=CARTESIAN_POINT('Ctrl Pts',(-7.62700505106574,-37.4241215347924,
29.356354825326));
#36114=CARTESIAN_POINT('Ctrl Pts',(-7.72218525187601,-37.5137691142794,
29.3480524135006));
#36115=CARTESIAN_POINT('Ctrl Pts',(-7.86722720113023,-37.6353596936616,
29.3363048842906));
#36116=CARTESIAN_POINT('Ctrl Pts',(-7.91311554080379,-37.6718447534405,
29.3327065933551));
#36117=CARTESIAN_POINT('Ctrl Pts',(-7.99843319002137,-37.7361395963207,
29.3262290696783));
#36118=CARTESIAN_POINT('Ctrl Pts',(-8.03755337391213,-37.7643323213405,
29.3233362606002));
#36119=CARTESIAN_POINT('Ctrl Pts',(-8.10129185662458,-37.8082314194474,
29.3187431584008));
#36120=CARTESIAN_POINT('Ctrl Pts',(-8.12553365844463,-37.8244702747154,
29.317023225757));
#36121=CARTESIAN_POINT('Ctrl Pts',(-8.17239670399396,-37.854993304413,29.3137485609934));
#36122=CARTESIAN_POINT('Ctrl Pts',(-8.19498319840252,-37.869326572894,29.3121921099086));
#36123=CARTESIAN_POINT('Ctrl Pts',(-8.24735732118121,-37.9016997150768,
29.3086315624225));
#36124=CARTESIAN_POINT('Ctrl Pts',(-8.27725825818875,-37.919551098129,29.3066343289466));
#36125=CARTESIAN_POINT('Ctrl Pts',(-8.37461928773071,-37.9756606656903,
29.3002395545177));
#36126=CARTESIAN_POINT('Ctrl Pts',(-8.44312077263089,-38.012066923236,29.295906109762));
#36127=CARTESIAN_POINT('Ctrl Pts',(-8.76828574431323,-38.1708212911649,
29.2759813179573));
#36128=CARTESIAN_POINT('Ctrl Pts',(-9.03841289963471,-38.262907974306,29.2613611154626));
#36129=CARTESIAN_POINT('Ctrl Pts',(-9.3826466085178,-38.3337353546587,29.2423341723327));
#36130=CARTESIAN_POINT('Ctrl Pts',(-9.44882123344469,-38.3453127941734,
29.2386533982827));
#36131=CARTESIAN_POINT('Ctrl Pts',(-9.56027391939214,-38.3614151181076,
29.2323531698479));
#36132=CARTESIAN_POINT('Ctrl Pts',(-9.60537925505668,-38.3670082684365,
29.2297759291608));
#36133=CARTESIAN_POINT('Ctrl Pts',(-9.6703289220231,-38.3737392027223,29.2260082337158));
#36134=CARTESIAN_POINT('Ctrl Pts',(-9.69009383672856,-38.3756121454315,
29.224854178764));
#36135=CARTESIAN_POINT('Ctrl Pts',(-9.72479870431629,-38.3785934519707,
29.222812880647));
#36136=CARTESIAN_POINT('Ctrl Pts',(-9.73973133779197,-38.3797765723892,
29.2219296579063));
#36137=CARTESIAN_POINT('Ctrl Pts',(-9.77269636957026,-38.3821686411594,
29.2199686438619));
#36138=CARTESIAN_POINT('Ctrl Pts',(-9.79073065098603,-38.3833323757695,
29.2188885870589));
#36139=CARTESIAN_POINT('Ctrl Pts',(-9.84339772183443,-38.3863082395444,
29.2157149675137));
#36140=CARTESIAN_POINT('Ctrl Pts',(-9.87804909260263,-38.3877330979374,
29.2136024398239));
#36141=CARTESIAN_POINT('Ctrl Pts',(-10.0992375914457,-38.3934305388155,
29.1999866938263));
#36142=CARTESIAN_POINT('Ctrl Pts',(-10.2858252244566,-38.3828261856222,
29.1879253988217));
#36143=CARTESIAN_POINT('Ctrl Pts',(-10.6270387969918,-38.3349945614687,
29.1657228109617));
#36144=CARTESIAN_POINT('Ctrl Pts',(-10.7817871966751,-38.3021481822025,
29.1555946626709));
#36145=CARTESIAN_POINT('Ctrl Pts',(-11.0257350640444,-38.2322500743586,
29.1397643006186));
#36146=CARTESIAN_POINT('Ctrl Pts',(-11.116627494615,-38.201986675398,29.1338946232812));
#36147=CARTESIAN_POINT('Ctrl Pts',(-11.2410006421076,-38.1546339265408,
29.125906158457));
#36148=CARTESIAN_POINT('Ctrl Pts',(-11.2756571009011,-38.140779669454,29.123684743495));
#36149=CARTESIAN_POINT('Ctrl Pts',(-11.33498627107,-38.1159181695847,29.1198883687044));
#36150=CARTESIAN_POINT('Ctrl Pts',(-11.3597686611631,-38.1051833495652,
29.1183045664951));
#36151=CARTESIAN_POINT('Ctrl Pts',(-11.4072312223114,-38.0839471196215,
29.1152742210495));
#36152=CARTESIAN_POINT('Ctrl Pts',(-11.4299286493282,-38.0734888410702,
29.1138263560431));
#36153=CARTESIAN_POINT('Ctrl Pts',(-11.4899341140477,-38.0450315386373,
29.110000783983));
#36154=CARTESIAN_POINT('Ctrl Pts',(-11.5270320409718,-38.0265977750521,
29.1076379452056));
#36155=CARTESIAN_POINT('Ctrl Pts',(-11.6739241603084,-37.9502192381555,
29.0982798932008));
#36156=CARTESIAN_POINT('Ctrl Pts',(-11.7808411519285,-37.8869403609809,
29.0914679645895));
#36157=CARTESIAN_POINT('Ctrl Pts',(-12.076976694583,-37.6889458770903,29.0722603903397));
#36158=CARTESIAN_POINT('Ctrl Pts',(-12.2561325260305,-37.5404959509894,
29.0602416907974));
#36159=CARTESIAN_POINT('Ctrl Pts',(-12.4836279800624,-37.3088053002554,
29.0426171665116));
#36160=CARTESIAN_POINT('Ctrl Pts',(-12.5458000791666,-37.2400645155497,
29.0374974802518));
#36161=CARTESIAN_POINT('Ctrl Pts',(-12.6212907351034,-37.1493911611895,
29.0307518206718));
#36162=CARTESIAN_POINT('Ctrl Pts',(-12.6372884116417,-37.1297317281637,
29.0292896486945));
#36163=CARTESIAN_POINT('Ctrl Pts',(-12.6629509068905,-37.0974627194914,
29.0268868801914));
#36164=CARTESIAN_POINT('Ctrl Pts',(-12.6727504658101,-37.0849609869787,
29.0259553337933));
#36165=CARTESIAN_POINT('Ctrl Pts',(-12.6909740369686,-37.0613727613137,
29.0241954972243));
#36166=CARTESIAN_POINT('Ctrl Pts',(-12.6994183450146,-37.0503022973416,
29.0233686649165));
#36167=CARTESIAN_POINT('Ctrl Pts',(-12.7217977374099,-37.0205850707344,
29.0211474484368));
#36168=CARTESIAN_POINT('Ctrl Pts',(-12.735609106206,-37.0018465734701,29.0197450777153));
#36169=CARTESIAN_POINT('Ctrl Pts',(-12.7872933816789,-36.9301904704465,
29.014380406756));
#36170=CARTESIAN_POINT('Ctrl Pts',(-12.8238307315121,-36.8763311371606,
29.0103442239218));
#36171=CARTESIAN_POINT('Ctrl Pts',(-12.9626713459625,-36.6584196172848,
28.9940987623408));
#36172=CARTESIAN_POINT('Ctrl Pts',(-13.0524094633405,-36.4867989293626,
28.9815119135545));
#36173=CARTESIAN_POINT('Ctrl Pts',(-13.1994769537249,-36.135331530575,28.9570738544806));
#36174=CARTESIAN_POINT('Ctrl Pts',(-13.2574284162014,-35.956456140612,28.9452554138676));
#36175=CARTESIAN_POINT('Ctrl Pts',(-13.3104556802108,-35.7302583670716,
28.9312104571741));
#36176=CARTESIAN_POINT('Ctrl Pts',(-13.3197773129748,-35.6866388934361,
28.9285407428772));
#36177=CARTESIAN_POINT('Ctrl Pts',(-13.3336179253263,-35.6149813238029,
28.9242162089102));
#36178=CARTESIAN_POINT('Ctrl Pts',(-13.3386500333267,-35.5870490004382,
28.9225455652366));
#36179=CARTESIAN_POINT('Ctrl Pts',(-13.3477776448171,-35.5324630223267,
28.9193090872333));
#36180=CARTESIAN_POINT('Ctrl Pts',(-13.351907065774,-35.5058172726549,28.9177423065832));
#36181=CARTESIAN_POINT('Ctrl Pts',(-13.360976406036,-35.4422969357932,28.9140369723842));
#36182=CARTESIAN_POINT('Ctrl Pts',(-13.3656281265312,-35.4053843239786,
28.9119074725128));
#36183=CARTESIAN_POINT('Ctrl Pts',(-13.3793607531627,-35.2797756250799,
28.904734764804));
#36184=CARTESIAN_POINT('Ctrl Pts',(-13.3855504025031,-35.1907976947157,
28.8997792954819));
#36185=CARTESIAN_POINT('Ctrl Pts',(-13.3963448169338,-34.8310795359271,
28.8800930409592));
#36186=CARTESIAN_POINT('Ctrl Pts',(-13.3720213298232,-34.5605060481494,
28.8661591960902));
#36187=CARTESIAN_POINT('Ctrl Pts',(-13.3020205114909,-34.2309418720216,
28.8479157967827));
#36188=CARTESIAN_POINT('Ctrl Pts',(-13.2863681330099,-34.166589248693,28.8442860523348));
#36189=CARTESIAN_POINT('Ctrl Pts',(-13.2569378835888,-34.0593708183655,
28.8380644260001));
#36190=CARTESIAN_POINT('Ctrl Pts',(-13.2441722875617,-34.0162452525518,
28.8355136982275));
#36191=CARTESIAN_POINT('Ctrl Pts',(-13.2245785486048,-33.9545874371081,
28.8317803780731));
#36192=CARTESIAN_POINT('Ctrl Pts',(-13.2184400212476,-33.9358392829293,
28.8306335529532));
#36193=CARTESIAN_POINT('Ctrl Pts',(-13.2073681900358,-33.9029962009852,
28.8286022971459));
#36194=CARTESIAN_POINT('Ctrl Pts',(-13.202504854457,-33.8888786357704,28.8277218147451));
#36195=CARTESIAN_POINT('Ctrl Pts',(-13.1915487826005,-33.8577442971194,
28.8257634062535));
#36196=CARTESIAN_POINT('Ctrl Pts',(-13.1854132048364,-33.8407440297242,
28.8246831712498));
#36197=CARTESIAN_POINT('Ctrl Pts',(-13.1790115181001,-33.8234410461142,
28.8235731461798));
#36198=CARTESIAN_POINT('Ctrl Pts',(-13.1788808503858,-33.8230880477997,
28.8235504960504));
#36199=CARTESIAN_POINT('Ctrl Pts',(-13.1787501240208,-33.8227350716437,
28.823527842849));
#36200=CARTESIAN_POINT('Origin',(130.,35.,32.7603849714045));
#36201=CARTESIAN_POINT('',(132.487160689988,38.2405642567579,18.0469660621892));
#36202=CARTESIAN_POINT('',(132.487160689988,38.2405642567579,17.9425407177715));
#36203=CARTESIAN_POINT('',(132.487160689988,38.2405642567579,32.7603849714045));
#36204=CARTESIAN_POINT('',(125.917571176467,34.9941421690681,17.135384982874));
#36205=CARTESIAN_POINT('Ctrl Pts',(132.487160689988,38.2405642567579,17.9425407177715));
#36206=CARTESIAN_POINT('Ctrl Pts',(132.581704160612,38.1680013371556,17.9367376591697));
#36207=CARTESIAN_POINT('Ctrl Pts',(132.673155546112,38.0912314422968,17.9309346005679));
#36208=CARTESIAN_POINT('Ctrl Pts',(132.761122989607,38.0105522477221,17.9251315419662));
#36209=CARTESIAN_POINT('Ctrl Pts',(132.849041292519,37.9299181223515,17.9193317250828));
#36210=CARTESIAN_POINT('Ctrl Pts',(132.933479223414,37.8453793164917,17.9135319081995));
#36211=CARTESIAN_POINT('Ctrl Pts',(133.014078181312,37.7572736021182,17.9077320913162));
#36212=CARTESIAN_POINT('Ctrl Pts',(133.094654295706,37.6691928588278,17.9019339182276));
#36213=CARTESIAN_POINT('Ctrl Pts',(133.171393324555,37.5775475187252,17.896135745139));
#36214=CARTESIAN_POINT('Ctrl Pts',(133.243974139683,37.4827115783087,17.8903375720504));
#36215=CARTESIAN_POINT('Ctrl Pts',(133.316551597246,37.3878800249717,17.8845396671834));
#36216=CARTESIAN_POINT('Ctrl Pts',(133.384970975045,37.2898584898196,17.8787417623164));
#36217=CARTESIAN_POINT('Ctrl Pts',(133.448952408548,37.1890528279536,17.8729438574494));
#36218=CARTESIAN_POINT('Ctrl Pts',(133.512946056224,37.0882279221019,17.8671448457517));
#36219=CARTESIAN_POINT('Ctrl Pts',(133.572499855678,36.9846181780772,17.861345834054));
#36220=CARTESIAN_POINT('Ctrl Pts',(133.627378475355,36.8786565403319,17.8555468223563));
#36221=CARTESIAN_POINT('Ctrl Pts',(133.682314831683,36.7725834225588,17.8497417096394));
#36222=CARTESIAN_POINT('Ctrl Pts',(133.732565995698,36.6641538329253,17.8439365969225));
#36223=CARTESIAN_POINT('Ctrl Pts',(133.777943536637,36.5538235530401,17.8381314842057));
#36224=CARTESIAN_POINT('Ctrl Pts',(133.823345530585,36.4434338184715,17.8323232432348));
#36225=CARTESIAN_POINT('Ctrl Pts',(133.863868530571,36.3311417379457,17.8265150022639));
#36226=CARTESIAN_POINT('Ctrl Pts',(133.89937362207,36.217419547857,17.8207067612931));
#36227=CARTESIAN_POINT('Ctrl Pts',(133.934935959653,36.1035139995584,17.8148891554949));
#36228=CARTESIAN_POINT('Ctrl Pts',(133.965464119497,35.9881741305205,17.8090715496968));
#36229=CARTESIAN_POINT('Ctrl Pts',(133.990869940087,35.8718842361849,17.8032539438986));
#36230=CARTESIAN_POINT('Ctrl Pts',(134.012612259543,35.7723632613325,17.7982752326903));
#36231=CARTESIAN_POINT('Ctrl Pts',(134.030603846559,35.6721467966439,17.7932965214821));
#36232=CARTESIAN_POINT('Ctrl Pts',(134.044819683309,35.5715406630487,17.7883178102738));
#36233=CARTESIAN_POINT('Ctrl Pts',(134.061475242332,35.4536685021903,17.7824846525185));
#36234=CARTESIAN_POINT('Ctrl Pts',(134.073000529151,35.3348804874062,17.7766514947632));
#36235=CARTESIAN_POINT('Ctrl Pts',(134.079303343295,35.2156599948512,17.7708183370079));
#36236=CARTESIAN_POINT('Ctrl Pts',(134.085598200645,35.0965900085528,17.7649925431439));
#36237=CARTESIAN_POINT('Ctrl Pts',(134.08668367818,34.9770890332654,17.7591667492798));
#36238=CARTESIAN_POINT('Ctrl Pts',(134.082518957228,34.8576484497061,17.7533409554158));
#36239=CARTESIAN_POINT('Ctrl Pts',(134.078358418247,34.7383278014458,17.7475210114756));
#36240=CARTESIAN_POINT('Ctrl Pts',(134.06895818348,34.6190678285839,17.7417010675355));
#36241=CARTESIAN_POINT('Ctrl Pts',(134.054329427311,34.5003622363787,17.7358811235954));
#36242=CARTESIAN_POINT('Ctrl Pts',(134.039180772276,34.3774379052638,17.7298543416833));
#36243=CARTESIAN_POINT('Ctrl Pts',(134.018425025373,34.2551085359106,17.7238275597712));
#36244=CARTESIAN_POINT('Ctrl Pts',(133.992133504218,34.133919700893,17.7178007778591));
#36245=CARTESIAN_POINT('Ctrl Pts',(133.966773400114,34.0170241643375,17.7119875038458));
#36246=CARTESIAN_POINT('Ctrl Pts',(133.936263183771,33.9011901548335,17.7061742298324));
#36247=CARTESIAN_POINT('Ctrl Pts',(133.900719174936,33.786898636434,17.7003609558191));
#36248=CARTESIAN_POINT('Ctrl Pts',(133.865180801703,33.672625239272,17.6945486035165));
#36249=CARTESIAN_POINT('Ctrl Pts',(133.82461034417,33.5598942351823,17.6887362512138));
#36250=CARTESIAN_POINT('Ctrl Pts',(133.779174119798,33.4491718430957,17.6829238989112));
#36251=CARTESIAN_POINT('Ctrl Pts',(133.733734473169,33.338441111396,17.6771111088221));
#36252=CARTESIAN_POINT('Ctrl Pts',(133.683428485553,33.2297196688949,17.671298318733));
#36253=CARTESIAN_POINT('Ctrl Pts',(133.628470545243,33.1234535704379,17.6654855286438));
#36254=CARTESIAN_POINT('Ctrl Pts',(133.573495612497,33.0171546155841,17.6596709412991));
#36255=CARTESIAN_POINT('Ctrl Pts',(133.513866053221,32.9133128758775,17.6538563539544));
#36256=CARTESIAN_POINT('Ctrl Pts',(133.44984179878,32.8123490764308,17.6480417666097));
#36257=CARTESIAN_POINT('Ctrl Pts',(133.385748640617,32.7112766184512,17.6422209215317));
#36258=CARTESIAN_POINT('Ctrl Pts',(133.317251564341,32.6130886271358,17.6364000764537));
#36259=CARTESIAN_POINT('Ctrl Pts',(133.244653443095,32.5181762685054,17.6305792313757));
#36260=CARTESIAN_POINT('Ctrl Pts',(133.172008829618,32.4232031274841,17.6247546585968));
#36261=CARTESIAN_POINT('Ctrl Pts',(133.095258200717,32.3315101087105,17.618930085818));
#36262=CARTESIAN_POINT('Ctrl Pts',(133.014743192293,32.2434535221544,17.6131055130391));
#36263=CARTESIAN_POINT('Ctrl Pts',(132.934115768986,32.1552739911792,17.6072728080041));
#36264=CARTESIAN_POINT('Ctrl Pts',(132.849713761962,32.070741313553,17.6014401029691));
#36265=CARTESIAN_POINT('Ctrl Pts',(132.761914021121,31.9901734369007,17.5956073979341));
#36266=CARTESIAN_POINT('Ctrl Pts',(132.739991625622,31.9700567390663,17.5941510511912));
#36267=CARTESIAN_POINT('Ctrl Pts',(132.717857555366,31.9501870155264,17.5926947044482));
#36268=CARTESIAN_POINT('Ctrl Pts',(132.695517967664,31.930568800901,17.5912383577053));
#36269=CARTESIAN_POINT('Ctrl Pts',(132.606179064856,31.852113021276,17.5854142385741));
#36270=CARTESIAN_POINT('Ctrl Pts',(132.51326988702,31.7774361102096,17.5795901194429));
#36271=CARTESIAN_POINT('Ctrl Pts',(132.417143370658,31.7068794547295,17.5737660003117));
#36272=CARTESIAN_POINT('Ctrl Pts',(132.3211364942,31.63641061468,17.5679491299301));
#36273=CARTESIAN_POINT('Ctrl Pts',(132.221920570064,31.5700520697725,17.5621322595485));
#36274=CARTESIAN_POINT('Ctrl Pts',(132.119883396255,31.5081066187121,17.5563153891669));
#36275=CARTESIAN_POINT('Ctrl Pts',(132.017946657148,31.4462221402628,17.550504244303));
#36276=CARTESIAN_POINT('Ctrl Pts',(131.913194539782,31.3887423246919,17.5446930994391));
#36277=CARTESIAN_POINT('Ctrl Pts',(131.806045274565,31.3359277482259,17.5388819545752));
#36278=CARTESIAN_POINT('Ctrl Pts',(131.694858288392,31.281122952585,17.5328518275152));
#36279=CARTESIAN_POINT('Ctrl Pts',(131.581090298122,31.2313421790629,17.5268217004553));
#36280=CARTESIAN_POINT('Ctrl Pts',(131.465238829872,31.1868254470279,17.5207915733954));
#36281=CARTESIAN_POINT('Ctrl Pts',(131.353715623188,31.1439718795879,17.514986734522));
#36282=CARTESIAN_POINT('Ctrl Pts',(131.240262240536,31.1059962332136,17.5091818956486));
#36283=CARTESIAN_POINT('Ctrl Pts',(131.125343875498,31.0730640237102,17.5033770567752));
#36284=CARTESIAN_POINT('Ctrl Pts',(131.010440813741,31.0401361996751,17.497572990912));
#36285=CARTESIAN_POINT('Ctrl Pts',(130.894073549817,31.0122505893171,17.4917689250489));
#36286=CARTESIAN_POINT('Ctrl Pts',(130.776722274975,30.9895227830646,17.4859648591858));
#36287=CARTESIAN_POINT('Ctrl Pts',(130.659358966333,30.9667926461867,17.4801601981441));
#36288=CARTESIAN_POINT('Ctrl Pts',(130.541011846842,30.9492214427428,17.4743555371023));
#36289=CARTESIAN_POINT('Ctrl Pts',(130.422170497491,30.9368734857196,17.4685508760606));
#36290=CARTESIAN_POINT('Ctrl Pts',(130.303288949406,30.9245213519327,17.4627442515607));
#36291=CARTESIAN_POINT('Ctrl Pts',(130.183913244704,30.9173960206188,17.4569376270608));
#36292=CARTESIAN_POINT('Ctrl Pts',(130.064536629376,30.9155098208627,17.4511310025609));
#36293=CARTESIAN_POINT('Ctrl Pts',(129.945025504436,30.9136214957993,17.445317835349));
#36294=CARTESIAN_POINT('Ctrl Pts',(129.825513875141,30.9169840921842,17.4395046681372));
#36295=CARTESIAN_POINT('Ctrl Pts',(129.706493698786,30.9255578233152,17.4336915009253));
#36296=CARTESIAN_POINT('Ctrl Pts',(129.587393980228,30.9341372843442,17.427874448724));
#36297=CARTESIAN_POINT('Ctrl Pts',(129.468786773136,30.9479347687692,17.4220573965227));
#36298=CARTESIAN_POINT('Ctrl Pts',(129.35115597566,30.9668589868344,17.4162403443214));
#36299=CARTESIAN_POINT('Ctrl Pts',(129.233354945568,30.9858105915978,17.4104148738144));
#36300=CARTESIAN_POINT('Ctrl Pts',(129.11653354369,31.0099036563026,17.4045894033074));
#36301=CARTESIAN_POINT('Ctrl Pts',(129.001162746281,31.0389964477946,17.3987639328003));
#36302=CARTESIAN_POINT('Ctrl Pts',(128.970762585872,31.0466623870788,17.3972289235792));
#36303=CARTESIAN_POINT('Ctrl Pts',(128.940463045509,31.0546752045074,17.395693914358));
#36304=CARTESIAN_POINT('Ctrl Pts',(128.910272516687,31.0630317486532,17.3941589051369));
#36305=CARTESIAN_POINT('Ctrl Pts',(128.796624973599,31.0944886574235,17.3883806020264));
#36306=CARTESIAN_POINT('Ctrl Pts',(128.684141022598,31.1309259262771,17.3826022989159));
#36307=CARTESIAN_POINT('Ctrl Pts',(128.573294016828,31.1722415126369,17.3768239958053));
#36308=CARTESIAN_POINT('Ctrl Pts',(128.462588204215,31.2135044726036,17.3710530529014));
#36309=CARTESIAN_POINT('Ctrl Pts',(128.353515576709,31.2596332518481,17.3652821099975));
#36310=CARTESIAN_POINT('Ctrl Pts',(128.246536858835,31.310475367669,17.3595111670936));
#36311=CARTESIAN_POINT('Ctrl Pts',(128.139665375776,31.3612665196631,17.3537460089476));
#36312=CARTESIAN_POINT('Ctrl Pts',(128.034884001239,31.4167614353966,17.3479808508016));
#36313=CARTESIAN_POINT('Ctrl Pts',(127.932635253745,31.4767588776894,17.3422156926557));
#36314=CARTESIAN_POINT('Ctrl Pts',(127.825381772362,31.5396929939268,17.3361683493187));
#36315=CARTESIAN_POINT('Ctrl Pts',(127.72091557039,31.6075814196211,17.3301210059818));
#36316=CARTESIAN_POINT('Ctrl Pts',(127.61972050568,31.6801363689273,17.3240736626448));
#36317=CARTESIAN_POINT('Ctrl Pts',(127.523350765193,31.7492316519403,17.3183146771677));
#36318=CARTESIAN_POINT('Ctrl Pts',(127.429947779764,31.8225584266251,17.3125556916906));
#36319=CARTESIAN_POINT('Ctrl Pts',(127.33990051386,31.899823275386,17.3067967062135));
#36320=CARTESIAN_POINT('Ctrl Pts',(127.249863444096,31.977079375373,17.301038372832));
#36321=CARTESIAN_POINT('Ctrl Pts',(127.163181654013,32.0582723926968,17.2952800394504));
#36322=CARTESIAN_POINT('Ctrl Pts',(127.080210638688,32.1430689393043,17.2895217060688));
#36323=CARTESIAN_POINT('Ctrl Pts',(126.997228643662,32.2278767071884,17.2837626106768));
#36324=CARTESIAN_POINT('Ctrl Pts',(126.917958690283,32.3162886553778,17.2780035152848));
#36325=CARTESIAN_POINT('Ctrl Pts',(126.842718523364,32.4079354411411,17.2722444198928));
#36326=CARTESIAN_POINT('Ctrl Pts',(126.767449922388,32.4996168611974,17.2664831480776));
#36327=CARTESIAN_POINT('Ctrl Pts',(126.696214399148,32.5945352284173,17.2607218762623));
#36328=CARTESIAN_POINT('Ctrl Pts',(126.62928816068,32.692289728699,17.2549606044471));
#36329=CARTESIAN_POINT('Ctrl Pts',(126.562279589997,32.7901644859184,17.2491922451535));
#36330=CARTESIAN_POINT('Ctrl Pts',(126.49959111936,32.8908819966749,17.2434238858598));
#36331=CARTESIAN_POINT('Ctrl Pts',(126.441454582281,32.994014080301,17.2376555265662));
#36332=CARTESIAN_POINT('Ctrl Pts',(126.383276299843,33.0972202186628,17.2318830252607));
#36333=CARTESIAN_POINT('Ctrl Pts',(126.329656643999,33.2028440115217,17.2261105239551));
#36334=CARTESIAN_POINT('Ctrl Pts',(126.280779817259,33.3104360822107,17.2203380226495));
#36335=CARTESIAN_POINT('Ctrl Pts',(126.231825524133,33.4181986788858,17.2145563723289));
#36336=CARTESIAN_POINT('Ctrl Pts',(126.187629215659,33.5279353952719,17.2087747220083));
#36337=CARTESIAN_POINT('Ctrl Pts',(126.148325715824,33.6391803173768,17.2029930716876));
#36338=CARTESIAN_POINT('Ctrl Pts',(126.134925509125,33.6771083633948,17.2010218653146));
#36339=CARTESIAN_POINT('Ctrl Pts',(126.122093612364,33.7152116296383,17.1990506589415));
#36340=CARTESIAN_POINT('Ctrl Pts',(126.109834007681,33.7534713993642,17.1970794525685));
#36341=CARTESIAN_POINT('Ctrl Pts',(126.063948535826,33.8966707628269,17.1897015854277));
#36342=CARTESIAN_POINT('Ctrl Pts',(126.025960954389,34.0424458435051,17.182323718287));
#36343=CARTESIAN_POINT('Ctrl Pts',(125.996105954063,34.1900262541832,17.1749458511462));
#36344=CARTESIAN_POINT('Ctrl Pts',(125.966728932655,34.3352439006973,17.1676861037478));
#36345=CARTESIAN_POINT('Ctrl Pts',(125.945226128074,34.482209666858,17.1604263563494));
#36346=CARTESIAN_POINT('Ctrl Pts',(125.931775537335,34.6301693341903,17.153166608951));
#36347=CARTESIAN_POINT('Ctrl Pts',(125.920793836325,34.7509706327901,17.1472394064299));
#36348=CARTESIAN_POINT('Ctrl Pts',(125.915178848841,34.8724341239438,17.1413122039088));
#36349=CARTESIAN_POINT('Ctrl Pts',(125.915004205853,34.9941381057528,17.1353850013877));
#36350=CARTESIAN_POINT('',(126.824949217806,37.5702679880679,17.));
#36351=CARTESIAN_POINT('Ctrl Pts',(125.919161438299,34.9941446863292,17.1353849714045));
#36352=CARTESIAN_POINT('Ctrl Pts',(125.92665550953,35.9198397886616,17.090256647603));
#36353=CARTESIAN_POINT('Ctrl Pts',(126.2419104066,36.8500404311903,17.0451283238015));
#36354=CARTESIAN_POINT('Ctrl Pts',(126.824949217806,37.5702679880679,17.));
#36355=CARTESIAN_POINT('',(128.537425954644,38.8141974466263,17.0000001263023));
#36356=CARTESIAN_POINT('Origin',(130.,35.,17.));
#36357=CARTESIAN_POINT('',(125.915001286801,35.0032424009398,17.239615028553));
#36358=CARTESIAN_POINT('Ctrl Pts',(125.915001286801,35.0032424009399,17.239615028553));
#36359=CARTESIAN_POINT('Ctrl Pts',(125.915121833596,35.1551155066225,17.2322214796527));
#36360=CARTESIAN_POINT('Ctrl Pts',(125.923715576038,35.3066295363267,17.2248279307525));
#36361=CARTESIAN_POINT('Ctrl Pts',(125.94064101634,35.4569788198348,17.2174343818523));
#36362=CARTESIAN_POINT('Ctrl Pts',(125.95789917151,35.610283621261,17.2098954929428));
#36363=CARTESIAN_POINT('Ctrl Pts',(125.983819809633,35.7623776772745,17.2023566040334));
#36364=CARTESIAN_POINT('Ctrl Pts',(126.018204397236,35.9124301495502,17.1948177151239));
#36365=CARTESIAN_POINT('Ctrl Pts',(126.025778835979,35.9454845887252,17.193157004433));
#36366=CARTESIAN_POINT('Ctrl Pts',(126.033763810909,35.9784400380016,17.1914962937421));
#36367=CARTESIAN_POINT('Ctrl Pts',(126.042156888354,36.0112877452039,17.1898355830512));
#36368=CARTESIAN_POINT('Ctrl Pts',(126.071413105751,36.1257868272338,17.1840467513238));
#36369=CARTESIAN_POINT('Ctrl Pts',(126.10569155362,36.2392087379591,17.1782579195964));
#36370=CARTESIAN_POINT('Ctrl Pts',(126.144897365093,36.3510768572991,17.1724690878689));
#36371=CARTESIAN_POINT('Ctrl Pts',(126.1840541934,36.4628052102548,17.1666874886228));
#36372=CARTESIAN_POINT('Ctrl Pts',(126.228126008179,36.5729832451381,17.1609058893767));
#36373=CARTESIAN_POINT('Ctrl Pts',(126.276967308782,36.681146210216,17.1551242901305));
#36374=CARTESIAN_POINT('Ctrl Pts',(126.325760720866,36.7892031223401,17.1493483596979));
#36375=CARTESIAN_POINT('Ctrl Pts',(126.379314148376,36.895248519388,17.1435724292653));
#36376=CARTESIAN_POINT('Ctrl Pts',(126.437433053197,36.9988350981372,17.1377964988327));
#36377=CARTESIAN_POINT('Ctrl Pts',(126.495512284402,37.1023509657452,17.1320245112142));
#36378=CARTESIAN_POINT('Ctrl Pts',(126.558150592357,37.2034109938462,17.1262525235958));
#36379=CARTESIAN_POINT('Ctrl Pts',(126.625106600157,37.3015906542424,17.1204805359774));
#36380=CARTESIAN_POINT('Ctrl Pts',(126.692038577867,37.3997350785762,17.114710619889));
#36381=CARTESIAN_POINT('Ctrl Pts',(126.7632849423,37.4950008487302,17.1089407038006));
#36382=CARTESIAN_POINT('Ctrl Pts',(126.838560236032,37.5869912289767,17.1031707877122));
#36383=CARTESIAN_POINT('Ctrl Pts',(126.913826833735,37.6789709822169,17.0974015381819));
#36384=CARTESIAN_POINT('Ctrl Pts',(126.993121173229,37.7676757778223,17.0916322886517));
#36385=CARTESIAN_POINT('Ctrl Pts',(127.076117092332,37.8527414432873,17.0858630391214));
#36386=CARTESIAN_POINT('Ctrl Pts',(127.159123622615,37.9378179845522,17.0800930519821));
#36387=CARTESIAN_POINT('Ctrl Pts',(127.245832384141,38.0192541748308,17.0743230648428));
#36388=CARTESIAN_POINT('Ctrl Pts',(127.335880412824,38.0967227556284,17.0685530777035));
#36389=CARTESIAN_POINT('Ctrl Pts',(127.426018169077,38.1742685293145,17.0627773411111));
#36390=CARTESIAN_POINT('Ctrl Pts',(127.519501524578,38.2478385262392,17.0570016045186));
#36391=CARTESIAN_POINT('Ctrl Pts',(127.615934339647,38.3171457500579,17.0512258679262));
#36392=CARTESIAN_POINT('Ctrl Pts',(127.712414812686,38.3864872261334,17.0454472769125));
#36393=CARTESIAN_POINT('Ctrl Pts',(127.811847302618,38.4515615061195,17.0396686858988));
#36394=CARTESIAN_POINT('Ctrl Pts',(127.913808126291,38.5121259183109,17.0338900948852));
#36395=CARTESIAN_POINT('Ctrl Pts',(128.015934147913,38.5727884575696,17.0281021413404));
#36396=CARTESIAN_POINT('Ctrl Pts',(128.120596323314,38.6289263334615,17.0223141877957));
#36397=CARTESIAN_POINT('Ctrl Pts',(128.227347413244,38.6803434359674,17.016526234251));
#36398=CARTESIAN_POINT('Ctrl Pts',(128.328948092551,38.7292798219659,17.0110175316014));
#36399=CARTESIAN_POINT('Ctrl Pts',(128.432440532449,38.7739402350394,17.0055088289519));
#36400=CARTESIAN_POINT('Ctrl Pts',(128.537425954644,38.8141974466263,17.0000001263023));
#36401=CARTESIAN_POINT('Ctrl Pts',(132.487160689988,38.2405642567579,18.0469660621892));
#36402=CARTESIAN_POINT('Ctrl Pts',(132.581995851227,38.1677774621218,18.0411567024933));
#36403=CARTESIAN_POINT('Ctrl Pts',(132.673587220315,38.0908594993528,18.0353473427975));
#36404=CARTESIAN_POINT('Ctrl Pts',(132.761569442504,38.0101427232324,18.0295379831017));
#36405=CARTESIAN_POINT('Ctrl Pts',(132.849596883711,37.9293844622157,18.0237256376488));
#36406=CARTESIAN_POINT('Ctrl Pts',(132.934011193521,37.8448237867974,18.0179132921958));
#36407=CARTESIAN_POINT('Ctrl Pts',(133.014484760213,37.756829089814,18.0121009467429));
#36408=CARTESIAN_POINT('Ctrl Pts',(133.095089119703,37.6686913760231,18.0062791545493));
#36409=CARTESIAN_POINT('Ctrl Pts',(133.171739674954,37.5771088012885,18.0004573623556));
#36410=CARTESIAN_POINT('Ctrl Pts',(133.244149517064,37.4824824089878,17.994635570162));
#36411=CARTESIAN_POINT('Ctrl Pts',(133.312483103624,37.3931829355919,17.9891415112163));
#36412=CARTESIAN_POINT('Ctrl Pts',(133.377040210958,37.3011732045948,17.9836474522707));
#36413=CARTESIAN_POINT('Ctrl Pts',(133.437616789531,37.2068112307882,17.978153393325));
#36414=CARTESIAN_POINT('Ctrl Pts',(133.50183711402,37.1067732834495,17.9723288608644));
#36415=CARTESIAN_POINT('Ctrl Pts',(133.561790434345,37.0037686003075,17.9665043284039));
#36416=CARTESIAN_POINT('Ctrl Pts',(133.61719148879,36.8981967056732,17.9606797959433));
#36417=CARTESIAN_POINT('Ctrl Pts',(133.672522632229,36.792758033002,17.9548626135037));
#36418=CARTESIAN_POINT('Ctrl Pts',(133.72331274761,36.6847589506059,17.9490454310642));
#36419=CARTESIAN_POINT('Ctrl Pts',(133.769319891238,36.5746277520473,17.9432282486247));
#36420=CARTESIAN_POINT('Ctrl Pts',(133.815280959147,36.4646068488419,17.9374168920383));
#36421=CARTESIAN_POINT('Ctrl Pts',(133.856468428238,36.3524584518935,17.931605535452));
#36422=CARTESIAN_POINT('Ctrl Pts',(133.892686612845,36.2386347057038,17.9257941788656));
#36423=CARTESIAN_POINT('Ctrl Pts',(133.930267513151,36.1205283206296,17.9197641689444));
#36424=CARTESIAN_POINT('Ctrl Pts',(133.962497634803,36.0006184357189,17.9137341590232));
#36425=CARTESIAN_POINT('Ctrl Pts',(133.989213388344,35.879432511484,17.907704149102));
#36426=CARTESIAN_POINT('Ctrl Pts',(134.014931363188,35.7627726334056,17.9018993477056));
#36427=CARTESIAN_POINT('Ctrl Pts',(134.03553938943,35.6449307561636,17.8960945463092));
#36428=CARTESIAN_POINT('Ctrl Pts',(134.05094274229,35.5263913930623,17.8902897449128));
#36429=CARTESIAN_POINT('Ctrl Pts',(134.06634380127,35.407869682942,17.8844858079723));
#36430=CARTESIAN_POINT('Ctrl Pts',(134.0765416757,35.2886510982102,17.8786818710318));
#36431=CARTESIAN_POINT('Ctrl Pts',(134.081493234088,35.1692275984909,17.8728779340913));
#36432=CARTESIAN_POINT('Ctrl Pts',(134.086445222649,35.0497937237118,17.8670734929268));
#36433=CARTESIAN_POINT('Ctrl Pts',(134.086149972063,34.9301553064141,17.8612690517624));
#36434=CARTESIAN_POINT('Ctrl Pts',(134.080616452514,34.8108060057166,17.8554646105979));
#36435=CARTESIAN_POINT('Ctrl Pts',(134.075081147455,34.691418194388,17.849658296505));
#36436=CARTESIAN_POINT('Ctrl Pts',(134.064304230807,34.5723200927413,17.8438519824122));
#36437=CARTESIAN_POINT('Ctrl Pts',(134.048346626875,34.4540012924314,17.8380456683193));
#36438=CARTESIAN_POINT('Ctrl Pts',(134.032371403262,34.3355518497259,17.8322329431507));
#36439=CARTESIAN_POINT('Ctrl Pts',(134.011204128747,34.2178838307071,17.8264202179822));
#36440=CARTESIAN_POINT('Ctrl Pts',(133.98495707752,34.1014778298091,17.8206074928137));
#36441=CARTESIAN_POINT('Ctrl Pts',(133.958692832105,33.9849955724731,17.8147909597854));
#36442=CARTESIAN_POINT('Ctrl Pts',(133.927342289602,33.8697773727218,17.8089744267572));
#36443=CARTESIAN_POINT('Ctrl Pts',(133.891067468789,33.7562882354296,17.803157893729));
#36444=CARTESIAN_POINT('Ctrl Pts',(133.854740822545,33.642636957475,17.797333050685));
#36445=CARTESIAN_POINT('Ctrl Pts',(133.813475996655,33.5307200542088,17.7915082076411));
#36446=CARTESIAN_POINT('Ctrl Pts',(133.767482984804,33.4209822802718,17.7856833645971));
#36447=CARTESIAN_POINT('Ctrl Pts',(133.755350967756,33.3920356970721,17.7841468899836));
#36448=CARTESIAN_POINT('Ctrl Pts',(133.742890211318,33.3632406005495,17.7826104153701));
#36449=CARTESIAN_POINT('Ctrl Pts',(133.730105090453,33.3346048474387,17.7810739407566));
#36450=CARTESIAN_POINT('Ctrl Pts',(133.681642154084,33.2260589294508,17.7752498212811));
#36451=CARTESIAN_POINT('Ctrl Pts',(133.628359295553,33.1194555429994,17.7694257018056));
#36452=CARTESIAN_POINT('Ctrl Pts',(133.570434327724,33.0152522297759,17.76360158233));
#36453=CARTESIAN_POINT('Ctrl Pts',(133.512582326264,32.9111801783859,17.7577847993257));
#36454=CARTESIAN_POINT('Ctrl Pts',(133.450100042775,32.8095025405984,17.7519680163213));
#36455=CARTESIAN_POINT('Ctrl Pts',(133.383213095,32.7106563923645,17.7461512333169));
#36456=CARTESIAN_POINT('Ctrl Pts',(133.316392979415,32.6119090093582,17.7403402623336));
#36457=CARTESIAN_POINT('Ctrl Pts',(133.245177182433,32.5159878237591,17.7345292913504));
#36458=CARTESIAN_POINT('Ctrl Pts',(133.169836623754,32.4233042906255,17.7287183203671));
#36459=CARTESIAN_POINT('Ctrl Pts',(133.091654233912,32.3271247527196,17.722688160693));
#36460=CARTESIAN_POINT('Ctrl Pts',(133.009030002331,32.2344323156608,17.7166580010188));
#36461=CARTESIAN_POINT('Ctrl Pts',(132.922315528805,32.1456529730768,17.7106278413447));
#36462=CARTESIAN_POINT('Ctrl Pts',(132.838846755965,32.0601966187024,17.7048233890133));
#36463=CARTESIAN_POINT('Ctrl Pts',(132.751588742913,31.9783660088873,17.6990189366818));
#36464=CARTESIAN_POINT('Ctrl Pts',(132.660894819584,31.9005058865823,17.6932144843504));
#36465=CARTESIAN_POINT('Ctrl Pts',(132.570214184431,31.8226571720872,17.6874108824682));
#36466=CARTESIAN_POINT('Ctrl Pts',(132.476098949816,31.748778054045,17.6816072805861));
#36467=CARTESIAN_POINT('Ctrl Pts',(132.378936948102,31.6791741995469,17.675803678704));
#36468=CARTESIAN_POINT('Ctrl Pts',(132.281766265341,31.6095641262146,17.6699995582926));
#36469=CARTESIAN_POINT('Ctrl Pts',(132.18154860613,31.5442303136562,17.6641954378812));
#36470=CARTESIAN_POINT('Ctrl Pts',(132.078701776204,31.4834357782623,17.6583913174697));
#36471=CARTESIAN_POINT('Ctrl Pts',(131.975821499723,31.4226214720326,17.6525853095151));
#36472=CARTESIAN_POINT('Ctrl Pts',(131.870310703314,31.3663495864621,17.6467793015605));
#36473=CARTESIAN_POINT('Ctrl Pts',(131.762612260656,31.3148374501812,17.6409732936059));
#36474=CARTESIAN_POINT('Ctrl Pts',(131.654794468821,31.2632682292214,17.6351608515539));
#36475=CARTESIAN_POINT('Ctrl Pts',(131.544784560114,31.21646946248,17.6293484095019));
#36476=CARTESIAN_POINT('Ctrl Pts',(131.433046022634,31.1746105953755,17.6235359674499));
#36477=CARTESIAN_POINT('Ctrl Pts',(131.321234031561,31.1327242114963,17.6177197044713));
#36478=CARTESIAN_POINT('Ctrl Pts',(131.207691535957,31.0957843204613,17.6119034414927));
#36479=CARTESIAN_POINT('Ctrl Pts',(131.092896241219,31.0639102136854,17.6060871785142));
#36480=CARTESIAN_POINT('Ctrl Pts',(130.97793651638,31.0319904511829,17.6002625844562));
#36481=CARTESIAN_POINT('Ctrl Pts',(130.861720807078,31.0051510472991,17.5944379903983));
#36482=CARTESIAN_POINT('Ctrl Pts',(130.744736168808,30.9834600663171,17.5886133963404));
#36483=CARTESIAN_POINT('Ctrl Pts',(130.71381319552,30.9777264107243,17.5870737602896));
#36484=CARTESIAN_POINT('Ctrl Pts',(130.682836516287,30.9723522053115,17.5855341242389));
#36485=CARTESIAN_POINT('Ctrl Pts',(130.651815156237,30.9673380997039,17.5839944881881));
#36486=CARTESIAN_POINT('Ctrl Pts',(130.534583178963,30.9483894297009,17.5781760915022));
#36487=CARTESIAN_POINT('Ctrl Pts',(130.416333096405,30.9345261234571,17.5723576948162));
#36488=CARTESIAN_POINT('Ctrl Pts',(130.297544102524,30.9258507014282,17.5665392981303));
#36489=CARTESIAN_POINT('Ctrl Pts',(130.178905374958,30.9171862536794,17.5607282616298));
#36490=CARTESIAN_POINT('Ctrl Pts',(130.059729496346,30.9136966673801,17.5549172251293));
#36491=CARTESIAN_POINT('Ctrl Pts',(129.940504821447,30.9154332758873,17.5491061886289));
#36492=CARTESIAN_POINT('Ctrl Pts',(129.821399734198,30.9171681424989,17.5433009808564));
#36493=CARTESIAN_POINT('Ctrl Pts',(129.702246354756,30.9241187699002,17.5374957730839));
#36494=CARTESIAN_POINT('Ctrl Pts',(129.583536504175,30.9362845625406,17.5316905653114));
#36495=CARTESIAN_POINT('Ctrl Pts',(129.460182596709,30.948926294059,17.5256582515742));
#36496=CARTESIAN_POINT('Ctrl Pts',(129.337308077732,30.9671995934947,17.519625937837));
#36497=CARTESIAN_POINT('Ctrl Pts',(129.215463336517,30.9910441230102,17.5135936240999));
#36498=CARTESIAN_POINT('Ctrl Pts',(129.09833760526,31.0139651611128,17.5077949400484));
#36499=CARTESIAN_POINT('Ctrl Pts',(128.982163809782,31.0420338337901,17.501996255997));
#36500=CARTESIAN_POINT('Ctrl Pts',(128.867423224995,31.0751439709566,17.4961975719455));
#36501=CARTESIAN_POINT('Ctrl Pts',(128.75269930978,31.108249297865,17.4903997303299));
#36502=CARTESIAN_POINT('Ctrl Pts',(128.639408584219,31.1463945193783,17.4846018887143));
#36503=CARTESIAN_POINT('Ctrl Pts',(128.5280185711,31.1894231836934,17.4788040470987));
#36504=CARTESIAN_POINT('Ctrl Pts',(128.416618323132,31.2324558016114,17.47300567276));
#36505=CARTESIAN_POINT('Ctrl Pts',(128.30711951653,31.2803726070192,17.4672072984214));
#36506=CARTESIAN_POINT('Ctrl Pts',(128.199970437257,31.3329686975358,17.4614089240827));
#36507=CARTESIAN_POINT('Ctrl Pts',(128.092786100998,31.3855820945907,17.4556086418115));
#36508=CARTESIAN_POINT('Ctrl Pts',(127.987953396773,31.4428776585701,17.4498083595403));
#36509=CARTESIAN_POINT('Ctrl Pts',(127.885896133519,31.5046044799294,17.4440080772692));
#36510=CARTESIAN_POINT('Ctrl Pts',(127.783724623509,31.5664004006247,17.4382013019429));
#36511=CARTESIAN_POINT('Ctrl Pts',(127.684335106399,31.6326372683155,17.4323945266166));
#36512=CARTESIAN_POINT('Ctrl Pts',(127.588122632924,31.7030206906646,17.4265877512904));
#36513=CARTESIAN_POINT('Ctrl Pts',(127.491846393153,31.7734507607088,17.4207771274345));
#36514=CARTESIAN_POINT('Ctrl Pts',(127.398751708728,31.8480326029509,17.4149665035786));
#36515=CARTESIAN_POINT('Ctrl Pts',(127.309199450961,31.9264324628711,17.4091558797227));
#36516=CARTESIAN_POINT('Ctrl Pts',(127.219517508456,32.0049458572306,17.4033368412354));
#36517=CARTESIAN_POINT('Ctrl Pts',(127.133388526181,32.0872880230325,17.3975178027482));
#36518=CARTESIAN_POINT('Ctrl Pts',(127.051135632554,32.1730893288947,17.3916987642609));
#36519=CARTESIAN_POINT('Ctrl Pts',(127.028596082769,32.1966012409975,17.3901041880472));
#36520=CARTESIAN_POINT('Ctrl Pts',(127.006347352703,32.220372719968,17.3885096118334));
#36521=CARTESIAN_POINT('Ctrl Pts',(126.984395538433,32.244395759298,17.3869150356197));
#36522=CARTESIAN_POINT('Ctrl Pts',(126.904949793899,32.3313374681727,17.3811441096744));
#36523=CARTESIAN_POINT('Ctrl Pts',(126.829126556866,32.4218715866098,17.3753731837292));
#36524=CARTESIAN_POINT('Ctrl Pts',(126.757272073936,32.5156609334618,17.3696022577839));
#36525=CARTESIAN_POINT('Ctrl Pts',(126.685531583472,32.609301489613,17.3638404870374));
#36526=CARTESIAN_POINT('Ctrl Pts',(126.617747567003,32.7061866680698,17.358078716291));
#36527=CARTESIAN_POINT('Ctrl Pts',(126.554228459588,32.8059435988822,17.3523169455445));
#36528=CARTESIAN_POINT('Ctrl Pts',(126.490767188589,32.9056096974456,17.3465604210962));
#36529=CARTESIAN_POINT('Ctrl Pts',(126.431563330612,33.0081420020447,17.3408038966478));
#36530=CARTESIAN_POINT('Ctrl Pts',(126.376884074655,33.1131359371927,17.3350473721994));
#36531=CARTESIAN_POINT('Ctrl Pts',(126.322241085739,33.2180602331461,17.3292946658737));
#36532=CARTESIAN_POINT('Ctrl Pts',(126.272116924162,33.325442545264,17.323541959548));
#36533=CARTESIAN_POINT('Ctrl Pts',(126.226734181323,33.4348514250694,17.3177892532224));
#36534=CARTESIAN_POINT('Ctrl Pts',(126.181370319882,33.5442147855327,17.3120389402985));
#36535=CARTESIAN_POINT('Ctrl Pts',(126.140744112726,33.6556026522314,17.3062886273746));
#36536=CARTESIAN_POINT('Ctrl Pts',(126.105030784296,33.7685618940773,17.3005383144507));
#36537=CARTESIAN_POINT('Ctrl Pts',(126.069314310588,33.8815310842595,17.2947874950959));
#36538=CARTESIAN_POINT('Ctrl Pts',(126.038511715076,33.9960715316613,17.2890366757411));
#36539=CARTESIAN_POINT('Ctrl Pts',(126.012748796744,34.1117135359975,17.2832858563864));
#36540=CARTESIAN_POINT('Ctrl Pts',(125.986984894525,34.2273599567015,17.2775348174078));
#36541=CARTESIAN_POINT('Ctrl Pts',(125.966261135726,34.3441076095336,17.2717837784293));
#36542=CARTESIAN_POINT('Ctrl Pts',(125.950652243617,34.4614763256111,17.2660327394508));
#36543=CARTESIAN_POINT('Ctrl Pts',(125.935032726191,34.5789249371669,17.2602777856129));
#36544=CARTESIAN_POINT('Ctrl Pts',(125.924535074559,34.696995041783,17.2545228317751));
#36545=CARTESIAN_POINT('Ctrl Pts',(125.919182137792,34.8152012568155,17.2487678779372));
#36546=CARTESIAN_POINT('Ctrl Pts',(125.916344314637,34.8778674807292,17.2457169281566));
#36547=CARTESIAN_POINT('Ctrl Pts',(125.914951543149,34.9405719254792,17.2426659783761));
#36548=CARTESIAN_POINT('Ctrl Pts',(125.9150012868,35.0032424000665,17.2396150285955));
#36549=CARTESIAN_POINT('Origin',(130.,35.,32.7603849714045));
#36550=CARTESIAN_POINT('',(132.487160689988,38.2405642567579,19.2967873935987));
#36551=CARTESIAN_POINT('',(132.487160689988,38.2405642567579,19.1927515487681));
#36552=CARTESIAN_POINT('',(132.487160689988,38.2405642567579,32.7603849714045));
#36553=CARTESIAN_POINT('',(125.915000065372,35.0007308119611,18.3853849714449));
#36554=CARTESIAN_POINT('Ctrl Pts',(132.487160689988,38.2405642567579,19.1927515487681));
#36555=CARTESIAN_POINT('Ctrl Pts',(132.581827195764,38.1679069066276,19.186927974649));
#36556=CARTESIAN_POINT('Ctrl Pts',(132.673193347444,38.0911853678094,19.1811044005299));
#36557=CARTESIAN_POINT('Ctrl Pts',(132.760910624345,38.0107470043793,19.1752808264108));
#36558=CARTESIAN_POINT('Ctrl Pts',(132.798099043779,37.9766445367301,19.1728118770248));
#36559=CARTESIAN_POINT('Ctrl Pts',(132.834632090439,37.9418744364773,19.1703429276389));
#36560=CARTESIAN_POINT('Ctrl Pts',(132.870485381438,37.9064649791367,19.1678739782529));
#36561=CARTESIAN_POINT('Ctrl Pts',(132.955052702871,37.8229445301852,19.1620504560461));
#36562=CARTESIAN_POINT('Ctrl Pts',(133.03610818715,37.7355954240947,19.1562269338393));
#36563=CARTESIAN_POINT('Ctrl Pts',(133.113286014791,37.6447448251409,19.1504034116324));
#36564=CARTESIAN_POINT('Ctrl Pts',(133.190366468885,37.5540088503632,19.1445872368338));
#36565=CARTESIAN_POINT('Ctrl Pts',(133.263578735065,37.4597804779985,19.1387710620352));
#36566=CARTESIAN_POINT('Ctrl Pts',(133.332592949286,37.3624244399279,19.1329548872366));
#36567=CARTESIAN_POINT('Ctrl Pts',(133.401538079113,37.2651658568956,19.1271445345271));
#36568=CARTESIAN_POINT('Ctrl Pts',(133.466293282176,37.164786167805,19.1213341818177));
#36569=CARTESIAN_POINT('Ctrl Pts',(133.526568598092,37.0616835166802,19.1155238291083));
#36570=CARTESIAN_POINT('Ctrl Pts',(133.589126507816,36.9546764235892,19.1094934414656));
#36571=CARTESIAN_POINT('Ctrl Pts',(133.646858231296,36.8447363991944,19.103463053823));
#36572=CARTESIAN_POINT('Ctrl Pts',(133.699488436065,36.7323424348039,19.0974326661803));
#36573=CARTESIAN_POINT('Ctrl Pts',(133.750141212168,36.6241713505636,19.0916288530198));
#36574=CARTESIAN_POINT('Ctrl Pts',(133.796068714334,36.513727802009,19.0858250398592));
#36575=CARTESIAN_POINT('Ctrl Pts',(133.837072404662,36.4014636496815,19.0800212266986));
#36576=CARTESIAN_POINT('Ctrl Pts',(133.878070040312,36.2892160744815,19.0742182705396));
#36577=CARTESIAN_POINT('Ctrl Pts',(133.914145169957,36.1751488135945,19.0684153143806));
#36578=CARTESIAN_POINT('Ctrl Pts',(133.945147964157,36.0597322968145,19.0626123582216));
#36579=CARTESIAN_POINT('Ctrl Pts',(133.976153497589,35.9443055824762,19.0568088893458));
#36580=CARTESIAN_POINT('Ctrl Pts',(134.00208569858,35.8275297696088,19.05100542047));
#36581=CARTESIAN_POINT('Ctrl Pts',(134.022845201741,35.709888359414,19.0452019515942));
#36582=CARTESIAN_POINT('Ctrl Pts',(134.043611438645,35.5922087899689,19.0393966002519));
#36583=CARTESIAN_POINT('Ctrl Pts',(134.059201569904,35.4736634667302,19.0335912489095));
#36584=CARTESIAN_POINT('Ctrl Pts',(134.06956781371,35.3547433010181,19.0277858975672));
#36585=CARTESIAN_POINT('Ctrl Pts',(134.079945539115,35.2356914199295,19.0219741162469));
#36586=CARTESIAN_POINT('Ctrl Pts',(134.085087792334,35.1162642746923,19.0161623349267));
#36587=CARTESIAN_POINT('Ctrl Pts',(134.084998865295,34.996955244281,19.0103505536064));
#36588=CARTESIAN_POINT('Ctrl Pts',(134.08490987984,34.8775678396986,19.0045349545236));
#36589=CARTESIAN_POINT('Ctrl Pts',(134.079582888704,34.758299111467,18.9987193554409));
#36590=CARTESIAN_POINT('Ctrl Pts',(134.069074134723,34.6396381178254,18.9929037563581));
#36591=CARTESIAN_POINT('Ctrl Pts',(134.058550325626,34.5208071273265,18.9870798256953));
#36592=CARTESIAN_POINT('Ctrl Pts',(134.042829990362,34.4025860125479,18.9812558950325));
#36593=CARTESIAN_POINT('Ctrl Pts',(134.022020616267,34.2854545764428,18.9754319643697));
#36594=CARTESIAN_POINT('Ctrl Pts',(134.016497302086,34.2543650434737,18.9738861514746));
#36595=CARTESIAN_POINT('Ctrl Pts',(134.010615737949,34.22335219832,18.9723403385795));
#36596=CARTESIAN_POINT('Ctrl Pts',(134.004378520531,34.1924248243584,18.9707945256844));
#36597=CARTESIAN_POINT('Ctrl Pts',(133.980880488013,34.0759093351174,18.9649708451492));
#36598=CARTESIAN_POINT('Ctrl Pts',(133.952254965815,33.9602324116435,18.9591471646139));
#36599=CARTESIAN_POINT('Ctrl Pts',(133.918575070159,33.8458793739264,18.9533234840787));
#36600=CARTESIAN_POINT('Ctrl Pts',(133.884937668285,33.7316706149524,18.9475071512565));
#36601=CARTESIAN_POINT('Ctrl Pts',(133.846258691171,33.6187828077004,18.9416908184343));
#36602=CARTESIAN_POINT('Ctrl Pts',(133.802662384732,33.5076917919737,18.9358744856121));
#36603=CARTESIAN_POINT('Ctrl Pts',(133.759109721393,33.3967119864997,18.9300639753656));
#36604=CARTESIAN_POINT('Ctrl Pts',(133.710649669962,33.2875257721358,18.9242534651191));
#36605=CARTESIAN_POINT('Ctrl Pts',(133.657456294753,33.180593928785,18.9184429548725));
#36606=CARTESIAN_POINT('Ctrl Pts',(133.602250554129,33.0696167331239,18.912412626466));
#36607=CARTESIAN_POINT('Ctrl Pts',(133.541946410013,32.9610682776073,18.9063822980595));
#36608=CARTESIAN_POINT('Ctrl Pts',(133.476793536316,32.8554413727221,18.900351969653));
#36609=CARTESIAN_POINT('Ctrl Pts',(133.414086300286,32.7537793756406,18.8945480011515));
#36610=CARTESIAN_POINT('Ctrl Pts',(133.346888019939,32.6548239292565,18.88874403265));
#36611=CARTESIAN_POINT('Ctrl Pts',(133.275467798784,32.5589887957797,18.8829400641485));
#36612=CARTESIAN_POINT('Ctrl Pts',(133.204058136611,32.4631678308599,18.8771369537233));
#36613=CARTESIAN_POINT('Ctrl Pts',(133.128428018869,32.3704665887504,18.8713338432981));
#36614=CARTESIAN_POINT('Ctrl Pts',(133.048888780157,32.281268272478,18.8655307328729));
#36615=CARTESIAN_POINT('Ctrl Pts',(132.96934253096,32.1920620943829,18.8597271109692));
#36616=CARTESIAN_POINT('Ctrl Pts',(132.885886747526,32.106359760753,18.8539234890655));
#36617=CARTESIAN_POINT('Ctrl Pts',(132.798871359905,32.024509433605,18.8481198671618));
#36618=CARTESIAN_POINT('Ctrl Pts',(132.711827768946,31.9426325772144,18.8423143641942));
#36619=CARTESIAN_POINT('Ctrl Pts',(132.621222576549,31.8646104899304,18.8365088612266));
#36620=CARTESIAN_POINT('Ctrl Pts',(132.527440187252,31.7907522532745,18.830703358259));
#36621=CARTESIAN_POINT('Ctrl Pts',(132.433553973492,31.7168122497553,18.824891428144));
#36622=CARTESIAN_POINT('Ctrl Pts',(132.336483862763,31.647045551026,18.8190794980291));
#36623=CARTESIAN_POINT('Ctrl Pts',(132.236644869113,31.581719038834,18.8132675679142));
#36624=CARTESIAN_POINT('Ctrl Pts',(132.136740318165,31.5163496312816,18.8074518215105));
#36625=CARTESIAN_POINT('Ctrl Pts',(132.03406361379,31.4554264245687,18.8016360751068));
#36626=CARTESIAN_POINT('Ctrl Pts',(131.929054635268,31.3991704824928,18.795820328703));
#36627=CARTESIAN_POINT('Ctrl Pts',(131.823895281049,31.3428339803865,18.7899962539932));
#36628=CARTESIAN_POINT('Ctrl Pts',(131.716397353196,31.2911782593473,18.7841721792834));
#36629=CARTESIAN_POINT('Ctrl Pts',(131.607021081889,31.2443764509253,18.7783481045735));
#36630=CARTESIAN_POINT('Ctrl Pts',(131.578018265652,31.2319662248956,18.7768037607543));
#36631=CARTESIAN_POINT('Ctrl Pts',(131.548883460521,31.2198970188987,18.7752594169352));
#36632=CARTESIAN_POINT('Ctrl Pts',(131.519625410735,31.2081714686646,18.773715073116));
#36633=CARTESIAN_POINT('Ctrl Pts',(131.409293645245,31.1639545550928,18.7678913705337));
#36634=CARTESIAN_POINT('Ctrl Pts',(131.296852536977,31.124485886127,18.7620676679513));
#36635=CARTESIAN_POINT('Ctrl Pts',(131.182748083465,31.089970336294,18.756243965369));
#36636=CARTESIAN_POINT('Ctrl Pts',(131.068787563187,31.0554983249433,18.7504276089009));
#36637=CARTESIAN_POINT('Ctrl Pts',(130.953168258269,31.0259671228756,18.7446112524328));
#36638=CARTESIAN_POINT('Ctrl Pts',(130.836356263406,31.0015336439252,18.7387948959647));
#36639=CARTESIAN_POINT('Ctrl Pts',(130.719661174336,30.9771246180736,18.7329843605235));
#36640=CARTESIAN_POINT('Ctrl Pts',(130.60177616731,30.9578032490152,18.7271738250824));
#36641=CARTESIAN_POINT('Ctrl Pts',(130.483182048679,30.9436765282051,18.7213632896412));
#36642=CARTESIAN_POINT('Ctrl Pts',(130.360102095237,30.9290154627183,18.7153329700957));
#36643=CARTESIAN_POINT('Ctrl Pts',(130.236258755539,30.919949910678,18.7093026505501));
#36644=CARTESIAN_POINT('Ctrl Pts',(130.112201061256,30.9165411815652,18.7032723310045));
#36645=CARTESIAN_POINT('Ctrl Pts',(129.99279934068,30.913260384486,18.6974683336506));
#36646=CARTESIAN_POINT('Ctrl Pts',(129.873199510158,30.9152194652718,18.6916643362967));
#36647=CARTESIAN_POINT('Ctrl Pts',(129.753895146443,30.9224201539325,18.6858603389427));
#36648=CARTESIAN_POINT('Ctrl Pts',(129.634608394418,30.9296197796288,18.680057198374));
#36649=CARTESIAN_POINT('Ctrl Pts',(129.515617429928,30.9420594498307,18.6742540578052));
#36650=CARTESIAN_POINT('Ctrl Pts',(129.397413419314,30.959688822284,18.6684509172365));
#36651=CARTESIAN_POINT('Ctrl Pts',(129.27919896491,30.9773197523619,18.6626472639374));
#36652=CARTESIAN_POINT('Ctrl Pts',(129.161772006497,31.0001412361272,18.6568436106384));
#36653=CARTESIAN_POINT('Ctrl Pts',(129.045615558698,31.0280514431579,18.6510399573393));
#36654=CARTESIAN_POINT('Ctrl Pts',(128.929421438311,31.0559707022019,18.645234421763));
#36655=CARTESIAN_POINT('Ctrl Pts',(128.814499044847,31.0889818714539,18.6394288861867));
#36656=CARTESIAN_POINT('Ctrl Pts',(128.701317603836,31.1269328647837,18.6336233506104));
#36657=CARTESIAN_POINT('Ctrl Pts',(128.588010831276,31.1649258831725,18.6278113862703));
#36658=CARTESIAN_POINT('Ctrl Pts',(128.476449246677,31.2078695145774,18.6219994219301));
#36659=CARTESIAN_POINT('Ctrl Pts',(128.367083559166,31.2555629398728,18.6161874575899));
#36660=CARTESIAN_POINT('Ctrl Pts',(128.257646040819,31.3032876899708,18.6103716759807));
#36661=CARTESIAN_POINT('Ctrl Pts',(128.150407657762,31.3557682677385,18.6045558943715));
#36662=CARTESIAN_POINT('Ctrl Pts',(128.045794427749,31.4127579421815,18.5987401127623));
#36663=CARTESIAN_POINT('Ctrl Pts',(127.9410313689,31.4698292381992,18.5929160016924));
#36664=CARTESIAN_POINT('Ctrl Pts',(127.838901315844,31.5314223105997,18.5870918906226));
#36665=CARTESIAN_POINT('Ctrl Pts',(127.739801352189,31.5972471332118,18.5812677795527));
#36666=CARTESIAN_POINT('Ctrl Pts',(127.713528570899,31.6146982109336,18.579723726551));
#36667=CARTESIAN_POINT('Ctrl Pts',(127.687468578554,31.6324465008316,18.5781796735493));
#36668=CARTESIAN_POINT('Ctrl Pts',(127.661628368802,31.6504861376001,18.5766356205475));
#36669=CARTESIAN_POINT('Ctrl Pts',(127.564645396162,31.718192151442,18.5708405108539));
#36670=CARTESIAN_POINT('Ctrl Pts',(127.470441308212,31.7902284102539,18.5650454011603));
#36671=CARTESIAN_POINT('Ctrl Pts',(127.379429631301,31.8663382533056,18.5592502914667));
#36672=CARTESIAN_POINT('Ctrl Pts',(127.288533111891,31.9423517942162,18.5534625143526));
#36673=CARTESIAN_POINT('Ctrl Pts',(127.200821284793,32.0224284072574,18.5476747372384));
#36674=CARTESIAN_POINT('Ctrl Pts',(127.11667878607,32.1062681918846,18.5418869601243));
#36675=CARTESIAN_POINT('Ctrl Pts',(127.032620235032,32.1900243308401,18.5361049573869));
#36676=CARTESIAN_POINT('Ctrl Pts',(126.952124220215,32.2775358841227,18.5303229546495));
#36677=CARTESIAN_POINT('Ctrl Pts',(126.875541831694,32.368463157297,18.5245409519122));
#36678=CARTESIAN_POINT('Ctrl Pts',(126.798745363373,32.4596446102215,18.5187427860594));
#36679=CARTESIAN_POINT('Ctrl Pts',(126.725884750906,32.5542606341769,18.5129446202066));
#36680=CARTESIAN_POINT('Ctrl Pts',(126.657276560392,32.6519316436068,18.5071464543538));
#36681=CARTESIAN_POINT('Ctrl Pts',(126.588934008571,32.7492244882857,18.5013707379664));
#36682=CARTESIAN_POINT('Ctrl Pts',(126.52481124611,32.8495483631417,18.4955950215789));
#36683=CARTESIAN_POINT('Ctrl Pts',(126.465179972521,32.9524960626813,18.4898193051915));
#36684=CARTESIAN_POINT('Ctrl Pts',(126.405556689024,33.055429968092,18.4840443627017));
#36685=CARTESIAN_POINT('Ctrl Pts',(126.350423904548,33.1609866418927,18.4782694202119));
#36686=CARTESIAN_POINT('Ctrl Pts',(126.300008551479,33.268732175292,18.4724944777221));
#36687=CARTESIAN_POINT('Ctrl Pts',(126.249587741316,33.3764893713586,18.4667189101369));
#36688=CARTESIAN_POINT('Ctrl Pts',(126.203885552365,33.4864355239355,18.4609433425517));
#36689=CARTESIAN_POINT('Ctrl Pts',(126.163081447441,33.5981151898151,18.4551677749666));
#36690=CARTESIAN_POINT('Ctrl Pts',(126.121997103856,33.7105618608782,18.4493525413398));
#36691=CARTESIAN_POINT('Ctrl Pts',(126.08587853268,33.8247655513889,18.443537307713));
#36692=CARTESIAN_POINT('Ctrl Pts',(126.054858023747,33.9402454118026,18.4377220740862));
#36693=CARTESIAN_POINT('Ctrl Pts',(126.02400421083,34.0551047139662,18.431938089988));
#36694=CARTESIAN_POINT('Ctrl Pts',(125.998193836137,34.1712260861413,18.4261541058898));
#36695=CARTESIAN_POINT('Ctrl Pts',(125.977505562765,34.2881267652104,18.4203701217916));
#36696=CARTESIAN_POINT('Ctrl Pts',(125.956649628456,34.4059748252858,18.4145392634005));
#36697=CARTESIAN_POINT('Ctrl Pts',(125.940999236854,34.5246144548944,18.4087084050094));
#36698=CARTESIAN_POINT('Ctrl Pts',(125.930581533309,34.6435475586353,18.4028775466183));
#36699=CARTESIAN_POINT('Ctrl Pts',(125.920163829764,34.7624806623761,18.3970466882272));
#36700=CARTESIAN_POINT('Ctrl Pts',(125.914978771819,34.8817068147453,18.3912158298361));
#36701=CARTESIAN_POINT('Ctrl Pts',(125.915000065372,35.0007308119611,18.3853849714449));
#36702=CARTESIAN_POINT('Ctrl Pts',(125.915000065372,35.0007308127869,18.3853849714045));
#36703=CARTESIAN_POINT('Ctrl Pts',(125.915007160729,35.040391496008,18.3834420369294));
#36704=CARTESIAN_POINT('Ctrl Pts',(125.915591831772,35.0800463838246,18.3814991024543));
#36705=CARTESIAN_POINT('Ctrl Pts',(125.916753658372,35.119684224453,18.3795561679791));
#36706=CARTESIAN_POINT('Ctrl Pts',(125.920236583737,35.2385105970872,18.3737316363627));
#36707=CARTESIAN_POINT('Ctrl Pts',(125.928916363599,35.3573761657475,18.3679071047463));
#36708=CARTESIAN_POINT('Ctrl Pts',(125.942802843878,35.4757901179652,18.3620825731299));
#36709=CARTESIAN_POINT('Ctrl Pts',(125.956671800716,35.5940546428387,18.3562653915282));
#36710=CARTESIAN_POINT('Ctrl Pts',(125.975734342444,35.7118682829417,18.3504482099265));
#36711=CARTESIAN_POINT('Ctrl Pts',(125.999948318737,35.8287409409616,18.3446310283248));
#36712=CARTESIAN_POINT('Ctrl Pts',(126.024138044988,35.9454965522483,18.338819672569));
#36713=CARTESIAN_POINT('Ctrl Pts',(126.053468859994,36.061312658808,18.3330083168133));
#36714=CARTESIAN_POINT('Ctrl Pts',(126.087846967805,36.1757055977941,18.3271969610575));
#36715=CARTESIAN_POINT('Ctrl Pts',(126.12351856505,36.2944026147938,18.3211669508223));
#36716=CARTESIAN_POINT('Ctrl Pts',(126.164624676602,36.4115668212268,18.315136940587));
#36717=CARTESIAN_POINT('Ctrl Pts',(126.211002489441,36.5266705161822,18.3091069303517));
#36718=CARTESIAN_POINT('Ctrl Pts',(126.255648177386,36.6374753026025,18.303302129763));
#36719=CARTESIAN_POINT('Ctrl Pts',(126.305178684521,36.7463703179019,18.2974973291744));
#36720=CARTESIAN_POINT('Ctrl Pts',(126.359398611619,36.8529021914066,18.2916925285857));
#36721=CARTESIAN_POINT('Ctrl Pts',(126.413610464331,36.9594182002729,18.2858885924432));
#36722=CARTESIAN_POINT('Ctrl Pts',(126.4725101631,37.0635714035169,18.2800846563006));
#36723=CARTESIAN_POINT('Ctrl Pts',(126.535855522528,37.1649314167436,18.2742807201581));
#36724=CARTESIAN_POINT('Ctrl Pts',(126.599206385276,37.2663002359281,18.268476279781));
#36725=CARTESIAN_POINT('Ctrl Pts',(126.667003460254,37.3648750364461,18.2626718394039));
#36726=CARTESIAN_POINT('Ctrl Pts',(126.738960601225,37.4602534502846,18.2568673990269));
#36727=CARTESIAN_POINT('Ctrl Pts',(126.810940960867,37.5556626402207,18.25106108571));
#36728=CARTESIAN_POINT('Ctrl Pts',(126.887083810414,37.6478730665739,18.2452547723932));
#36729=CARTESIAN_POINT('Ctrl Pts',(126.967062420869,37.7365150540593,18.2394484590764));
#36730=CARTESIAN_POINT('Ctrl Pts',(127.047129340469,37.8252549164404,18.2336357346633));
#36731=CARTESIAN_POINT('Ctrl Pts',(127.131040201393,37.9104181718577,18.2278230102503));
#36732=CARTESIAN_POINT('Ctrl Pts',(127.218430974147,37.991671565265,18.2220102858372));
#36733=CARTESIAN_POINT('Ctrl Pts',(127.305878995919,38.0729781871409,18.2161937535535));
#36734=CARTESIAN_POINT('Ctrl Pts',(127.39681115944,38.1503695820478,18.2103772212697));
#36735=CARTESIAN_POINT('Ctrl Pts',(127.490831181968,38.2235534496289,18.2045606889859));
#36736=CARTESIAN_POINT('Ctrl Pts',(127.58498553022,38.2968418744708,18.1987358466646));
#36737=CARTESIAN_POINT('Ctrl Pts',(127.6822362112,38.365910538259,18.1929110043434));
#36738=CARTESIAN_POINT('Ctrl Pts',(127.782158781132,38.4305109426864,18.1870861620221));
#36739=CARTESIAN_POINT('Ctrl Pts',(127.808516447484,38.4475512961048,18.1855496798183));
#36740=CARTESIAN_POINT('Ctrl Pts',(127.83505989868,38.4642809979911,18.1840131976145));
#36741=CARTESIAN_POINT('Ctrl Pts',(127.861781087519,38.4806960341731,18.1824767154107));
#36742=CARTESIAN_POINT('Ctrl Pts',(127.96306915626,38.5429180903552,18.1766525989758));
#36743=CARTESIAN_POINT('Ctrl Pts',(128.067238419904,38.6008153648951,18.1708284825408));
#36744=CARTESIAN_POINT('Ctrl Pts',(128.173883774923,38.6541106349578,18.1650043661059));
#36745=CARTESIAN_POINT('Ctrl Pts',(128.280394791564,38.7073387703559,18.1591875861589));
#36746=CARTESIAN_POINT('Ctrl Pts',(128.389375333819,38.7559762505954,18.1533708062119));
#36747=CARTESIAN_POINT('Ctrl Pts',(128.500392399092,38.799789736722,18.1475540262648));
#36748=CARTESIAN_POINT('Ctrl Pts',(128.611298537879,38.8435594451104,18.1417430583518));
#36749=CARTESIAN_POINT('Ctrl Pts',(128.724236773994,38.8825145993402,18.1359320904387));
#36750=CARTESIAN_POINT('Ctrl Pts',(128.838751182359,38.9164685857959,18.1301211225256));
#36751=CARTESIAN_POINT('Ctrl Pts',(128.957585137217,38.9517033353034,18.1240909617055));
#36752=CARTESIAN_POINT('Ctrl Pts',(129.07811611319,38.981551993627,18.1180608008853));
#36753=CARTESIAN_POINT('Ctrl Pts',(129.19981338699,39.0058615033922,18.1120306400652));
#36754=CARTESIAN_POINT('Ctrl Pts',(129.316955478314,39.0292610975165,18.1062261908164));
#36755=CARTESIAN_POINT('Ctrl Pts',(129.435177690273,39.0475286695622,18.1004217415676));
#36756=CARTESIAN_POINT('Ctrl Pts',(129.55399375061,39.0605791982801,18.0946172923188));
#36757=CARTESIAN_POINT('Ctrl Pts',(129.672792402414,39.073627814878,18.0888136935185));
#36758=CARTESIAN_POINT('Ctrl Pts',(129.79218432387,39.0814608637114,18.0830100947182));
#36759=CARTESIAN_POINT('Ctrl Pts',(129.911676830767,39.0840450557966,18.0772064959179));
#36760=CARTESIAN_POINT('Ctrl Pts',(130.031180013947,39.0866294787713,18.0714023785842));
#36761=CARTESIAN_POINT('Ctrl Pts',(130.150783392269,39.0839641037346,18.0655982612505));
#36762=CARTESIAN_POINT('Ctrl Pts',(130.269993626076,39.0760677670861,18.0597941439168));
#36763=CARTESIAN_POINT('Ctrl Pts',(130.389242628115,39.0681688624785,18.0539881390323));
#36764=CARTESIAN_POINT('Ctrl Pts',(130.508097824223,39.0550356399889,18.0481821341479));
#36765=CARTESIAN_POINT('Ctrl Pts',(130.62607098278,39.0367387981539,18.0423761292634));
#36766=CARTESIAN_POINT('Ctrl Pts',(130.744174877349,39.0184216800444,18.036563690255));
#36767=CARTESIAN_POINT('Ctrl Pts',(130.861394379612,38.994929583096,18.0307512512465));
#36768=CARTESIAN_POINT('Ctrl Pts',(130.977251281277,38.9663843652933,18.0249388122381));
#36769=CARTESIAN_POINT('Ctrl Pts',(131.093184344101,38.9378203826447,18.0191225522911));
#36770=CARTESIAN_POINT('Ctrl Pts',(131.207752631618,38.9041967783932,18.0133062923442));
#36771=CARTESIAN_POINT('Ctrl Pts',(131.320494520823,38.8656848320156,18.0074900323972));
#36772=CARTESIAN_POINT('Ctrl Pts',(131.433397899752,38.827117721727,18.0016654413302));
#36773=CARTESIAN_POINT('Ctrl Pts',(131.544469279945,38.7836484419674,17.9958408502633));
#36774=CARTESIAN_POINT('Ctrl Pts',(131.653268246692,38.7354958311422,17.9900162591963));
#36775=CARTESIAN_POINT('Ctrl Pts',(131.682028035717,38.7227672274637,17.988476593745));
#36776=CARTESIAN_POINT('Ctrl Pts',(131.710629181738,38.7097116203617,17.9869369282936));
#36777=CARTESIAN_POINT('Ctrl Pts',(131.739063868762,38.6963335699539,17.9853972628422));
#36778=CARTESIAN_POINT('Ctrl Pts',(131.846528305251,38.6457733282606,17.9795783389351));
#36779=CARTESIAN_POINT('Ctrl Pts',(131.951961213614,38.5904402353699,17.9737594150281));
#36780=CARTESIAN_POINT('Ctrl Pts',(132.054909090144,38.5305203060235,17.967940491121));
#36781=CARTESIAN_POINT('Ctrl Pts',(132.157711917597,38.4706848012496,17.9621297658244));
#36782=CARTESIAN_POINT('Ctrl Pts',(132.258036329994,38.4062755242499,17.9563190405279));
#36783=CARTESIAN_POINT('Ctrl Pts',(132.355450358798,38.3375258212094,17.9505083152313));
#36784=CARTESIAN_POINT('Ctrl Pts',(132.399974678273,38.3061028959946,17.9478524494114));
#36785=CARTESIAN_POINT('Ctrl Pts',(132.443891305796,38.2737738779582,17.9451965835914));
#36786=CARTESIAN_POINT('Ctrl Pts',(132.487160689988,38.2405642567579,17.9425407177715));
#36787=CARTESIAN_POINT('',(125.915000466471,34.998047803468,18.4896150286331));
#36788=CARTESIAN_POINT('Ctrl Pts',(125.915000466471,34.9980478042441,18.4896150285955));
#36789=CARTESIAN_POINT('Ctrl Pts',(125.914942432928,35.1194838827728,18.483727517173));
#36790=CARTESIAN_POINT('Ctrl Pts',(125.920303700289,35.2409117170285,18.4778400057506));
#36791=CARTESIAN_POINT('Ctrl Pts',(125.931055605702,35.3618238744374,18.4719524943281));
#36792=CARTESIAN_POINT('Ctrl Pts',(125.941810869906,35.482773803618,18.4660631437048));
#36793=CARTESIAN_POINT('Ctrl Pts',(125.957960090728,35.6032073451722,18.4601737930816));
#36794=CARTESIAN_POINT('Ctrl Pts',(125.979422790103,35.7226229302054,18.4542844424583));
#36795=CARTESIAN_POINT('Ctrl Pts',(126.000896649805,35.8421006098063,18.4483920294485));
#36796=CARTESIAN_POINT('Ctrl Pts',(126.027689420367,35.9605588938576,18.4424996164387));
#36797=CARTESIAN_POINT('Ctrl Pts',(126.059669749903,36.0775075499385,18.4366072034289));
#36798=CARTESIAN_POINT('Ctrl Pts',(126.091695456131,36.1946221437388,18.430706429711));
#36799=CARTESIAN_POINT('Ctrl Pts',(126.128923319468,36.3102224531799,18.424805655993));
#36800=CARTESIAN_POINT('Ctrl Pts',(126.171172255081,36.4238339438785,18.4189048822751));
#36801=CARTESIAN_POINT('Ctrl Pts',(126.213453803262,36.5375331329366,18.4129995536643));
#36802=CARTESIAN_POINT('Ctrl Pts',(126.260763995858,36.6492400836464,18.4070942250534));
#36803=CARTESIAN_POINT('Ctrl Pts',(126.312874497657,36.75850235427,18.4011888964426));
#36804=CARTESIAN_POINT('Ctrl Pts',(126.365076841081,36.8679571930732,18.3952731600453));
#36805=CARTESIAN_POINT('Ctrl Pts',(126.422096212423,36.9749583984458,18.389357423648));
#36806=CARTESIAN_POINT('Ctrl Pts',(126.483659079887,37.0790794918762,18.3834416872507));
#36807=CARTESIAN_POINT('Ctrl Pts',(126.522265549195,37.1443744978332,18.3797318909878));
#36808=CARTESIAN_POINT('Ctrl Pts',(126.562657939128,37.2085374477177,18.3760220947248));
#36809=CARTESIAN_POINT('Ctrl Pts',(126.604760614711,37.2714696820741,18.3723122984619));
#36810=CARTESIAN_POINT('Ctrl Pts',(126.670854131373,37.3702618044849,18.3664885953902));
#36811=CARTESIAN_POINT('Ctrl Pts',(126.741369638143,37.4663260767103,18.3606648923186));
#36812=CARTESIAN_POINT('Ctrl Pts',(126.816054720177,37.5592415781028,18.3548411892469));
#36813=CARTESIAN_POINT('Ctrl Pts',(126.890645593262,37.652039874407,18.3490248322867));
#36814=CARTESIAN_POINT('Ctrl Pts',(126.969395326886,37.7416969844718,18.3432084753265));
#36815=CARTESIAN_POINT('Ctrl Pts',(127.052007838526,37.8278202234029,18.3373921183664));
#36816=CARTESIAN_POINT('Ctrl Pts',(127.134537671353,37.9138572699768,18.3315815824311));
#36817=CARTESIAN_POINT('Ctrl Pts',(127.220922310471,37.9963671882897,18.3257710464958));
#36818=CARTESIAN_POINT('Ctrl Pts',(127.310825342853,38.0749901891484,18.3199605105605));
#36819=CARTESIAN_POINT('Ctrl Pts',(127.40412895595,38.1565871037164,18.3139301911993));
#36820=CARTESIAN_POINT('Ctrl Pts',(127.501222103233,38.2339969004973,18.3078998718382));
#36821=CARTESIAN_POINT('Ctrl Pts',(127.601686269053,38.3068589700728,18.3018695524771));
#36822=CARTESIAN_POINT('Ctrl Pts',(127.698379954332,38.3769864823738,18.2960655546269));
#36823=CARTESIAN_POINT('Ctrl Pts',(127.798195825115,38.4429012124677,18.2902615567767));
#36824=CARTESIAN_POINT('Ctrl Pts',(127.900727493049,38.5043230361313,18.2844575589266));
#36825=CARTESIAN_POINT('Ctrl Pts',(128.003244025274,38.5657357927145,18.2786544178617));
#36826=CARTESIAN_POINT('Ctrl Pts',(128.108475207192,38.6226567520707,18.2728512767968));
#36827=CARTESIAN_POINT('Ctrl Pts',(128.215987237424,38.67485012796,18.2670481357319));
#36828=CARTESIAN_POINT('Ctrl Pts',(128.323508766756,38.7270481153337,18.2612444819373));
#36829=CARTESIAN_POINT('Ctrl Pts',(128.433311177737,38.77451751042,18.2554408281427));
#36830=CARTESIAN_POINT('Ctrl Pts',(128.544938324261,38.8170696246983,18.2496371743481));
#36831=CARTESIAN_POINT('Ctrl Pts',(128.656601674374,38.8596355397352,18.2438316382774));
#36832=CARTESIAN_POINT('Ctrl Pts',(128.770090555666,38.8972808568925,18.2380261022068));
#36833=CARTESIAN_POINT('Ctrl Pts',(128.884931825912,38.9298661513004,18.2322205661361));
#36834=CARTESIAN_POINT('Ctrl Pts',(128.999900265625,38.9624875290299,18.2264086013059));
#36835=CARTESIAN_POINT('Ctrl Pts',(129.116223690522,38.9900375879859,18.2205966364756));
#36836=CARTESIAN_POINT('Ctrl Pts',(129.233416723662,39.0124275794635,18.2147846716453));
#36837=CARTESIAN_POINT('Ctrl Pts',(129.350686728555,39.0348322765668,18.2089688895479));
#36838=CARTESIAN_POINT('Ctrl Pts',(129.468827076049,39.0520700978789,18.2031531074504));
#36839=CARTESIAN_POINT('Ctrl Pts',(129.587346843827,39.0641041291656,18.197337325353));
#36840=CARTESIAN_POINT('Ctrl Pts',(129.706036357474,39.0761553957803,18.1915132138014));
#36841=CARTESIAN_POINT('Ctrl Pts',(129.825105969824,39.0829879733735,18.1856891022498));
#36842=CARTESIAN_POINT('Ctrl Pts',(129.944064192394,39.0846170182071,18.1798649906981));
#36843=CARTESIAN_POINT('Ctrl Pts',(129.97560157555,39.085048899333,18.1783209424299));
#36844=CARTESIAN_POINT('Ctrl Pts',(130.007131156836,39.0851153331897,18.1767768941617));
#36845=CARTESIAN_POINT('Ctrl Pts',(130.038643852423,39.0848172116595,18.1752328458935));
#36846=CARTESIAN_POINT('Ctrl Pts',(130.157465235959,39.0836931182737,18.1694108764283));
#36847=CARTESIAN_POINT('Ctrl Pts',(130.276429348989,39.0773783961636,18.1635889069632));
#36848=CARTESIAN_POINT('Ctrl Pts',(130.395046143852,39.0658533599022,18.157766937498));
#36849=CARTESIAN_POINT('Ctrl Pts',(130.513522752562,39.0543419443973,18.1519518486731));
#36850=CARTESIAN_POINT('Ctrl Pts',(130.631652456621,39.037632497184,18.1461367598482));
#36851=CARTESIAN_POINT('Ctrl Pts',(130.748944759515,39.0157573068096,18.1403216710233));
#36852=CARTESIAN_POINT('Ctrl Pts',(130.866126151197,38.9939028015426,18.1345120809271));
#36853=CARTESIAN_POINT('Ctrl Pts',(130.982471317448,38.9668923420503,18.1287024908309));
#36854=CARTESIAN_POINT('Ctrl Pts',(131.097495075478,38.934809977534,18.1228929007347));
#36855=CARTESIAN_POINT('Ctrl Pts',(131.212437236041,38.9027503721395,18.1170874319422));
#36856=CARTESIAN_POINT('Ctrl Pts',(131.326059461223,38.8656261288792,18.1112819631497));
#36857=CARTESIAN_POINT('Ctrl Pts',(131.437887584763,38.8235721901886,18.1054764943573));
#36858=CARTESIAN_POINT('Ctrl Pts',(131.54967089478,38.7815351040131,18.0996733520235));
#36859=CARTESIAN_POINT('Ctrl Pts',(131.659661151168,38.7345723942665,18.0938702096897));
#36860=CARTESIAN_POINT('Ctrl Pts',(131.767400673247,38.6828684283051,18.0880670673559));
#36861=CARTESIAN_POINT('Ctrl Pts',(131.875115437006,38.6311763438082,18.0822652585723));
#36862=CARTESIAN_POINT('Ctrl Pts',(131.980580129119,38.57474535076,18.0764634497886));
#36863=CARTESIAN_POINT('Ctrl Pts',(132.083359010499,38.513807085395,18.0706616410049));
#36864=CARTESIAN_POINT('Ctrl Pts',(132.186158212569,38.4528567717608,18.0648586851299));
#36865=CARTESIAN_POINT('Ctrl Pts',(132.286270192468,38.3873976150219,18.059055729255));
#36866=CARTESIAN_POINT('Ctrl Pts',(132.383286005582,38.3177059567715,18.05325277338));
#36867=CARTESIAN_POINT('Ctrl Pts',(132.418320472563,38.2925388214203,18.051157202983));
#36868=CARTESIAN_POINT('Ctrl Pts',(132.452951454051,38.2668201369431,18.0490616325861));
#36869=CARTESIAN_POINT('Ctrl Pts',(132.487160689988,38.2405642567579,18.0469660621892));
#36870=CARTESIAN_POINT('Ctrl Pts',(132.487160689988,38.2405642567579,19.2967873935987));
#36871=CARTESIAN_POINT('Ctrl Pts',(132.581876183315,38.1678693082642,19.2909824695503));
#36872=CARTESIAN_POINT('Ctrl Pts',(132.673459504492,38.0909741961783,19.2851775455019));
#36873=CARTESIAN_POINT('Ctrl Pts',(132.761523565565,38.0101848110752,19.2793726214535));
#36874=CARTESIAN_POINT('Ctrl Pts',(132.849563259112,37.9294177805789,19.2735693036408));
#36875=CARTESIAN_POINT('Ctrl Pts',(132.934085328219,37.8447588955322,19.2677659858281));
#36876=CARTESIAN_POINT('Ctrl Pts',(133.014736884083,37.7565533769093,19.2619626680154));
#36877=CARTESIAN_POINT('Ctrl Pts',(133.095385157486,37.6683514481887,19.2561595863937));
#36878=CARTESIAN_POINT('Ctrl Pts',(133.172162955497,37.5766034744098,19.250356504772));
#36879=CARTESIAN_POINT('Ctrl Pts',(133.244755734828,37.4816899929886,19.2445534231502));
#36880=CARTESIAN_POINT('Ctrl Pts',(133.317362691672,37.3867579747784,19.2387492081752));
#36881=CARTESIAN_POINT('Ctrl Pts',(133.385782756442,37.2886595438449,19.2329449932002));
#36882=CARTESIAN_POINT('Ctrl Pts',(133.449743394979,37.1878060948816,19.2271407782253));
#36883=CARTESIAN_POINT('Ctrl Pts',(133.513770844082,37.0868472986892,19.2213305004138));
#36884=CARTESIAN_POINT('Ctrl Pts',(133.573329344478,36.983128082249,19.2155202226024));
#36885=CARTESIAN_POINT('Ctrl Pts',(133.628191099959,36.8770866634695,19.209709944791));
#36886=CARTESIAN_POINT('Ctrl Pts',(133.683082542347,36.7709878633391,19.2038965229101));
#36887=CARTESIAN_POINT('Ctrl Pts',(133.733272005007,36.6625647278601,19.1980831010292));
#36888=CARTESIAN_POINT('Ctrl Pts',(133.778579578207,36.5522761903602,19.1922696791483));
#36889=CARTESIAN_POINT('Ctrl Pts',(133.823958933984,36.4418129183755,19.1864470468335));
#36890=CARTESIAN_POINT('Ctrl Pts',(133.864440809216,36.3294787240977,19.1806244145188));
#36891=CARTESIAN_POINT('Ctrl Pts',(133.899894803097,36.2157489563125,19.1748017822041));
#36892=CARTESIAN_POINT('Ctrl Pts',(133.928658564759,36.1234801996423,19.1700778910479));
#36893=CARTESIAN_POINT('Ctrl Pts',(133.954113891697,36.0302932286143,19.1653539998918));
#36894=CARTESIAN_POINT('Ctrl Pts',(133.976216024986,35.9364460062615,19.1606301087357));
#36895=CARTESIAN_POINT('Ctrl Pts',(134.003463478975,35.8207513880271,19.1548065076723));
#36896=CARTESIAN_POINT('Ctrl Pts',(134.025701189063,35.7036800028105,19.1489829066089));
#36897=CARTESIAN_POINT('Ctrl Pts',(134.042793156527,35.5857034177309,19.1431593055455));
#36898=CARTESIAN_POINT('Ctrl Pts',(134.059863559811,35.4678756784928,19.1373430518622));
#36899=CARTESIAN_POINT('Ctrl Pts',(134.071801075186,35.3491454114585,19.1315267981788));
#36900=CARTESIAN_POINT('Ctrl Pts',(134.078520127143,35.229996896702,19.1257105444954));
#36901=CARTESIAN_POINT('Ctrl Pts',(134.085232453231,35.1109676513335,19.1199001129661));
#36902=CARTESIAN_POINT('Ctrl Pts',(134.086736685061,34.991521396484,19.1140896814369));
#36903=CARTESIAN_POINT('Ctrl Pts',(134.0829988062,34.872149506973,19.1082792499076));
#36904=CARTESIAN_POINT('Ctrl Pts',(134.079119447524,34.7482593563155,19.1022488918351));
#36905=CARTESIAN_POINT('Ctrl Pts',(134.069593242631,34.6244497553083,19.0962185337626));
#36906=CARTESIAN_POINT('Ctrl Pts',(134.054441532323,34.5012727589446,19.0901881756901));
#36907=CARTESIAN_POINT('Ctrl Pts',(134.039858836088,34.3827216063255,19.0843842843686));
#36908=CARTESIAN_POINT('Ctrl Pts',(134.020065594881,34.2647568426569,19.0785803930471));
#36909=CARTESIAN_POINT('Ctrl Pts',(133.995133781885,34.1478667564042,19.0727765017256));
#36910=CARTESIAN_POINT('Ctrl Pts',(133.970205651937,34.0309939377167,19.0669734677828));
#36911=CARTESIAN_POINT('Ctrl Pts',(133.940140544955,33.9151958799733,19.0611704338401));
#36912=CARTESIAN_POINT('Ctrl Pts',(133.905061562992,33.8009507144231,19.0553673998973));
#36913=CARTESIAN_POINT('Ctrl Pts',(133.86997948447,33.6866954640075,19.0495638536981));
#36914=CARTESIAN_POINT('Ctrl Pts',(133.829882770845,33.5739937687013,19.043760307499));
#36915=CARTESIAN_POINT('Ctrl Pts',(133.784944218305,33.4633080125401,19.0379567612998));
#36916=CARTESIAN_POINT('Ctrl Pts',(133.739991093487,33.3525863641815,19.0321513331781));
#36917=CARTESIAN_POINT('Ctrl Pts',(133.690193160771,33.243882333199,19.0263459050563));
#36918=CARTESIAN_POINT('Ctrl Pts',(133.635770850116,33.1376371660055,19.0205404769345));
#36919=CARTESIAN_POINT('Ctrl Pts',(133.581288273529,33.0312743455166,19.0147286200239));
#36920=CARTESIAN_POINT('Ctrl Pts',(133.522171283474,32.927376187576,19.0089167631132));
#36921=CARTESIAN_POINT('Ctrl Pts',(133.458685732184,32.8263583538243,19.0031049062026));
#36922=CARTESIAN_POINT('Ctrl Pts',(133.395158484336,32.7252741727576,18.9972892321333));
#36923=CARTESIAN_POINT('Ctrl Pts',(133.327257192831,32.6270744184652,18.991473558064));
#36924=CARTESIAN_POINT('Ctrl Pts',(133.255289420561,32.5321434830236,18.9856578839946));
#36925=CARTESIAN_POINT('Ctrl Pts',(133.183218564689,32.437076572513,18.979833879799));
#36926=CARTESIAN_POINT('Ctrl Pts',(133.107069862149,32.3452881392585,18.9740098756034));
#36927=CARTESIAN_POINT('Ctrl Pts',(133.027189365608,32.2571275011857,18.9681858714078));
#36928=CARTESIAN_POINT('Ctrl Pts',(133.005997571408,32.2337390374252,18.9666407996609));
#36929=CARTESIAN_POINT('Ctrl Pts',(132.984543319394,32.210605687761,18.9650957279141));
#36930=CARTESIAN_POINT('Ctrl Pts',(132.962833467122,32.1877335037192,18.9635506561672));
#36931=CARTESIAN_POINT('Ctrl Pts',(132.881005719069,32.1015247497516,18.9577270448391));
#36932=CARTESIAN_POINT('Ctrl Pts',(132.795280312383,32.0187513282001,18.9519034335109));
#36933=CARTESIAN_POINT('Ctrl Pts',(132.705977105291,31.9397854804535,18.9460798221827));
#36934=CARTESIAN_POINT('Ctrl Pts',(132.616786565085,31.8609192577542,18.9402635580505));
#36935=CARTESIAN_POINT('Ctrl Pts',(132.524027505579,31.7858513224785,18.9344472939182));
#36936=CARTESIAN_POINT('Ctrl Pts',(132.428058057757,31.7149187120923,18.928631029786));
#36937=CARTESIAN_POINT('Ctrl Pts',(132.332184673777,31.6440571040848,18.9228205876386));
#36938=CARTESIAN_POINT('Ctrl Pts',(132.233107620922,31.5773228274695,18.9170101454913));
#36939=CARTESIAN_POINT('Ctrl Pts',(132.131219226661,31.5150136861229,18.911199703344));
#36940=CARTESIAN_POINT('Ctrl Pts',(132.02547458861,31.4503462856131,18.9051693491879));
#36941=CARTESIAN_POINT('Ctrl Pts',(131.916701934944,31.390445897466,18.8991389950319));
#36942=CARTESIAN_POINT('Ctrl Pts',(131.805374685602,31.335597286789,18.8931086408758));
#36943=CARTESIAN_POINT('Ctrl Pts',(131.698227997263,31.2828083512071,18.8873047385864));
#36944=CARTESIAN_POINT('Ctrl Pts',(131.588715513263,31.2346988224533,18.881500836297));
#36945=CARTESIAN_POINT('Ctrl Pts',(131.477285079027,31.1914761658506,18.8756969340076));
#36946=CARTESIAN_POINT('Ctrl Pts',(131.365871103701,31.1482598934805,18.8698938889876));
#36947=CARTESIAN_POINT('Ctrl Pts',(131.252540122111,31.1099292054201,18.8640908439676));
#36948=CARTESIAN_POINT('Ctrl Pts',(131.137759511339,31.0766432364164,18.8582877989476));
#36949=CARTESIAN_POINT('Ctrl Pts',(131.022968766545,31.0433543285821,18.8524842415746));
#36950=CARTESIAN_POINT('Ctrl Pts',(130.906728530291,31.015111139103,18.8466806842017));
#36951=CARTESIAN_POINT('Ctrl Pts',(130.789520249559,30.9920226079061,18.8408771268287));
#36952=CARTESIAN_POINT('Ctrl Pts',(130.672273959939,30.9689265894446,18.8350716874491));
#36953=CARTESIAN_POINT('Ctrl Pts',(130.554059401948,30.9509886325373,18.8292662480694));
#36954=CARTESIAN_POINT('Ctrl Pts',(130.435366454686,30.9382662507085,18.8234608086898));
#36955=CARTESIAN_POINT('Ctrl Pts',(130.316542068664,30.925529780308,18.8176489404551));
#36956=CARTESIAN_POINT('Ctrl Pts',(130.197238642173,30.9180204572198,18.8118370722204));
#36957=CARTESIAN_POINT('Ctrl Pts',(130.077949554722,30.9157437804517,18.8060252039858));
#36958=CARTESIAN_POINT('Ctrl Pts',(129.958582118705,30.913465608372,18.8002095185407));
#36959=CARTESIAN_POINT('Ctrl Pts',(129.839229447754,30.9164269169426,18.7943938330956));
#36960=CARTESIAN_POINT('Ctrl Pts',(129.72038163265,30.9245811787449,18.7885781476506));
#36961=CARTESIAN_POINT('Ctrl Pts',(129.601363585529,30.932747120328,18.7827541320914));
#36962=CARTESIAN_POINT('Ctrl Pts',(129.482852241905,30.946120815644,18.7769301165323));
#36963=CARTESIAN_POINT('Ctrl Pts',(129.365329456219,30.9646043191706,18.7711061009732));
#36964=CARTESIAN_POINT('Ctrl Pts',(129.334153597955,30.9695075307717,18.7695611351817));
#36965=CARTESIAN_POINT('Ctrl Pts',(129.303047230723,30.9747700493633,18.7680161693902));
#36966=CARTESIAN_POINT('Ctrl Pts',(129.272019173074,30.98038945722,18.7664712035988));
#36967=CARTESIAN_POINT('Ctrl Pts',(129.155063459534,31.0015709911399,18.7606476815923));
#36968=CARTESIAN_POINT('Ctrl Pts',(129.038844342866,31.0278953878007,18.7548241595859));
#36969=CARTESIAN_POINT('Ctrl Pts',(128.923848478047,31.0592991864645,18.7490006375794));
#36970=CARTESIAN_POINT('Ctrl Pts',(128.808997700956,31.0906633636534,18.7431844629813));
#36971=CARTESIAN_POINT('Ctrl Pts',(128.695367496481,31.1270940897332,18.7373682883832));
#36972=CARTESIAN_POINT('Ctrl Pts',(128.583436056807,31.1684765960723,18.731552113785));
#36973=CARTESIAN_POINT('Ctrl Pts',(128.471616662397,31.209817677823,18.725741761276));
#36974=CARTESIAN_POINT('Ctrl Pts',(128.361493030679,31.2561005380775,18.7199314087669));
#36975=CARTESIAN_POINT('Ctrl Pts',(128.253529286087,31.3071603006027,18.7141210562579));
#36976=CARTESIAN_POINT('Ctrl Pts',(128.141477007272,31.3601536713711,18.7080906685401));
#36977=CARTESIAN_POINT('Ctrl Pts',(128.031751869413,31.4182927759754,18.7020602808223));
#36978=CARTESIAN_POINT('Ctrl Pts',(127.924851574246,31.4813377526267,18.6960298931045));
#36979=CARTESIAN_POINT('Ctrl Pts',(127.821967755206,31.5420139926597,18.6902260801428));
#36980=CARTESIAN_POINT('Ctrl Pts',(127.721700721023,31.607233881173,18.6844222671811));
#36981=CARTESIAN_POINT('Ctrl Pts',(127.624469472989,31.6767365865402,18.6786184542194));
#36982=CARTESIAN_POINT('Ctrl Pts',(127.527252582283,31.7462290290226,18.6728154982583));
#36983=CARTESIAN_POINT('Ctrl Pts',(127.433070918374,31.8200027932999,18.6670125422973));
#36984=CARTESIAN_POINT('Ctrl Pts',(127.342313766925,31.8977542188724,18.6612095863362));
#36985=CARTESIAN_POINT('Ctrl Pts',(127.251548596664,31.9755125141414,18.6554061176573));
#36986=CARTESIAN_POINT('Ctrl Pts',(127.164208850573,32.0572489037796,18.6496026489784));
#36987=CARTESIAN_POINT('Ctrl Pts',(127.080649545393,32.1426204446752,18.6437991802994));
#36988=CARTESIAN_POINT('Ctrl Pts',(126.997063136129,32.2280196774902,18.6379938291526));
#36989=CARTESIAN_POINT('Ctrl Pts',(126.917259892013,32.3170561149127,18.6321884780057));
#36990=CARTESIAN_POINT('Ctrl Pts',(126.84155644026,32.40935157153,18.6263831268588));
#36991=CARTESIAN_POINT('Ctrl Pts',(126.765769139704,32.5017492541796,18.6205713457312));
#36992=CARTESIAN_POINT('Ctrl Pts',(126.694090954679,32.5974128453291,18.6147595646035));
#36993=CARTESIAN_POINT('Ctrl Pts',(126.626796927584,32.6959327196799,18.6089477834759));
#36994=CARTESIAN_POINT('Ctrl Pts',(126.559458694985,32.7945173118204,18.6031321845842));
#36995=CARTESIAN_POINT('Ctrl Pts',(126.496510570627,32.8959615776701,18.5973165856926));
#36996=CARTESIAN_POINT('Ctrl Pts',(126.438182280427,32.9998301240808,18.5915009868009));
#36997=CARTESIAN_POINT('Ctrl Pts',(126.379770427547,33.1038474753693,18.5856770563256));
#36998=CARTESIAN_POINT('Ctrl Pts',(126.325991802468,33.2102956761344,18.5798531258504));
#36999=CARTESIAN_POINT('Ctrl Pts',(126.277028611372,33.3187180368966,18.5740291953751));
#37000=CARTESIAN_POINT('Ctrl Pts',(126.264032572894,33.3474960054232,18.5724833805935));
#37001=CARTESIAN_POINT('Ctrl Pts',(126.251375512216,33.3764129658833,18.5709375658119));
#37002=CARTESIAN_POINT('Ctrl Pts',(126.23906024573,33.4054602028317,18.5693917510304));
#37003=CARTESIAN_POINT('Ctrl Pts',(126.186096181761,33.5303831768987,18.5627436908306));
#37004=CARTESIAN_POINT('Ctrl Pts',(126.139308119113,33.6580710664456,18.5560956306308));
#37005=CARTESIAN_POINT('Ctrl Pts',(126.098961571862,33.7879256696925,18.549447570431));
#37006=CARTESIAN_POINT('Ctrl Pts',(126.059996556184,33.913333839565,18.5430271506538));
#37007=CARTESIAN_POINT('Ctrl Pts',(126.027039357914,34.040762517582,18.5366067308765));
#37008=CARTESIAN_POINT('Ctrl Pts',(126.000282123105,34.169649528663,18.5301863110992));
#37009=CARTESIAN_POINT('Ctrl Pts',(125.973599397814,34.298177634609,18.5237837699399));
#37010=CARTESIAN_POINT('Ctrl Pts',(125.953082277172,34.4281557287952,18.5173812287806));
#37011=CARTESIAN_POINT('Ctrl Pts',(125.93887329776,34.5590069066826,18.5109786876212));
#37012=CARTESIAN_POINT('Ctrl Pts',(125.924722847556,34.6893190862678,18.5046025196201));
#37013=CARTESIAN_POINT('Ctrl Pts',(125.916828775928,34.8204969250766,18.4982263516189));
#37014=CARTESIAN_POINT('Ctrl Pts',(125.915282546901,34.9519549342306,18.4918501836178));
#37015=CARTESIAN_POINT('Ctrl Pts',(125.915101870904,34.9673157290102,18.4911051319563));
#37016=CARTESIAN_POINT('Ctrl Pts',(125.915007810492,34.9826803339909,18.4903600802947));
#37017=CARTESIAN_POINT('Ctrl Pts',(125.915000466471,34.998047803468,18.4896150286331));
#37018=CARTESIAN_POINT('Origin',(130.,35.,32.7603849714045));
#37019=CARTESIAN_POINT('',(132.487160689988,38.2405642567579,20.546920386683));
#37020=CARTESIAN_POINT('',(132.487160689988,38.2405642567579,20.4426725202732));
#37021=CARTESIAN_POINT('',(132.487160689988,38.2405642567579,32.7603849714045));
#37022=CARTESIAN_POINT('',(125.915000768169,35.0025051829245,19.6353849713624));
#37023=CARTESIAN_POINT('Ctrl Pts',(132.487160689988,38.2405642567579,20.4426725202732));
#37024=CARTESIAN_POINT('Ctrl Pts',(132.581973835524,38.1677943593616,20.4368690147981));
#37025=CARTESIAN_POINT('Ctrl Pts',(132.673580961777,38.0908673687084,20.431065509323));
#37026=CARTESIAN_POINT('Ctrl Pts',(132.76160895586,38.0101064723553,20.4252620038479));
#37027=CARTESIAN_POINT('Ctrl Pts',(132.849664893768,37.9293199390622,20.4194566560935));
#37028=CARTESIAN_POINT('Ctrl Pts',(132.934139139189,37.8446973555699,20.4136513083391));
#37029=CARTESIAN_POINT('Ctrl Pts',(133.014694994994,37.7565991887033,20.4078459605848));
#37030=CARTESIAN_POINT('Ctrl Pts',(133.09533980489,37.6684037391209,20.4020342022544));
#37031=CARTESIAN_POINT('Ctrl Pts',(133.172057312327,37.5767253466558,20.396222443924));
#37032=CARTESIAN_POINT('Ctrl Pts',(133.244550630625,37.4819581393143,20.3904106855936));
#37033=CARTESIAN_POINT('Ctrl Pts',(133.317091117818,37.3871292702292,20.3845951457531));
#37034=CARTESIAN_POINT('Ctrl Pts',(133.385401708896,37.2892079178341,20.3787796059127));
#37035=CARTESIAN_POINT('Ctrl Pts',(133.449229365947,37.1886164079366,20.3729640660722));
#37036=CARTESIAN_POINT('Ctrl Pts',(133.513148940274,37.0878800376765,20.3671401513578));
#37037=CARTESIAN_POINT('Ctrl Pts',(133.572572491666,36.9844661874427,20.3613162366434));
#37038=CARTESIAN_POINT('Ctrl Pts',(133.627293266933,36.8788210547205,20.355492321929));
#37039=CARTESIAN_POINT('Ctrl Pts',(133.643396632603,36.8477315426449,20.3537784458405));
#37040=CARTESIAN_POINT('Ctrl Pts',(133.659093048241,36.8164489212308,20.352064569752));
#37041=CARTESIAN_POINT('Ctrl Pts',(133.674378053835,36.7849848507742,20.3503506936635));
#37042=CARTESIAN_POINT('Ctrl Pts',(133.726315092397,36.678072842759,20.3445271008653));
#37043=CARTESIAN_POINT('Ctrl Pts',(133.773665842193,36.568719760455,20.3387035080672));
#37044=CARTESIAN_POINT('Ctrl Pts',(133.816194276692,36.4573559079866,20.332879915269));
#37045=CARTESIAN_POINT('Ctrl Pts',(133.858669055247,36.3461325575771,20.3270636697991));
#37046=CARTESIAN_POINT('Ctrl Pts',(133.896333475179,36.2329038609136,20.3212474243291));
#37047=CARTESIAN_POINT('Ctrl Pts',(133.928997921923,36.118123575246,20.3154311788592));
#37048=CARTESIAN_POINT('Ctrl Pts',(133.961629671378,36.0034581852706,20.3096207554827));
#37049=CARTESIAN_POINT('Ctrl Pts',(133.989271293348,35.8872446865745,20.3038103321063));
#37050=CARTESIAN_POINT('Ctrl Pts',(134.011781924604,35.7699550567527,20.2979999087298));
#37051=CARTESIAN_POINT('Ctrl Pts',(134.035144634587,35.6482257469733,20.2919695475783));
#37052=CARTESIAN_POINT('Ctrl Pts',(134.052980079561,35.5253376470726,20.2859391864269));
#37053=CARTESIAN_POINT('Ctrl Pts',(134.065188110961,35.4018340733461,20.2799088252754));
#37054=CARTESIAN_POINT('Ctrl Pts',(134.076937654419,35.2829688313354,20.2741049419055));
#37055=CARTESIAN_POINT('Ctrl Pts',(134.083474806991,35.163533954478,20.2683010585356));
#37056=CARTESIAN_POINT('Ctrl Pts',(134.084762795526,35.0440216342746,20.2624971751656));
#37057=CARTESIAN_POINT('Ctrl Pts',(134.086050593813,34.9245269672265,20.2566941490869));
#37058=CARTESIAN_POINT('Ctrl Pts',(134.082090765599,34.8049552877843,20.2508911230081));
#37059=CARTESIAN_POINT('Ctrl Pts',(134.072898649705,34.685800080789,20.2450880969293));
#37060=CARTESIAN_POINT('Ctrl Pts',(134.063705722235,34.5666343535193,20.2392845584984));
#37061=CARTESIAN_POINT('Ctrl Pts',(134.049279620003,34.4478855789528,20.2334810200674));
#37062=CARTESIAN_POINT('Ctrl Pts',(134.029687618859,34.3300427667274,20.2276774816365));
#37063=CARTESIAN_POINT('Ctrl Pts',(134.010089264234,34.2121617393149,20.2218720611789));
#37064=CARTESIAN_POINT('Ctrl Pts',(133.985321745944,34.0951876611345,20.2160666407214));
#37065=CARTESIAN_POINT('Ctrl Pts',(133.955503447749,33.9795993557207,20.2102612202639));
#37066=CARTESIAN_POINT('Ctrl Pts',(133.925652128473,33.8638830466644,20.2044493708258));
#37067=CARTESIAN_POINT('Ctrl Pts',(133.89073896668,33.749555969232,20.1986375213877));
#37068=CARTESIAN_POINT('Ctrl Pts',(133.850932270771,33.6370819371911,20.1928256719496));
#37069=CARTESIAN_POINT('Ctrl Pts',(133.81109942956,33.5245340314549,20.18701000525));
#37070=CARTESIAN_POINT('Ctrl Pts',(133.766366805904,33.4138419727021,20.1811943385504));
#37071=CARTESIAN_POINT('Ctrl Pts',(133.716950257121,33.3054482049546,20.1753786718509));
#37072=CARTESIAN_POINT('Ctrl Pts',(133.667462924315,33.1968991745076,20.1695546748189));
#37073=CARTESIAN_POINT('Ctrl Pts',(133.613278459981,33.0906553683099,20.1637306777869));
#37074=CARTESIAN_POINT('Ctrl Pts',(133.554657961418,32.9871334427427,20.157906680755));
#37075=CARTESIAN_POINT('Ctrl Pts',(133.53910553912,32.9596683623857,20.1563615342017));
#37076=CARTESIAN_POINT('Ctrl Pts',(133.523241105127,32.9323947026958,20.1548163876484));
#37077=CARTESIAN_POINT('Ctrl Pts',(133.507070025083,32.9053198718738,20.1532712410951));
#37078=CARTESIAN_POINT('Ctrl Pts',(133.446121885334,32.8032759410962,20.1474476468882));
#37079=CARTESIAN_POINT('Ctrl Pts',(133.380618063269,32.7037297433222,20.1416240526814));
#37080=CARTESIAN_POINT('Ctrl Pts',(133.310789071845,32.6071145615065,20.1358004584745));
#37081=CARTESIAN_POINT('Ctrl Pts',(133.241048180136,32.5106212741907,20.1299842116026));
#37082=CARTESIAN_POINT('Ctrl Pts',(133.166993209696,32.4170519757968,20.1241679647307));
#37083=CARTESIAN_POINT('Ctrl Pts',(133.088899730347,32.3268139877923,20.1183517178588));
#37084=CARTESIAN_POINT('Ctrl Pts',(133.010884423089,32.2366663286133,20.1125412930887));
#37085=CARTESIAN_POINT('Ctrl Pts',(132.9288389148,32.149843652915,20.1067308683186));
#37086=CARTESIAN_POINT('Ctrl Pts',(132.843080737974,32.0667224956783,20.1009204435484));
#37087=CARTESIAN_POINT('Ctrl Pts',(132.754076447697,31.9804550412993,20.0948900829225));
#37088=CARTESIAN_POINT('Ctrl Pts',(132.661073134668,31.8981752246436,20.0888597222966));
#37089=CARTESIAN_POINT('Ctrl Pts',(132.564470314927,31.8202646330463,20.0828293616707));
#37090=CARTESIAN_POINT('Ctrl Pts',(132.471495505365,31.7452800473365,20.0770254769364));
#37091=CARTESIAN_POINT('Ctrl Pts',(132.375187025588,31.6743427036232,20.071221592202));
#37092=CARTESIAN_POINT('Ctrl Pts',(132.275936372796,31.6077531594853,20.0654177074677));
#37093=CARTESIAN_POINT('Ctrl Pts',(132.17670038053,31.5411734514312,20.0596146800376));
#37094=CARTESIAN_POINT('Ctrl Pts',(132.074523418519,31.4789404932156,20.0538116526075));
#37095=CARTESIAN_POINT('Ctrl Pts',(131.969826631561,31.4213119664334,20.0480086251774));
#37096=CARTESIAN_POINT('Ctrl Pts',(131.865120601135,31.3636783517444,20.0422050854096));
#37097=CARTESIAN_POINT('Ctrl Pts',(131.757894661182,31.3106501736544,20.0364015456419));
#37098=CARTESIAN_POINT('Ctrl Pts',(131.648594683564,31.2624392219892,20.0305980058741));
#37099=CARTESIAN_POINT('Ctrl Pts',(131.539259261419,31.2142126361546,20.0247925840957));
#37100=CARTESIAN_POINT('Ctrl Pts',(131.427848837409,31.170806548242,20.0189871623173));
#37101=CARTESIAN_POINT('Ctrl Pts',(131.31482877954,31.1323844192456,20.013181740539));
#37102=CARTESIAN_POINT('Ctrl Pts',(131.201683562745,31.093919741409,20.0073698898101));
#37103=CARTESIAN_POINT('Ctrl Pts',(131.086925540872,31.0604501709099,20.0015580390813));
#37104=CARTESIAN_POINT('Ctrl Pts',(130.971034895071,31.0320891854081,19.9957461883525));
#37105=CARTESIAN_POINT('Ctrl Pts',(130.855068131856,31.003709572304,19.9899305203781));
#37106=CARTESIAN_POINT('Ctrl Pts',(130.737967662783,30.9804453058232,19.9841148524038));
#37107=CARTESIAN_POINT('Ctrl Pts',(130.62022186056,30.9623583809749,19.9782991844295));
#37108=CARTESIAN_POINT('Ctrl Pts',(130.502307400535,30.9442455486129,19.9724751861559));
#37109=CARTESIAN_POINT('Ctrl Pts',(130.383746166865,30.9313249038325,19.9666511878823));
#37110=CARTESIAN_POINT('Ctrl Pts',(130.265029763147,30.9236064683784,19.9608271896087));
#37111=CARTESIAN_POINT('Ctrl Pts',(130.233533751851,30.9215587317335,19.9592820559146));
#37112=CARTESIAN_POINT('Ctrl Pts',(130.202026806011,30.9198768764323,19.9577369222206));
#37113=CARTESIAN_POINT('Ctrl Pts',(130.170518062656,30.9185604757257,19.9561917885266));
#37114=CARTESIAN_POINT('Ctrl Pts',(130.051761867873,30.9135989722801,19.9503681923312));
#37115=CARTESIAN_POINT('Ctrl Pts',(129.932597446704,30.913816880325,19.9445445961357));
#37116=CARTESIAN_POINT('Ctrl Pts',(129.813513543656,30.9192589151478,19.9387209999403));
#37117=CARTESIAN_POINT('Ctrl Pts',(129.694579882291,30.9246940840514,19.9329047510593));
#37118=CARTESIAN_POINT('Ctrl Pts',(129.575726941313,30.9353402519184,19.9270885021784));
#37119=CARTESIAN_POINT('Ctrl Pts',(129.457446450288,30.9511902186328,19.9212722532974));
#37120=CARTESIAN_POINT('Ctrl Pts',(129.339284358416,30.9670243194793,19.9154618265004));
#37121=CARTESIAN_POINT('Ctrl Pts',(129.221693978929,30.9880518025519,19.9096513997034));
#37122=CARTESIAN_POINT('Ctrl Pts',(129.105164294844,31.0142134953341,19.9038409729064));
#37123=CARTESIAN_POINT('Ctrl Pts',(128.984223793319,31.0413654461064,19.8978106130335));
#37124=CARTESIAN_POINT('Ctrl Pts',(128.864426319196,31.0740479401577,19.8917802531607));
#37125=CARTESIAN_POINT('Ctrl Pts',(128.746310020765,31.1121360059841,19.8857498932878));
#37126=CARTESIAN_POINT('Ctrl Pts',(128.632629637027,31.1487936560838,19.8799460064956));
#37127=CARTESIAN_POINT('Ctrl Pts',(128.520506854986,31.1904580455362,19.8741421197033));
#37128=CARTESIAN_POINT('Ctrl Pts',(128.410407657071,31.2369664918712,19.868338232911));
#37129=CARTESIAN_POINT('Ctrl Pts',(128.300324721989,31.2834680684093,19.8625352034151));
#37130=CARTESIAN_POINT('Ctrl Pts',(128.192265152654,31.3348121200356,19.8567321739192));
#37131=CARTESIAN_POINT('Ctrl Pts',(128.08667532298,31.3907876648352,19.8509291444233));
#37132=CARTESIAN_POINT('Ctrl Pts',(127.981076170894,31.4467681516547,19.8451256025843));
#37133=CARTESIAN_POINT('Ctrl Pts',(127.877947552801,31.507380753393,19.8393220607452));
#37134=CARTESIAN_POINT('Ctrl Pts',(127.777711014526,31.5723686509429,19.8335185189062));
#37135=CARTESIAN_POINT('Ctrl Pts',(127.677441970831,31.6373776232314,19.8277130950533));
#37136=CARTESIAN_POINT('Ctrl Pts',(127.580067214605,31.7067644910825,19.8219076712003));
#37137=CARTESIAN_POINT('Ctrl Pts',(127.485978557904,31.7802296372751,19.8161022473474));
#37138=CARTESIAN_POINT('Ctrl Pts',(127.391785707129,31.8537761390013,19.8102903945498));
#37139=CARTESIAN_POINT('Ctrl Pts',(127.300886541748,31.9314096825366,19.8044785417523));
#37140=CARTESIAN_POINT('Ctrl Pts',(127.213639189223,32.0127908623322,19.7986666889547));
#37141=CARTESIAN_POINT('Ctrl Pts',(127.126334532342,32.0942254935615,19.7928510189126));
#37142=CARTESIAN_POINT('Ctrl Pts',(127.042686750473,32.1794123724234,19.7870353488705));
#37143=CARTESIAN_POINT('Ctrl Pts',(126.96301540279,32.2679770212694,19.7812196788284));
#37144=CARTESIAN_POINT('Ctrl Pts',(126.883229935017,32.3566685288428,19.7753956785043));
#37145=CARTESIAN_POINT('Ctrl Pts',(126.807432528508,32.4487471491802,19.7695716781802));
#37146=CARTESIAN_POINT('Ctrl Pts',(126.735901044559,32.543807212556,19.7637476778561));
#37147=CARTESIAN_POINT('Ctrl Pts',(126.716923659823,32.5690267564012,19.7622025638901));
#37148=CARTESIAN_POINT('Ctrl Pts',(126.69824628613,32.5944560030195,19.7606574499241));
#37149=CARTESIAN_POINT('Ctrl Pts',(126.679873574968,32.6200870768437,19.7591123359582));
#37150=CARTESIAN_POINT('Ctrl Pts',(126.610112055718,32.7174087314556,19.7532455100591));
#37151=CARTESIAN_POINT('Ctrl Pts',(126.544521954283,32.8179553758546,19.7473786841601));
#37152=CARTESIAN_POINT('Ctrl Pts',(126.483412466926,32.9213376603614,19.7415118582611));
#37153=CARTESIAN_POINT('Ctrl Pts',(126.422382087734,33.0245861132317,19.7356526271537));
#37154=CARTESIAN_POINT('Ctrl Pts',(126.365820987408,33.130662563725,19.7297933960463));
#37155=CARTESIAN_POINT('Ctrl Pts',(126.313996696666,33.2391466137661,19.7239341649389));
#37156=CARTESIAN_POINT('Ctrl Pts',(126.262227894924,33.3475145084027,19.7180812073931));
#37157=CARTESIAN_POINT('Ctrl Pts',(126.215185984125,33.4582845152963,19.7122282498472));
#37158=CARTESIAN_POINT('Ctrl Pts',(126.173093649867,33.5710098715147,19.7063752923013));
#37159=CARTESIAN_POINT('Ctrl Pts',(126.130548943581,33.6849467024306,19.7004594322266));
#37160=CARTESIAN_POINT('Ctrl Pts',(126.093061051587,33.800880808957,19.6945435721518));
#37161=CARTESIAN_POINT('Ctrl Pts',(126.06081105525,33.9183274721267,19.6886277120771));
#37162=CARTESIAN_POINT('Ctrl Pts',(126.028952030982,34.0343503098646,19.682783570958));
#37163=CARTESIAN_POINT('Ctrl Pts',(126.002204712039,34.1518488359259,19.6769394298389));
#37164=CARTESIAN_POINT('Ctrl Pts',(125.980694158516,34.2703387411867,19.6710952887198));
#37165=CARTESIAN_POINT('Ctrl Pts',(125.958787640624,34.3910097981563,19.6651435691673));
#37166=CARTESIAN_POINT('Ctrl Pts',(125.942312718303,34.5127086884001,19.6591918496147));
#37167=CARTESIAN_POINT('Ctrl Pts',(125.931347179938,34.6349120245762,19.6532401300621));
#37168=CARTESIAN_POINT('Ctrl Pts',(125.920381641572,34.7571153607523,19.6472884105096));
#37169=CARTESIAN_POINT('Ctrl Pts',(125.91492553145,34.8798227059536,19.641336690957));
#37170=CARTESIAN_POINT('Ctrl Pts',(125.915000768169,35.002505182056,19.6353849714045));
#37171=CARTESIAN_POINT('Ctrl Pts',(125.915000768169,35.0025051829244,19.6353849713624));
#37172=CARTESIAN_POINT('Ctrl Pts',(125.915083357689,35.137177234539,19.6288515991299));
#37173=CARTESIAN_POINT('Ctrl Pts',(125.921829701157,35.271602954508,19.6223182268974));
#37174=CARTESIAN_POINT('Ctrl Pts',(125.935142558203,35.4051653710125,19.6157848546649));
#37175=CARTESIAN_POINT('Ctrl Pts',(125.948507987173,35.5392552199948,19.6092256824147));
#37176=CARTESIAN_POINT('Ctrl Pts',(125.968491780739,35.6724747379491,19.6026665101645));
#37177=CARTESIAN_POINT('Ctrl Pts',(125.994945663421,35.8042168619514,19.5961073379143));
#37178=CARTESIAN_POINT('Ctrl Pts',(126.021539621793,35.9366565723635,19.5895134342565));
#37179=CARTESIAN_POINT('Ctrl Pts',(126.054672268095,36.0676030087451,19.5829195305986));
#37180=CARTESIAN_POINT('Ctrl Pts',(126.094144257802,36.1964597448879,19.5763256269407));
#37181=CARTESIAN_POINT('Ctrl Pts',(126.122663682996,36.2895617160448,19.5715613790904));
#37182=CARTESIAN_POINT('Ctrl Pts',(126.154491475474,36.3815731981222,19.5667971312401));
#37183=CARTESIAN_POINT('Ctrl Pts',(126.189537223157,36.4722766133754,19.5620328833897));
#37184=CARTESIAN_POINT('Ctrl Pts',(126.23237555976,36.5831483650317,19.5562092823377));
#37185=CARTESIAN_POINT('Ctrl Pts',(126.280125989353,36.6923276736055,19.5503856812857));
#37186=CARTESIAN_POINT('Ctrl Pts',(126.332634487451,36.7993485480485,19.5445620802337));
#37187=CARTESIAN_POINT('Ctrl Pts',(126.385076737899,36.9062343989887,19.5387458265615));
#37188=CARTESIAN_POINT('Ctrl Pts',(126.442264938661,37.0109668688231,19.5329295728893));
#37189=CARTESIAN_POINT('Ctrl Pts',(126.503996270988,37.1130979453719,19.5271133192172));
#37190=CARTESIAN_POINT('Ctrl Pts',(126.56566580936,37.2151267872377,19.5213028876989));
#37191=CARTESIAN_POINT('Ctrl Pts',(126.631869222121,37.3145590687665,19.5154924561807));
#37192=CARTESIAN_POINT('Ctrl Pts',(126.7023571311,37.410970034902,19.5096820246624));
#37193=CARTESIAN_POINT('Ctrl Pts',(126.775513028367,37.5110301847367,19.5036516665857));
#37194=CARTESIAN_POINT('Ctrl Pts',(126.853283971465,37.6078353825645,19.497621308509));
#37195=CARTESIAN_POINT('Ctrl Pts',(126.93534063123,37.7009420492502,19.4915909504323));
#37196=CARTESIAN_POINT('Ctrl Pts',(127.014315698474,37.7905521465116,19.4857870591213));
#37197=CARTESIAN_POINT('Ctrl Pts',(127.097260097391,37.8767361619249,19.4799831678102));
#37198=CARTESIAN_POINT('Ctrl Pts',(127.183838715792,37.9591317343657,19.4741792764992));
#37199=CARTESIAN_POINT('Ctrl Pts',(127.270404544387,38.04151513494,19.4683762425667));
#37200=CARTESIAN_POINT('Ctrl Pts',(127.360603229098,38.1201109240758,19.4625732086341));
#37201=CARTESIAN_POINT('Ctrl Pts',(127.454063194637,38.1945939934676,19.4567701747016));
#37202=CARTESIAN_POINT('Ctrl Pts',(127.547531410255,38.2690836377729,19.4509666285124));
#37203=CARTESIAN_POINT('Ctrl Pts',(127.644261159742,38.3394595860072,19.4451630823233));
#37204=CARTESIAN_POINT('Ctrl Pts',(127.743848745212,38.4054377861764,19.4393595361341));
#37205=CARTESIAN_POINT('Ctrl Pts',(127.843468624067,38.4714373811751,19.4335541080221));
#37206=CARTESIAN_POINT('Ctrl Pts',(127.945947841699,38.5330361665828,19.4277486799101));
#37207=CARTESIAN_POINT('Ctrl Pts',(128.050855321786,38.5899944322228,19.4219432517981));
#37208=CARTESIAN_POINT('Ctrl Pts',(128.155878973854,38.6470157720548,19.4161313948968));
#37209=CARTESIAN_POINT('Ctrl Pts',(128.263335896781,38.6993861396859,19.4103195379955));
#37210=CARTESIAN_POINT('Ctrl Pts',(128.372771972104,38.746912588416,19.4045076810943));
#37211=CARTESIAN_POINT('Ctrl Pts',(128.482279923749,38.7944702519559,19.3986920070341));
#37212=CARTESIAN_POINT('Ctrl Pts',(128.593769236102,38.8371775149667,19.3928763329739));
#37213=CARTESIAN_POINT('Ctrl Pts',(128.70676902177,38.8748907903252,19.3870606589137));
#37214=CARTESIAN_POINT('Ctrl Pts',(128.819930663574,38.9126580845915,19.3812366547268));
#37215=CARTESIAN_POINT('Ctrl Pts',(128.934606705762,38.945417002089,19.37541265054));
#37216=CARTESIAN_POINT('Ctrl Pts',(129.050314298558,38.9730746366606,19.3695886463531));
#37217=CARTESIAN_POINT('Ctrl Pts',(129.081010798426,38.980412033935,19.3680435745092));
#37218=CARTESIAN_POINT('Ctrl Pts',(129.1117798641,38.9873906812343,19.3664985026652));
#37219=CARTESIAN_POINT('Ctrl Pts',(129.142612418835,38.994009456131,19.3649534308213));
#37220=CARTESIAN_POINT('Ctrl Pts',(129.258835029318,39.0189587768508,19.3591293178138));
#37221=CARTESIAN_POINT('Ctrl Pts',(129.376334977682,39.0388711371857,19.3533052048063));
#37222=CARTESIAN_POINT('Ctrl Pts',(129.494637966386,39.0536198902934,19.3474810917988));
#37223=CARTESIAN_POINT('Ctrl Pts',(129.612789294764,39.0683497360112,19.3416644451021));
#37224=CARTESIAN_POINT('Ctrl Pts',(129.731741213936,39.0779290916249,19.3358477984054));
#37225=CARTESIAN_POINT('Ctrl Pts',(129.851007742483,39.0822819975107,19.3300311517087));
#37226=CARTESIAN_POINT('Ctrl Pts',(129.970134823259,39.0866298139298,19.324221305901));
#37227=CARTESIAN_POINT('Ctrl Pts',(130.089575375356,39.0857633314435,19.3184114600933));
#37228=CARTESIAN_POINT('Ctrl Pts',(130.208837595067,39.0796583017315,19.3126016142855));
#37229=CARTESIAN_POINT('Ctrl Pts',(130.328021353255,39.0735572884627,19.3067955907223));
#37230=CARTESIAN_POINT('Ctrl Pts',(130.447026606094,39.0622246020963,19.300989567159));
#37231=CARTESIAN_POINT('Ctrl Pts',(130.565361077398,39.0456880567047,19.2951835435957));
#37232=CARTESIAN_POINT('Ctrl Pts',(130.68364562509,39.0291584878439,19.2893799695103));
#37233=CARTESIAN_POINT('Ctrl Pts',(130.801259550487,39.0074294834135,19.2835763954249));
#37234=CARTESIAN_POINT('Ctrl Pts',(130.917715867536,38.9805806845827,19.2777728213395));
#37235=CARTESIAN_POINT('Ctrl Pts',(131.034150536512,38.9537368766769,19.2719703260808));
#37236=CARTESIAN_POINT('Ctrl Pts',(131.149427627894,38.9217752605688,19.2661678308222));
#37237=CARTESIAN_POINT('Ctrl Pts',(131.263071145331,38.8848264159204,19.2603653355635));
#37238=CARTESIAN_POINT('Ctrl Pts',(131.37676781597,38.847860289605,19.2545601263691));
#37239=CARTESIAN_POINT('Ctrl Pts',(131.488828995976,38.8059023962963,19.2487549171747));
#37240=CARTESIAN_POINT('Ctrl Pts',(131.598794668697,38.7591329595196,19.2429497079803));
#37241=CARTESIAN_POINT('Ctrl Pts',(131.708783845301,38.7123535263197,19.23714325799));
#37242=CARTESIAN_POINT('Ctrl Pts',(131.816676250757,38.6607606708509,19.2313368079997));
#37243=CARTESIAN_POINT('Ctrl Pts',(131.922033903607,38.6045818999415,19.2255303580094));
#37244=CARTESIAN_POINT('Ctrl Pts',(132.027506875214,38.5483416388044,19.2197175525946));
#37245=CARTESIAN_POINT('Ctrl Pts',(132.130439195344,38.4875056352456,19.2139047471799));
#37246=CARTESIAN_POINT('Ctrl Pts',(132.2304191985,38.4223464463672,19.2080919417651));
#37247=CARTESIAN_POINT('Ctrl Pts',(132.318370565114,38.3650265871113,19.2029784774328));
#37248=CARTESIAN_POINT('Ctrl Pts',(132.404037544159,38.304361979733,19.1978650131004));
#37249=CARTESIAN_POINT('Ctrl Pts',(132.487160689988,38.2405642567579,19.1927515487681));
#37250=CARTESIAN_POINT('',(125.915000261184,34.9985392205114,19.7396150285596));
#37251=CARTESIAN_POINT('Ctrl Pts',(125.915000261184,34.9985392205114,19.7396150285596));
#37252=CARTESIAN_POINT('Ctrl Pts',(125.914958122368,35.1163783992937,19.7338448931807));
#37253=CARTESIAN_POINT('Ctrl Pts',(125.920019141926,35.2344196377308,19.7280747578017));
#37254=CARTESIAN_POINT('Ctrl Pts',(125.93020956506,35.3521800898317,19.7223046224228));
#37255=CARTESIAN_POINT('Ctrl Pts',(125.940387587581,35.4697972405372,19.716541508658));
#37256=CARTESIAN_POINT('Ctrl Pts',(125.95568256745,35.5871338729639,19.7107783948932));
#37257=CARTESIAN_POINT('Ctrl Pts',(125.976068747181,35.7037060981617,19.7050152811284));
#37258=CARTESIAN_POINT('Ctrl Pts',(125.996435680781,35.8201682701516,19.6992576081893));
#37259=CARTESIAN_POINT('Ctrl Pts',(126.021884184085,35.9358670620511,19.6934999352502));
#37260=CARTESIAN_POINT('Ctrl Pts',(126.05233666646,36.0503233811675,19.6877422623111));
#37261=CARTESIAN_POINT('Ctrl Pts',(126.082770032881,36.1647078525486,19.6819882036395));
#37262=CARTESIAN_POINT('Ctrl Pts',(126.118201025284,36.2778510007493,19.6762341449679));
#37263=CARTESIAN_POINT('Ctrl Pts',(126.158501038498,36.3892842505328,19.6704800862964));
#37264=CARTESIAN_POINT('Ctrl Pts',(126.198788206548,36.5006819822548,19.6647278616646));
#37265=CARTESIAN_POINT('Ctrl Pts',(126.243941169226,36.6103705075494,19.6589756370328));
#37266=CARTESIAN_POINT('Ctrl Pts',(126.293781763915,36.717897373685,19.6532234124009));
#37267=CARTESIAN_POINT('Ctrl Pts',(126.343618775968,36.8254165105849,19.64747160125));
#37268=CARTESIAN_POINT('Ctrl Pts',(126.398142574683,36.930773919495,19.641719790099));
#37269=CARTESIAN_POINT('Ctrl Pts',(126.457127560654,37.0335387575654,19.6359679789481));
#37270=CARTESIAN_POINT('Ctrl Pts',(126.516122868011,37.1363215777649,19.6302151613263));
#37271=CARTESIAN_POINT('Ctrl Pts',(126.579580706571,37.2365105644042,19.6244623437045));
#37272=CARTESIAN_POINT('Ctrl Pts',(126.647230782592,37.3337016893336,19.6187095260827));
#37273=CARTESIAN_POINT('Ctrl Pts',(126.714949685714,37.4309916963915,19.6129508555515));
#37274=CARTESIAN_POINT('Ctrl Pts',(126.786869104481,37.5252774092623,19.6071921850203));
#37275=CARTESIAN_POINT('Ctrl Pts',(126.86267680895,37.6161858104691,19.6014335144891));
#37276=CARTESIAN_POINT('Ctrl Pts',(126.938525657696,37.7071435517858,19.5956717184663));
#37277=CARTESIAN_POINT('Ctrl Pts',(127.018266713924,37.7947200239878,19.5899099224436));
#37278=CARTESIAN_POINT('Ctrl Pts',(127.101550292612,37.8785785196416,19.5841481264209));
#37279=CARTESIAN_POINT('Ctrl Pts',(127.184962488914,37.9625665207726,19.578377432264));
#37280=CARTESIAN_POINT('Ctrl Pts',(127.271927827361,38.0428247965871,19.5726067381072));
#37281=CARTESIAN_POINT('Ctrl Pts',(127.362062681504,38.1190562200269,19.5668360439503));
#37282=CARTESIAN_POINT('Ctrl Pts',(127.424785193413,38.172103694391,19.5628203672577));
#37283=CARTESIAN_POINT('Ctrl Pts',(127.489041833165,38.2232020634187,19.5588046905651));
#37284=CARTESIAN_POINT('Ctrl Pts',(127.554695457864,38.2722638488067,19.5547890138726));
#37285=CARTESIAN_POINT('Ctrl Pts',(127.649907355902,38.3434140058528,19.548965417665));
#37286=CARTESIAN_POINT('Ctrl Pts',(127.748380712973,38.4105199278196,19.5431418214574));
#37287=CARTESIAN_POINT('Ctrl Pts',(127.849737400486,38.4732687418528,19.5373182252498));
#37288=CARTESIAN_POINT('Ctrl Pts',(127.950966211782,38.5359383891217,19.5315019763567));
#37289=CARTESIAN_POINT('Ctrl Pts',(128.055070774009,38.594261649066,19.5256857274635));
#37290=CARTESIAN_POINT('Ctrl Pts',(128.161641181065,38.6479668108197,19.5198694785704));
#37291=CARTESIAN_POINT('Ctrl Pts',(128.268104910799,38.7016182135334,19.5140590517611));
#37292=CARTESIAN_POINT('Ctrl Pts',(128.377029212391,38.7506605317018,19.5082486249519));
#37293=CARTESIAN_POINT('Ctrl Pts',(128.487977100522,38.7948664998198,19.5024381981426));
#37294=CARTESIAN_POINT('Ctrl Pts',(128.603124526696,38.8407457277713,19.4964078382744));
#37295=CARTESIAN_POINT('Ctrl Pts',(128.720451376436,38.8814150100987,19.4903774784061));
#37296=CARTESIAN_POINT('Ctrl Pts',(128.839442933545,38.9166736263699,19.4843471185378));
#37297=CARTESIAN_POINT('Ctrl Pts',(128.953965705526,38.9506080883576,19.4785432317333));
#37298=CARTESIAN_POINT('Ctrl Pts',(129.070029975251,38.9795308293925,19.4727393449288));
#37299=CARTESIAN_POINT('Ctrl Pts',(129.187159294016,39.0033130013397,19.4669354581243));
#37300=CARTESIAN_POINT('Ctrl Pts',(129.304271311523,39.0270916604047,19.4611324286162));
#37301=CARTESIAN_POINT('Ctrl Pts',(129.422447665148,39.0457311791947,19.4553293991081));
#37302=CARTESIAN_POINT('Ctrl Pts',(129.541200817629,39.0591536445737,19.4495263696));
#37303=CARTESIAN_POINT('Ctrl Pts',(129.659964454696,39.0725772950075,19.4437228277488));
#37304=CARTESIAN_POINT('Ctrl Pts',(129.779304586097,39.0807829303666,19.4379192858975));
#37305=CARTESIAN_POINT('Ctrl Pts',(129.898728284197,39.083744487548,19.4321157440463));
#37306=CARTESIAN_POINT('Ctrl Pts',(130.018190709863,39.0867070051242,19.4263103201812));
#37307=CARTESIAN_POINT('Ctrl Pts',(130.137736348122,39.0844220523211,19.4205048963161));
#37308=CARTESIAN_POINT('Ctrl Pts',(130.256872645791,39.0769156777942,19.4146994724511));
#37309=CARTESIAN_POINT('Ctrl Pts',(130.376140875368,39.0694009906848,19.4088876196415));
#37310=CARTESIAN_POINT('Ctrl Pts',(130.494998451751,39.0566533657399,19.4030757668319));
#37311=CARTESIAN_POINT('Ctrl Pts',(130.612958156422,39.0387507101176,19.3972639140223));
#37312=CARTESIAN_POINT('Ctrl Pts',(130.730995337425,39.0208362959708,19.3914482439682));
#37313=CARTESIAN_POINT('Ctrl Pts',(130.848133072549,38.9977601869015,19.3856325739142));
#37314=CARTESIAN_POINT('Ctrl Pts',(130.963896171616,38.9696510136715,19.3798169038601));
#37315=CARTESIAN_POINT('Ctrl Pts',(131.079825088075,38.9415015772678,19.3739929035243));
#37316=CARTESIAN_POINT('Ctrl Pts',(131.194375047637,38.9083048006121,19.3681689031884));
#37317=CARTESIAN_POINT('Ctrl Pts',(131.307087662258,38.8702386028736,19.3623449028525));
#37318=CARTESIAN_POINT('Ctrl Pts',(131.33699044588,38.8601395977345,19.360799789003));
#37319=CARTESIAN_POINT('Ctrl Pts',(131.366764028469,38.8496981178781,19.3592546751536));
#37320=CARTESIAN_POINT('Ctrl Pts',(131.39640012409,38.8389180368224,19.3577095613041));
#37321=CARTESIAN_POINT('Ctrl Pts',(131.508084011547,38.7982932063865,19.3518867861492));
#37322=CARTESIAN_POINT('Ctrl Pts',(131.618173684637,38.7527250769583,19.3460640109944));
#37323=CARTESIAN_POINT('Ctrl Pts',(131.726200385228,38.7023583335542,19.3402412358395));
#37324=CARTESIAN_POINT('Ctrl Pts',(131.834107404725,38.6520473906786,19.3344249116463));
#37325=CARTESIAN_POINT('Ctrl Pts',(131.939955627691,38.5969485711775,19.3286085874531));
#37326=CARTESIAN_POINT('Ctrl Pts',(132.043293086022,38.5372557674861,19.3227922632599));
#37327=CARTESIAN_POINT('Ctrl Pts',(132.146519157764,38.4776273061725,19.3169822084343));
#37328=CARTESIAN_POINT('Ctrl Pts',(132.247239499223,38.413414918366,19.3111721536086));
#37329=CARTESIAN_POINT('Ctrl Pts',(132.345024570039,38.3448594538358,19.305362098783));
#37330=CARTESIAN_POINT('Ctrl Pts',(132.393129575289,38.3111338456868,19.3025038637216));
#37331=CARTESIAN_POINT('Ctrl Pts',(132.440524568373,38.2763578776289,19.2996456286602));
#37332=CARTESIAN_POINT('Ctrl Pts',(132.487160689988,38.2405642567579,19.2967873935987));
#37333=CARTESIAN_POINT('Ctrl Pts',(132.487160689988,38.2405642567579,20.546920386683));
#37334=CARTESIAN_POINT('Ctrl Pts',(132.523548081502,38.2126366236008,20.5446756833603));
#37335=CARTESIAN_POINT('Ctrl Pts',(132.559444026617,38.1841121588552,20.5424309800375));
#37336=CARTESIAN_POINT('Ctrl Pts',(132.594828390309,38.1550104001174,20.5401862767148));
#37337=CARTESIAN_POINT('Ctrl Pts',(132.68662856323,38.0795096363405,20.5343626831359));
#37338=CARTESIAN_POINT('Ctrl Pts',(132.775278808925,37.9998771827638,20.528539089557));
#37339=CARTESIAN_POINT('Ctrl Pts',(132.860385118191,37.9164056603347,20.5227154959782));
#37340=CARTESIAN_POINT('Ctrl Pts',(132.945384053206,37.8330394496301,20.5168992497277));
#37341=CARTESIAN_POINT('Ctrl Pts',(133.026847655955,37.7458440871956,20.5110830034771));
#37342=CARTESIAN_POINT('Ctrl Pts',(133.104414314992,37.6551528695865,20.5052667572266));
#37343=CARTESIAN_POINT('Ctrl Pts',(133.181903329377,37.5645524343848,20.4994563330706));
#37344=CARTESIAN_POINT('Ctrl Pts',(133.255502896449,37.4704634141061,20.4936459089145));
#37345=CARTESIAN_POINT('Ctrl Pts',(133.324888111454,37.3732560010055,20.4878354847585));
#37346=CARTESIAN_POINT('Ctrl Pts',(133.396899701919,37.2723690840767,20.4818051238996));
#37347=CARTESIAN_POINT('Ctrl Pts',(133.464371272435,37.1681233483222,20.4757747630408));
#37348=CARTESIAN_POINT('Ctrl Pts',(133.526985163058,37.0609708051235,20.469744402182));
#37349=CARTESIAN_POINT('Ctrl Pts',(133.587247521374,36.9578424914445,20.4639405180399));
#37350=CARTESIAN_POINT('Ctrl Pts',(133.643010266116,36.852022153747,20.4581366338979));
#37351=CARTESIAN_POINT('Ctrl Pts',(133.694034661703,36.7439417760174,20.4523327497559));
#37352=CARTESIAN_POINT('Ctrl Pts',(133.745051520445,36.6358773629053,20.4465297229091));
#37353=CARTESIAN_POINT('Ctrl Pts',(133.791331247645,36.5255539428036,20.4407266960623));
#37354=CARTESIAN_POINT('Ctrl Pts',(133.832681929684,36.4134264133219,20.4349236692155));
#37355=CARTESIAN_POINT('Ctrl Pts',(133.87403626256,36.3012889841392,20.4291201300214));
#37356=CARTESIAN_POINT('Ctrl Pts',(133.910460543732,36.1873475120151,20.4233165908274));
#37357=CARTESIAN_POINT('Ctrl Pts',(133.941811928858,36.0720744925205,20.4175130516333));
#37358=CARTESIAN_POINT('Ctrl Pts',(133.973173480877,35.9567640913145,20.4117076304184));
#37359=CARTESIAN_POINT('Ctrl Pts',(133.999458758044,35.8401216777956,20.4059022092035));
#37360=CARTESIAN_POINT('Ctrl Pts',(134.020575614029,35.7226318093414,20.4000967879886));
#37361=CARTESIAN_POINT('Ctrl Pts',(134.041715854984,35.6050118316994,20.3942849378054));
#37362=CARTESIAN_POINT('Ctrl Pts',(134.057676177786,35.4865429279749,20.3884730876222));
#37363=CARTESIAN_POINT('Ctrl Pts',(134.06841607087,35.367716839817,20.382661237439));
#37364=CARTESIAN_POINT('Ctrl Pts',(134.079163017976,35.2488127060289,20.3768455700005));
#37365=CARTESIAN_POINT('Ctrl Pts',(134.084682687974,35.1295513275569,20.3710299025621));
#37366=CARTESIAN_POINT('Ctrl Pts',(134.084986697936,35.010424859097,20.3652142351236));
#37367=CARTESIAN_POINT('Ctrl Pts',(134.085291143359,34.8911277547944,20.3593902373676));
#37368=CARTESIAN_POINT('Ctrl Pts',(134.080365034098,34.7719663527491,20.3535662396115));
#37369=CARTESIAN_POINT('Ctrl Pts',(134.070271860309,34.6534282423887,20.3477422418555));
#37370=CARTESIAN_POINT('Ctrl Pts',(134.067594084752,34.6219794175441,20.3461971026191));
#37371=CARTESIAN_POINT('Ctrl Pts',(134.064552893823,34.59057440942,20.3446519633827));
#37372=CARTESIAN_POINT('Ctrl Pts',(134.061150073727,34.5592221890063,20.3431068241463));
#37373=CARTESIAN_POINT('Ctrl Pts',(134.048324924256,34.4410564024724,20.3372832304498));
#37374=CARTESIAN_POINT('Ctrl Pts',(134.030317473102,34.3232602823623,20.3314596367534));
#37375=CARTESIAN_POINT('Ctrl Pts',(134.007156478495,34.2063237707623,20.3256360430569));
#37376=CARTESIAN_POINT('Ctrl Pts',(133.984024704926,34.0895347919567,20.3198197966896));
#37377=CARTESIAN_POINT('Ctrl Pts',(133.95575239879,33.9736036615937,20.3140035503224));
#37378=CARTESIAN_POINT('Ctrl Pts',(133.922420097489,33.8590155220973,20.3081873039552));
#37379=CARTESIAN_POINT('Ctrl Pts',(133.88912116201,33.7445420859765,20.3023768796834));
#37380=CARTESIAN_POINT('Ctrl Pts',(133.850772421122,33.6314093561535,20.2965664554117));
#37381=CARTESIAN_POINT('Ctrl Pts',(133.807505391998,33.5200919995129,20.2907560311399));
#37382=CARTESIAN_POINT('Ctrl Pts',(133.762600616579,33.4045610513189,20.2847256703248));
#37383=CARTESIAN_POINT('Ctrl Pts',(133.712397948555,33.2909860626496,20.2786953095098));
#37384=CARTESIAN_POINT('Ctrl Pts',(133.657101307583,33.1798804912659,20.2726649486947));
#37385=CARTESIAN_POINT('Ctrl Pts',(133.603881390284,33.0729476067983,20.2668610644402));
#37386=CARTESIAN_POINT('Ctrl Pts',(133.545943417349,32.968302399856,20.2610571801857));
#37387=CARTESIAN_POINT('Ctrl Pts',(133.483517821575,32.8663813398906,20.2552532959313));
#37388=CARTESIAN_POINT('Ctrl Pts',(133.421101446739,32.7644753347703,20.2494502689734));
#37389=CARTESIAN_POINT('Ctrl Pts',(133.354198980522,32.6652930245269,20.2436472420155));
#37390=CARTESIAN_POINT('Ctrl Pts',(133.28308568611,32.5692442784881,20.2378442150577));
#37391=CARTESIAN_POINT('Ctrl Pts',(133.211966113147,32.4731870523636,20.2320406757541));
#37392=CARTESIAN_POINT('Ctrl Pts',(133.136635215808,32.3802642687055,20.2262371364504));
#37393=CARTESIAN_POINT('Ctrl Pts',(133.057409873693,32.2908544032772,20.2204335971468));
#37394=CARTESIAN_POINT('Ctrl Pts',(132.978158839736,32.2014155432858,20.214628175824));
#37395=CARTESIAN_POINT('Ctrl Pts',(132.895011120002,32.1154921725934,20.2088227545011));
#37396=CARTESIAN_POINT('Ctrl Pts',(132.808321473045,32.0334269764534,20.2030173331783));
#37397=CARTESIAN_POINT('Ctrl Pts',(132.721535825349,31.9512709007244,20.19720548289));
#37398=CARTESIAN_POINT('Ctrl Pts',(132.631200717785,31.8729818088505,20.1913936326018));
#37399=CARTESIAN_POINT('Ctrl Pts',(132.537705221925,31.7988631384122,20.1855817823136));
#37400=CARTESIAN_POINT('Ctrl Pts',(132.444148317733,31.7246957864433,20.1797661147717));
#37401=CARTESIAN_POINT('Ctrl Pts',(132.347427221364,31.6547045498409,20.1739504472298));
#37402=CARTESIAN_POINT('Ctrl Pts',(132.247959924866,31.5891494937191,20.1681347796878));
#37403=CARTESIAN_POINT('Ctrl Pts',(132.148350152228,31.5235005370726,20.1623107818314));
#37404=CARTESIAN_POINT('Ctrl Pts',(132.045986677373,31.4623006526354,20.1564867839751));
#37405=CARTESIAN_POINT('Ctrl Pts',(131.941312109028,31.4057640178554,20.1506627861187));
#37406=CARTESIAN_POINT('Ctrl Pts',(131.913541379017,31.3907645423858,20.1491176479384));
#37407=CARTESIAN_POINT('Ctrl Pts',(131.885608085199,31.3760930353291,20.1475725097581));
#37408=CARTESIAN_POINT('Ctrl Pts',(131.857520709764,31.3617529203202,20.1460273715779));
#37409=CARTESIAN_POINT('Ctrl Pts',(131.751659969633,31.3077053218923,20.1402037775669));
#37410=CARTESIAN_POINT('Ctrl Pts',(131.643267658667,31.2581946893293,20.134380183556));
#37411=CARTESIAN_POINT('Ctrl Pts',(131.532769314566,31.213465538474,20.1285565895451));
#37412=CARTESIAN_POINT('Ctrl Pts',(131.422410380504,31.1687928200722,20.1227403428612));
#37413=CARTESIAN_POINT('Ctrl Pts',(131.309951073329,31.1288897366471,20.1169240961773));
#37414=CARTESIAN_POINT('Ctrl Pts',(131.195841299892,31.0939548664318,20.1111078494933));
#37415=CARTESIAN_POINT('Ctrl Pts',(131.081845750943,31.0590549662062,20.1052974249031));
#37416=CARTESIAN_POINT('Ctrl Pts',(130.966203410636,31.0291135044589,20.0994870003129));
#37417=CARTESIAN_POINT('Ctrl Pts',(130.849383369636,31.0042806791034,20.0936765757226));
#37418=CARTESIAN_POINT('Ctrl Pts',(130.728141458162,30.9785078820077,20.0876462150263));
#37419=CARTESIAN_POINT('Ctrl Pts',(130.605631343258,30.9582382749794,20.0816158543299));
#37420=CARTESIAN_POINT('Ctrl Pts',(130.482394247442,30.943582764306,20.0755854936335));
#37421=CARTESIAN_POINT('Ctrl Pts',(130.363785441842,30.9294776557354,20.069781609058));
#37422=CARTESIAN_POINT('Ctrl Pts',(130.244503717505,30.9205726148075,20.0639777244826));
#37423=CARTESIAN_POINT('Ctrl Pts',(130.125040439799,30.9169141708244,20.0581738399072));
#37424=CARTESIAN_POINT('Ctrl Pts',(130.005594808104,30.9132562672328,20.052370812628));
#37425=CARTESIAN_POINT('Ctrl Pts',(129.885968084407,30.9148434318936,20.0465677853488));
#37426=CARTESIAN_POINT('Ctrl Pts',(129.766653960882,30.9216701180474,20.0407647580696));
#37427=CARTESIAN_POINT('Ctrl Pts',(129.647329303186,30.928497406925,20.0349612184447));
#37428=CARTESIAN_POINT('Ctrl Pts',(129.528317708227,30.9405651137181,20.0291576788197));
#37429=CARTESIAN_POINT('Ctrl Pts',(129.410109424112,30.9578156760882,20.0233541391948));
#37430=CARTESIAN_POINT('Ctrl Pts',(129.291862806457,30.9750718326105,20.017548717551));
#37431=CARTESIAN_POINT('Ctrl Pts',(129.174420421579,30.9975141283841,20.0117432959072));
#37432=CARTESIAN_POINT('Ctrl Pts',(129.058263347298,31.0250337011544,20.0059378742634));
#37433=CARTESIAN_POINT('Ctrl Pts',(128.941977639887,31.0525837492859,20.0001260236563));
#37434=CARTESIAN_POINT('Ctrl Pts',(128.826980481798,31.0852222034352,19.9943141730493));
#37435=CARTESIAN_POINT('Ctrl Pts',(128.713738934376,31.1227899887859,19.9885023224423));
#37436=CARTESIAN_POINT('Ctrl Pts',(128.600423009333,31.1603824488475,19.9826866545824));
#37437=CARTESIAN_POINT('Ctrl Pts',(128.488865372048,31.2029105427706,19.9768709867226));
#37438=CARTESIAN_POINT('Ctrl Pts',(128.379512661538,31.2501672322775,19.9710553188628));
#37439=CARTESIAN_POINT('Ctrl Pts',(128.270003315182,31.297491611845,19.9652313206922));
#37440=CARTESIAN_POINT('Ctrl Pts',(128.162705565496,31.3495579282979,19.9594073225216));
#37441=CARTESIAN_POINT('Ctrl Pts',(128.05804116635,31.4061134007303,19.953583324351));
#37442=CARTESIAN_POINT('Ctrl Pts',(128.030273190889,31.4211178433444,19.9520381892371));
#37443=CARTESIAN_POINT('Ctrl Pts',(128.002690406456,31.4364380287196,19.9504930541233));
#37444=CARTESIAN_POINT('Ctrl Pts',(127.975300326065,31.4520687393403,19.9489479190094));
#37445=CARTESIAN_POINT('Ctrl Pts',(127.872067493297,31.5109806706853,19.9431243262148));
#37446=CARTESIAN_POINT('Ctrl Pts',(127.771241531522,31.5744969326317,19.9373007334202));
#37447=CARTESIAN_POINT('Ctrl Pts',(127.673260210899,31.6423956525798,19.9314771406255));
#37448=CARTESIAN_POINT('Ctrl Pts',(127.575402508281,31.7102087081967,19.9256608951591));
#37449=CARTESIAN_POINT('Ctrl Pts',(127.48038264117,31.7823929939895,19.9198446496927));
#37450=CARTESIAN_POINT('Ctrl Pts',(127.388613317128,31.8586810743706,19.9140284042263));
#37451=CARTESIAN_POINT('Ctrl Pts',(127.296935854679,31.934892789967,19.9082179808534));
#37452=CARTESIAN_POINT('Ctrl Pts',(127.208502774446,32.0151998684178,19.9024075574804));
#37453=CARTESIAN_POINT('Ctrl Pts',(127.123696835961,32.0992923090149,19.8965971341075));
#37454=CARTESIAN_POINT('Ctrl Pts',(127.035680799239,32.1865678403263,19.8905667729547));
#37455=CARTESIAN_POINT('Ctrl Pts',(126.951572289371,32.2779207098561,19.8845364118019));
#37456=CARTESIAN_POINT('Ctrl Pts',(126.871760743885,32.3729590493298,19.8785060506492));
#37457=CARTESIAN_POINT('Ctrl Pts',(126.794946621221,32.4644281046105,19.8727021672827));
#37458=CARTESIAN_POINT('Ctrl Pts',(126.722112813876,32.559310456321,19.8668982839163));
#37459=CARTESIAN_POINT('Ctrl Pts',(126.653567586128,32.6572206464574,19.8610944005499));
#37460=CARTESIAN_POINT('Ctrl Pts',(126.585032483189,32.755116374288,19.8552913744746));
#37461=CARTESIAN_POINT('Ctrl Pts',(126.520784934205,32.8560387167024,19.8494883483992));
#37462=CARTESIAN_POINT('Ctrl Pts',(126.461090924009,32.9595717234202,19.8436853223239));
#37463=CARTESIAN_POINT('Ctrl Pts',(126.401391643397,33.0631138711207,19.8378817838964));
#37464=CARTESIAN_POINT('Ctrl Pts',(126.346246904886,33.1692667876409,19.8320782454689));
#37465=CARTESIAN_POINT('Ctrl Pts',(126.295877301067,33.2775888901753,19.8262747070414));
#37466=CARTESIAN_POINT('Ctrl Pts',(126.245491362913,33.3859461204306,19.8204692865874));
#37467=CARTESIAN_POINT('Ctrl Pts',(126.199883811203,33.496473565618,19.8146638661333));
#37468=CARTESIAN_POINT('Ctrl Pts',(126.159227305938,33.6087091919549,19.8088584456792));
#37469=CARTESIAN_POINT('Ctrl Pts',(126.118525777253,33.7210691091459,19.8030465962445));
#37470=CARTESIAN_POINT('Ctrl Pts',(126.082786378384,33.8351405992439,19.7972347468098));
#37471=CARTESIAN_POINT('Ctrl Pts',(126.05213208967,33.9504458267486,19.7914228973751));
#37472=CARTESIAN_POINT('Ctrl Pts',(126.021457667015,34.0658267874974,19.7856072306788));
#37473=CARTESIAN_POINT('Ctrl Pts',(125.995875093377,34.1824427015039,19.7797915639825));
#37474=CARTESIAN_POINT('Ctrl Pts',(125.975456039064,34.2998065220979,19.7739758972863));
#37475=CARTESIAN_POINT('Ctrl Pts',(125.955007736599,34.4173384540524,19.7681519002576));
#37476=CARTESIAN_POINT('Ctrl Pts',(125.939737767967,34.5356200273075,19.7623279032289));
#37477=CARTESIAN_POINT('Ctrl Pts',(125.929665904531,34.6541599339824,19.7565039062002));
#37478=CARTESIAN_POINT('Ctrl Pts',(125.926993769684,34.6856093889272,19.7549587596138));
#37479=CARTESIAN_POINT('Ctrl Pts',(125.924687233368,34.7170770343997,19.7534136130274));
#37480=CARTESIAN_POINT('Ctrl Pts',(125.922746050155,34.7485537264753,19.751868466441));
#37481=CARTESIAN_POINT('Ctrl Pts',(125.917614677709,34.8317600046202,19.7477839871591));
#37482=CARTESIAN_POINT('Ctrl Pts',(125.915030089811,34.9151249404383,19.7436995078773));
#37483=CARTESIAN_POINT('Ctrl Pts',(125.915000261185,34.9985392197775,19.7396150285955));
#37484=CARTESIAN_POINT('Origin',(130.,35.,32.7603849714045));
#37485=CARTESIAN_POINT('',(132.487160689988,38.2405642567579,21.7969524304342));
#37486=CARTESIAN_POINT('',(132.487160689988,38.2405642567579,21.6925409181329));
#37487=CARTESIAN_POINT('',(132.487160689988,38.2405642567579,32.7603849714045));
#37488=CARTESIAN_POINT('',(125.915001474033,34.9965297189326,20.8853849714288));
#37489=CARTESIAN_POINT('Ctrl Pts',(132.487160689988,38.2405642567579,21.6925409181329));
#37490=CARTESIAN_POINT('Ctrl Pts',(132.581750090941,38.1679660852364,21.6867311890074));
#37491=CARTESIAN_POINT('Ctrl Pts',(132.673252114311,38.09115093877,21.6809214598819));
#37492=CARTESIAN_POINT('Ctrl Pts',(132.761272906671,38.010414744663,21.6751117307563));
#37493=CARTESIAN_POINT('Ctrl Pts',(132.851093350277,37.9280278383955,21.6691832173529));
#37494=CARTESIAN_POINT('Ctrl Pts',(132.937288287603,37.8415580245174,21.6632547039495));
#37495=CARTESIAN_POINT('Ctrl Pts',(133.019473914611,37.7513637125949,21.6573261905461));
#37496=CARTESIAN_POINT('Ctrl Pts',(133.099929353202,37.6630681895418,21.6515224854041));
#37497=CARTESIAN_POINT('Ctrl Pts',(133.176542345868,37.5712037625444,21.6457187802621));
#37498=CARTESIAN_POINT('Ctrl Pts',(133.248990095402,37.4761438488063,21.6399150751201));
#37499=CARTESIAN_POINT('Ctrl Pts',(133.321429243592,37.3810952210364,21.6341120590217));
#37500=CARTESIAN_POINT('Ctrl Pts',(133.389703884664,37.2828521857437,21.6283090429234));
#37501=CARTESIAN_POINT('Ctrl Pts',(133.453532325283,37.1818202213349,21.6225060268251));
#37502=CARTESIAN_POINT('Ctrl Pts',(133.517368251397,37.0807764083789,21.6167023301767));
#37503=CARTESIAN_POINT('Ctrl Pts',(133.57675672216,36.9769433611896,21.6108986335283));
#37504=CARTESIAN_POINT('Ctrl Pts',(133.631460439649,36.8707538788577,21.6050949368799));
#37505=CARTESIAN_POINT('Ctrl Pts',(133.688224583038,36.7605647495264,21.5990726428961));
#37506=CARTESIAN_POINT('Ctrl Pts',(133.739943909793,36.6478386067895,21.5930503489123));
#37507=CARTESIAN_POINT('Ctrl Pts',(133.786407181534,36.5330837079656,21.5870280549285));
#37508=CARTESIAN_POINT('Ctrl Pts',(133.83125090894,36.4223287566105,21.5812156766853));
#37509=CARTESIAN_POINT('Ctrl Pts',(133.871198793406,36.3096845276156,21.5754032984421));
#37510=CARTESIAN_POINT('Ctrl Pts',(133.906111590045,36.1956242077342,21.5695909201989));
#37511=CARTESIAN_POINT('Ctrl Pts',(133.941048500748,36.0814851070565,21.56377452738));
#37512=CARTESIAN_POINT('Ctrl Pts',(133.970943296275,35.965928361928,21.5579581345612));
#37513=CARTESIAN_POINT('Ctrl Pts',(133.995707691937,35.8494380734306,21.5521417417423));
#37514=CARTESIAN_POINT('Ctrl Pts',(134.020506526533,35.7327857861762,21.54631726028));
#37515=CARTESIAN_POINT('Ctrl Pts',(134.040160658276,35.6151977659667,21.5404927788177));
#37516=CARTESIAN_POINT('Ctrl Pts',(134.054633518213,35.4971639900348,21.5346682973554));
#37517=CARTESIAN_POINT('Ctrl Pts',(134.056158284461,35.4847287202569,21.5340546679283));
#37518=CARTESIAN_POINT('Ctrl Pts',(134.057625589601,35.4722885030589,21.5334410385013));
#37519=CARTESIAN_POINT('Ctrl Pts',(134.059035424522,35.4598439109867,21.5328274090742));
#37520=CARTESIAN_POINT('Ctrl Pts',(134.072415333228,35.3417396540498,21.5270038154121));
#37521=CARTESIAN_POINT('Ctrl Pts',(134.080657885567,35.2228604950866,21.52118022175));
#37522=CARTESIAN_POINT('Ctrl Pts',(134.083683781112,35.1036907704711,21.5153566280879));
#37523=CARTESIAN_POINT('Ctrl Pts',(134.086705859041,34.9846713961642,21.5095403817543));
#37524=CARTESIAN_POINT('Ctrl Pts',(134.084524360526,34.8653625899546,21.5037241354206));
#37525=CARTESIAN_POINT('Ctrl Pts',(134.077111557626,34.7462553514382,21.4979078890869));
#37526=CARTESIAN_POINT('Ctrl Pts',(134.069706174982,34.6272673399242,21.4920974648479));
#37527=CARTESIAN_POINT('Ctrl Pts',(134.057079930669,34.5084808999122,21.4862870406089));
#37528=CARTESIAN_POINT('Ctrl Pts',(134.039257132993,34.3903879811164,21.4804766163699));
#37529=CARTESIAN_POINT('Ctrl Pts',(134.02075970552,34.267825000818,21.4744462555422));
#37530=CARTESIAN_POINT('Ctrl Pts',(133.996664539723,34.1460095296057,21.4684158947145));
#37531=CARTESIAN_POINT('Ctrl Pts',(133.967058086598,34.0254872306836,21.4623855338869));
#37532=CARTESIAN_POINT('Ctrl Pts',(133.938563535254,33.9094912746623,21.4565816496628));
#37533=CARTESIAN_POINT('Ctrl Pts',(133.904964301934,33.7946935418835,21.4507777654388));
#37534=CARTESIAN_POINT('Ctrl Pts',(133.866389576651,33.6815703880888,21.4449738812147));
#37535=CARTESIAN_POINT('Ctrl Pts',(133.827820549267,33.5684639437924,21.4391708542864));
#37536=CARTESIAN_POINT('Ctrl Pts',(133.784277623226,33.4570319729531,21.433367827358));
#37537=CARTESIAN_POINT('Ctrl Pts',(133.735939558197,33.3477347012361,21.4275648004297));
#37538=CARTESIAN_POINT('Ctrl Pts',(133.687597225422,33.2384277797115,21.4217612611547));
#37539=CARTESIAN_POINT('Ctrl Pts',(133.634459077085,33.1312563054996,21.4159577218797));
#37540=CARTESIAN_POINT('Ctrl Pts',(133.576751357029,33.0266589929783,21.4101541826047));
#37541=CARTESIAN_POINT('Ctrl Pts',(133.519024923031,32.9220277607668,21.4043487613095));
#37542=CARTESIAN_POINT('Ctrl Pts',(133.456726167385,32.8199727077647,21.3985433400143));
#37543=CARTESIAN_POINT('Ctrl Pts',(133.390126134964,32.7209059279976,21.3927379187191));
#37544=CARTESIAN_POINT('Ctrl Pts',(133.323452349169,32.6217294409386,21.386926068457));
#37545=CARTESIAN_POINT('Ctrl Pts',(133.252468006667,32.5255481717115,21.3811142181949));
#37546=CARTESIAN_POINT('Ctrl Pts',(133.177486231652,32.4327434394553,21.3753023679327));
#37547=CARTESIAN_POINT('Ctrl Pts',(133.102455208204,32.3398777525513,21.3694867004161));
#37548=CARTESIAN_POINT('Ctrl Pts',(133.023421793114,32.2503933246318,21.3636710328994));
#37549=CARTESIAN_POINT('Ctrl Pts',(132.940736832276,32.1646354937511,21.3578553653828));
#37550=CARTESIAN_POINT('Ctrl Pts',(132.857933434157,32.0787548240348,21.3520313675502));
#37551=CARTESIAN_POINT('Ctrl Pts',(132.771468345597,31.9966116858572,21.3462073697176));
#37552=CARTESIAN_POINT('Ctrl Pts',(132.681726486134,31.9185120390361,21.340383371885));
#37553=CARTESIAN_POINT('Ctrl Pts',(132.657917480278,31.8977917758313,21.3388382334252));
#37554=CARTESIAN_POINT('Ctrl Pts',(132.633877994582,31.877355888102,21.3372930949655));
#37555=CARTESIAN_POINT('Ctrl Pts',(132.60961555488,31.8572095749588,21.3357479565057));
#37556=CARTESIAN_POINT('Ctrl Pts',(132.518170940721,31.7812785533999,21.3299243628355));
#37557=CARTESIAN_POINT('Ctrl Pts',(132.423262109218,31.7092194954134,21.3241007691653));
#37558=CARTESIAN_POINT('Ctrl Pts',(132.325250675735,31.6413642211468,21.3182771754951));
#37559=CARTESIAN_POINT('Ctrl Pts',(132.227362898236,31.5735945563889,21.3124609291534));
#37560=CARTESIAN_POINT('Ctrl Pts',(132.126380637163,31.5100183568043,21.3066446828117));
#37561=CARTESIAN_POINT('Ctrl Pts',(132.022699350964,31.4509279613385,21.30082843647));
#37562=CARTESIAN_POINT('Ctrl Pts',(131.919121850307,31.3918967156854,21.2950180122231));
#37563=CARTESIAN_POINT('Ctrl Pts',(131.812851052025,31.3373425422531,21.2892075879762));
#37564=CARTESIAN_POINT('Ctrl Pts',(131.704311733595,31.2875147791901,21.2833971637293));
#37565=CARTESIAN_POINT('Ctrl Pts',(131.591663977427,31.2358009322168,21.2773668029046));
#37566=CARTESIAN_POINT('Ctrl Pts',(131.476572940032,31.189178629305,21.2713364420799));
#37567=CARTESIAN_POINT('Ctrl Pts',(131.359542387655,31.147874678029,21.2653060812553));
#37568=CARTESIAN_POINT('Ctrl Pts',(131.246907041727,31.1081219404262,21.2595021970237));
#37569=CARTESIAN_POINT('Ctrl Pts',(131.13247565441,31.0732954338841,21.2536983127921));
#37570=CARTESIAN_POINT('Ctrl Pts',(131.016717453162,31.0435482284708,21.2478944285605));
#37571=CARTESIAN_POINT('Ctrl Pts',(130.90097635064,31.0138054170383,21.2420914016247));
#37572=CARTESIAN_POINT('Ctrl Pts',(130.783909219319,30.989140516294,21.236288374689));
#37573=CARTESIAN_POINT('Ctrl Pts',(130.665998968207,30.969656295755,21.2304853477532));
#37574=CARTESIAN_POINT('Ctrl Pts',(130.548078306854,30.9501703549633,21.224681808471));
#37575=CARTESIAN_POINT('Ctrl Pts',(130.429314780602,30.9358660703749,21.2188782691887));
#37576=CARTESIAN_POINT('Ctrl Pts',(130.310199336132,30.9267947054116,21.2130747299064));
#37577=CARTESIAN_POINT('Ctrl Pts',(130.191045263914,30.9177203987105,21.2072693086041));
#37578=CARTESIAN_POINT('Ctrl Pts',(130.071539453462,30.9138824175259,21.2014638873018));
#37579=CARTESIAN_POINT('Ctrl Pts',(129.952175145256,30.9152799626818,21.1956584659995));
#37580=CARTESIAN_POINT('Ctrl Pts',(129.832678652129,30.9166790554896,21.1898466157305));
#37581=CARTESIAN_POINT('Ctrl Pts',(129.713324382588,30.9233252428812,21.1840347654616));
#37582=CARTESIAN_POINT('Ctrl Pts',(129.594602904237,30.9351656620784,21.1782229151926));
#37583=CARTESIAN_POINT('Ctrl Pts',(129.475803448983,30.9470138581263,21.1724072476693));
#37584=CARTESIAN_POINT('Ctrl Pts',(129.357638015862,30.9640630220881,21.1665915801459));
#37585=CARTESIAN_POINT('Ctrl Pts',(129.240587756598,30.9862090183255,21.1607759126225));
#37586=CARTESIAN_POINT('Ctrl Pts',(129.123369835479,31.008386736311,21.1549519147835));
#37587=CARTESIAN_POINT('Ctrl Pts',(129.007270672566,31.0356757651948,21.1491279169445));
#37588=CARTESIAN_POINT('Ctrl Pts',(128.892757162696,31.0679218854099,21.1433039191054));
#37589=CARTESIAN_POINT('Ctrl Pts',(128.862376103998,31.0764769569655,21.141758780716));
#37590=CARTESIAN_POINT('Ctrl Pts',(128.832106548079,31.085380679455,21.1402136423267));
#37591=CARTESIAN_POINT('Ctrl Pts',(128.801956968712,31.0946296084517,21.1386685039373));
#37592=CARTESIAN_POINT('Ctrl Pts',(128.688323845554,31.1294886250555,21.1328449102228));
#37593=CARTESIAN_POINT('Ctrl Pts',(128.576030163277,31.1693674825615,21.1270213165084));
#37594=CARTESIAN_POINT('Ctrl Pts',(128.465551671054,31.2141456280259,21.1211977227939));
#37595=CARTESIAN_POINT('Ctrl Pts',(128.355212563856,31.25886727921,21.1153814764078));
#37596=CARTESIAN_POINT('Ctrl Pts',(128.246684466793,31.3084757721005,21.1095652300216));
#37597=CARTESIAN_POINT('Ctrl Pts',(128.140428659644,31.362800606218,21.1037489836355));
#37598=CARTESIAN_POINT('Ctrl Pts',(128.034279215143,31.417071060878,21.0979385593439));
#37599=CARTESIAN_POINT('Ctrl Pts',(127.930397897057,31.4760482799395,21.0921281350523));
#37600=CARTESIAN_POINT('Ctrl Pts',(127.829226092164,31.5395136698642,21.0863177107608));
#37601=CARTESIAN_POINT('Ctrl Pts',(127.724224726258,31.6053813553999,21.0802873499528));
#37602=CARTESIAN_POINT('Ctrl Pts',(127.622142463116,31.6760835298159,21.0742569891448));
#37603=CARTESIAN_POINT('Ctrl Pts',(127.523445144343,31.7513231852151,21.0682266283368));
#37604=CARTESIAN_POINT('Ctrl Pts',(127.428454507002,31.8237371363593,21.0624227440604));
#37605=CARTESIAN_POINT('Ctrl Pts',(127.33659950276,31.9003536251871,21.056618859784));
#37606=CARTESIAN_POINT('Ctrl Pts',(127.248265368412,31.9808641108226,21.0508149755076));
#37607=CARTESIAN_POINT('Ctrl Pts',(127.159944281962,32.061362704197,21.0450119485271));
#37608=CARTESIAN_POINT('Ctrl Pts',(127.075143332861,32.1457538755285,21.0392089215466));
#37609=CARTESIAN_POINT('Ctrl Pts',(126.994213187701,32.2336900681575,21.0334058945661));
#37610=CARTESIAN_POINT('Ctrl Pts',(126.913275897258,32.3216340246304,21.0276023552391));
#37611=CARTESIAN_POINT('Ctrl Pts',(126.836210366775,32.4131233242236,21.0217988159121));
#37612=CARTESIAN_POINT('Ctrl Pts',(126.763328590591,32.5077754540341,21.0159952765852));
#37613=CARTESIAN_POINT('Ctrl Pts',(126.6904231797,32.6024582784232,21.0101898552383));
#37614=CARTESIAN_POINT('Ctrl Pts',(126.621704470357,32.7003056494819,21.0043844338914));
#37615=CARTESIAN_POINT('Ctrl Pts',(126.557442170625,32.8009045970199,20.9985790125445));
#37616=CARTESIAN_POINT('Ctrl Pts',(126.49310870635,32.9016149485715,20.9927671622313));
#37617=CARTESIAN_POINT('Ctrl Pts',(126.433241722442,33.0050826145845,20.9869553119182));
#37618=CARTESIAN_POINT('Ctrl Pts',(126.378065917296,33.1108683210143,20.9811434616051));
#37619=CARTESIAN_POINT('Ctrl Pts',(126.322853872387,33.2167235080591,20.9753277940377));
#37620=CARTESIAN_POINT('Ctrl Pts',(126.272339314883,33.3248993984854,20.9695121264703));
#37621=CARTESIAN_POINT('Ctrl Pts',(126.226698898596,33.4349364875044,20.963696458903));
#37622=CARTESIAN_POINT('Ctrl Pts',(126.180993107347,33.5451311927576,20.9578724610206));
#37623=CARTESIAN_POINT('Ctrl Pts',(126.140175531625,33.6571920354107,20.9520484631381));
#37624=CARTESIAN_POINT('Ctrl Pts',(126.104373121381,33.7706439805395,20.9462244652557));
#37625=CARTESIAN_POINT('Ctrl Pts',(126.094874549382,33.8007433917773,20.9446793272934));
#37626=CARTESIAN_POINT('Ctrl Pts',(126.085728700532,33.8309406629967,20.9431341893312));
#37627=CARTESIAN_POINT('Ctrl Pts',(126.076937339023,33.8612268188767,20.9415890513689));
#37628=CARTESIAN_POINT('Ctrl Pts',(126.035980316616,34.0023233673116,20.9343905929645));
#37629=CARTESIAN_POINT('Ctrl Pts',(126.00261494991,34.1457149065662,20.9271921345601));
#37630=CARTESIAN_POINT('Ctrl Pts',(125.977056286359,34.290670121258,20.9199936761557));
#37631=CARTESIAN_POINT('Ctrl Pts',(125.951848625682,34.4336346333908,20.9128940757993));
#37632=CARTESIAN_POINT('Ctrl Pts',(125.93423472575,34.578120220996,20.9057944754429));
#37633=CARTESIAN_POINT('Ctrl Pts',(125.924374885705,34.7234047583076,20.8986948750864));
#37634=CARTESIAN_POINT('Ctrl Pts',(125.918213340712,34.8141949951977,20.8942582405339));
#37635=CARTESIAN_POINT('Ctrl Pts',(125.915078978048,34.9052968247186,20.8898216059814));
#37636=CARTESIAN_POINT('Ctrl Pts',(125.915001474033,34.9965297189326,20.8853849714288));
#37637=CARTESIAN_POINT('Ctrl Pts',(125.915001474033,34.9965297194327,20.8853849714045));
#37638=CARTESIAN_POINT('Ctrl Pts',(125.914898933796,35.1172337107693,20.8795151642127));
#37639=CARTESIAN_POINT('Ctrl Pts',(125.920150846961,35.2380430349758,20.8736453570208));
#37640=CARTESIAN_POINT('Ctrl Pts',(125.930756371624,35.3584428726101,20.867775549829));
#37641=CARTESIAN_POINT('Ctrl Pts',(125.941161880961,35.4765720245721,20.8620164445065));
#37642=CARTESIAN_POINT('Ctrl Pts',(125.956720796162,35.5943065688732,20.8562573391839));
#37643=CARTESIAN_POINT('Ctrl Pts',(125.97737978277,35.7111621389884,20.8504982338614));
#37644=CARTESIAN_POINT('Ctrl Pts',(125.998035648517,35.8280000562575,20.844739998541));
#37645=CARTESIAN_POINT('Ctrl Pts',(126.023789981673,35.9439588544505,20.8389817632207));
#37646=CARTESIAN_POINT('Ctrl Pts',(126.0545379871,36.0585624708827,20.8332235279003));
#37647=CARTESIAN_POINT('Ctrl Pts',(126.085288892145,36.1731768947406,20.8274647495631));
#37648=CARTESIAN_POINT('Ctrl Pts',(126.121034297587,36.2864354817355,20.8217059712258));
#37649=CARTESIAN_POINT('Ctrl Pts',(126.161619205866,36.397876203111,20.8159471928886));
#37650=CARTESIAN_POINT('Ctrl Pts',(126.203573824738,36.5130779662902,20.8099940600479));
#37651=CARTESIAN_POINT('Ctrl Pts',(126.250700225613,36.626336539789,20.8040409272072));
#37652=CARTESIAN_POINT('Ctrl Pts',(126.302773206647,36.7371640793301,20.7980877943665));
#37653=CARTESIAN_POINT('Ctrl Pts',(126.353220680841,36.8445320334945,20.7923204941394));
#37654=CARTESIAN_POINT('Ctrl Pts',(126.408310257637,36.9496181249756,20.7865531939122));
#37655=CARTESIAN_POINT('Ctrl Pts',(126.467791010032,37.0520050319609,20.780785893685));
#37656=CARTESIAN_POINT('Ctrl Pts',(126.53014662499,37.1593405697867,20.7747398445376));
#37657=CARTESIAN_POINT('Ctrl Pts',(126.597328220367,37.2637090356662,20.7686937953902));
#37658=CARTESIAN_POINT('Ctrl Pts',(126.668997397388,37.3646662896468,20.7626477462427));
#37659=CARTESIAN_POINT('Ctrl Pts',(126.740666574409,37.4656235436273,20.7566016970953));
#37660=CARTESIAN_POINT('Ctrl Pts',(126.816822954775,37.5631692246295,20.7505556479479));
#37661=CARTESIAN_POINT('Ctrl Pts',(126.897082912045,37.6569024342794,20.7445095988004));
#37662=CARTESIAN_POINT('Ctrl Pts',(126.974389822698,37.7471868688851,20.7386860051039));
#37663=CARTESIAN_POINT('Ctrl Pts',(127.055765126527,37.8342400373365,20.7328624114073));
#37664=CARTESIAN_POINT('Ctrl Pts',(127.140908444354,37.9176738125491,20.7270388177108));
#37665=CARTESIAN_POINT('Ctrl Pts',(127.225944341228,38.00100232365,20.7212225713435));
#37666=CARTESIAN_POINT('Ctrl Pts',(127.314738507605,38.0807202407039,20.7154063249762));
#37667=CARTESIAN_POINT('Ctrl Pts',(127.406950539365,38.1564726348727,20.7095900786089));
#37668=CARTESIAN_POINT('Ctrl Pts',(127.49907026636,38.232149200467,20.7037796543371));
#37669=CARTESIAN_POINT('Ctrl Pts',(127.594600738774,38.3038678823147,20.6979692300653));
#37670=CARTESIAN_POINT('Ctrl Pts',(127.69316539218,38.3713111829319,20.6921588057935));
#37671=CARTESIAN_POINT('Ctrl Pts',(127.795460921016,38.4413073515857,20.6861284449784));
#37672=CARTESIAN_POINT('Ctrl Pts',(127.901024549234,38.5066977662147,20.6800980841633));
#37673=CARTESIAN_POINT('Ctrl Pts',(128.009398053129,38.5671737957537,20.6740677233483));
#37674=CARTESIAN_POINT('Ctrl Pts',(128.113701475785,38.6253785842204,20.6682638390937));
#37675=CARTESIAN_POINT('Ctrl Pts',(128.22060713591,38.6790312437783,20.6624599548392));
#37676=CARTESIAN_POINT('Ctrl Pts',(128.329678398805,38.7279016548969,20.6566560705846));
#37677=CARTESIAN_POINT('Ctrl Pts',(128.438733550694,38.7767648473262,20.6508530436267));
#37678=CARTESIAN_POINT('Ctrl Pts',(128.549953296667,38.8208470291823,20.6450500166687));
#37679=CARTESIAN_POINT('Ctrl Pts',(128.662879021701,38.8599653482115,20.6392469897108));
#37680=CARTESIAN_POINT('Ctrl Pts',(128.77581471688,38.8990871209735,20.6334434504071));
#37681=CARTESIAN_POINT('Ctrl Pts',(128.890456304727,38.9332440258836,20.6276399111034));
#37682=CARTESIAN_POINT('Ctrl Pts',(129.006328549086,38.9623026193918,20.6218363717997));
#37683=CARTESIAN_POINT('Ctrl Pts',(129.122238369446,38.9913706362585,20.6160309504767));
#37684=CARTESIAN_POINT('Ctrl Pts',(129.239379244144,39.0153369543624,20.6102255291538));
#37685=CARTESIAN_POINT('Ctrl Pts',(129.357264883265,39.0341190574542,20.6044201078308));
#37686=CARTESIAN_POINT('Ctrl Pts',(129.475281069791,39.0529219599822,20.5986082575425));
#37687=CARTESIAN_POINT('Ctrl Pts',(129.594043263537,39.0665291236107,20.5927964072542));
#37688=CARTESIAN_POINT('Ctrl Pts',(129.713059015985,39.0749097992093,20.5869845569659));
#37689=CARTESIAN_POINT('Ctrl Pts',(129.832152938601,39.0832959792795,20.5811688894239));
#37690=CARTESIAN_POINT('Ctrl Pts',(129.951500344329,39.0864488240838,20.5753532218819));
#37691=CARTESIAN_POINT('Ctrl Pts',(130.070609405738,39.084389711061,20.5695375543399));
#37692=CARTESIAN_POINT('Ctrl Pts',(130.189889077989,39.0823276485817,20.5637135564834));
#37693=CARTESIAN_POINT('Ctrl Pts',(130.308929318374,39.0750387522796,20.5578895586269));
#37694=CARTESIAN_POINT('Ctrl Pts',(130.427243892813,39.0625961719145,20.5520655607704));
#37695=CARTESIAN_POINT('Ctrl Pts',(130.458633390312,39.0592950879432,20.5505204225909));
#37696=CARTESIAN_POINT('Ctrl Pts',(130.489971870865,39.0556315297765,20.5489752844114));
#37697=CARTESIAN_POINT('Ctrl Pts',(130.521250400697,39.051607461215,20.547430146232));
#37698=CARTESIAN_POINT('Ctrl Pts',(130.639133823974,39.0364414358271,20.5416067849997));
#37699=CARTESIAN_POINT('Ctrl Pts',(130.756544891981,39.0161018747522,20.5357834237673));
#37700=CARTESIAN_POINT('Ctrl Pts',(130.872994388094,38.9906272437245,20.529960062535));
#37701=CARTESIAN_POINT('Ctrl Pts',(130.989303093201,38.9651834123056,20.5241437419246));
#37702=CARTESIAN_POINT('Ctrl Pts',(131.104652142888,38.9346169431329,20.5183274213143));
#37703=CARTESIAN_POINT('Ctrl Pts',(131.218558069069,38.8990179830705,20.5125111007039));
#37704=CARTESIAN_POINT('Ctrl Pts',(131.332533735131,38.8633972272391,20.5066912190014));
#37705=CARTESIAN_POINT('Ctrl Pts',(131.445064103599,38.822737875531,20.5008713372988));
#37706=CARTESIAN_POINT('Ctrl Pts',(131.555674912321,38.7771815639674,20.4950514555963));
#37707=CARTESIAN_POINT('Ctrl Pts',(131.666021161126,38.7317342143953,20.4892454939386));
#37708=CARTESIAN_POINT('Ctrl Pts',(131.774456635541,38.6814134370787,20.4834395322809));
#37709=CARTESIAN_POINT('Ctrl Pts',(131.880526444515,38.6264094213808,20.4776335706232));
#37710=CARTESIAN_POINT('Ctrl Pts',(131.98697771394,38.5712075939134,20.4718067288982));
#37711=CARTESIAN_POINT('Ctrl Pts',(132.091045879827,38.5112889201177,20.4659798871732));
#37712=CARTESIAN_POINT('Ctrl Pts',(132.192293114386,38.4468936596034,20.4601530454482));
#37713=CARTESIAN_POINT('Ctrl Pts',(132.293540348946,38.3824983990892,20.4543262037232));
#37714=CARTESIAN_POINT('Ctrl Pts',(132.391966295005,38.3136267663548,20.4484993619982));
#37715=CARTESIAN_POINT('Ctrl Pts',(132.487160689988,38.2405642567579,20.4426725202732));
#37716=CARTESIAN_POINT('',(125.915001496759,35.0034969295637,20.989615028551));
#37717=CARTESIAN_POINT('Ctrl Pts',(125.915001496759,35.0034969295637,20.989615028551));
#37718=CARTESIAN_POINT('Ctrl Pts',(125.91512689229,35.1499798789446,20.9824905061117));
#37719=CARTESIAN_POINT('Ctrl Pts',(125.923135046557,35.2961228105776,20.9753659836725));
#37720=CARTESIAN_POINT('Ctrl Pts',(125.938894207773,35.4411856121167,20.9682414612332));
#37721=CARTESIAN_POINT('Ctrl Pts',(125.954891578429,35.5884411273641,20.9610092472435));
#37722=CARTESIAN_POINT('Ctrl Pts',(125.97887600381,35.7345836830536,20.9537770332538));
#37723=CARTESIAN_POINT('Ctrl Pts',(126.010660788168,35.8788615664252,20.9465448192641));
#37724=CARTESIAN_POINT('Ctrl Pts',(126.028532809329,35.9599864642905,20.9424782734599));
#37725=CARTESIAN_POINT('Ctrl Pts',(126.048870132568,36.0405222218269,20.9384117276558));
#37726=CARTESIAN_POINT('Ctrl Pts',(126.071632971448,36.1203381136909,20.9343451818516));
#37727=CARTESIAN_POINT('Ctrl Pts',(126.104231036441,36.2346403606165,20.9285215881814));
#37728=CARTESIAN_POINT('Ctrl Pts',(126.14187452446,36.3477030067233,20.9226979945112));
#37729=CARTESIAN_POINT('Ctrl Pts',(126.184452343526,36.4590480050958,20.916874400841));
#37730=CARTESIAN_POINT('Ctrl Pts',(126.226976444347,36.5702525252123,20.9110581544994));
#37731=CARTESIAN_POINT('Ctrl Pts',(126.274422349496,36.6797433298009,20.9052419081577));
#37732=CARTESIAN_POINT('Ctrl Pts',(126.32662874226,36.7870558477034,20.8994256618161));
#37733=CARTESIAN_POINT('Ctrl Pts',(126.378782876136,36.8942609451816,20.8936152375692));
#37734=CARTESIAN_POINT('Ctrl Pts',(126.435687840096,36.9992917286827,20.8878048133223));
#37735=CARTESIAN_POINT('Ctrl Pts',(126.497133839223,37.1017025621347,20.8819943890754));
#37736=CARTESIAN_POINT('Ctrl Pts',(126.56090569653,37.2079898574904,20.8759640282507));
#37737=CARTESIAN_POINT('Ctrl Pts',(126.629568996516,37.3114545241766,20.869933667426));
#37738=CARTESIAN_POINT('Ctrl Pts',(126.702836030425,37.4116249206166,20.8639033066014));
#37739=CARTESIAN_POINT('Ctrl Pts',(126.773351443211,37.5080333116351,20.8580994223698));
#37740=CARTESIAN_POINT('Ctrl Pts',(126.84813076695,37.6013900505575,20.8522955381382));
#37741=CARTESIAN_POINT('Ctrl Pts',(126.926873163261,37.6913038559994,20.8464916539067));
#37742=CARTESIAN_POINT('Ctrl Pts',(127.005603928478,37.7812043802096,20.840688626971));
#37743=CARTESIAN_POINT('Ctrl Pts',(127.088296333164,37.8676626751938,20.8348856000352));
#37744=CARTESIAN_POINT('Ctrl Pts',(127.174609845077,37.950321249028,20.8290825730995));
#37745=CARTESIAN_POINT('Ctrl Pts',(127.26093097757,38.0329871207488,20.8232790338173));
#37746=CARTESIAN_POINT('Ctrl Pts',(127.350873558014,38.1118523218728,20.817475494535));
#37747=CARTESIAN_POINT('Ctrl Pts',(127.444061337677,38.1865973317067,20.8116719552528));
#37748=CARTESIAN_POINT('Ctrl Pts',(127.537279337048,38.2613665804747,20.8058665339505));
#37749=CARTESIAN_POINT('Ctrl Pts',(127.633744310216,38.3320127253313,20.8000611126482));
#37750=CARTESIAN_POINT('Ctrl Pts',(127.733048718338,38.3982579193712,20.7942556913459));
#37751=CARTESIAN_POINT('Ctrl Pts',(127.832463096898,38.4645764738308,20.788443841077));
#37752=CARTESIAN_POINT('Ctrl Pts',(127.934722847035,38.5264841225207,20.7826319908081));
#37753=CARTESIAN_POINT('Ctrl Pts',(128.039393238391,38.583747497569,20.7768201405392));
#37754=CARTESIAN_POINT('Ctrl Pts',(128.14413237782,38.6410484835088,20.7710044730158));
#37755=CARTESIAN_POINT('Ctrl Pts',(128.25128494605,38.6936989412284,20.7651888054925));
#37756=CARTESIAN_POINT('Ctrl Pts',(128.360395032919,38.7415131366766,20.7593731379692));
#37757=CARTESIAN_POINT('Ctrl Pts',(128.469661408204,38.7893958207961,20.7535491401302));
#37758=CARTESIAN_POINT('Ctrl Pts',(128.58089051915,38.8324282690709,20.7477251422912));
#37759=CARTESIAN_POINT('Ctrl Pts',(128.693609942561,38.8704741334653,20.7419011444522));
#37760=CARTESIAN_POINT('Ctrl Pts',(128.723515020342,38.8805679087839,20.7403560060625));
#37761=CARTESIAN_POINT('Ctrl Pts',(128.753524935728,38.8903109713712,20.7388108676728));
#37762=CARTESIAN_POINT('Ctrl Pts',(128.783630750152,38.8997013793397,20.7372657292832));
#37763=CARTESIAN_POINT('Ctrl Pts',(128.897101477997,38.9350944237508,20.7314420044962));
#37764=CARTESIAN_POINT('Ctrl Pts',(129.01230123453,38.9655878970989,20.7256182797092));
#37765=CARTESIAN_POINT('Ctrl Pts',(129.128769267178,38.9910126547265,20.7197945549222));
#37766=CARTESIAN_POINT('Ctrl Pts',(129.245089716665,39.0164051952208,20.7139782097027));
#37767=CARTESIAN_POINT('Ctrl Pts',(129.36267485024,39.0367417088495,20.7081618644833));
#37768=CARTESIAN_POINT('Ctrl Pts',(129.481047661256,39.0519024507152,20.7023455192638));
#37769=CARTESIAN_POINT('Ctrl Pts',(129.59930132911,39.0670479331754,20.6965350282415));
#37770=CARTESIAN_POINT('Ctrl Pts',(129.718340694445,39.077027956149,20.6907245372191));
#37771=CARTESIAN_POINT('Ctrl Pts',(129.837678020953,39.0817737045454,20.6849140461967));
#37772=CARTESIAN_POINT('Ctrl Pts',(129.956926128178,39.086515904913,20.6791078992288));
#37773=CARTESIAN_POINT('Ctrl Pts',(130.076471346657,39.0860316017462,20.6733017522609));
#37774=CARTESIAN_POINT('Ctrl Pts',(130.195820874239,39.0803038104058,20.667495605293));
#37775=CARTESIAN_POINT('Ctrl Pts',(130.315122580235,39.0745783141066,20.6616917847621));
#37776=CARTESIAN_POINT('Ctrl Pts',(130.434228344052,39.0636135270521,20.6558879642312));
#37777=CARTESIAN_POINT('Ctrl Pts',(130.552645896426,39.0474445657925,20.6500841437003));
#37778=CARTESIAN_POINT('Ctrl Pts',(130.671043947295,39.0312782673062,20.6442812789672));
#37779=CARTESIAN_POINT('Ctrl Pts',(130.788753607771,39.0099095547256,20.6384784142341));
#37780=CARTESIAN_POINT('Ctrl Pts',(130.905288900066,38.9834252857832,20.632675549501));
#37781=CARTESIAN_POINT('Ctrl Pts',(131.021832502854,38.9569391281655,20.6268722709477));
#37782=CARTESIAN_POINT('Ctrl Pts',(131.137201172945,38.9253367799129,20.6210689923943));
#37783=CARTESIAN_POINT('Ctrl Pts',(131.250920904916,38.8887558279795,20.6152657138409));
#37784=CARTESIAN_POINT('Ctrl Pts',(131.364740372946,38.8521427933116,20.6094573456156));
#37785=CARTESIAN_POINT('Ctrl Pts',(131.476907624348,38.8105425571125,20.6036489773903));
#37786=CARTESIAN_POINT('Ctrl Pts',(131.58696538028,38.7641421176404,20.5978406091649));
#37787=CARTESIAN_POINT('Ctrl Pts',(131.69707088304,38.7177215480663,20.5920297210703));
#37788=CARTESIAN_POINT('Ctrl Pts',(131.805064697077,38.6664967994386,20.5862188329756));
#37789=CARTESIAN_POINT('Ctrl Pts',(131.910512544746,38.6107017069218,20.5804079448809));
#37790=CARTESIAN_POINT('Ctrl Pts',(132.016116110569,38.5548242200367,20.574588475665));
#37791=CARTESIAN_POINT('Ctrl Pts',(132.119165843905,38.4943631085868,20.5687690064491));
#37792=CARTESIAN_POINT('Ctrl Pts',(132.219254498625,38.4295968378704,20.5629495372332));
#37793=CARTESIAN_POINT('Ctrl Pts',(132.311149254851,38.3701327490009,20.5576064870498));
#37794=CARTESIAN_POINT('Ctrl Pts',(132.400548059744,38.3070401887662,20.5522634368664));
#37795=CARTESIAN_POINT('Ctrl Pts',(132.487160689988,38.2405642567579,20.546920386683));
#37796=CARTESIAN_POINT('Ctrl Pts',(132.487160689988,38.2405642567579,21.7969524304342));
#37797=CARTESIAN_POINT('Ctrl Pts',(132.581957177288,38.1678071446994,21.791146991881));
#37798=CARTESIAN_POINT('Ctrl Pts',(132.673521086805,38.0909156600229,21.7853415533277));
#37799=CARTESIAN_POINT('Ctrl Pts',(132.761485648567,38.010219595438,21.7795361147745));
#37800=CARTESIAN_POINT('Ctrl Pts',(132.849547686816,37.9294341088323,21.7737242430197));
#37801=CARTESIAN_POINT('Ctrl Pts',(132.934002114785,37.844835903111,21.7679123712649));
#37802=CARTESIAN_POINT('Ctrl Pts',(133.01451890325,37.7567917552742,21.7621004995101));
#37803=CARTESIAN_POINT('Ctrl Pts',(133.095088689876,37.6686896545807,21.7562848022362));
#37804=CARTESIAN_POINT('Ctrl Pts',(133.171715413802,37.577137407004,21.7504691049623));
#37805=CARTESIAN_POINT('Ctrl Pts',(133.244110279065,37.4825336850213,21.7446534076884));
#37806=CARTESIAN_POINT('Ctrl Pts',(133.316608713784,37.3877946211746,21.7388293903686));
#37807=CARTESIAN_POINT('Ctrl Pts',(133.384862973331,37.2899957033854,21.7330053730487));
#37808=CARTESIAN_POINT('Ctrl Pts',(133.448628308412,37.189563378945,21.7271813557289));
#37809=CARTESIAN_POINT('Ctrl Pts',(133.465118356053,37.1635910569523,21.7256752345277));
#37810=CARTESIAN_POINT('Ctrl Pts',(133.481308443058,37.137442740957,21.7241691133266));
#37811=CARTESIAN_POINT('Ctrl Pts',(133.497194851732,37.1111260429021,21.7226629921254));
#37812=CARTESIAN_POINT('Ctrl Pts',(133.558621507787,37.0093694537885,21.7168393984549));
#37813=CARTESIAN_POINT('Ctrl Pts',(133.615702371735,36.9047655862021,21.7110158047843));
#37814=CARTESIAN_POINT('Ctrl Pts',(133.668163334243,36.7977215449891,21.7051922111138));
#37815=CARTESIAN_POINT('Ctrl Pts',(133.720558109454,36.690812555734,21.6993759647717));
#37816=CARTESIAN_POINT('Ctrl Pts',(133.768344398241,36.581469879636,21.6935597184296));
#37817=CARTESIAN_POINT('Ctrl Pts',(133.811292182913,36.4701281904866,21.6877434720874));
#37818=CARTESIAN_POINT('Ctrl Pts',(133.854196976616,36.3588979549822,21.68193304784));
#37819=CARTESIAN_POINT('Ctrl Pts',(133.892272755379,36.2456730660014,21.6761226235926));
#37820=CARTESIAN_POINT('Ctrl Pts',(133.925336397825,36.1309107674382,21.6703121993451));
#37821=CARTESIAN_POINT('Ctrl Pts',(133.959651567533,36.01180447848,21.6642818385206));
#37822=CARTESIAN_POINT('Ctrl Pts',(133.988567467094,35.8910424945094,21.6582514776961));
#37823=CARTESIAN_POINT('Ctrl Pts',(134.011935046681,35.7691567988476,21.6522211168716));
#37824=CARTESIAN_POINT('Ctrl Pts',(134.03442503205,35.6518486496693,21.6464172326392));
#37825=CARTESIAN_POINT('Ctrl Pts',(134.051775844245,35.5335001081353,21.6406133484069));
#37826=CARTESIAN_POINT('Ctrl Pts',(134.063906187566,35.4145979964538,21.6348094641745));
#37827=CARTESIAN_POINT('Ctrl Pts',(134.076034739105,35.2957134478856,21.629006437238));
#37828=CARTESIAN_POINT('Ctrl Pts',(134.082944313849,35.1762758978996,21.6232034103014));
#37829=CARTESIAN_POINT('Ctrl Pts',(134.084605395569,35.0567781867096,21.6174003833648));
#37830=CARTESIAN_POINT('Ctrl Pts',(134.086266623946,34.9372699251213,21.6115968440816));
#37831=CARTESIAN_POINT('Ctrl Pts',(134.082678432297,34.8177019000858,21.6057933047984));
#37832=CARTESIAN_POINT('Ctrl Pts',(134.073863433234,34.6985672092126,21.5999897655152));
#37833=CARTESIAN_POINT('Ctrl Pts',(134.065045575569,34.5793938843484,21.5941843442119));
#37834=CARTESIAN_POINT('Ctrl Pts',(134.050997569646,34.4606545801337,21.5883789229086));
#37835=CARTESIAN_POINT('Ctrl Pts',(134.031793849583,34.3428368889937,21.5825735016053));
#37836=CARTESIAN_POINT('Ctrl Pts',(134.012568863177,34.2248887256653,21.5767616513353));
#37837=CARTESIAN_POINT('Ctrl Pts',(133.988176831755,34.1078646158765,21.5709498010652));
#37838=CARTESIAN_POINT('Ctrl Pts',(133.958743270378,33.9922417357144,21.5651379507951));
#37839=CARTESIAN_POINT('Ctrl Pts',(133.92929037688,33.8765429138237,21.5593222832706));
#37840=CARTESIAN_POINT('Ctrl Pts',(133.894789476611,33.7622475444473,21.553506615746));
#37841=CARTESIAN_POINT('Ctrl Pts',(133.855415376923,33.6498158379754,21.5476909482215));
#37842=CARTESIAN_POINT('Ctrl Pts',(133.81598487809,33.5372230852242,21.5418669503811));
#37843=CARTESIAN_POINT('Ctrl Pts',(133.771667398672,33.4264997012987,21.5360429525408));
#37844=CARTESIAN_POINT('Ctrl Pts',(133.722685139917,33.3180843216608,21.5302189547005));
#37845=CARTESIAN_POINT('Ctrl Pts',(133.709689879603,33.2893211303304,21.5286738163193));
#37846=CARTESIAN_POINT('Ctrl Pts',(133.696366524453,33.2607202477137,21.5271286779382));
#37847=CARTESIAN_POINT('Ctrl Pts',(133.682719745472,33.2322895383264,21.525583539557));
#37848=CARTESIAN_POINT('Ctrl Pts',(133.631285325959,33.1251347997844,21.5197599458861));
#37849=CARTESIAN_POINT('Ctrl Pts',(133.575087319942,33.0200539820138,21.5139363522152));
#37850=CARTESIAN_POINT('Ctrl Pts',(133.514315961415,32.9174995021992,21.5081127585444));
#37851=CARTESIAN_POINT('Ctrl Pts',(133.453621274985,32.8150744100946,21.502296512202));
#37852=CARTESIAN_POINT('Ctrl Pts',(133.3883649187,32.7151696645755,21.4964802658595));
#37853=CARTESIAN_POINT('Ctrl Pts',(133.318784353857,32.6182159181412,21.4906640195171));
#37854=CARTESIAN_POINT('Ctrl Pts',(133.249273439543,32.5213592229423,21.4848535952694));
#37855=CARTESIAN_POINT('Ctrl Pts',(133.175447164514,32.4274479801172,21.4790431710217));
#37856=CARTESIAN_POINT('Ctrl Pts',(133.097587573901,32.3368859915481,21.473232746774));
#37857=CARTESIAN_POINT('Ctrl Pts',(133.016780836731,32.2428960443836,21.4672023859496));
#37858=CARTESIAN_POINT('Ctrl Pts',(132.93162964079,32.1525142992767,21.4611720251252));
#37859=CARTESIAN_POINT('Ctrl Pts',(132.842497217893,32.0661570310819,21.4551416643008));
#37860=CARTESIAN_POINT('Ctrl Pts',(132.756712257601,31.9830430016163,21.4493377800682));
#37861=CARTESIAN_POINT('Ctrl Pts',(132.667240035615,31.9036569231099,21.4435338958356));
#37862=CARTESIAN_POINT('Ctrl Pts',(132.574443152638,31.8283336471449,21.437730011603));
#37863=CARTESIAN_POINT('Ctrl Pts',(132.481659976754,31.7530214972334,21.4319269846662));
#37864=CARTESIAN_POINT('Ctrl Pts',(132.385553433453,31.6817712136875,21.4261239577293));
#37865=CARTESIAN_POINT('Ctrl Pts',(132.286519540348,31.6148776400836,21.4203209307925));
#37866=CARTESIAN_POINT('Ctrl Pts',(132.187476903586,31.5479781604763,21.4145173915091));
#37867=CARTESIAN_POINT('Ctrl Pts',(132.085506741543,31.485436384164,21.4087138522256));
#37868=CARTESIAN_POINT('Ctrl Pts',(131.981033862242,31.4275036967617,21.4029103129421));
#37869=CARTESIAN_POINT('Ctrl Pts',(131.876527103605,31.3695522224648,21.3971048916386));
#37870=CARTESIAN_POINT('Ctrl Pts',(131.769516370539,31.316213007569,21.3912994703351));
#37871=CARTESIAN_POINT('Ctrl Pts',(131.660450273352,31.2676910779353,21.3854940490316));
#37872=CARTESIAN_POINT('Ctrl Pts',(131.551263395558,31.2191154147557,21.3796821987613));
#37873=CARTESIAN_POINT('Ctrl Pts',(131.440016983603,31.1753678514284,21.373870348491));
#37874=CARTESIAN_POINT('Ctrl Pts',(131.327178936584,31.1366049813295,21.3680584982208));
#37875=CARTESIAN_POINT('Ctrl Pts',(131.214266776929,31.0978166515693,21.362242830696));
#37876=CARTESIAN_POINT('Ctrl Pts',(131.099761291014,31.0640196505654,21.3564271631713));
#37877=CARTESIAN_POINT('Ctrl Pts',(130.984143208553,31.0353200450656,21.3506114956465));
#37878=CARTESIAN_POINT('Ctrl Pts',(130.868359515674,31.00657933048,21.344787497806));
#37879=CARTESIAN_POINT('Ctrl Pts',(130.751460444184,30.9829506653462,21.3389634999656));
#37880=CARTESIAN_POINT('Ctrl Pts',(130.633934658758,30.9644886509359,21.3331395021251));
#37881=CARTESIAN_POINT('Ctrl Pts',(130.602754427147,30.95959057786,21.3315943637462));
#37882=CARTESIAN_POINT('Ctrl Pts',(130.571530096222,30.9550558855625,21.3300492253674));
#37883=CARTESIAN_POINT('Ctrl Pts',(130.540270804111,30.9508849783904,21.3285040869885));
#37884=CARTESIAN_POINT('Ctrl Pts',(130.422455197195,30.9351649179955,21.3226804933118));
#37885=CARTESIAN_POINT('Ctrl Pts',(130.303762933155,30.9245658317405,21.316856899635));
#37886=CARTESIAN_POINT('Ctrl Pts',(130.184676680017,30.9191766120233,21.3110333059582));
#37887=CARTESIAN_POINT('Ctrl Pts',(130.065740671877,30.9137941916072,21.3052170596099));
#37888=CARTESIAN_POINT('Ctrl Pts',(129.946412067636,30.9136085824429,21.2994008132616));
#37889=CARTESIAN_POINT('Ctrl Pts',(129.827181220253,30.9186572467671,21.2935845669133));
#37890=CARTESIAN_POINT('Ctrl Pts',(129.708069723606,30.9237008573504,21.2877741426596));
#37891=CARTESIAN_POINT('Ctrl Pts',(129.589056194773,30.9339683008373,21.281963718406));
#37892=CARTESIAN_POINT('Ctrl Pts',(129.470632968865,30.9494450323014,21.2761532941524));
#37893=CARTESIAN_POINT('Ctrl Pts',(129.347727179069,30.965507590043,21.2701229333302));
#37894=CARTESIAN_POINT('Ctrl Pts',(129.225457711304,30.9871816126831,21.264092572508));
#37895=CARTESIAN_POINT('Ctrl Pts',(129.104371836297,31.0143914903265,21.2580622116858));
#37896=CARTESIAN_POINT('Ctrl Pts',(128.987833469492,31.0405794722142,21.2522583274473));
#37897=CARTESIAN_POINT('Ctrl Pts',(128.872391830745,31.0718949003306,21.2464544432088));
#37898=CARTESIAN_POINT('Ctrl Pts',(128.758525744759,31.1082180593493,21.2406505589702));
#37899=CARTESIAN_POINT('Ctrl Pts',(128.644676478012,31.144535853049,21.2348475320275));
#37900=CARTESIAN_POINT('Ctrl Pts',(128.532402690125,31.1858597825661,21.2290445050847));
#37901=CARTESIAN_POINT('Ctrl Pts',(128.422168062189,31.2320202527054,21.223241478142));
#37902=CARTESIAN_POINT('Ctrl Pts',(128.311923701688,31.2781847983314,21.2174379388526));
#37903=CARTESIAN_POINT('Ctrl Pts',(128.20371923576,31.3291865758626,21.2116343995633));
#37904=CARTESIAN_POINT('Ctrl Pts',(128.097997780366,31.3848080885647,21.205830860274));
#37905=CARTESIAN_POINT('Ctrl Pts',(127.992242040738,31.4404476386743,21.2000254389646));
#37906=CARTESIAN_POINT('Ctrl Pts',(127.888971274215,31.5007097133633,21.1942200176552));
#37907=CARTESIAN_POINT('Ctrl Pts',(127.788602870344,31.5653314956245,21.1884145963458));
#37908=CARTESIAN_POINT('Ctrl Pts',(127.688123317757,31.6300248405274,21.1826027460697));
#37909=CARTESIAN_POINT('Ctrl Pts',(127.590552886969,31.6990873088665,21.1767908957936));
#37910=CARTESIAN_POINT('Ctrl Pts',(127.496279033403,31.7722134021245,21.1709790455175));
#37911=CARTESIAN_POINT('Ctrl Pts',(127.401943260266,31.8453875249926,21.165163377987));
#37912=CARTESIAN_POINT('Ctrl Pts',(127.310908687063,31.9226303246013,21.1593477104565));
#37913=CARTESIAN_POINT('Ctrl Pts',(127.223527543484,32.0035978744157,21.153532042926));
#37914=CARTESIAN_POINT('Ctrl Pts',(127.136021235853,32.0846814015008,21.1477080450798));
#37915=CARTESIAN_POINT('Ctrl Pts',(127.052179088958,32.1695000383912,21.1418840472337));
#37916=CARTESIAN_POINT('Ctrl Pts',(126.972314637902,32.257675010481,21.1360600493875));
#37917=CARTESIAN_POINT('Ctrl Pts',(126.951126164419,32.2810683104198,21.134514911065));
#37918=CARTESIAN_POINT('Ctrl Pts',(126.930217438476,32.3046976858427,21.1329697727426));
#37919=CARTESIAN_POINT('Ctrl Pts',(126.909593807446,32.3285557155312,21.1314246344201));
#37920=CARTESIAN_POINT('Ctrl Pts',(126.830727378882,32.4197907454494,21.1255159008441));
#37921=CARTESIAN_POINT('Ctrl Pts',(126.755762331176,32.5146859737786,21.119607167268));
#37922=CARTESIAN_POINT('Ctrl Pts',(126.685059339014,32.6128692088321,21.113698433692));
#37923=CARTESIAN_POINT('Ctrl Pts',(126.616054083285,32.7086948455693,21.1079315819792));
#37924=CARTESIAN_POINT('Ctrl Pts',(126.551108816856,32.8076520357571,21.1021647302665));
#37925=CARTESIAN_POINT('Ctrl Pts',(126.490521185756,32.9093581243135,21.0963978785537));
#37926=CARTESIAN_POINT('Ctrl Pts',(126.429989538291,33.0109702353308,21.0906363554751));
#37927=CARTESIAN_POINT('Ctrl Pts',(126.373807733832,33.1153258409295,21.0848748323964));
#37928=CARTESIAN_POINT('Ctrl Pts',(126.322231234451,33.2220118371735,21.0791133093178));
#37929=CARTESIAN_POINT('Ctrl Pts',(126.270689699325,33.3286255098504,21.0733556920367));
#37930=CARTESIAN_POINT('Ctrl Pts',(126.223747441911,33.4375660589538,21.0675980747555));
#37931=CARTESIAN_POINT('Ctrl Pts',(126.181614543347,33.5483948524396,21.0618404574744));
#37932=CARTESIAN_POINT('Ctrl Pts',(126.137570474999,33.6642508965696,21.0558216717345));
#37933=CARTESIAN_POINT('Ctrl Pts',(126.098782575629,33.7821701062652,21.0498028859946));
#37934=CARTESIAN_POINT('Ctrl Pts',(126.065434963677,33.901627123905,21.0437841002547));
#37935=CARTESIAN_POINT('Ctrl Pts',(126.033547892698,34.0158522266135,21.0380289220918));
#37936=CARTESIAN_POINT('Ctrl Pts',(126.00663474156,34.1314828411935,21.032273743929));
#37937=CARTESIAN_POINT('Ctrl Pts',(125.984805368352,34.248044502657,21.0265185657661));
#37938=CARTESIAN_POINT('Ctrl Pts',(125.962975205302,34.3646103816137,21.0207631793664));
#37939=CARTESIAN_POINT('Ctrl Pts',(125.946229255171,34.4821069644494,21.0150077929668));
#37940=CARTESIAN_POINT('Ctrl Pts',(125.934625988469,34.6000510703047,21.0092524065671));
#37941=CARTESIAN_POINT('Ctrl Pts',(125.923016652512,34.718056868503,21.0034940097307));
#37942=CARTESIAN_POINT('Ctrl Pts',(125.916555398921,34.8365102423957,20.9977356128943));
#37943=CARTESIAN_POINT('Ctrl Pts',(125.915248694863,34.9549247830873,20.9919772160579));
#37944=CARTESIAN_POINT('Ctrl Pts',(125.915070017821,34.9711166359783,20.9911898202371));
#37945=CARTESIAN_POINT('Ctrl Pts',(125.91498763816,34.9873077646516,20.9904024244163));
#37946=CARTESIAN_POINT('Ctrl Pts',(125.915001496758,35.0034969286478,20.9896150285955));
#37947=CARTESIAN_POINT('Origin',(130.,35.,32.7603849714045));
#37948=CARTESIAN_POINT('',(132.487160689988,38.2405642567579,23.046779218902));
#37949=CARTESIAN_POINT('',(132.487160689988,38.2405642567579,22.9427607387674));
#37950=CARTESIAN_POINT('',(132.487160689988,38.2405642567579,32.7603849714045));
#37951=CARTESIAN_POINT('',(125.915000225098,35.0013561159219,22.1353849714387));
#37952=CARTESIAN_POINT('Ctrl Pts',(132.487160689988,38.2405642567579,22.9427607387674));
#37953=CARTESIAN_POINT('Ctrl Pts',(132.581883195482,38.1678639263663,22.9369379450951));
#37954=CARTESIAN_POINT('Ctrl Pts',(132.673310088235,38.0910879523884,22.9311151514228));
#37955=CARTESIAN_POINT('Ctrl Pts',(132.761090362255,38.010582171518,22.9252923577505));
#37956=CARTESIAN_POINT('Ctrl Pts',(132.825958211529,37.9510900257316,22.9209894308514));
#37957=CARTESIAN_POINT('Ctrl Pts',(132.888835416071,37.8895618693979,22.9166865039523));
#37958=CARTESIAN_POINT('Ctrl Pts',(132.949594421577,37.82614892534,22.9123835770533));
#37959=CARTESIAN_POINT('Ctrl Pts',(133.031825834812,37.7403256640177,22.9065599833817));
#37960=CARTESIAN_POINT('Ctrl Pts',(133.110440991607,37.6507720417041,22.9007363897102));
#37961=CARTESIAN_POINT('Ctrl Pts',(133.185083236695,37.5578252042159,22.8949127960387));
#37962=CARTESIAN_POINT('Ctrl Pts',(133.259631309504,37.4649956329692,22.8890965496956));
#37963=CARTESIAN_POINT('Ctrl Pts',(133.330216186761,37.3687816770207,22.8832803033525));
#37964=CARTESIAN_POINT('Ctrl Pts',(133.396518192138,37.2695570427899,22.8774640570094));
#37965=CARTESIAN_POINT('Ctrl Pts',(133.462753828841,37.1704317329654,22.8716536327609));
#37966=CARTESIAN_POINT('Ctrl Pts',(133.524714896913,37.0683020778175,22.8658432085125));
#37967=CARTESIAN_POINT('Ctrl Pts',(133.582122530858,36.9635740815967,22.8600327842641));
#37968=CARTESIAN_POINT('Ctrl Pts',(133.641703162486,36.8548819141061,22.8540024234399));
#37969=CARTESIAN_POINT('Ctrl Pts',(133.696378554533,36.7433911632705,22.8479720626158));
#37970=CARTESIAN_POINT('Ctrl Pts',(133.74588670753,36.6295882223287,22.8419417017917));
#37971=CARTESIAN_POINT('Ctrl Pts',(133.793535529379,36.5200592714251,22.8361378175583));
#37972=CARTESIAN_POINT('Ctrl Pts',(133.836398057633,36.4083890800444,22.830333933325));
#37973=CARTESIAN_POINT('Ctrl Pts',(133.874288296302,36.2950348246802,22.8245300490917));
#37974=CARTESIAN_POINT('Ctrl Pts',(133.912172938179,36.1816973129518,22.8187270221542));
#37975=CARTESIAN_POINT('Ctrl Pts',(133.945086621664,36.0666766191031,22.8129239952166));
#37976=CARTESIAN_POINT('Ctrl Pts',(133.972892553101,35.9504471376738,22.8071209682791));
#37977=CARTESIAN_POINT('Ctrl Pts',(134.000700939511,35.8342073943968,22.8013174289949));
#37978=CARTESIAN_POINT('Ctrl Pts',(134.023400582241,35.7167590484978,22.7955138897108));
#37979=CARTESIAN_POINT('Ctrl Pts',(134.040905493144,35.598588168512,22.7897103504266));
#37980=CARTESIAN_POINT('Ctrl Pts',(134.058416080684,35.480378967088,22.7839049291224));
#37981=CARTESIAN_POINT('Ctrl Pts',(134.070728526322,35.3614471693103,22.7780995078181));
#37982=CARTESIAN_POINT('Ctrl Pts',(134.077808610295,35.2422848278376,22.7722940865139));
#37983=CARTESIAN_POINT('Ctrl Pts',(134.084896534807,35.1229905251014,22.7664822362429));
#37984=CARTESIAN_POINT('Ctrl Pts',(134.086740507389,35.0034655769178,22.7606703859719));
#37985=CARTESIAN_POINT('Ctrl Pts',(134.083358430272,34.8842030659968,22.7548585357009));
#37986=CARTESIAN_POINT('Ctrl Pts',(134.079974131789,34.7648622228184,22.7490428681754));
#37987=CARTESIAN_POINT('Ctrl Pts',(134.071356977107,34.6457845665179,22.7432272006499));
#37988=CARTESIAN_POINT('Ctrl Pts',(134.057576680408,34.5274574277291,22.7374115331245));
#37989=CARTESIAN_POINT('Ctrl Pts',(134.043776644923,34.4089607980912,22.7315875352833));
#37990=CARTESIAN_POINT('Ctrl Pts',(134.024798770866,34.29121723338,22.7257635374421));
#37991=CARTESIAN_POINT('Ctrl Pts',(134.000763742125,34.1747033989525,22.7199395396009));
#37992=CARTESIAN_POINT('Ctrl Pts',(133.994387117992,34.1437916435994,22.7183944012289));
#37993=CARTESIAN_POINT('Ctrl Pts',(133.987654806676,34.1129663576886,22.7168492628568));
#37994=CARTESIAN_POINT('Ctrl Pts',(133.980569642328,34.0822362381437,22.7153041244848));
#37995=CARTESIAN_POINT('Ctrl Pts',(133.953865808544,33.9664150709629,22.7094805308134));
#37996=CARTESIAN_POINT('Ctrl Pts',(133.9220597084,33.8515735882992,22.7036569371421));
#37997=CARTESIAN_POINT('Ctrl Pts',(133.885237815503,33.7381948973842,22.6978333434707));
#37998=CARTESIAN_POINT('Ctrl Pts',(133.848462378892,33.6249592505289,22.6920170971277));
#37999=CARTESIAN_POINT('Ctrl Pts',(133.806683861123,33.5131831096538,22.6862008507848));
#38000=CARTESIAN_POINT('Ctrl Pts',(133.760039584541,33.4033386950636,22.6803846044418));
#38001=CARTESIAN_POINT('Ctrl Pts',(133.713441999138,33.2936042353385,22.6745741801936));
#38002=CARTESIAN_POINT('Ctrl Pts',(133.661988503165,33.1857980287977,22.6687637559453));
#38003=CARTESIAN_POINT('Ctrl Pts',(133.605865802955,33.0803758672377,22.6629533316971));
#38004=CARTESIAN_POINT('Ctrl Pts',(133.547618742458,32.9709632588102,22.6569229708729));
#38005=CARTESIAN_POINT('Ctrl Pts',(133.48434215393,32.8641191697739,22.6508926100487));
#38006=CARTESIAN_POINT('Ctrl Pts',(133.416299224074,32.7603293519825,22.6448622492245));
#38007=CARTESIAN_POINT('Ctrl Pts',(133.350811718553,32.6604374707826,22.6390583649913));
#38008=CARTESIAN_POINT('Ctrl Pts',(133.280909669464,32.5633749574022,22.6332544807582));
#38009=CARTESIAN_POINT('Ctrl Pts',(133.206873489809,32.4695479810198,22.627450596525));
#38010=CARTESIAN_POINT('Ctrl Pts',(133.13284824609,32.3757348638852,22.6216475695876));
#38011=CARTESIAN_POINT('Ctrl Pts',(133.054690339081,32.2851566537826,22.6158445426502));
#38012=CARTESIAN_POINT('Ctrl Pts',(132.972721553387,32.1981878067883,22.6100415157128));
#38013=CARTESIAN_POINT('Ctrl Pts',(132.890745530706,32.1112112813543,22.6042379764288));
#38014=CARTESIAN_POINT('Ctrl Pts',(132.804958240457,32.0278450497876,22.5984344371448));
#38015=CARTESIAN_POINT('Ctrl Pts',(132.715719080768,31.948427475161,22.5926308978608));
#38016=CARTESIAN_POINT('Ctrl Pts',(132.62645098186,31.8689841463411,22.5868254765567));
#38017=CARTESIAN_POINT('Ctrl Pts',(132.533729092154,31.7934922924173,22.5810200552526));
#38018=CARTESIAN_POINT('Ctrl Pts',(132.437946192268,31.7222502591559,22.5752146339485));
#38019=CARTESIAN_POINT('Ctrl Pts',(132.342057221687,31.6509293319369,22.5694027836777));
#38020=CARTESIAN_POINT('Ctrl Pts',(132.243100802464,31.5838678633661,22.5635909334068));
#38021=CARTESIAN_POINT('Ctrl Pts',(132.141499148099,31.521321170517,22.557779083136));
#38022=CARTESIAN_POINT('Ctrl Pts',(132.039830761221,31.4587333966643,22.5519634156107));
#38023=CARTESIAN_POINT('Ctrl Pts',(131.935514035084,31.4006665022058,22.5461477480853));
#38024=CARTESIAN_POINT('Ctrl Pts',(131.828994773743,31.347329317113,22.54033208056));
#38025=CARTESIAN_POINT('Ctrl Pts',(131.722322935062,31.2939157322621,22.534508082719));
#38026=CARTESIAN_POINT('Ctrl Pts',(131.613442635645,31.2452455449521,22.5286840848779));
#38027=CARTESIAN_POINT('Ctrl Pts',(131.502818699154,31.201479109249,22.5228600870369));
#38028=CARTESIAN_POINT('Ctrl Pts',(131.473469565799,31.1898676352888,22.5213149486634));
#38029=CARTESIAN_POINT('Ctrl Pts',(131.443997778231,31.1786010472255,22.5197698102899));
#38030=CARTESIAN_POINT('Ctrl Pts',(131.414412163886,31.1676817419932,22.5182246719164));
#38031=CARTESIAN_POINT('Ctrl Pts',(131.302904612573,31.1265271127782,22.512401078245));
#38032=CARTESIAN_POINT('Ctrl Pts',(131.189419564544,31.0901768992921,22.5065774845737));
#38033=CARTESIAN_POINT('Ctrl Pts',(131.07440847843,31.0588235992945,22.5007538909023));
#38034=CARTESIAN_POINT('Ctrl Pts',(130.959542495884,31.0275098561421,22.4949376445594));
#38035=CARTESIAN_POINT('Ctrl Pts',(130.843154695164,31.0011805937281,22.4891213982165));
#38036=CARTESIAN_POINT('Ctrl Pts',(130.725715302816,30.9799798135757,22.4833051518736));
#38037=CARTESIAN_POINT('Ctrl Pts',(130.608393467947,30.9588002555212,22.4774947276254));
#38038=CARTESIAN_POINT('Ctrl Pts',(130.490022535097,30.9427390391147,22.4716843033771));
#38039=CARTESIAN_POINT('Ctrl Pts',(130.371086060982,30.9318898570289,22.4658738791289));
#38040=CARTESIAN_POINT('Ctrl Pts',(130.247647595317,30.9206300109608,22.4598435183047));
#38041=CARTESIAN_POINT('Ctrl Pts',(130.123600361081,30.9149846857911,22.4538131574805));
#38042=CARTESIAN_POINT('Ctrl Pts',(129.999494896475,30.9150000312276,22.4477827966563));
#38043=CARTESIAN_POINT('Ctrl Pts',(129.880050344106,30.91501480035,22.4419789124232));
#38044=CARTESIAN_POINT('Ctrl Pts',(129.760552301349,30.9202727227172,22.43617502819));
#38045=CARTESIAN_POINT('Ctrl Pts',(129.641494188579,30.930761916135,22.4303711439569));
#38046=CARTESIAN_POINT('Ctrl Pts',(129.522453661966,30.9412495601867,22.4245681170196));
#38047=CARTESIAN_POINT('Ctrl Pts',(129.403853342763,30.9569669027769,22.4187650900822));
#38048=CARTESIAN_POINT('Ctrl Pts',(129.286182805827,30.9778500757303,22.4129620631448));
#38049=CARTESIAN_POINT('Ctrl Pts',(129.168501879813,30.9987350924494,22.4071585238609));
#38050=CARTESIAN_POINT('Ctrl Pts',(129.051751301354,31.0247867749896,22.4013549845769));
#38051=CARTESIAN_POINT('Ctrl Pts',(128.936411076524,31.0558900114399,22.395551445293));
#38052=CARTESIAN_POINT('Ctrl Pts',(128.821033448205,31.087003334307,22.3897460239889));
#38053=CARTESIAN_POINT('Ctrl Pts',(128.707067477153,31.123171362753,22.3839406026848));
#38054=CARTESIAN_POINT('Ctrl Pts',(128.594977999189,31.1642291286838,22.3781351813808));
#38055=CARTESIAN_POINT('Ctrl Pts',(128.482764392503,31.2053323622901,22.37232333111));
#38056=CARTESIAN_POINT('Ctrl Pts',(128.372431810507,31.2513360015191,22.3665114808392));
#38057=CARTESIAN_POINT('Ctrl Pts',(128.264425235097,31.3020268747014,22.3606996305683));
#38058=CARTESIAN_POINT('Ctrl Pts',(128.156347720387,31.3527510419214,22.3548839630431));
#38059=CARTESIAN_POINT('Ctrl Pts',(128.050599615635,31.4081683851012,22.3490682955178));
#38060=CARTESIAN_POINT('Ctrl Pts',(127.947599953747,31.4680205195754,22.3432526279925));
#38061=CARTESIAN_POINT('Ctrl Pts',(127.844452755965,31.5279583857694,22.3374286301515));
#38062=CARTESIAN_POINT('Ctrl Pts',(127.744062201283,31.5923435025609,22.3316046323105));
#38063=CARTESIAN_POINT('Ctrl Pts',(127.646817204615,31.6608750051096,22.3257806344695));
#38064=CARTESIAN_POINT('Ctrl Pts',(127.621017576916,31.6790567863011,22.3242354960956));
#38065=CARTESIAN_POINT('Ctrl Pts',(127.595439167258,31.6975302058238,22.3226903577218));
#38066=CARTESIAN_POINT('Ctrl Pts',(127.570088819246,31.7162891945781,22.321145219348));
#38067=CARTESIAN_POINT('Ctrl Pts',(127.475346633759,31.7863974073423,22.315370553598));
#38068=CARTESIAN_POINT('Ctrl Pts',(127.383475506378,31.8607319425041,22.309595887848));
#38069=CARTESIAN_POINT('Ctrl Pts',(127.29488013663,31.9390276831043,22.3038212220981));
#38070=CARTESIAN_POINT('Ctrl Pts',(127.206396987135,32.017224249585,22.2980538708889));
#38071=CARTESIAN_POINT('Ctrl Pts',(127.121181654223,32.0993717724542,22.2922865196798));
#38072=CARTESIAN_POINT('Ctrl Pts',(127.039608898643,32.1851626109122,22.2865191684707));
#38073=CARTESIAN_POINT('Ctrl Pts',(126.958117264671,32.2708681330083,22.2807575527157));
#38074=CARTESIAN_POINT('Ctrl Pts',(126.880261289031,32.3602094655443,22.2749959369607));
#38075=CARTESIAN_POINT('Ctrl Pts',(126.806381191527,32.4528400312956,22.2692343212058));
#38076=CARTESIAN_POINT('Ctrl Pts',(126.732553088089,32.5454054070996,22.2634767602617));
#38077=CARTESIAN_POINT('Ctrl Pts',(126.662695556032,32.6412550877788,22.2577191993177));
#38078=CARTESIAN_POINT('Ctrl Pts',(126.597110128044,32.7400076284779,22.2519616383736));
#38079=CARTESIAN_POINT('Ctrl Pts',(126.531548751071,32.838723955358,22.2462061888008));
#38080=CARTESIAN_POINT('Ctrl Pts',(126.470256594024,32.9403406802227,22.2404507392279));
#38081=CARTESIAN_POINT('Ctrl Pts',(126.413492877873,33.0444459447694,22.234695289655));
#38082=CARTESIAN_POINT('Ctrl Pts',(126.356735998232,33.1485386710813,22.2289405332573));
#38083=CARTESIAN_POINT('Ctrl Pts',(126.304506673963,33.2551189758186,22.2231857768595));
#38084=CARTESIAN_POINT('Ctrl Pts',(126.257018645827,33.3637495355807,22.2174310204618));
#38085=CARTESIAN_POINT('Ctrl Pts',(126.209524641705,33.4723937656241,22.2116755398743));
#38086=CARTESIAN_POINT('Ctrl Pts',(126.166773285702,33.5830883820817,22.2059200592868));
#38087=CARTESIAN_POINT('Ctrl Pts',(126.128930263854,33.6953758786946,22.2001645786993));
#38088=CARTESIAN_POINT('Ctrl Pts',(126.091051218588,33.8077702636893,22.1944036193717));
#38089=CARTESIAN_POINT('Ctrl Pts',(126.058089971145,33.9217601619959,22.1886426600441));
#38090=CARTESIAN_POINT('Ctrl Pts',(126.030162393893,34.0368726038889,22.1828817007166));
#38091=CARTESIAN_POINT('Ctrl Pts',(126.002220875287,34.1520425095357,22.177117865537));
#38092=CARTESIAN_POINT('Ctrl Pts',(125.979318111483,34.2683356667431,22.1713540303574));
#38093=CARTESIAN_POINT('Ctrl Pts',(125.961518545287,34.3852703521541,22.1655901951778));
#38094=CARTESIAN_POINT('Ctrl Pts',(125.943692203765,34.5023809387283,22.1598176896425));
#38095=CARTESIAN_POINT('Ctrl Pts',(125.930984437042,34.6201345674989,22.1540451841073));
#38096=CARTESIAN_POINT('Ctrl Pts',(125.923407691792,34.7380455141447,22.148272678572));
#38097=CARTESIAN_POINT('Ctrl Pts',(125.917769073044,34.8257949174097,22.1439767761942));
#38098=CARTESIAN_POINT('Ctrl Pts',(125.914971102718,34.9136313779439,22.1396808738165));
#38099=CARTESIAN_POINT('Ctrl Pts',(125.915000225098,35.0013561159219,22.1353849714387));
#38100=CARTESIAN_POINT('Ctrl Pts',(125.915000225098,35.0013561166197,22.1353849714045));
#38101=CARTESIAN_POINT('Ctrl Pts',(125.915025803142,35.078404287374,22.1316119031962));
#38102=CARTESIAN_POINT('Ctrl Pts',(125.917231078305,35.1554131039327,22.1278388349879));
#38103=CARTESIAN_POINT('Ctrl Pts',(125.921610227948,35.2322969376113,22.1240657667795));
#38104=CARTESIAN_POINT('Ctrl Pts',(125.928369286289,35.3509643410231,22.118242173109));
#38105=CARTESIAN_POINT('Ctrl Pts',(125.940322775489,35.4695278608721,22.1124185794384));
#38106=CARTESIAN_POINT('Ctrl Pts',(125.957467056685,35.5874967252762,22.1065949857679));
#38107=CARTESIAN_POINT('Ctrl Pts',(125.974589707823,35.7053167544351,22.1007787394258));
#38108=CARTESIAN_POINT('Ctrl Pts',(125.99689006703,35.8225432198411,22.0949624930836));
#38109=CARTESIAN_POINT('Ctrl Pts',(126.024312538453,35.9386874922439,22.0891462467415));
#38110=CARTESIAN_POINT('Ctrl Pts',(126.05170755983,36.0547155035892,22.0833358224941));
#38111=CARTESIAN_POINT('Ctrl Pts',(126.084214400078,36.1696630818593,22.0775253982467));
#38112=CARTESIAN_POINT('Ctrl Pts',(126.121726014142,36.2830494497948,22.0717149739992));
#38113=CARTESIAN_POINT('Ctrl Pts',(126.160657520395,36.400727726305,22.0656846131747));
#38114=CARTESIAN_POINT('Ctrl Pts',(126.204980104197,36.5167238235885,22.0596542523502));
#38115=CARTESIAN_POINT('Ctrl Pts',(126.254516398774,36.6305145178578,22.0536238915257));
#38116=CARTESIAN_POINT('Ctrl Pts',(126.302192305306,36.7400316820007,22.0478200072933));
#38117=CARTESIAN_POINT('Ctrl Pts',(126.354697194334,36.8475057002338,22.042016123061));
#38118=CARTESIAN_POINT('Ctrl Pts',(126.411823279439,36.9524888788482,22.0362122388286));
#38119=CARTESIAN_POINT('Ctrl Pts',(126.468940926411,37.0574565503245,22.0304092118921));
#38120=CARTESIAN_POINT('Ctrl Pts',(126.530678216865,37.1599337552884,22.0246061849555));
#38121=CARTESIAN_POINT('Ctrl Pts',(126.596781231034,37.259497070269,22.0188031580189));
#38122=CARTESIAN_POINT('Ctrl Pts',(126.662890081407,37.3590691756493,22.0129996187357));
#38123=CARTESIAN_POINT('Ctrl Pts',(126.733365195989,37.4557265393365,22.0071960794525));
#38124=CARTESIAN_POINT('Ctrl Pts',(126.807909486028,37.5490749597867,22.0013925401693));
#38125=CARTESIAN_POINT('Ctrl Pts',(126.882477949912,37.6424536520411,21.995587118866));
#38126=CARTESIAN_POINT('Ctrl Pts',(126.961117958937,37.7325209480832,21.9897816975627));
#38127=CARTESIAN_POINT('Ctrl Pts',(127.043492762843,37.8189164508089,21.9839762762594));
#38128=CARTESIAN_POINT('Ctrl Pts',(127.125958789221,37.9054076285574,21.9781644259893));
#38129=CARTESIAN_POINT('Ctrl Pts',(127.212167584224,37.9882186008555,21.9723525757192));
#38130=CARTESIAN_POINT('Ctrl Pts',(127.301746120356,38.0670264102195,21.9665407254491));
#38131=CARTESIAN_POINT('Ctrl Pts',(127.391383492151,38.1458859809759,21.9607250579246));
#38132=CARTESIAN_POINT('Ctrl Pts',(127.48439469546,38.2207368970648,21.9549093904001));
#38133=CARTESIAN_POINT('Ctrl Pts',(127.580375599856,38.2912980360687,21.9490937228755));
#38134=CARTESIAN_POINT('Ctrl Pts',(127.676493986535,38.3619602462851,21.9432697250352));
#38135=CARTESIAN_POINT('Ctrl Pts',(127.775590226523,38.4283201886456,21.9374457271949));
#38136=CARTESIAN_POINT('Ctrl Pts',(127.877233255863,38.4901413080254,21.9316217293546));
#38137=CARTESIAN_POINT('Ctrl Pts',(127.904199705734,38.5065427880636,21.9300765909734));
#38138=CARTESIAN_POINT('Ctrl Pts',(127.931345296024,38.5226250517945,21.9285314525923));
#38139=CARTESIAN_POINT('Ctrl Pts',(127.958661730927,38.5383842458413,21.9269863142111));
#38140=CARTESIAN_POINT('Ctrl Pts',(128.061616792656,38.5977803127745,21.9211627205402));
#38141=CARTESIAN_POINT('Ctrl Pts',(128.167332366969,38.6527749624344,21.9153391268693));
#38142=CARTESIAN_POINT('Ctrl Pts',(128.275395991734,38.703102214991,21.9095155331985));
#38143=CARTESIAN_POINT('Ctrl Pts',(128.383323278184,38.753365972243,21.903699286856));
#38144=CARTESIAN_POINT('Ctrl Pts',(128.493592356013,38.798973873836,21.8978830405136));
#38145=CARTESIAN_POINT('Ctrl Pts',(128.605764074193,38.8397045697801,21.8920667941712));
#38146=CARTESIAN_POINT('Ctrl Pts',(128.717823507865,38.8803944940726,21.8862563699235));
#38147=CARTESIAN_POINT('Ctrl Pts',(128.831781411403,38.916216786502,21.8804459456757));
#38148=CARTESIAN_POINT('Ctrl Pts',(128.947176998382,38.9469974318795,21.874635521428));
#38149=CARTESIAN_POINT('Ctrl Pts',(129.066940547024,38.9789431883545,21.8686051606036));
#38150=CARTESIAN_POINT('Ctrl Pts',(129.188252361852,39.0054578937423,21.8625747997792));
#38151=CARTESIAN_POINT('Ctrl Pts',(129.310577607581,39.026403080273,21.8565444389548));
#38152=CARTESIAN_POINT('Ctrl Pts',(129.428308799066,39.0465616481256,21.8507405547222));
#38153=CARTESIAN_POINT('Ctrl Pts',(129.546978234583,39.061561416186,21.8449366704896));
#38154=CARTESIAN_POINT('Ctrl Pts',(129.666097575086,39.0713307616351,21.839132786257));
#38155=CARTESIAN_POINT('Ctrl Pts',(129.785199320388,39.0810986640474,21.8333297593201));
#38156=CARTESIAN_POINT('Ctrl Pts',(129.904750431655,39.0856376469167,21.8275267323833));
#38157=CARTESIAN_POINT('Ctrl Pts',(130.024257580145,39.0849279760854,21.8217237054465));
#38158=CARTESIAN_POINT('Ctrl Pts',(130.143775279867,39.0842182425977,21.815920166163));
#38159=CARTESIAN_POINT('Ctrl Pts',(130.263248600746,39.0782589364807,21.8101166268796));
#38160=CARTESIAN_POINT('Ctrl Pts',(130.382184990753,39.0670824472641,21.8043130875962));
#38161=CARTESIAN_POINT('Ctrl Pts',(130.501159950443,39.0559023336424,21.7985076662927));
#38162=CARTESIAN_POINT('Ctrl Pts',(130.619597226639,39.0395017103539,21.7927022449891));
#38163=CARTESIAN_POINT('Ctrl Pts',(130.737010799373,39.0179646690342,21.7868968236856));
#38164=CARTESIAN_POINT('Ctrl Pts',(130.854554396771,38.9964037774347,21.7810849734153));
#38165=CARTESIAN_POINT('Ctrl Pts',(130.971071625958,38.9696951875696,21.7752731231451));
#38166=CARTESIAN_POINT('Ctrl Pts',(131.086087894525,38.9379738553431,21.7694612728748));
#38167=CARTESIAN_POINT('Ctrl Pts',(131.201179706396,38.9062316883752,21.7636456053501));
#38168=CARTESIAN_POINT('Ctrl Pts',(131.31476820672,38.8694703475989,21.7578299378253));
#38169=CARTESIAN_POINT('Ctrl Pts',(131.426396743239,38.8278737349704,21.7520142703006));
#38170=CARTESIAN_POINT('Ctrl Pts',(131.538185175584,38.7862175396861,21.7461902724601));
#38171=CARTESIAN_POINT('Ctrl Pts',(131.648007665954,38.7397124072811,21.7403662746196));
#38172=CARTESIAN_POINT('Ctrl Pts',(131.755430072909,38.6885891963088,21.7345422767792));
#38173=CARTESIAN_POINT('Ctrl Pts',(131.783929823129,38.6750259297199,21.7329971384003));
#38174=CARTESIAN_POINT('Ctrl Pts',(131.812260788293,38.6611378525022,21.7314520000215));
#38175=CARTESIAN_POINT('Ctrl Pts',(131.840415198091,38.6469297907468,21.7299068616426));
#38176=CARTESIAN_POINT('Ctrl Pts',(131.946546836177,38.5933706900952,21.7240822654818));
#38177=CARTESIAN_POINT('Ctrl Pts',(132.050509721288,38.535088452653,21.7182576693209));
#38178=CARTESIAN_POINT('Ctrl Pts',(132.151855068785,38.4722823564543,21.71243307316));
#38179=CARTESIAN_POINT('Ctrl Pts',(132.253060538413,38.4095629458616,21.7066165161654));
#38180=CARTESIAN_POINT('Ctrl Pts',(132.351655314935,38.3423323141637,21.7007999591708));
#38181=CARTESIAN_POINT('Ctrl Pts',(132.447213477525,38.2708364672387,21.6949834021762));
#38182=CARTESIAN_POINT('Ctrl Pts',(132.460589047044,38.2608289739493,21.6941692408284));
#38183=CARTESIAN_POINT('Ctrl Pts',(132.473905160772,38.250737988423,21.6933550794807));
#38184=CARTESIAN_POINT('Ctrl Pts',(132.487160689988,38.2405642567579,21.6925409181329));
#38185=CARTESIAN_POINT('',(125.915000722565,34.9975703175708,22.2396150286373));
#38186=CARTESIAN_POINT('Ctrl Pts',(125.915000722565,34.9975703184334,22.2396150285955));
#38187=CARTESIAN_POINT('Ctrl Pts',(125.914929010373,35.1181393078882,22.233766442302));
#38188=CARTESIAN_POINT('Ctrl Pts',(125.920199535175,35.2387276668891,22.2279178560086));
#38189=CARTESIAN_POINT('Ctrl Pts',(125.930790852349,35.35883410188,22.2220692697151));
#38190=CARTESIAN_POINT('Ctrl Pts',(125.941383317302,35.4789535527799,22.2162200496116));
#38191=CARTESIAN_POINT('Ctrl Pts',(125.957297687507,35.598590577951,22.2103708295081));
#38192=CARTESIAN_POINT('Ctrl Pts',(125.978460616567,35.7172489020554,22.2045216094045));
#38193=CARTESIAN_POINT('Ctrl Pts',(125.999630529126,35.8359463819032,22.1986704591325));
#38194=CARTESIAN_POINT('Ctrl Pts',(126.026052377496,35.9536641249839,22.1928193088604));
#38195=CARTESIAN_POINT('Ctrl Pts',(126.057601774297,36.069916459344,22.1869681585884));
#38196=CARTESIAN_POINT('Ctrl Pts',(126.089190817938,36.1863148832701,22.1811096554145));
#38197=CARTESIAN_POINT('Ctrl Pts',(126.12592017732,36.3012438337314,22.1752511522406));
#38198=CARTESIAN_POINT('Ctrl Pts',(126.167615514836,36.4142327099436,22.1693926490667));
#38199=CARTESIAN_POINT('Ctrl Pts',(126.209337132695,36.5272928024257,22.1635304533103));
#38200=CARTESIAN_POINT('Ctrl Pts',(126.256030811639,36.6384100158507,22.157668257554));
#38201=CARTESIAN_POINT('Ctrl Pts',(126.307474687367,36.7471353169011,22.1518060617976));
#38202=CARTESIAN_POINT('Ctrl Pts',(126.359011363293,36.8560567487707,22.145933291159));
#38203=CARTESIAN_POINT('Ctrl Pts',(126.415315175186,36.9625772912076,22.1400605205204));
#38204=CARTESIAN_POINT('Ctrl Pts',(126.476118646655,37.0662732654585,22.1341877498818));
#38205=CARTESIAN_POINT('Ctrl Pts',(126.536050842732,37.1684833418082,22.128399132342));
#38206=CARTESIAN_POINT('Ctrl Pts',(126.600354320997,37.2679490084583,22.1226105148022));
#38207=CARTESIAN_POINT('Ctrl Pts',(126.668734188096,37.3642954744359,22.1168218972623));
#38208=CARTESIAN_POINT('Ctrl Pts',(126.73752722176,37.461224087471,22.110998303591));
#38209=CARTESIAN_POINT('Ctrl Pts',(126.81066514483,37.5553040447173,22.1051747099196));
#38210=CARTESIAN_POINT('Ctrl Pts',(126.887884046831,37.6461215569259,22.0993511162483));
#38211=CARTESIAN_POINT('Ctrl Pts',(126.965005525716,37.736824489353,22.0935348699054));
#38212=CARTESIAN_POINT('Ctrl Pts',(127.046197480592,37.8242728551419,22.0877186235625));
#38213=CARTESIAN_POINT('Ctrl Pts',(127.131153127974,37.9080822933454,22.0819023772196));
#38214=CARTESIAN_POINT('Ctrl Pts',(127.216023734286,37.9918078378393,22.0760919529713));
#38215=CARTESIAN_POINT('Ctrl Pts',(127.304650249154,38.0719014161008,22.0702815287231));
#38216=CARTESIAN_POINT('Ctrl Pts',(127.396686480553,38.1480126618971,22.0644711044748));
#38217=CARTESIAN_POINT('Ctrl Pts',(127.492206473676,38.2270048757737,22.0584407436506));
#38218=CARTESIAN_POINT('Ctrl Pts',(127.591399122868,38.3017069799212,22.0524103828264));
#38219=CARTESIAN_POINT('Ctrl Pts',(127.693836109116,38.3717700260225,22.0463800220022));
#38220=CARTESIAN_POINT('Ctrl Pts',(127.792425965794,38.4392017801822,22.0405761377691));
#38221=CARTESIAN_POINT('Ctrl Pts',(127.894020497764,38.502336390691,22.034772253536));
#38222=CARTESIAN_POINT('Ctrl Pts',(127.998205759725,38.5609050562464,22.0289683693028));
#38223=CARTESIAN_POINT('Ctrl Pts',(128.102375632408,38.6194650705837,22.0231653423655));
#38224=CARTESIAN_POINT('Ctrl Pts',(128.209135118203,38.6734602811682,22.0173623154281));
#38225=CARTESIAN_POINT('Ctrl Pts',(128.318044091939,38.722666963796,22.0115592884908));
#38226=CARTESIAN_POINT('Ctrl Pts',(128.426962681199,38.7718779908594,22.0057557492068));
#38227=CARTESIAN_POINT('Ctrl Pts',(128.538030763587,38.8162994812468,21.9999522099228));
#38228=CARTESIAN_POINT('Ctrl Pts',(128.650787176773,38.8557554068741,21.9941486706389));
#38229=CARTESIAN_POINT('Ctrl Pts',(128.763580155547,38.8952241275978,21.9883432493348));
#38230=CARTESIAN_POINT('Ctrl Pts',(128.878062168761,38.9297239462904,21.9825378280307));
#38231=CARTESIAN_POINT('Ctrl Pts',(128.993756423475,38.9591285486457,21.9767324067267));
#38232=CARTESIAN_POINT('Ctrl Pts',(129.109578798867,38.9885657138764,21.9709205564559));
#38233=CARTESIAN_POINT('Ctrl Pts',(129.226615699405,39.0128962992518,21.9651087061851));
#38234=CARTESIAN_POINT('Ctrl Pts',(129.344379500267,39.032044984909,21.9592968559143));
#38235=CARTESIAN_POINT('Ctrl Pts',(129.462220649026,39.0512062475257,21.953481188389));
#38236=CARTESIAN_POINT('Ctrl Pts',(129.580789244328,39.0651787845898,21.9476655208637));
#38237=CARTESIAN_POINT('Ctrl Pts',(129.699593548546,39.0739392440149,21.9418498533385));
#38238=CARTESIAN_POINT('Ctrl Pts',(129.818568027101,39.0827122518522,21.9360258554975));
#38239=CARTESIAN_POINT('Ctrl Pts',(129.937778481751,39.0862582687448,21.9302018576565));
#38240=CARTESIAN_POINT('Ctrl Pts',(130.056734045959,39.0846060089107,21.9243778598155));
#38241=CARTESIAN_POINT('Ctrl Pts',(130.088293605571,39.0841676553702,21.9228327214416));
#38242=CARTESIAN_POINT('Ctrl Pts',(130.119835259209,39.08336369314,21.9212875830677));
#38243=CARTESIAN_POINT('Ctrl Pts',(130.151349931726,39.0821952670305,21.9197424446939));
#38244=CARTESIAN_POINT('Ctrl Pts',(130.27011093384,39.0777921289183,21.9139196908137));
#38245=CARTESIAN_POINT('Ctrl Pts',(130.388871112726,39.0681950208969,21.9080969369335));
#38246=CARTESIAN_POINT('Ctrl Pts',(130.507139933391,39.0533978447668,21.9022741830533));
#38247=CARTESIAN_POINT('Ctrl Pts',(130.62526825698,39.0386182468959,21.8964583462954));
#38248=CARTESIAN_POINT('Ctrl Pts',(130.742905981608,39.0186509139388,21.8906425095375));
#38249=CARTESIAN_POINT('Ctrl Pts',(130.859563574334,38.9935417190357,21.8848266727795));
#38250=CARTESIAN_POINT('Ctrl Pts',(130.976110128426,38.9684564239118,21.8790163717313));
#38251=CARTESIAN_POINT('Ctrl Pts',(131.09167800926,38.9382390860377,21.8732060706831));
#38252=CARTESIAN_POINT('Ctrl Pts',(131.205784439578,38.9029871746231,21.8673957696348));
#38253=CARTESIAN_POINT('Ctrl Pts',(131.321068741101,38.8673713730115,21.8615254913681));
#38254=CARTESIAN_POINT('Ctrl Pts',(131.434860828287,38.8266165141782,21.8556552131014));
#38255=CARTESIAN_POINT('Ctrl Pts',(131.546674680978,38.7808758814883,21.8497849348347));
#38256=CARTESIAN_POINT('Ctrl Pts',(131.657218090426,38.7356549596963,21.8439813554178));
#38257=CARTESIAN_POINT('Ctrl Pts',(131.765827603802,38.6855611445331,21.8381777760008));
#38258=CARTESIAN_POINT('Ctrl Pts',(131.872050999628,38.6307919321813,21.8323741965839));
#38259=CARTESIAN_POINT('Ctrl Pts',(131.98010558733,38.5750785498944,21.8264705688923));
#38260=CARTESIAN_POINT('Ctrl Pts',(132.085690620244,38.5145272308984,21.8205669412007));
#38261=CARTESIAN_POINT('Ctrl Pts',(132.188354536684,38.4493955154161,21.8146633135091));
#38262=CARTESIAN_POINT('Ctrl Pts',(132.291018453125,38.3842637999337,21.8087596858175));
#38263=CARTESIAN_POINT('Ctrl Pts',(132.390760881023,38.3145519318612,21.8028560581259));
#38264=CARTESIAN_POINT('Ctrl Pts',(132.487160689988,38.2405642567579,21.7969524304342));
#38265=CARTESIAN_POINT('Ctrl Pts',(132.487160689988,38.2405642567579,23.046779218902));
#38266=CARTESIAN_POINT('Ctrl Pts',(132.583414831562,38.1666883826194,23.0408775725951));
#38267=CARTESIAN_POINT('Ctrl Pts',(132.67644286449,38.0884679419452,23.0349759262882));
#38268=CARTESIAN_POINT('Ctrl Pts',(132.765836782572,38.006222196075,23.0290742799813));
#38269=CARTESIAN_POINT('Ctrl Pts',(132.853746494384,37.9253419754465,23.0232706186451));
#38270=CARTESIAN_POINT('Ctrl Pts',(132.938141535144,37.8405693820216,23.0174669573089));
#38271=CARTESIAN_POINT('Ctrl Pts',(133.018667715259,37.752248212799,23.0116632959726));
#38272=CARTESIAN_POINT('Ctrl Pts',(133.099184950673,37.6639368541298,23.0058602792965));
#38273=CARTESIAN_POINT('Ctrl Pts',(133.175833905052,37.5720780052852,23.0000572626203));
#38274=CARTESIAN_POINT('Ctrl Pts',(133.24829854086,37.4770509864441,22.9942542459441));
#38275=CARTESIAN_POINT('Ctrl Pts',(133.320772229082,37.3820120966564,22.9884505043446));
#38276=CARTESIAN_POINT('Ctrl Pts',(133.389060311758,37.2838045746224,22.9826467627452));
#38277=CARTESIAN_POINT('Ctrl Pts',(133.452888595304,37.1828388278622,22.9768430211457));
#38278=CARTESIAN_POINT('Ctrl Pts',(133.518603378227,37.0788889523138,22.9708677450115));
#38279=CARTESIAN_POINT('Ctrl Pts',(133.579590382795,36.9720156591103,22.9648924688774));
#38280=CARTESIAN_POINT('Ctrl Pts',(133.635600513666,36.8626953333903,22.9589171927433));
#38281=CARTESIAN_POINT('Ctrl Pts',(133.690084473718,36.7563537811241,22.9531047316557));
#38282=CARTESIAN_POINT('Ctrl Pts',(133.739859158313,36.6476972275852,22.9472922705682));
#38283=CARTESIAN_POINT('Ctrl Pts',(133.784744135206,36.5371847094689,22.9414798094807));
#38284=CARTESIAN_POINT('Ctrl Pts',(133.831515047203,36.4220287794182,22.9354231258233));
#38285=CARTESIAN_POINT('Ctrl Pts',(133.872976214816,36.3048579910485,22.9293664421658));
#38286=CARTESIAN_POINT('Ctrl Pts',(133.908981333389,36.1862082174812,22.9233097585084));
#38287=CARTESIAN_POINT('Ctrl Pts',(133.944986451961,36.0675584439138,22.917253074851));
#38288=CARTESIAN_POINT('Ctrl Pts',(133.975535466143,35.9474301811147,22.9111963911935));
#38289=CARTESIAN_POINT('Ctrl Pts',(134.00054240192,35.8263688585874,22.9051397075361));
#38290=CARTESIAN_POINT('Ctrl Pts',(134.024586951902,35.7099665513837,22.8993161138646));
#38291=CARTESIAN_POINT('Ctrl Pts',(134.043585686199,35.5923262426363,22.8934925201932));
#38292=CARTESIAN_POINT('Ctrl Pts',(134.057415670364,35.4739230716969,22.8876689265217));
#38293=CARTESIAN_POINT('Ctrl Pts',(134.071228205949,35.355669283945,22.8818526801787));
#38294=CARTESIAN_POINT('Ctrl Pts',(134.079884914853,35.236654950324,22.8760364338357));
#38295=CARTESIAN_POINT('Ctrl Pts',(134.083313617438,35.1173665269401,22.8702201874926));
#38296=CARTESIAN_POINT('Ctrl Pts',(134.086738887873,34.9981975119262,22.8644097632443));
#38297=CARTESIAN_POINT('Ctrl Pts',(134.084946551254,34.8787553587877,22.8585993389959));
#38298=CARTESIAN_POINT('Ctrl Pts',(134.077916163162,34.7595321929578,22.8527889147476));
#38299=CARTESIAN_POINT('Ctrl Pts',(134.070619660339,34.6357961837054,22.8467585539234));
#38300=CARTESIAN_POINT('Ctrl Pts',(134.05768067683,34.5122965127613,22.8407281930993));
#38301=CARTESIAN_POINT('Ctrl Pts',(134.039135779025,34.3895844377817,22.8346978322751));
#38302=CARTESIAN_POINT('Ctrl Pts',(134.021287354509,34.2714809448121,22.8288939480419));
#38303=CARTESIAN_POINT('Ctrl Pts',(133.998246560816,34.1541073966982,22.8230900638086));
#38304=CARTESIAN_POINT('Ctrl Pts',(133.970098817708,34.0379499089793,22.8172861795754));
#38305=CARTESIAN_POINT('Ctrl Pts',(133.941955232323,33.9218095789634,22.8114831526379));
#38306=CARTESIAN_POINT('Ctrl Pts',(133.908706293831,33.806885348869,22.8056801257005));
#38307=CARTESIAN_POINT('Ctrl Pts',(133.870488251105,33.6936517699877,22.799877098763));
#38308=CARTESIAN_POINT('Ctrl Pts',(133.832266834126,33.5804081937656,22.7940735594789));
#38309=CARTESIAN_POINT('Ctrl Pts',(133.789075571222,33.4688559524485,22.7882700201949));
#38310=CARTESIAN_POINT('Ctrl Pts',(133.741099951931,33.3594524847903,22.7824664809108));
#38311=CARTESIAN_POINT('Ctrl Pts',(133.693108774706,33.2500135388629,22.7766610596066));
#38312=CARTESIAN_POINT('Ctrl Pts',(133.640330319395,33.1427251261848,22.7708556383024));
#38313=CARTESIAN_POINT('Ctrl Pts',(133.582997107868,33.0380222414584,22.7650502169982));
#38314=CARTESIAN_POINT('Ctrl Pts',(133.525600405115,32.9332034079791,22.7592383667273));
#38315=CARTESIAN_POINT('Ctrl Pts',(133.463639074184,32.8309761760786,22.7534265164563));
#38316=CARTESIAN_POINT('Ctrl Pts',(133.397390335891,32.7317487119825,22.7476146661854));
#38317=CARTESIAN_POINT('Ctrl Pts',(133.331098085071,32.6324560747552,22.74179899866));
#38318=CARTESIAN_POINT('Ctrl Pts',(133.26051305963,32.5361674577333,22.7359833311347));
#38319=CARTESIAN_POINT('Ctrl Pts',(133.185953312242,32.4432586184335,22.7301676636093));
#38320=CARTESIAN_POINT('Ctrl Pts',(133.111286766067,32.3502166972537,22.7243436657682));
#38321=CARTESIAN_POINT('Ctrl Pts',(133.032634402644,32.2605645223657,22.718519667927));
#38322=CARTESIAN_POINT('Ctrl Pts',(132.950351781855,32.1746417283278,22.7126956700859));
#38323=CARTESIAN_POINT('Ctrl Pts',(132.928521754052,32.1518459427206,22.7111505317131));
#38324=CARTESIAN_POINT('Ctrl Pts',(132.906436386135,32.1293124389526,22.7096053933404));
#38325=CARTESIAN_POINT('Ctrl Pts',(132.884102700967,32.1070470777639,22.7080602549676));
#38326=CARTESIAN_POINT('Ctrl Pts',(132.799927516468,32.0231294048895,22.7022366612962));
#38327=CARTESIAN_POINT('Ctrl Pts',(132.711950970825,31.9427532793061,22.6964130676247));
#38328=CARTESIAN_POINT('Ctrl Pts',(132.620503068697,31.8662819739243,22.6905894739533));
#38329=CARTESIAN_POINT('Ctrl Pts',(132.52917054168,31.7899071484529,22.6847732276102));
#38330=CARTESIAN_POINT('Ctrl Pts',(132.434375679649,31.7174276041057,22.6789569812672));
#38331=CARTESIAN_POINT('Ctrl Pts',(132.336485774206,31.649170367367,22.6731407349242));
#38332=CARTESIAN_POINT('Ctrl Pts',(132.238693857099,31.5809814564991,22.6673303106759));
#38333=CARTESIAN_POINT('Ctrl Pts',(132.137813393001,31.5170066772483,22.6615198864275));
#38334=CARTESIAN_POINT('Ctrl Pts',(132.034244774538,31.4575328939755,22.6557094621792));
#38335=CARTESIAN_POINT('Ctrl Pts',(131.926755869649,31.3958079049927,22.649679101355));
#38336=CARTESIAN_POINT('Ctrl Pts',(131.816371628907,31.3389316760974,22.6436487405309));
#38337=CARTESIAN_POINT('Ctrl Pts',(131.703573152673,31.2871758035839,22.6376183797067));
#38338=CARTESIAN_POINT('Ctrl Pts',(131.595010942742,31.2373636777067,22.6318144954735));
#38339=CARTESIAN_POINT('Ctrl Pts',(131.484212969967,31.1922944287699,22.6260106112402));
#38340=CARTESIAN_POINT('Ctrl Pts',(131.37163263136,31.1521630849803,22.620206727007));
#38341=CARTESIAN_POINT('Ctrl Pts',(131.259068922073,31.1120376690194,22.6144037000696));
#38342=CARTESIAN_POINT('Ctrl Pts',(131.144723755051,31.0768488447679,22.6086006731321));
#38343=CARTESIAN_POINT('Ctrl Pts',(131.02906871797,31.0467427893324,22.6027976461946));
#38344=CARTESIAN_POINT('Ctrl Pts',(130.913403469759,31.0166340758469,22.5969941069106));
#38345=CARTESIAN_POINT('Ctrl Pts',(130.796428516742,30.9916091262824,22.5911905676265));
#38346=CARTESIAN_POINT('Ctrl Pts',(130.678628126101,30.9717635538037,22.5853870283424));
#38347=CARTESIAN_POINT('Ctrl Pts',(130.560789534168,30.9519115456373,22.5795816070382));
#38348=CARTESIAN_POINT('Ctrl Pts',(130.442125374713,30.9372423227259,22.573776185734));
#38349=CARTESIAN_POINT('Ctrl Pts',(130.323126924773,30.927799858739,22.5679707644298));
#38350=CARTESIAN_POINT('Ctrl Pts',(130.203996695066,30.9183469380971,22.5621589141589));
#38351=CARTESIAN_POINT('Ctrl Pts',(130.084531843231,30.914132362345,22.556347063888));
#38352=CARTESIAN_POINT('Ctrl Pts',(129.965225710076,30.9151480138492,22.5505352136171));
#38353=CARTESIAN_POINT('Ctrl Pts',(129.845841216012,30.9161643324387,22.5447195460917));
#38354=CARTESIAN_POINT('Ctrl Pts',(129.726616055079,30.9224176983156,22.5389038785664));
#38355=CARTESIAN_POINT('Ctrl Pts',(129.608038844912,30.9338480779855,22.533088211041));
#38356=CARTESIAN_POINT('Ctrl Pts',(129.489291785694,30.9452948304402,22.5272642131999));
#38357=CARTESIAN_POINT('Ctrl Pts',(129.371194932627,30.9619333408839,22.5214402153588));
#38358=CARTESIAN_POINT('Ctrl Pts',(129.254227251232,30.9836524045852,22.5156162175177));
#38359=CARTESIAN_POINT('Ctrl Pts',(129.223195087787,30.9894145905719,22.5140710791449));
#38360=CARTESIAN_POINT('Ctrl Pts',(129.192242321155,30.9955341090142,22.512525940772));
#38361=CARTESIAN_POINT('Ctrl Pts',(129.161377702766,31.0020082988353,22.5109808023992));
#38362=CARTESIAN_POINT('Ctrl Pts',(129.04504961236,31.0264093826046,22.5051572087277));
#38363=CARTESIAN_POINT('Ctrl Pts',(128.929599802198,31.0559311623785,22.4993336150561));
#38364=CARTESIAN_POINT('Ctrl Pts',(128.815512999794,31.0904967647611,22.4935100213846));
#38365=CARTESIAN_POINT('Ctrl Pts',(128.701570134838,31.125018757502,22.4876937750415));
#38366=CARTESIAN_POINT('Ctrl Pts',(128.588987244671,31.1645717985791,22.4818775286984));
#38367=CARTESIAN_POINT('Ctrl Pts',(128.47823918069,31.2090279599011,22.4760612823553));
#38368=CARTESIAN_POINT('Ctrl Pts',(128.367601976132,31.25343962036,22.4702508581069));
#38369=CARTESIAN_POINT('Ctrl Pts',(128.258796320696,31.3027444858643,22.4644404338585));
#38370=CARTESIAN_POINT('Ctrl Pts',(128.152281620112,31.3567649281685,22.4586300096101));
#38371=CARTESIAN_POINT('Ctrl Pts',(128.041735117801,31.4128301559468,22.452599648786));
#38372=CARTESIAN_POINT('Ctrl Pts',(127.933656860862,31.4739748727617,22.4465692879619));
#38373=CARTESIAN_POINT('Ctrl Pts',(127.828537726293,31.5399455793491,22.4405389271377));
#38374=CARTESIAN_POINT('Ctrl Pts',(127.727366452212,31.6034386861449,22.4347350429044));
#38375=CARTESIAN_POINT('Ctrl Pts',(127.628936419793,31.6714015928606,22.4289311586711));
#38376=CARTESIAN_POINT('Ctrl Pts',(127.533659280729,31.7435619986761,22.4231272744378));
#38377=CARTESIAN_POINT('Ctrl Pts',(127.438396215118,31.815711745628,22.4173242475002));
#38378=CARTESIAN_POINT('Ctrl Pts',(127.346285442125,31.8920575121955,22.4115212205627));
#38379=CARTESIAN_POINT('Ctrl Pts',(127.257707727254,31.9722850050182,22.4057181936251));
#38380=CARTESIAN_POINT('Ctrl Pts',(127.169122191897,32.0525195810893,22.399914654341));
#38381=CARTESIAN_POINT('Ctrl Pts',(127.084070637523,32.1366362906841,22.3941111150568));
#38382=CARTESIAN_POINT('Ctrl Pts',(127.002898489856,32.2242825183578,22.3883075757727));
#38383=CARTESIAN_POINT('Ctrl Pts',(126.921700019009,32.311957168681,22.3825021544684));
#38384=CARTESIAN_POINT('Ctrl Pts',(126.844383734156,32.403163313961,22.3766967331642));
#38385=CARTESIAN_POINT('Ctrl Pts',(126.771255713786,32.4975141690231,22.37089131186));
#38386=CARTESIAN_POINT('Ctrl Pts',(126.698046710902,32.5919695089241,22.365079461589));
#38387=CARTESIAN_POINT('Ctrl Pts',(126.629035480871,32.6895761869886,22.359267611318));
#38388=CARTESIAN_POINT('Ctrl Pts',(126.564485665802,32.7899171374091,22.353455761047));
#38389=CARTESIAN_POINT('Ctrl Pts',(126.499893454068,32.890323992304,22.3476400935216));
#38390=CARTESIAN_POINT('Ctrl Pts',(126.439768698191,32.9934683441391,22.3418244259961));
#38391=CARTESIAN_POINT('Ctrl Pts',(126.384329030281,33.098908619048,22.3360087584707));
#38392=CARTESIAN_POINT('Ctrl Pts',(126.328809951032,33.2044999257654,22.3301847606295));
#38393=CARTESIAN_POINT('Ctrl Pts',(126.27798952769,33.3123933514493,22.3243607627883));
#38394=CARTESIAN_POINT('Ctrl Pts',(126.232037303278,33.4221273447744,22.3185367649471));
#38395=CARTESIAN_POINT('Ctrl Pts',(126.219845927669,33.4512403713306,22.316991626575));
#38396=CARTESIAN_POINT('Ctrl Pts',(126.207996937056,33.4804828693213,22.3154464882029));
#38397=CARTESIAN_POINT('Ctrl Pts',(126.196492903007,33.5098460605958,22.3139013498308));
#38398=CARTESIAN_POINT('Ctrl Pts',(126.147593400052,33.6346584048845,22.3073335234432));
#38399=CARTESIAN_POINT('Ctrl Pts',(126.104798671119,33.7619885269551,22.3007656970556));
#38400=CARTESIAN_POINT('Ctrl Pts',(126.06834304772,33.8912626056695,22.294197870668));
#38401=CARTESIAN_POINT('Ctrl Pts',(126.032001969344,34.0201305000708,22.287650680653));
#38402=CARTESIAN_POINT('Ctrl Pts',(126.001960341605,34.1509299687405,22.281103490638));
#38403=CARTESIAN_POINT('Ctrl Pts',(125.978403669591,34.2830704670304,22.274556300623));
#38404=CARTESIAN_POINT('Ctrl Pts',(125.95498504246,34.414436606382,22.2680474779153));
#38405=CARTESIAN_POINT('Ctrl Pts',(125.937975683312,34.5471279041211,22.2615386552076));
#38406=CARTESIAN_POINT('Ctrl Pts',(125.927510148758,34.6805451338116,22.2550298324999));
#38407=CARTESIAN_POINT('Ctrl Pts',(125.919248328881,34.7858688623325,22.2498915645457));
#38408=CARTESIAN_POINT('Ctrl Pts',(125.915063725241,34.8916445871987,22.2447532965915));
#38409=CARTESIAN_POINT('Ctrl Pts',(125.915000722565,34.9975703175707,22.2396150286373));
#38410=CARTESIAN_POINT('Origin',(130.,35.,32.7603849714045));
#38411=CARTESIAN_POINT('',(132.487160689988,38.2405642567579,24.2969444281512));
#38412=CARTESIAN_POINT('',(132.487160689988,38.2405642567579,24.1926561440539));
#38413=CARTESIAN_POINT('',(132.487160689988,38.2405642567579,32.7603849714045));
#38414=CARTESIAN_POINT('',(125.915000507333,35.0020359057478,23.3853849713659));
#38415=CARTESIAN_POINT('Ctrl Pts',(132.487160689988,38.2405642567579,24.1926561440539));
#38416=CARTESIAN_POINT('Ctrl Pts',(132.581972335864,38.1677955103636,24.1868529351341));
#38417=CARTESIAN_POINT('Ctrl Pts',(132.673586459642,38.0908633554204,24.1810497262143));
#38418=CARTESIAN_POINT('Ctrl Pts',(132.761628091852,38.0100889160108,24.1752465172945));
#38419=CARTESIAN_POINT('Ctrl Pts',(132.849691138964,37.9292948293431,24.1694418968249));
#38420=CARTESIAN_POINT('Ctrl Pts',(132.934179665622,37.844656875635,24.1636372763553));
#38421=CARTESIAN_POINT('Ctrl Pts',(133.014754852225,37.7565337257115,24.1578326558858));
#38422=CARTESIAN_POINT('Ctrl Pts',(133.095416153948,37.668316393746,24.1520218317));
#38423=CARTESIAN_POINT('Ctrl Pts',(133.172155488284,37.5766067295761,24.1462110075143));
#38424=CARTESIAN_POINT('Ctrl Pts',(133.244673577683,37.4817974079864,24.1404001833285));
#38425=CARTESIAN_POINT('Ctrl Pts',(133.317234025714,37.3869327072038,24.1345859649749));
#38426=CARTESIAN_POINT('Ctrl Pts',(133.385568083947,37.28896507707,24.1287717466213));
#38427=CARTESIAN_POINT('Ctrl Pts',(133.449420133897,37.1883157313022,24.1229575282677));
#38428=CARTESIAN_POINT('Ctrl Pts',(133.513369630861,37.0875127807842,24.1171344366169));
#38429=CARTESIAN_POINT('Ctrl Pts',(133.572823255309,36.984020294514,24.1113113449661));
#38430=CARTESIAN_POINT('Ctrl Pts',(133.627571432369,36.8782839250383,24.1054882533153));
#38431=CARTESIAN_POINT('Ctrl Pts',(133.660879138846,36.8139560122651,24.1019455996981));
#38432=CARTESIAN_POINT('Ctrl Pts',(133.692446166234,36.7487979930244,24.098402946081));
#38433=CARTESIAN_POINT('Ctrl Pts',(133.722234217902,36.6829133747994,24.0948602924639));
#38434=CARTESIAN_POINT('Ctrl Pts',(133.771201327851,36.5746088982088,24.0890366987924));
#38435=CARTESIAN_POINT('Ctrl Pts',(133.81551653434,36.4639908317772,24.0832131051209));
#38436=CARTESIAN_POINT('Ctrl Pts',(133.854955774648,36.3514958288903,24.0773895114494));
#38437=CARTESIAN_POINT('Ctrl Pts',(133.894345256496,36.2391427551591,24.0715732651064));
#38438=CARTESIAN_POINT('Ctrl Pts',(133.928870873956,36.1249178368819,24.0657570187633));
#38439=CARTESIAN_POINT('Ctrl Pts',(133.958355605775,36.0092798909276,24.0599407724203));
#38440=CARTESIAN_POINT('Ctrl Pts',(133.987810823214,35.8937576991956,24.0541303481719));
#38441=CARTESIAN_POINT('Ctrl Pts',(134.012235093006,35.7768256870598,24.0483199239236));
#38442=CARTESIAN_POINT('Ctrl Pts',(134.03150062945,35.6589595395331,24.0425094996752));
#38443=CARTESIAN_POINT('Ctrl Pts',(134.051495406297,35.5366319145338,24.0364791388511));
#38444=CARTESIAN_POINT('Ctrl Pts',(134.065933047646,35.4132984619357,24.0304487780269));
#38445=CARTESIAN_POINT('Ctrl Pts',(134.074728435545,35.2895050544698,24.0244184172028));
#38446=CARTESIAN_POINT('Ctrl Pts',(134.08319350333,35.1703608396006,24.0186145329695));
#38447=CARTESIAN_POINT('Ctrl Pts',(134.086432445026,35.05079103895,24.0128106487363));
#38448=CARTESIAN_POINT('Ctrl Pts',(134.084422083151,34.9312886714402,24.007006764503));
#38449=CARTESIAN_POINT('Ctrl Pts',(134.082412018227,34.8118039557081,24.0012037375655));
#38450=CARTESIAN_POINT('Ctrl Pts',(134.075154198583,34.6923870614772,23.995400710628));
#38451=CARTESIAN_POINT('Ctrl Pts',(134.062677574554,34.5735308625269,23.9895976836906));
#38452=CARTESIAN_POINT('Ctrl Pts',(134.050199848969,34.4546641698173,23.9837941444065));
#38453=CARTESIAN_POINT('Ctrl Pts',(134.032502445518,34.3363586769388,23.9779906051224));
#38454=CARTESIAN_POINT('Ctrl Pts',(134.009666108294,34.2191013510092,23.9721870658384));
#38455=CARTESIAN_POINT('Ctrl Pts',(133.986822365513,34.1018059998969,23.9663816445342));
#38456=CARTESIAN_POINT('Ctrl Pts',(133.958836452693,33.9855598923348,23.9605762232301));
#38457=CARTESIAN_POINT('Ctrl Pts',(133.925839921305,33.870838402935,23.9547708019259));
#38458=CARTESIAN_POINT('Ctrl Pts',(133.892806849312,33.7559898701031,23.948958951655));
#38459=CARTESIAN_POINT('Ctrl Pts',(133.854752195816,33.6426697182315,23.943147101384));
#38460=CARTESIAN_POINT('Ctrl Pts',(133.811857003736,33.5313369402508,23.9373352511131));
#38461=CARTESIAN_POINT('Ctrl Pts',(133.768933637862,33.4199310383039,23.9315195835877));
#38462=CARTESIAN_POINT('Ctrl Pts',(133.721163564774,33.3105154831865,23.9257039160623));
#38463=CARTESIAN_POINT('Ctrl Pts',(133.668774768513,33.2035265941507,23.9198882485369));
#38464=CARTESIAN_POINT('Ctrl Pts',(133.616310930958,33.0963844550843,23.9140642506958));
#38465=CARTESIAN_POINT('Ctrl Pts',(133.559215360203,32.9916762771116,23.9082402528546));
#38466=CARTESIAN_POINT('Ctrl Pts',(133.497760551462,32.8898113533061,23.9024162550135));
#38467=CARTESIAN_POINT('Ctrl Pts',(133.481456255726,32.8627860337759,23.9008711166408));
#38468=CARTESIAN_POINT('Ctrl Pts',(133.464845352462,32.8359606696453,23.8993259782681));
#38469=CARTESIAN_POINT('Ctrl Pts',(133.447933409606,32.8093425181181,23.8977808398955));
#38470=CARTESIAN_POINT('Ctrl Pts',(133.384192656586,32.7090192710078,23.891957246224));
#38471=CARTESIAN_POINT('Ctrl Pts',(133.315966879742,32.6113185160414,23.8861336525526));
#38472=CARTESIAN_POINT('Ctrl Pts',(133.243498460342,32.5166670102944,23.8803100588811));
#38473=CARTESIAN_POINT('Ctrl Pts',(133.171121470617,32.4221349214812,23.8744938125381));
#38474=CARTESIAN_POINT('Ctrl Pts',(133.094512730826,32.3306447514966,23.8686775661951));
#38475=CARTESIAN_POINT('Ctrl Pts',(133.013958945554,32.2425960625046,23.862861319852));
#38476=CARTESIAN_POINT('Ctrl Pts',(132.933485795066,32.1546355107361,23.8570508956037));
#38477=CARTESIAN_POINT('Ctrl Pts',(132.849075729215,32.0701098862198,23.8512404713554));
#38478=CARTESIAN_POINT('Ctrl Pts',(132.761056549753,31.989386818426,23.845430047107));
#38479=CARTESIAN_POINT('Ctrl Pts',(132.669705662293,31.9056082155521,23.8393996862829));
#38480=CARTESIAN_POINT('Ctrl Pts',(132.574467310382,31.8259260824054,23.8333693254587));
#38481=CARTESIAN_POINT('Ctrl Pts',(132.475751387658,31.7507108367356,23.8273389646345));
#38482=CARTESIAN_POINT('Ctrl Pts',(132.380742846018,31.6783203793199,23.8215350804013));
#38483=CARTESIAN_POINT('Ctrl Pts',(132.28251358474,31.6100676123452,23.815731196168));
#38484=CARTESIAN_POINT('Ctrl Pts',(132.181463245575,31.5462421758025,23.8099273119348));
#38485=CARTESIAN_POINT('Ctrl Pts',(132.080427832626,31.4824261669595,23.8041242849973));
#38486=CARTESIAN_POINT('Ctrl Pts',(131.976572515625,31.4230364060209,23.7983212580598));
#38487=CARTESIAN_POINT('Ctrl Pts',(131.8703253895,31.3683188552144,23.7925182311224));
#38488=CARTESIAN_POINT('Ctrl Pts',(131.764068882865,31.3135964734205,23.7867146918383));
#38489=CARTESIAN_POINT('Ctrl Pts',(131.655420510287,31.26354730889,23.7809111525542));
#38490=CARTESIAN_POINT('Ctrl Pts',(131.544831817983,31.2183707672292,23.7751076132702));
#38491=CARTESIAN_POINT('Ctrl Pts',(131.434207263056,31.1731795753427,23.769302191966));
#38492=CARTESIAN_POINT('Ctrl Pts',(131.321641514838,31.1328643031993,23.7634967706618));
#38493=CARTESIAN_POINT('Ctrl Pts',(131.207604274663,31.097575507993,23.7576913493577));
#38494=CARTESIAN_POINT('Ctrl Pts',(131.093440748799,31.0622476337123,23.7518794990868));
#38495=CARTESIAN_POINT('Ctrl Pts',(130.977802868592,31.0319574680796,23.7460676488158));
#38496=CARTESIAN_POINT('Ctrl Pts',(130.861173763619,31.0068051952284,23.7402557985449));
#38497=CARTESIAN_POINT('Ctrl Pts',(130.744468056023,30.9816364022294,23.7344401310195));
#38498=CARTESIAN_POINT('Ctrl Pts',(130.626770228722,30.9616122909336,23.7286244634941));
#38499=CARTESIAN_POINT('Ctrl Pts',(130.508570179098,30.9467813563869,23.7228087959687));
#38500=CARTESIAN_POINT('Ctrl Pts',(130.390200820666,30.931929178128,23.7169847981276));
#38501=CARTESIAN_POINT('Ctrl Pts',(130.271328209624,30.9222850566915,23.7111608002865));
#38502=CARTESIAN_POINT('Ctrl Pts',(130.152444038842,30.917845444496,23.7053368024453));
#38503=CARTESIAN_POINT('Ctrl Pts',(130.120903420317,30.9166675911811,23.7037916640726));
#38504=CARTESIAN_POINT('Ctrl Pts',(130.089361967641,30.9158557838219,23.7022465256998));
#38505=CARTESIAN_POINT('Ctrl Pts',(130.057828802667,30.915409343694,23.700701387327));
#38506=CARTESIAN_POINT('Ctrl Pts',(129.938980974396,30.9137267203452,23.6948777936555));
#38507=CARTESIAN_POINT('Ctrl Pts',(129.81986799618,30.9172327961846,23.6890541999841));
#38508=CARTESIAN_POINT('Ctrl Pts',(129.700979659909,30.9259587831967,23.6832306063126));
#38509=CARTESIAN_POINT('Ctrl Pts',(129.582241318934,30.93467376108,23.6774143599696));
#38510=CARTESIAN_POINT('Ctrl Pts',(129.463727459842,30.94859552172,23.6715981136265));
#38511=CARTESIAN_POINT('Ctrl Pts',(129.345929425908,30.9677032990977,23.6657818672835));
#38512=CARTESIAN_POINT('Ctrl Pts',(129.228249308457,30.9867919494848,23.6599714430351));
#38513=CARTESIAN_POINT('Ctrl Pts',(129.111283991439,31.0110562242926,23.6541610187868));
#38514=CARTESIAN_POINT('Ctrl Pts',(128.995520638518,31.0404234806793,23.6483505945384));
#38515=CARTESIAN_POINT('Ctrl Pts',(128.875375403249,31.070902348462,23.6423202337143));
#38516=CARTESIAN_POINT('Ctrl Pts',(128.75652537064,31.1068781148392,23.6362898728901));
#38517=CARTESIAN_POINT('Ctrl Pts',(128.639505036172,31.1482110061169,23.6302595120659));
#38518=CARTESIAN_POINT('Ctrl Pts',(128.526879524368,31.1879915968636,23.6244556278327));
#38519=CARTESIAN_POINT('Ctrl Pts',(128.415949176261,31.2327340357753,23.6186517435995));
#38520=CARTESIAN_POINT('Ctrl Pts',(128.307175307434,31.2822628441164,23.6128478593662));
#38521=CARTESIAN_POINT('Ctrl Pts',(128.19841750567,31.3317843365228,23.6070448324287));
#38522=CARTESIAN_POINT('Ctrl Pts',(128.091815921246,31.3860906231938,23.6012418054913));
#38523=CARTESIAN_POINT('Ctrl Pts',(127.987810935919,31.4449584854194,23.5954387785538));
#38524=CARTESIAN_POINT('Ctrl Pts',(127.883796768038,31.5038315450616,23.5896352392697));
#38525=CARTESIAN_POINT('Ctrl Pts',(127.782380010443,31.5672667798531,23.5838316999857));
#38526=CARTESIAN_POINT('Ctrl Pts',(127.683974961419,31.6349958364567,23.5780281607016));
#38527=CARTESIAN_POINT('Ctrl Pts',(127.585538000784,31.7027468568034,23.5722227393974));
#38528=CARTESIAN_POINT('Ctrl Pts',(127.490115027274,31.7747942368127,23.5664173180933));
#38529=CARTESIAN_POINT('Ctrl Pts',(127.398089435742,31.8508276618127,23.5606118967891));
#38530=CARTESIAN_POINT('Ctrl Pts',(127.305961934386,31.9269452867933,23.5548000465182));
#38531=CARTESIAN_POINT('Ctrl Pts',(127.217239639832,32.0070575075962,23.5489881962472));
#38532=CARTESIAN_POINT('Ctrl Pts',(127.132271177237,32.0908151658766,23.5431763459763));
#38533=CARTESIAN_POINT('Ctrl Pts',(127.047246906899,32.1746278366364,23.5373606784509));
#38534=CARTESIAN_POINT('Ctrl Pts',(126.965981656005,32.2620904148143,23.5315450109256));
#38535=CARTESIAN_POINT('Ctrl Pts',(126.888784528312,32.3528197475937,23.5257293434002));
#38536=CARTESIAN_POINT('Ctrl Pts',(126.81147682407,32.4436790403455,23.5199053455591));
#38537=CARTESIAN_POINT('Ctrl Pts',(126.738249123527,32.5378141061151,23.5140813477179));
#38538=CARTESIAN_POINT('Ctrl Pts',(126.669367987711,32.6348117625195,23.5082573498768));
#38539=CARTESIAN_POINT('Ctrl Pts',(126.651093446921,32.660545769479,23.506712211504));
#38540=CARTESIAN_POINT('Ctrl Pts',(126.633124599155,32.6864811271597,23.5051670731313));
#38541=CARTESIAN_POINT('Ctrl Pts',(126.615465877015,32.7126098342537,23.5036219347586));
#38542=CARTESIAN_POINT('Ctrl Pts',(126.547946051236,32.8125154637126,23.4977139492936));
#38543=CARTESIAN_POINT('Ctrl Pts',(126.484750138236,32.915565828757,23.4918059638287));
#38544=CARTESIAN_POINT('Ctrl Pts',(126.426178854133,33.0213571779229,23.4858979783637));
#38545=CARTESIAN_POINT('Ctrl Pts',(126.367686936568,33.1270051753913,23.4799979984658));
#38546=CARTESIAN_POINT('Ctrl Pts',(126.313807367996,33.2353864267341,23.474098018568));
#38547=CARTESIAN_POINT('Ctrl Pts',(126.264798248165,33.346067452075,23.4681980386701));
#38548=CARTESIAN_POINT('Ctrl Pts',(126.215845205529,33.4566218340164,23.462304809645));
#38549=CARTESIAN_POINT('Ctrl Pts',(126.171751679285,33.5694703964249,23.4564115806198));
#38550=CARTESIAN_POINT('Ctrl Pts',(126.132730167001,33.6841546296112,23.4505183515946));
#38551=CARTESIAN_POINT('Ctrl Pts',(126.093751609523,33.7987126186111,23.4446316098248));
#38552=CARTESIAN_POINT('Ctrl Pts',(126.059834070599,33.9151018831637,23.438744868055));
#38553=CARTESIAN_POINT('Ctrl Pts',(126.03114191344,34.032844123862,23.4328581262852));
#38554=CARTESIAN_POINT('Ctrl Pts',(126.002468405446,34.1505098351301,23.4269752107462));
#38555=CARTESIAN_POINT('Ctrl Pts',(125.979013612726,34.269526392017,23.4210922952072));
#38556=CARTESIAN_POINT('Ctrl Pts',(125.96089200761,34.3894006012016,23.4152093796682));
#38557=CARTESIAN_POINT('Ctrl Pts',(125.942777952188,34.5092248692456,23.4093289150277));
#38558=CARTESIAN_POINT('Ctrl Pts',(125.929992721259,34.6299056907607,23.4034484503871));
#38559=CARTESIAN_POINT('Ctrl Pts',(125.922599567219,34.7509403469827,23.3975679857466));
#38560=CARTESIAN_POINT('Ctrl Pts',(125.917493910484,34.8345259728802,23.3935069809659));
#38561=CARTESIAN_POINT('Ctrl Pts',(125.914958764663,34.9182801351293,23.3894459761852));
#38562=CARTESIAN_POINT('Ctrl Pts',(125.915000507333,35.0020359049515,23.3853849714045));
#38563=CARTESIAN_POINT('Ctrl Pts',(125.915000507333,35.0020359057478,23.3853849713659));
#38564=CARTESIAN_POINT('Ctrl Pts',(125.915068041878,35.1375424641031,23.3788147639346));
#38565=CARTESIAN_POINT('Ctrl Pts',(125.921882638121,35.2728211146023,23.3722445565033));
#38566=CARTESIAN_POINT('Ctrl Pts',(125.935349060719,35.4072318035249,23.365674349072));
#38567=CARTESIAN_POINT('Ctrl Pts',(125.948524496332,35.5387381011079,23.359246112891));
#38568=CARTESIAN_POINT('Ctrl Pts',(125.968067066153,35.6694133588767,23.35281787671));
#38569=CARTESIAN_POINT('Ctrl Pts',(125.993836675525,35.7986741623662,23.346389640529));
#38570=CARTESIAN_POINT('Ctrl Pts',(126.020459989606,35.9322171633448,23.3397484474725));
#38571=CARTESIAN_POINT('Ctrl Pts',(126.053729887509,36.064250078893,23.333107254416));
#38572=CARTESIAN_POINT('Ctrl Pts',(126.093437848864,36.1941512296656,23.3264660613596));
#38573=CARTESIAN_POINT('Ctrl Pts',(126.13314581022,36.3240523804383,23.3198248683031));
#38574=CARTESIAN_POINT('Ctrl Pts',(126.179291657195,36.4518215248695,23.3131836752466));
#38575=CARTESIAN_POINT('Ctrl Pts',(126.231614536202,36.576862706844,23.3065424821901));
#38576=CARTESIAN_POINT('Ctrl Pts',(126.277495928968,36.6865100292193,23.3007188885187));
#38577=CARTESIAN_POINT('Ctrl Pts',(126.328240832554,36.7943300130216,23.2948952948472));
#38578=CARTESIAN_POINT('Ctrl Pts',(126.38368242305,36.8998610956174,23.2890717011758));
#38579=CARTESIAN_POINT('Ctrl Pts',(126.439054065743,37.0052590350772,23.2832554548327));
#38580=CARTESIAN_POINT('Ctrl Pts',(126.499110421294,37.1083734587737,23.2774392084897));
#38581=CARTESIAN_POINT('Ctrl Pts',(126.563636386211,37.208762122508,23.2716229621467));
#38582=CARTESIAN_POINT('Ctrl Pts',(126.628097760281,37.3090502966359,23.2658125378983));
#38583=CARTESIAN_POINT('Ctrl Pts',(126.697019623523,37.4066177972911,23.26000211365));
#38584=CARTESIAN_POINT('Ctrl Pts',(126.770140972507,37.501046913299,23.2541916894017));
#38585=CARTESIAN_POINT('Ctrl Pts',(126.846030115791,37.5990503666608,23.2481613285775));
#38586=CARTESIAN_POINT('Ctrl Pts',(126.926442736364,37.693672755502,23.2421309677533));
#38587=CARTESIAN_POINT('Ctrl Pts',(127.0110373891,37.7844797558322,23.2361006069292));
#38588=CARTESIAN_POINT('Ctrl Pts',(127.092455000009,37.8718764030399,23.2302967226959));
#38589=CARTESIAN_POINT('Ctrl Pts',(127.177745883189,37.9557387498791,23.2244928384627));
#38590=CARTESIAN_POINT('Ctrl Pts',(127.26656505548,38.0357138211753,23.2186889542294));
#38591=CARTESIAN_POINT('Ctrl Pts',(127.355371108229,38.1156770792981,23.212885927292));
#38592=CARTESIAN_POINT('Ctrl Pts',(127.447704110287,38.1917539306043,23.2070829003545));
#38593=CARTESIAN_POINT('Ctrl Pts',(127.54318365727,38.2636296447502,23.201279873417));
#38594=CARTESIAN_POINT('Ctrl Pts',(127.638671634098,38.33551170477,23.195476334133));
#38595=CARTESIAN_POINT('Ctrl Pts',(127.73730638195,38.4031916445622,23.1896727948489));
#38596=CARTESIAN_POINT('Ctrl Pts',(127.838676519036,38.4663966608907,23.1838692555648));
#38597=CARTESIAN_POINT('Ctrl Pts',(127.940079529276,38.529622173869,23.1780638342607));
#38598=CARTESIAN_POINT('Ctrl Pts',(128.044219346578,38.588369661408,23.1722584129565));
#38599=CARTESIAN_POINT('Ctrl Pts',(128.150658444778,38.6424114007245,23.1664529916523));
#38600=CARTESIAN_POINT('Ctrl Pts',(128.257215414427,38.6965129862652,23.1606411413814));
#38601=CARTESIAN_POINT('Ctrl Pts',(128.366076383177,38.7458982366508,23.1548292911105));
#38602=CARTESIAN_POINT('Ctrl Pts',(128.476782081956,38.7903868106238,23.1490174408395));
#38603=CARTESIAN_POINT('Ctrl Pts',(128.587560492833,38.8349046049311,23.1432017733141));
#38604=CARTESIAN_POINT('Ctrl Pts',(128.700185662412,38.8745191825761,23.1373861057887));
#38605=CARTESIAN_POINT('Ctrl Pts',(128.814182921208,38.9091000058385,23.1315704382634));
#38606=CARTESIAN_POINT('Ctrl Pts',(128.928343468769,38.943730362396,23.1257464404222));
#38607=CARTESIAN_POINT('Ctrl Pts',(129.043879634147,38.9733124722603,23.1199224425811));
#38608=CARTESIAN_POINT('Ctrl Pts',(129.160306188626,38.997766789489,23.11409844474));
#38609=CARTESIAN_POINT('Ctrl Pts',(129.191194788149,39.0042546531456,23.1125533063672));
#38610=CARTESIAN_POINT('Ctrl Pts',(129.222146031754,39.0103818700825,23.1110081679945));
#38611=CARTESIAN_POINT('Ctrl Pts',(129.253150813995,39.0161475686737,23.1094630296217));
#38612=CARTESIAN_POINT('Ctrl Pts',(129.370019603657,39.0378806745759,23.1036388167605));
#38613=CARTESIAN_POINT('Ctrl Pts',(129.488026301745,39.0545433209723,23.0978146038993));
#38614=CARTESIAN_POINT('Ctrl Pts',(129.606693270703,39.066021989204,23.0919903910381));
#38615=CARTESIAN_POINT('Ctrl Pts',(129.725207575949,39.0774858902588,23.0861736709608));
#38616=CARTESIAN_POINT('Ctrl Pts',(129.844380059345,39.0837790401912,23.0803569508835));
#38617=CARTESIAN_POINT('Ctrl Pts',(129.963722808179,39.0848389154719,23.0745402308063));
#38618=CARTESIAN_POINT('Ctrl Pts',(130.082924450889,39.0858975375981,23.0687303881877));
#38619=CARTESIAN_POINT('Ctrl Pts',(130.202295552219,39.0817352005574,23.0629205455691));
#38620=CARTESIAN_POINT('Ctrl Pts',(130.321343825432,39.0723412364212,23.0571107029505));
#38621=CARTESIAN_POINT('Ctrl Pts',(130.440313011482,39.0629535129633,23.0513047199761));
#38622=CARTESIAN_POINT('Ctrl Pts',(130.558959390372,39.0483411060576,23.0454987370016));
#38623=CARTESIAN_POINT('Ctrl Pts',(130.676791649192,39.0285454029443,23.0396927540272));
#38624=CARTESIAN_POINT('Ctrl Pts',(130.794573438413,39.008758178674,23.033889257856));
#38625=CARTESIAN_POINT('Ctrl Pts',(130.911541399292,38.9837921422135,23.0280857616847));
#38626=CARTESIAN_POINT('Ctrl Pts',(131.027210946424,38.9537403394188,23.0222822655135));
#38627=CARTESIAN_POINT('Ctrl Pts',(131.142858248279,38.9236943161113,23.0164798854561));
#38628=CARTESIAN_POINT('Ctrl Pts',(131.257207238654,38.888564576425,23.0106775053986));
#38629=CARTESIAN_POINT('Ctrl Pts',(131.369785731834,38.8484947770346,23.0048751253412));
#38630=CARTESIAN_POINT('Ctrl Pts',(131.482409236858,38.8084089566845,22.9990704253396));
#38631=CARTESIAN_POINT('Ctrl Pts',(131.593260444399,38.7633792645602,22.993265725338));
#38632=CARTESIAN_POINT('Ctrl Pts',(131.701884602901,38.7135984972002,22.9874610253364));
#38633=CARTESIAN_POINT('Ctrl Pts',(131.810531700835,38.6638072170545,22.9816550994886));
#38634=CARTESIAN_POINT('Ctrl Pts',(131.916950446241,38.6092630430451,22.9758491736407));
#38635=CARTESIAN_POINT('Ctrl Pts',(132.020709414015,38.5502054115374,22.9700432477929));
#38636=CARTESIAN_POINT('Ctrl Pts',(132.124565043898,38.4910927617963,22.9642319131304));
#38637=CARTESIAN_POINT('Ctrl Pts',(132.225755598352,38.4274584690791,22.9584205784678));
#38638=CARTESIAN_POINT('Ctrl Pts',(132.323877385381,38.3595861200027,22.9526092438053));
#38639=CARTESIAN_POINT('Ctrl Pts',(132.379306586531,38.3212448891362,22.9493264087927));
#38640=CARTESIAN_POINT('Ctrl Pts',(132.433757053346,38.2815520030995,22.94604357378));
#38641=CARTESIAN_POINT('Ctrl Pts',(132.487160689988,38.2405642567579,22.9427607387674));
#38642=CARTESIAN_POINT('',(125.915000083441,34.9991743389388,23.4896150285496));
#38643=CARTESIAN_POINT('Ctrl Pts',(125.915000083441,34.9991743389388,23.4896150285496));
#38644=CARTESIAN_POINT('Ctrl Pts',(125.914976188112,35.1173976913889,23.4838237303786));
#38645=CARTESIAN_POINT('Ctrl Pts',(125.920088782344,35.2358210967536,23.4780324322077));
#38646=CARTESIAN_POINT('Ctrl Pts',(125.930363891994,35.3539589643083,23.4722411340368));
#38647=CARTESIAN_POINT('Ctrl Pts',(125.940626165892,35.4719492530606,23.4664570704035));
#38648=CARTESIAN_POINT('Ctrl Pts',(125.956038095578,35.5896543051829,23.4606730067702));
#38649=CARTESIAN_POINT('Ctrl Pts',(125.976573711133,35.7065875020528,23.4548889431369));
#38650=CARTESIAN_POINT('Ctrl Pts',(125.997089184842,35.8234060079085,23.4491105526584));
#38651=CARTESIAN_POINT('Ctrl Pts',(126.022718277938,35.9394537594368,23.4433321621799));
#38652=CARTESIAN_POINT('Ctrl Pts',(126.053383190379,36.0542489070512,23.4375537717014));
#38653=CARTESIAN_POINT('Ctrl Pts',(126.0840271413,36.1689655844951,23.4317793311397));
#38654=CARTESIAN_POINT('Ctrl Pts',(126.119699958342,36.2824309630115,23.4260048905781));
#38655=CARTESIAN_POINT('Ctrl Pts',(126.160272822346,36.3941736624924,23.4202304500164));
#38656=CARTESIAN_POINT('Ctrl Pts',(126.200831076437,36.5058761244586,23.4144580887775));
#38657=CARTESIAN_POINT('Ctrl Pts',(126.246285729108,36.6158567524298,23.4086857275385));
#38658=CARTESIAN_POINT('Ctrl Pts',(126.296458370552,36.7236601750191,23.4029133662996));
#38659=CARTESIAN_POINT('Ctrl Pts',(126.346625133143,36.8314509660127,23.3971416814227));
#38660=CARTESIAN_POINT('Ctrl Pts',(126.401508610812,36.9370646841817,23.3913699965457));
#38661=CARTESIAN_POINT('Ctrl Pts',(126.46088288993,37.0400674207511,23.3855983116687));
#38662=CARTESIAN_POINT('Ctrl Pts',(126.520264635338,37.1430831098706,23.3798259010049));
#38663=CARTESIAN_POINT('Ctrl Pts',(126.584138098126,37.2434868066722,23.374053490341));
#38664=CARTESIAN_POINT('Ctrl Pts',(126.652232561365,37.3408712431088,23.3682810796771));
#38665=CARTESIAN_POINT('Ctrl Pts',(126.720394941295,37.4383528097444,23.3625029116724));
#38666=CARTESIAN_POINT('Ctrl Pts',(126.792786493865,37.5328087612892,23.3567247436676));
#38667=CARTESIAN_POINT('Ctrl Pts',(126.869094375303,37.6238626048713,23.3509465756629));
#38668=CARTESIAN_POINT('Ctrl Pts',(126.94543975801,37.7149611965786,23.3451655679956));
#38669=CARTESIAN_POINT('Ctrl Pts',(127.025705024388,37.8026540447933,23.3393845603284));
#38670=CARTESIAN_POINT('Ctrl Pts',(127.109539652372,37.8866007653973,23.3336035526611));
#38671=CARTESIAN_POINT('Ctrl Pts',(127.193510877074,37.9706842653575,23.3278131256562));
#38672=CARTESIAN_POINT('Ctrl Pts',(127.281062779313,38.0510091615353,23.3220226986513));
#38673=CARTESIAN_POINT('Ctrl Pts',(127.37181044764,38.1272743206927,23.3162322716464));
#38674=CARTESIAN_POINT('Ctrl Pts',(127.460271975996,38.2016181871945,23.3105877186552));
#38675=CARTESIAN_POINT('Ctrl Pts',(127.551769842018,38.2721042776296,23.3049431656641));
#38676=CARTESIAN_POINT('Ctrl Pts',(127.645922334694,38.338494173382,23.299298612673));
#38677=CARTESIAN_POINT('Ctrl Pts',(127.743061268699,38.4069899032227,23.2934750190015));
#38678=CARTESIAN_POINT('Ctrl Pts',(127.8433488203,38.4713529449552,23.28765142533));
#38679=CARTESIAN_POINT('Ctrl Pts',(127.946398371878,38.5312809790464,23.2818278316586));
#38680=CARTESIAN_POINT('Ctrl Pts',(128.04931791114,38.5911334050212,23.2760115853155));
#38681=CARTESIAN_POINT('Ctrl Pts',(128.154992169571,38.6465617490467,23.2701953389725));
#38682=CARTESIAN_POINT('Ctrl Pts',(128.263003899946,38.6973057147599,23.2643790926295));
#38683=CARTESIAN_POINT('Ctrl Pts',(128.370907509982,38.7479988854833,23.2585686683812));
#38684=CARTESIAN_POINT('Ctrl Pts',(128.481143569717,38.794016833623,23.2527582441328));
#38685=CARTESIAN_POINT('Ctrl Pts',(128.593268989434,38.8351444384681,23.2469478198845));
#38686=CARTESIAN_POINT('Ctrl Pts',(128.709638588204,38.8778288082233,23.2409174590603));
#38687=CARTESIAN_POINT('Ctrl Pts',(128.828043017951,38.915245075191,23.2348870982362));
#38688=CARTESIAN_POINT('Ctrl Pts',(128.947962219256,38.9472067982166,23.228856737412));
#38689=CARTESIAN_POINT('Ctrl Pts',(129.063377727881,38.9779681648651,23.2230528531788));
#38690=CARTESIAN_POINT('Ctrl Pts',(129.180195852156,39.0036771868587,23.2172489689455));
#38691=CARTESIAN_POINT('Ctrl Pts',(129.297936769711,39.0242182123583,23.2114450847123));
#38692=CARTESIAN_POINT('Ctrl Pts',(129.415660295673,39.0447562037287,23.2056420577748));
#38693=CARTESIAN_POINT('Ctrl Pts',(129.534305941693,39.0601276465444,23.1998390308373));
#38694=CARTESIAN_POINT('Ctrl Pts',(129.653384206569,39.070268110548,23.1940360038998));
#38695=CARTESIAN_POINT('Ctrl Pts',(129.772472984811,39.0804094698486,23.1882324646158));
#38696=CARTESIAN_POINT('Ctrl Pts',(129.891994050966,39.0853188974369,23.1824289253317));
#38697=CARTESIAN_POINT('Ctrl Pts',(130.011453946273,39.0849839420877,23.1766253860476));
#38698=CARTESIAN_POINT('Ctrl Pts',(130.130952581032,39.0846488781165,23.1708199647434));
#38699=CARTESIAN_POINT('Ctrl Pts',(130.250389597366,39.0790660500591,23.1650145434393));
#38700=CARTESIAN_POINT('Ctrl Pts',(130.369273348812,39.0682750882724,23.1592091221351));
#38701=CARTESIAN_POINT('Ctrl Pts',(130.488288753008,39.0574721764943,23.1533972718641));
#38702=CARTESIAN_POINT('Ctrl Pts',(130.606749262428,39.0414496554454,23.1475854215932));
#38703=CARTESIAN_POINT('Ctrl Pts',(130.724169994242,39.020298847031,23.1417735713223));
#38704=CARTESIAN_POINT('Ctrl Pts',(130.841667848624,38.9991341466521,23.1359579037969));
#38705=CARTESIAN_POINT('Ctrl Pts',(130.958124167934,38.9728345406235,23.1301422362715));
#38706=CARTESIAN_POINT('Ctrl Pts',(131.073067492794,38.9415417232231,23.1243265687461));
#38707=CARTESIAN_POINT('Ctrl Pts',(131.188175461555,38.9102040822408,23.118502570905));
#38708=CARTESIAN_POINT('Ctrl Pts',(131.301765722717,38.8738590784098,23.1126785730638));
#38709=CARTESIAN_POINT('Ctrl Pts',(131.413384972727,38.8326972119995,23.1068545752227));
#38710=CARTESIAN_POINT('Ctrl Pts',(131.44299816817,38.8217767444755,23.10530943685));
#38711=CARTESIAN_POINT('Ctrl Pts',(131.472472757078,38.810517487096,23.1037642984772));
#38712=CARTESIAN_POINT('Ctrl Pts',(131.50180056317,38.7989235407499,23.1022191601045));
#38713=CARTESIAN_POINT('Ctrl Pts',(131.612327895283,38.7552295817026,23.0963960166497));
#38714=CARTESIAN_POINT('Ctrl Pts',(131.721124991532,38.7066375787159,23.090572873195));
#38715=CARTESIAN_POINT('Ctrl Pts',(131.827727178123,38.6533051285585,23.0847497297402));
#38716=CARTESIAN_POINT('Ctrl Pts',(131.934210987083,38.6000319020367,23.0789330526623));
#38717=CARTESIAN_POINT('Ctrl Pts',(132.038504368927,38.5420288721397,23.0731163755845));
#38718=CARTESIAN_POINT('Ctrl Pts',(132.140160799598,38.4795023712974,23.0672996985067));
#38719=CARTESIAN_POINT('Ctrl Pts',(132.241707615457,38.4170432919709,23.0614892934764));
#38720=CARTESIAN_POINT('Ctrl Pts',(132.340622792899,38.3500706613965,23.0556788884461));
#38721=CARTESIAN_POINT('Ctrl Pts',(132.436483529595,38.2788371429535,23.0498684834158));
#38722=CARTESIAN_POINT('Ctrl Pts',(132.453472544451,38.2662127114628,23.0488387285779));
#38723=CARTESIAN_POINT('Ctrl Pts',(132.470365686899,38.2534545647911,23.0478089737399));
#38724=CARTESIAN_POINT('Ctrl Pts',(132.487160689988,38.2405642567579,23.046779218902));
#38725=CARTESIAN_POINT('Ctrl Pts',(132.487160689988,38.2405642567579,24.2969444281512));
#38726=CARTESIAN_POINT('Ctrl Pts',(132.553405712622,38.1897206372063,24.2928615772725));
#38727=CARTESIAN_POINT('Ctrl Pts',(132.618025640998,38.1368950920944,24.2887787263938));
#38728=CARTESIAN_POINT('Ctrl Pts',(132.680900483629,38.0822066116468,24.2846958755152));
#38729=CARTESIAN_POINT('Ctrl Pts',(132.770582312949,38.0042014387652,24.2788722818436));
#38730=CARTESIAN_POINT('Ctrl Pts',(132.857001403456,37.9221530692289,24.2730486881721));
#38731=CARTESIAN_POINT('Ctrl Pts',(132.939771970637,37.8363648849645,24.2672250945006));
#38732=CARTESIAN_POINT('Ctrl Pts',(133.022438110453,37.7506849352373,24.2614088481575));
#38733=CARTESIAN_POINT('Ctrl Pts',(133.101464601485,37.6612748467026,24.2555926018144));
#38734=CARTESIAN_POINT('Ctrl Pts',(133.176499167056,37.5684777674127,24.2497763554713));
#38735=CARTESIAN_POINT('Ctrl Pts',(133.251458622613,37.4757735785112,24.2439659312229));
#38736=CARTESIAN_POINT('Ctrl Pts',(133.322433846866,37.3796894593263,24.2381555069745));
#38737=CARTESIAN_POINT('Ctrl Pts',(133.389110273962,37.280604426666,24.232345082726));
#38738=CARTESIAN_POINT('Ctrl Pts',(133.458310541732,37.1777688205781,24.2263147219019));
#38739=CARTESIAN_POINT('Ctrl Pts',(133.522879834287,37.0717009532646,24.2202843610778));
#38740=CARTESIAN_POINT('Ctrl Pts',(133.58251308558,36.9628614295592,24.2142540002536));
#38741=CARTESIAN_POINT('Ctrl Pts',(133.63990674693,36.8581094894984,24.2084501160203));
#38742=CARTESIAN_POINT('Ctrl Pts',(133.692728223576,36.750790713992,24.202646231787));
#38743=CARTESIAN_POINT('Ctrl Pts',(133.740750791123,36.6413435102733,24.1968423475537));
#38744=CARTESIAN_POINT('Ctrl Pts',(133.788766265222,36.531912473077,24.1910393206161));
#38745=CARTESIAN_POINT('Ctrl Pts',(133.831984075877,36.4203540067187,24.1852362936786));
#38746=CARTESIAN_POINT('Ctrl Pts',(133.870224935108,36.3071281313119,24.179433266741));
#38747=CARTESIAN_POINT('Ctrl Pts',(133.908469170607,36.1938922592443,24.1736297274569));
#38748=CARTESIAN_POINT('Ctrl Pts',(133.941735450357,36.0789890723168,24.1678261881727));
#38749=CARTESIAN_POINT('Ctrl Pts',(133.969894022572,35.9628948278725,24.1620226488886));
#38750=CARTESIAN_POINT('Ctrl Pts',(133.998061726284,35.8467629354186,24.1562172275843));
#38751=CARTESIAN_POINT('Ctrl Pts',(134.021118332114,35.7294396139184,24.1504118062801));
#38752=CARTESIAN_POINT('Ctrl Pts',(134.038985099818,35.6114117789552,24.1446063849758));
#38753=CARTESIAN_POINT('Ctrl Pts',(134.056871653315,35.4932532390895,24.1387945347048));
#38754=CARTESIAN_POINT('Ctrl Pts',(134.069556835499,35.3743890324245,24.1329826844338));
#38755=CARTESIAN_POINT('Ctrl Pts',(134.077013719479,35.2553118312562,24.1271708341628));
#38756=CARTESIAN_POINT('Ctrl Pts',(134.084475501181,35.1361564195428,24.1213551666374));
#38757=CARTESIAN_POINT('Ctrl Pts',(134.086702138233,35.0167881420473,24.1155394991119));
#38758=CARTESIAN_POINT('Ctrl Pts',(134.083718823924,34.8976986455048,24.1097238315864));
#38759=CARTESIAN_POINT('Ctrl Pts',(134.080731236339,34.778438566118,24.1038998337452));
#38760=CARTESIAN_POINT('Ctrl Pts',(134.072518830281,34.6594584706342,24.098075835904));
#38761=CARTESIAN_POINT('Ctrl Pts',(134.059158526398,34.5412440108601,24.0922518380628));
#38762=CARTESIAN_POINT('Ctrl Pts',(134.055613964955,34.5098810703326,24.0907066996908));
#38763=CARTESIAN_POINT('Ctrl Pts',(134.051707336022,34.4785719579602,24.0891615613188));
#38764=CARTESIAN_POINT('Ctrl Pts',(134.047440672667,34.4473255920128,24.0876164229467));
#38765=CARTESIAN_POINT('Ctrl Pts',(134.031359709197,34.3295587031176,24.0817928292753));
#38766=CARTESIAN_POINT('Ctrl Pts',(134.010108618132,34.2123043416824,24.0759692356038));
#38767=CARTESIAN_POINT('Ctrl Pts',(133.983729666343,34.0960514696623,24.0701456419324));
#38768=CARTESIAN_POINT('Ctrl Pts',(133.95738399552,33.9799452679082,24.0643293955894));
#38769=CARTESIAN_POINT('Ctrl Pts',(133.925923421333,33.8648384371461,24.0585131492463));
#38770=CARTESIAN_POINT('Ctrl Pts',(133.88944183767,33.7512137126879,24.0526969029033));
#38771=CARTESIAN_POINT('Ctrl Pts',(133.852996772274,33.6377027272058,24.046886478655));
#38772=CARTESIAN_POINT('Ctrl Pts',(133.811540820233,33.5256712831501,24.0410760544067));
#38773=CARTESIAN_POINT('Ctrl Pts',(133.765218546725,33.4155902375328,24.0352656301583));
#38774=CARTESIAN_POINT('Ctrl Pts',(133.717142879353,33.3013423966518,24.0292352693342));
#38775=CARTESIAN_POINT('Ctrl Pts',(133.663825310019,33.189195961943,24.02320490851));
#38776=CARTESIAN_POINT('Ctrl Pts',(133.605483849221,33.079658568637,24.0171745476858));
#38777=CARTESIAN_POINT('Ctrl Pts',(133.549333463805,32.97423496821,24.0113706634526));
#38778=CARTESIAN_POINT('Ctrl Pts',(133.488529946166,32.8712283654428,24.0055667792194));
#38779=CARTESIAN_POINT('Ctrl Pts',(133.423315685409,32.7710687049548,23.9997628949861));
#38780=CARTESIAN_POINT('Ctrl Pts',(133.358111057495,32.6709238391197,23.9939598680487));
#38781=CARTESIAN_POINT('Ctrl Pts',(133.288497204862,32.5736254213771,23.9881568411112));
#38782=CARTESIAN_POINT('Ctrl Pts',(133.21476059592,32.4795755692898,23.9823538141738));
#38783=CARTESIAN_POINT('Ctrl Pts',(133.141017476806,32.3855174135841,23.9765502748897));
#38784=CARTESIAN_POINT('Ctrl Pts',(133.063151129624,32.2947087151536,23.9707467356057));
#38785=CARTESIAN_POINT('Ctrl Pts',(132.981488757071,32.2075190615763,23.9649431963216));
#38786=CARTESIAN_POINT('Ctrl Pts',(132.899799902363,32.1203011334112,23.9591377750174));
#38787=CARTESIAN_POINT('Ctrl Pts',(132.814312853082,32.0367048820292,23.9533323537133));
#38788=CARTESIAN_POINT('Ctrl Pts',(132.72539168884,31.957063072885,23.9475269324091));
#38789=CARTESIAN_POINT('Ctrl Pts',(132.63637205264,31.8773330678088,23.9417150821382));
#38790=CARTESIAN_POINT('Ctrl Pts',(132.543911014787,31.8015665187781,23.9359032318673));
#38791=CARTESIAN_POINT('Ctrl Pts',(132.448405871834,31.730056011677,23.9300913815964));
#38792=CARTESIAN_POINT('Ctrl Pts',(132.35283800059,31.6584985360909,23.924275714071));
#38793=CARTESIAN_POINT('Ctrl Pts',(132.254222378932,31.5912028991635,23.9184600465456));
#38794=CARTESIAN_POINT('Ctrl Pts',(132.152984016046,31.5284175327888,23.9126443790203));
#38795=CARTESIAN_POINT('Ctrl Pts',(132.051600640138,31.4655422331564,23.9068203811791));
#38796=CARTESIAN_POINT('Ctrl Pts',(131.947587379505,31.4071902979126,23.900996383338));
#38797=CARTESIAN_POINT('Ctrl Pts',(131.841392584402,31.35356360948,23.8951723854969));
#38798=CARTESIAN_POINT('Ctrl Pts',(131.813218526412,31.3393361567288,23.893627247124));
#38799=CARTESIAN_POINT('Ctrl Pts',(131.784891016527,31.3254410334131,23.8920821087512));
#38800=CARTESIAN_POINT('Ctrl Pts',(131.756418628184,31.3118814278052,23.8905369703783));
#38801=CARTESIAN_POINT('Ctrl Pts',(131.649106801958,31.260775562601,23.8847133767068));
#38802=CARTESIAN_POINT('Ctrl Pts',(131.539389563276,31.2142747918228,23.8788897830354));
#38803=CARTESIAN_POINT('Ctrl Pts',(131.427699034967,31.1726117958123,23.8730661893639));
#38804=CARTESIAN_POINT('Ctrl Pts',(131.31614942085,31.1310013638599,23.8672499430209));
#38805=CARTESIAN_POINT('Ctrl Pts',(131.202631848072,31.0942167082698,23.8614336966779));
#38806=CARTESIAN_POINT('Ctrl Pts',(131.087601531727,31.0624439168204,23.8556174503348));
#38807=CARTESIAN_POINT('Ctrl Pts',(130.972686361364,31.0307029301105,23.8498070260865));
#38808=CARTESIAN_POINT('Ctrl Pts',(130.856261851212,31.0039639351245,23.8439966018382));
#38809=CARTESIAN_POINT('Ctrl Pts',(130.738801057856,30.9823641283821,23.8381861775898));
#38810=CARTESIAN_POINT('Ctrl Pts',(130.61689413052,30.9599467242784,23.8321558167656));
#38811=CARTESIAN_POINT('Ctrl Pts',(130.493871338943,30.9430654100478,23.8261254559415));
#38812=CARTESIAN_POINT('Ctrl Pts',(130.370276759999,30.9318161151436,23.8200950951173));
#38813=CARTESIAN_POINT('Ctrl Pts',(130.251323906435,30.9209892994301,23.8142912108841));
#38814=CARTESIAN_POINT('Ctrl Pts',(130.131841882371,30.9153791393266,23.8084873266508));
#38815=CARTESIAN_POINT('Ctrl Pts',(130.012323149958,30.9150185875606,23.8026834424176));
#38816=CARTESIAN_POINT('Ctrl Pts',(129.892822071739,30.914658089052,23.7968804154801));
#38817=CARTESIAN_POINT('Ctrl Pts',(129.77328470418,30.9195456580404,23.7910773885427));
#38818=CARTESIAN_POINT('Ctrl Pts',(129.654204398354,30.9296621268152,23.7852743616052));
#38819=CARTESIAN_POINT('Ctrl Pts',(129.535113578983,30.9397794887685,23.7794708223211));
#38820=CARTESIAN_POINT('Ctrl Pts',(129.416480308469,30.9551266338267,23.7736672830371));
#38821=CARTESIAN_POINT('Ctrl Pts',(129.298793059801,30.9756324935443,23.767863743753));
#38822=CARTESIAN_POINT('Ctrl Pts',(129.18106764653,30.9961450030731,23.7620583224488));
#38823=CARTESIAN_POINT('Ctrl Pts',(129.064289267297,31.0218194842469,23.7562529011446));
#38824=CARTESIAN_POINT('Ctrl Pts',(128.948935812708,31.0525338412861,23.7504474798405));
#38825=CARTESIAN_POINT('Ctrl Pts',(128.833454614845,31.0832822116328,23.7446356295696));
#38826=CARTESIAN_POINT('Ctrl Pts',(128.719401886217,31.1190814932634,23.7388237792986));
#38827=CARTESIAN_POINT('Ctrl Pts',(128.607240120712,31.1597597837314,23.7330119290277));
#38828=CARTESIAN_POINT('Ctrl Pts',(128.495004686758,31.200464791919,23.7271962615023));
#38829=CARTESIAN_POINT('Ctrl Pts',(128.384663065917,31.2460550353343,23.7213805939769));
#38830=CARTESIAN_POINT('Ctrl Pts',(128.276656014013,31.2963112298734,23.7155649264516));
#38831=CARTESIAN_POINT('Ctrl Pts',(128.168494253669,31.3466394109844,23.7097409286104));
#38832=CARTESIAN_POINT('Ctrl Pts',(128.062674097764,31.4016466953972,23.7039169307693));
#38833=CARTESIAN_POINT('Ctrl Pts',(127.95961016421,31.4610687604865,23.6980929329282));
#38834=CARTESIAN_POINT('Ctrl Pts',(127.932266740855,31.4768337582534,23.6965477945554));
#38835=CARTESIAN_POINT('Ctrl Pts',(127.905117151512,31.4929092696491,23.6950026561826));
#38836=CARTESIAN_POINT('Ctrl Pts',(127.878168762405,31.5092898717932,23.6934575178098));
#38837=CARTESIAN_POINT('Ctrl Pts',(127.776600856886,31.5710280129601,23.6876339241383));
#38838=CARTESIAN_POINT('Ctrl Pts',(127.677565959971,31.6373023167307,23.6818103304669));
#38839=CARTESIAN_POINT('Ctrl Pts',(127.581495552781,31.7078789149269,23.6759867367954));
#38840=CARTESIAN_POINT('Ctrl Pts',(127.48554635268,31.7783664702613,23.6701704904523));
#38841=CARTESIAN_POINT('Ctrl Pts',(127.392554529425,31.8531452842667,23.6643542441093));
#38842=CARTESIAN_POINT('Ctrl Pts',(127.302925253798,31.9319366347155,23.6585379977663));
#38843=CARTESIAN_POINT('Ctrl Pts',(127.213385697571,32.0106491145877,23.6527275735179));
#38844=CARTESIAN_POINT('Ctrl Pts',(127.127202297795,32.0933658723822,23.6469171492695));
#38845=CARTESIAN_POINT('Ctrl Pts',(127.044749114069,32.1797664633571,23.6411067250212));
#38846=CARTESIAN_POINT('Ctrl Pts',(126.959174906797,32.2694374954071,23.635076364197));
#38847=CARTESIAN_POINT('Ctrl Pts',(126.877619249221,32.3630764869371,23.6290460033729));
#38848=CARTESIAN_POINT('Ctrl Pts',(126.800460617091,32.4602809727813,23.6230156425487));
#38849=CARTESIAN_POINT('Ctrl Pts',(126.726199759154,32.5538348411556,23.6172117583155));
#38850=CARTESIAN_POINT('Ctrl Pts',(126.65601188945,32.650690873066,23.6114078740822));
#38851=CARTESIAN_POINT('Ctrl Pts',(126.590194518505,32.7504552508632,23.6056039898489));
#38852=CARTESIAN_POINT('Ctrl Pts',(126.52438686949,32.850204892395,23.5998009629115));
#38853=CARTESIAN_POINT('Ctrl Pts',(126.462948660204,32.9528616847348,23.593997935974));
#38854=CARTESIAN_POINT('Ctrl Pts',(126.406134296418,33.0580024962384,23.5881949090365));
#38855=CARTESIAN_POINT('Ctrl Pts',(126.349314916517,33.1631525905762,23.5823913697524));
#38856=CARTESIAN_POINT('Ctrl Pts',(126.297120387921,33.270786780864,23.5765878304683));
#38857=CARTESIAN_POINT('Ctrl Pts',(126.249759034133,33.3804575652569,23.5707842911842));
#38858=CARTESIAN_POINT('Ctrl Pts',(126.20238232161,33.4901639146062,23.56497886988));
#38859=CARTESIAN_POINT('Ctrl Pts',(126.159842062791,33.6019077968527,23.5591734485759));
#38860=CARTESIAN_POINT('Ctrl Pts',(126.122298102512,33.7152225896231,23.5533680272717));
#38861=CARTESIAN_POINT('Ctrl Pts',(126.084712565772,33.8286628680381,23.5475561770007));
#38862=CARTESIAN_POINT('Ctrl Pts',(126.052134500293,33.9436771415982,23.5417443267298));
#38863=CARTESIAN_POINT('Ctrl Pts',(126.024673654135,34.0597843630996,23.5359324764588));
#38864=CARTESIAN_POINT('Ctrl Pts',(125.997194771546,34.1759678444474,23.5301168089334));
#38865=CARTESIAN_POINT('Ctrl Pts',(125.97483987811,34.2932453031681,23.5243011414081));
#38866=CARTESIAN_POINT('Ctrl Pts',(125.957667177219,34.4111279002503,23.5184854738827));
#38867=CARTESIAN_POINT('Ctrl Pts',(125.940469878288,34.5291793514236,23.5126614760415));
#38868=CARTESIAN_POINT('Ctrl Pts',(125.92846962861,34.6478372662121,23.5068374782004));
#38869=CARTESIAN_POINT('Ctrl Pts',(125.921672634806,34.7666099781222,23.5010134803592));
#38870=CARTESIAN_POINT('Ctrl Pts',(125.919869355301,34.7981210259965,23.4994683419866));
#38871=CARTESIAN_POINT('Ctrl Pts',(125.91843203318,34.829640168958,23.497923203614));
#38872=CARTESIAN_POINT('Ctrl Pts',(125.917360170799,34.8611582734836,23.4963780652414));
#38873=CARTESIAN_POINT('Ctrl Pts',(125.915796331449,34.9071429567317,23.4941237196927));
#38874=CARTESIAN_POINT('Ctrl Pts',(125.91500938505,34.9531542090983,23.4918693741441));
#38875=CARTESIAN_POINT('Ctrl Pts',(125.915000083442,34.9991743380008,23.4896150285955));
#38876=CARTESIAN_POINT('Origin',(130.,35.,32.7603849714045));
#38877=CARTESIAN_POINT('',(132.487160689988,38.2405642567579,25.5469383384863));
#38878=CARTESIAN_POINT('',(132.487160689988,38.2405642567579,25.4425452635723));
#38879=CARTESIAN_POINT('',(132.487160689988,38.2405642567579,32.7603849714045));
#38880=CARTESIAN_POINT('',(125.915001572211,34.9964160126988,24.6353849714487));
#38881=CARTESIAN_POINT('Ctrl Pts',(132.487160689988,38.2405642567579,25.4425452635723));
#38882=CARTESIAN_POINT('Ctrl Pts',(132.581714449096,38.1679934406562,25.4367339314664));
#38883=CARTESIAN_POINT('Ctrl Pts',(132.673191731151,38.0912022458023,25.4309225993606));
#38884=CARTESIAN_POINT('Ctrl Pts',(132.761197162703,38.0104842183082,25.4251112672547));
#38885=CARTESIAN_POINT('Ctrl Pts',(132.849133422777,37.9298296344581,25.4193045028035));
#38886=CARTESIAN_POINT('Ctrl Pts',(132.933602962308,37.8452546342454,25.4134977383524));
#38887=CARTESIAN_POINT('Ctrl Pts',(133.014243166955,37.7570932393496,25.4076909739013));
#38888=CARTESIAN_POINT('Ctrl Pts',(133.094848377427,37.6689701024821,25.4018867293214));
#38889=CARTESIAN_POINT('Ctrl Pts',(133.171627281874,37.5772639660214,25.3960824847415));
#38890=CARTESIAN_POINT('Ctrl Pts',(133.244254201368,37.4823455998115,25.3902782401616));
#38891=CARTESIAN_POINT('Ctrl Pts',(133.316866735388,37.3874460344237,25.3844751452492));
#38892=CARTESIAN_POINT('Ctrl Pts',(133.385328671829,37.2893358286794,25.3786720503369));
#38893=CARTESIAN_POINT('Ctrl Pts',(133.449355121551,37.1884182062456,25.3728689554245));
#38894=CARTESIAN_POINT('Ctrl Pts',(133.513383999606,37.0874967563074,25.3670656404181));
#38895=CARTESIAN_POINT('Ctrl Pts',(133.572976837807,36.9837680228594,25.3612623254117));
#38896=CARTESIAN_POINT('Ctrl Pts',(133.627892878756,36.877662978351,25.3554590104053));
#38897=CARTESIAN_POINT('Ctrl Pts',(133.682823962638,36.7715288689096,25.3496541057199));
#38898=CARTESIAN_POINT('Ctrl Pts',(133.733075513914,36.6630175164213,25.3438492010345));
#38899=CARTESIAN_POINT('Ctrl Pts',(133.778453692629,36.5525825880322,25.338044296349));
#38900=CARTESIAN_POINT('Ctrl Pts',(133.823881049005,36.4420279780761,25.3322331007184));
#38901=CARTESIAN_POINT('Ctrl Pts',(133.864424332967,36.3295460082749,25.3264219050877));
#38902=CARTESIAN_POINT('Ctrl Pts',(133.899938580265,36.2156085184639,25.320610709457));
#38903=CARTESIAN_POINT('Ctrl Pts',(133.935474549376,36.101601340314,25.3147959594864));
#38904=CARTESIAN_POINT('Ctrl Pts',(133.965975251114,35.9861372631882,25.3089812095157));
#38905=CARTESIAN_POINT('Ctrl Pts',(133.991346554824,35.8696997638825,25.3031664595451));
#38906=CARTESIAN_POINT('Ctrl Pts',(134.016755660803,35.7530887771672,25.29734304582));
#38907=CARTESIAN_POINT('Ctrl Pts',(134.037020039342,35.6355018738937,25.2915196320948));
#38908=CARTESIAN_POINT('Ctrl Pts',(134.052097211822,35.5174294018909,25.2856962183697));
#38909=CARTESIAN_POINT('Ctrl Pts',(134.059311380028,35.4609337509584,25.2829098148713));
#38910=CARTESIAN_POINT('Ctrl Pts',(134.065338727778,35.4043269619072,25.280123411373));
#38911=CARTESIAN_POINT('Ctrl Pts',(134.07017882144,35.347662712266,25.2773370078746));
#38912=CARTESIAN_POINT('Ctrl Pts',(134.080294635191,35.2292342198261,25.2715134142025));
#38913=CARTESIAN_POINT('Ctrl Pts',(134.085253665983,35.1101728820045,25.2656898205305));
#38914=CARTESIAN_POINT('Ctrl Pts',(134.084990008492,34.9909650389812,25.2598662268584));
#38915=CARTESIAN_POINT('Ctrl Pts',(134.084726683644,34.8719075943584,25.2540499805148));
#38916=CARTESIAN_POINT('Ctrl Pts',(134.079253777168,34.7527044169091,25.2482337341712));
#38917=CARTESIAN_POINT('Ctrl Pts',(134.068557120453,34.6338470843927,25.2424174878276));
#38918=CARTESIAN_POINT('Ctrl Pts',(134.057871171151,34.5151087287217,25.2366070635786));
#38919=CARTESIAN_POINT('Ctrl Pts',(134.041971910454,34.396715933632,25.2307966393297));
#38920=CARTESIAN_POINT('Ctrl Pts',(134.020897212403,34.2791597907377,25.2249862150807));
#38921=CARTESIAN_POINT('Ctrl Pts',(133.999024793444,34.1571539047043,25.2189558542568));
#38922=CARTESIAN_POINT('Ctrl Pts',(133.971577394719,34.0360497085776,25.2129254934328));
#38923=CARTESIAN_POINT('Ctrl Pts',(133.938656491479,33.9163902722225,25.2068951326089));
#38924=CARTESIAN_POINT('Ctrl Pts',(133.90697196764,33.8012247727823,25.201091248375));
#38925=CARTESIAN_POINT('Ctrl Pts',(133.87021776973,33.687397900253,25.1952873641412));
#38926=CARTESIAN_POINT('Ctrl Pts',(133.828536183256,33.5753822640807,25.1894834799073));
#38927=CARTESIAN_POINT('Ctrl Pts',(133.786860753599,33.4633831738158,25.1836804529692));
#38928=CARTESIAN_POINT('Ctrl Pts',(133.740259525162,33.3531951704548,25.1778774260311));
#38929=CARTESIAN_POINT('Ctrl Pts',(133.688923889136,33.2452733716717,25.172074399093));
#38930=CARTESIAN_POINT('Ctrl Pts',(133.637583720709,33.1373420445223,25.1662708598083));
#38931=CARTESIAN_POINT('Ctrl Pts',(133.581508489022,33.0316776885258,25.1604673205236));
#38932=CARTESIAN_POINT('Ctrl Pts',(133.520936457764,32.9287126079691,25.1546637812389));
#38933=CARTESIAN_POINT('Ctrl Pts',(133.460344783703,32.8257141370377,25.1488583599341));
#38934=CARTESIAN_POINT('Ctrl Pts',(133.395253616862,32.7254170341788,25.1430529386293));
#38935=CARTESIAN_POINT('Ctrl Pts',(133.325945270333,32.6282257572131,25.1372475173245));
#38936=CARTESIAN_POINT('Ctrl Pts',(133.256560171226,32.5309268499041,25.1314356670529));
#38937=CARTESIAN_POINT('Ctrl Pts',(133.182948807664,32.4367409665134,25.1256238167814));
#38938=CARTESIAN_POINT('Ctrl Pts',(133.105434706827,32.3460406405456,25.1198119665098));
#38939=CARTESIAN_POINT('Ctrl Pts',(133.027869694312,32.2552807421168,25.1139962989838));
#38940=CARTESIAN_POINT('Ctrl Pts',(132.946397117583,32.1680112581697,25.1081806314578));
#38941=CARTESIAN_POINT('Ctrl Pts',(132.861377218282,32.0845677139234,25.1023649639318));
#38942=CARTESIAN_POINT('Ctrl Pts',(132.776235537156,32.0010046458104,25.09654096609));
#38943=CARTESIAN_POINT('Ctrl Pts',(132.687536694358,31.9212787276694,25.0907169682483));
#38944=CARTESIAN_POINT('Ctrl Pts',(132.595673905589,31.8456851812407,25.0848929704065));
#38945=CARTESIAN_POINT('Ctrl Pts',(132.571302207099,31.8256298014067,25.0833478320397));
#38946=CARTESIAN_POINT('Ctrl Pts',(132.546707963692,31.8058650486462,25.0818026936729));
#38947=CARTESIAN_POINT('Ctrl Pts',(132.521898841803,31.7863959124194,25.0802575553061));
#38948=CARTESIAN_POINT('Ctrl Pts',(132.428393788576,31.713017151686,25.0744339616348));
#38949=CARTESIAN_POINT('Ctrl Pts',(132.331532681142,31.6436044726346,25.0686103679634));
#38950=CARTESIAN_POINT('Ctrl Pts',(132.231686153495,31.5784795905477,25.0627867742921));
#38951=CARTESIAN_POINT('Ctrl Pts',(132.131965597074,31.5134368731729,25.0569705279491));
#38952=CARTESIAN_POINT('Ctrl Pts',(132.029267451023,31.4526714141239,25.0511542816062));
#38953=CARTESIAN_POINT('Ctrl Pts',(131.92399509008,31.3964645286401,25.0453380352633));
#38954=CARTESIAN_POINT('Ctrl Pts',(131.818828107351,31.3403139065589,25.0395276110151));
#38955=CARTESIAN_POINT('Ctrl Pts',(131.711092394101,31.2887129714239,25.0337171867669));
#38956=CARTESIAN_POINT('Ctrl Pts',(131.601219446355,31.2418992450154,25.0279067625186));
#38957=CARTESIAN_POINT('Ctrl Pts',(131.487187580277,31.1933135222336,25.0218764016944));
#38958=CARTESIAN_POINT('Ctrl Pts',(131.37085386077,31.1498848252301,25.0158460408702));
#38959=CARTESIAN_POINT('Ctrl Pts',(131.252728120834,31.111825974153,25.009815680046));
#38960=CARTESIAN_POINT('Ctrl Pts',(131.139038718239,31.0751964635588,25.0040117958129));
#38961=CARTESIAN_POINT('Ctrl Pts',(131.023689893895,31.0435408685883,24.9982079115798));
#38962=CARTESIAN_POINT('Ctrl Pts',(130.907154920439,31.0169992530349,24.9924040273466));
#38963=CARTESIAN_POINT('Ctrl Pts',(130.790637160444,30.9904615579621,24.9866010004093));
#38964=CARTESIAN_POINT('Ctrl Pts',(130.6729339978,30.9690364307302,24.9807979734719));
#38965=CARTESIAN_POINT('Ctrl Pts',(130.554530993477,30.9528132762037,24.9749949465345));
#38966=CARTESIAN_POINT('Ctrl Pts',(130.436117535407,30.9365886893422,24.9691914072506));
#38967=CARTESIAN_POINT('Ctrl Pts',(130.317004517383,30.925567043779,24.9633878679666));
#38968=CARTESIAN_POINT('Ctrl Pts',(130.197684113714,30.9197860361024,24.9575843286827));
#38969=CARTESIAN_POINT('Ctrl Pts',(130.07832501583,30.9140031537125,24.9517789073786));
#38970=CARTESIAN_POINT('Ctrl Pts',(129.958758806199,30.9134643088372,24.9459734860746));
#38971=CARTESIAN_POINT('Ctrl Pts',(129.839478515427,30.918155091997,24.9401680647705));
#38972=CARTESIAN_POINT('Ctrl Pts',(129.720066132773,30.9228510697649,24.9343562144997));
#38973=CARTESIAN_POINT('Ctrl Pts',(129.600940709258,30.9327882195011,24.9285443642289));
#38974=CARTESIAN_POINT('Ctrl Pts',(129.482591166975,30.9479001617053,24.9227325139581));
#38975=CARTESIAN_POINT('Ctrl Pts',(129.364163892077,30.9630220295143,24.9169168464328));
#38976=CARTESIAN_POINT('Ctrl Pts',(129.24651391476,30.9833253893675,24.9111011789075));
#38977=CARTESIAN_POINT('Ctrl Pts',(129.130119329984,31.0086928682532,24.9052855113822));
#38978=CARTESIAN_POINT('Ctrl Pts',(129.013558022534,31.0340966833132,24.8994615135412));
#38979=CARTESIAN_POINT('Ctrl Pts',(128.898256090136,31.0645789916075,24.8936375157002));
#38980=CARTESIAN_POINT('Ctrl Pts',(128.78467599426,31.0999727486757,24.8878135178592));
#38981=CARTESIAN_POINT('Ctrl Pts',(128.754542575699,31.1093629053571,24.8862683794854));
#38982=CARTESIAN_POINT('Ctrl Pts',(128.724530238221,31.119098503364,24.8847232411115));
#38983=CARTESIAN_POINT('Ctrl Pts',(128.694647357325,31.129175865754,24.8831781027377));
#38984=CARTESIAN_POINT('Ctrl Pts',(128.582019414728,31.1671572302927,24.8773545090663));
#38985=CARTESIAN_POINT('Ctrl Pts',(128.470868921732,31.2101195632545,24.8715309153949));
#38986=CARTESIAN_POINT('Ctrl Pts',(128.361668119774,31.2579292296597,24.8657073217235));
#38987=CARTESIAN_POINT('Ctrl Pts',(128.252605090848,31.3056785770691,24.8598910753806));
#38988=CARTESIAN_POINT('Ctrl Pts',(128.145487231186,31.3582629317509,24.8540748290376));
#38989=CARTESIAN_POINT('Ctrl Pts',(128.040770940076,31.4154991294813,24.8482585826947));
#38990=CARTESIAN_POINT('Ctrl Pts',(127.936159470551,31.4726780334621,24.8424481584464));
#38991=CARTESIAN_POINT('Ctrl Pts',(127.833945143399,31.5344993222014,24.8366377341982));
#38992=CARTESIAN_POINT('Ctrl Pts',(127.734563145388,31.6007323056627,24.8308273099499));
#38993=CARTESIAN_POINT('Ctrl Pts',(127.631419333193,31.6694723445425,24.8247969491257));
#38994=CARTESIAN_POINT('Ctrl Pts',(127.531326916347,31.7429644809081,24.8187665883015));
#38995=CARTESIAN_POINT('Ctrl Pts',(127.434743363362,31.8208989654019,24.8127362274773));
#38996=CARTESIAN_POINT('Ctrl Pts',(127.341787108057,31.8959065377445,24.8069323432442));
#38997=CARTESIAN_POINT('Ctrl Pts',(127.252081257699,31.9750285219347,24.801128459011));
#38998=CARTESIAN_POINT('Ctrl Pts',(127.166002388425,32.0579458642664,24.7953245747778));
#38999=CARTESIAN_POINT('Ctrl Pts',(127.07993623392,32.14085095882,24.7895215478404));
#39000=CARTESIAN_POINT('Ctrl Pts',(126.997496289081,32.2275500134187,24.783718520903));
#39001=CARTESIAN_POINT('Ctrl Pts',(126.919023496395,32.3176859273693,24.7779154939656));
#39002=CARTESIAN_POINT('Ctrl Pts',(126.840543775381,32.4078297993785,24.7721119546817));
#39003=CARTESIAN_POINT('Ctrl Pts',(126.766032171056,32.5014108260591,24.7663084153977));
#39004=CARTESIAN_POINT('Ctrl Pts',(126.695790003786,32.5980380309179,24.7605048761137));
#39005=CARTESIAN_POINT('Ctrl Pts',(126.6255250578,32.6946965708524,24.7546994548096));
#39006=CARTESIAN_POINT('Ctrl Pts',(126.559532542362,32.7944029234367,24.7488940335055));
#39007=CARTESIAN_POINT('Ctrl Pts',(126.498070667218,32.8967368333466,24.7430886122014));
#39008=CARTESIAN_POINT('Ctrl Pts',(126.436540728737,32.9991840685898,24.7372767619306));
#39009=CARTESIAN_POINT('Ctrl Pts',(126.379551655807,33.1042643190611,24.7314649116597));
#39010=CARTESIAN_POINT('Ctrl Pts',(126.327315939812,33.2115322776071,24.7256530613889));
#39011=CARTESIAN_POINT('Ctrl Pts',(126.275045915119,33.318870690324,24.7198373938636));
#39012=CARTESIAN_POINT('Ctrl Pts',(126.227535627084,33.4283992989842,24.7140217263383));
#39013=CARTESIAN_POINT('Ctrl Pts',(126.184948982552,33.5396538991489,24.708206058813));
#39014=CARTESIAN_POINT('Ctrl Pts',(126.14230133725,33.651067859515,24.7023820609719));
#39015=CARTESIAN_POINT('Ctrl Pts',(126.104591540685,33.7642123599422,24.6965580631309));
#39016=CARTESIAN_POINT('Ctrl Pts',(126.071933386224,33.8786090433122,24.6907340652898));
#39017=CARTESIAN_POINT('Ctrl Pts',(126.063268999828,33.90895910698,24.6891889269163));
#39018=CARTESIAN_POINT('Ctrl Pts',(126.054959902828,33.9393972602767,24.6876437885428));
#39019=CARTESIAN_POINT('Ctrl Pts',(126.047007611079,33.9699144826103,24.6860986501693));
#39020=CARTESIAN_POINT('Ctrl Pts',(126.008453455647,34.1178675218615,24.6786075385627));
#39021=CARTESIAN_POINT('Ctrl Pts',(125.978189862157,34.2680627700817,24.6711164269561));
#39022=CARTESIAN_POINT('Ctrl Pts',(125.956429349326,34.4196885379352,24.6636253153494));
#39023=CARTESIAN_POINT('Ctrl Pts',(125.935075376485,34.5684815628806,24.6562741561637));
#39024=CARTESIAN_POINT('Ctrl Pts',(125.921909712315,34.7186523616112,24.6489229969779));
#39025=CARTESIAN_POINT('Ctrl Pts',(125.917087813762,34.8694125600498,24.6415718377922));
#39026=CARTESIAN_POINT('Ctrl Pts',(125.915735081896,34.9117067150295,24.639509549011));
#39027=CARTESIAN_POINT('Ctrl Pts',(125.915038744708,34.9540471158435,24.6374472602299));
#39028=CARTESIAN_POINT('Ctrl Pts',(125.915001572211,34.9964160126988,24.6353849714487));
#39029=CARTESIAN_POINT('Ctrl Pts',(125.915001572211,34.9964160136077,24.6353849714045));
#39030=CARTESIAN_POINT('Ctrl Pts',(125.914897993777,35.1144738661888,24.629638553561));
#39031=CARTESIAN_POINT('Ctrl Pts',(125.919916516331,35.2326545958854,24.6238921357174));
#39032=CARTESIAN_POINT('Ctrl Pts',(125.930062305213,35.3504741938474,24.6181457178739));
#39033=CARTESIAN_POINT('Ctrl Pts',(125.940202397681,35.4682276412864,24.6124025263913));
#39034=CARTESIAN_POINT('Ctrl Pts',(125.955463997557,35.5856199446566,24.6066593349086));
#39035=CARTESIAN_POINT('Ctrl Pts',(125.975800204933,35.7021687898124,24.600916143426));
#39036=CARTESIAN_POINT('Ctrl Pts',(125.996130870098,35.8186858719973,24.5951745171311));
#39037=CARTESIAN_POINT('Ctrl Pts',(126.021533322221,35.9343595413328,24.5894328908362));
#39038=CARTESIAN_POINT('Ctrl Pts',(126.051909088729,36.0487150024369,24.5836912645414));
#39039=CARTESIAN_POINT('Ctrl Pts',(126.082284131011,36.1630677370576,24.5779497751393));
#39040=CARTESIAN_POINT('Ctrl Pts',(126.11763214416,36.2761019219958,24.5722082857373));
#39041=CARTESIAN_POINT('Ctrl Pts',(126.157804255104,36.3873560674535,24.5664667963353));
#39042=CARTESIAN_POINT('Ctrl Pts',(126.197985399101,36.4986352293892,24.5607240159087));
#39043=CARTESIAN_POINT('Ctrl Pts',(126.242992654503,36.6081331633545,24.554981235482));
#39044=CARTESIAN_POINT('Ctrl Pts',(126.292628585109,36.7154072962566,24.5492384550554));
#39045=CARTESIAN_POINT('Ctrl Pts',(126.34231651387,36.8227938085766,24.5434896585436));
#39046=CARTESIAN_POINT('Ctrl Pts',(126.396642621412,36.9279514897126,24.5377408620317));
#39047=CARTESIAN_POINT('Ctrl Pts',(126.455362953409,37.0304613288446,24.5319920655199));
#39048=CARTESIAN_POINT('Ctrl Pts',(126.514117959328,37.133031699279,24.5262398743862));
#39049=CARTESIAN_POINT('Ctrl Pts',(126.577272131778,37.2329507626782,24.5204876832526));
#39050=CARTESIAN_POINT('Ctrl Pts',(126.644538532043,37.3298290360142,24.5147354921189));
#39051=CARTESIAN_POINT('Ctrl Pts',(126.711905430002,37.4268520479276,24.5089747070669));
#39052=CARTESIAN_POINT('Ctrl Pts',(126.783396567164,37.5208248695185,24.503213922015));
#39053=CARTESIAN_POINT('Ctrl Pts',(126.858685058135,37.6113914750605,24.4974531369631));
#39054=CARTESIAN_POINT('Ctrl Pts',(126.895426495388,37.6555887648685,24.4946418238423));
#39055=CARTESIAN_POINT('Ctrl Pts',(126.933071724442,37.6989754169815,24.4918305107216));
#39056=CARTESIAN_POINT('Ctrl Pts',(126.971579748943,37.7415134110539,24.4890191976008));
#39057=CARTESIAN_POINT('Ctrl Pts',(127.051348553824,37.829630238471,24.4831956039294));
#39058=CARTESIAN_POINT('Ctrl Pts',(127.135095038228,37.9144047658769,24.4773720102579));
#39059=CARTESIAN_POINT('Ctrl Pts',(127.22250822728,37.9954573027292,24.4715484165865));
#39060=CARTESIAN_POINT('Ctrl Pts',(127.30981113161,38.076407579767,24.4657321702435));
#39061=CARTESIAN_POINT('Ctrl Pts',(127.400771242611,38.1536449309834,24.4599159239005));
#39062=CARTESIAN_POINT('Ctrl Pts',(127.495038491786,38.2268239558998,24.4540996775574));
#39063=CARTESIAN_POINT('Ctrl Pts',(127.589211378925,38.2999297282083,24.4482892533091));
#39064=CARTESIAN_POINT('Ctrl Pts',(127.686684497781,38.3689850069155,24.4424788290608));
#39065=CARTESIAN_POINT('Ctrl Pts',(127.787072666214,38.4336828064603,24.4366684048125));
#39066=CARTESIAN_POINT('Ctrl Pts',(127.89126073446,38.5008295515361,24.4306380439883));
#39067=CARTESIAN_POINT('Ctrl Pts',(127.998588565236,38.5632821156029,24.4246076831641));
#39068=CARTESIAN_POINT('Ctrl Pts',(128.108589592872,38.6207446294659,24.4185773223399));
#39069=CARTESIAN_POINT('Ctrl Pts',(128.21445941535,38.6760490777296,24.4127734381067));
#39070=CARTESIAN_POINT('Ctrl Pts',(128.322804871712,38.7267313236994,24.4069695538735));
#39071=CARTESIAN_POINT('Ctrl Pts',(128.433183143552,38.7725733840906,24.4011656696403));
#39072=CARTESIAN_POINT('Ctrl Pts',(128.54354511134,38.8184086731193,24.3953626427028));
#39073=CARTESIAN_POINT('Ctrl Pts',(128.655938920462,38.8594050417968,24.3895596157653));
#39074=CARTESIAN_POINT('Ctrl Pts',(128.769901084859,38.895392362647,24.3837565888279));
#39075=CARTESIAN_POINT('Ctrl Pts',(128.883873310923,38.9313828608012,24.3779530495438));
#39076=CARTESIAN_POINT('Ctrl Pts',(128.99941377817,38.9623633088683,24.3721495102598));
#39077=CARTESIAN_POINT('Ctrl Pts',(129.116043749136,38.9882134279095,24.3663459709757));
#39078=CARTESIAN_POINT('Ctrl Pts',(129.232711541841,39.014071929843,24.3605405496715));
#39079=CARTESIAN_POINT('Ctrl Pts',(129.350469142469,39.0347967057002,24.3547351283673));
#39080=CARTESIAN_POINT('Ctrl Pts',(129.468828169307,39.050318689471,24.3489297070631));
#39081=CARTESIAN_POINT('Ctrl Pts',(129.58731826781,39.0658578624019,24.3431178567922));
#39082=CARTESIAN_POINT('Ctrl Pts',(129.706410716854,39.0761826894508,24.3373060065213));
#39083=CARTESIAN_POINT('Ctrl Pts',(129.825612406944,39.0812760219554,24.3314941562504));
#39084=CARTESIAN_POINT('Ctrl Pts',(129.944892389344,39.0863726997882,24.325678488725));
#39085=CARTESIAN_POINT('Ctrl Pts',(130.064281348285,39.0862310405327,24.3198628211997));
#39086=CARTESIAN_POINT('Ctrl Pts',(130.183288233519,39.0808859851083,24.3140471536743));
#39087=CARTESIAN_POINT('Ctrl Pts',(130.302465583266,39.0755332734691,24.3082231558332));
#39088=CARTESIAN_POINT('Ctrl Pts',(130.42125936168,39.0649623253379,24.302399157992));
#39089=CARTESIAN_POINT('Ctrl Pts',(130.539185538355,39.0492596798957,24.2965751601509));
#39090=CARTESIAN_POINT('Ctrl Pts',(130.570471995822,39.0450936824675,24.2950300217781));
#39091=CARTESIAN_POINT('Ctrl Pts',(130.601697453545,39.0405667565578,24.2934848834052));
#39092=CARTESIAN_POINT('Ctrl Pts',(130.632853035338,39.035681111741,24.2919397450324));
#39093=CARTESIAN_POINT('Ctrl Pts',(130.750277186331,39.0172673103726,24.2861161798426));
#39094=CARTESIAN_POINT('Ctrl Pts',(130.867086359088,38.9936946159999,24.2802926146529));
#39095=CARTESIAN_POINT('Ctrl Pts',(130.982792533448,38.9650149856211,24.2744690494631));
#39096=CARTESIAN_POINT('Ctrl Pts',(131.09835807508,38.9363702133184,24.2686525624077));
#39097=CARTESIAN_POINT('Ctrl Pts',(131.212822891387,38.9026309457919,24.2628360753524));
#39098=CARTESIAN_POINT('Ctrl Pts',(131.325706145027,38.8639006479251,24.257019588297));
#39099=CARTESIAN_POINT('Ctrl Pts',(131.438460699236,38.8252145068943,24.2512097326821));
#39100=CARTESIAN_POINT('Ctrl Pts',(131.549636896164,38.7815487945288,24.2453998770673));
#39101=CARTESIAN_POINT('Ctrl Pts',(131.658766976276,38.7330573419674,24.2395900214524));
#39102=CARTESIAN_POINT('Ctrl Pts',(131.767824304215,38.6845982165012,24.2337840390099));
#39103=CARTESIAN_POINT('Ctrl Pts',(131.874837856289,38.6313199139055,24.2279780565674));
#39104=CARTESIAN_POINT('Ctrl Pts',(131.979358124367,38.5734250258685,24.2221720741249));
#39105=CARTESIAN_POINT('Ctrl Pts',(132.083838706936,38.5155521200567,24.2163682961674));
#39106=CARTESIAN_POINT('Ctrl Pts',(132.185827530776,38.4530663107781,24.21056451821));
#39107=CARTESIAN_POINT('Ctrl Pts',(132.284898567803,38.3862166993345,24.2047607402525));
#39108=CARTESIAN_POINT('Ctrl Pts',(132.353774100659,38.339741939934,24.200725874853));
#39109=CARTESIAN_POINT('Ctrl Pts',(132.421239880535,38.2911590399292,24.1966910094534));
#39110=CARTESIAN_POINT('Ctrl Pts',(132.487160689988,38.2405642567579,24.1926561440539));
#39111=CARTESIAN_POINT('',(125.915001332191,35.0032990905112,24.7396150285626));
#39112=CARTESIAN_POINT('Ctrl Pts',(125.915001332191,35.0032990905112,24.7396150285626));
#39113=CARTESIAN_POINT('Ctrl Pts',(125.915116126591,35.1454397707582,24.73270773086));
#39114=CARTESIAN_POINT('Ctrl Pts',(125.922653598402,35.2872683007052,24.7258004331575));
#39115=CARTESIAN_POINT('Ctrl Pts',(125.937493194041,35.4280928071526,24.7188931354549));
#39116=CARTESIAN_POINT('Ctrl Pts',(125.952505705088,35.5705582428807,24.711905351853));
#39117=CARTESIAN_POINT('Ctrl Pts',(125.974991434027,35.7119960748056,24.7049175682512));
#39118=CARTESIAN_POINT('Ctrl Pts',(126.004776161893,35.8517109154073,24.6979297846493));
#39119=CARTESIAN_POINT('Ctrl Pts',(126.031877926701,35.9788404553204,24.6915714499835));
#39120=CARTESIAN_POINT('Ctrl Pts',(126.065022300519,36.1045436835966,24.6852131153178));
#39121=CARTESIAN_POINT('Ctrl Pts',(126.104043775727,36.2283118897705,24.678854780652));
#39122=CARTESIAN_POINT('Ctrl Pts',(126.139783513885,36.3416710915234,24.6730311869807));
#39123=CARTESIAN_POINT('Ctrl Pts',(126.180532547933,36.4536519397547,24.6672075933093));
#39124=CARTESIAN_POINT('Ctrl Pts',(126.226166636842,36.5637796350878,24.661383999638));
#39125=CARTESIAN_POINT('Ctrl Pts',(126.271743151569,36.6737683879751,24.6555677532951));
#39126=CARTESIAN_POINT('Ctrl Pts',(126.322192307714,36.7819082643388,24.6497515069522));
#39127=CARTESIAN_POINT('Ctrl Pts',(126.377340030494,36.8877393213422,24.6439352606093));
#39128=CARTESIAN_POINT('Ctrl Pts',(126.432432550099,36.9934644408733,24.6381248363611));
#39129=CARTESIAN_POINT('Ctrl Pts',(126.49221409211,37.0968849787328,24.6323144121128));
#39130=CARTESIAN_POINT('Ctrl Pts',(126.556462644497,37.1975612576805,24.6265039878646));
#39131=CARTESIAN_POINT('Ctrl Pts',(126.623143137483,37.3020483420238,24.6204736270404));
#39132=CARTESIAN_POINT('Ctrl Pts',(126.694635322155,37.403578896778,24.6144432662162));
#39133=CARTESIAN_POINT('Ctrl Pts',(126.770638584712,37.5016893990765,24.608412905392));
#39134=CARTESIAN_POINT('Ctrl Pts',(126.843787464204,37.5961152574942,24.6026090211589));
#39135=CARTESIAN_POINT('Ctrl Pts',(126.921114422886,37.6873729663813,24.5968051369258));
#39136=CARTESIAN_POINT('Ctrl Pts',(127.002307939814,37.7750796947647,24.5910012526926));
#39137=CARTESIAN_POINT('Ctrl Pts',(127.08348946359,37.8627734679264,24.5851982257553));
#39138=CARTESIAN_POINT('Ctrl Pts',(127.168536132488,37.946917004116,24.5793951988179));
#39139=CARTESIAN_POINT('Ctrl Pts',(127.257097679211,38.0271623442769,24.5735921718806));
#39140=CARTESIAN_POINT('Ctrl Pts',(127.345667044992,38.1074147692622,24.5677886325966));
#39141=CARTESIAN_POINT('Ctrl Pts',(127.437751602993,38.1837680397314,24.5619850933127));
#39142=CARTESIAN_POINT('Ctrl Pts',(127.532966430815,38.2559131389697,24.5561815540288));
#39143=CARTESIAN_POINT('Ctrl Pts',(127.628212135696,38.3280816340225,24.5503761327247));
#39144=CARTESIAN_POINT('Ctrl Pts',(127.726589803929,38.3960389973639,24.5445707114206));
#39145=CARTESIAN_POINT('Ctrl Pts',(127.82768438488,38.4595187336255,24.5387652901166));
#39146=CARTESIAN_POINT('Ctrl Pts',(127.928890918722,38.5230687678194,24.5329534398458));
#39147=CARTESIAN_POINT('Ctrl Pts',(128.032820024943,38.5821310599545,24.527141589575));
#39148=CARTESIAN_POINT('Ctrl Pts',(128.139030699114,38.6364843270883,24.5213297393042));
#39149=CARTESIAN_POINT('Ctrl Pts',(128.245311133025,38.6908732937396,24.5155140717789));
#39150=CARTESIAN_POINT('Ctrl Pts',(128.353875748817,38.7405469062713,24.5096984042536));
#39151=CARTESIAN_POINT('Ctrl Pts',(128.464263684739,38.7853320818639,24.5038827367284));
#39152=CARTESIAN_POINT('Ctrl Pts',(128.57480973946,38.8301814073847,24.4980587388874));
#39153=CARTESIAN_POINT('Ctrl Pts',(128.687183943756,38.8701281837541,24.4922347410464));
#39154=CARTESIAN_POINT('Ctrl Pts',(128.800910291905,38.9050491510276,24.4864107432054));
#39155=CARTESIAN_POINT('Ctrl Pts',(128.831082511993,38.9143138739999,24.4848656048314));
#39156=CARTESIAN_POINT('Ctrl Pts',(128.861349852103,38.923225124881,24.4833204664575));
#39157=CARTESIAN_POINT('Ctrl Pts',(128.891703323487,38.9317812091761,24.4817753280836));
#39158=CARTESIAN_POINT('Ctrl Pts',(129.006109646572,38.9640302436215,24.4759514933802));
#39159=CARTESIAN_POINT('Ctrl Pts',(129.122109200102,38.9913336746322,24.4701276586767));
#39160=CARTESIAN_POINT('Ctrl Pts',(129.239236713012,39.0135351276863,24.4643038239732));
#39161=CARTESIAN_POINT('Ctrl Pts',(129.356215278892,39.035708347916,24.4584873952401));
#39162=CARTESIAN_POINT('Ctrl Pts',(129.474318553341,39.0527924198107,24.452670966507));
#39163=CARTESIAN_POINT('Ctrl Pts',(129.593066386042,39.0646808034372,24.4468545377739));
#39164=CARTESIAN_POINT('Ctrl Pts',(129.711694163112,39.0765571677505,24.4410439895273));
#39165=CARTESIAN_POINT('Ctrl Pts',(129.830964797949,39.0832482538911,24.4352334412806));
#39166=CARTESIAN_POINT('Ctrl Pts',(129.950388826311,39.0846987320297,24.429422893034));
#39167=CARTESIAN_POINT('Ctrl Pts',(130.06972128596,39.0861480980101,24.4236168000417));
#39168=CARTESIAN_POINT('Ctrl Pts',(130.18920649813,39.0823648482055,24.4178107070494));
#39169=CARTESIAN_POINT('Ctrl Pts',(130.308351393325,39.0733456050567,24.4120046140571));
#39170=CARTESIAN_POINT('Ctrl Pts',(130.427447782066,39.0643300338361,24.4062008848503));
#39171=CARTESIAN_POINT('Ctrl Pts',(130.546203722888,39.0500827393781,24.4003971556436));
#39172=CARTESIAN_POINT('Ctrl Pts',(130.664128126283,39.0306524077226,24.3945934264368));
#39173=CARTESIAN_POINT('Ctrl Pts',(130.782032350306,39.0112254010099,24.3887906903715));
#39174=CARTESIAN_POINT('Ctrl Pts',(130.899104917338,38.9866171881897,24.3829879543062));
#39175=CARTESIAN_POINT('Ctrl Pts',(131.014862463638,38.9569279978158,24.3771852182409));
#39176=CARTESIAN_POINT('Ctrl Pts',(131.130627519588,38.9272368813867,24.3713821057291));
#39177=CARTESIAN_POINT('Ctrl Pts',(131.245076990016,38.89246423446,24.3655789932174));
#39178=CARTESIAN_POINT('Ctrl Pts',(131.357740886639,38.8527606575999,24.3597758807056));
#39179=CARTESIAN_POINT('Ctrl Pts',(131.47049454896,38.8130254466545,24.3539681445259));
#39180=CARTESIAN_POINT('Ctrl Pts',(131.581459410512,38.7683515950809,24.3481604083462));
#39181=CARTESIAN_POINT('Ctrl Pts',(131.69018367222,38.7189385789711,24.3423526721665));
#39182=CARTESIAN_POINT('Ctrl Pts',(131.798954823004,38.6695042527084,24.3365424313078));
#39183=CARTESIAN_POINT('Ctrl Pts',(131.905483084016,38.6153268732889,24.330732190449));
#39184=CARTESIAN_POINT('Ctrl Pts',(132.009340932926,38.556652079592,24.3249219495903));
#39185=CARTESIAN_POINT('Ctrl Pts',(132.113332546574,38.497901715118,24.3191042253747));
#39186=CARTESIAN_POINT('Ctrl Pts',(132.214646531527,38.4346425819258,24.3132865011591));
#39187=CARTESIAN_POINT('Ctrl Pts',(132.312883826795,38.3671640001268,24.3074687769436));
#39188=CARTESIAN_POINT('Ctrl Pts',(132.372121398138,38.3264740840157,24.3039606606794));
#39189=CARTESIAN_POINT('Ctrl Pts',(132.430240844462,38.2842507233904,24.3004525444153));
#39190=CARTESIAN_POINT('Ctrl Pts',(132.487160689988,38.2405642567579,24.2969444281512));
#39191=CARTESIAN_POINT('Ctrl Pts',(132.487160689988,38.2405642567579,25.5469383384863));
#39192=CARTESIAN_POINT('Ctrl Pts',(132.581965737722,38.1678005744939,25.5411336424445));
#39193=CARTESIAN_POINT('Ctrl Pts',(132.673546042516,38.0908953076657,25.5353289464028));
#39194=CARTESIAN_POINT('Ctrl Pts',(132.76153287122,38.0101762741028,25.529524250361));
#39195=CARTESIAN_POINT('Ctrl Pts',(132.849614100948,37.9293706371293,25.5237133264638));
#39196=CARTESIAN_POINT('Ctrl Pts',(132.93409385506,37.8447433396171,25.5179024025666));
#39197=CARTESIAN_POINT('Ctrl Pts',(133.014639843564,37.7566595026581,25.5120914786694));
#39198=CARTESIAN_POINT('Ctrl Pts',(133.095233487448,37.6685235505189,25.5062771167141));
#39199=CARTESIAN_POINT('Ctrl Pts',(133.171888467963,37.5769272981436,25.5004627547588));
#39200=CARTESIAN_POINT('Ctrl Pts',(133.244313509706,37.4822680859934,25.4946483928035));
#39201=CARTESIAN_POINT('Ctrl Pts',(133.316848358064,37.3874653570778,25.4888252154524));
#39202=CARTESIAN_POINT('Ctrl Pts',(133.385140226788,37.2895907287106,25.4830020381014));
#39203=CARTESIAN_POINT('Ctrl Pts',(133.448941598171,37.189069860102,25.4771788607503));
#39204=CARTESIAN_POINT('Ctrl Pts',(133.485486007905,37.1314931069743,25.4738434374755));
#39205=CARTESIAN_POINT('Ctrl Pts',(133.520558014452,37.0730486299488,25.4705080142006));
#39206=CARTESIAN_POINT('Ctrl Pts',(133.554118108443,37.0138196223183,25.4671725909258));
#39207=CARTESIAN_POINT('Ctrl Pts',(133.612713475523,36.9104067580779,25.4613489972493));
#39208=CARTESIAN_POINT('Ctrl Pts',(133.666886136783,36.8042676185213,25.4555254035728));
#39209=CARTESIAN_POINT('Ctrl Pts',(133.71637332103,36.6958167173178,25.4497018098963));
#39210=CARTESIAN_POINT('Ctrl Pts',(133.765798069844,36.587502643034,25.4438855635482));
#39211=CARTESIAN_POINT('Ctrl Pts',(133.810548931311,36.4768829764279,25.4380693172001));
#39212=CARTESIAN_POINT('Ctrl Pts',(133.850407969834,36.3643985729397,25.4322530708519));
#39213=CARTESIAN_POINT('Ctrl Pts',(133.890227109239,36.2520267669589,25.4264426465985));
#39214=CARTESIAN_POINT('Ctrl Pts',(133.92516403156,36.1377943201641,25.420632222345));
#39215=CARTESIAN_POINT('Ctrl Pts',(133.955048302462,36.022163355434,25.4148217980915));
#39216=CARTESIAN_POINT('Ctrl Pts',(133.986063754791,35.9021555196673,25.4087914372692));
#39217=CARTESIAN_POINT('Ctrl Pts',(134.011636305304,35.780641608255,25.402761076447));
#39218=CARTESIAN_POINT('Ctrl Pts',(134.031631640618,35.6581575148611,25.3967307156247));
#39219=CARTESIAN_POINT('Ctrl Pts',(134.05087602995,35.5402734412426,25.3909268313862));
#39220=CARTESIAN_POINT('Ctrl Pts',(134.064954494204,35.4214911831432,25.3851229471477));
#39221=CARTESIAN_POINT('Ctrl Pts',(134.073799202137,35.3022996206876,25.3793190629092));
#39222=CARTESIAN_POINT('Ctrl Pts',(134.082642603612,35.1831256640998,25.3735160359664));
#39223=CARTESIAN_POINT('Ctrl Pts',(134.086253755971,35.0635429304962,25.3677130090237));
#39224=CARTESIAN_POINT('Ctrl Pts',(134.084616753787,34.9440448868994,25.3619099820809));
#39225=CARTESIAN_POINT('Ctrl Pts',(134.082979607073,34.8245362928745,25.3561064427915));
#39226=CARTESIAN_POINT('Ctrl Pts',(134.076093390145,34.7051128120416,25.3503029035021));
#39227=CARTESIAN_POINT('Ctrl Pts',(134.063994313667,34.5862667302641,25.3444993642127));
#39228=CARTESIAN_POINT('Ctrl Pts',(134.051891313599,34.4673821080882,25.3386939429032));
#39229=CARTESIAN_POINT('Ctrl Pts',(134.034572133354,34.3490756633815,25.3328885215937));
#39230=CARTESIAN_POINT('Ctrl Pts',(134.012124633458,34.2318327489431,25.3270831002842));
#39231=CARTESIAN_POINT('Ctrl Pts',(133.989652275035,34.1144599988288,25.321271250008));
#39232=CARTESIAN_POINT('Ctrl Pts',(133.962040337743,33.9981535311854,25.3154593997317));
#39233=CARTESIAN_POINT('Ctrl Pts',(133.929427456172,33.8833868768994,25.3096475494554));
#39234=CARTESIAN_POINT('Ctrl Pts',(133.896793154285,33.7685448432586,25.3038318819247));
#39235=CARTESIAN_POINT('Ctrl Pts',(133.859151495108,33.6552450237393,25.298016214394));
#39236=CARTESIAN_POINT('Ctrl Pts',(133.816689918595,33.5439426298069,25.2922005468632));
#39237=CARTESIAN_POINT('Ctrl Pts',(133.774167520459,33.4324808072145,25.2863765490168));
#39238=CARTESIAN_POINT('Ctrl Pts',(133.726811586519,33.3230224942386,25.2805525511703));
#39239=CARTESIAN_POINT('Ctrl Pts',(133.674856337234,33.2160000278322,25.2747285533238));
#39240=CARTESIAN_POINT('Ctrl Pts',(133.661072326864,33.1876063850914,25.2731834150017));
#39241=CARTESIAN_POINT('Ctrl Pts',(133.646964825408,33.1593840427803,25.2716382766795));
#39242=CARTESIAN_POINT('Ctrl Pts',(133.632538719108,33.1313407335263,25.2700931383574));
#39243=CARTESIAN_POINT('Ctrl Pts',(133.578167029443,33.0256460938044,25.2642695446866));
#39244=CARTESIAN_POINT('Ctrl Pts',(133.519090795536,32.9221560327778,25.2584459510158));
#39245=CARTESIAN_POINT('Ctrl Pts',(133.455512663061,32.8213175459866,25.252622357345));
#39246=CARTESIAN_POINT('Ctrl Pts',(133.392014743844,32.7206062819248,25.2468061110026));
#39247=CARTESIAN_POINT('Ctrl Pts',(133.324026438936,32.6225402806349,25.2409898646602));
#39248=CARTESIAN_POINT('Ctrl Pts',(133.251797002751,32.5275434780567,25.2351736183179));
#39249=CARTESIAN_POINT('Ctrl Pts',(133.179639868629,32.4326417678017,25.2293631940702));
#39250=CARTESIAN_POINT('Ctrl Pts',(133.103250294645,32.3408034675099,25.2235527698225));
#39251=CARTESIAN_POINT('Ctrl Pts',(133.022921361145,32.2524244424704,25.2177423455748));
#39252=CARTESIAN_POINT('Ctrl Pts',(132.93955181135,32.1607000885202,25.2117119847504));
#39253=CARTESIAN_POINT('Ctrl Pts',(132.851939022808,32.0727024447851,25.2056816239259));
#39254=CARTESIAN_POINT('Ctrl Pts',(132.760457575814,31.9888376044902,25.1996512631015));
#39255=CARTESIAN_POINT('Ctrl Pts',(132.672411811515,31.9081223971538,25.193847378869));
#39256=CARTESIAN_POINT('Ctrl Pts',(132.58078305967,31.8312354684651,25.1880434946364));
#39257=CARTESIAN_POINT('Ctrl Pts',(132.48594302289,31.7585015367975,25.1822396104038));
#39258=CARTESIAN_POINT('Ctrl Pts',(132.391116994998,31.6857783487093,25.1764365834669));
#39259=CARTESIAN_POINT('Ctrl Pts',(132.293080949418,31.6172071861275,25.1706335565301));
#39260=CARTESIAN_POINT('Ctrl Pts',(132.192238888955,31.5530718525396,25.1648305295933));
#39261=CARTESIAN_POINT('Ctrl Pts',(132.091387925192,31.4889308564725,25.1590269903099));
#39262=CARTESIAN_POINT('Ctrl Pts',(131.987730798546,31.429226687216,25.1532234510264));
#39263=CARTESIAN_POINT('Ctrl Pts',(131.881699092076,31.3741989123944,25.147419911743));
#39264=CARTESIAN_POINT('Ctrl Pts',(131.775633000759,31.3191532927071,25.1416144904395));
#39265=CARTESIAN_POINT('Ctrl Pts',(131.667191160414,31.2687872714294,25.1358090691359));
#39266=CARTESIAN_POINT('Ctrl Pts',(131.556827668057,31.2232934172784,25.1300036478324));
#39267=CARTESIAN_POINT('Ctrl Pts',(131.446341958347,31.1777491828949,25.1241917975621));
#39268=CARTESIAN_POINT('Ctrl Pts',(131.333930726595,31.1370880411794,25.1183799472918));
#39269=CARTESIAN_POINT('Ctrl Pts',(131.220066014801,31.1014536145473,25.1125680970215));
#39270=CARTESIAN_POINT('Ctrl Pts',(131.106126516054,31.0657957830323,25.1067524294967));
#39271=CARTESIAN_POINT('Ctrl Pts',(130.990732029815,31.0351713462691,25.1009367619719));
#39272=CARTESIAN_POINT('Ctrl Pts',(130.874366029576,31.0096730652335,25.0951210944471));
#39273=CARTESIAN_POINT('Ctrl Pts',(130.757833347607,30.9841382606636,25.0892970966066));
#39274=CARTESIAN_POINT('Ctrl Pts',(130.640326774996,30.963744336958,25.0834730987661));
#39275=CARTESIAN_POINT('Ctrl Pts',(130.522336297019,30.9485323902546,25.0776491009256));
#39276=CARTESIAN_POINT('Ctrl Pts',(130.491032779941,30.9444965778603,25.0761039625467));
#39277=CARTESIAN_POINT('Ctrl Pts',(130.459695207566,30.9408252247593,25.0745588241678));
#39278=CARTESIAN_POINT('Ctrl Pts',(130.428332725702,30.9375184829844,25.0730136857889));
#39279=CARTESIAN_POINT('Ctrl Pts',(130.310128198923,30.9250554436,25.0671900921183));
#39280=CARTESIAN_POINT('Ctrl Pts',(130.191188658355,30.9177356190145,25.0613664984476));
#39281=CARTESIAN_POINT('Ctrl Pts',(130.071999041145,30.915634548908,25.055542904777));
#39282=CARTESIAN_POINT('Ctrl Pts',(129.952959799343,30.9135361296135,25.0497266584348));
#39283=CARTESIAN_POINT('Ctrl Pts',(129.833671513114,30.9166433760446,25.0439104120926));
#39284=CARTESIAN_POINT('Ctrl Pts',(129.714625382436,30.9249802052444,25.0380941657504));
#39285=CARTESIAN_POINT('Ctrl Pts',(129.595698417591,30.9333086892322,25.0322837415029));
#39286=CARTESIAN_POINT('Ctrl Pts',(129.477013531073,30.9468563135583,25.0264733172554));
#39287=CARTESIAN_POINT('Ctrl Pts',(129.359062469156,30.9655949532111,25.0206628930079));
#39288=CARTESIAN_POINT('Ctrl Pts',(129.236646715558,30.9850428891366,25.0146325321834));
#39289=CARTESIAN_POINT('Ctrl Pts',(129.115021885922,31.0100825943153,25.008602171359));
#39290=CARTESIAN_POINT('Ctrl Pts',(128.994732956179,31.0406233861114,25.0025718105345));
#39291=CARTESIAN_POINT('Ctrl Pts',(128.878961604683,31.0700171861025,24.9967679263021));
#39292=CARTESIAN_POINT('Ctrl Pts',(128.764428051714,31.1045062164083,24.9909640420697));
#39293=CARTESIAN_POINT('Ctrl Pts',(128.651607636186,31.1439575944749,24.9851601578374));
#39294=CARTESIAN_POINT('Ctrl Pts',(128.538803885439,31.1834031451509,24.9793571309008));
#39295=CARTESIAN_POINT('Ctrl Pts',(128.427713154245,31.2278094511495,24.9735541039642));
#39296=CARTESIAN_POINT('Ctrl Pts',(128.318794267271,31.2769941869184,24.9677510770276));
#39297=CARTESIAN_POINT('Ctrl Pts',(128.209865763899,31.3261832651849,24.9619475377444));
#39298=CARTESIAN_POINT('Ctrl Pts',(128.103109858166,31.3801514439701,24.9561439984613));
#39299=CARTESIAN_POINT('Ctrl Pts',(127.998963495633,31.4386690819032,24.9503404591781));
#39300=CARTESIAN_POINT('Ctrl Pts',(127.89478335965,31.497205696424,24.9445350378748));
#39301=CARTESIAN_POINT('Ctrl Pts',(127.793214805663,31.5602945042832,24.9387296165715));
#39302=CARTESIAN_POINT('Ctrl Pts',(127.694667812036,31.6276612709962,24.9329241952683));
#39303=CARTESIAN_POINT('Ctrl Pts',(127.596011686736,31.6951026401677,24.9271123449983));
#39304=CARTESIAN_POINT('Ctrl Pts',(127.500384138194,31.7668311939581,24.9213004947282));
#39305=CARTESIAN_POINT('Ctrl Pts',(127.408164044287,31.8425308586352,24.9154886444582));
#39306=CARTESIAN_POINT('Ctrl Pts',(127.315883379726,31.9182802432584,24.9096729769338));
#39307=CARTESIAN_POINT('Ctrl Pts',(127.227014930153,31.9980056611063,24.9038573094093));
#39308=CARTESIAN_POINT('Ctrl Pts',(127.141901300727,32.0813535970907,24.8980416418848));
#39309=CARTESIAN_POINT('Ctrl Pts',(127.056665755219,32.164820919993,24.8922176440446));
#39310=CARTESIAN_POINT('Ctrl Pts',(126.97519604275,32.2519208205696,24.8863936462044));
#39311=CARTESIAN_POINT('Ctrl Pts',(126.897795127026,32.3422660166799,24.8805696483642));
#39312=CARTESIAN_POINT('Ctrl Pts',(126.87726024207,32.3662350897981,24.879024509983));
#39313=CARTESIAN_POINT('Ctrl Pts',(126.857011512479,32.3904324290943,24.8774793716017));
#39314=CARTESIAN_POINT('Ctrl Pts',(126.837054078806,32.4148504686183,24.8759342332205));
#39315=CARTESIAN_POINT('Ctrl Pts',(126.762195742137,32.5064400914854,24.8701385737665));
#39316=CARTESIAN_POINT('Ctrl Pts',(126.691190191979,32.6014415258938,24.8643429143124));
#39317=CARTESIAN_POINT('Ctrl Pts',(126.624365980108,32.6994957153382,24.8585472548584));
#39318=CARTESIAN_POINT('Ctrl Pts',(126.557622092834,32.7974320408669,24.8527585619513));
#39319=CARTESIAN_POINT('Ctrl Pts',(126.495049783105,32.8984134903318,24.8469698690443));
#39320=CARTESIAN_POINT('Ctrl Pts',(126.436938220602,33.0020471086147,24.8411811761372));
#39321=CARTESIAN_POINT('Ctrl Pts',(126.378882465277,33.1055812028186,24.8353980423754));
#39322=CARTESIAN_POINT('Ctrl Pts',(126.325279140325,33.2117620446582,24.8296149086135));
#39323=CARTESIAN_POINT('Ctrl Pts',(126.276374442191,33.3201673579696,24.8238317748516));
#39324=CARTESIAN_POINT('Ctrl Pts',(126.227504892711,33.4284947585027,24.8180527975283));
#39325=CARTESIAN_POINT('Ctrl Pts',(126.183327422776,33.5390430764458,24.8122738202049));
#39326=CARTESIAN_POINT('Ctrl Pts',(126.144042212233,33.6513656763384,24.8064948428816));
#39327=CARTESIAN_POINT('Ctrl Pts',(126.104770622543,33.7636493320684,24.8007178692283));
#39328=CARTESIAN_POINT('Ctrl Pts',(126.070388060113,33.8777056596514,24.794940895575));
#39329=CARTESIAN_POINT('Ctrl Pts',(126.041046289915,33.9930687603403,24.7891639219217));
#39330=CARTESIAN_POINT('Ctrl Pts',(126.011711368872,34.1084049321902,24.7833882967689));
#39331=CARTESIAN_POINT('Ctrl Pts',(125.98741499763,34.2250468699919,24.7776126716161));
#39332=CARTESIAN_POINT('Ctrl Pts',(125.968258611743,34.3425151117976,24.7718370464633));
#39333=CARTESIAN_POINT('Ctrl Pts',(125.949095050159,34.4600273554534,24.7660592578475));
#39334=CARTESIAN_POINT('Ctrl Pts',(125.935075389371,34.5783661145012,24.7602814692317));
#39335=CARTESIAN_POINT('Ctrl Pts',(125.926249593193,34.6970435294684,24.7545036806159));
#39336=CARTESIAN_POINT('Ctrl Pts',(125.918668595408,34.7989825729109,24.7495407966091));
#39337=CARTESIAN_POINT('Ctrl Pts',(125.914918852587,34.9011712043574,24.7445779126023));
#39338=CARTESIAN_POINT('Ctrl Pts',(125.91500133219,35.0032990898339,24.7396150285955));
#39339=CARTESIAN_POINT('Origin',(130.,35.,32.7603849714045));
#39340=CARTESIAN_POINT('',(132.487160689988,38.2405642567579,26.7967734493137));
#39341=CARTESIAN_POINT('',(132.487160689988,38.2405642567579,26.6927660706478));
#39342=CARTESIAN_POINT('',(132.487160689988,38.2405642567579,32.7603849714045));
#39343=CARTESIAN_POINT('',(125.91500046357,35.0019461147839,25.8853849714464));
#39344=CARTESIAN_POINT('Ctrl Pts',(132.487160689988,38.2405642567579,26.6927660706478));
#39345=CARTESIAN_POINT('Ctrl Pts',(132.584486306372,38.1658660165692,26.6867872548488));
#39346=CARTESIAN_POINT('Ctrl Pts',(132.678341590377,38.0868578909177,26.6808084390498));
#39347=CARTESIAN_POINT('Ctrl Pts',(132.768344338777,38.0039132181141,26.6748296232508));
#39348=CARTESIAN_POINT('Ctrl Pts',(132.858347087177,37.9209685453105,26.6688508074517));
#39349=CARTESIAN_POINT('Ctrl Pts',(132.944497019818,37.8340876999327,26.6628719916527));
#39350=CARTESIAN_POINT('Ctrl Pts',(133.02645672952,37.7436808605129,26.6568931758537));
#39351=CARTESIAN_POINT('Ctrl Pts',(133.106288598548,37.6556211664249,26.6510695822666));
#39352=CARTESIAN_POINT('Ctrl Pts',(133.182402651793,37.563932319849,26.6452459886796));
#39353=CARTESIAN_POINT('Ctrl Pts',(133.254451673087,37.4689611798372,26.6394223950925));
#39354=CARTESIAN_POINT('Ctrl Pts',(133.32640979382,37.3741098600497,26.6336061488353));
#39355=CARTESIAN_POINT('Ctrl Pts',(133.39431283873,37.275984805828,26.6277899025781));
#39356=CARTESIAN_POINT('Ctrl Pts',(133.457851565369,37.1749684024999,26.6219736563209));
#39357=CARTESIAN_POINT('Ctrl Pts',(133.521326689378,37.0740531171726,26.6161632321596));
#39358=CARTESIAN_POINT('Ctrl Pts',(133.580445969959,36.9702525841654,26.6103528079983));
#39359=CARTESIAN_POINT('Ctrl Pts',(133.634941851192,36.8639803481948,26.604542383837));
#39360=CARTESIAN_POINT('Ctrl Pts',(133.691500515394,36.7536854860428,26.5985120229807));
#39361=CARTESIAN_POINT('Ctrl Pts',(133.743078583032,36.6407284626116,26.5924816621244));
#39362=CARTESIAN_POINT('Ctrl Pts',(133.789427576046,36.5256027156187,26.5864513012681));
#39363=CARTESIAN_POINT('Ctrl Pts',(133.834035882586,36.4148006403525,26.5806474171245));
#39364=CARTESIAN_POINT('Ctrl Pts',(133.873800632328,36.3019902142375,26.574843532981));
#39365=CARTESIAN_POINT('Ctrl Pts',(133.908548515556,36.1876335720844,26.5690396488374));
#39366=CARTESIAN_POINT('Ctrl Pts',(133.943291266146,36.0732938216467,26.5632366219905));
#39367=CARTESIAN_POINT('Ctrl Pts',(133.973018505244,35.9574086999655,26.5574335951435));
#39368=CARTESIAN_POINT('Ctrl Pts',(133.997606581845,35.8404561956399,26.5516305682966));
#39369=CARTESIAN_POINT('Ctrl Pts',(134.022196829313,35.7234933656456,26.5458270291037));
#39370=CARTESIAN_POINT('Ctrl Pts',(134.041646928137,35.6054633652587,26.5400234899109));
#39371=CARTESIAN_POINT('Ctrl Pts',(134.05588433561,35.4868544506889,26.5342199507181));
#39372=CARTESIAN_POINT('Ctrl Pts',(134.070126360107,35.3682070726434,26.5284145295058));
#39373=CARTESIAN_POINT('Ctrl Pts',(134.079152282759,35.2489808122703,26.5226091082934));
#39374=CARTESIAN_POINT('Ctrl Pts',(134.082941474663,35.1296684791143,26.5168036870811));
#39375=CARTESIAN_POINT('Ctrl Pts',(134.086734862746,35.0102240186003,26.5109918369025));
#39376=CARTESIAN_POINT('Ctrl Pts',(134.085279931423,34.8906937034143,26.5051799867239));
#39377=CARTESIAN_POINT('Ctrl Pts',(134.078608182355,34.7715699344925,26.4993681365453));
#39378=CARTESIAN_POINT('Ctrl Pts',(134.071932051247,34.6523679244463,26.4935524691127));
#39379=CARTESIAN_POINT('Ctrl Pts',(134.060032319172,34.5335733978143,26.48773680168));
#39380=CARTESIAN_POINT('Ctrl Pts',(134.042992121292,34.4156715759345,26.4819211342473));
#39381=CARTESIAN_POINT('Ctrl Pts',(134.025927515168,34.2976008724203,26.4760971364987));
#39382=CARTESIAN_POINT('Ctrl Pts',(134.003707822574,34.1804258256439,26.4702731387502));
#39383=CARTESIAN_POINT('Ctrl Pts',(133.976466834666,34.0646195892561,26.4644491410016));
#39384=CARTESIAN_POINT('Ctrl Pts',(133.969239647923,34.0338955457959,26.4629040017628));
#39385=CARTESIAN_POINT('Ctrl Pts',(133.961659295102,34.0032677538822,26.461358862524));
#39386=CARTESIAN_POINT('Ctrl Pts',(133.953728849266,33.9727448289353,26.4598137232852));
#39387=CARTESIAN_POINT('Ctrl Pts',(133.923839184085,33.8577046375087,26.4539901295726));
#39388=CARTESIAN_POINT('Ctrl Pts',(133.888876229057,33.7437845508683,26.44816653586));
#39389=CARTESIAN_POINT('Ctrl Pts',(133.848939755856,33.6314651061112,26.4423429421474));
#39390=CARTESIAN_POINT('Ctrl Pts',(133.809053668444,33.519287369007,26.4365266957627));
#39391=CARTESIAN_POINT('Ctrl Pts',(133.764206678945,33.4087066385016,26.4307104493781));
#39392=CARTESIAN_POINT('Ctrl Pts',(133.714549087991,33.3001911657764,26.4248942029934));
#39393=CARTESIAN_POINT('Ctrl Pts',(133.664941204556,33.1917843176292,26.419083778703));
#39394=CARTESIAN_POINT('Ctrl Pts',(133.610532468321,33.0854389837292,26.4132733544126));
#39395=CARTESIAN_POINT('Ctrl Pts',(133.551522091769,32.98160563029,26.4074629301222));
#39396=CARTESIAN_POINT('Ctrl Pts',(133.490278051012,32.8738419707181,26.4014325693136));
#39397=CARTESIAN_POINT('Ctrl Pts',(133.42407727388,32.7687846385915,26.3954022085051));
#39398=CARTESIAN_POINT('Ctrl Pts',(133.353196250823,32.6669119383383,26.3893718476965));
#39399=CARTESIAN_POINT('Ctrl Pts',(133.284977239016,32.568865174316,26.3835679634204));
#39400=CARTESIAN_POINT('Ctrl Pts',(133.212423438947,32.4737685168427,26.3777640791442));
#39401=CARTESIAN_POINT('Ctrl Pts',(133.135826364783,32.3820202426427,26.3719601948681));
#39402=CARTESIAN_POINT('Ctrl Pts',(133.059240604823,32.2902855206403,26.3661571678875));
#39403=CARTESIAN_POINT('Ctrl Pts',(132.978613020103,32.2018985116969,26.360354140907));
#39404=CARTESIAN_POINT('Ctrl Pts',(132.894275605537,32.1172246498917,26.3545511139264));
#39405=CARTESIAN_POINT('Ctrl Pts',(132.809930744858,32.0325433122674,26.348747574599));
#39406=CARTESIAN_POINT('Ctrl Pts',(132.721875691282,31.9515760629171,26.3429440352717));
#39407=CARTESIAN_POINT('Ctrl Pts',(132.630479042968,31.8746512187425,26.3371404959443));
#39408=CARTESIAN_POINT('Ctrl Pts',(132.539052755784,31.7977014287365,26.3313350745967));
#39409=CARTESIAN_POINT('Ctrl Pts',(132.444283030994,31.7247969138078,26.3255296532491));
#39410=CARTESIAN_POINT('Ctrl Pts',(132.346570732286,31.656225067625,26.3197242319015));
#39411=CARTESIAN_POINT('Ctrl Pts',(132.248750226252,31.5875772844704,26.3139123815872));
#39412=CARTESIAN_POINT('Ctrl Pts',(132.147980976242,31.5232719820419,26.3081005312729));
#39413=CARTESIAN_POINT('Ctrl Pts',(132.044692080272,31.4635527295215,26.3022886809585));
#39414=CARTESIAN_POINT('Ctrl Pts',(131.9413353436,31.4037942530754,26.2964730133897));
#39415=CARTESIAN_POINT('Ctrl Pts',(131.835456026457,31.3486280135417,26.2906573458209));
#39416=CARTESIAN_POINT('Ctrl Pts',(131.727505525656,31.2982504597383,26.2848416782521));
#39417=CARTESIAN_POINT('Ctrl Pts',(131.619400397425,31.2478007455318,26.2790176803678));
#39418=CARTESIAN_POINT('Ctrl Pts',(131.509218539976,31.2021535635289,26.2731936824835));
#39419=CARTESIAN_POINT('Ctrl Pts',(131.397429024825,31.1614563802691,26.2673696845992));
#39420=CARTESIAN_POINT('Ctrl Pts',(131.367770665239,31.1506591986764,26.2658245466384));
#39421=CARTESIAN_POINT('Ctrl Pts',(131.33799921508,31.1402101560168,26.2642794086776));
#39422=CARTESIAN_POINT('Ctrl Pts',(131.308123564557,31.1301114047234,26.2627342707168));
#39423=CARTESIAN_POINT('Ctrl Pts',(131.195522843021,31.0920494157021,26.2569106770474));
#39424=CARTESIAN_POINT('Ctrl Pts',(131.081077952103,31.0588445804792,26.251087083378));
#39425=CARTESIAN_POINT('Ctrl Pts',(130.965245490355,31.0306768658436,26.2452634897086));
#39426=CARTESIAN_POINT('Ctrl Pts',(130.849559168461,31.0025446889636,26.2394472433676));
#39427=CARTESIAN_POINT('Ctrl Pts',(130.732489150968,30.9794370882101,26.2336309970266));
#39428=CARTESIAN_POINT('Ctrl Pts',(130.614509458979,30.9614850347156,26.2278147506856));
#39429=CARTESIAN_POINT('Ctrl Pts',(130.49664786531,30.9435509513255,26.2220043264392));
#39430=CARTESIAN_POINT('Ctrl Pts',(130.377878810019,30.9307622096322,26.2161939021928));
#39431=CARTESIAN_POINT('Ctrl Pts',(130.258688251068,30.923199123239,26.2103834779464));
#39432=CARTESIAN_POINT('Ctrl Pts',(130.134986082876,30.915349758379,26.2043531171215));
#39433=CARTESIAN_POINT('Ctrl Pts',(130.010830306498,30.9131295749625,26.1983227562966));
#39434=CARTESIAN_POINT('Ctrl Pts',(129.88677252396,30.9165695134275,26.1922923954716));
#39435=CARTESIAN_POINT('Ctrl Pts',(129.767373862957,30.9198802613568,26.1864885112402));
#39436=CARTESIAN_POINT('Ctrl Pts',(129.648066412887,30.9284336419937,26.1806846270087));
#39437=CARTESIAN_POINT('Ctrl Pts',(129.529343078354,30.9422041620965,26.1748807427772));
#39438=CARTESIAN_POINT('Ctrl Pts',(129.410637280526,30.9559726481463,26.1690777158414));
#39439=CARTESIAN_POINT('Ctrl Pts',(129.29251583216,30.9749566940936,26.1632746889056));
#39440=CARTESIAN_POINT('Ctrl Pts',(129.175466359288,30.9990789466257,26.1574716619699));
#39441=CARTESIAN_POINT('Ctrl Pts',(129.05840655217,31.0232033289008,26.1516681226874));
#39442=CARTESIAN_POINT('Ctrl Pts',(128.942419308674,31.0524667373019,26.1458645834049));
#39443=CARTESIAN_POINT('Ctrl Pts',(128.827981275663,31.0867408583377,26.1400610441225));
#39444=CARTESIAN_POINT('Ctrl Pts',(128.713506131731,31.1210260940716,26.1342556228199));
#39445=CARTESIAN_POINT('Ctrl Pts',(128.600581588393,31.1603251569359,26.1284502015172));
#39446=CARTESIAN_POINT('Ctrl Pts',(128.489667752289,31.2044603148532,26.1226447802146));
#39447=CARTESIAN_POINT('Ctrl Pts',(128.378631089375,31.2486443483737,26.1168329299451));
#39448=CARTESIAN_POINT('Ctrl Pts',(128.269609957951,31.2976750159768,26.1110210796756));
#39449=CARTESIAN_POINT('Ctrl Pts',(128.16304328815,31.3513269482195,26.1052092294061));
#39450=CARTESIAN_POINT('Ctrl Pts',(128.056406624787,31.40501411934,26.099393561882));
#39451=CARTESIAN_POINT('Ctrl Pts',(127.952227989088,31.4633284009306,26.093577894358));
#39452=CARTESIAN_POINT('Ctrl Pts',(127.85091912446,31.5259999438126,26.087762226834));
#39453=CARTESIAN_POINT('Ctrl Pts',(127.749465145822,31.5887612569136,26.0819382289941));
#39454=CARTESIAN_POINT('Ctrl Pts',(127.650889479172,31.6558920595854,26.0761142311542));
#39455=CARTESIAN_POINT('Ctrl Pts',(127.555572589185,31.7270808697345,26.0702902333143));
#39456=CARTESIAN_POINT('Ctrl Pts',(127.530284498452,31.7459676493019,26.0687450949257));
#39457=CARTESIAN_POINT('Ctrl Pts',(127.505225589071,31.7651398518029,26.067199956537));
#39458=CARTESIAN_POINT('Ctrl Pts',(127.480402534567,31.7845912216043,26.0656548181484));
#39459=CARTESIAN_POINT('Ctrl Pts',(127.387890871814,31.8570834510718,26.0598963277298));
#39460=CARTESIAN_POINT('Ctrl Pts',(127.298344601785,31.9337015222224,26.0541378373113));
#39461=CARTESIAN_POINT('Ctrl Pts',(127.212159759072,32.0141715067564,26.0483793468928));
#39462=CARTESIAN_POINT('Ctrl Pts',(127.126084184855,32.0945394683149,26.0426281573123));
#39463=CARTESIAN_POINT('Ctrl Pts',(127.043361868386,32.1787493515523,26.0368769677318));
#39464=CARTESIAN_POINT('Ctrl Pts',(126.964357841701,32.2664854698104,26.0311257781514));
#39465=CARTESIAN_POINT('Ctrl Pts',(126.885432208038,32.3541345304871,26.0253802952817));
#39466=CARTESIAN_POINT('Ctrl Pts',(126.810217805867,32.4453025593198,26.0196348124121));
#39467=CARTESIAN_POINT('Ctrl Pts',(126.739044130039,32.5396358370833,26.0138893295424));
#39468=CARTESIAN_POINT('Ctrl Pts',(126.667920512356,32.6339027680003,26.0081478876081));
#39469=CARTESIAN_POINT('Ctrl Pts',(126.600832219958,32.731330187218,26.0024064456737));
#39470=CARTESIAN_POINT('Ctrl Pts',(126.538069144984,32.8315305501143,25.9966650037393));
#39471=CARTESIAN_POINT('Ctrl Pts',(126.47532866335,32.9316948430618,25.990925628599));
#39472=CARTESIAN_POINT('Ctrl Pts',(126.416910526326,33.0346297414538,25.9851862534588));
#39473=CARTESIAN_POINT('Ctrl Pts',(126.363061503255,33.1399184504729,25.9794468783185));
#39474=CARTESIAN_POINT('Ctrl Pts',(126.309218443451,33.2451954997685,25.9737081387594));
#39475=CARTESIAN_POINT('Ctrl Pts',(126.259943681612,33.3528254686493,25.9679693992004));
#39476=CARTESIAN_POINT('Ctrl Pts',(126.215437817399,33.4623673761183,25.9622306596413));
#39477=CARTESIAN_POINT('Ctrl Pts',(126.170925788959,33.5719244555462,25.9564911252456));
#39478=CARTESIAN_POINT('Ctrl Pts',(126.131184127378,33.6833936117948,25.9507515908499));
#39479=CARTESIAN_POINT('Ctrl Pts',(126.09636482613,33.7963150622686,25.9450120564542));
#39480=CARTESIAN_POINT('Ctrl Pts',(126.061513761249,33.9093395244424,25.9392672862137));
#39481=CARTESIAN_POINT('Ctrl Pts',(126.031594144115,34.0238185252172,25.9335225159732));
#39482=CARTESIAN_POINT('Ctrl Pts',(126.006707715964,34.1392783642426,25.9277777457326));
#39483=CARTESIAN_POINT('Ctrl Pts',(125.981808406242,34.2547979669366,25.9220300019166));
#39484=CARTESIAN_POINT('Ctrl Pts',(125.961947542634,34.3712990066402,25.9162822581006));
#39485=CARTESIAN_POINT('Ctrl Pts',(125.947175220413,34.4883005706798,25.9105345142846));
#39486=CARTESIAN_POINT('Ctrl Pts',(125.932382690921,34.6054621828346,25.9047789080475));
#39487=CARTESIAN_POINT('Ctrl Pts',(125.922692631631,34.7231252698855,25.8990233018104));
#39488=CARTESIAN_POINT('Ctrl Pts',(125.91810307506,34.8408067395617,25.8932676955733));
#39489=CARTESIAN_POINT('Ctrl Pts',(125.916007830481,34.8945312024069,25.8906401208644));
#39490=CARTESIAN_POINT('Ctrl Pts',(125.914974887006,34.9482595324203,25.8880125461554));
#39491=CARTESIAN_POINT('Ctrl Pts',(125.91500046357,35.0019461147839,25.8853849714464));
#39492=CARTESIAN_POINT('Ctrl Pts',(125.91500046357,35.0019461156404,25.8853849714045));
#39493=CARTESIAN_POINT('Ctrl Pts',(125.915055004632,35.1164306863377,25.879781769463));
#39494=CARTESIAN_POINT('Ctrl Pts',(125.919921914211,35.2307950927835,25.8741785675215));
#39495=CARTESIAN_POINT('Ctrl Pts',(125.92957331797,35.3447486420832,25.8685753655799));
#39496=CARTESIAN_POINT('Ctrl Pts',(125.939604342104,35.4631843465316,25.8627517719035));
#39497=CARTESIAN_POINT('Ctrl Pts',(125.954824952508,35.5813728704778,25.856928178227));
#39498=CARTESIAN_POINT('Ctrl Pts',(125.975217969216,35.6988237293334,25.8511045845505));
#39499=CARTESIAN_POINT('Ctrl Pts',(125.995585257104,35.8161264064861,25.8452883382024));
#39500=CARTESIAN_POINT('Ctrl Pts',(126.021111902476,35.932692870866,25.8394720918543));
#39501=CARTESIAN_POINT('Ctrl Pts',(126.051728847284,36.0480362134157,25.8336558455062));
#39502=CARTESIAN_POINT('Ctrl Pts',(126.082315144361,36.1632640966445,25.8278454212528));
#39503=CARTESIAN_POINT('Ctrl Pts',(126.117981500012,36.2772709013383,25.8220349969993));
#39504=CARTESIAN_POINT('Ctrl Pts',(126.158607643251,36.3895789871435,25.8162245727458));
#39505=CARTESIAN_POINT('Ctrl Pts',(126.20077156999,36.5061381661497,25.8101942119235));
#39506=CARTESIAN_POINT('Ctrl Pts',(126.248278102885,36.6208670436773,25.8041638511013));
#39507=CARTESIAN_POINT('Ctrl Pts',(126.300935504727,36.7332474894862,25.798133490279));
#39508=CARTESIAN_POINT('Ctrl Pts',(126.351615302105,36.8414073686986,25.7923296060405));
#39509=CARTESIAN_POINT('Ctrl Pts',(126.407065864032,36.9473916277977,25.7865257218021));
#39510=CARTESIAN_POINT('Ctrl Pts',(126.467067129435,37.050758477266,25.7807218375636));
#39511=CARTESIAN_POINT('Ctrl Pts',(126.527059532009,37.1541100583459,25.7749188106208));
#39512=CARTESIAN_POINT('Ctrl Pts',(126.59160109635,37.2548446456019,25.7691157836781));
#39513=CARTESIAN_POINT('Ctrl Pts',(126.660426315324,37.352545983529,25.7633127567354));
#39514=CARTESIAN_POINT('Ctrl Pts',(126.729257610845,37.4502559474628,25.757509217446));
#39515=CARTESIAN_POINT('Ctrl Pts',(126.802373077781,37.5449317957676,25.7517056781567));
#39516=CARTESIAN_POINT('Ctrl Pts',(126.879464862812,37.6361876749538,25.7459021388673));
#39517=CARTESIAN_POINT('Ctrl Pts',(126.956581647811,37.7274731473578,25.7400967175578));
#39518=CARTESIAN_POINT('Ctrl Pts',(127.037677051997,37.8153361332125,25.7342912962484));
#39519=CARTESIAN_POINT('Ctrl Pts',(127.12240450845,37.8994256650257,25.7284858749389));
#39520=CARTESIAN_POINT('Ctrl Pts',(127.207225792718,37.9836083182119,25.7226740246626));
#39521=CARTESIAN_POINT('Ctrl Pts',(127.295686867834,38.0640088883964,25.7168621743864));
#39522=CARTESIAN_POINT('Ctrl Pts',(127.387405936573,38.1403148344941,25.7110503241102));
#39523=CARTESIAN_POINT('Ctrl Pts',(127.479185246888,38.2166708987469,25.7052346565794));
#39524=CARTESIAN_POINT('Ctrl Pts',(127.574226488114,38.2889267363997,25.6994189890488));
#39525=CARTESIAN_POINT('Ctrl Pts',(127.672117926347,38.3568124837658,25.6936033215181));
#39526=CARTESIAN_POINT('Ctrl Pts',(127.770149583495,38.4247954701341,25.6877793236716));
#39527=CARTESIAN_POINT('Ctrl Pts',(127.871039242095,38.4883956552465,25.6819553258252));
#39528=CARTESIAN_POINT('Ctrl Pts',(127.97434947477,38.5473884689492,25.6761313279788));
#39529=CARTESIAN_POINT('Ctrl Pts',(128.001758241705,38.5630395834591,25.6745861896563));
#39530=CARTESIAN_POINT('Ctrl Pts',(128.029337272291,38.5783666599941,25.6730410513339));
#39531=CARTESIAN_POINT('Ctrl Pts',(128.057078167552,38.5933660755618,25.6714959130115));
#39532=CARTESIAN_POINT('Ctrl Pts',(128.161633015309,38.6498985557273,25.6656723193407));
#39533=CARTESIAN_POINT('Ctrl Pts',(128.268825870595,38.7019551203421,25.6598487256699));
#39534=CARTESIAN_POINT('Ctrl Pts',(128.378237088824,38.7492812724484,25.6540251319991));
#39535=CARTESIAN_POINT('Ctrl Pts',(128.487510268548,38.7965477155841,25.6482088856567));
#39536=CARTESIAN_POINT('Ctrl Pts',(128.598995873004,38.8390954559754,25.6423926393143));
#39537=CARTESIAN_POINT('Ctrl Pts',(128.712248810399,38.8767153459701,25.636576392972));
#39538=CARTESIAN_POINT('Ctrl Pts',(128.825388380978,38.9142975782473,25.6307659687243));
#39539=CARTESIAN_POINT('Ctrl Pts',(128.940291379782,38.9469616453496,25.6249555444766));
#39540=CARTESIAN_POINT('Ctrl Pts',(129.056492394029,38.9745463134143,25.6191451202289));
#39541=CARTESIAN_POINT('Ctrl Pts',(129.177091857028,39.0031751182245,25.6131147594045));
#39542=CARTESIAN_POINT('Ctrl Pts',(129.299089130788,39.0263322167952,25.6070843985801));
#39543=CARTESIAN_POINT('Ctrl Pts',(129.42194576277,39.0438939524696,25.6010540377557));
#39544=CARTESIAN_POINT('Ctrl Pts',(129.540188383733,39.0607961385487,25.5952501535231));
#39545=CARTESIAN_POINT('Ctrl Pts',(129.65922653817,39.0725155991235,25.5894462692905));
#39546=CARTESIAN_POINT('Ctrl Pts',(129.778570096612,39.0789942140049,25.5836423850578));
#39547=CARTESIAN_POINT('Ctrl Pts',(129.897896026733,39.0854718719255,25.577839358121));
#39548=CARTESIAN_POINT('Ctrl Pts',(130.017526863521,39.0867102015225,25.5720363311842));
#39549=CARTESIAN_POINT('Ctrl Pts',(130.13696892154,39.0827030891962,25.5662333042473));
#39550=CARTESIAN_POINT('Ctrl Pts',(130.256421525044,39.0786956230838,25.5604297649639));
#39551=CARTESIAN_POINT('Ctrl Pts',(130.375684908514,39.0694418079503,25.5546262256805));
#39552=CARTESIAN_POINT('Ctrl Pts',(130.494267601246,39.0549876126023,25.548822686397));
#39553=CARTESIAN_POINT('Ctrl Pts',(130.612888748963,39.0405287299273,25.5430172650935));
#39554=CARTESIAN_POINT('Ctrl Pts',(130.730828361813,39.0208661625053,25.5372118437899));
#39555=CARTESIAN_POINT('Ctrl Pts',(130.84760292535,38.9960973813133,25.5314064224864));
#39556=CARTESIAN_POINT('Ctrl Pts',(130.964506805907,38.9713011709886,25.5255945722161));
#39557=CARTESIAN_POINT('Ctrl Pts',(131.080242662145,38.9413875444868,25.5197827219458));
#39558=CARTESIAN_POINT('Ctrl Pts',(131.194339806388,38.9065045023494,25.5139708716754));
#39559=CARTESIAN_POINT('Ctrl Pts',(131.308511890249,38.8715985488427,25.5081552041507));
#39560=CARTESIAN_POINT('Ctrl Pts',(131.421042734611,38.8317168155747,25.5023395366259));
#39561=CARTESIAN_POINT('Ctrl Pts',(131.531480935746,38.7870557354556,25.4965238691011));
#39562=CARTESIAN_POINT('Ctrl Pts',(131.642077327679,38.7423306831618,25.4906998712606));
#39563=CARTESIAN_POINT('Ctrl Pts',(131.750574723409,38.6928127889152,25.48487587342));
#39564=CARTESIAN_POINT('Ctrl Pts',(131.856545517186,38.6387448031729,25.4790518755795));
#39565=CARTESIAN_POINT('Ctrl Pts',(131.884660146514,38.6244002717834,25.4775067372007));
#39566=CARTESIAN_POINT('Ctrl Pts',(131.91259709215,38.6097357109502,25.4759615988218));
#39567=CARTESIAN_POINT('Ctrl Pts',(131.940348719912,38.594756159343,25.474416460443));
#39568=CARTESIAN_POINT('Ctrl Pts',(132.044926391121,38.5383080606497,25.4685938479917));
#39569=CARTESIAN_POINT('Ctrl Pts',(132.147207370059,38.4772016462083,25.4627712355404));
#39570=CARTESIAN_POINT('Ctrl Pts',(132.246748991069,38.4116482777579,25.456948623089));
#39571=CARTESIAN_POINT('Ctrl Pts',(132.3288274834,38.3575952937399,25.4521475032501));
#39572=CARTESIAN_POINT('Ctrl Pts',(132.409043673025,38.3005197331551,25.4473463834112));
#39573=CARTESIAN_POINT('Ctrl Pts',(132.487160689988,38.2405642567579,25.4425452635723));
#39574=CARTESIAN_POINT('',(125.915000988625,34.9971579821973,25.9896150286367));
#39575=CARTESIAN_POINT('Ctrl Pts',(125.915000988624,34.997157983046,25.9896150285955));
#39576=CARTESIAN_POINT('Ctrl Pts',(125.914917631215,35.1169725160829,25.98379925565));
#39577=CARTESIAN_POINT('Ctrl Pts',(125.920109897601,35.2368329689649,25.9779834827046));
#39578=CARTESIAN_POINT('Ctrl Pts',(125.930563220773,35.3562433155562,25.9721677097591));
#39579=CARTESIAN_POINT('Ctrl Pts',(125.94101582311,35.4756454279067,25.9663523378549));
#39580=CARTESIAN_POINT('Ctrl Pts',(125.956728725647,35.594597091786,25.9605369659506));
#39581=CARTESIAN_POINT('Ctrl Pts',(125.977635392703,35.7126064593879,25.9547215940464));
#39582=CARTESIAN_POINT('Ctrl Pts',(125.998545461783,35.8306350299897,25.9489052758395));
#39583=CARTESIAN_POINT('Ctrl Pts',(126.024650905994,35.9477206000163,25.9430889576325));
#39584=CARTESIAN_POINT('Ctrl Pts',(126.055833996177,36.0633811801447,25.9372726394256));
#39585=CARTESIAN_POINT('Ctrl Pts',(126.087029385138,36.1790873774281,25.9314540272315));
#39586=CARTESIAN_POINT('Ctrl Pts',(126.123306298704,36.2933670755061,25.9256354150373));
#39587=CARTESIAN_POINT('Ctrl Pts',(126.164497225096,36.4057536995169,25.9198168028432));
#39588=CARTESIAN_POINT('Ctrl Pts',(126.205738353568,36.5182772964668,25.9139910991253));
#39589=CARTESIAN_POINT('Ctrl Pts',(126.251905311341,36.6289028324717,25.9081653954074));
#39590=CARTESIAN_POINT('Ctrl Pts',(126.302782435844,36.7371837218019,25.9023396916895));
#39591=CARTESIAN_POINT('Ctrl Pts',(126.353695625473,36.8455413679057,25.8965098583212));
#39592=CARTESIAN_POINT('Ctrl Pts',(126.40932544393,36.9515506989297,25.8906800249529));
#39593=CARTESIAN_POINT('Ctrl Pts',(126.469411107916,37.0547912485437,25.8848501915846));
#39594=CARTESIAN_POINT('Ctrl Pts',(126.529589512789,37.1581911476518,25.879011359998));
#39595=CARTESIAN_POINT('Ctrl Pts',(126.594237274574,37.2588133939343,25.8731725284114));
#39596=CARTESIAN_POINT('Ctrl Pts',(126.663051158455,37.3562676904181,25.8673336968249));
#39597=CARTESIAN_POINT('Ctrl Pts',(126.686630918671,37.3896613722392,25.8653329632375));
#39598=CARTESIAN_POINT('Ctrl Pts',(126.710699509632,37.422683385099,25.8633322296501));
#39599=CARTESIAN_POINT('Ctrl Pts',(126.735243706803,37.4553189906879,25.8613314960627));
#39600=CARTESIAN_POINT('Ctrl Pts',(126.80668521814,37.5503124007564,25.8555079023934));
#39601=CARTESIAN_POINT('Ctrl Pts',(126.882391357813,37.6423383457659,25.849684308724));
#39602=CARTESIAN_POINT('Ctrl Pts',(126.962086897633,37.7309904764516,25.8438607150547));
#39603=CARTESIAN_POINT('Ctrl Pts',(127.041681889693,37.8195307593073,25.8380444687137));
#39604=CARTESIAN_POINT('Ctrl Pts',(127.125256000358,37.9047053930594,25.8322282223727));
#39605=CARTESIAN_POINT('Ctrl Pts',(127.212491956809,37.9861386285879,25.8264119760317));
#39606=CARTESIAN_POINT('Ctrl Pts',(127.299640589587,38.067490348999,25.8206015517854));
#39607=CARTESIAN_POINT('Ctrl Pts',(127.390443479258,38.1451078446809,25.814791127539));
#39608=CARTESIAN_POINT('Ctrl Pts',(127.484544897527,38.2186504357325,25.8089807032926));
#39609=CARTESIAN_POINT('Ctrl Pts',(127.582208249157,38.2949767660032,25.8029503424677));
#39610=CARTESIAN_POINT('Ctrl Pts',(127.683424475913,38.3669132759528,25.7969199816428));
#39611=CARTESIAN_POINT('Ctrl Pts',(127.787755792911,38.4341229692894,25.7908896208178));
#39612=CARTESIAN_POINT('Ctrl Pts',(127.888168836699,38.4988085313446,25.7850857365864));
#39613=CARTESIAN_POINT('Ctrl Pts',(127.9914668351,38.5591156742766,25.7792818523549));
#39614=CARTESIAN_POINT('Ctrl Pts',(128.097228583066,38.6147871216571,25.7734779681235));
#39615=CARTESIAN_POINT('Ctrl Pts',(128.202974708892,38.6704503457703,25.7676749411877));
#39616=CARTESIAN_POINT('Ctrl Pts',(128.311183499321,38.7214790459172,25.761871914252));
#39617=CARTESIAN_POINT('Ctrl Pts',(128.421408823275,38.7676617280172,25.7560688873162));
#39618=CARTESIAN_POINT('Ctrl Pts',(128.531643878974,38.8138484875657,25.7502653480338));
#39619=CARTESIAN_POINT('Ctrl Pts',(128.643895445548,38.8551882205887,25.7444618087514));
#39620=CARTESIAN_POINT('Ctrl Pts',(128.757697678908,38.8915176914681,25.738658269469));
#39621=CARTESIAN_POINT('Ctrl Pts',(128.871536817006,38.9278589435716,25.7328528481664));
#39622=CARTESIAN_POINT('Ctrl Pts',(128.986927233176,38.9591865781146,25.7270474268638));
#39623=CARTESIAN_POINT('Ctrl Pts',(129.103388830487,38.9853874856412,25.7212420055612));
#39624=CARTESIAN_POINT('Ctrl Pts',(129.219979398241,39.0116174082482,25.7154301552917));
#39625=CARTESIAN_POINT('Ctrl Pts',(129.337643116344,39.0327091816321,25.7096183050222));
#39626=CARTESIAN_POINT('Ctrl Pts',(129.455890467265,39.0486009702596,25.7038064547528));
#39627=CARTESIAN_POINT('Ctrl Pts',(129.574215483682,39.0645031966995,25.6979907872288));
#39628=CARTESIAN_POINT('Ctrl Pts',(129.693124490574,39.0751986000751,25.6921751197048));
#39629=CARTESIAN_POINT('Ctrl Pts',(129.812125293181,39.0806774063307,25.6863594521808));
#39630=CARTESIAN_POINT('Ctrl Pts',(129.931296551591,39.0861640603848,25.6805354543409));
#39631=CARTESIAN_POINT('Ctrl Pts',(130.05055946127,39.0864192023192,25.6747114565011));
#39632=CARTESIAN_POINT('Ctrl Pts',(130.16942413495,39.0814850805187,25.6688874586612));
#39633=CARTESIAN_POINT('Ctrl Pts',(130.200959581124,39.080176031096,25.6673423202722));
#39634=CARTESIAN_POINT('Ctrl Pts',(130.23246703944,39.0785020063004,25.6657971818833));
#39635=CARTESIAN_POINT('Ctrl Pts',(130.263937469796,39.0764644009285,25.6642520434943));
#39636=CARTESIAN_POINT('Ctrl Pts',(130.382535283496,39.0687855881652,25.6584291159804));
#39637=CARTESIAN_POINT('Ctrl Pts',(130.500988941927,39.0559144961333,25.6526061884665));
#39638=CARTESIAN_POINT('Ctrl Pts',(130.618807884703,39.037858566348,25.6467832609526));
#39639=CARTESIAN_POINT('Ctrl Pts',(130.736486110335,39.0198242016761,25.6409672880565));
#39640=CARTESIAN_POINT('Ctrl Pts',(130.853530727797,38.9966173737414,25.6351513151605));
#39641=CARTESIAN_POINT('Ctrl Pts',(130.969453622282,38.9682974528435,25.6293353422645));
#39642=CARTESIAN_POINT('Ctrl Pts',(131.085265436093,38.9400046689139,25.6235249424021));
#39643=CARTESIAN_POINT('Ctrl Pts',(131.199957270419,38.906608633073,25.6177145425397));
#39644=CARTESIAN_POINT('Ctrl Pts',(131.313049197558,38.8682201081106,25.6119041426773));
#39645=CARTESIAN_POINT('Ctrl Pts',(131.426056890354,38.8298601761014,25.6060980705793));
#39646=CARTESIAN_POINT('Ctrl Pts',(131.537466661937,38.7865152853884,25.6002919984813));
#39647=CARTESIAN_POINT('Ctrl Pts',(131.646812448058,38.738346393918,25.5944859263833));
#39648=CARTESIAN_POINT('Ctrl Pts',(131.756109391884,38.6901990184048,25.5886824477267));
#39649=CARTESIAN_POINT('Ctrl Pts',(131.863343811702,38.6372320940027,25.5828789690701));
#39650=CARTESIAN_POINT('Ctrl Pts',(131.968068894652,38.5796549869927,25.5770754904136));
#39651=CARTESIAN_POINT('Ctrl Pts',(132.072791333086,38.5220793339191,25.5712721583064));
#39652=CARTESIAN_POINT('Ctrl Pts',(132.175004198713,38.4598939186473,25.5654688261992));
#39653=CARTESIAN_POINT('Ctrl Pts',(132.274284934972,38.3933542453682,25.559665494092));
#39654=CARTESIAN_POINT('Ctrl Pts',(132.346861709583,38.3447120308537,25.5554231088901));
#39655=CARTESIAN_POINT('Ctrl Pts',(132.417872043576,38.2937438835033,25.5511807236882));
#39656=CARTESIAN_POINT('Ctrl Pts',(132.487160689988,38.2405642567579,25.5469383384863));
#39657=CARTESIAN_POINT('Ctrl Pts',(132.487160689988,38.2405642567579,26.7967734493137));
#39658=CARTESIAN_POINT('Ctrl Pts',(132.581820861397,38.1679117683082,26.7909668267509));
#39659=CARTESIAN_POINT('Ctrl Pts',(132.673369460366,38.0910510166544,26.7851602041881));
#39660=CARTESIAN_POINT('Ctrl Pts',(132.761416222849,38.0102832830462,26.7793535816253));
#39661=CARTESIAN_POINT('Ctrl Pts',(132.849425891177,37.9295495769333,26.7735494053961));
#39662=CARTESIAN_POINT('Ctrl Pts',(132.933936355778,37.8449124368826,26.7677452291669));
#39663=CARTESIAN_POINT('Ctrl Pts',(133.014590961074,37.7567129588351,26.7619410529378));
#39664=CARTESIAN_POINT('Ctrl Pts',(133.09523030081,37.6685301743726,26.7561379752696));
#39665=CARTESIAN_POINT('Ctrl Pts',(133.17201495707,37.5767866939246,26.7503348976015));
#39666=CARTESIAN_POINT('Ctrl Pts',(133.244626098886,37.4818594799925,26.7445318199333));
#39667=CARTESIAN_POINT('Ctrl Pts',(133.317240633817,37.386927830117,26.7387284710877));
#39668=CARTESIAN_POINT('Ctrl Pts',(133.385681018521,37.2888124753689,26.732925122242));
#39669=CARTESIAN_POINT('Ctrl Pts',(133.449669983221,37.1879218466071,26.7271217733964));
#39670=CARTESIAN_POINT('Ctrl Pts',(133.513677039465,37.0870026931285,26.7213167837751));
#39671=CARTESIAN_POINT('Ctrl Pts',(133.573229954184,36.9833070498957,26.7155117941538));
#39672=CARTESIAN_POINT('Ctrl Pts',(133.628096231385,36.8772700220825,26.7097068045326));
#39673=CARTESIAN_POINT('Ctrl Pts',(133.683022200258,36.7711176314681,26.7038954993829));
#39674=CARTESIAN_POINT('Ctrl Pts',(133.733251164245,36.6626191337229,26.6980841942332));
#39675=CARTESIAN_POINT('Ctrl Pts',(133.778597745551,36.5522319663369,26.6922728890835));
#39676=CARTESIAN_POINT('Ctrl Pts',(133.823972420527,36.4417764105393,26.6864579836428));
#39677=CARTESIAN_POINT('Ctrl Pts',(133.864458550049,36.3294302381281,26.6806430782021));
#39678=CARTESIAN_POINT('Ctrl Pts',(133.89992038785,36.2156668821802,26.6748281727614));
#39679=CARTESIAN_POINT('Ctrl Pts',(133.935434699861,36.1017351863354,26.6690046627874));
#39680=CARTESIAN_POINT('Ctrl Pts',(133.965909772143,35.9863825138731,26.6631811528134));
#39681=CARTESIAN_POINT('Ctrl Pts',(133.991260721223,35.8700935899234,26.6573576428394));
#39682=CARTESIAN_POINT('Ctrl Pts',(134.002446051436,35.8187846621822,26.6547881973384));
#39683=CARTESIAN_POINT('Ctrl Pts',(134.012634523012,35.7672935534363,26.6522187518375));
#39684=CARTESIAN_POINT('Ctrl Pts',(134.021822060171,35.7156621523631,26.6496493063365));
#39685=CARTESIAN_POINT('Ctrl Pts',(134.042645419236,35.5986406715131,26.6438257123367));
#39686=CARTESIAN_POINT('Ctrl Pts',(134.058390721623,35.4805208961929,26.638002118337));
#39687=CARTESIAN_POINT('Ctrl Pts',(134.068948190853,35.3617811771706,26.6321785243373));
#39688=CARTESIAN_POINT('Ctrl Pts',(134.079492340275,35.2431912658604,26.6263622776624));
#39689=CARTESIAN_POINT('Ctrl Pts',(134.084861638982,35.1239833696746,26.6205460309876));
#39690=CARTESIAN_POINT('Ctrl Pts',(134.08499735826,35.004645751279,26.6147297843128));
#39691=CARTESIAN_POINT('Ctrl Pts',(134.085132941683,34.885427590427,26.6089193597295));
#39692=CARTESIAN_POINT('Ctrl Pts',(134.080045367236,34.7660803716804,26.6031089351462));
#39693=CARTESIAN_POINT('Ctrl Pts',(134.069727778162,34.6470965972725,26.5972985105629));
#39694=CARTESIAN_POINT('Ctrl Pts',(134.059019647839,34.5236090505677,26.5912681498631));
#39695=CARTESIAN_POINT('Ctrl Pts',(134.042677707309,34.4005134524778,26.5852377891634));
#39696=CARTESIAN_POINT('Ctrl Pts',(134.020753720616,34.2783598416417,26.5792074284636));
#39697=CARTESIAN_POINT('Ctrl Pts',(133.999653110801,34.1607938297783,26.5734035438897));
#39698=CARTESIAN_POINT('Ctrl Pts',(133.973382250782,34.0441007646693,26.5675996593159));
#39699=CARTESIAN_POINT('Ctrl Pts',(133.94203994183,33.9287642196906,26.561795774742));
#39700=CARTESIAN_POINT('Ctrl Pts',(133.910702262464,33.8134447111223,26.5559927474624));
#39701=CARTESIAN_POINT('Ctrl Pts',(133.874294730951,33.6994817181475,26.5501897201829));
#39702=CARTESIAN_POINT('Ctrl Pts',(133.832966639211,33.5873458517037,26.5443866929033));
#39703=CARTESIAN_POINT('Ctrl Pts',(133.791634898624,33.4752000848145,26.538583153276));
#39704=CARTESIAN_POINT('Ctrl Pts',(133.745381875263,33.3648821483549,26.5327796136487));
#39705=CARTESIAN_POINT('Ctrl Pts',(133.694405610753,33.2568441884794,26.5269760740214));
#39706=CARTESIAN_POINT('Ctrl Pts',(133.643412815229,33.1487711931414,26.5211706523733));
#39707=CARTESIAN_POINT('Ctrl Pts',(133.587693906521,33.0429800139307,26.5153652307251));
#39708=CARTESIAN_POINT('Ctrl Pts',(133.527493321346,32.9398990636727,26.509559809077));
#39709=CARTESIAN_POINT('Ctrl Pts',(133.467226069606,32.8367039608211,26.5037479584627));
#39710=CARTESIAN_POINT('Ctrl Pts',(133.402467440795,32.7362254306461,26.4979361078484));
#39711=CARTESIAN_POINT('Ctrl Pts',(133.333505813242,32.6388638342777,26.4921242572341));
#39712=CARTESIAN_POINT('Ctrl Pts',(133.264498891324,32.5414382902933,26.4863085893653));
#39713=CARTESIAN_POINT('Ctrl Pts',(133.191283722793,32.447134079003,26.4804929214966));
#39714=CARTESIAN_POINT('Ctrl Pts',(133.114188607991,32.3563180384441,26.4746772536278));
#39715=CARTESIAN_POINT('Ctrl Pts',(133.036983062804,32.2653719137611,26.4688532554458));
#39716=CARTESIAN_POINT('Ctrl Pts',(132.955886755349,32.1779242307475,26.4630292572638));
#39717=CARTESIAN_POINT('Ctrl Pts',(132.871264482113,32.0943046832542,26.4572052590819));
#39718=CARTESIAN_POINT('Ctrl Pts',(132.848813780563,32.0721200097315,26.4556601239772));
#39719=CARTESIAN_POINT('Ctrl Pts',(132.82611507466,32.0502045629611,26.4541149888726));
#39720=CARTESIAN_POINT('Ctrl Pts',(132.803175546272,32.0285640076244,26.452569853768));
#39721=CARTESIAN_POINT('Ctrl Pts',(132.716716768458,31.9470010419913,26.4467462600813));
#39722=CARTESIAN_POINT('Ctrl Pts',(132.626555803418,31.8690831708606,26.4409226663946));
#39723=CARTESIAN_POINT('Ctrl Pts',(132.5330325544,31.7951644225721,26.4350990727078));
#39724=CARTESIAN_POINT('Ctrl Pts',(132.439627298836,31.7213389337506,26.4292828263485));
#39725=CARTESIAN_POINT('Ctrl Pts',(132.342868514105,31.6515027833869,26.4234665799891));
#39726=CARTESIAN_POINT('Ctrl Pts',(132.24313237601,31.5859727382908,26.4176503336298));
#39727=CARTESIAN_POINT('Ctrl Pts',(132.143496074322,31.5205082891196,26.4118399093641));
#39728=CARTESIAN_POINT('Ctrl Pts',(132.040888687605,31.4593415930756,26.4060294850984));
#39729=CARTESIAN_POINT('Ctrl Pts',(131.935718371835,31.4027483567394,26.4002190608327));
#39730=CARTESIAN_POINT('Ctrl Pts',(131.82656714252,31.344012949588,26.3941887000147));
#39731=CARTESIAN_POINT('Ctrl Pts',(131.714655477875,31.2902043508118,26.3881583391966));
#39732=CARTESIAN_POINT('Ctrl Pts',(131.60047178956,31.2415807776645,26.3821279783786));
#39733=CARTESIAN_POINT('Ctrl Pts',(131.49057639017,31.194783314124,26.3763240941255));
#39734=CARTESIAN_POINT('Ctrl Pts',(131.378576955507,31.1527886157344,26.3705202098724));
#39735=CARTESIAN_POINT('Ctrl Pts',(131.264932091598,31.1157791252756,26.3647163256193));
#39736=CARTESIAN_POINT('Ctrl Pts',(131.151304014234,31.0787751015087,26.3589132986611));
#39737=CARTESIAN_POINT('Ctrl Pts',(131.036031379132,31.0467549476782,26.3531102717029));
#39738=CARTESIAN_POINT('Ctrl Pts',(130.919589628044,31.0198517721077,26.3473072447447));
#39739=CARTESIAN_POINT('Ctrl Pts',(130.803137596349,30.9929462212639,26.341503705439));
#39740=CARTESIAN_POINT('Ctrl Pts',(130.685516641316,30.9711586388476,26.3357001661333));
#39741=CARTESIAN_POINT('Ctrl Pts',(130.567213484101,30.9545712386134,26.3298966268277));
#39742=CARTESIAN_POINT('Ctrl Pts',(130.448871962534,30.9379784592763,26.324091205501));
#39743=CARTESIAN_POINT('Ctrl Pts',(130.329848202982,30.9265892725787,26.3182857841744));
#39744=CARTESIAN_POINT('Ctrl Pts',(130.210634508829,30.9204340790116,26.3124803628477));
#39745=CARTESIAN_POINT('Ctrl Pts',(130.091288796521,30.9142720691361,26.3066685125532));
#39746=CARTESIAN_POINT('Ctrl Pts',(129.971753137802,30.9133556430981,26.3008566622587));
#39747=CARTESIAN_POINT('Ctrl Pts',(129.852520461619,30.9176630729741,26.2950448119641));
#39748=CARTESIAN_POINT('Ctrl Pts',(129.733209472761,30.9219733319937,26.2892291444144));
#39749=CARTESIAN_POINT('Ctrl Pts',(129.61420226885,30.9315142474071,26.2834134768647));
#39750=CARTESIAN_POINT('Ctrl Pts',(129.49598562488,30.9462123255316,26.277597809315));
#39751=CARTESIAN_POINT('Ctrl Pts',(129.377599648315,30.960931457068,26.2717738114487));
#39752=CARTESIAN_POINT('Ctrl Pts',(129.260006893072,30.9808224276629,26.2659498135824));
#39753=CARTESIAN_POINT('Ctrl Pts',(129.143683073674,31.005760858225,26.2601258157161));
#39754=CARTESIAN_POINT('Ctrl Pts',(129.112821734468,31.0123771589003,26.2585806775439));
#39755=CARTESIAN_POINT('Ctrl Pts',(129.082049622144,31.0193484649703,26.2570355393718));
#39756=CARTESIAN_POINT('Ctrl Pts',(129.051375411368,31.0266718748834,26.2554904011996));
#39757=CARTESIAN_POINT('Ctrl Pts',(128.935764949877,31.0542736543036,26.2496668076129));
#39758=CARTESIAN_POINT('Ctrl Pts',(128.82117373592,31.086969944146,26.2438432140263));
#39759=CARTESIAN_POINT('Ctrl Pts',(128.708084191153,31.1246705246067,26.2380196204396));
#39760=CARTESIAN_POINT('Ctrl Pts',(128.595137325676,31.1623235401752,26.2322033741828));
#39761=CARTESIAN_POINT('Ctrl Pts',(128.483688745079,31.2049681606443,26.226387127926));
#39762=CARTESIAN_POINT('Ctrl Pts',(128.374209589848,31.2524634034799,26.2205708816692));
#39763=CARTESIAN_POINT('Ctrl Pts',(128.26484002388,31.2999111033045,26.2147604575083));
#39764=CARTESIAN_POINT('Ctrl Pts',(128.157436333859,31.352199604498,26.2089500333474));
#39765=CARTESIAN_POINT('Ctrl Pts',(128.052452849047,31.4091386695092,26.2031396091865));
#39766=CARTESIAN_POINT('Ctrl Pts',(127.943495519968,31.4682329971073,26.1971092483301));
#39767=CARTESIAN_POINT('Ctrl Pts',(127.837145661094,31.5323367701793,26.1910788874736));
#39768=CARTESIAN_POINT('Ctrl Pts',(127.733886967399,31.6011830406042,26.1850485266171));
#39769=CARTESIAN_POINT('Ctrl Pts',(127.634506265441,31.6674437150053,26.179244642474));
#39770=CARTESIAN_POINT('Ctrl Pts',(127.537989102006,31.738096844609,26.1734407583309));
#39771=CARTESIAN_POINT('Ctrl Pts',(127.444739458086,31.8128588730749,26.1676368741878));
#39772=CARTESIAN_POINT('Ctrl Pts',(127.351503588149,31.8876098583789,26.1618338473412));
#39773=CARTESIAN_POINT('Ctrl Pts',(127.261534596394,31.9664682802003,26.1560308204947));
#39774=CARTESIAN_POINT('Ctrl Pts',(127.175204430632,32.04910945793,26.1502277936482));
#39775=CARTESIAN_POINT('Ctrl Pts',(127.088866642829,32.1317579320015,26.1444242544558));
#39776=CARTESIAN_POINT('Ctrl Pts',(127.006168614767,32.2181895436282,26.1386207152633));
#39777=CARTESIAN_POINT('Ctrl Pts',(126.927445910466,32.3080422798845,26.1328171760709));
#39778=CARTESIAN_POINT('Ctrl Pts',(126.848697677319,32.397924154326,26.127011754859));
#39779=CARTESIAN_POINT('Ctrl Pts',(126.773927600712,32.4912290528291,26.1212063336472));
#39780=CARTESIAN_POINT('Ctrl Pts',(126.703430969524,32.5875618915072,26.1154009124353));
#39781=CARTESIAN_POINT('Ctrl Pts',(126.632856269847,32.6840014098815,26.1095890622571));
#39782=CARTESIAN_POINT('Ctrl Pts',(126.566564703245,32.7834752319111,26.1037772120789));
#39783=CARTESIAN_POINT('Ctrl Pts',(126.504808302805,32.8855591756076,26.0979653619008));
#39784=CARTESIAN_POINT('Ctrl Pts',(126.443011340433,32.9877101685807,26.0921496944685));
#39785=CARTESIAN_POINT('Ctrl Pts',(126.385755671798,33.0924743398825,26.0863340270363));
#39786=CARTESIAN_POINT('Ctrl Pts',(126.333246661229,33.19940427841,26.080518359604));
#39787=CARTESIAN_POINT('Ctrl Pts',(126.280662437169,33.306487382533,26.0746943618559));
#39788=CARTESIAN_POINT('Ctrl Pts',(126.232838604917,33.415742073018,26.0688703641078));
#39789=CARTESIAN_POINT('Ctrl Pts',(126.189931906767,33.5267022958927,26.0630463663596));
#39790=CARTESIAN_POINT('Ctrl Pts',(126.17854851928,33.5561406648911,26.0615012271168));
#39791=CARTESIAN_POINT('Ctrl Pts',(126.167510959468,33.5856990082987,26.059956087874));
#39792=CARTESIAN_POINT('Ctrl Pts',(126.156821555699,33.6153684803317,26.0584109486312));
#39793=CARTESIAN_POINT('Ctrl Pts',(126.110323273242,33.7444289518687,26.0516896831146));
#39794=CARTESIAN_POINT('Ctrl Pts',(126.070293444538,33.8759349209088,26.0449684175981));
#39795=CARTESIAN_POINT('Ctrl Pts',(126.036959458656,34.0092756853371,26.0382471520816));
#39796=CARTESIAN_POINT('Ctrl Pts',(126.003758284162,34.1420851850052,26.0315526658589));
#39797=CARTESIAN_POINT('Ctrl Pts',(125.977199802163,34.2767147548031,26.0248581796363));
#39798=CARTESIAN_POINT('Ctrl Pts',(125.957461778025,34.4125395980401,26.0181636934136));
#39799=CARTESIAN_POINT('Ctrl Pts',(125.937867450412,34.5473756108934,26.0115179443087));
#39800=CARTESIAN_POINT('Ctrl Pts',(125.924994719636,34.6833894081815,26.0048721952038));
#39801=CARTESIAN_POINT('Ctrl Pts',(125.918969827263,34.8199507589276,25.9982264460989));
#39802=CARTESIAN_POINT('Ctrl Pts',(125.916367519002,34.8789351704621,25.9953559736115));
#39803=CARTESIAN_POINT('Ctrl Pts',(125.915042131088,34.9380215056026,25.9924855011241));
#39804=CARTESIAN_POINT('Ctrl Pts',(125.915000988625,34.9971579821973,25.9896150286367));
#39805=CARTESIAN_POINT('Origin',(130.,35.,32.7603849714045));
#39806=CARTESIAN_POINT('',(132.487160689988,38.2405642567579,28.0469635225512));
#39807=CARTESIAN_POINT('',(132.487160689988,38.2405642567579,27.9426397356904));
#39808=CARTESIAN_POINT('',(132.487160689988,38.2405642567579,32.7603849714045));
#39809=CARTESIAN_POINT('',(125.915000279441,35.001510971197,27.1353849713731));
#39810=CARTESIAN_POINT('Ctrl Pts',(132.487160689988,38.2405642567579,27.9426397356904));
#39811=CARTESIAN_POINT('Ctrl Pts',(132.581967895796,38.1677989181535,27.9368366805219));
#39812=CARTESIAN_POINT('Ctrl Pts',(132.67358627189,38.0908641165998,27.9310336253533));
#39813=CARTESIAN_POINT('Ctrl Pts',(132.761639023741,38.010078886433,27.9252305701847));
#39814=CARTESIAN_POINT('Ctrl Pts',(132.849706660417,37.9292799999757,27.9194265340421));
#39815=CARTESIAN_POINT('Ctrl Pts',(132.934207173398,37.8446296666309,27.9136224978996));
#39816=CARTESIAN_POINT('Ctrl Pts',(133.014799649079,37.7564847316669,27.907818461757));
#39817=CARTESIAN_POINT('Ctrl Pts',(133.095475204053,37.6682489319074,27.902008442485));
#39818=CARTESIAN_POINT('Ctrl Pts',(133.172234398533,37.5765116365957,27.896198423213));
#39819=CARTESIAN_POINT('Ctrl Pts',(133.244775590758,37.4816640315769,27.8903884039409));
#39820=CARTESIAN_POINT('Ctrl Pts',(133.317354327839,37.38676733666,27.8845753776003));
#39821=CARTESIAN_POINT('Ctrl Pts',(133.385710479367,37.288757459556,27.8787623512597));
#39822=CARTESIAN_POINT('Ctrl Pts',(133.4495858686,37.1880544634797,27.8729493249191));
#39823=CARTESIAN_POINT('Ctrl Pts',(133.51356454696,37.087188626525,27.8671268986763));
#39824=CARTESIAN_POINT('Ctrl Pts',(133.573047781196,36.9836213230422,27.8613044724335));
#39825=CARTESIAN_POINT('Ctrl Pts',(133.627823186965,36.877797625975,27.8554820461907));
#39826=CARTESIAN_POINT('Ctrl Pts',(133.678349078126,36.7801838059562,27.8501113278819));
#39827=CARTESIAN_POINT('Ctrl Pts',(133.724869709531,36.6806505966967,27.8447406095731));
#39828=CARTESIAN_POINT('Ctrl Pts',(133.767255489852,36.5795604053595,27.8393698912644));
#39829=CARTESIAN_POINT('Ctrl Pts',(133.813215309703,36.4699461208672,27.8335463050505));
#39830=CARTESIAN_POINT('Ctrl Pts',(133.854461171629,36.3581474944634,27.8277227188367));
#39831=CARTESIAN_POINT('Ctrl Pts',(133.890781146696,36.2446071944646,27.8218991326229));
#39832=CARTESIAN_POINT('Ctrl Pts',(133.927055297973,36.1312101447551,27.8160828938479));
#39833=CARTESIAN_POINT('Ctrl Pts',(133.958415800245,36.0160761775544,27.8102666550729));
#39834=CARTESIAN_POINT('Ctrl Pts',(133.984698359649,35.8996688182933,27.8044504162979));
#39835=CARTESIAN_POINT('Ctrl Pts',(134.010954609579,35.7833779856037,27.7986399997181));
#39836=CARTESIAN_POINT('Ctrl Pts',(134.03214293951,35.6658166927262,27.7928295831383));
#39837=CARTESIAN_POINT('Ctrl Pts',(134.048148737804,35.5474639683296,27.7870191665584));
#39838=CARTESIAN_POINT('Ctrl Pts',(134.064760418407,35.4246311286238,27.7809888028975));
#39839=CARTESIAN_POINT('Ctrl Pts',(134.075789319717,35.3009461827978,27.7749584392366));
#39840=CARTESIAN_POINT('Ctrl Pts',(134.081165417923,35.1769571460836,27.7689280755756));
#39841=CARTESIAN_POINT('Ctrl Pts',(134.086339601614,35.0576248669875,27.7631241992128));
#39842=CARTESIAN_POINT('Ctrl Pts',(134.086277919083,34.9380113716758,27.7573203228499));
#39843=CARTESIAN_POINT('Ctrl Pts',(134.080970805455,34.818610129774,27.7515164464871));
#39844=CARTESIAN_POINT('Ctrl Pts',(134.075664475803,34.699226525991,27.745713427481));
#39845=CARTESIAN_POINT('Ctrl Pts',(134.065114274137,34.5800555210893,27.7399104084748));
#39846=CARTESIAN_POINT('Ctrl Pts',(134.049362739548,34.4615890012616,27.7341073894687));
#39847=CARTESIAN_POINT('Ctrl Pts',(134.033609814403,34.343112023136,27.7283038581685));
#39848=CARTESIAN_POINT('Ctrl Pts',(134.012654697202,34.2253400585338,27.7225003268683));
#39849=CARTESIAN_POINT('Ctrl Pts',(133.986591538088,34.108757660092,27.7166967955681));
#39850=CARTESIAN_POINT('Ctrl Pts',(133.960519927182,33.9921374561701,27.7108913822917));
#39851=CARTESIAN_POINT('Ctrl Pts',(133.929337069116,33.8767079838822,27.7050859690154));
#39852=CARTESIAN_POINT('Ctrl Pts',(133.89318758219,33.7629408058307,27.6992805557391));
#39853=CARTESIAN_POINT('Ctrl Pts',(133.856998063155,33.6490476414779,27.6934687135212));
#39854=CARTESIAN_POINT('Ctrl Pts',(133.815831060382,33.5368208352156,27.6876568713032));
#39855=CARTESIAN_POINT('Ctrl Pts',(133.769880212744,33.4267142085565,27.6818450290853));
#39856=CARTESIAN_POINT('Ctrl Pts',(133.723899184492,33.3165352636299,27.6760293696369));
#39857=CARTESIAN_POINT('Ctrl Pts',(133.673128227175,33.2084796403079,27.6702137101886));
#39858=CARTESIAN_POINT('Ctrl Pts',(133.617807277261,33.1029771997682,27.6643980507403));
#39859=CARTESIAN_POINT('Ctrl Pts',(133.562407085701,32.9973236376917,27.6585740609501));
#39860=CARTESIAN_POINT('Ctrl Pts',(133.50244409774,32.8942309096409,27.65275007116));
#39861=CARTESIAN_POINT('Ctrl Pts',(133.438201998309,32.7941006326619,27.6469260813698));
#39862=CARTESIAN_POINT('Ctrl Pts',(133.421157358906,32.7675341835642,27.6453808671452));
#39863=CARTESIAN_POINT('Ctrl Pts',(133.403811716603,32.7411760946367,27.6438356529206));
#39864=CARTESIAN_POINT('Ctrl Pts',(133.386170838338,32.7150334677315,27.6422904386959));
#39865=CARTESIAN_POINT('Ctrl Pts',(133.319685978813,32.616507257681,27.6364668425507));
#39866=CARTESIAN_POINT('Ctrl Pts',(133.248790165876,32.5207263059491,27.6306432464055));
#39867=CARTESIAN_POINT('Ctrl Pts',(133.173737465054,32.4281105189154,27.6248196502604));
#39868=CARTESIAN_POINT('Ctrl Pts',(133.098779454018,32.3356115800302,27.6190034014201));
#39869=CARTESIAN_POINT('Ctrl Pts',(133.019675241128,32.2462701776917,27.6131871525798));
#39870=CARTESIAN_POINT('Ctrl Pts',(132.936722447901,32.1604778106176,27.6073709037396));
#39871=CARTESIAN_POINT('Ctrl Pts',(132.853852690552,32.07477132184,27.6015604769737));
#39872=CARTESIAN_POINT('Ctrl Pts',(132.767142299016,31.9926070927561,27.5957500502078));
#39873=CARTESIAN_POINT('Ctrl Pts',(132.676929095141,31.9143435674743,27.5899396234419));
#39874=CARTESIAN_POINT('Ctrl Pts',(132.583301190007,31.8331176536858,27.5839092635538));
#39875=CARTESIAN_POINT('Ctrl Pts',(132.485900342307,31.756093921046,27.5778789036657));
#39876=CARTESIAN_POINT('Ctrl Pts',(132.385146510728,31.6836313349749,27.5718485437776));
#39877=CARTESIAN_POINT('Ctrl Pts',(132.288176538371,31.6138901166196,27.5660446569924));
#39878=CARTESIAN_POINT('Ctrl Pts',(132.188101247688,31.5483738906348,27.5602407702073));
#39879=CARTESIAN_POINT('Ctrl Pts',(132.085328121047,31.4873611589618,27.5544368834221));
#39880=CARTESIAN_POINT('Ctrl Pts',(131.982570174944,31.4263574394312,27.5486338539245));
#39881=CARTESIAN_POINT('Ctrl Pts',(131.877115536391,31.3698560997177,27.5428308244269));
#39882=CARTESIAN_POINT('Ctrl Pts',(131.769398924827,31.3180911954772,27.5370277949292));
#39883=CARTESIAN_POINT('Ctrl Pts',(131.661672802915,31.2663217208905,27.5312242530796));
#39884=CARTESIAN_POINT('Ctrl Pts',(131.55168467898,31.2192896901016,27.5254207112299));
#39885=CARTESIAN_POINT('Ctrl Pts',(131.439891430112,31.1771819727471,27.5196171693803));
#39886=CARTESIAN_POINT('Ctrl Pts',(131.328061927962,31.1350606003377,27.5138117455078));
#39887=CARTESIAN_POINT('Ctrl Pts',(131.21442651862,31.0978668610919,27.5080063216354));
#39888=CARTESIAN_POINT('Ctrl Pts',(131.099458879435,31.0657382938559,27.502200897763));
#39889=CARTESIAN_POINT('Ctrl Pts',(130.984363924466,31.0335741472714,27.4963890449329));
#39890=CARTESIAN_POINT('Ctrl Pts',(130.867934188295,31.0064864791049,27.4905771921028));
#39891=CARTESIAN_POINT('Ctrl Pts',(130.750655381388,30.9845621037809,27.4847653392727));
#39892=CARTESIAN_POINT('Ctrl Pts',(130.633299545212,30.9626233284244,27.4789496691905));
#39893=CARTESIAN_POINT('Ctrl Pts',(130.515093931039,30.9458546569408,27.4731339991082));
#39894=CARTESIAN_POINT('Ctrl Pts',(130.396529588248,30.9342910475977,27.467318329026));
#39895=CARTESIAN_POINT('Ctrl Pts',(130.277795415379,30.9227108746858,27.4614943286509));
#39896=CARTESIAN_POINT('Ctrl Pts',(130.158701894607,30.9163506667168,27.4556703282757));
#39897=CARTESIAN_POINT('Ctrl Pts',(130.039740434039,30.9151933096042,27.4498463279006));
#39898=CARTESIAN_POINT('Ctrl Pts',(130.008179823231,30.9148862614457,27.4483012139762));
#39899=CARTESIAN_POINT('Ctrl Pts',(129.976628479121,30.9149451312888,27.4467561000519));
#39900=CARTESIAN_POINT('Ctrl Pts',(129.945095500927,30.9153689890051,27.4452109861275));
#39901=CARTESIAN_POINT('Ctrl Pts',(129.826246487297,30.9169665251206,27.4393873920247));
#39902=CARTESIAN_POINT('Ctrl Pts',(129.707275603486,30.9237581021851,27.4335637979218));
#39903=CARTESIAN_POINT('Ctrl Pts',(129.588673316226,30.9357614047382,27.427740203819));
#39904=CARTESIAN_POINT('Ctrl Pts',(129.470220663086,30.9477495633707,27.4219239570313));
#39905=CARTESIAN_POINT('Ctrl Pts',(129.352136084225,30.9649363285143,27.4161077102436));
#39906=CARTESIAN_POINT('Ctrl Pts',(129.234910162862,30.9872873836881,27.4102914634559));
#39907=CARTESIAN_POINT('Ctrl Pts',(129.117801585028,31.0096160653829,27.4044810387502));
#39908=CARTESIAN_POINT('Ctrl Pts',(129.001550353591,31.0370986770465,27.3986706140445));
#39909=CARTESIAN_POINT('Ctrl Pts',(128.88664144223,31.0696491604642,27.3928601893387));
#39910=CARTESIAN_POINT('Ctrl Pts',(128.767383003585,31.1034317434123,27.3868298286812));
#39911=CARTESIAN_POINT('Ctrl Pts',(128.649570957668,31.1426733911688,27.3807994680238));
#39912=CARTESIAN_POINT('Ctrl Pts',(128.533735739348,31.1872196341864,27.3747691073663));
#39913=CARTESIAN_POINT('Ctrl Pts',(128.422250822974,31.230092900621,27.3689652226467));
#39914=CARTESIAN_POINT('Ctrl Pts',(128.312597344001,31.2778793496121,27.3631613379271));
#39915=CARTESIAN_POINT('Ctrl Pts',(128.205231600169,31.3303908394807,27.3573574532075));
#39916=CARTESIAN_POINT('Ctrl Pts',(128.097881715221,31.3828945729307,27.3515544257738));
#39917=CARTESIAN_POINT('Ctrl Pts',(127.992819260116,31.4401217799373,27.3457513983401));
#39918=CARTESIAN_POINT('Ctrl Pts',(127.890478289381,31.5018371746835,27.3399483709064));
#39919=CARTESIAN_POINT('Ctrl Pts',(127.788128282844,31.5635580183531,27.3341448311167));
#39920=CARTESIAN_POINT('Ctrl Pts',(127.688500588112,31.629767626759,27.3283412913271));
#39921=CARTESIAN_POINT('Ctrl Pts',(127.592001940709,31.7001863164031,27.3225377515374));
#39922=CARTESIAN_POINT('Ctrl Pts',(127.495471999776,31.7706278421129,27.3167323297187));
#39923=CARTESIAN_POINT('Ctrl Pts',(127.402073453898,31.845280923083,27.3109269079));
#39924=CARTESIAN_POINT('Ctrl Pts',(127.31218098904,31.9238247832211,27.3051214860814));
#39925=CARTESIAN_POINT('Ctrl Pts',(127.222188976442,32.002455623551,27.2993096352853));
#39926=CARTESIAN_POINT('Ctrl Pts',(127.135711102675,32.0849855747184,27.2934977844892));
#39927=CARTESIAN_POINT('Ctrl Pts',(127.053086225376,32.1710559911988,27.2876859336931));
#39928=CARTESIAN_POINT('Ctrl Pts',(126.970407079522,32.2571829392871,27.2818702656357));
#39929=CARTESIAN_POINT('Ctrl Pts',(126.891586239002,32.3468546777902,27.2760545975783));
#39930=CARTESIAN_POINT('Ctrl Pts',(126.816922117047,32.4396796702254,27.2702389295209));
#39931=CARTESIAN_POINT('Ctrl Pts',(126.742151046733,32.5326376245228,27.2644149311418));
#39932=CARTESIAN_POINT('Ctrl Pts',(126.671548819826,32.6287575199072,27.2585909327626));
#39933=CARTESIAN_POINT('Ctrl Pts',(126.605370494381,32.727618975704,27.2527669343835));
#39934=CARTESIAN_POINT('Ctrl Pts',(126.587813079677,32.7538473755006,27.2512218007753));
#39935=CARTESIAN_POINT('Ctrl Pts',(126.570566795796,32.7802686127526,27.2496766671671));
#39936=CARTESIAN_POINT('Ctrl Pts',(126.553635852822,32.8068745669608,27.248131533559));
#39937=CARTESIAN_POINT('Ctrl Pts',(126.488371803229,32.9094330787663,27.2421754756724));
#39938=CARTESIAN_POINT('Ctrl Pts',(126.427594206498,33.015056667611,27.2362194177857));
#39939=CARTESIAN_POINT('Ctrl Pts',(126.371595291591,33.1233262744958,27.2302633598991));
#39940=CARTESIAN_POINT('Ctrl Pts',(126.315676623204,33.2314407308912,27.2243158370513));
#39941=CARTESIAN_POINT('Ctrl Pts',(126.264523181674,33.3421933208752,27.2183683142034));
#39942=CARTESIAN_POINT('Ctrl Pts',(126.218383658613,33.4551366252794,27.2124207913556));
#39943=CARTESIAN_POINT('Ctrl Pts',(126.172301362892,33.5679398449035,27.2064806452835));
#39944=CARTESIAN_POINT('Ctrl Pts',(126.131220750027,33.6829280171375,27.2005404992115));
#39945=CARTESIAN_POINT('Ctrl Pts',(126.095344190094,33.7996300544536,27.1946003531394));
#39946=CARTESIAN_POINT('Ctrl Pts',(126.059514012288,33.9161812164208,27.1886678866386));
#39947=CARTESIAN_POINT('Ctrl Pts',(126.02887459329,34.0344414634443,27.1827354201378));
#39948=CARTESIAN_POINT('Ctrl Pts',(126.003579608595,34.153921365851,27.176802953637));
#39949=CARTESIAN_POINT('Ctrl Pts',(125.978303893947,34.2733102469177,27.1708750065662));
#39950=CARTESIAN_POINT('Ctrl Pts',(125.958364588403,34.3939165600159,27.1649470594953));
#39951=CARTESIAN_POINT('Ctrl Pts',(125.9438651346,34.5152372191622,27.1590191124245));
#39952=CARTESIAN_POINT('Ctrl Pts',(125.929375293507,34.6364774462863,27.1530950954079));
#39953=CARTESIAN_POINT('Ctrl Pts',(125.92031816485,34.7584306959922,27.1471710783913));
#39954=CARTESIAN_POINT('Ctrl Pts',(125.916745755823,34.8805856900996,27.1412470613746));
#39955=CARTESIAN_POINT('Ctrl Pts',(125.91556740094,34.920878370092,27.1392930313846));
#39956=CARTESIAN_POINT('Ctrl Pts',(125.914985366504,34.9611929501148,27.1373390013945));
#39957=CARTESIAN_POINT('Ctrl Pts',(125.915000279441,35.0015109705496,27.1353849714045));
#39958=CARTESIAN_POINT('Ctrl Pts',(125.915000279441,35.001510971197,27.1353849713731));
#39959=CARTESIAN_POINT('Ctrl Pts',(125.915048271955,35.1312615634159,27.1290965537948));
#39960=CARTESIAN_POINT('Ctrl Pts',(125.921282283117,35.2608260686367,27.1228081362166));
#39961=CARTESIAN_POINT('Ctrl Pts',(125.93362428894,35.3896326173498,27.1165197186383));
#39962=CARTESIAN_POINT('Ctrl Pts',(125.946018781118,35.5189869365177,27.1102045585582));
#39963=CARTESIAN_POINT('Ctrl Pts',(125.964573240673,35.6475765570869,27.1038893984782));
#39964=CARTESIAN_POINT('Ctrl Pts',(125.989158035468,35.7748365863507,27.0975742383981));
#39965=CARTESIAN_POINT('Ctrl Pts',(126.01379677885,35.9023758735403,27.0912452204043));
#39966=CARTESIAN_POINT('Ctrl Pts',(126.044492226899,36.0285794609645,27.0849162024105));
#39967=CARTESIAN_POINT('Ctrl Pts',(126.081064803515,36.1528971878489,27.0785871844168));
#39968=CARTESIAN_POINT('Ctrl Pts',(126.117752827032,36.2776073425498,27.0722381879149));
#39969=CARTESIAN_POINT('Ctrl Pts',(126.160355004852,36.4004194525701,27.065889191413));
#39970=CARTESIAN_POINT('Ctrl Pts',(126.208642673224,36.5208006512037,27.0595401949112));
#39971=CARTESIAN_POINT('Ctrl Pts',(126.230161624026,36.5744474139953,27.0567108236043));
#39972=CARTESIAN_POINT('Ctrl Pts',(126.252809073841,36.6276117300588,27.0538814522974));
#39973=CARTESIAN_POINT('Ctrl Pts',(126.276561884097,36.6802480760414,27.0510520809906));
#39974=CARTESIAN_POINT('Ctrl Pts',(126.325451445855,36.788587588709,27.0452284869925));
#39975=CARTESIAN_POINT('Ctrl Pts',(126.379152242878,36.8949662532005,27.0394048929945));
#39976=CARTESIAN_POINT('Ctrl Pts',(126.437484778236,36.9989272859964,27.0335812989965));
#39977=CARTESIAN_POINT('Ctrl Pts',(126.495743718476,37.102757156578,27.0277650523234));
#39978=CARTESIAN_POINT('Ctrl Pts',(126.558622576169,37.2041751092696,27.0219488056503));
#39979=CARTESIAN_POINT('Ctrl Pts',(126.625894126271,37.3027450038749,27.0161325589771));
#39980=CARTESIAN_POINT('Ctrl Pts',(126.693098337221,37.4012162295303,27.0103221343956));
#39981=CARTESIAN_POINT('Ctrl Pts',(126.76468626422,37.4968447333148,27.004511709814));
#39982=CARTESIAN_POINT('Ctrl Pts',(126.840385476734,37.589220165294,26.9987012852324));
#39983=CARTESIAN_POINT('Ctrl Pts',(126.918950054896,37.6850921909736,26.992670924532));
#39984=CARTESIAN_POINT('Ctrl Pts',(127.001943089512,37.7774596175838,26.9866405638316));
#39985=CARTESIAN_POINT('Ctrl Pts',(127.08901128064,37.8658977085305,26.9806102031311));
#39986=CARTESIAN_POINT('Ctrl Pts',(127.1728095402,37.9510144199724,26.9748063185591));
#39987=CARTESIAN_POINT('Ctrl Pts',(127.260382070995,38.0324912962786,26.969002433987));
#39988=CARTESIAN_POINT('Ctrl Pts',(127.351374281094,38.1099850162262,26.9631985494149));
#39989=CARTESIAN_POINT('Ctrl Pts',(127.442353050695,38.1874672895432,26.9573955221371));
#39990=CARTESIAN_POINT('Ctrl Pts',(127.53675018428,38.2609673118662,26.9515924948594));
#39991=CARTESIAN_POINT('Ctrl Pts',(127.634176737521,38.3301809696641,26.9457894675816));
#39992=CARTESIAN_POINT('Ctrl Pts',(127.731611892525,38.3994007383172,26.9399859279561));
#39993=CARTESIAN_POINT('Ctrl Pts',(127.832076666072,38.4643331535117,26.9341823883306));
#39994=CARTESIAN_POINT('Ctrl Pts',(127.93515230517,38.5247168676583,26.9283788487051));
#39995=CARTESIAN_POINT('Ctrl Pts',(128.038261370507,38.5851201635458,26.9225734270587));
#39996=CARTESIAN_POINT('Ctrl Pts',(128.143982633088,38.6409716184659,26.9167680054124));
#39997=CARTESIAN_POINT('Ctrl Pts',(128.251872449466,38.6920556695512,26.910962583766));
#39998=CARTESIAN_POINT('Ctrl Pts',(128.359881743812,38.743196291486,26.9051507331535));
#39999=CARTESIAN_POINT('Ctrl Pts',(128.470064016221,38.7895587964898,26.899338882541));
#40000=CARTESIAN_POINT('Ctrl Pts',(128.581955196081,38.8309755851582,26.8935270319286));
#40001=CARTESIAN_POINT('Ctrl Pts',(128.693919866665,38.8724195765945,26.8877113640616));
#40002=CARTESIAN_POINT('Ctrl Pts',(128.807595292124,38.9089112579561,26.8818956961946));
#40003=CARTESIAN_POINT('Ctrl Pts',(128.922503381589,38.9403332393737,26.8760800283276));
#40004=CARTESIAN_POINT('Ctrl Pts',(129.037576064424,38.9718002293703,26.8702560301474));
#40005=CARTESIAN_POINT('Ctrl Pts',(129.153884538615,38.9981829352654,26.8644320319673));
#40006=CARTESIAN_POINT('Ctrl Pts',(129.270941565159,39.0194152309243,26.8586080337871));
#40007=CARTESIAN_POINT('Ctrl Pts',(129.301997365204,39.0250482625156,26.8570628986654));
#40008=CARTESIAN_POINT('Ctrl Pts',(129.333105833467,39.0303190576262,26.8555177635438));
#40009=CARTESIAN_POINT('Ctrl Pts',(129.364257843975,39.0352269962237,26.8539726284221));
#40010=CARTESIAN_POINT('Ctrl Pts',(129.481684253281,39.053727298362,26.8481482958581));
#40011=CARTESIAN_POINT('Ctrl Pts',(129.600108263132,39.0671274622222,26.8423239632942));
#40012=CARTESIAN_POINT('Ctrl Pts',(129.719049255623,39.0753271867709,26.8364996307302));
#40013=CARTESIAN_POINT('Ctrl Pts',(129.841350910667,39.0837585934895,26.8305107323934));
#40014=CARTESIAN_POINT('Ctrl Pts',(129.964198791598,39.0866911624357,26.8245218340567));
#40015=CARTESIAN_POINT('Ctrl Pts',(130.087058568312,39.0840722086765,26.8185329357199));
#40016=CARTESIAN_POINT('Ctrl Pts',(130.206242812632,39.0815316048023,26.812723204157));
#40017=CARTESIAN_POINT('Ctrl Pts',(130.325437804712,39.0737668911315,26.8069134725942));
#40018=CARTESIAN_POINT('Ctrl Pts',(130.444151133482,39.0607825318068,26.8011037410314));
#40019=CARTESIAN_POINT('Ctrl Pts',(130.562785665313,39.0478067909563,26.7952978657252));
#40020=CARTESIAN_POINT('Ctrl Pts',(130.680938765249,39.029618339027,26.7894919904189));
#40021=CARTESIAN_POINT('Ctrl Pts',(130.798120612488,39.0062736411684,26.7836861151127));
#40022=CARTESIAN_POINT('Ctrl Pts',(130.915252335739,38.9829389288958,26.7778827232427));
#40023=CARTESIAN_POINT('Ctrl Pts',(131.031413233102,38.9544524383411,26.7720793313726));
#40024=CARTESIAN_POINT('Ctrl Pts',(131.146121812408,38.9209220587922,26.7662759395025));
#40025=CARTESIAN_POINT('Ctrl Pts',(131.260808396864,38.8873981085414,26.7604736604065));
#40026=CARTESIAN_POINT('Ctrl Pts',(131.374042826227,38.8488323097756,26.7546713813104));
#40027=CARTESIAN_POINT('Ctrl Pts',(131.485357573226,38.805382750744,26.7488691022144));
#40028=CARTESIAN_POINT('Ctrl Pts',(131.596710419228,38.7619183205032,26.7430648372085));
#40029=CARTESIAN_POINT('Ctrl Pts',(131.706141889195,38.7135669378079,26.7372605722027));
#40030=CARTESIAN_POINT('Ctrl Pts',(131.813203483573,38.6605352241386,26.7314563071968));
#40031=CARTESIAN_POINT('Ctrl Pts',(131.920288084238,38.6074921145727,26.7256507949221));
#40032=CARTESIAN_POINT('Ctrl Pts',(132.025001434137,38.5497668617555,26.7198452826475));
#40033=CARTESIAN_POINT('Ctrl Pts',(132.126919784333,38.4876119668069,26.7140397703728));
#40034=CARTESIAN_POINT('Ctrl Pts',(132.228918119051,38.4254082933057,26.7082297019889));
#40035=CARTESIAN_POINT('Ctrl Pts',(132.328116733961,38.3587682615466,26.7024196336051));
#40036=CARTESIAN_POINT('Ctrl Pts',(132.424121131059,38.2879874911491,26.6966095652212));
#40037=CARTESIAN_POINT('Ctrl Pts',(132.445290840541,38.2723797857573,26.6953284003634));
#40038=CARTESIAN_POINT('Ctrl Pts',(132.466305362836,38.2565708981207,26.6940472355056));
#40039=CARTESIAN_POINT('Ctrl Pts',(132.487160689988,38.2405642567579,26.6927660706478));
#40040=CARTESIAN_POINT('',(125.915000003014,34.9998430692718,27.2396150285593));
#40041=CARTESIAN_POINT('Ctrl Pts',(125.915000003014,34.9998430692718,27.2396150285593));
#40042=CARTESIAN_POINT('Ctrl Pts',(125.914995442005,35.1185688455264,27.233798040471));
#40043=CARTESIAN_POINT('Ctrl Pts',(125.920171118825,35.2374883957075,27.2279810523828));
#40044=CARTESIAN_POINT('Ctrl Pts',(125.930551771767,35.3561125071268,27.2221640642946));
#40045=CARTESIAN_POINT('Ctrl Pts',(125.940919324587,35.4745869179101,27.2163544170986));
#40046=CARTESIAN_POINT('Ctrl Pts',(125.956478754098,35.5927662272477,27.2105447699026));
#40047=CARTESIAN_POINT('Ctrl Pts',(125.977202804292,35.7101603496408,27.2047351227065));
#40048=CARTESIAN_POINT('Ctrl Pts',(125.997906137723,35.8274371191898,27.1989312831149));
#40049=CARTESIAN_POINT('Ctrl Pts',(126.023763750782,35.9439298623713,27.1931274435233));
#40050=CARTESIAN_POINT('Ctrl Pts',(126.054696570429,36.0591533640682,27.1873236039317));
#40051=CARTESIAN_POINT('Ctrl Pts',(126.086567251909,36.1778703631443,27.1813437959126));
#40052=CARTESIAN_POINT('Ctrl Pts',(126.123825766443,36.2952394869812,27.1753639878935));
#40053=CARTESIAN_POINT('Ctrl Pts',(126.166328678407,36.4107406558232,27.1693841798744));
#40054=CARTESIAN_POINT('Ctrl Pts',(126.207534872459,36.5227180088249,27.1635868093356));
#40055=CARTESIAN_POINT('Ctrl Pts',(126.25366995735,36.6329393186652,27.1577894387969));
#40056=CARTESIAN_POINT('Ctrl Pts',(126.304552755165,36.7409464841407,27.1519920682581));
#40057=CARTESIAN_POINT('Ctrl Pts',(126.355428249845,36.8489381475025,27.1461955298076));
#40058=CARTESIAN_POINT('Ctrl Pts',(126.411049927902,36.9547159282086,27.1403989913572));
#40059=CARTESIAN_POINT('Ctrl Pts',(126.471189154825,37.0578432931049,27.1346024529067));
#40060=CARTESIAN_POINT('Ctrl Pts',(126.531334033706,37.1609803500354,27.1288053696905));
#40061=CARTESIAN_POINT('Ctrl Pts',(126.595997099273,37.2614661422752,27.1230082864743));
#40062=CARTESIAN_POINT('Ctrl Pts',(126.664904941967,37.3588908312773,27.1172112032582));
#40063=CARTESIAN_POINT('Ctrl Pts',(126.733835626964,37.4563478156505,27.1114121983633));
#40064=CARTESIAN_POINT('Ctrl Pts',(126.807013651039,37.5507413448013,27.1056131934684));
#40065=CARTESIAN_POINT('Ctrl Pts',(126.884124077338,37.6416930621432,27.0998141885735));
#40066=CARTESIAN_POINT('Ctrl Pts',(126.961320031876,37.7327456600085,27.0940087516214));
#40067=CARTESIAN_POINT('Ctrl Pts',(127.042456829378,37.8203485141111,27.0882033146693));
#40068=CARTESIAN_POINT('Ctrl Pts',(127.127181195765,37.9041585903719,27.0823978777172));
#40069=CARTESIAN_POINT('Ctrl Pts',(127.211961990312,37.9880244858578,27.0765885742253));
#40070=CARTESIAN_POINT('Ctrl Pts',(127.300334809232,38.0680922990568,27.0707792707334));
#40071=CARTESIAN_POINT('Ctrl Pts',(127.391912961667,38.1440590007952,27.0649699672416));
#40072=CARTESIAN_POINT('Ctrl Pts',(127.483621025753,38.2201334679702,27.0591524227426));
#40073=CARTESIAN_POINT('Ctrl Pts',(127.578543172832,38.2920949669791,27.0533348782437));
#40074=CARTESIAN_POINT('Ctrl Pts',(127.67626334802,38.3596834631023,27.0475173337447));
#40075=CARTESIAN_POINT('Ctrl Pts',(127.69703133574,38.3740477134203,27.0462809596543));
#40076=CARTESIAN_POINT('Ctrl Pts',(127.717925613344,38.3882146140039,27.0450445855638));
#40077=CARTESIAN_POINT('Ctrl Pts',(127.738942050042,38.4021819391287,27.0438082114734));
#40078=CARTESIAN_POINT('Ctrl Pts',(127.837934092801,38.467971114801,27.0379846173702));
#40079=CARTESIAN_POINT('Ctrl Pts',(127.93995951586,38.5295422912216,27.0321610232671));
#40080=CARTESIAN_POINT('Ctrl Pts',(128.044623506409,38.5866039324562,27.026337429164));
#40081=CARTESIAN_POINT('Ctrl Pts',(128.149155448036,38.6435935820906,27.0205211823759));
#40082=CARTESIAN_POINT('Ctrl Pts',(128.256318980616,38.6960848189604,27.0147049355879));
#40083=CARTESIAN_POINT('Ctrl Pts',(128.365689833005,38.7438289595088,27.0088886887999));
#40084=CARTESIAN_POINT('Ctrl Pts',(128.474951204815,38.7915253080173,27.0030782640938));
#40085=CARTESIAN_POINT('Ctrl Pts',(128.586415128756,38.8344838510123,26.9972678393877));
#40086=CARTESIAN_POINT('Ctrl Pts',(128.699632747636,38.8725017764978,26.9914574146816));
#40087=CARTESIAN_POINT('Ctrl Pts',(128.817135875057,38.9119587548976,26.9854270540242));
#40088=CARTESIAN_POINT('Ctrl Pts',(128.936527688606,38.946093487041,26.9793966933669));
#40089=CARTESIAN_POINT('Ctrl Pts',(129.057283182258,38.9747339535555,26.9733663327095));
#40090=CARTESIAN_POINT('Ctrl Pts',(129.173503588349,39.0022988000752,26.9675624479895));
#40091=CARTESIAN_POINT('Ctrl Pts',(129.290986660056,39.0247745208024,26.9617585632694));
#40092=CARTESIAN_POINT('Ctrl Pts',(129.409249566314,39.0420587483484,26.9559546785494));
#40093=CARTESIAN_POINT('Ctrl Pts',(129.52749500408,39.059340422859,26.9501516511152));
#40094=CARTESIAN_POINT('Ctrl Pts',(129.646519643388,39.0714320701358,26.9443486236811));
#40095=CARTESIAN_POINT('Ctrl Pts',(129.765832391457,39.0782827919492,26.9385455962469));
#40096=CARTESIAN_POINT('Ctrl Pts',(129.885155673786,39.0851341186208,26.9327420564567));
#40097=CARTESIAN_POINT('Ctrl Pts',(130.004766707767,39.0867435764065,26.9269385166666));
#40098=CARTESIAN_POINT('Ctrl Pts',(130.124171878897,39.0831123355219,26.9211349768764));
#40099=CARTESIAN_POINT('Ctrl Pts',(130.243615771911,39.0794799170628,26.9153295550572));
#40100=CARTESIAN_POINT('Ctrl Pts',(130.362853261368,39.0706034324065,26.909524133238));
#40101=CARTESIAN_POINT('Ctrl Pts',(130.481393981532,39.0565360635085,26.9037187114188));
#40102=CARTESIAN_POINT('Ctrl Pts',(130.600065974779,39.0424531162769,26.8979068606221));
#40103=CARTESIAN_POINT('Ctrl Pts',(130.718039252805,39.0231678585879,26.8920950098255));
#40104=CARTESIAN_POINT('Ctrl Pts',(130.834831637331,38.998784957623,26.8862831590288));
#40105=CARTESIAN_POINT('Ctrl Pts',(130.951700731853,38.9743860418104,26.8804674909709));
#40106=CARTESIAN_POINT('Ctrl Pts',(131.067386993449,38.9448829154418,26.8746518229129));
#40107=CARTESIAN_POINT('Ctrl Pts',(131.181423052175,38.9104302284774,26.8688361548549));
#40108=CARTESIAN_POINT('Ctrl Pts',(131.295622455345,38.8759281917278,26.8630121564751));
#40109=CARTESIAN_POINT('Ctrl Pts',(131.408166553786,38.8364625783396,26.8571881580953));
#40110=CARTESIAN_POINT('Ctrl Pts',(131.518607473237,38.7922363246809,26.8513641597155));
#40111=CARTESIAN_POINT('Ctrl Pts',(131.547907958011,38.780502895818,26.849819026112));
#40112=CARTESIAN_POINT('Ctrl Pts',(131.577060541272,38.768434632946,26.8482738925085));
#40113=CARTESIAN_POINT('Ctrl Pts',(131.606057163088,38.7560358609703,26.8467287589049));
#40114=CARTESIAN_POINT('Ctrl Pts',(131.71534415374,38.7093054354188,26.8409052183987));
#40115=CARTESIAN_POINT('Ctrl Pts',(131.822766155655,38.6577259138305,26.8350816778925));
#40116=CARTESIAN_POINT('Ctrl Pts',(131.92786292703,38.6014676917309,26.8292581373863));
#40117=CARTESIAN_POINT('Ctrl Pts',(132.032811661782,38.5452887135238,26.8234427997703));
#40118=CARTESIAN_POINT('Ctrl Pts',(132.13544132709,38.4844443406247,26.8176274621543));
#40119=CARTESIAN_POINT('Ctrl Pts',(132.235311565709,38.4191529951451,26.8118121245382));
#40120=CARTESIAN_POINT('Ctrl Pts',(132.321400925854,38.3628710613767,26.8067992327967));
#40121=CARTESIAN_POINT('Ctrl Pts',(132.405440001865,38.3032855814883,26.8017863410552));
#40122=CARTESIAN_POINT('Ctrl Pts',(132.487160689988,38.2405642567579,26.7967734493137));
#40123=CARTESIAN_POINT('Ctrl Pts',(132.487160689988,38.2405642567579,28.0469635225512));
#40124=CARTESIAN_POINT('Ctrl Pts',(132.583285477107,38.166787663266,28.0410441731393));
#40125=CARTESIAN_POINT('Ctrl Pts',(132.675995746464,38.0888295148761,28.0351248237274));
#40126=CARTESIAN_POINT('Ctrl Pts',(132.764929492593,38.0070566840336,28.0292054743156));
#40127=CARTESIAN_POINT('Ctrl Pts',(132.852423572582,37.9266075978979,28.0233819477751));
#40128=CARTESIAN_POINT('Ctrl Pts',(132.93654471212,37.8422069564201,28.0175584212346));
#40129=CARTESIAN_POINT('Ctrl Pts',(133.016915646074,37.7541686557783,28.0117348946941));
#40130=CARTESIAN_POINT('Ctrl Pts',(133.097185165944,37.6662414440985,28.0059187164272));
#40131=CARTESIAN_POINT('Ctrl Pts',(133.173713619382,37.5746860017517,28.0001025381602));
#40132=CARTESIAN_POINT('Ctrl Pts',(133.246158332574,37.4798550521875,27.9942863598933));
#40133=CARTESIAN_POINT('Ctrl Pts',(133.318530516696,37.3851190439971,27.9884760045772));
#40134=CARTESIAN_POINT('Ctrl Pts',(133.386826847656,37.2871143750181,27.9826656492611));
#40135=CARTESIAN_POINT('Ctrl Pts',(133.450743337022,37.186228584115,27.976855293945));
#40136=CARTESIAN_POINT('Ctrl Pts',(133.517080265402,37.0815223721155,27.9708249076034));
#40137=CARTESIAN_POINT('Ctrl Pts',(133.57869877448,36.9737128468161,27.9647945212618));
#40138=CARTESIAN_POINT('Ctrl Pts',(133.63530660868,36.8632688643578,27.9587641349203));
#40139=CARTESIAN_POINT('Ctrl Pts',(133.689787582147,36.7569744660143,27.9529603213155));
#40140=CARTESIAN_POINT('Ctrl Pts',(133.739627405286,36.6482403978658,27.9471565077107));
#40141=CARTESIAN_POINT('Ctrl Pts',(133.784611536174,36.5375111447598,27.9413526941059));
#40142=CARTESIAN_POINT('Ctrl Pts',(133.829589018434,36.4267982573705,27.9355497383013));
#40143=CARTESIAN_POINT('Ctrl Pts',(133.869712082004,36.314091149679,27.9297467824967));
#40144=CARTESIAN_POINT('Ctrl Pts',(133.904814199417,36.1998546028725,27.923943826692));
#40145=CARTESIAN_POINT('Ctrl Pts',(133.939919413428,36.0856079784762,27.9181403589688));
#40146=CARTESIAN_POINT('Ctrl Pts',(133.970002680679,35.9698320370626,27.9123368912457));
#40147=CARTESIAN_POINT('Ctrl Pts',(133.994947438924,35.8530064244976,27.9065334235225));
#40148=CARTESIAN_POINT('Ctrl Pts',(134.01990028505,35.7361429333669,27.9007280741311));
#40149=CARTESIAN_POINT('Ctrl Pts',(134.039711223514,35.6182294933733,27.8949227247398));
#40150=CARTESIAN_POINT('Ctrl Pts',(134.05431497822,35.4997549973523,27.8891173753485));
#40151=CARTESIAN_POINT('Ctrl Pts',(134.068934905027,35.3811493034675,27.8833055971521));
#40152=CARTESIAN_POINT('Ctrl Pts',(134.078336087863,35.2619817188892,27.8774938189557));
#40153=CARTESIAN_POINT('Ctrl Pts',(134.082505203085,35.1427454615142,27.8716820407593));
#40154=CARTESIAN_POINT('Ctrl Pts',(134.086677056511,35.0234308918224,27.8658664454873));
#40155=CARTESIAN_POINT('Ctrl Pts',(134.085610002428,34.9040479669033,27.8600508502152));
#40156=CARTESIAN_POINT('Ctrl Pts',(134.079342789243,34.7850874413916,27.8542352549432));
#40157=CARTESIAN_POINT('Ctrl Pts',(134.073066598532,34.6659565097759,27.848411329068));
#40158=CARTESIAN_POINT('Ctrl Pts',(134.061575420097,34.5472495902595,27.8425874031927));
#40159=CARTESIAN_POINT('Ctrl Pts',(134.044959544605,34.4294500175206,27.8367634773175));
#40160=CARTESIAN_POINT('Ctrl Pts',(134.040549267299,34.3981830052858,27.835217658794));
#40161=CARTESIAN_POINT('Ctrl Pts',(134.035778227379,34.3669798459467,27.8336718402706));
#40162=CARTESIAN_POINT('Ctrl Pts',(134.030648706343,34.3358494101089,27.8321260217471));
#40163=CARTESIAN_POINT('Ctrl Pts',(134.011324098492,34.2185707284023,27.8263024104256));
#40164=CARTESIAN_POINT('Ctrl Pts',(133.986845442737,34.1019470596537,27.8204787991041));
#40165=CARTESIAN_POINT('Ctrl Pts',(133.957268485043,33.9864660157217,27.8146551877826));
#40166=CARTESIAN_POINT('Ctrl Pts',(133.927728842282,33.8711306651854,27.8088389236557));
#40167=CARTESIAN_POINT('Ctrl Pts',(133.893103791357,33.7569354643154,27.8030226595288));
#40168=CARTESIAN_POINT('Ctrl Pts',(133.85350051373,33.6443603758074,27.797206395402));
#40169=CARTESIAN_POINT('Ctrl Pts',(133.813936878326,33.531897973091,27.7913959532588));
#40170=CARTESIAN_POINT('Ctrl Pts',(133.769405064257,33.4210528395336,27.7855855111156));
#40171=CARTESIAN_POINT('Ctrl Pts',(133.720062577152,33.312291665579,27.7797750689724));
#40172=CARTESIAN_POINT('Ctrl Pts',(133.668852589176,33.1994141286498,27.7737447148143));
#40173=CARTESIAN_POINT('Ctrl Pts',(133.612460699163,33.0887818482519,27.7677143606563));
#40174=CARTESIAN_POINT('Ctrl Pts',(133.551118842144,32.9808962461116,27.7616840064982));
#40175=CARTESIAN_POINT('Ctrl Pts',(133.492080494645,32.8770619642861,27.7558801042097));
#40176=CARTESIAN_POINT('Ctrl Pts',(133.42845745895,32.7757721807581,27.7500762019212));
#40177=CARTESIAN_POINT('Ctrl Pts',(133.36050389807,32.6774499895463,27.7442722996327));
#40178=CARTESIAN_POINT('Ctrl Pts',(133.292560374304,32.5791423210627,27.7384692546125));
#40179=CARTESIAN_POINT('Ctrl Pts',(133.220287829496,32.4838017090188,27.7326662095923));
#40180=CARTESIAN_POINT('Ctrl Pts',(133.14398372125,32.3918222145501,27.7268631645721));
#40181=CARTESIAN_POINT('Ctrl Pts',(133.06767287607,32.299834599159,27.7210596071977));
#40182=CARTESIAN_POINT('Ctrl Pts',(132.987330020464,32.2112090056498,27.7152560498233));
#40183=CARTESIAN_POINT('Ctrl Pts',(132.903292433126,32.1263058534778,27.7094524924489));
#40184=CARTESIAN_POINT('Ctrl Pts',(132.819227593641,32.0413751684698,27.7036470530667));
#40185=CARTESIAN_POINT('Ctrl Pts',(132.731465926685,31.9601696155756,27.6978416136845));
#40186=CARTESIAN_POINT('Ctrl Pts',(132.640380557726,31.8830117885395,27.6920361743024));
#40187=CARTESIAN_POINT('Ctrl Pts',(132.54919432219,31.8057685180788,27.6862243060634));
#40188=CARTESIAN_POINT('Ctrl Pts',(132.454677349579,31.7325821848003,27.6804124378244));
#40189=CARTESIAN_POINT('Ctrl Pts',(132.35723486092,31.6637343015785,27.6746005695854));
#40190=CARTESIAN_POINT('Ctrl Pts',(132.259728372431,31.5948411993473,27.668784884135));
#40191=CARTESIAN_POINT('Ctrl Pts',(132.159292883962,31.5302924422394,27.6629691986846));
#40192=CARTESIAN_POINT('Ctrl Pts',(132.056360100272,31.4703246412723,27.6571535132342));
#40193=CARTESIAN_POINT('Ctrl Pts',(131.953279880483,31.4102709452354,27.6513294976683));
#40194=CARTESIAN_POINT('Ctrl Pts',(131.847695586173,31.3548114910392,27.6455054821024));
#40195=CARTESIAN_POINT('Ctrl Pts',(131.740060969837,31.3041357139024,27.6396814665365));
#40196=CARTESIAN_POINT('Ctrl Pts',(131.71150819594,31.2906926966291,27.6381365007506));
#40197=CARTESIAN_POINT('Ctrl Pts',(131.682811231503,31.2775860416633,27.6365915349646));
#40198=CARTESIAN_POINT('Ctrl Pts',(131.653978731735,31.2648186985144,27.6350465691787));
#40199=CARTESIAN_POINT('Ctrl Pts',(131.545297395629,31.2166934258846,27.6292229691716));
#40200=CARTESIAN_POINT('Ctrl Pts',(131.43433863683,31.1732378844396,27.6233993691645));
#40201=CARTESIAN_POINT('Ctrl Pts',(131.321540835858,31.1346727410012,27.6175757691575));
#40202=CARTESIAN_POINT('Ctrl Pts',(131.208885343006,31.0961562521731,27.6117595163288));
#40203=CARTESIAN_POINT('Ctrl Pts',(131.094395805726,31.0625180206387,27.6059432635002));
#40204=CARTESIAN_POINT('Ctrl Pts',(130.978532402161,31.0339315011057,27.6001270106715));
#40205=CARTESIAN_POINT('Ctrl Pts',(130.862784975558,31.0053735961101,27.5943165797962));
#40206=CARTESIAN_POINT('Ctrl Pts',(130.745666812655,30.9818574407616,27.5885061489209));
#40207=CARTESIAN_POINT('Ctrl Pts',(130.627654577018,30.9635071247495,27.5826957180457));
#40208=CARTESIAN_POINT('Ctrl Pts',(130.505175523237,30.9444622407201,27.5766653596525));
#40209=CARTESIAN_POINT('Ctrl Pts',(130.381733801461,30.9309821262726,27.5706350012594));
#40210=CARTESIAN_POINT('Ctrl Pts',(130.257875927179,30.9231476595072,27.5646046428662));
#40211=CARTESIAN_POINT('Ctrl Pts',(130.138669476049,30.9156074123892,27.5588007516946));
#40212=CARTESIAN_POINT('Ctrl Pts',(130.019078009738,30.9132964485294,27.5529968605229));
#40213=CARTESIAN_POINT('Ctrl Pts',(129.899594713185,30.9162341180744,27.5471929693512));
#40214=CARTESIAN_POINT('Ctrl Pts',(129.780129063444,30.919171353747,27.541389935372));
#40215=CARTESIAN_POINT('Ctrl Pts',(129.660771959791,30.9273556711925,27.5355869013928));
#40216=CARTESIAN_POINT('Ctrl Pts',(129.542016037412,30.9407542954371,27.5297838674136));
#40217=CARTESIAN_POINT('Ctrl Pts',(129.423249628174,30.9541541028605,27.5239803209917));
#40218=CARTESIAN_POINT('Ctrl Pts',(129.305084911542,30.9727690867957,27.5181767745699));
#40219=CARTESIAN_POINT('Ctrl Pts',(129.18800821421,30.9965147259158,27.512373228148));
#40220=CARTESIAN_POINT('Ctrl Pts',(129.070893548525,31.0202680658237,27.5065677996172));
#40221=CARTESIAN_POINT('Ctrl Pts',(128.954868003857,31.0491552888899,27.5007623710865));
#40222=CARTESIAN_POINT('Ctrl Pts',(128.840405920406,31.0830411579172,27.4949569425557));
#40223=CARTESIAN_POINT('Ctrl Pts',(128.725817079056,31.1169645529219,27.4891450849621));
#40224=CARTESIAN_POINT('Ctrl Pts',(128.61279554674,31.155897527465,27.4833332273686));
#40225=CARTESIAN_POINT('Ctrl Pts',(128.501798898363,31.1996554815314,27.477521369775));
#40226=CARTESIAN_POINT('Ctrl Pts',(128.39072934565,31.2434421765072,27.4717056948624));
#40227=CARTESIAN_POINT('Ctrl Pts',(128.281687697644,31.2920599964923,27.4658900199498));
#40228=CARTESIAN_POINT('Ctrl Pts',(128.175108491949,31.3452775777301,27.4600743450371));
#40229=CARTESIAN_POINT('Ctrl Pts',(128.06837662253,31.3985713876661,27.4542503397698));
#40230=CARTESIAN_POINT('Ctrl Pts',(127.964114591217,31.4564779119516,27.4484263345025));
#40231=CARTESIAN_POINT('Ctrl Pts',(127.862729564812,31.5187214867423,27.4426023292352));
#40232=CARTESIAN_POINT('Ctrl Pts',(127.835832773983,31.5352343039789,27.4410572583602));
#40233=CARTESIAN_POINT('Ctrl Pts',(127.809138294224,31.5520521409498,27.4395121874852));
#40234=CARTESIAN_POINT('Ctrl Pts',(127.782653338354,31.5691693743226,27.4379671166102));
#40235=CARTESIAN_POINT('Ctrl Pts',(127.682827870344,31.6336865983971,27.4321435304219));
#40236=CARTESIAN_POINT('Ctrl Pts',(127.585659605872,31.7026683513086,27.4263199442336));
#40237=CARTESIAN_POINT('Ctrl Pts',(127.491573407953,31.775868949265,27.4204963580452));
#40238=CARTESIAN_POINT('Ctrl Pts',(127.397605915691,31.8489771922829,27.4146801192961));
#40239=CARTESIAN_POINT('Ctrl Pts',(127.306713075196,31.9262934449156,27.408863880547));
#40240=CARTESIAN_POINT('Ctrl Pts',(127.219292211587,32.0075279123338,27.4030476417979));
#40241=CARTESIAN_POINT('Ctrl Pts',(127.131958858376,32.0886810620874,27.3972372252443));
#40242=CARTESIAN_POINT('Ctrl Pts',(127.048090865319,32.173744347478,27.3914268086907));
#40243=CARTESIAN_POINT('Ctrl Pts',(126.968053307013,32.2623871254526,27.3856163921371));
#40244=CARTESIAN_POINT('Ctrl Pts',(126.884986012364,32.3543853811768,27.3795860284665));
#40245=CARTESIAN_POINT('Ctrl Pts',(126.806045230369,32.4502392046965,27.3735556647959));
#40246=CARTESIAN_POINT('Ctrl Pts',(126.731598188848,32.549535839712,27.3675253011252));
#40247=CARTESIAN_POINT('Ctrl Pts',(126.659947216176,32.6451031092299,27.3617214247893));
#40248=CARTESIAN_POINT('Ctrl Pts',(126.592458788309,32.743858889048,27.3559175484534));
#40249=CARTESIAN_POINT('Ctrl Pts',(126.529419435327,32.8454013032322,27.3501136721175));
#40250=CARTESIAN_POINT('Ctrl Pts',(126.466389394609,32.946928717425,27.3443106531385));
#40251=CARTESIAN_POINT('Ctrl Pts',(126.407807337083,33.0512416005238,27.3385076341595));
#40252=CARTESIAN_POINT('Ctrl Pts',(126.353915895638,33.1579099631354,27.3327046151806));
#40253=CARTESIAN_POINT('Ctrl Pts',(126.300019696624,33.2645877424926,27.3269010839077));
#40254=CARTESIAN_POINT('Ctrl Pts',(126.250815121148,33.3736210503216,27.3210975526348));
#40255=CARTESIAN_POINT('Ctrl Pts',(126.20649806493,33.4845568078543,27.315294021362));
#40256=CARTESIAN_POINT('Ctrl Pts',(126.162166637525,33.5955285397647,27.3094886081131));
#40257=CARTESIAN_POINT('Ctrl Pts',(126.122726032854,33.7084035693056,27.3036831948643));
#40258=CARTESIAN_POINT('Ctrl Pts',(126.088323158834,33.8227110421468,27.2978777816155));
#40259=CARTESIAN_POINT('Ctrl Pts',(126.053882186911,33.9371450996128,27.2920659394252));
#40260=CARTESIAN_POINT('Ctrl Pts',(126.024490199166,34.0530143755138,27.2862540972348));
#40261=CARTESIAN_POINT('Ctrl Pts',(126.000243627778,34.1698349785303,27.2804422550445));
#40262=CARTESIAN_POINT('Ctrl Pts',(125.975981131191,34.2867323095666,27.2746265956239));
#40263=CARTESIAN_POINT('Ctrl Pts',(125.956870846573,34.4045818099437,27.2688109362033));
#40264=CARTESIAN_POINT('Ctrl Pts',(125.942957466058,34.5228932218206,27.2629952767826));
#40265=CARTESIAN_POINT('Ctrl Pts',(125.929024156037,34.6413741027878,27.2571712870201));
#40266=CARTESIAN_POINT('Ctrl Pts',(125.920302637767,34.7603178100554,27.2513472972576));
#40267=CARTESIAN_POINT('Ctrl Pts',(125.916785548389,34.879232694178,27.2455233074951));
#40268=CARTESIAN_POINT('Ctrl Pts',(125.915852398148,34.9107830589372,27.2439780930107));
#40269=CARTESIAN_POINT('Ctrl Pts',(125.915285325455,34.9423314174167,27.2424328785262));
#40270=CARTESIAN_POINT('Ctrl Pts',(125.915083580702,34.9738686519398,27.2408876640418));
#40271=CARTESIAN_POINT('Ctrl Pts',(125.915028195182,34.9825266522665,27.2404634522263));
#40272=CARTESIAN_POINT('Ctrl Pts',(125.915000335634,34.9911848288518,27.2400392404109));
#40273=CARTESIAN_POINT('Ctrl Pts',(125.915000003014,34.999843068532,27.2396150285955));
#40274=CARTESIAN_POINT('Origin',(130.,35.,32.7603849714045));
#40275=CARTESIAN_POINT('',(132.487160689988,38.2405642567579,29.2969312480094));
#40276=CARTESIAN_POINT('',(132.487160689988,38.2405642567579,29.1925548573102));
#40277=CARTESIAN_POINT('',(132.487160689988,38.2405642567579,32.7603849714045));
#40278=CARTESIAN_POINT('',(125.917751830235,34.9961206828433,29.7396160661079));
#40279=CARTESIAN_POINT('Ctrl Pts',(125.915001824241,34.996139424357,29.7396150285955));
#40280=CARTESIAN_POINT('Ctrl Pts',(125.914889749838,35.1147289232925,29.7338556081825));
#40281=CARTESIAN_POINT('Ctrl Pts',(125.919946015895,35.2333981463432,29.7280961877695));
#40282=CARTESIAN_POINT('Ctrl Pts',(125.930164564399,35.3516596751537,29.7223367673564));
#40283=CARTESIAN_POINT('Ctrl Pts',(125.940380529293,35.4698913032599,29.7165788031289));
#40284=CARTESIAN_POINT('Ctrl Pts',(125.955756146661,35.5877150288388,29.7108208389015));
#40285=CARTESIAN_POINT('Ctrl Pts',(125.976233330414,35.7046465700795,29.705062874674));
#40286=CARTESIAN_POINT('Ctrl Pts',(125.996710352475,35.8215771880147,29.699304955912));
#40287=CARTESIAN_POINT('Ctrl Pts',(126.022288789158,35.937615226823,29.6935470371501));
#40288=CARTESIAN_POINT('Ctrl Pts',(126.052859197963,36.0522853647639,29.6877891183882));
#40289=CARTESIAN_POINT('Ctrl Pts',(126.083436853566,36.1669826855672,29.6820298346963));
#40290=CARTESIAN_POINT('Ctrl Pts',(126.11900872687,36.280311059955,29.6762705510044));
#40291=CARTESIAN_POINT('Ctrl Pts',(126.159415358592,36.3918098333407,29.6705112673124));
#40292=CARTESIAN_POINT('Ctrl Pts',(126.199867100876,36.5034330856062,29.664745553871));
#40293=CARTESIAN_POINT('Ctrl Pts',(126.245164237707,36.6132222675609,29.6589798404296));
#40294=CARTESIAN_POINT('Ctrl Pts',(126.29509887264,36.7207360740361,29.6532141269882));
#40295=CARTESIAN_POINT('Ctrl Pts',(126.345063092839,36.8283135802748,29.6474449974777));
#40296=CARTESIAN_POINT('Ctrl Pts',(126.399670090961,36.9336126589249,29.6416758679673));
#40297=CARTESIAN_POINT('Ctrl Pts',(126.458666546603,37.0362176631811,29.6359067384569));
#40298=CARTESIAN_POINT('Ctrl Pts',(126.517759864122,37.1389911269355,29.6301281370433));
#40299=CARTESIAN_POINT('Ctrl Pts',(126.581256810047,37.2390613324478,29.6243495356297));
#40300=CARTESIAN_POINT('Ctrl Pts',(126.648861158634,37.3360422654332,29.6185709342161));
#40301=CARTESIAN_POINT('Ctrl Pts',(126.69850364912,37.4072562500898,29.6143276544318));
#40302=CARTESIAN_POINT('Ctrl Pts',(126.750360003743,37.4768051112654,29.6100843746475));
#40303=CARTESIAN_POINT('Ctrl Pts',(126.804299961969,37.5445483424232,29.6058410948631));
#40304=CARTESIAN_POINT('Ctrl Pts',(126.878347528946,37.6375447334366,29.600016015379));
#40305=CARTESIAN_POINT('Ctrl Pts',(126.956578022739,37.7274571730994,29.5941909358949));
#40306=CARTESIAN_POINT('Ctrl Pts',(127.038705298708,37.8138867589329,29.5883658564108));
#40307=CARTESIAN_POINT('Ctrl Pts',(127.120727860562,37.900206145111,29.5825482040334));
#40308=CARTESIAN_POINT('Ctrl Pts',(127.206637043737,37.9830512167573,29.5767305516559));
#40309=CARTESIAN_POINT('Ctrl Pts',(127.296105493946,38.0620547839862,29.5709128992785));
#40310=CARTESIAN_POINT('Ctrl Pts',(127.38548316037,38.1409781861636,29.5651011500826));
#40311=CARTESIAN_POINT('Ctrl Pts',(127.47841260485,38.2160675699333,29.5592894008868));
#40312=CARTESIAN_POINT('Ctrl Pts',(127.574528968689,38.2869918278376,29.5534776516909));
#40313=CARTESIAN_POINT('Ctrl Pts',(127.674252076596,38.3605775019278,29.547447817966));
#40314=CARTESIAN_POINT('Ctrl Pts',(127.777405659419,38.4296790098314,29.5414179842412));
#40315=CARTESIAN_POINT('Ctrl Pts',(127.883543317398,38.4939713952275,29.5353881505164));
#40316=CARTESIAN_POINT('Ctrl Pts',(127.985723378708,38.5558664851201,29.5295831535772));
#40317=CARTESIAN_POINT('Ctrl Pts',(128.090668581765,38.6133044408925,29.523778156638));
#40318=CARTESIAN_POINT('Ctrl Pts',(128.197950853518,38.666039262428,29.5179731596989));
#40319=CARTESIAN_POINT('Ctrl Pts',(128.305215790772,38.7187655631543,29.5121691007219));
#40320=CARTESIAN_POINT('Ctrl Pts',(128.414816679574,38.7667900609737,29.506365041745));
#40321=CARTESIAN_POINT('Ctrl Pts',(128.526301742813,38.8099131810009,29.5005609827681));
#40322=CARTESIAN_POINT('Ctrl Pts',(128.637795070035,38.8530394975884,29.4947564935573));
#40323=CARTESIAN_POINT('Ctrl Pts',(128.751172468688,38.8912635668722,29.4889520043466));
#40324=CARTESIAN_POINT('Ctrl Pts',(128.865963731343,38.9244345760084,29.4831475151359));
#40325=CARTESIAN_POINT('Ctrl Pts',(128.980790559682,38.9576158624917,29.4773412275249));
#40326=CARTESIAN_POINT('Ctrl Pts',(129.097031731301,38.9857408620556,29.471534939914));
#40327=CARTESIAN_POINT('Ctrl Pts',(129.214204113059,39.0087092466362,29.465728652303));
#40328=CARTESIAN_POINT('Ctrl Pts',(129.331503629525,39.0317025524383,29.4599160647375));
#40329=CARTESIAN_POINT('Ctrl Pts',(129.449735972206,39.0495279964193,29.454103477172));
#40330=CARTESIAN_POINT('Ctrl Pts',(129.568409950964,39.062136756631,29.4482908896064));
#40331=CARTESIAN_POINT('Ctrl Pts',(129.687160346985,39.0747536359515,29.4424745591645));
#40332=CARTESIAN_POINT('Ctrl Pts',(129.806352538996,39.0821471161672,29.4366582287226));
#40333=CARTESIAN_POINT('Ctrl Pts',(129.925494024779,39.0843204893417,29.4308418982807));
#40334=CARTESIAN_POINT('Ctrl Pts',(130.044803802069,39.0864969324816,29.4250173520691));
#40335=CARTESIAN_POINT('Ctrl Pts',(130.164062323563,39.0834385615248,29.4191928058575));
#40336=CARTESIAN_POINT('Ctrl Pts',(130.282780763463,39.0752006134441,29.4133682596459));
#40337=CARTESIAN_POINT('Ctrl Pts',(130.314078791113,39.0730288233917,29.4118327205288));
#40338=CARTESIAN_POINT('Ctrl Pts',(130.345339331425,39.0704973189299,29.4102971814117));
#40339=CARTESIAN_POINT('Ctrl Pts',(130.376553548765,39.0676077029272,29.4087616422947));
#40340=CARTESIAN_POINT('Ctrl Pts',(130.495101696714,39.0566332606825,29.4029298344217));
#40341=CARTESIAN_POINT('Ctrl Pts',(130.613354340383,39.0404549061107,29.3970980265487));
#40342=CARTESIAN_POINT('Ctrl Pts',(130.730819924737,39.0190953257677,29.3912662186756));
#40343=CARTESIAN_POINT('Ctrl Pts',(130.848147554704,38.9977608306259,29.385441259817));
#40344=CARTESIAN_POINT('Ctrl Pts',(130.964689566696,38.9712572826434,29.3796163009584));
#40345=CARTESIAN_POINT('Ctrl Pts',(131.079958497732,38.9396592039384,29.3737913420998));
#40346=CARTESIAN_POINT('Ctrl Pts',(131.195119026777,38.9080908409133,29.3679718611886));
#40347=CARTESIAN_POINT('Ctrl Pts',(131.30900846612,38.8714375842934,29.3621523802774));
#40348=CARTESIAN_POINT('Ctrl Pts',(131.421149147708,38.8298250743302,29.3563328993662));
#40349=CARTESIAN_POINT('Ctrl Pts',(131.533206202672,38.7882435960469,29.3505177582141));
#40350=CARTESIAN_POINT('Ctrl Pts',(131.643516715352,38.7417103665766,29.3447026170619));
#40351=CARTESIAN_POINT('Ctrl Pts',(131.751618452759,38.6904007635967,29.3388874759098));
#40352=CARTESIAN_POINT('Ctrl Pts',(131.859673491464,38.6391133257726,29.3330748468315));
#40353=CARTESIAN_POINT('Ctrl Pts',(131.965521286858,38.5830537948526,29.3272622177532));
#40354=CARTESIAN_POINT('Ctrl Pts',(132.068720326361,38.5224453453957,29.3214495886748));
#40355=CARTESIAN_POINT('Ctrl Pts',(132.171909973374,38.4618424121171,29.3156374886234));
#40356=CARTESIAN_POINT('Ctrl Pts',(132.272450991652,38.3966915867888,29.3098253885719));
#40357=CARTESIAN_POINT('Ctrl Pts',(132.369927599751,38.327261362132,29.3040132885205));
#40358=CARTESIAN_POINT('Ctrl Pts',(132.409519329725,38.2990611327622,29.3016526083501));
#40359=CARTESIAN_POINT('Ctrl Pts',(132.448605844018,38.270155429686,29.2992919281797));
#40360=CARTESIAN_POINT('Ctrl Pts',(132.487160689988,38.2405642567579,29.2969312480094));
#40361=CARTESIAN_POINT('',(128.942095577027,31.0543614925016,30.));
#40362=CARTESIAN_POINT('Ctrl Pts',(128.942095577027,31.0543614925016,30.));
#40363=CARTESIAN_POINT('Ctrl Pts',(127.639207105396,31.4036918921719,29.9343068491439));
#40364=CARTESIAN_POINT('Ctrl Pts',(126.178813659546,32.7814902171539,29.8475123998616));
#40365=CARTESIAN_POINT('Ctrl Pts',(125.916229948997,34.5620777500272,29.7607179505793));
#40366=CARTESIAN_POINT('Ctrl Pts',(125.919305187798,34.9961100965856,29.7396166521532));
#40367=CARTESIAN_POINT('',(131.058681707805,31.0545699801468,29.9999998737456));
#40368=CARTESIAN_POINT('Origin',(130.,35.,30.));
#40369=CARTESIAN_POINT('',(125.915000700078,35.0023915761614,29.6353849714475));
#40370=CARTESIAN_POINT('Ctrl Pts',(131.058681707805,31.0545699801468,29.9999998737456));
#40371=CARTESIAN_POINT('Ctrl Pts',(130.944553694239,31.0239458809479,29.9942106310195));
#40372=CARTESIAN_POINT('Ctrl Pts',(130.828901062776,30.9982256960231,29.9884213882935));
#40373=CARTESIAN_POINT('Ctrl Pts',(130.71218552957,30.9775608430368,29.9826321455674));
#40374=CARTESIAN_POINT('Ctrl Pts',(130.595617536489,30.9569221124944,29.976850221024));
#40375=CARTESIAN_POINT('Ctrl Pts',(130.477989717063,30.941326078079,29.9710682964807));
#40376=CARTESIAN_POINT('Ctrl Pts',(130.359778326282,30.9308742270682,29.9652863719373));
#40377=CARTESIAN_POINT('Ctrl Pts',(130.241684578543,30.920432777657,29.9595102015195));
#40378=CARTESIAN_POINT('Ctrl Pts',(130.123008824251,30.9151253657466,29.9537340311018));
#40379=CARTESIAN_POINT('Ctrl Pts',(130.004236212763,30.915002196512,29.9479578606841));
#40380=CARTESIAN_POINT('Ctrl Pts',(129.885547348981,30.9148791141253,29.9421857630994));
#40381=CARTESIAN_POINT('Ctrl Pts',(129.76676217621,30.9199330037176,29.9364136655148));
#40382=CARTESIAN_POINT('Ctrl Pts',(129.648369007186,30.9301620861645,29.9306415679301));
#40383=CARTESIAN_POINT('Ctrl Pts',(129.530019950461,30.9403873573414,29.9248716209805));
#40384=CARTESIAN_POINT('Ctrl Pts',(129.412063018777,30.9557839527955,29.9191016740308));
#40385=CARTESIAN_POINT('Ctrl Pts',(129.294983975858,30.9762980471084,29.9133317270811));
#40386=CARTESIAN_POINT('Ctrl Pts',(129.177920061441,30.9968094906693,29.9075625257017));
#40387=CARTESIAN_POINT('Ctrl Pts',(129.061734217666,31.0224370467372,29.9017933243223));
#40388=CARTESIAN_POINT('Ctrl Pts',(128.946903845468,31.0530754391158,29.8960241229428));
#40389=CARTESIAN_POINT('Ctrl Pts',(128.832060363897,31.0837173292635,29.8902542629344));
#40390=CARTESIAN_POINT('Ctrl Pts',(128.718573061178,31.1193710858633,29.8844844029259));
#40391=CARTESIAN_POINT('Ctrl Pts',(128.606905268368,31.1598812428911,29.8787145429175));
#40392=CARTESIAN_POINT('Ctrl Pts',(128.495128598352,31.2004308977242,29.8729390572382));
#40393=CARTESIAN_POINT('Ctrl Pts',(128.385175371563,31.2458462698854,29.867163571559));
#40394=CARTESIAN_POINT('Ctrl Pts',(128.277490140854,31.2959232209435,29.8613880858797));
#40395=CARTESIAN_POINT('Ctrl Pts',(128.169752954189,31.3460243331225,29.8556098136449));
#40396=CARTESIAN_POINT('Ctrl Pts',(128.064286310647,31.4007913138103,29.8498315414101));
#40397=CARTESIAN_POINT('Ctrl Pts',(127.961509692585,31.4599742562271,29.8440532691753));
#40398=CARTESIAN_POINT('Ctrl Pts',(127.858568541823,31.5192519432417,29.8382657466387));
#40399=CARTESIAN_POINT('Ctrl Pts',(127.758326370728,31.5829594952617,29.8324782241021));
#40400=CARTESIAN_POINT('Ctrl Pts',(127.661173674137,31.6508036161713,29.8266907015654));
#40401=CARTESIAN_POINT('Ctrl Pts',(127.568700420687,31.7153799666809,29.8211819400266));
#40402=CARTESIAN_POINT('Ctrl Pts',(127.479026186404,31.7837034796188,29.8156731784877));
#40403=CARTESIAN_POINT('Ctrl Pts',(127.392457758307,31.855489154449,29.8101644169488));
#40404=CARTESIAN_POINT('Ctrl Pts',(127.302025752593,31.9304786477225,29.8044097975579));
#40405=CARTESIAN_POINT('Ctrl Pts',(127.214671299808,32.0095052659351,29.798655178167));
#40406=CARTESIAN_POINT('Ctrl Pts',(127.130781969864,32.0922839038963,29.7929005587761));
#40407=CARTESIAN_POINT('Ctrl Pts',(127.046997055345,32.1749595088883,29.7871531020486));
#40408=CARTESIAN_POINT('Ctrl Pts',(126.966668984812,32.2613775576429,29.7814056453211));
#40409=CARTESIAN_POINT('Ctrl Pts',(126.890153096931,32.351212118822,29.7756581885937));
#40410=CARTESIAN_POINT('Ctrl Pts',(126.812342378029,32.4425668946896,29.7698134712126));
#40411=CARTESIAN_POINT('Ctrl Pts',(126.73847439577,32.5374546098222,29.7639687538315));
#40412=CARTESIAN_POINT('Ctrl Pts',(126.668884897651,32.635492191829,29.7581240364504));
#40413=CARTESIAN_POINT('Ctrl Pts',(126.600566657509,32.7317388274777,29.7523860901166));
#40414=CARTESIAN_POINT('Ctrl Pts',(126.536372168709,32.8310208696339,29.7466481437828));
#40415=CARTESIAN_POINT('Ctrl Pts',(126.476578752887,32.9329422563966,29.7409101974491));
#40416=CARTESIAN_POINT('Ctrl Pts',(126.416805312543,33.0348295937833,29.7351741680191));
#40417=CARTESIAN_POINT('Ctrl Pts',(126.361430234331,33.1393541620145,29.7294381385891));
#40418=CARTESIAN_POINT('Ctrl Pts',(126.310686796147,33.2460920537632,29.7237021091591));
#40419=CARTESIAN_POINT('Ctrl Pts',(126.259947629509,33.3528209603905,29.7179665625841));
#40420=CARTESIAN_POINT('Ctrl Pts',(126.213839506695,33.461762441258,29.7122310160091));
#40421=CARTESIAN_POINT('Ctrl Pts',(126.172548779272,33.5724699117186,29.7064954694341));
#40422=CARTESIAN_POINT('Ctrl Pts',(126.129887861217,33.6868510965559,29.7005695946018));
#40423=CARTESIAN_POINT('Ctrl Pts',(126.092369808768,33.8031170769029,29.6946437197696));
#40424=CARTESIAN_POINT('Ctrl Pts',(126.060144907995,33.9207563509546,29.6887178449374));
#40425=CARTESIAN_POINT('Ctrl Pts',(126.028921947958,34.0347379696549,29.6829762181632));
#40426=CARTESIAN_POINT('Ctrl Pts',(126.002667911715,34.1500083207628,29.677234591389));
#40427=CARTESIAN_POINT('Ctrl Pts',(125.981467580148,34.2660911564792,29.6714929646148));
#40428=CARTESIAN_POINT('Ctrl Pts',(125.959246774748,34.3877616168948,29.6654749657536));
#40429=CARTESIAN_POINT('Ctrl Pts',(125.942578397506,34.5103242084155,29.6594569668924));
#40430=CARTESIAN_POINT('Ctrl Pts',(125.931498882735,34.6332253296512,29.6534389680311));
#40431=CARTESIAN_POINT('Ctrl Pts',(125.920419367963,34.7561264508869,29.6474209691699));
#40432=CARTESIAN_POINT('Ctrl Pts',(125.914928674105,34.8793655759917,29.6414029703087));
#40433=CARTESIAN_POINT('Ctrl Pts',(125.915000700078,35.0023915761614,29.6353849714475));
#40434=CARTESIAN_POINT('Ctrl Pts',(125.915000700078,35.0023915770396,29.6353849714045));
#40435=CARTESIAN_POINT('Ctrl Pts',(125.915089665438,35.1543513193162,29.6279516357298));
#40436=CARTESIAN_POINT('Ctrl Pts',(125.923657514619,35.3060550304906,29.6205183000551));
#40437=CARTESIAN_POINT('Ctrl Pts',(125.940621235519,35.4568030718808,29.6130849643803));
#40438=CARTESIAN_POINT('Ctrl Pts',(125.953900081771,35.5748054887038,29.6072663045385));
#40439=CARTESIAN_POINT('Ctrl Pts',(125.972350307904,35.6924218713687,29.6014476446966));
#40440=CARTESIAN_POINT('Ctrl Pts',(125.995942053243,35.8091631226211,29.5956289848548));
#40441=CARTESIAN_POINT('Ctrl Pts',(126.019503759575,35.9257557290356,29.5898177338229));
#40442=CARTESIAN_POINT('Ctrl Pts',(126.048193884333,36.0414750228149,29.584006482791));
#40443=CARTESIAN_POINT('Ctrl Pts',(126.081930799845,36.1558368149516,29.5781952317592));
#40444=CARTESIAN_POINT('Ctrl Pts',(126.115633595803,36.2700829482247,29.5723898578885));
#40445=CARTESIAN_POINT('Ctrl Pts',(126.154372914053,36.3829739208238,29.5665844840179));
#40446=CARTESIAN_POINT('Ctrl Pts',(126.198016172837,36.4940361367748,29.5607791101473));
#40447=CARTESIAN_POINT('Ctrl Pts',(126.243364900283,36.6094383844783,29.5547468768833));
#40448=CARTESIAN_POINT('Ctrl Pts',(126.294008557267,36.7228655953719,29.5487146436193));
#40449=CARTESIAN_POINT('Ctrl Pts',(126.34974131207,36.833803836618,29.5426824103553));
#40450=CARTESIAN_POINT('Ctrl Pts',(126.403316678513,36.940447711448,29.5368836819645));
#40451=CARTESIAN_POINT('Ctrl Pts',(126.461594280714,37.0447913246213,29.5310849535736));
#40452=CARTESIAN_POINT('Ctrl Pts',(126.524342668129,37.1463995693751,29.5252862251827));
#40453=CARTESIAN_POINT('Ctrl Pts',(126.58708145292,37.2479922646317,29.5194883841933));
#40454=CARTESIAN_POINT('Ctrl Pts',(126.654289447445,37.3468500758802,29.513690543204));
#40455=CARTESIAN_POINT('Ctrl Pts',(126.725690452848,37.442564633623,29.5078927022146));
#40456=CARTESIAN_POINT('Ctrl Pts',(126.797097465056,37.5382872436164,29.5020943734659));
#40457=CARTESIAN_POINT('Ctrl Pts',(126.872697944781,37.6308657464102,29.4962960447173));
#40458=CARTESIAN_POINT('Ctrl Pts',(126.952174179912,37.7199233023017,29.4904977159686));
#40459=CARTESIAN_POINT('Ctrl Pts',(127.031675949859,37.8090094713801,29.4846975242824));
#40460=CARTESIAN_POINT('Ctrl Pts',(127.115055679291,37.8945721387752,29.4788973325961));
#40461=CARTESIAN_POINT('Ctrl Pts',(127.201957902164,37.9762703873701,29.4730971409099));
#40462=CARTESIAN_POINT('Ctrl Pts',(127.288956415624,38.0580591603736,29.4672905224161));
#40463=CARTESIAN_POINT('Ctrl Pts',(127.379484914967,38.1359746871951,29.4614839039223));
#40464=CARTESIAN_POINT('Ctrl Pts',(127.473153764485,38.2097154238444,29.4556772854286));
#40465=CARTESIAN_POINT('Ctrl Pts',(127.566884071184,38.283504542617,29.4498668571473));
#40466=CARTESIAN_POINT('Ctrl Pts',(127.663758499734,38.3531131782535,29.4440564288661));
#40467=CARTESIAN_POINT('Ctrl Pts',(127.763358663228,38.4182832724397,29.4382460005849));
#40468=CARTESIAN_POINT('Ctrl Pts',(127.863102118224,38.4835471247119,29.4324272130302));
#40469=CARTESIAN_POINT('Ctrl Pts',(127.965578784413,38.5443594823737,29.4266084254756));
#40470=CARTESIAN_POINT('Ctrl Pts',(128.070345840423,38.6005082730676,29.420789637921));
#40471=CARTESIAN_POINT('Ctrl Pts',(128.099058511997,38.6158965243734,29.4191949292179));
#40472=CARTESIAN_POINT('Ctrl Pts',(128.12794310216,38.6309347754804,29.4176002205149));
#40473=CARTESIAN_POINT('Ctrl Pts',(128.156990257709,38.6456193012738,29.4160055118118));
#40474=CARTESIAN_POINT('Ctrl Pts',(128.263076081415,38.6992500263856,29.4101813275454));
#40475=CARTESIAN_POINT('Ctrl Pts',(128.371675713506,38.7483327447696,29.4043571432789));
#40476=CARTESIAN_POINT('Ctrl Pts',(128.482362553069,38.7926246294185,29.3985329590124));
#40477=CARTESIAN_POINT('Ctrl Pts',(128.592909718891,38.8368606229313,29.3927161241797));
#40478=CARTESIAN_POINT('Ctrl Pts',(128.70553847789,38.8763176567245,29.3868992893471));
#40479=CARTESIAN_POINT('Ctrl Pts',(128.819798047079,38.9107989401556,29.3810824545145));
#40480=CARTESIAN_POINT('Ctrl Pts',(128.933943197743,38.9452456943333,29.375271444609));
#40481=CARTESIAN_POINT('Ctrl Pts',(129.049715521187,38.9747264933347,29.3694604347034));
#40482=CARTESIAN_POINT('Ctrl Pts',(129.166645246435,38.9990930040086,29.3636494247979));
#40483=CARTESIAN_POINT('Ctrl Pts',(129.287984334121,39.0243783638176,29.3576192845665));
#40484=CARTESIAN_POINT('Ctrl Pts',(129.41056941624,39.0441559609298,29.3515891443351));
#40485=CARTESIAN_POINT('Ctrl Pts',(129.533858961883,39.058317081326,29.3455590041036));
#40486=CARTESIAN_POINT('Ctrl Pts',(129.65253432744,39.0719482138845,29.3397545452373));
#40487=CARTESIAN_POINT('Ctrl Pts',(129.771861932216,39.0803756644309,29.3339500863711));
#40488=CARTESIAN_POINT('Ctrl Pts',(129.891350147677,39.0835548495876,29.3281456275048));
#40489=CARTESIAN_POINT('Ctrl Pts',(130.010820609899,39.0867335623894,29.3223420310495));
#40490=CARTESIAN_POINT('Ctrl Pts',(130.130451227362,39.084665549682,29.3165384345942));
#40491=CARTESIAN_POINT('Ctrl Pts',(130.249748250667,39.0773583128404,29.3107348381389));
#40492=CARTESIAN_POINT('Ctrl Pts',(130.369055686952,39.0700504381781,29.3049307351099));
#40493=CARTESIAN_POINT('Ctrl Pts',(130.488029063686,39.0575024550998,29.2991266320808));
#40494=CARTESIAN_POINT('Ctrl Pts',(130.6061782799,39.0397738665644,29.2933225290518));
#40495=CARTESIAN_POINT('Ctrl Pts',(130.72436567581,39.0220395490693,29.287516550438));
#40496=CARTESIAN_POINT('Ctrl Pts',(130.84172797802,38.9991213572441,29.2817105718241));
#40497=CARTESIAN_POINT('Ctrl Pts',(130.957784456089,38.9711300577636,29.2759045932102));
#40498=CARTESIAN_POINT('Ctrl Pts',(131.073969195103,38.9431078234264,29.2700921980626));
#40499=CARTESIAN_POINT('Ctrl Pts',(131.188844832233,38.910001385947,29.264279802915));
#40500=CARTESIAN_POINT('Ctrl Pts',(131.301944849458,38.8719716694431,29.2584674077674));
#40501=CARTESIAN_POINT('Ctrl Pts',(131.415119015703,38.8339170204391,29.2526512019802));
#40502=CARTESIAN_POINT('Ctrl Pts',(131.526514863675,38.7909328108809,29.2468349961931));
#40503=CARTESIAN_POINT('Ctrl Pts',(131.635686482147,38.7432278493461,29.2410187904059));
#40504=CARTESIAN_POINT('Ctrl Pts',(131.745014202512,38.6954546756252,29.2351942681649));
#40505=CARTESIAN_POINT('Ctrl Pts',(131.852110980245,38.6429474561582,29.2293697459239));
#40506=CARTESIAN_POINT('Ctrl Pts',(131.956555965445,38.5859606459191,29.2235452236829));
#40507=CARTESIAN_POINT('Ctrl Pts',(131.984166159126,38.5708960943285,29.2220055022031));
#40508=CARTESIAN_POINT('Ctrl Pts',(132.011591202502,38.5555187329759,29.2204657807233));
#40509=CARTESIAN_POINT('Ctrl Pts',(132.038823681523,38.5398337525458,29.2189260592435));
#40510=CARTESIAN_POINT('Ctrl Pts',(132.141833725687,38.4805034754318,29.2131018822557));
#40511=CARTESIAN_POINT('Ctrl Pts',(132.242417367041,38.4165776982603,29.2072777052679));
#40512=CARTESIAN_POINT('Ctrl Pts',(132.34013773286,38.3482802139672,29.2014535282802));
#40513=CARTESIAN_POINT('Ctrl Pts',(132.389906217135,38.3134966532983,29.1984873046235));
#40514=CARTESIAN_POINT('Ctrl Pts',(132.438932345851,38.2775799219866,29.1955210809668));
#40515=CARTESIAN_POINT('Ctrl Pts',(132.487160689988,38.2405642567579,29.1925548573102));
#40516=CARTESIAN_POINT('Origin',(130.,35.,23.));
#40517=CARTESIAN_POINT('',(126.821241978387,36.1772436037332,17.9148965215314));
#40518=CARTESIAN_POINT('',(126.821241918358,36.1772434416438,17.5703600964394));
#40519=CARTESIAN_POINT('',(126.821241918358,36.1772434416438,23.));
#40520=CARTESIAN_POINT('',(133.378768828602,34.7273715616999,17.));
#40521=CARTESIAN_POINT('Ctrl Pts',(126.821241918358,36.1772434416438,17.5703600964394));
#40522=CARTESIAN_POINT('Ctrl Pts',(126.857212034457,36.2743688901323,17.564266760725));
#40523=CARTESIAN_POINT('Ctrl Pts',(126.897684533608,36.3699708793764,17.5581734250105));
#40524=CARTESIAN_POINT('Ctrl Pts',(126.942506728596,36.463605123598,17.5520800892961));
#40525=CARTESIAN_POINT('Ctrl Pts',(126.987285374674,36.5571483934848,17.5459926738213));
#40526=CARTESIAN_POINT('Ctrl Pts',(127.036405128703,36.6487273364925,17.5399052583465));
#40527=CARTESIAN_POINT('Ctrl Pts',(127.089664831134,36.737916645688,17.5338178428716));
#40528=CARTESIAN_POINT('Ctrl Pts',(127.142890869842,36.827049581227,17.5277342750538));
#40529=CARTESIAN_POINT('Ctrl Pts',(127.200251435528,36.9137955199106,17.521650707236));
#40530=CARTESIAN_POINT('Ctrl Pts',(127.261499337811,36.9977535347711,17.5155671394182));
#40531=CARTESIAN_POINT('Ctrl Pts',(127.322727742955,37.0816848231479,17.5094855081918));
#40532=CARTESIAN_POINT('Ctrl Pts',(127.387840773444,37.162829606467,17.5034038769654));
#40533=CARTESIAN_POINT('Ctrl Pts',(127.456548273972,37.240816453855,17.4973222457391));
#40534=CARTESIAN_POINT('Ctrl Pts',(127.525251681103,37.3187986550072,17.4912409768391));
#40535=CARTESIAN_POINT('Ctrl Pts',(127.597548849614,37.3936229736636,17.4851597079391));
#40536=CARTESIAN_POINT('Ctrl Pts',(127.673110352901,37.4649522576963,17.4790784390392));
#40537=CARTESIAN_POINT('Ctrl Pts',(127.748686906051,37.5362957486466,17.4729959589104));
#40538=CARTESIAN_POINT('Ctrl Pts',(127.827528775038,37.6041425282067,17.4669134787816));
#40539=CARTESIAN_POINT('Ctrl Pts',(127.909271498311,37.6681940324353,17.4608309986528));
#40540=CARTESIAN_POINT('Ctrl Pts',(127.99110242648,37.732314651762,17.4547419551932));
#40541=CARTESIAN_POINT('Ctrl Pts',(128.075840121827,37.7926315545442,17.4486529117336));
#40542=CARTESIAN_POINT('Ctrl Pts',(128.163089061849,37.8488880756887,17.442563868274));
#40543=CARTESIAN_POINT('Ctrl Pts',(128.250388792041,37.9051773454059,17.4364712802034));
#40544=CARTESIAN_POINT('Ctrl Pts',(128.34020230886,37.9574013112638,17.4303786921328));
#40545=CARTESIAN_POINT('Ctrl Pts',(128.432109016913,38.0053490525485,17.4242861040622));
#40546=CARTESIAN_POINT('Ctrl Pts',(128.524163516949,38.0533738969294,17.4181837187125));
#40547=CARTESIAN_POINT('Ctrl Pts',(128.618317543001,38.0971086033436,17.4120813333628));
#40548=CARTESIAN_POINT('Ctrl Pts',(128.714129913534,38.1363901516284,17.4059789480131));
#40549=CARTESIAN_POINT('Ctrl Pts',(128.775991314876,38.1617523424422,17.402038933721));
#40550=CARTESIAN_POINT('Ctrl Pts',(128.838543662247,38.1852591658188,17.3980989194289));
#40551=CARTESIAN_POINT('Ctrl Pts',(128.901665328744,38.2068779229052,17.3941589051368));
#40552=CARTESIAN_POINT('Ctrl Pts',(128.998656487735,38.2400967591959,17.3881047786563));
#40553=CARTESIAN_POINT('Ctrl Pts',(129.097334659593,38.2689724799459,17.3820506521758));
#40554=CARTESIAN_POINT('Ctrl Pts',(129.197271488593,38.2933314439143,17.3759965256953));
#40555=CARTESIAN_POINT('Ctrl Pts',(129.297075621052,38.317658063948,17.3699504379094));
#40556=CARTESIAN_POINT('Ctrl Pts',(129.398134670601,38.3374797432278,17.3639043501235));
#40557=CARTESIAN_POINT('Ctrl Pts',(129.50000249191,38.3526717039406,17.3578582623376));
#40558=CARTESIAN_POINT('Ctrl Pts',(129.601765401025,38.367848018673,17.3518184013299));
#40559=CARTESIAN_POINT('Ctrl Pts',(129.704334998244,38.3784040286015,17.3457785403222));
#40560=CARTESIAN_POINT('Ctrl Pts',(129.807253184598,38.3842656112741,17.3397386793146));
#40561=CARTESIAN_POINT('Ctrl Pts',(129.910101948709,38.3901232400856,17.3337028924236));
#40562=CARTESIAN_POINT('Ctrl Pts',(130.013298401426,38.3912927099096,17.3276671055327));
#40563=CARTESIAN_POINT('Ctrl Pts',(130.116378419083,38.3877516328786,17.3216313186417));
#40564=CARTESIAN_POINT('Ctrl Pts',(130.219422807154,38.3842117798201,17.3155976180191));
#40565=CARTESIAN_POINT('Ctrl Pts',(130.322350405517,38.3759646290582,17.3095639173966));
#40566=CARTESIAN_POINT('Ctrl Pts',(130.424697118526,38.363039907586,17.303530216774));
#40567=CARTESIAN_POINT('Ctrl Pts',(130.527036045825,38.350116169322,17.2974969751465));
#40568=CARTESIAN_POINT('Ctrl Pts',(130.628793743683,38.3325156220224,17.2914637335191));
#40569=CARTESIAN_POINT('Ctrl Pts',(130.729512283087,38.3103197566588,17.2854304918916));
#40570=CARTESIAN_POINT('Ctrl Pts',(130.830250313128,38.2881195960425,17.2793960827361));
#40571=CARTESIAN_POINT('Ctrl Pts',(130.929948360132,38.2613224445899,17.2733616735805));
#40572=CARTESIAN_POINT('Ctrl Pts',(131.028160713027,38.2300604654848,17.267327264425));
#40573=CARTESIAN_POINT('Ctrl Pts',(131.126487251052,38.1987621401049,17.2612858394534));
#40574=CARTESIAN_POINT('Ctrl Pts',(131.223324230169,38.1629887538537,17.2552444144819));
#40575=CARTESIAN_POINT('Ctrl Pts',(131.318243140881,38.1229217223651,17.2492029895103));
#40576=CARTESIAN_POINT('Ctrl Pts',(131.413218328448,38.082830935373,17.243157982614));
#40577=CARTESIAN_POINT('Ctrl Pts',(131.506272791327,38.0384416233783,17.2371129757177));
#40578=CARTESIAN_POINT('Ctrl Pts',(131.597001957699,37.9899815734557,17.2310679688214));
#40579=CARTESIAN_POINT('Ctrl Pts',(131.687895393117,37.9414337845353,17.2250120171809));
#40580=CARTESIAN_POINT('Ctrl Pts',(131.776454748566,37.8888007586748,17.2189560655405));
#40581=CARTESIAN_POINT('Ctrl Pts',(131.862303584688,37.8323542188361,17.2129001139001));
#40582=CARTESIAN_POINT('Ctrl Pts',(131.937061191894,37.7832002821719,17.2076265601229));
#40583=CARTESIAN_POINT('Ctrl Pts',(132.009763752858,37.731155332992,17.2023530063457));
#40584=CARTESIAN_POINT('Ctrl Pts',(132.08018436874,37.6764226225598,17.1970794525685));
#40585=CARTESIAN_POINT('Ctrl Pts',(132.163723907917,37.6114935481666,17.1908234684812));
#40586=CARTESIAN_POINT('Ctrl Pts',(132.244339475961,37.5425575647275,17.184567484394));
#40587=CARTESIAN_POINT('Ctrl Pts',(132.32163556536,37.4699014887554,17.1783115003068));
#40588=CARTESIAN_POINT('Ctrl Pts',(132.398818569831,37.397351709326,17.1720646687848));
#40589=CARTESIAN_POINT('Ctrl Pts',(132.472691470397,37.3210929417983,17.1658178372629));
#40590=CARTESIAN_POINT('Ctrl Pts',(132.542890861188,37.2414529061721,17.159571005741));
#40591=CARTESIAN_POINT('Ctrl Pts',(132.613003795704,37.161910953744,17.1533318677014));
#40592=CARTESIAN_POINT('Ctrl Pts',(132.679451961912,37.0789963218649,17.1470927296619));
#40593=CARTESIAN_POINT('Ctrl Pts',(132.741908352732,36.9930739192816,17.1408535916224));
#40594=CARTESIAN_POINT('Ctrl Pts',(132.804291895857,36.9072517346084,17.1346217307697));
#40595=CARTESIAN_POINT('Ctrl Pts',(132.862692703684,36.8184290914577,17.128389869917));
#40596=CARTESIAN_POINT('Ctrl Pts',(132.91682416608,36.7270037193567,17.1221580090643));
#40597=CARTESIAN_POINT('Ctrl Pts',(132.970918848672,36.6356404665325,17.1159303824704));
#40598=CARTESIAN_POINT('Ctrl Pts',(133.020749755062,36.5416783486704,17.1097027558765));
#40599=CARTESIAN_POINT('Ctrl Pts',(133.066073812794,36.4455436475593,17.1034751292826));
#40600=CARTESIAN_POINT('Ctrl Pts',(133.111376567789,36.3494541306691,17.0972504297323));
#40601=CARTESIAN_POINT('Ctrl Pts',(133.152176520114,36.2511944258449,17.091025730182));
#40602=CARTESIAN_POINT('Ctrl Pts',(133.188277021192,36.1512144451147,17.0848010306316));
#40603=CARTESIAN_POINT('Ctrl Pts',(133.224368111105,36.0512605285103,17.0785779538197));
#40604=CARTESIAN_POINT('Ctrl Pts',(133.255762053786,35.9495876065114,17.0723548770077));
#40605=CARTESIAN_POINT('Ctrl Pts',(133.28231094227,35.846664007002,17.0661318001958));
#40606=CARTESIAN_POINT('Ctrl Pts',(133.308865996869,35.7437165029613,17.0599072780425));
#40607=CARTESIAN_POINT('Ctrl Pts',(133.3305736438,35.6395181286387,17.0536827558892));
#40608=CARTESIAN_POINT('Ctrl Pts',(133.347336361986,35.5345505983788,17.0474582337359));
#40609=CARTESIAN_POINT('Ctrl Pts',(133.364100783892,35.4295723994877,17.041233078938));
#40610=CARTESIAN_POINT('Ctrl Pts',(133.375919219294,35.323825286508,17.0350079241402));
#40611=CARTESIAN_POINT('Ctrl Pts',(133.38274577431,35.2177982756766,17.0287827693424));
#40612=CARTESIAN_POINT('Ctrl Pts',(133.389577148137,35.1116964212249,17.0225532202575));
#40613=CARTESIAN_POINT('Ctrl Pts',(133.391409583697,35.00531467558,17.0163236711726));
#40614=CARTESIAN_POINT('Ctrl Pts',(133.3882492794,34.8991442458638,17.0100941220878));
#40615=CARTESIAN_POINT('Ctrl Pts',(133.386542334164,34.8417994169385,17.0067294147252));
#40616=CARTESIAN_POINT('Ctrl Pts',(133.383379756271,34.7845162190167,17.0033647073626));
#40617=CARTESIAN_POINT('Ctrl Pts',(133.378768828602,34.7273715616999,17.));
#40618=CARTESIAN_POINT('',(126.821241918358,36.1772434416438,17.));
#40619=CARTESIAN_POINT('Origin',(130.,35.,17.));
#40620=CARTESIAN_POINT('',(126.821241918358,36.1772434416438,16.));
#40621=CARTESIAN_POINT('',(126.821241918358,36.1772434416438,23.));
#40622=CARTESIAN_POINT('Origin',(130.,35.,16.));
#40623=CARTESIAN_POINT('',(129.213982665103,31.6996256275318,16.9983013856386));
#40624=CARTESIAN_POINT('Origin',(130.,35.,17.));
#40625=CARTESIAN_POINT('Ctrl Pts',(129.214786777099,31.7024485967492,16.9966190365833));
#40626=CARTESIAN_POINT('Ctrl Pts',(129.256053829841,31.6926220826116,16.9991917406743));
#40627=CARTESIAN_POINT('Ctrl Pts',(129.297500078023,31.6835714753038,17.0018012218908));
#40628=CARTESIAN_POINT('Ctrl Pts',(129.548086858706,31.6337588604023,17.0176889557332));
#40629=CARTESIAN_POINT('Ctrl Pts',(129.760512272923,31.6120146819001,17.0315845883753));
#40630=CARTESIAN_POINT('Ctrl Pts',(130.135243116705,31.6090921467174,17.0556509826498));
#40631=CARTESIAN_POINT('Ctrl Pts',(130.29681991899,31.6194001831478,17.0658890691968));
#40632=CARTESIAN_POINT('Ctrl Pts',(130.520207798137,31.6497984413332,17.0797091662821));
#40633=CARTESIAN_POINT('Ctrl Pts',(130.583104281854,31.6601711351688,17.0835647414702));
#40634=CARTESIAN_POINT('Ctrl Pts',(130.677489035867,31.6784846893831,17.0892993156514));
#40635=CARTESIAN_POINT('Ctrl Pts',(130.709214482815,31.6851138363018,17.0912181161196));
#40636=CARTESIAN_POINT('Ctrl Pts',(130.764319284931,31.6974555291198,17.0945368170202));
#40637=CARTESIAN_POINT('Ctrl Pts',(130.787741520862,31.702963862566,17.0959429544309));
#40638=CARTESIAN_POINT('Ctrl Pts',(130.840719066106,31.7160196622147,17.0991141296805));
#40639=CARTESIAN_POINT('Ctrl Pts',(130.870235354469,31.7237176676327,17.1008743302695));
#40640=CARTESIAN_POINT('Ctrl Pts',(130.950332475085,31.7457662628929,17.1056355540019));
#40641=CARTESIAN_POINT('Ctrl Pts',(131.000690775141,31.7608971289618,17.1086120847421));
#40642=CARTESIAN_POINT('Ctrl Pts',(131.238908929887,31.8385594907758,17.1226431799184));
#40643=CARTESIAN_POINT('Ctrl Pts',(131.421406384604,31.9162985684089,17.133216313784));
#40644=CARTESIAN_POINT('Ctrl Pts',(131.725430740833,32.0785638487485,17.1515544639106));
#40645=CARTESIAN_POINT('Ctrl Pts',(131.850152450992,32.1559128162313,17.159325683362));
#40646=CARTESIAN_POINT('Ctrl Pts',(132.030118336166,32.2843826609484,17.1714595483403));
#40647=CARTESIAN_POINT('Ctrl Pts',(132.089320185824,32.329663387505,17.1756172476579));
#40648=CARTESIAN_POINT('Ctrl Pts',(132.165497339867,32.3920124481424,17.1812605520124));
#40649=CARTESIAN_POINT('Ctrl Pts',(132.183855379003,32.4073655454486,17.1826440849071));
#40650=CARTESIAN_POINT('Ctrl Pts',(132.214046292267,32.433162819123,17.1849617166224));
#40651=CARTESIAN_POINT('Ctrl Pts',(132.225971876318,32.4434978415772,17.1858883880591));
#40652=CARTESIAN_POINT('Ctrl Pts',(132.248662271818,32.4634410634607,17.1876740525311));
#40653=CARTESIAN_POINT('Ctrl Pts',(132.259438741034,32.4730354553383,17.1885320010811));
#40654=CARTESIAN_POINT('Ctrl Pts',(132.289089160876,32.4997748000613,17.1909192311729));
#40655=CARTESIAN_POINT('Ctrl Pts',(132.30783102106,32.5170640099366,17.1924584541783));
#40656=CARTESIAN_POINT('Ctrl Pts',(132.388244092172,32.5929414102011,17.1991883157391));
#40657=CARTESIAN_POINT('Ctrl Pts',(132.447888831647,32.6536242931822,17.2045056416654));
#40658=CARTESIAN_POINT('Ctrl Pts',(132.638301290146,32.8625203523798,17.2224225312086));
#40659=CARTESIAN_POINT('Ctrl Pts',(132.758393696422,33.0199194313757,17.2352902026146));
#40660=CARTESIAN_POINT('Ctrl Pts',(132.921444906087,33.2774837773379,17.254725338315));
#40661=CARTESIAN_POINT('Ctrl Pts',(132.974470512632,33.3707576341683,17.2614776983359));
#40662=CARTESIAN_POINT('Ctrl Pts',(133.056883876579,33.5332079471359,17.2727195785379));
#40663=CARTESIAN_POINT('Ctrl Pts',(133.088556623231,33.6011300106074,17.2772753840721));
#40664=CARTESIAN_POINT('Ctrl Pts',(133.131415650891,33.7016093502931,17.2838090485015));
#40665=CARTESIAN_POINT('Ctrl Pts',(133.144397524753,33.7333719593913,17.2858453465296));
#40666=CARTESIAN_POINT('Ctrl Pts',(133.166618610394,33.7901883355841,17.2894377257179));
#40667=CARTESIAN_POINT('Ctrl Pts',(133.176048108349,33.8151640785858,17.2909999390836));
#40668=CARTESIAN_POINT('Ctrl Pts',(133.195419414843,33.8683661369843,17.2942929285406));
#40669=CARTESIAN_POINT('Ctrl Pts',(133.205284517565,33.8966180713018,17.2960211040488));
#40670=CARTESIAN_POINT('Ctrl Pts',(133.231105658644,33.9738357080404,17.3006914072849));
#40671=CARTESIAN_POINT('Ctrl Pts',(133.246322378529,34.0230412821123,17.3036098254026));
#40672=CARTESIAN_POINT('Ctrl Pts',(133.32887334135,34.3132540723406,17.3205224061402));
#40673=CARTESIAN_POINT('Ctrl Pts',(133.370475705977,34.5607707380538,17.3336730298819));
#40674=CARTESIAN_POINT('Ctrl Pts',(133.3910920424,34.9292245629098,17.3532786977632));
#40675=CARTESIAN_POINT('Ctrl Pts',(133.391489250819,35.0480822365796,17.3596215874846));
#40676=CARTESIAN_POINT('Ctrl Pts',(133.382391868143,35.2328396975454,17.3698126049527));
#40677=CARTESIAN_POINT('Ctrl Pts',(133.377198846605,35.2988576339488,17.3735208978539));
#40678=CARTESIAN_POINT('Ctrl Pts',(133.367621652711,35.3873630947391,17.3786313817447));
#40679=CARTESIAN_POINT('Ctrl Pts',(133.364937805755,35.4100234940586,17.3799521708365));
#40680=CARTESIAN_POINT('Ctrl Pts',(133.360059674416,35.4479299655111,17.3821848132151));
#40681=CARTESIAN_POINT('Ctrl Pts',(133.357989823929,35.4631917550789,17.3830900428655));
#40682=CARTESIAN_POINT('Ctrl Pts',(133.353490979985,35.4947470832102,17.3849757365669));
#40683=CARTESIAN_POINT('Ctrl Pts',(133.351047108622,35.5110378458802,17.3859569407812));
#40684=CARTESIAN_POINT('Ctrl Pts',(133.344091127534,35.5552092178813,17.3886371281077));
#40685=CARTESIAN_POINT('Ctrl Pts',(133.339349241684,35.5830516901481,17.3903478967372));
#40686=CARTESIAN_POINT('Ctrl Pts',(133.307519271215,35.7567977261702,17.4011439813479));
#40687=CARTESIAN_POINT('Ctrl Pts',(133.271224299842,35.9008385191964,17.4106199888271));
#40688=CARTESIAN_POINT('Ctrl Pts',(133.149206735442,36.2785475651372,17.4361683743766));
#40689=CARTESIAN_POINT('Ctrl Pts',(133.047002676611,36.5059859337552,17.4522420755618));
#40690=CARTESIAN_POINT('Ctrl Pts',(132.886706005581,36.7781607319369,17.4716546143215));
#40691=CARTESIAN_POINT('Ctrl Pts',(132.850861697118,36.8350792068487,17.4757307172299));
#40692=CARTESIAN_POINT('Ctrl Pts',(132.795064660788,36.918096088445,17.4817027646984));
#40693=CARTESIAN_POINT('Ctrl Pts',(132.776389620987,36.9450295238551,17.483644769349));
#40694=CARTESIAN_POINT('Ctrl Pts',(132.742022944406,36.9930899243442,17.4871194115867));
#40695=CARTESIAN_POINT('Ctrl Pts',(132.726470514619,37.0143127525817,17.4886571324941));
#40696=CARTESIAN_POINT('Ctrl Pts',(132.692444659841,37.0596282080693,17.4919488491056));
#40697=CARTESIAN_POINT('Ctrl Pts',(132.673891398734,37.0836581956447,17.49369958371));
#40698=CARTESIAN_POINT('Ctrl Pts',(132.621997465262,37.1490358758255,17.4984797980984));
#40699=CARTESIAN_POINT('Ctrl Pts',(132.58800326071,37.1898551219723,17.501483430422));
#40700=CARTESIAN_POINT('Ctrl Pts',(132.434371431055,37.3657547803364,17.5145418678149));
#40701=CARTESIAN_POINT('Ctrl Pts',(132.305015769537,37.4919612267376,17.5241999022469));
#40702=CARTESIAN_POINT('Ctrl Pts',(132.037011113224,37.714628667599,17.5426817072915));
#40703=CARTESIAN_POINT('Ctrl Pts',(131.900011104562,37.8122188774766,17.5514967832702));
#40704=CARTESIAN_POINT('Ctrl Pts',(131.70981897151,37.9274364229952,17.5636359301029));
#40705=CARTESIAN_POINT('Ctrl Pts',(131.662616984004,37.9544998130361,17.5666422126796));
#40706=CARTESIAN_POINT('Ctrl Pts',(131.580493160447,37.9989944457297,17.5718963707584));
#40707=CARTESIAN_POINT('Ctrl Pts',(131.545883218952,38.0169804634852,17.5741176902827));
#40708=CARTESIAN_POINT('Ctrl Pts',(131.494308721456,38.0426621619099,17.5774493246284));
#40709=CARTESIAN_POINT('Ctrl Pts',(131.477577550123,38.0508222064118,17.5785334219615));
#40710=CARTESIAN_POINT('Ctrl Pts',(131.447365767591,38.0652501352356,17.5804983809761));
#40711=CARTESIAN_POINT('Ctrl Pts',(131.433909895837,38.0715677502068,17.5813762555213));
#40712=CARTESIAN_POINT('Ctrl Pts',(131.403191513728,38.0857443797491,17.5833864630216));
#40713=CARTESIAN_POINT('Ctrl Pts',(131.385904250794,38.0935471827659,17.5845219643156));
#40714=CARTESIAN_POINT('Ctrl Pts',(131.331448069326,38.1175785448481,17.5881099995059));
#40715=CARTESIAN_POINT('Ctrl Pts',(131.294054099791,38.1332847973099,17.5905899529291));
#40716=CARTESIAN_POINT('Ctrl Pts',(131.056162769399,38.2282194003898,17.6064281276034));
#40717=CARTESIAN_POINT('Ctrl Pts',(130.848781323682,38.2888360148737,17.6204724988471));
#40718=CARTESIAN_POINT('Ctrl Pts',(130.440745680061,38.3669123578759,17.6471661438228));
#40719=CARTESIAN_POINT('Ctrl Pts',(130.241469432651,38.387044316396,17.6597903817292));
#40720=CARTESIAN_POINT('Ctrl Pts',(129.996506531816,38.3900475755061,17.6746051661624));
#40721=CARTESIAN_POINT('Ctrl Pts',(129.951449604967,38.3897017450249,17.6773027627754));
#40722=CARTESIAN_POINT('Ctrl Pts',(129.877902889586,38.3876703951481,17.6816632465928));
#40723=CARTESIAN_POINT('Ctrl Pts',(129.849404953391,38.386523234332,17.6833423620265));
#40724=CARTESIAN_POINT('Ctrl Pts',(129.793967616118,38.3835904615584,17.6865893445222));
#40725=CARTESIAN_POINT('Ctrl Pts',(129.767028459358,38.3818424087642,17.6881582385486));
#40726=CARTESIAN_POINT('Ctrl Pts',(129.703132675972,38.3769291443102,17.6918595795546));
#40727=CARTESIAN_POINT('Ctrl Pts',(129.666201066581,38.3734787799783,17.6939831299917));
#40728=CARTESIAN_POINT('Ctrl Pts',(129.54189455585,38.3598039193035,17.7010839038258));
#40729=CARTESIAN_POINT('Ctrl Pts',(129.454860058891,38.3467845966391,17.7059763365416));
#40730=CARTESIAN_POINT('Ctrl Pts',(129.10221998013,38.2799100549687,17.7256263531402));
#40731=CARTESIAN_POINT('Ctrl Pts',(128.843045855803,38.1976971015985,17.739581742613));
#40732=CARTESIAN_POINT('Ctrl Pts',(128.536169929559,38.0581022270475,17.7578433972716));
#40733=CARTESIAN_POINT('Ctrl Pts',(128.476728958214,38.0289325129175,17.761473224389));
#40734=CARTESIAN_POINT('Ctrl Pts',(128.378398813746,37.9770519101292,17.7676955224079));
#40735=CARTESIAN_POINT('Ctrl Pts',(128.33903808698,37.9552721714332,17.7702470670211));
#40736=CARTESIAN_POINT('Ctrl Pts',(128.283021334896,37.9228034683209,17.7739834723889));
#40737=CARTESIAN_POINT('Ctrl Pts',(128.26600578852,37.9127409573522,17.77513270959));
#40738=CARTESIAN_POINT('Ctrl Pts',(128.236261987666,37.8947983289512,17.7771685689308));
#40739=CARTESIAN_POINT('Ctrl Pts',(128.223496403707,37.8869818326433,17.7780512402675));
#40740=CARTESIAN_POINT('Ctrl Pts',(128.195387142569,37.8695132089198,17.7800150093219));
#40741=CARTESIAN_POINT('Ctrl Pts',(128.180069046386,37.8598225317122,17.781098428686));
#40742=CARTESIAN_POINT('Ctrl Pts',(128.13452235746,37.8304942363568,17.7843579676676));
#40743=CARTESIAN_POINT('Ctrl Pts',(128.104529426571,37.8104973827608,17.7865550862689));
#40744=CARTESIAN_POINT('Ctrl Pts',(127.950110117423,37.7039470079332,17.7981104116921));
#40745=CARTESIAN_POINT('Ctrl Pts',(127.831281128646,37.6096032713602,17.8078309064383));
#40746=CARTESIAN_POINT('Ctrl Pts',(127.620279360132,37.41768599197,17.8262053149537));
#40747=CARTESIAN_POINT('Ctrl Pts',(127.526789265926,37.3219619234952,17.8348348817654));
#40748=CARTESIAN_POINT('Ctrl Pts',(127.345742658711,37.1132124023311,17.8523761566041));
#40749=CARTESIAN_POINT('Ctrl Pts',(127.259176362926,36.9996606608383,17.861249438756));
#40750=CARTESIAN_POINT('Ctrl Pts',(127.156629279089,36.8459208960606,17.8723961566983));
#40751=CARTESIAN_POINT('Ctrl Pts',(127.133899662632,36.8104281557498,17.8749143843333));
#40752=CARTESIAN_POINT('Ctrl Pts',(127.097225695315,36.7507385372235,17.8790605106294));
#40753=CARTESIAN_POINT('Ctrl Pts',(127.082908338469,36.7267774603061,17.8807017188277));
#40754=CARTESIAN_POINT('Ctrl Pts',(127.055322243062,36.6792877698506,17.8839102545656));
#40755=CARTESIAN_POINT('Ctrl Pts',(127.042035574973,36.6557720338785,17.8854781361535));
#40756=CARTESIAN_POINT('Ctrl Pts',(127.013288075251,36.6034419352456,17.888922594587));
#40757=CARTESIAN_POINT('Ctrl Pts',(126.997960158449,36.5745574159066,17.8907944549291));
#40758=CARTESIAN_POINT('Ctrl Pts',(126.945863854365,36.4728580197233,17.8972879241734));
#40759=CARTESIAN_POINT('Ctrl Pts',(126.911306278239,36.3989391827768,17.9018351064256));
#40760=CARTESIAN_POINT('Ctrl Pts',(126.858898761487,36.2754044254345,17.9092032564979));
#40761=CARTESIAN_POINT('Ctrl Pts',(126.839493178286,36.2265249486466,17.9120613358438));
#40762=CARTESIAN_POINT('Ctrl Pts',(126.821241978387,36.177243603733,17.9148965215314));
#40763=CARTESIAN_POINT('Origin',(130.,35.,23.));
#40764=CARTESIAN_POINT('',(126.821241918361,36.1772434416541,19.1602707349979));
#40765=CARTESIAN_POINT('',(126.821241895921,36.1772433810614,18.8206074156906));
#40766=CARTESIAN_POINT('',(126.821241918358,36.1772434416438,23.));
#40767=CARTESIAN_POINT('',(126.610251067793,35.0026905576773,17.6410178032139));
#40768=CARTESIAN_POINT('Ctrl Pts',(126.821241895921,36.1772433810614,18.8206074156907));
#40769=CARTESIAN_POINT('Ctrl Pts',(126.87248024585,36.315595673116,18.8127842064404));
#40770=CARTESIAN_POINT('Ctrl Pts',(126.932707594695,36.450485456493,18.8049940225583));
#40771=CARTESIAN_POINT('Ctrl Pts',(127.037872295089,36.64992988607,18.7926712384784));
#40772=CARTESIAN_POINT('Ctrl Pts',(127.076553861729,36.7175360552938,18.7883412642631));
#40773=CARTESIAN_POINT('Ctrl Pts',(127.130542646606,36.8047801705939,18.7824702309081));
#40774=CARTESIAN_POINT('Ctrl Pts',(127.143788989377,36.8256712611168,18.7810422009026));
#40775=CARTESIAN_POINT('Ctrl Pts',(127.164997599031,36.8583240058767,18.7787719917869));
#40776=CARTESIAN_POINT('Ctrl Pts',(127.172807439942,36.870184198587,18.7779393462207));
#40777=CARTESIAN_POINT('Ctrl Pts',(127.189337259138,36.8949465745617,18.7761831728303));
#40778=CARTESIAN_POINT('Ctrl Pts',(127.198071961823,36.9078382534364,18.7752586153802));
#40779=CARTESIAN_POINT('Ctrl Pts',(127.220391954919,36.940296781993,18.7729055925757));
#40780=CARTESIAN_POINT('Ctrl Pts',(127.234095108078,36.9597812493265,18.7714697071747));
#40781=CARTESIAN_POINT('Ctrl Pts',(127.292177676172,37.0405460258041,18.7654248830377));
#40782=CARTESIAN_POINT('Ctrl Pts',(127.338394516333,37.1004724244658,18.7607137757227));
#40783=CARTESIAN_POINT('Ctrl Pts',(127.482317041684,37.274704071611,18.7464417876623));
#40784=CARTESIAN_POINT('Ctrl Pts',(127.585661973826,37.3841089498847,18.7367066242889));
#40785=CARTESIAN_POINT('Ctrl Pts',(127.843966419205,37.6234829787011,18.7140370578109));
#40786=CARTESIAN_POINT('Ctrl Pts',(128.003984501788,37.747196078182,18.7012121749373));
#40787=CARTESIAN_POINT('Ctrl Pts',(128.218745600126,37.8845013835324,18.6856911020411));
#40788=CARTESIAN_POINT('Ctrl Pts',(128.2640760315,37.9120068540927,18.6824995257721));
#40789=CARTESIAN_POINT('Ctrl Pts',(128.336414869096,37.953610612944,18.6775354148027));
#40790=CARTESIAN_POINT('Ctrl Pts',(128.362998474652,37.9684267275989,18.6757377687823));
#40791=CARTESIAN_POINT('Ctrl Pts',(128.413061686458,37.9954518727168,18.6724006678971));
#40792=CARTESIAN_POINT('Ctrl Pts',(128.436491538058,38.0077477422027,18.6708582659369));
#40793=CARTESIAN_POINT('Ctrl Pts',(128.489529580288,38.034794592065,18.6674089100431));
#40794=CARTESIAN_POINT('Ctrl Pts',(128.519214766559,38.0493891695994,18.6655074397703));
#40795=CARTESIAN_POINT('Ctrl Pts',(128.610903412516,38.092812745173,18.6597190466952));
#40796=CARTESIAN_POINT('Ctrl Pts',(128.673571107819,38.1202030814715,18.6558802750143));
#40797=CARTESIAN_POINT('Ctrl Pts',(128.824331379956,38.1807324572684,18.64688316939));
#40798=CARTESIAN_POINT('Ctrl Pts',(128.913060165231,38.212136213326,18.6417758581226));
#40799=CARTESIAN_POINT('Ctrl Pts',(129.210781287315,38.3037565930303,18.6250582816421));
#40800=CARTESIAN_POINT('Ctrl Pts',(129.424236175831,38.3475605703756,18.6137674282016));
#40801=CARTESIAN_POINT('Ctrl Pts',(129.728487297146,38.3800196392524,18.5971371931572));
#40802=CARTESIAN_POINT('Ctrl Pts',(129.816897734108,38.3859596899436,18.59223721716));
#40803=CARTESIAN_POINT('Ctrl Pts',(129.931167798521,38.3891488672371,18.585705185037));
#40804=CARTESIAN_POINT('Ctrl Pts',(129.956910246894,38.3895738823913,18.5842206373326));
#40805=CARTESIAN_POINT('Ctrl Pts',(129.998628598167,38.3897873635103,18.5817901210079));
#40806=CARTESIAN_POINT('Ctrl Pts',(130.014603017186,38.3897561829211,18.5808535925426));
#40807=CARTESIAN_POINT('Ctrl Pts',(130.046312262046,38.3894701472027,18.5789819174312));
#40808=CARTESIAN_POINT('Ctrl Pts',(130.062046655227,38.389218625304,18.5780469586368));
#40809=CARTESIAN_POINT('Ctrl Pts',(130.102436035239,38.3882916411268,18.5756319814212));
#40810=CARTESIAN_POINT('Ctrl Pts',(130.127086084326,38.387456632403,18.5741437579073));
#40811=CARTESIAN_POINT('Ctrl Pts',(130.236230461578,38.3825664672057,18.5674971535528));
#40812=CARTESIAN_POINT('Ctrl Pts',(130.320559300819,38.3756184991256,18.5622105756659));
#40813=CARTESIAN_POINT('Ctrl Pts',(130.590813244682,38.343134227466,18.5449549781606));
#40814=CARTESIAN_POINT('Ctrl Pts',(130.774911066735,38.3053169292088,18.5327388934676));
#40815=CARTESIAN_POINT('Ctrl Pts',(131.119295622711,38.2042043830394,18.5097818407508));
#40816=CARTESIAN_POINT('Ctrl Pts',(131.27977958601,38.1435531476361,18.4990361545404));
#40817=CARTESIAN_POINT('Ctrl Pts',(131.475320558502,38.0521818814147,18.4859895638434));
#40818=CARTESIAN_POINT('Ctrl Pts',(131.515259546502,38.0325523535024,18.4833261619053));
#40819=CARTESIAN_POINT('Ctrl Pts',(131.580009801197,37.9991296790951,18.4790086222447));
#40820=CARTESIAN_POINT('Ctrl Pts',(131.605053872544,37.9858017253813,18.4773387763856));
#40821=CARTESIAN_POINT('Ctrl Pts',(131.653591430057,37.9591838044692,18.47410165509));
#40822=CARTESIAN_POINT('Ctrl Pts',(131.677099256104,37.9459245667767,18.4725334619888));
#40823=CARTESIAN_POINT('Ctrl Pts',(131.732712118216,37.9136754975161,18.4688212471967));
#40824=CARTESIAN_POINT('Ctrl Pts',(131.764667350311,37.8944335349394,18.4666863555279));
#40825=CARTESIAN_POINT('Ctrl Pts',(131.877453359147,37.8239567092158,18.4591374887046));
#40826=CARTESIAN_POINT('Ctrl Pts',(131.956427564045,37.7698295925829,18.4538275268168));
#40827=CARTESIAN_POINT('Ctrl Pts',(132.159302616883,37.617771402432,18.439991554405));
#40828=CARTESIAN_POINT('Ctrl Pts',(132.278833958426,37.5144052792231,18.4316396574227));
#40829=CARTESIAN_POINT('Ctrl Pts',(132.523367481538,37.271128920475,18.4133518658377));
#40830=CARTESIAN_POINT('Ctrl Pts',(132.644838726892,37.1284321186654,18.4034405792336));
#40831=CARTESIAN_POINT('Ctrl Pts',(132.774104647215,36.9483194160737,18.3909149737066));
#40832=CARTESIAN_POINT('Ctrl Pts',(132.793870030508,36.9198685370061,18.3889355758593));
#40833=CARTESIAN_POINT('Ctrl Pts',(132.823265666583,36.8761401540952,18.3858839425556));
#40834=CARTESIAN_POINT('Ctrl Pts',(132.833216153357,36.8610795518944,18.3848312703753));
#40835=CARTESIAN_POINT('Ctrl Pts',(132.851183787997,36.8334065020716,18.3828926576297));
#40836=CARTESIAN_POINT('Ctrl Pts',(132.859238491519,36.8208194904161,18.3820091395464));
#40837=CARTESIAN_POINT('Ctrl Pts',(132.877759974971,36.7914501869744,18.3799437546177));
#40838=CARTESIAN_POINT('Ctrl Pts',(132.888163360505,36.7746291464406,18.378758040084));
#40839=CARTESIAN_POINT('Ctrl Pts',(132.921850621045,36.7190799866892,18.3748357670751));
#40840=CARTESIAN_POINT('Ctrl Pts',(132.94450642991,36.6799787255777,18.3720644432014));
#40841=CARTESIAN_POINT('Ctrl Pts',(132.998624479861,36.5821181130448,18.3651244156822));
#40842=CARTESIAN_POINT('Ctrl Pts',(133.029147782316,36.5228622104135,18.3609187463534));
#40843=CARTESIAN_POINT('Ctrl Pts',(133.177029559179,36.2137125720987,18.3390896502157));
#40844=CARTESIAN_POINT('Ctrl Pts',(133.265305735195,35.9510135113245,18.3210225740503));
#40845=CARTESIAN_POINT('Ctrl Pts',(133.337662414383,35.5979305862962,18.2986410848175));
#40846=CARTESIAN_POINT('Ctrl Pts',(133.351500474047,35.5147405082691,18.2934893926472));
#40847=CARTESIAN_POINT('Ctrl Pts',(133.3664294725,35.3983108026939,18.2864478760855));
#40848=CARTESIAN_POINT('Ctrl Pts',(133.370155552454,35.3654456968944,18.2844786248739));
#40849=CARTESIAN_POINT('Ctrl Pts',(133.376058769605,35.3055597069388,18.2809226777195));
#40850=CARTESIAN_POINT('Ctrl Pts',(133.378393897172,35.2785575155212,18.2793312477473));
#40851=CARTESIAN_POINT('Ctrl Pts',(133.382467060372,35.2238166823131,18.2761281486082));
#40852=CARTESIAN_POINT('Ctrl Pts',(133.384188303239,35.1960788540938,18.274517114199));
#40853=CARTESIAN_POINT('Ctrl Pts',(133.387630458186,35.1268447406939,18.2705242179988));
#40854=CARTESIAN_POINT('Ctrl Pts',(133.388930281703,35.085331514346,18.2681553830466));
#40855=CARTESIAN_POINT('Ctrl Pts',(133.39121103627,34.9088494569434,18.2581801986537));
#40856=CARTESIAN_POINT('Ctrl Pts',(133.384893898044,34.773904426956,18.2507957250303));
#40857=CARTESIAN_POINT('Ctrl Pts',(133.355829856776,34.5020268851899,18.2360960643925));
#40858=CARTESIAN_POINT('Ctrl Pts',(133.332694452756,34.3653980004879,18.2288011249671));
#40859=CARTESIAN_POINT('Ctrl Pts',(133.263075714489,34.066697281545,18.2125024725059));
#40860=CARTESIAN_POINT('Ctrl Pts',(133.212737920476,33.9059160707499,18.203491929951));
#40861=CARTESIAN_POINT('Ctrl Pts',(133.140089443307,33.7228673456335,18.1922828968995));
#40862=CARTESIAN_POINT('Ctrl Pts',(133.129159010321,33.6963154900323,18.1906324624966));
#40863=CARTESIAN_POINT('Ctrl Pts',(133.111371025662,33.6546183926077,18.187996918356));
#40864=CARTESIAN_POINT('Ctrl Pts',(133.104736852428,33.6393786784438,18.1870243375158));
#40865=CARTESIAN_POINT('Ctrl Pts',(133.091756152517,33.6101493121529,18.1851398192257));
#40866=CARTESIAN_POINT('Ctrl Pts',(133.08542617895,33.596153035037,18.1842288214532));
#40867=CARTESIAN_POINT('Ctrl Pts',(133.069542392545,33.5616585886085,18.1819630452997));
#40868=CARTESIAN_POINT('Ctrl Pts',(133.059878228435,33.5412122559957,18.1806019539656));
#40869=CARTESIAN_POINT('Ctrl Pts',(133.021778943699,33.4626506641772,18.1753064284028));
#40870=CARTESIAN_POINT('Ctrl Pts',(132.991888301063,33.4052604415645,18.1712980687489));
#40871=CARTESIAN_POINT('Ctrl Pts',(132.904593433789,33.2487560246889,18.160042703045));
#40872=CARTESIAN_POINT('Ctrl Pts',(132.843781303579,33.1516429017063,18.1526878848765));
#40873=CARTESIAN_POINT('Ctrl Pts',(132.631458231587,32.8479305530217,18.1288191297898));
#40874=CARTESIAN_POINT('Ctrl Pts',(132.461408326268,32.6553285333291,18.1123734291639));
#40875=CARTESIAN_POINT('Ctrl Pts',(132.233805168996,32.4498890057896,18.0937501968404));
#40876=CARTESIAN_POINT('Ctrl Pts',(132.195593123958,32.4169160178009,18.0907182864872));
#40877=CARTESIAN_POINT('Ctrl Pts',(132.133794797976,32.3659531135047,18.0859603433323));
#40878=CARTESIAN_POINT('Ctrl Pts',(132.110685336914,32.3473992512977,18.0842120789908));
#40879=CARTESIAN_POINT('Ctrl Pts',(132.066359913357,32.3127578375997,18.0809159306526));
#40880=CARTESIAN_POINT('Ctrl Pts',(132.045192050467,32.2966126309671,18.0793658686812));
#40881=CARTESIAN_POINT('Ctrl Pts',(131.996184423646,32.2601385210175,18.0758306015773));
#40882=CARTESIAN_POINT('Ctrl Pts',(131.968220136515,32.2399813776653,18.0738520336952));
#40883=CARTESIAN_POINT('Ctrl Pts',(131.877339669921,32.1765569597681,18.0675401299282));
#40884=CARTESIAN_POINT('Ctrl Pts',(131.813265558445,32.1349862074306,18.0632690241334));
#40885=CARTESIAN_POINT('Ctrl Pts',(131.653357551499,32.0387547600556,18.0529816333626));
#40886=CARTESIAN_POINT('Ctrl Pts',(131.556154469199,31.9865385307356,18.0470404414384));
#40887=CARTESIAN_POINT('Ctrl Pts',(131.264104201861,31.8475597544215,18.0297869175985));
#40888=CARTESIAN_POINT('Ctrl Pts',(131.063437966269,31.7743331077711,18.0186943680113));
#40889=CARTESIAN_POINT('Ctrl Pts',(130.790473298534,31.7029832373987,18.003195016087));
#40890=CARTESIAN_POINT('Ctrl Pts',(130.72319256574,31.6875750852163,17.9993403335762));
#40891=CARTESIAN_POINT('Ctrl Pts',(130.632160906495,31.6696331739001,17.9940233385062));
#40892=CARTESIAN_POINT('Ctrl Pts',(130.608781531844,31.6652802837068,17.9926488624029));
#40893=CARTESIAN_POINT('Ctrl Pts',(130.571551987399,31.6587532444534,17.9904432298382));
#40894=CARTESIAN_POINT('Ctrl Pts',(130.557730357359,31.6564183292848,17.989620690504));
#40895=CARTESIAN_POINT('Ctrl Pts',(130.528428062453,31.6516549773845,17.9878683284136));
#40896=CARTESIAN_POINT('Ctrl Pts',(130.512944460081,31.6492480608296,17.9869372731682));
#40897=CARTESIAN_POINT('Ctrl Pts',(130.473115642621,31.6433392178584,17.9845301810449));
#40898=CARTESIAN_POINT('Ctrl Pts',(130.448748292474,31.639994805001,17.9830459200954));
#40899=CARTESIAN_POINT('Ctrl Pts',(130.340346950717,31.6263169313836,17.9763979586799));
#40900=CARTESIAN_POINT('Ctrl Pts',(130.255985054799,31.6188695819594,17.9711048865904));
#40901=CARTESIAN_POINT('Ctrl Pts',(129.983738169625,31.6050827755293,17.9538160869072));
#40902=CARTESIAN_POINT('Ctrl Pts',(129.795572970168,31.611204142361,17.9415699169901));
#40903=CARTESIAN_POINT('Ctrl Pts',(129.437554275498,31.6527907012639,17.9185000912174));
#40904=CARTESIAN_POINT('Ctrl Pts',(129.267974550023,31.685741688705,17.9076742440456));
#40905=CARTESIAN_POINT('Ctrl Pts',(129.058756573483,31.7432467112076,17.8945574509352));
#40906=CARTESIAN_POINT('Ctrl Pts',(129.016127209777,31.75587056552,17.891896477551));
#40907=CARTESIAN_POINT('Ctrl Pts',(128.946809468332,31.7778897900518,17.8875869577688));
#40908=CARTESIAN_POINT('Ctrl Pts',(128.919969596392,31.7867868260764,17.8859226090341));
#40909=CARTESIAN_POINT('Ctrl Pts',(128.867868723641,31.8047841156217,17.8826992466475));
#40910=CARTESIAN_POINT('Ctrl Pts',(128.842598396971,31.8138506995025,17.8811392774795));
#40911=CARTESIAN_POINT('Ctrl Pts',(128.782755637444,31.8361272520725,17.8774519681663));
#40912=CARTESIAN_POINT('Ctrl Pts',(128.748286211656,31.8496052075382,17.8753336019401));
#40913=CARTESIAN_POINT('Ctrl Pts',(128.626836571071,31.8994015414512,17.8678825385324));
#40914=CARTESIAN_POINT('Ctrl Pts',(128.541154632015,31.938781142968,17.8626508409049));
#40915=CARTESIAN_POINT('Ctrl Pts',(128.320114402638,32.0517634781844,17.8490983991985));
#40916=CARTESIAN_POINT('Ctrl Pts',(128.187938268294,32.1311065329734,17.8409428588115));
#40917=CARTESIAN_POINT('Ctrl Pts',(127.903307425618,32.3295090783609,17.8225563427342));
#40918=CARTESIAN_POINT('Ctrl Pts',(127.754731619268,32.4531597390088,17.8123579889865));
#40919=CARTESIAN_POINT('Ctrl Pts',(127.592922670229,32.6130401575447,17.7995059555737));
#40920=CARTESIAN_POINT('Ctrl Pts',(127.568721838565,32.6376950092199,17.7975319177641));
#40921=CARTESIAN_POINT('Ctrl Pts',(127.532494092718,32.6757488220761,17.7944887760614));
#40922=CARTESIAN_POINT('Ctrl Pts',(127.520189449006,32.688881539147,17.7934392115406));
#40923=CARTESIAN_POINT('Ctrl Pts',(127.497850604482,32.7131075244158,17.7915028825141));
#40924=CARTESIAN_POINT('Ctrl Pts',(127.487784409678,32.7241701314554,17.7906184884705));
#40925=CARTESIAN_POINT('Ctrl Pts',(127.464539050253,32.7500585961633,17.7885487090714));
#40926=CARTESIAN_POINT('Ctrl Pts',(127.451416408212,32.7649339646857,17.7873594230574));
#40927=CARTESIAN_POINT('Ctrl Pts',(127.40876029033,32.8141515543885,17.7834269456304));
#40928=CARTESIAN_POINT('Ctrl Pts',(127.379785658728,32.8489693060977,17.7806489412827));
#40929=CARTESIAN_POINT('Ctrl Pts',(127.309831191951,32.9365421781534,17.7736927242533));
#40930=CARTESIAN_POINT('Ctrl Pts',(127.269697128841,32.9899473311812,17.7694775166303));
#40931=CARTESIAN_POINT('Ctrl Pts',(127.078820544506,33.2602132837539,17.7484013821303));
#40932=CARTESIAN_POINT('Ctrl Pts',(126.952181650762,33.4930239990634,17.7311279219902));
#40933=CARTESIAN_POINT('Ctrl Pts',(126.819019163725,33.8250425217869,17.7088163251872));
#40934=CARTESIAN_POINT('Ctrl Pts',(126.787790788331,33.9133176097124,17.7030777165375));
#40935=CARTESIAN_POINT('Ctrl Pts',(126.749044769385,34.0391946533027,17.6951654139186));
#40936=CARTESIAN_POINT('Ctrl Pts',(126.738450107674,34.0757980185335,17.692895841337));
#40937=CARTESIAN_POINT('Ctrl Pts',(126.721411621202,34.1386109226143,17.689052750274));
#40938=CARTESIAN_POINT('Ctrl Pts',(126.714659686153,34.1647323873027,17.6874696153411));
#40939=CARTESIAN_POINT('Ctrl Pts',(126.70146453161,34.2184183036083,17.6842456706485));
#40940=CARTESIAN_POINT('Ctrl Pts',(126.695053272865,34.2459884712467,17.6826059764113));
#40941=CARTESIAN_POINT('Ctrl Pts',(126.682822066228,34.3017424608683,17.6793207038594));
#40942=CARTESIAN_POINT('Ctrl Pts',(126.677014194088,34.3299265414582,17.6776756166388));
#40943=CARTESIAN_POINT('Ctrl Pts',(126.663704420292,34.3989503009543,17.6736825629904));
#40944=CARTESIAN_POINT('Ctrl Pts',(126.656592556841,34.4398609086381,17.6713463499338));
#40945=CARTESIAN_POINT('Ctrl Pts',(126.623481629572,34.6535237469232,17.659285139113));
#40946=CARTESIAN_POINT('Ctrl Pts',(126.610113399899,34.8279690245501,17.6499298854475));
#40947=CARTESIAN_POINT('Ctrl Pts',(126.610251052227,35.0026708751785,17.6406473680219));
#40948=CARTESIAN_POINT('Ctrl Pts',(126.610251067793,35.0026905576773,17.6410178032139));
#40949=CARTESIAN_POINT('Ctrl Pts',(126.610355874084,35.1347327056219,17.6332712403869));
#40950=CARTESIAN_POINT('Ctrl Pts',(126.618179561376,35.2664475840005,17.6255246775599));
#40951=CARTESIAN_POINT('Ctrl Pts',(126.633586026562,35.3970667726449,17.6177781147329));
#40952=CARTESIAN_POINT('Ctrl Pts',(126.649300794567,35.5302998161686,17.6098765334033));
#40953=CARTESIAN_POINT('Ctrl Pts',(126.672904863042,35.6623931370086,17.6019749520736));
#40954=CARTESIAN_POINT('Ctrl Pts',(126.704205303174,35.7925543381198,17.594073370744));
#40955=CARTESIAN_POINT('Ctrl Pts',(126.70794873765,35.808121209563,17.5931283663978));
#40956=CARTESIAN_POINT('Ctrl Pts',(126.711802200231,35.8236604689481,17.5921833620516));
#40957=CARTESIAN_POINT('Ctrl Pts',(126.715765315128,35.8391707795115,17.5912383577054));
#40958=CARTESIAN_POINT('Ctrl Pts',(126.741359185109,35.9393366546373,17.5851355019987));
#40959=CARTESIAN_POINT('Ctrl Pts',(126.771582343066,36.0384975902312,17.5790326462921));
#40960=CARTESIAN_POINT('Ctrl Pts',(126.806339543602,36.1361945043616,17.5729297905854));
#40961=CARTESIAN_POINT('Ctrl Pts',(126.811217881386,36.149906729173,17.5720732258701));
#40962=CARTESIAN_POINT('Ctrl Pts',(126.816185454427,36.1635901266068,17.5712166611547));
#40963=CARTESIAN_POINT('Ctrl Pts',(126.821241918358,36.1772434416438,17.5703600964394));
#40964=CARTESIAN_POINT('Ctrl Pts',(126.821241978387,36.177243603733,17.9148965215314));
#40965=CARTESIAN_POINT('Ctrl Pts',(126.742546241387,35.9647517248556,17.9271213083101));
#40966=CARTESIAN_POINT('Ctrl Pts',(126.685311358021,35.7447864351744,17.9388787175516));
#40967=CARTESIAN_POINT('Ctrl Pts',(126.640195531105,35.4545256772944,17.9547792722127));
#40968=CARTESIAN_POINT('Ctrl Pts',(126.631880982833,35.3881405025059,17.9584446854921));
#40969=CARTESIAN_POINT('Ctrl Pts',(126.621238178706,35.2764532248012,17.9647213719342));
#40970=CARTESIAN_POINT('Ctrl Pts',(126.617845166975,35.2312706375423,17.9672906172474));
#40971=CARTESIAN_POINT('Ctrl Pts',(126.614272277592,35.1662673452647,17.9710470344894));
#40972=CARTESIAN_POINT('Ctrl Pts',(126.613358944124,35.1464901294407,17.9721979026875));
#40973=CARTESIAN_POINT('Ctrl Pts',(126.612060269939,35.1117712954401,17.9742339924007));
#40974=CARTESIAN_POINT('Ctrl Pts',(126.611600418236,35.0968333602536,17.9751152105004));
#40975=CARTESIAN_POINT('Ctrl Pts',(126.61080362177,35.0638614028776,17.9770721062152));
#40976=CARTESIAN_POINT('Ctrl Pts',(126.610511814138,35.0458276635016,17.9781500494998));
#40977=CARTESIAN_POINT('Ctrl Pts',(126.610071561826,34.9921342820039,17.9813805203113));
#40978=CARTESIAN_POINT('Ctrl Pts',(126.610341901981,34.9564747577097,17.9835535674568));
#40979=CARTESIAN_POINT('Ctrl Pts',(126.615219407709,34.7477020361011,17.9964122326283));
#40980=CARTESIAN_POINT('Ctrl Pts',(126.632524599149,34.5751536643685,18.0075755379586));
#40981=CARTESIAN_POINT('Ctrl Pts',(126.692217018682,34.2405378086125,18.0294866602718));
#40982=CARTESIAN_POINT('Ctrl Pts',(126.733577150869,34.0787502140273,18.0402038879868));
#40983=CARTESIAN_POINT('Ctrl Pts',(126.818119250642,33.8270600122975,18.0567902395979));
#40984=CARTESIAN_POINT('Ctrl Pts',(126.853633551103,33.7348777119108,18.0628493365591));
#40985=CARTESIAN_POINT('Ctrl Pts',(126.908200170215,33.6098202123117,18.0710429882789));
#40986=CARTESIAN_POINT('Ctrl Pts',(126.923851153912,33.5755230860111,18.0732875477297));
#40987=CARTESIAN_POINT('Ctrl Pts',(126.951712557756,33.517070223067,18.0771099676546));
#40988=CARTESIAN_POINT('Ctrl Pts',(126.963645872865,33.4927870980784,18.0786970237425));
#40989=CARTESIAN_POINT('Ctrl Pts',(126.988628967601,33.4434501732003,18.0819206478605));
#40990=CARTESIAN_POINT('Ctrl Pts',(127.001703758499,33.4184113756944,18.0835561967026));
#40991=CARTESIAN_POINT('Ctrl Pts',(127.035892868566,33.3548857959607,18.0877063705702));
#40992=CARTESIAN_POINT('Ctrl Pts',(127.05744490944,33.3166397834125,18.0902055783659));
#40993=CARTESIAN_POINT('Ctrl Pts',(127.158033903537,33.1459737895013,18.1013762506651));
#40994=CARTESIAN_POINT('Ctrl Pts',(127.24531105253,33.0186165773679,18.1097523459911));
#40995=CARTESIAN_POINT('Ctrl Pts',(127.361761445937,32.8713321806519,18.1197876019496));
#40996=CARTESIAN_POINT('Ctrl Pts',(127.382946724188,32.8453395766729,18.1215733837784));
#40997=CARTESIAN_POINT('Ctrl Pts',(127.527380692029,32.6734043649703,18.1335084875933));
#40998=CARTESIAN_POINT('Ctrl Pts',(127.662381895831,32.5378006275309,18.1435045424293));
#40999=CARTESIAN_POINT('Ctrl Pts',(127.859996595019,32.3702806282698,18.1577440844689));
#41000=CARTESIAN_POINT('Ctrl Pts',(127.913230917842,32.3278412987898,18.1615479663073));
#41001=CARTESIAN_POINT('Ctrl Pts',(127.986638331475,32.2728513773428,18.1668048627691));
#41002=CARTESIAN_POINT('Ctrl Pts',(128.005721201017,32.2588657780271,18.1681724601006));
#41003=CARTESIAN_POINT('Ctrl Pts',(128.036321696988,32.236927720345,18.1703698026233));
#41004=CARTESIAN_POINT('Ctrl Pts',(128.047745232028,32.2288446081433,18.171191040011));
#41005=CARTESIAN_POINT('Ctrl Pts',(128.072168384419,32.2117891373327,18.1729495671063));
#41006=CARTESIAN_POINT('Ctrl Pts',(128.085181247708,32.2028364948273,18.173888171196));
#41007=CARTESIAN_POINT('Ctrl Pts',(128.118876410211,32.1800000679827,18.1763217913346));
#41008=CARTESIAN_POINT('Ctrl Pts',(128.139649702765,32.1662529631809,18.177825228659));
#41009=CARTESIAN_POINT('Ctrl Pts',(128.233893786655,32.1053681125815,18.1846531334195));
#41010=CARTESIAN_POINT('Ctrl Pts',(128.30901250583,32.06085321654,18.1901140412535));
#41011=CARTESIAN_POINT('Ctrl Pts',(128.562546017882,31.9235489159507,18.2084097286551));
#41012=CARTESIAN_POINT('Ctrl Pts',(128.747499924802,31.8437250689561,18.221516927988));
#41013=CARTESIAN_POINT('Ctrl Pts',(129.086235515022,31.7320253942136,18.244250922917));
#41014=CARTESIAN_POINT('Ctrl Pts',(129.237225025532,31.6935202390104,18.2539748213305));
#41015=CARTESIAN_POINT('Ctrl Pts',(129.433609078563,31.6576144940119,18.2660366970994));
#41016=CARTESIAN_POINT('Ctrl Pts',(129.477025933926,31.6505466199134,18.2686683877804));
#41017=CARTESIAN_POINT('Ctrl Pts',(129.548562908793,31.6403260226463,18.2729490669459));
#41018=CARTESIAN_POINT('Ctrl Pts',(129.576605739499,31.6366769328558,18.2746132132756));
#41019=CARTESIAN_POINT('Ctrl Pts',(129.63157699661,31.6302222115512,18.2778492054007));
#41020=CARTESIAN_POINT('Ctrl Pts',(129.658499792333,31.6273874335503,18.279421837717));
#41021=CARTESIAN_POINT('Ctrl Pts',(129.722982761085,31.6213779237874,18.2831606566718));
#41022=CARTESIAN_POINT('Ctrl Pts',(129.760568002501,31.6185065187469,18.2853173810689));
#41023=CARTESIAN_POINT('Ctrl Pts',(129.896594485887,31.6103939202397,18.2930490414176));
#41024=CARTESIAN_POINT('Ctrl Pts',(129.995208673525,31.608820047677,18.2985129515031));
#41025=CARTESIAN_POINT('Ctrl Pts',(130.259959113656,31.6161456368023,18.3129483022094));
#41026=CARTESIAN_POINT('Ctrl Pts',(130.425602307241,31.6329664633323,18.3217237909728));
#41027=CARTESIAN_POINT('Ctrl Pts',(130.760475617407,31.6920881649874,18.3397647250944));
#41028=CARTESIAN_POINT('Ctrl Pts',(130.929013609413,31.7354134548875,18.3490111740306));
#41029=CARTESIAN_POINT('Ctrl Pts',(131.127200967488,31.8029555699515,18.3608338450197));
#41030=CARTESIAN_POINT('Ctrl Pts',(131.160748774204,31.814982389136,18.3628694454939));
#41031=CARTESIAN_POINT('Ctrl Pts',(131.210982991434,31.8338902892475,18.3659782457726));
#41032=CARTESIAN_POINT('Ctrl Pts',(131.227815254768,31.8403797420406,18.3670303206979));
#41033=CARTESIAN_POINT('Ctrl Pts',(131.258501465979,31.8524926272814,18.3689687542648));
#41034=CARTESIAN_POINT('Ctrl Pts',(131.272371144512,31.8580738001621,18.3698527063661));
#41035=CARTESIAN_POINT('Ctrl Pts',(131.304535273696,31.871264575023,18.3719206601585));
#41036=CARTESIAN_POINT('Ctrl Pts',(131.322800363333,31.8789430000731,18.3731085350634));
#41037=CARTESIAN_POINT('Ctrl Pts',(131.382696251912,31.9047427205764,18.3770461251084));
#41038=CARTESIAN_POINT('Ctrl Pts',(131.424028728645,31.9235396463993,18.3798309649126));
#41039=CARTESIAN_POINT('Ctrl Pts',(131.525477260062,31.9721581395079,18.3868134968949));
#41040=CARTESIAN_POINT('Ctrl Pts',(131.585108234746,32.002945082609,18.3910486898686));
#41041=CARTESIAN_POINT('Ctrl Pts',(131.890825315708,32.1724607189888,18.4133193928842));
#41042=CARTESIAN_POINT('Ctrl Pts',(132.119819874756,32.3398120099157,18.4318065454864));
#41043=CARTESIAN_POINT('Ctrl Pts',(132.382931237471,32.5878854709709,18.454201068933));
#41044=CARTESIAN_POINT('Ctrl Pts',(132.438552519559,32.6441305380867,18.4590234769016));
#41045=CARTESIAN_POINT('Ctrl Pts',(132.514053240739,32.7260200908385,18.4656985686129));
#41046=CARTESIAN_POINT('Ctrl Pts',(132.535607369955,32.750079179548,18.4676201817227));
#41047=CARTESIAN_POINT('Ctrl Pts',(132.574478959797,32.7947365278488,18.471116463134));
#41048=CARTESIAN_POINT('Ctrl Pts',(132.591901152447,32.8152397444662,18.4726953321628));
#41049=CARTESIAN_POINT('Ctrl Pts',(132.626974786088,32.8575260971522,18.4758993192026));
#41050=CARTESIAN_POINT('Ctrl Pts',(132.644603806424,32.8793251718146,18.477523471693));
#41051=CARTESIAN_POINT('Ctrl Pts',(132.688455542825,32.9349471654516,18.4816004990672));
#41052=CARTESIAN_POINT('Ctrl Pts',(132.71431232592,32.969053116442,18.4840390888703));
#41053=CARTESIAN_POINT('Ctrl Pts',(132.828963321908,33.1263836979172,18.4950279302835));
#41054=CARTESIAN_POINT('Ctrl Pts',(132.910064047675,33.2550055622229,18.5032906401355));
#41055=CARTESIAN_POINT('Ctrl Pts',(133.003568860762,33.428062806557,18.513815122184));
#41056=CARTESIAN_POINT('Ctrl Pts',(133.024083442999,33.4678995292755,18.5162003376815));
#41057=CARTESIAN_POINT('Ctrl Pts',(133.132772115783,33.689652903948,18.5293176883215));
#41058=CARTESIAN_POINT('Ctrl Pts',(133.205318101077,33.8787537201437,18.5398966152786));
#41059=CARTESIAN_POINT('Ctrl Pts',(133.275454673363,34.1254940731038,18.5541310903519));
#41060=CARTESIAN_POINT('Ctrl Pts',(133.289065123496,34.1781643232198,18.5571949839945));
#41061=CARTESIAN_POINT('Ctrl Pts',(133.306337299053,34.2523288043128,18.561573042761));
#41062=CARTESIAN_POINT('Ctrl Pts',(133.311068548516,34.2735679208276,18.5628340847204));
#41063=CARTESIAN_POINT('Ctrl Pts',(133.318754853112,34.3097087284038,18.5649944377829));
#41064=CARTESIAN_POINT('Ctrl Pts',(133.321814883292,34.3245877626973,18.5658880420751));
#41065=CARTESIAN_POINT('Ctrl Pts',(133.328071979391,34.3560836357715,18.5677892266493));
#41066=CARTESIAN_POINT('Ctrl Pts',(133.331244750567,34.3727044005923,18.5687980055136));
#41067=CARTESIAN_POINT('Ctrl Pts',(133.339727786571,34.4190236110607,18.5716232609083));
#41068=CARTESIAN_POINT('Ctrl Pts',(133.344766074707,34.4487695380154,18.573453546162));
#41069=CARTESIAN_POINT('Ctrl Pts',(133.375784942935,34.6480221962763,18.5858023000113));
#41070=CARTESIAN_POINT('Ctrl Pts',(133.389265015778,34.8192101094648,18.5968266613978));
#41071=CARTESIAN_POINT('Ctrl Pts',(133.390420937885,35.2389850114804,18.623882369893));
#41072=CARTESIAN_POINT('Ctrl Pts',(133.363816223294,35.486667187147,18.6398130228803));
#41073=CARTESIAN_POINT('Ctrl Pts',(133.299433756028,35.7789289146008,18.6580061864668));
#41074=CARTESIAN_POINT('Ctrl Pts',(133.287371268884,35.8283621941867,18.6610652605315));
#41075=CARTESIAN_POINT('Ctrl Pts',(133.266441994318,35.9064545728802,18.6658708893789));
#41076=CARTESIAN_POINT('Ctrl Pts',(133.258300210081,35.9352983600492,18.6676399863917));
#41077=CARTESIAN_POINT('Ctrl Pts',(133.242237231528,35.989447126699,18.67095104707));
#41078=CARTESIAN_POINT('Ctrl Pts',(133.234399629447,36.0147743482699,18.6724955426171));
#41079=CARTESIAN_POINT('Ctrl Pts',(133.215909066259,36.072134957112,18.6759851024794));
#41080=CARTESIAN_POINT('Ctrl Pts',(133.205073027559,36.1041066496398,18.6779241033504));
#41081=CARTESIAN_POINT('Ctrl Pts',(133.169539064105,36.2040149040705,18.6839686999769));
#41082=CARTESIAN_POINT('Ctrl Pts',(133.143144040371,36.2713285665895,18.6880194187991));
#41083=CARTESIAN_POINT('Ctrl Pts',(133.074418379635,36.4313390057888,18.6976408883267));
#41084=CARTESIAN_POINT('Ctrl Pts',(133.030021848069,36.523072290355,18.7031496040599));
#41085=CARTESIAN_POINT('Ctrl Pts',(132.959071284069,36.6542480354957,18.7111278680029));
#41086=CARTESIAN_POINT('Ctrl Pts',(132.935715629613,36.6953504833347,18.7136433451992));
#41087=CARTESIAN_POINT('Ctrl Pts',(132.805291792699,36.9140950918857,18.7271664321003));
#41088=CARTESIAN_POINT('Ctrl Pts',(132.682960009724,37.0820980196311,18.7380208971892));
#41089=CARTESIAN_POINT('Ctrl Pts',(132.51435251491,37.2739268041217,18.7522611643245));
#41090=CARTESIAN_POINT('Ctrl Pts',(132.481884300105,37.3093205768481,18.7549764757324));
#41091=CARTESIAN_POINT('Ctrl Pts',(132.43562723658,37.3576431369403,18.7588279989734));
#41092=CARTESIAN_POINT('Ctrl Pts',(132.422464293886,37.3711659382404,18.7599221570405));
#41093=CARTESIAN_POINT('Ctrl Pts',(132.398522361287,37.3953549798407,18.7619105862145));
#41094=CARTESIAN_POINT('Ctrl Pts',(132.387783216076,37.4060603283625,18.7628018996168));
#41095=CARTESIAN_POINT('Ctrl Pts',(132.365157085566,37.4283145770245,18.7646793874163));
#41096=CARTESIAN_POINT('Ctrl Pts',(132.353256762334,37.4398488292339,18.7656665265122));
#41097=CARTESIAN_POINT('Ctrl Pts',(132.320642396286,37.4709993515242,18.7683697897685));
#41098=CARTESIAN_POINT('Ctrl Pts',(132.299764975184,37.4904417016217,18.770097933796));
#41099=CARTESIAN_POINT('Ctrl Pts',(132.156781517908,37.6202657074694,18.781903085186));
#41100=CARTESIAN_POINT('Ctrl Pts',(132.027030599381,37.7218809890255,18.7924574440581));
#41101=CARTESIAN_POINT('Ctrl Pts',(131.673834989838,37.9591841060868,18.8198717167916));
#41102=CARTESIAN_POINT('Ctrl Pts',(131.441125990381,38.0792356839474,18.8366487595532));
#41103=CARTESIAN_POINT('Ctrl Pts',(131.150174562146,38.1890437212003,18.8555318610879));
#41104=CARTESIAN_POINT('Ctrl Pts',(131.103043680384,38.2056507009389,18.8585329874527));
#41105=CARTESIAN_POINT('Ctrl Pts',(131.027522097631,38.2303984271242,18.8632528745699));
#41106=CARTESIAN_POINT('Ctrl Pts',(130.999363862019,38.2392202167762,18.8649933376576));
#41107=CARTESIAN_POINT('Ctrl Pts',(130.945605667774,38.2552945622307,18.868280525615));
#41108=CARTESIAN_POINT('Ctrl Pts',(130.920028642327,38.2626155339666,18.8698293423279));
#41109=CARTESIAN_POINT('Ctrl Pts',(130.861011504662,38.2787589307017,18.8733696216589));
#41110=CARTESIAN_POINT('Ctrl Pts',(130.827516976007,38.2873723118489,18.8753543221127));
#41111=CARTESIAN_POINT('Ctrl Pts',(130.718830584855,38.3135554052211,18.8817203776833));
#41112=CARTESIAN_POINT('Ctrl Pts',(130.643166270144,38.3290697197368,18.8860377990188));
#41113=CARTESIAN_POINT('Ctrl Pts',(130.456433095637,38.3607526820474,18.8964725612023));
#41114=CARTESIAN_POINT('Ctrl Pts',(130.344964319985,38.3740171372746,18.9025115751598));
#41115=CARTESIAN_POINT('Ctrl Pts',(130.008601358767,38.3971962179771,18.9204871399848));
#41116=CARTESIAN_POINT('Ctrl Pts',(129.783202324511,38.3902800222877,18.9321782231361));
#41117=CARTESIAN_POINT('Ctrl Pts',(129.503449075565,38.3536718245008,18.9478013513118));
#41118=CARTESIAN_POINT('Ctrl Pts',(129.446927449652,38.3448150198062,18.9510179170686));
#41119=CARTESIAN_POINT('Ctrl Pts',(129.368811794962,38.3305404688155,18.9555799362431));
#41120=CARTESIAN_POINT('Ctrl Pts',(129.347003575775,38.3263334135453,18.9568662782091));
#41121=CARTESIAN_POINT('Ctrl Pts',(129.310425472703,38.3189035125199,18.9590475939386));
#41122=CARTESIAN_POINT('Ctrl Pts',(129.295632541086,38.3157955351844,18.9599363506415));
#41123=CARTESIAN_POINT('Ctrl Pts',(129.264560332171,38.3090499826678,18.961817842263));
#41124=CARTESIAN_POINT('Ctrl Pts',(129.248286507376,38.3053910649048,18.9628116548701));
#41125=CARTESIAN_POINT('Ctrl Pts',(129.203764717212,38.2950352391742,18.9655523172462));
#41126=CARTESIAN_POINT('Ctrl Pts',(129.175575370177,38.2880954609688,18.9673117239182));
#41127=CARTESIAN_POINT('Ctrl Pts',(128.968963945849,38.2344071168139,18.9803678973837));
#41128=CARTESIAN_POINT('Ctrl Pts',(128.794546970786,38.1735305746779,18.992258032739));
#41129=CARTESIAN_POINT('Ctrl Pts',(128.410956614533,38.0034418956255,19.0193064456423));
#41130=CARTESIAN_POINT('Ctrl Pts',(128.206424363278,37.8859729330732,19.0343583198718));
#41131=CARTESIAN_POINT('Ctrl Pts',(127.97346294431,37.7177683206549,19.051842332571));
#41132=CARTESIAN_POINT('Ctrl Pts',(127.931947756927,37.6863129848495,19.0549758765532));
#41133=CARTESIAN_POINT('Ctrl Pts',(127.867505825599,37.6351067140699,19.059870547961));
#41134=CARTESIAN_POINT('Ctrl Pts',(127.84409164397,37.6159851007693,19.0616556511919));
#41135=CARTESIAN_POINT('Ctrl Pts',(127.800848156695,37.5796945423823,19.0649662175627));
#41136=CARTESIAN_POINT('Ctrl Pts',(127.780956426011,37.5626038389947,19.0664946315759));
#41137=CARTESIAN_POINT('Ctrl Pts',(127.736316380893,37.5233401409695,19.0699385334073));
#41138=CARTESIAN_POINT('Ctrl Pts',(127.711691529643,37.501030477779,19.0718482369088));
#41139=CARTESIAN_POINT('Ctrl Pts',(127.636778639792,37.4311279729294,19.0776930075945));
#41140=CARTESIAN_POINT('Ctrl Pts',(127.587616103598,37.3823524623555,19.0815784721774));
#41141=CARTESIAN_POINT('Ctrl Pts',(127.474094213918,37.2626038158982,19.0907118047235));
#41142=CARTESIAN_POINT('Ctrl Pts',(127.411180981337,37.1903410253636,19.0959063479186));
#41143=CARTESIAN_POINT('Ctrl Pts',(127.268165118088,37.0112868643171,19.1081957732661));
#41144=CARTESIAN_POINT('Ctrl Pts',(127.191144049104,36.9022421973285,19.1152224965472));
#41145=CARTESIAN_POINT('Ctrl Pts',(127.040808513353,36.66028164785,19.1303671904146));
#41146=CARTESIAN_POINT('Ctrl Pts',(126.969589237825,36.5264178094058,19.1384873583599));
#41147=CARTESIAN_POINT('Ctrl Pts',(126.892808770643,36.3553840947005,19.1490687482448));
#41148=CARTESIAN_POINT('Ctrl Pts',(126.878577645659,36.3222804727807,19.1511261932591));
#41149=CARTESIAN_POINT('Ctrl Pts',(126.857989616,36.2722043574716,19.1542615354382));
#41150=CARTESIAN_POINT('Ctrl Pts',(126.851236298365,36.2553964710475,19.1553177519522));
#41151=CARTESIAN_POINT('Ctrl Pts',(126.839211380758,36.22476093345,19.1572512624016));
#41152=CARTESIAN_POINT('Ctrl Pts',(126.833895150909,36.21095173283,19.1581259722701));
#41153=CARTESIAN_POINT('Ctrl Pts',(126.826172897444,36.1904942512583,19.1594263879238));
#41154=CARTESIAN_POINT('Ctrl Pts',(126.823697025162,36.1838726487564,19.1598479919515));
#41155=CARTESIAN_POINT('Ctrl Pts',(126.821241918361,36.1772434416541,19.1602707349979));
#41156=CARTESIAN_POINT('Origin',(130.,35.,23.));
#41157=CARTESIAN_POINT('',(126.821241918623,36.1772434423597,20.4155867593643));
#41158=CARTESIAN_POINT('',(126.821241918282,36.1772434414401,20.0676575318486));
#41159=CARTESIAN_POINT('',(126.821241918358,36.1772434416438,23.));
#41160=CARTESIAN_POINT('Ctrl Pts',(126.821241918282,36.1772434414401,20.0676575318486));
#41161=CARTESIAN_POINT('Ctrl Pts',(126.838313316203,36.223339127512,20.0646699192867));
#41162=CARTESIAN_POINT('Ctrl Pts',(126.856386171251,36.2690602397116,20.0617137706984));
#41163=CARTESIAN_POINT('Ctrl Pts',(126.88719367022,36.3422963180723,20.0569885070641));
#41164=CARTESIAN_POINT('Ctrl Pts',(126.899313304811,36.3700601299697,20.0551994726895));
#41165=CARTESIAN_POINT('Ctrl Pts',(126.922717144669,36.4217720843826,20.051870578595));
#41166=CARTESIAN_POINT('Ctrl Pts',(126.933912790088,36.4457575562487,20.0503278929043));
#41167=CARTESIAN_POINT('Ctrl Pts',(126.959808776478,36.499582844253,20.0468678737414));
#41168=CARTESIAN_POINT('Ctrl Pts',(126.974669814071,36.5293425910029,20.0449561846332));
#41169=CARTESIAN_POINT('Ctrl Pts',(127.021899865511,36.6205388731543,20.0390980357143));
#41170=CARTESIAN_POINT('Ctrl Pts',(127.055721265314,36.6812050115015,20.0352015225534));
#41171=CARTESIAN_POINT('Ctrl Pts',(127.21935292679,36.954610185972,20.0175670034843));
#41172=CARTESIAN_POINT('Ctrl Pts',(127.370504130951,37.1536608253841,20.0045824710504));
#41173=CARTESIAN_POINT('Ctrl Pts',(127.641910865143,37.4394306972192,19.9835579244436));
#41174=CARTESIAN_POINT('Ctrl Pts',(127.748335192292,37.5379920054062,19.9757264785971));
#41175=CARTESIAN_POINT('Ctrl Pts',(127.882496567301,37.647144119824,19.9658745128229));
#41176=CARTESIAN_POINT('Ctrl Pts',(127.904485999794,37.6645850981208,19.9642602295987));
#41177=CARTESIAN_POINT('Ctrl Pts',(127.939721701358,37.6918264767577,19.9616697763209));
#41178=CARTESIAN_POINT('Ctrl Pts',(127.952827692047,37.7018071666238,19.9607054477949));
#41179=CARTESIAN_POINT('Ctrl Pts',(127.978176842652,37.7208211386307,19.9588376341886));
#41180=CARTESIAN_POINT('Ctrl Pts',(127.990408913683,37.7298681618174,19.957935087149));
#41181=CARTESIAN_POINT('Ctrl Pts',(128.021098991778,37.7522489627446,19.9556682852218));
#41182=CARTESIAN_POINT('Ctrl Pts',(128.039631072615,37.7654795533561,19.9542974387843));
#41183=CARTESIAN_POINT('Ctrl Pts',(128.108443954546,37.8135678359851,19.9492039622959));
#41184=CARTESIAN_POINT('Ctrl Pts',(128.159530009071,37.8472473567515,19.9454163695027));
#41185=CARTESIAN_POINT('Ctrl Pts',(128.378371716914,37.9831723539694,19.9292536977309));
#41186=CARTESIAN_POINT('Ctrl Pts',(128.553936282953,38.0721152533477,19.9164623009833));
#41187=CARTESIAN_POINT('Ctrl Pts',(128.897764879805,38.2102642207699,19.8926891645032));
#41188=CARTESIAN_POINT('Ctrl Pts',(129.064097228688,38.2626397742953,19.881699514965));
#41189=CARTESIAN_POINT('Ctrl Pts',(129.285170060892,38.3139419251281,19.8678891337791));
#41190=CARTESIAN_POINT('Ctrl Pts',(129.336877393315,38.3246746912017,19.8647123190013));
#41191=CARTESIAN_POINT('Ctrl Pts',(129.418409882472,38.3396202157039,19.8597842710571));
#41192=CARTESIAN_POINT('Ctrl Pts',(129.448074724989,38.3446507782061,19.8580079200008));
#41193=CARTESIAN_POINT('Ctrl Pts',(129.503982091926,38.3533674542995,19.8546903828047));
#41194=CARTESIAN_POINT('Ctrl Pts',(129.530208317651,38.3571420706641,19.8531465580247));
#41195=CARTESIAN_POINT('Ctrl Pts',(129.589760971225,38.3650016557467,19.8496679083141));
#41196=CARTESIAN_POINT('Ctrl Pts',(129.623109508572,38.3688998021047,19.8477389910857));
#41197=CARTESIAN_POINT('Ctrl Pts',(129.727362141837,38.3795185421538,19.8417640328731));
#41198=CARTESIAN_POINT('Ctrl Pts',(129.798425793449,38.3845008186541,19.837770994365));
#41199=CARTESIAN_POINT('Ctrl Pts',(130.116659500623,38.3967522467673,19.8201643971113));
#41200=CARTESIAN_POINT('Ctrl Pts',(130.36401463301,38.3792059167859,19.8072817520666));
#41201=CARTESIAN_POINT('Ctrl Pts',(130.749143077332,38.3090762602486,19.7863955276807));
#41202=CARTESIAN_POINT('Ctrl Pts',(130.889211108111,38.2742168663908,19.7786002792756));
#41203=CARTESIAN_POINT('Ctrl Pts',(131.053345896833,38.2220574163343,19.7687897292882));
#41204=CARTESIAN_POINT('Ctrl Pts',(131.079966213413,38.213232709006,19.7671766465327));
#41205=CARTESIAN_POINT('Ctrl Pts',(131.122040160227,38.1987032022382,19.7645876738518));
#41206=CARTESIAN_POINT('Ctrl Pts',(131.137567536321,38.1932141132004,19.7636236022546));
#41207=CARTESIAN_POINT('Ctrl Pts',(131.1673634614,38.1824360428259,19.7617559037374));
#41208=CARTESIAN_POINT('Ctrl Pts',(131.181637392499,38.1771637756751,19.7608532097101));
#41209=CARTESIAN_POINT('Ctrl Pts',(131.217193461896,38.1637579279225,19.75858546073));
#41210=CARTESIAN_POINT('Ctrl Pts',(131.238429816801,38.1555056135505,19.7572138024292));
#41211=CARTESIAN_POINT('Ctrl Pts',(131.316470494942,38.1242703795731,19.7521136189361));
#41212=CARTESIAN_POINT('Ctrl Pts',(131.372728919534,38.0999636022879,19.7483199184271));
#41213=CARTESIAN_POINT('Ctrl Pts',(131.628498753288,37.9811291799073,19.7306248670867));
#41214=CARTESIAN_POINT('Ctrl Pts',(131.819134171518,37.8687784602382,19.7161983189973));
#41215=CARTESIAN_POINT('Ctrl Pts',(132.087568468324,37.6729932815203,19.6949729183076));
#41216=CARTESIAN_POINT('Ctrl Pts',(132.174354804678,37.6028868133298,19.6879373289241));
#41217=CARTESIAN_POINT('Ctrl Pts',(132.31489246437,37.4774160618863,19.6762954007704));
#41218=CARTESIAN_POINT('Ctrl Pts',(132.37049516893,37.4242672157061,19.6716154379592));
#41219=CARTESIAN_POINT('Ctrl Pts',(132.448379216812,37.3445759730336,19.6649482415669));
#41220=CARTESIAN_POINT('Ctrl Pts',(132.472134907321,37.3195142627256,19.6628984280716));
#41221=CARTESIAN_POINT('Ctrl Pts',(132.513503416582,37.2745137862741,19.6592984039978));
#41222=CARTESIAN_POINT('Ctrl Pts',(132.531271939957,37.2547227800684,19.6577417481747));
#41223=CARTESIAN_POINT('Ctrl Pts',(132.568275239355,37.2125188107682,19.6544767718267));
#41224=CARTESIAN_POINT('Ctrl Pts',(132.587453801296,37.1900593825253,19.6527708188554));
#41225=CARTESIAN_POINT('Ctrl Pts',(132.638365249114,37.128836100136,19.6482022830898));
#41226=CARTESIAN_POINT('Ctrl Pts',(132.669537019233,37.0896140299767,19.6453619244202));
#41227=CARTESIAN_POINT('Ctrl Pts',(132.85702833402,36.8426554166803,19.6279691714365));
#41228=CARTESIAN_POINT('Ctrl Pts',(132.989885680575,36.6182040441577,19.6143479070092));
#41229=CARTESIAN_POINT('Ctrl Pts',(133.141860843739,36.2774617212924,19.5945150488444));
#41230=CARTESIAN_POINT('Ctrl Pts',(133.18273122213,36.1719287943705,19.5884639721829));
#41231=CARTESIAN_POINT('Ctrl Pts',(133.238413724641,36.0035958223691,19.5786863703352));
#41232=CARTESIAN_POINT('Ctrl Pts',(133.256841611507,35.9420773275853,19.5750872065185));
#41233=CARTESIAN_POINT('Ctrl Pts',(133.279358595488,35.8583237513932,19.5701073453748));
#41234=CARTESIAN_POINT('Ctrl Pts',(133.284989717365,35.8365135731561,19.5688033183606));
#41235=CARTESIAN_POINT('Ctrl Pts',(133.29408504791,35.7997771598081,19.5665922812221));
#41236=CARTESIAN_POINT('Ctrl Pts',(133.297666278472,35.7848801931986,19.5656916638655));
#41237=CARTESIAN_POINT('Ctrl Pts',(133.304919996886,35.7537803918626,19.5638022668399));
#41238=CARTESIAN_POINT('Ctrl Pts',(133.30857452461,35.7375741688122,19.5628126139723));
#41239=CARTESIAN_POINT('Ctrl Pts',(133.318220915109,35.6932818660515,19.560095236951));
#41240=CARTESIAN_POINT('Ctrl Pts',(133.323975084396,35.6651460794271,19.5583552909788));
#41241=CARTESIAN_POINT('Ctrl Pts',(133.361081287394,35.4711874685795,19.546281753768));
#41242=CARTESIAN_POINT('Ctrl Pts',(133.380366464866,35.3033109185356,19.5354479155878));
#41243=CARTESIAN_POINT('Ctrl Pts',(133.392592144583,34.9959244576744,19.5156240732214));
#41244=CARTESIAN_POINT('Ctrl Pts',(133.38957661798,34.8569204630671,19.5066632203482));
#41245=CARTESIAN_POINT('Ctrl Pts',(133.366891386618,34.584705020195,19.4893666414945));
#41246=CARTESIAN_POINT('Ctrl Pts',(133.347803882861,34.4516901609415,19.4810349002571));
#41247=CARTESIAN_POINT('Ctrl Pts',(133.312558489191,34.2795278009172,19.4704419343739));
#41248=CARTESIAN_POINT('Ctrl Pts',(133.303498608372,34.239065635466,19.4679657641418));
#41249=CARTESIAN_POINT('Ctrl Pts',(133.28713513935,34.1717979330685,19.4638700483873));
#41250=CARTESIAN_POINT('Ctrl Pts',(133.280240473037,34.1448984881648,19.4622378426566));
#41251=CARTESIAN_POINT('Ctrl Pts',(133.265965941213,34.0919219173324,19.4590334806381));
#41252=CARTESIAN_POINT('Ctrl Pts',(133.258602358757,34.0658425918495,19.4574609444333));
#41253=CARTESIAN_POINT('Ctrl Pts',(133.239769558168,34.0020772464524,19.4536266016018));
#41254=CARTESIAN_POINT('Ctrl Pts',(133.227954509137,33.9644969911269,19.4513760038306));
#41255=CARTESIAN_POINT('Ctrl Pts',(133.182615305874,33.8286113604183,19.4432629137138));
#41256=CARTESIAN_POINT('Ctrl Pts',(133.145231859928,33.7316503843303,19.4375236190794));
#41257=CARTESIAN_POINT('Ctrl Pts',(133.001643736974,33.4048179298836,19.4181281512654));
#41258=CARTESIAN_POINT('Ctrl Pts',(132.874208001904,33.1852299619745,19.4050647672162));
#41259=CARTESIAN_POINT('Ctrl Pts',(132.6849716892,32.9298488920332,19.3878357014475));
#41260=CARTESIAN_POINT('Ctrl Pts',(132.644936544191,32.8789369577672,19.3842823130487));
#41261=CARTESIAN_POINT('Ctrl Pts',(132.575117343171,32.7952016260257,19.378177452747));
#41262=CARTESIAN_POINT('Ctrl Pts',(132.546102549189,32.7617581393349,19.3756650870185));
#41263=CARTESIAN_POINT('Ctrl Pts',(132.503296450845,32.714327902328,19.371977315955));
#41264=CARTESIAN_POINT('Ctrl Pts',(132.490024432862,32.6998764505742,19.3708364209009));
#41265=CARTESIAN_POINT('Ctrl Pts',(132.46652399942,32.6747293889774,19.3688189032017));
#41266=CARTESIAN_POINT('Ctrl Pts',(132.456349846543,32.6639842737757,19.3679462246099));
#41267=CARTESIAN_POINT('Ctrl Pts',(132.433566691075,32.6402359734058,19.3659933978659));
#41268=CARTESIAN_POINT('Ctrl Pts',(132.420923784493,32.627267166686,19.3649108086282));
#41269=CARTESIAN_POINT('Ctrl Pts',(132.382828919204,32.5888117526327,19.3616537484923));
#41270=CARTESIAN_POINT('Ctrl Pts',(132.35707478753,32.5636296165956,19.3594582945023));
#41271=CARTESIAN_POINT('Ctrl Pts',(132.221046275514,32.4347979361299,19.347918580759));
#41272=CARTESIAN_POINT('Ctrl Pts',(132.104329592541,32.3382152625028,19.3382127669818));
#41273=CARTESIAN_POINT('Ctrl Pts',(131.873582654614,32.1719608252962,19.3198902792961));
#41274=CARTESIAN_POINT('Ctrl Pts',(131.761110457621,32.1005845308409,19.3112980290594));
#41275=CARTESIAN_POINT('Ctrl Pts',(131.519273404115,31.9663884424842,19.2937356517235));
#41276=CARTESIAN_POINT('Ctrl Pts',(131.389512599476,31.9048014737679,19.2848074402785));
#41277=CARTESIAN_POINT('Ctrl Pts',(131.21703212536,31.8359806477901,19.2736057126022));
#41278=CARTESIAN_POINT('Ctrl Pts',(131.177549883331,31.8210753125312,19.271084092216));
#41279=CARTESIAN_POINT('Ctrl Pts',(131.111503703831,31.7975409807139,19.2669344341869));
#41280=CARTESIAN_POINT('Ctrl Pts',(131.085093875232,31.7884963637949,19.2652930201818));
#41281=CARTESIAN_POINT('Ctrl Pts',(131.032938182203,31.7713513618545,19.2620855462872));
#41282=CARTESIAN_POINT('Ctrl Pts',(131.007201388366,31.7632301994539,19.260518913496));
#41283=CARTESIAN_POINT('Ctrl Pts',(130.950128104293,31.7459675809355,19.2570789735167));
#41284=CARTESIAN_POINT('Ctrl Pts',(130.918750827823,31.7369695956267,19.2552103495467));
#41285=CARTESIAN_POINT('Ctrl Pts',(130.808833596239,31.7071601493692,19.248738127973));
#41286=CARTESIAN_POINT('Ctrl Pts',(130.72967672223,31.6887193812411,19.2442083350159));
#41287=CARTESIAN_POINT('Ctrl Pts',(130.375379926847,31.6195046218141,19.2243840733658));
#41288=CARTESIAN_POINT('Ctrl Pts',(130.095267838498,31.6000627146817,19.2100006264721));
#41289=CARTESIAN_POINT('Ctrl Pts',(129.749159321002,31.6188819426312,19.1912383501271));
#41290=CARTESIAN_POINT('Ctrl Pts',(129.682485705748,31.6244905362487,19.1875727259415));
#41291=CARTESIAN_POINT('Ctrl Pts',(129.571009799945,31.6371997976817,19.1812958833176));
#41292=CARTESIAN_POINT('Ctrl Pts',(129.526103981189,31.6432337067365,19.1787267069632));
#41293=CARTESIAN_POINT('Ctrl Pts',(129.461771518752,31.6531944985399,19.1749704832532));
#41294=CARTESIAN_POINT('Ctrl Pts',(129.44223558273,31.6563947935735,19.1738197457957));
#41295=CARTESIAN_POINT('Ctrl Pts',(129.408000793346,31.6623113670737,19.1717837322616));
#41296=CARTESIAN_POINT('Ctrl Pts',(129.393290128869,31.6649540345882,19.1709024567523));
#41297=CARTESIAN_POINT('Ctrl Pts',(129.360859074363,31.6710017252495,19.1689450798905));
#41298=CARTESIAN_POINT('Ctrl Pts',(129.34314831837,31.6744509517548,19.1678667074907));
#41299=CARTESIAN_POINT('Ctrl Pts',(129.291571290214,31.6849238210788,19.1647003864993));
#41300=CARTESIAN_POINT('Ctrl Pts',(129.257784896839,31.6923244036375,19.162593565563));
#41301=CARTESIAN_POINT('Ctrl Pts',(129.040878762479,31.7433260956211,19.148882121011));
#41302=CARTESIAN_POINT('Ctrl Pts',(128.861558937872,31.8015972045417,19.1367083555732));
#41303=CARTESIAN_POINT('Ctrl Pts',(128.543161218256,31.9352477836216,19.1144553900244));
#41304=CARTESIAN_POINT('Ctrl Pts',(128.402697262378,32.006053317412,19.1043862980713));
#41305=CARTESIAN_POINT('Ctrl Pts',(128.185600072744,32.1351320462352,19.0886319858509));
#41306=CARTESIAN_POINT('Ctrl Pts',(128.105649233421,32.1873583046328,19.0827812912004));
#41307=CARTESIAN_POINT('Ctrl Pts',(127.997684446767,32.2645791948164,19.0748138624817));
#41308=CARTESIAN_POINT('Ctrl Pts',(127.967724402689,32.2867638106526,19.0725951371822));
#41309=CARTESIAN_POINT('Ctrl Pts',(127.916708904024,32.3258586460368,19.068802150162));
#41310=CARTESIAN_POINT('Ctrl Pts',(127.89547881506,32.3425342116142,19.067219076462));
#41311=CARTESIAN_POINT('Ctrl Pts',(127.852330015534,32.3772676416313,19.0639910175615));
#41312=CARTESIAN_POINT('Ctrl Pts',(127.830434449913,32.3953509294012,19.0623472121573));
#41313=CARTESIAN_POINT('Ctrl Pts',(127.774750041403,32.4425294494292,19.058149906065));
#41314=CARTESIAN_POINT('Ctrl Pts',(127.741302807031,32.4720205210908,19.0556125216747));
#41315=CARTESIAN_POINT('Ctrl Pts',(127.579358418923,32.6205908415125,19.0432273776828));
#41316=CARTESIAN_POINT('Ctrl Pts',(127.459639173474,32.7488514927911,19.0337718430185));
#41317=CARTESIAN_POINT('Ctrl Pts',(127.251122778964,33.0101769008517,19.0159734992701));
#41318=CARTESIAN_POINT('Ctrl Pts',(127.160767145408,33.1413779889753,19.0076257709077));
#41319=CARTESIAN_POINT('Ctrl Pts',(127.043624215135,33.3400702720867,18.9951759296494));
#41320=CARTESIAN_POINT('Ctrl Pts',(127.009248185643,33.4028378244243,18.9912669950647));
#41321=CARTESIAN_POINT('Ctrl Pts',(126.955399667325,33.5090036900048,18.984619844174));
#41322=CARTESIAN_POINT('Ctrl Pts',(126.934807447617,33.5518096346547,18.9819303912349));
#41323=CARTESIAN_POINT('Ctrl Pts',(126.906767773882,33.6133761243421,18.9780296576747));
#41324=CARTESIAN_POINT('Ctrl Pts',(126.8985771034,33.6317941125114,18.9768586467859));
#41325=CARTESIAN_POINT('Ctrl Pts',(126.88458751446,33.6640230359214,18.974800619948));
#41326=CARTESIAN_POINT('Ctrl Pts',(126.878715093955,33.6778011007988,18.9739179233641));
#41327=CARTESIAN_POINT('Ctrl Pts',(126.866067290281,33.7080296737048,18.9719745837945));
#41328=CARTESIAN_POINT('Ctrl Pts',(126.8593300736,33.7244946352306,18.9709119097829));
#41329=CARTESIAN_POINT('Ctrl Pts',(126.840325171231,33.7720039581988,18.9678352076368));
#41330=CARTESIAN_POINT('Ctrl Pts',(126.828386367307,33.8031766683817,18.9658038103239));
#41331=CARTESIAN_POINT('Ctrl Pts',(126.745805523571,34.0287164216908,18.9510412492212));
#41332=CARTESIAN_POINT('Ctrl Pts',(126.69262624817,34.2289997088213,18.9376151077583));
#41333=CARTESIAN_POINT('Ctrl Pts',(126.626335361854,34.6196328651339,18.9121062604779));
#41334=CARTESIAN_POINT('Ctrl Pts',(126.610349292147,34.8087500903616,18.9000496557075));
#41335=CARTESIAN_POINT('Ctrl Pts',(126.610221451071,35.0538508416271,18.8850414854699));
#41336=CARTESIAN_POINT('Ctrl Pts',(126.611561327143,35.1094642706032,18.8816749265113));
#41337=CARTESIAN_POINT('Ctrl Pts',(126.615917242948,35.1988338719619,18.8763258610371));
#41338=CARTESIAN_POINT('Ctrl Pts',(126.618071689148,35.232619947923,18.8743176435631));
#41339=CARTESIAN_POINT('Ctrl Pts',(126.622816080097,35.2928092606606,18.8707637878997));
#41340=CARTESIAN_POINT('Ctrl Pts',(126.625210499963,35.3192246571491,18.8692122757323));
#41341=CARTESIAN_POINT('Ctrl Pts',(126.630964759736,35.3753684772599,18.8659310449551));
#41342=CARTESIAN_POINT('Ctrl Pts',(126.634408632626,35.4050861321382,18.8642040567425));
#41343=CARTESIAN_POINT('Ctrl Pts',(126.644909116979,35.4862814016571,18.8595099690902));
#41344=CARTESIAN_POINT('Ctrl Pts',(126.652756686038,35.5376495456957,18.856567332348));
#41345=CARTESIAN_POINT('Ctrl Pts',(126.690907102404,35.7539373965398,18.8442657023842));
#41346=CARTESIAN_POINT('Ctrl Pts',(126.73224342609,35.9166743742564,18.8352430771744));
#41347=CARTESIAN_POINT('Ctrl Pts',(126.796850563314,36.1097421483453,18.8244143192971));
#41348=CARTESIAN_POINT('Ctrl Pts',(126.808780385848,36.1435951764742,18.8225100726071));
#41349=CARTESIAN_POINT('Ctrl Pts',(126.821241895921,36.1772433810614,18.8206074156907));
#41350=CARTESIAN_POINT('',(126.610251372965,35.0022124562256,19.2361965387239));
#41351=CARTESIAN_POINT('Ctrl Pts',(126.821241918361,36.1772434416541,19.1602707349979));
#41352=CARTESIAN_POINT('Ctrl Pts',(126.816884277129,36.1654770670927,19.1610210740581));
#41353=CARTESIAN_POINT('Ctrl Pts',(126.81259205494,36.1536867351834,19.1617750013141));
#41354=CARTESIAN_POINT('Ctrl Pts',(126.79345944527,36.1002094234563,19.1652030231718));
#41355=CARTESIAN_POINT('Ctrl Pts',(126.779371421115,36.0582600185024,19.1679151873821));
#41356=CARTESIAN_POINT('Ctrl Pts',(126.746713334263,35.9543155480196,19.174672025003));
#41357=CARTESIAN_POINT('Ctrl Pts',(126.729090018245,35.892042234783,19.1787514066441));
#41358=CARTESIAN_POINT('Ctrl Pts',(126.645037231307,35.5589208321272,19.2006150216373));
#41359=CARTESIAN_POINT('Ctrl Pts',(126.610433081745,35.281113965657,19.2188765528856));
#41360=CARTESIAN_POINT('Ctrl Pts',(126.610250724592,35.0022163872186,19.2361974238064));
#41361=CARTESIAN_POINT('Ctrl Pts',(126.61025072207,35.002212526495,19.2361976635757));
#41362=CARTESIAN_POINT('Ctrl Pts',(126.610215475997,34.9482130149684,19.2395512894302));
#41363=CARTESIAN_POINT('Ctrl Pts',(126.611470566056,34.8942177721856,19.242871423061));
#41364=CARTESIAN_POINT('Ctrl Pts',(126.615959719839,34.7990542651036,19.2486629964747));
#41365=CARTESIAN_POINT('Ctrl Pts',(126.618656662605,34.7578734542219,19.2511494081819));
#41366=CARTESIAN_POINT('Ctrl Pts',(126.624315581862,34.6903878890029,19.2551924379648));
#41367=CARTESIAN_POINT('Ctrl Pts',(126.626834801365,34.6640512652279,19.2567623423169));
#41368=CARTESIAN_POINT('Ctrl Pts',(126.632351176298,34.6127279931673,19.2598068611335));
#41369=CARTESIAN_POINT('Ctrl Pts',(126.635318749466,34.5877399604904,19.2612822844822));
#41370=CARTESIAN_POINT('Ctrl Pts',(126.64220756733,34.5347765169189,19.2643957347701));
#41371=CARTESIAN_POINT('Ctrl Pts',(126.64620082992,34.506812300338,19.2660314093717));
#41372=CARTESIAN_POINT('Ctrl Pts',(126.657283871333,34.4355741254906,19.2701791168379));
#41373=CARTESIAN_POINT('Ctrl Pts',(126.664864724642,34.3923811822919,19.2726757978637));
#41374=CARTESIAN_POINT('Ctrl Pts',(126.703952825049,34.1925282584387,19.2841595650102));
#41375=CARTESIAN_POINT('Ctrl Pts',(126.745675022395,34.0380675173494,19.2928265120144));
#41376=CARTESIAN_POINT('Ctrl Pts',(126.846191473988,33.7488743124589,19.3091736487917));
#41377=CARTESIAN_POINT('Ctrl Pts',(126.903141208669,33.6138945107815,19.3168610374973));
#41378=CARTESIAN_POINT('Ctrl Pts',(127.00896571753,33.4024266075271,19.32951259195));
#41379=CARTESIAN_POINT('Ctrl Pts',(127.052492408531,33.3234785901044,19.3343850312158));
#41380=CARTESIAN_POINT('Ctrl Pts',(127.118914203371,33.2136027453504,19.3415086168363));
#41381=CARTESIAN_POINT('Ctrl Pts',(127.139271258006,33.1811813274849,19.3436550925338));
#41382=CARTESIAN_POINT('Ctrl Pts',(127.176554363478,33.1239776239996,19.3475351285399));
#41383=CARTESIAN_POINT('Ctrl Pts',(127.193268909451,33.0990618967346,19.3492574520608));
#41384=CARTESIAN_POINT('Ctrl Pts',(127.219904039347,33.0604751456602,19.3519811636848));
#41385=CARTESIAN_POINT('Ctrl Pts',(127.229600213642,33.0466502596012,19.3529685483001));
#41386=CARTESIAN_POINT('Ctrl Pts',(127.24822240275,33.0205161538322,19.3548582693453));
#41387=CARTESIAN_POINT('Ctrl Pts',(127.257128544283,33.0081936879496,19.3557593455908));
#41388=CARTESIAN_POINT('Ctrl Pts',(127.27903030596,32.9783160342607,19.3579681317384));
#41389=CARTESIAN_POINT('Ctrl Pts',(127.29211316751,32.960825907217,19.3592815020715));
#41390=CARTESIAN_POINT('Ctrl Pts',(127.338673867667,32.8998183941126,19.363931200705));
#41391=CARTESIAN_POINT('Ctrl Pts',(127.373037585497,32.8569910574747,19.3673193409019));
#41392=CARTESIAN_POINT('Ctrl Pts',(127.538429896875,32.6608214414603,19.3833578502994));
#41393=CARTESIAN_POINT('Ctrl Pts',(127.681933424734,32.5185394030912,19.3964933842812));
#41394=CARTESIAN_POINT('Ctrl Pts',(127.868724280745,32.3637636657869,19.4120639340809));
#41395=CARTESIAN_POINT('Ctrl Pts',(127.900691026352,32.3382373999543,19.4146815651004));
#41396=CARTESIAN_POINT('Ctrl Pts',(128.056011306919,32.2187491707369,19.4271647980074));
#41397=CARTESIAN_POINT('Ctrl Pts',(128.185264214849,32.1327377679348,19.436844872648));
#41398=CARTESIAN_POINT('Ctrl Pts',(128.357316725156,32.0345580619004,19.4488028814114));
#41399=CARTESIAN_POINT('Ctrl Pts',(128.395068961342,32.0139573268592,19.4513741070718));
#41400=CARTESIAN_POINT('Ctrl Pts',(128.458100352968,31.9811030575805,19.4555826658498));
#41401=CARTESIAN_POINT('Ctrl Pts',(128.483157179875,31.9684358492142,19.4572341720212));
#41402=CARTESIAN_POINT('Ctrl Pts',(128.532503490119,31.9442543629499,19.4604457364178));
#41403=CARTESIAN_POINT('Ctrl Pts',(128.556778206111,31.932714829135,19.4620065706786));
#41404=CARTESIAN_POINT('Ctrl Pts',(128.610418075977,31.9079936926775,19.4654152814497));
#41405=CARTESIAN_POINT('Ctrl Pts',(128.639839081657,31.8949390819526,19.4672587930637));
#41406=CARTESIAN_POINT('Ctrl Pts',(128.741511200457,31.8515478495679,19.4735446997745));
#41407=CARTESIAN_POINT('Ctrl Pts',(128.814628140774,31.823297336191,19.4779189981552));
#41408=CARTESIAN_POINT('Ctrl Pts',(129.113363869955,31.7196261181302,19.4953116820124));
#41409=CARTESIAN_POINT('Ctrl Pts',(129.345642425038,31.6655142638856,19.5077026835536));
#41410=CARTESIAN_POINT('Ctrl Pts',(129.676644533757,31.6243512293255,19.525513086473));
#41411=CARTESIAN_POINT('Ctrl Pts',(129.772064593741,31.6165687833369,19.5306728352778));
#41412=CARTESIAN_POINT('Ctrl Pts',(129.90737668874,31.6112828082849,19.538173803025));
#41413=CARTESIAN_POINT('Ctrl Pts',(129.947095925998,31.6104300863342,19.5403981242804));
#41414=CARTESIAN_POINT('Ctrl Pts',(130.01768011138,31.610155626858,19.5444049381334));
#41415=CARTESIAN_POINT('Ctrl Pts',(130.04853988523,31.6104570811399,19.5461750907755));
#41416=CARTESIAN_POINT('Ctrl Pts',(130.096452395897,31.611579530182,19.5489577493476));
#41417=CARTESIAN_POINT('Ctrl Pts',(130.113511052364,31.6121080951875,19.5499552468336));
#41418=CARTESIAN_POINT('Ctrl Pts',(130.145695236496,31.6133486690801,19.5518511789087));
#41419=CARTESIAN_POINT('Ctrl Pts',(130.160821042584,31.6140332403618,19.5527481627375));
#41420=CARTESIAN_POINT('Ctrl Pts',(130.197356008177,31.6159321086878,19.5549285505349));
#41421=CARTESIAN_POINT('Ctrl Pts',(130.218758977666,31.6172482585219,19.5562172644105));
#41422=CARTESIAN_POINT('Ctrl Pts',(130.292321933773,31.6224729663525,19.5606825525034));
#41423=CARTESIAN_POINT('Ctrl Pts',(130.344400844976,31.6273855222876,19.563905875816));
#41424=CARTESIAN_POINT('Ctrl Pts',(130.598851739203,31.6573423427301,19.5798944445524));
#41425=CARTESIAN_POINT('Ctrl Pts',(130.798788946252,31.6994068819552,19.5931753681602));
#41426=CARTESIAN_POINT('Ctrl Pts',(131.037416819557,31.7725769276712,19.6091988973403));
#41427=CARTESIAN_POINT('Ctrl Pts',(131.080832171088,31.7868558527562,19.6121229553687));
#41428=CARTESIAN_POINT('Ctrl Pts',(131.267340977157,31.8524050832161,19.6247062034626));
#41429=CARTESIAN_POINT('Ctrl Pts',(131.40719715903,31.9123936512726,19.6341869007031));
#41430=CARTESIAN_POINT('Ctrl Pts',(131.580681828565,32.0010531908516,19.6459455090507));
#41431=CARTESIAN_POINT('Ctrl Pts',(131.618423355812,32.0212514204674,19.6485043627907));
#41432=CARTESIAN_POINT('Ctrl Pts',(131.680236057183,32.0558536396961,19.6526982152746));
#41433=CARTESIAN_POINT('Ctrl Pts',(131.70452825394,32.0698507715849,19.6543471872561));
#41434=CARTESIAN_POINT('Ctrl Pts',(131.751785854678,32.0978671435549,19.6575576304384));
#41435=CARTESIAN_POINT('Ctrl Pts',(131.774763468423,32.111861587575,19.659119827834));
#41436=CARTESIAN_POINT('Ctrl Pts',(131.824951892556,32.1432538505546,19.6625360124278));
#41437=CARTESIAN_POINT('Ctrl Pts',(131.852085745882,32.1607700931624,19.6643855583066));
#41438=CARTESIAN_POINT('Ctrl Pts',(131.945453727437,32.2229518873537,19.6707635209743));
#41439=CARTESIAN_POINT('Ctrl Pts',(132.010358611324,32.2695703624621,19.6752207033964));
#41440=CARTESIAN_POINT('Ctrl Pts',(132.296512356373,32.490843439481,19.6951027662234));
#41441=CARTESIAN_POINT('Ctrl Pts',(132.497079056264,32.6903631863241,19.7095900446456));
#41442=CARTESIAN_POINT('Ctrl Pts',(132.71193065259,32.9652192616336,19.7284720558489));
#41443=CARTESIAN_POINT('Ctrl Pts',(132.751644429959,33.0192545477198,19.7321455607671));
#41444=CARTESIAN_POINT('Ctrl Pts',(132.815505665414,33.1117753924046,19.738434448976));
#41445=CARTESIAN_POINT('Ctrl Pts',(132.840529738639,33.149633897141,19.7410075794933));
#41446=CARTESIAN_POINT('Ctrl Pts',(132.875373842545,33.204722109738,19.7447685587133));
#41447=CARTESIAN_POINT('Ctrl Pts',(132.885815397581,33.2215549241941,19.7459199700929));
#41448=CARTESIAN_POINT('Ctrl Pts',(132.903876512259,33.2512490999676,19.7479567284362));
#41449=CARTESIAN_POINT('Ctrl Pts',(132.911559461917,33.26407085494,19.7488380645543));
#41450=CARTESIAN_POINT('Ctrl Pts',(132.928325555692,33.2924755344085,19.7507950343929));
#41451=CARTESIAN_POINT('Ctrl Pts',(132.937369181284,33.3080801965146,19.751872931568));
#41452=CARTESIAN_POINT('Ctrl Pts',(132.963908493675,33.3547276074281,19.7551016980135));
#41453=CARTESIAN_POINT('Ctrl Pts',(132.981039163648,33.3859739491876,19.7572730398491));
#41454=CARTESIAN_POINT('Ctrl Pts',(133.065042432382,33.5450966522167,19.7683519239015));
#41455=CARTESIAN_POINT('Ctrl Pts',(133.12418869657,33.6768721730859,19.7775891689094));
#41456=CARTESIAN_POINT('Ctrl Pts',(133.218141340569,33.9279473334658,19.7948513252321));
#41457=CARTESIAN_POINT('Ctrl Pts',(133.255145042948,34.0461850538247,19.8028503594678));
#41458=CARTESIAN_POINT('Ctrl Pts',(133.311610149504,34.268682164028,19.8174851066821));
#41459=CARTESIAN_POINT('Ctrl Pts',(133.332813066236,34.3723475531884,19.8241425327511));
#41460=CARTESIAN_POINT('Ctrl Pts',(133.360583704125,34.550128626364,19.8352447292932));
#41461=CARTESIAN_POINT('Ctrl Pts',(133.369623624833,34.6237753526897,19.8397542238034));
#41462=CARTESIAN_POINT('Ctrl Pts',(133.37927968976,34.7316063198114,19.8462282611237));
#41463=CARTESIAN_POINT('Ctrl Pts',(133.381807227682,34.7655935342041,19.8482503908452));
#41464=CARTESIAN_POINT('Ctrl Pts',(133.38539109811,34.8261126414777,19.8518195887479));
#41465=CARTESIAN_POINT('Ctrl Pts',(133.386649027488,34.8526292949401,19.8533727220192));
#41466=CARTESIAN_POINT('Ctrl Pts',(133.388657002526,34.9089196459588,19.8566480451033));
#41467=CARTESIAN_POINT('Ctrl Pts',(133.389326419478,34.9386940821686,19.8583676302957));
#41468=CARTESIAN_POINT('Ctrl Pts',(133.390080505381,35.0197721314512,19.8630175474119));
#41469=CARTESIAN_POINT('Ctrl Pts',(133.389393065676,35.0710760452747,19.8659242135125));
#41470=CARTESIAN_POINT('Ctrl Pts',(133.378519205452,35.3721523378395,19.8828075085769));
#41471=CARTESIAN_POINT('Ctrl Pts',(133.3418949116,35.6201926046446,19.8959386289498));
#41472=CARTESIAN_POINT('Ctrl Pts',(133.248186194223,35.976596114098,19.9155099675868));
#41473=CARTESIAN_POINT('Ctrl Pts',(133.21205675139,36.0895603652594,19.9218371819471));
#41474=CARTESIAN_POINT('Ctrl Pts',(133.146694708057,36.2621733250101,19.9320033556803));
#41475=CARTESIAN_POINT('Ctrl Pts',(133.12150147322,36.3232522451485,19.9357024722337));
#41476=CARTESIAN_POINT('Ctrl Pts',(133.085256002473,36.4043212047064,19.94079961858));
#41477=CARTESIAN_POINT('Ctrl Pts',(133.075761638448,36.424995764854,19.942116272941));
#41478=CARTESIAN_POINT('Ctrl Pts',(133.059508800271,36.4594680427605,19.944342360807));
#41479=CARTESIAN_POINT('Ctrl Pts',(133.052863128391,36.4733186278345,19.9452451975962));
#41480=CARTESIAN_POINT('Ctrl Pts',(133.038870526682,36.5019801294892,19.9471318765351));
#41481=CARTESIAN_POINT('Ctrl Pts',(133.031509081146,36.5167831265571,19.9481165035166));
#41482=CARTESIAN_POINT('Ctrl Pts',(133.011235405754,36.5568139115607,19.9508057499079));
#41483=CARTESIAN_POINT('Ctrl Pts',(132.998114880788,36.5819340287823,19.9525221906066));
#41484=CARTESIAN_POINT('Ctrl Pts',(132.911121095869,36.7435190886185,19.963737286436));
#41485=CARTESIAN_POINT('Ctrl Pts',(132.828271729794,36.8749280251083,19.9736614331718));
#41486=CARTESIAN_POINT('Ctrl Pts',(132.663495844683,37.1003799075204,19.9916405905087));
#41487=CARTESIAN_POINT('Ctrl Pts',(132.584819242997,37.1964782963118,19.9996605192366));
#41488=CARTESIAN_POINT('Ctrl Pts',(132.429157746115,37.3666308130073,20.0143671888637));
#41489=CARTESIAN_POINT('Ctrl Pts',(132.353598703044,37.4417872405959,20.0210745655852));
#41490=CARTESIAN_POINT('Ctrl Pts',(132.219354394296,37.5632844868713,20.0322484271455));
#41491=CARTESIAN_POINT('Ctrl Pts',(132.162450354701,37.6114691349756,20.0367807790335));
#41492=CARTESIAN_POINT('Ctrl Pts',(132.077233120315,37.6789313407534,20.0432807784136));
#41493=CARTESIAN_POINT('Ctrl Pts',(132.05014671505,37.6997164923903,20.0453066711331));
#41494=CARTESIAN_POINT('Ctrl Pts',(132.001443936004,37.7359335193256,20.0488800443693));
#41495=CARTESIAN_POINT('Ctrl Pts',(131.979951853488,37.7515269885172,20.0504336415287));
#41496=CARTESIAN_POINT('Ctrl Pts',(131.933999042895,37.7840505623483,20.0537074751487));
#41497=CARTESIAN_POINT('Ctrl Pts',(131.909494112783,37.8009145196306,20.0554251400922));
#41498=CARTESIAN_POINT('Ctrl Pts',(131.842272486488,37.8458832343145,20.0600635680516));
#41499=CARTESIAN_POINT('Ctrl Pts',(131.799135953524,37.8733481346034,20.0629608712329));
#41500=CARTESIAN_POINT('Ctrl Pts',(131.540255949763,38.0300595587384,20.0799218042565));
#41501=CARTESIAN_POINT('Ctrl Pts',(131.311296675074,38.13594665252,20.09312732666));
#41502=CARTESIAN_POINT('Ctrl Pts',(130.912063395239,38.2691324831501,20.1154815794123));
#41503=CARTESIAN_POINT('Ctrl Pts',(130.747636453235,38.3106063008307,20.1245383787699));
#41504=CARTESIAN_POINT('Ctrl Pts',(130.551302308289,38.3447523832865,20.1358630227778));
#41505=CARTESIAN_POINT('Ctrl Pts',(130.521718428879,38.3494943635632,20.1375830440217));
#41506=CARTESIAN_POINT('Ctrl Pts',(130.475377767808,38.3562934759243,20.1403039214023));
#41507=CARTESIAN_POINT('Ctrl Pts',(130.458661187484,38.3586187350332,20.1412908218481));
#41508=CARTESIAN_POINT('Ctrl Pts',(130.426850202386,38.3628016962361,20.1431802661079));
#41509=CARTESIAN_POINT('Ctrl Pts',(130.411759624031,38.364682796465,20.1440815590659));
#41510=CARTESIAN_POINT('Ctrl Pts',(130.3749451936,38.3690204993416,20.1462918044247));
#41511=CARTESIAN_POINT('Ctrl Pts',(130.353209454592,38.3713685721479,20.1476064351758));
#41512=CARTESIAN_POINT('Ctrl Pts',(130.276685573544,38.3788871836712,20.1522652030586));
#41513=CARTESIAN_POINT('Ctrl Pts',(130.221798175942,38.3829333966169,20.1556614032598));
#41514=CARTESIAN_POINT('Ctrl Pts',(129.939814673572,38.3968291765303,20.1733101359939));
#41515=CARTESIAN_POINT('Ctrl Pts',(129.712245570642,38.385153868756,20.1881747003921));
#41516=CARTESIAN_POINT('Ctrl Pts',(129.3208767496,38.325301460879,20.2134766473903));
#41517=CARTESIAN_POINT('Ctrl Pts',(129.156310677016,38.2874062313545,20.2240419260026));
#41518=CARTESIAN_POINT('Ctrl Pts',(128.953410942571,38.2244338557998,20.2368754455562));
#41519=CARTESIAN_POINT('Ctrl Pts',(128.911845984703,38.2106453328931,20.2394950603042));
#41520=CARTESIAN_POINT('Ctrl Pts',(128.843937732295,38.1866474939306,20.2437611512652));
#41521=CARTESIAN_POINT('Ctrl Pts',(128.817435123822,38.1769077108209,20.2454225912506));
#41522=CARTESIAN_POINT('Ctrl Pts',(128.766036147631,38.1572861026596,20.2486389291301));
#41523=CARTESIAN_POINT('Ctrl Pts',(128.741129183889,38.1474381092643,20.2501947938823));
#41524=CARTESIAN_POINT('Ctrl Pts',(128.681546192648,38.1230590745161,20.2539116027744));
#41525=CARTESIAN_POINT('Ctrl Pts',(128.646989697383,38.1082441515366,20.2560629736201));
#41526=CARTESIAN_POINT('Ctrl Pts',(128.5295892068,38.0555836605759,20.2633642096277));
#41527=CARTESIAN_POINT('Ctrl Pts',(128.448024481866,38.0149748403744,20.2684222294066));
#41528=CARTESIAN_POINT('Ctrl Pts',(128.133258071286,37.8420979863815,20.2880480871323));
#41529=CARTESIAN_POINT('Ctrl Pts',(127.914475180346,37.6856699827746,20.301851211184));
#41530=CARTESIAN_POINT('Ctrl Pts',(127.667622304673,37.4606455684475,20.3199420153383));
#41531=CARTESIAN_POINT('Ctrl Pts',(127.620151193681,37.4147631596853,20.3235610891487));
#41532=CARTESIAN_POINT('Ctrl Pts',(127.542706359243,37.3354072977552,20.3297666890232));
#41533=CARTESIAN_POINT('Ctrl Pts',(127.512002969112,37.3026701152911,20.3323124026134));
#41534=CARTESIAN_POINT('Ctrl Pts',(127.468755201416,37.2546826570976,20.3360403655702));
#41535=CARTESIAN_POINT('Ctrl Pts',(127.455678794946,37.2399159983098,20.3371870531825));
#41536=CARTESIAN_POINT('Ctrl Pts',(127.432924454016,37.2137640941348,20.3392187472868));
#41537=CARTESIAN_POINT('Ctrl Pts',(127.423191772147,37.2024276759358,20.3400998173157));
#41538=CARTESIAN_POINT('Ctrl Pts',(127.401835537115,37.1772170435596,20.3420603521003));
#41539=CARTESIAN_POINT('Ctrl Pts',(127.390248090003,37.1633140240806,20.3431421393011));
#41540=CARTESIAN_POINT('Ctrl Pts',(127.356676801105,37.1223717696203,20.346327893368));
#41541=CARTESIAN_POINT('Ctrl Pts',(127.334998547728,37.0950862795405,20.3484510631975));
#41542=CARTESIAN_POINT('Ctrl Pts',(127.202225605103,36.9225752233857,20.361849984847));
#41543=CARTESIAN_POINT('Ctrl Pts',(127.102620100327,36.7689028080485,20.3736611928492));
#41544=CARTESIAN_POINT('Ctrl Pts',(126.941073937568,36.4691009803107,20.395611037577));
#41545=CARTESIAN_POINT('Ctrl Pts',(126.876029297552,36.325178709834,20.4057321322366));
#41546=CARTESIAN_POINT('Ctrl Pts',(126.821241918623,36.1772434423596,20.4155867593643));
#41547=CARTESIAN_POINT('Origin',(130.,35.,23.));
#41548=CARTESIAN_POINT('',(126.821242031451,36.1772437470164,21.6644319010721));
#41549=CARTESIAN_POINT('',(126.821241909055,36.1772434165241,21.3230640339373));
#41550=CARTESIAN_POINT('',(126.821241918358,36.1772434416438,23.));
#41551=CARTESIAN_POINT('',(126.610250158159,34.9989645099258,20.1438717258877));
#41552=CARTESIAN_POINT('Ctrl Pts',(126.821241909055,36.1772434165241,21.3230640339373));
#41553=CARTESIAN_POINT('Ctrl Pts',(126.859773903997,36.2812863773632,21.3161350653242));
#41554=CARTESIAN_POINT('Ctrl Pts',(126.903394320183,36.3833843634471,21.3090329747309));
#41555=CARTESIAN_POINT('Ctrl Pts',(127.068467069802,36.7226249430287,21.2847520874349));
#41556=CARTESIAN_POINT('Ctrl Pts',(127.212819820697,36.9475604108426,21.2675616869289));
#41557=CARTESIAN_POINT('Ctrl Pts',(127.416491132104,37.1951831280408,21.2480209068817));
#41558=CARTESIAN_POINT('Ctrl Pts',(127.451948183293,37.2362422683576,21.2447531923312));
#41559=CARTESIAN_POINT('Ctrl Pts',(127.508986235131,37.2991731708688,21.2396986178727));
#41560=CARTESIAN_POINT('Ctrl Pts',(127.52990385391,37.3216313161839,21.2378851049007));
#41561=CARTESIAN_POINT('Ctrl Pts',(127.569399031353,37.362897068256,21.2345335289934));
#41562=CARTESIAN_POINT('Ctrl Pts',(127.58789702295,37.3817772587843,21.2329922850979));
#41563=CARTESIAN_POINT('Ctrl Pts',(127.629780723482,37.4235378802346,21.2295644274639));
#41564=CARTESIAN_POINT('Ctrl Pts',(127.653280823025,37.4463001629194,21.2276829950934));
#41565=CARTESIAN_POINT('Ctrl Pts',(127.725455321044,37.5142113314142,21.2220259185415));
#41566=CARTESIAN_POINT('Ctrl Pts',(127.775131198867,37.5582751482987,21.2182951812326));
#41567=CARTESIAN_POINT('Ctrl Pts',(127.895325328536,37.6587396365478,21.2096088609643));
#41568=CARTESIAN_POINT('Ctrl Pts',(127.966866282428,37.7138387320578,21.2046993131418));
#41569=CARTESIAN_POINT('Ctrl Pts',(128.153677743463,37.8461778372522,21.1923912548147));
#41570=CARTESIAN_POINT('Ctrl Pts',(128.271644792969,37.919318963708,21.1850850707741));
#41571=CARTESIAN_POINT('Ctrl Pts',(128.542152146433,38.0648786214799,21.1687631300698));
#41572=CARTESIAN_POINT('Ctrl Pts',(128.696276544516,38.1335433499011,21.1597407285242));
#41573=CARTESIAN_POINT('Ctrl Pts',(128.881868478032,38.2001580021678,21.1485178132625));
#41574=CARTESIAN_POINT('Ctrl Pts',(128.909011949439,38.2095130934921,21.1468675771204));
#41575=CARTESIAN_POINT('Ctrl Pts',(128.95204259432,38.2237348350978,21.1442327676826));
#41576=CARTESIAN_POINT('Ctrl Pts',(128.967852925842,38.2288315848197,21.1432607386928));
#41577=CARTESIAN_POINT('Ctrl Pts',(128.99831762532,38.238405822477,21.1413790499639));
#41578=CARTESIAN_POINT('Ctrl Pts',(129.012965885151,38.2429004721552,21.1404703491986));
#41579=CARTESIAN_POINT('Ctrl Pts',(129.049227118738,38.2537583814401,21.1382119370871));
#41580=CARTESIAN_POINT('Ctrl Pts',(129.070873840434,38.2600057049292,21.1368559570382));
#41581=CARTESIAN_POINT('Ctrl Pts',(129.154484328788,38.2832356286813,21.1315928515003));
#41582=CARTESIAN_POINT('Ctrl Pts',(129.21686063471,38.2986701251505,21.1276125975374));
#41583=CARTESIAN_POINT('Ctrl Pts',(129.390261968804,38.3363815928937,21.1164673879257));
#41584=CARTESIAN_POINT('Ctrl Pts',(129.502021381481,38.3548826352365,21.1091963482551));
#41585=CARTESIAN_POINT('Ctrl Pts',(129.872530616487,38.3972950443711,21.0851686096351));
#41586=CARTESIAN_POINT('Ctrl Pts',(130.133154773504,38.3970831089794,21.0684730652064));
#41587=CARTESIAN_POINT('Ctrl Pts',(130.441009027953,38.3613134515819,21.0496518691833));
#41588=CARTESIAN_POINT('Ctrl Pts',(130.490661591863,38.3544252393884,21.0466410324632));
#41589=CARTESIAN_POINT('Ctrl Pts',(130.569305440546,38.3417314150562,21.0419096513212));
#41590=CARTESIAN_POINT('Ctrl Pts',(130.598403569848,38.3366436407367,21.0401672201116));
#41591=CARTESIAN_POINT('Ctrl Pts',(130.653567164916,38.3262534918557,21.0368784958857));
#41592=CARTESIAN_POINT('Ctrl Pts',(130.679643832563,38.3210234343219,21.0353300796019));
#41593=CARTESIAN_POINT('Ctrl Pts',(130.73941873039,38.3083011510789,21.0317937564636));
#41594=CARTESIAN_POINT('Ctrl Pts',(130.773069759708,38.3005999207,21.0298125585877));
#41595=CARTESIAN_POINT('Ctrl Pts',(130.88121963861,38.2741043937956,21.0234714993874));
#41596=CARTESIAN_POINT('Ctrl Pts',(130.955201323526,38.2532905287884,21.0191748438486));
#41597=CARTESIAN_POINT('Ctrl Pts',(131.134521171187,38.1961956236317,21.0088046393751));
#41598=CARTESIAN_POINT('Ctrl Pts',(131.238901799692,38.1572027677842,21.002808042536));
#41599=CARTESIAN_POINT('Ctrl Pts',(131.543169920483,38.0261204288703,20.9851405701074));
#41600=CARTESIAN_POINT('Ctrl Pts',(131.736196387073,37.9196551404937,20.9737041402769));
#41601=CARTESIAN_POINT('Ctrl Pts',(131.968740899677,37.7601304575795,20.958142263));
#41602=CARTESIAN_POINT('Ctrl Pts',(132.018967873357,37.7236058168674,20.9546606472044));
#41603=CARTESIAN_POINT('Ctrl Pts',(132.086300708757,37.671755720168,20.9497838716541));
#41604=CARTESIAN_POINT('Ctrl Pts',(132.104298621711,37.6576035304019,20.9484590681646));
#41605=CARTESIAN_POINT('Ctrl Pts',(132.134032912165,37.6337313382546,20.9462321289046));
#41606=CARTESIAN_POINT('Ctrl Pts',(132.145849962852,37.6241122616264,20.9453368325388));
#41607=CARTESIAN_POINT('Ctrl Pts',(132.170274514188,37.603955371336,20.9434640348684));
#41608=CARTESIAN_POINT('Ctrl Pts',(132.182870819327,37.5934050983523,20.9424857228924));
#41609=CARTESIAN_POINT('Ctrl Pts',(132.216622668194,37.5647155000754,20.9398316931834));
#41610=CARTESIAN_POINT('Ctrl Pts',(132.237631596953,37.5464065615667,20.9381446477804));
#41611=CARTESIAN_POINT('Ctrl Pts',(132.361877603458,37.4354033020382,20.9279682533703));
#41612=CARTESIAN_POINT('Ctrl Pts',(132.45956161267,37.3367080852637,20.9191370598177));
#41613=CARTESIAN_POINT('Ctrl Pts',(132.737038599959,37.0196293690367,20.8920590685854));
#41614=CARTESIAN_POINT('Ctrl Pts',(132.895867974043,36.7844559407551,20.8737590725844));
#41615=CARTESIAN_POINT('Ctrl Pts',(133.047326312648,36.4855798004533,20.8533670879347));
#41616=CARTESIAN_POINT('Ctrl Pts',(133.069903827152,36.4383448640673,20.8502169691593));
#41617=CARTESIAN_POINT('Ctrl Pts',(133.103803420997,36.3629844389975,20.8453025190111));
#41618=CARTESIAN_POINT('Ctrl Pts',(133.115857154668,36.3351990630656,20.8435138872781));
#41619=CARTESIAN_POINT('Ctrl Pts',(133.137647747116,36.2830662512792,20.8402001431143));
#41620=CARTESIAN_POINT('Ctrl Pts',(133.1474775322,36.2587603550308,20.8386720278866));
#41621=CARTESIAN_POINT('Ctrl Pts',(133.169092669416,36.20347624448,20.8352331414668));
#41622=CARTESIAN_POINT('Ctrl Pts',(133.180707762597,36.1724340742095,20.8333280839539));
#41623=CARTESIAN_POINT('Ctrl Pts',(133.21501571764,36.076479003973,20.8275144436089));
#41624=CARTESIAN_POINT('Ctrl Pts',(133.236190933134,36.0110401764402,20.8236546678834));
#41625=CARTESIAN_POINT('Ctrl Pts',(133.28180126676,35.8539203223413,20.8145961836113));
#41626=CARTESIAN_POINT('Ctrl Pts',(133.304407701448,35.7617682263128,20.809449534563));
#41627=CARTESIAN_POINT('Ctrl Pts',(133.349653796137,35.5369453069032,20.7971459936452));
#41628=CARTESIAN_POINT('Ctrl Pts',(133.368317781167,35.403641728636,20.7900615511808));
#41629=CARTESIAN_POINT('Ctrl Pts',(133.392117086667,35.1053354404899,20.7741527820009));
#41630=CARTESIAN_POINT('Ctrl Pts',(133.393226501035,34.9403686561349,20.7653174067637));
#41631=CARTESIAN_POINT('Ctrl Pts',(133.380454588038,34.747519728963,20.7543148342302));
#41632=CARTESIAN_POINT('Ctrl Pts',(133.37820921087,34.7190695405162,20.7526741829412));
#41633=CARTESIAN_POINT('Ctrl Pts',(133.374092343868,34.6741462786159,20.7500511983063));
#41634=CARTESIAN_POINT('Ctrl Pts',(133.372458705202,34.6576521517151,20.7490812203024));
#41635=CARTESIAN_POINT('Ctrl Pts',(133.369080253733,34.6259162492986,20.747200458455));
#41636=CARTESIAN_POINT('Ctrl Pts',(133.367352831741,34.610673298244,20.746290592111));
#41637=CARTESIAN_POINT('Ctrl Pts',(133.362821118539,34.5729738311149,20.7440248689902));
#41638=CARTESIAN_POINT('Ctrl Pts',(133.359895304586,34.5505328647262,20.7426626541281));
#41639=CARTESIAN_POINT('Ctrl Pts',(133.347686779179,34.463686173746,20.7373427594258));
#41640=CARTESIAN_POINT('Ctrl Pts',(133.336775458194,34.399527092683,20.7333100066618));
#41641=CARTESIAN_POINT('Ctrl Pts',(133.301371734932,34.2223668785452,20.7219583603378));
#41642=CARTESIAN_POINT('Ctrl Pts',(133.272934966972,34.1102456245439,20.7145292406759));
#41643=CARTESIAN_POINT('Ctrl Pts',(133.163511984265,33.7559135697023,20.6906320529056));
#41644=CARTESIAN_POINT('Ctrl Pts',(133.060876093169,33.5212720577741,20.6742366225189));
#41645=CARTESIAN_POINT('Ctrl Pts',(132.907439745488,33.2565070191544,20.6556449589559));
#41646=CARTESIAN_POINT('Ctrl Pts',(132.88104667393,33.2132308134881,20.6525993914144));
#41647=CARTESIAN_POINT('Ctrl Pts',(132.83768829327,33.1455972621944,20.6478268030638));
#41648=CARTESIAN_POINT('Ctrl Pts',(132.821357398191,33.1208441046411,20.6460772340298));
#41649=CARTESIAN_POINT('Ctrl Pts',(132.789781765757,33.0743238296701,20.6427826614634));
#41650=CARTESIAN_POINT('Ctrl Pts',(132.774601874469,33.052515594185,20.6412354241289));
#41651=CARTESIAN_POINT('Ctrl Pts',(132.739239630386,33.0029651817673,20.6377123150111));
#41652=CARTESIAN_POINT('Ctrl Pts',(132.718889245161,32.9753461498168,20.6357429701379));
#41653=CARTESIAN_POINT('Ctrl Pts',(132.652402776801,32.8879230786819,20.6294865179868));
#41654=CARTESIAN_POINT('Ctrl Pts',(132.604684550671,32.8293482663888,20.625260173382));
#41655=CARTESIAN_POINT('Ctrl Pts',(132.483691850073,32.6905693739704,20.615106945444));
#41656=CARTESIAN_POINT('Ctrl Pts',(132.408442874244,32.6121976473872,20.609252488354));
#41657=CARTESIAN_POINT('Ctrl Pts',(132.181477407186,32.3974791597942,20.5925767954797));
#41658=CARTESIAN_POINT('Ctrl Pts',(132.021070943205,32.271040157098,20.5819558147157));
#41659=CARTESIAN_POINT('Ctrl Pts',(131.784297425951,32.1167915523867,20.5665191552995));
#41660=CARTESIAN_POINT('Ctrl Pts',(131.716831735546,32.0761164095478,20.5621417253791));
#41661=CARTESIAN_POINT('Ctrl Pts',(131.626327066921,32.0257637355334,20.5562158652508));
#41662=CARTESIAN_POINT('Ctrl Pts',(131.6045068089,32.0139358833589,20.5547831804933));
#41663=CARTESIAN_POINT('Ctrl Pts',(131.569987930202,31.995712222606,20.5525074075938));
#41664=CARTESIAN_POINT('Ctrl Pts',(131.557375158093,31.9891546450765,20.5516739359601));
#41665=CARTESIAN_POINT('Ctrl Pts',(131.530878723303,31.975589767939,20.5499182048072));
#41666=CARTESIAN_POINT('Ctrl Pts',(131.516987548718,31.968598399602,20.5489949393953));
#41667=CARTESIAN_POINT('Ctrl Pts',(131.481777788953,31.951180088561,20.5466486102724));
#41668=CARTESIAN_POINT('Ctrl Pts',(131.460397114415,31.9408810962929,20.5452182023479));
#41669=CARTESIAN_POINT('Ctrl Pts',(131.371145206879,31.8990376669984,20.5392291788145));
#41670=CARTESIAN_POINT('Ctrl Pts',(131.302350761252,31.8695228087357,20.5345705861357));
#41671=CARTESIAN_POINT('Ctrl Pts',(131.095389043063,31.7887328491178,20.5205443409293));
#41672=CARTESIAN_POINT('Ctrl Pts',(130.95479400898,31.7441622139968,20.5110080389748));
#41673=CARTESIAN_POINT('Ctrl Pts',(130.611692869122,31.6595367409439,20.4882519648145));
#41674=CARTESIAN_POINT('Ctrl Pts',(130.407528221975,31.6285306872071,20.4751468618438));
#41675=CARTESIAN_POINT('Ctrl Pts',(130.148915167921,31.6131083825935,20.4593722385477));
#41676=CARTESIAN_POINT('Ctrl Pts',(130.095973493688,31.6111948836301,20.4561835158768));
#41677=CARTESIAN_POINT('Ctrl Pts',(130.012590694451,31.610136905362,20.4512230206748));
#41678=CARTESIAN_POINT('Ctrl Pts',(129.982170472456,31.6101603984439,20.4494261852978));
#41679=CARTESIAN_POINT('Ctrl Pts',(129.92530224412,31.6109698819658,20.446090163745));
#41680=CARTESIAN_POINT('Ctrl Pts',(129.898855346249,31.6116560515182,20.4445480376383));
#41681=CARTESIAN_POINT('Ctrl Pts',(129.839362280935,31.6138968034491,20.4410987729732));
#41682=CARTESIAN_POINT('Ctrl Pts',(129.806325140639,31.6156256865156,20.4391971252134));
#41683=CARTESIAN_POINT('Ctrl Pts',(129.705056377855,31.6224130111299,20.4334062744793));
#41684=CARTESIAN_POINT('Ctrl Pts',(129.636946332503,31.6290537658916,20.4295653003918));
#41685=CARTESIAN_POINT('Ctrl Pts',(129.475680747019,31.6497222200078,20.4205614437672));
#41686=CARTESIAN_POINT('Ctrl Pts',(129.382816476291,31.6655798147327,20.4154497086736));
#41687=CARTESIAN_POINT('Ctrl Pts',(129.077472695527,31.7309162045898,20.3986922981087));
#41688=CARTESIAN_POINT('Ctrl Pts',(128.869130297171,31.7970184268176,20.3873681541716));
#41689=CARTESIAN_POINT('Ctrl Pts',(128.587761860459,31.9171906427938,20.3707332724647));
#41690=CARTESIAN_POINT('Ctrl Pts',(128.508312514633,31.954840539049,20.3658698027734));
#41691=CARTESIAN_POINT('Ctrl Pts',(128.407672868194,32.0074161413867,20.3593810107789));
#41692=CARTESIAN_POINT('Ctrl Pts',(128.38505984811,32.0195584107695,20.357900896062));
#41693=CARTESIAN_POINT('Ctrl Pts',(128.348615685208,32.0396639487203,20.3554758637301));
#41694=CARTESIAN_POINT('Ctrl Pts',(128.334698658286,32.047470387921,20.354540308711));
#41695=CARTESIAN_POINT('Ctrl Pts',(128.307145219324,32.0631826410323,20.3526680653655));
#41696=CARTESIAN_POINT('Ctrl Pts',(128.293507841715,32.0710858673643,20.3517315367736));
#41697=CARTESIAN_POINT('Ctrl Pts',(128.258594996109,32.0916453962602,20.3493094458053));
#41698=CARTESIAN_POINT('Ctrl Pts',(128.237402478598,32.1044399871423,20.3478156042256));
#41699=CARTESIAN_POINT('Ctrl Pts',(128.143631372421,32.1624634244914,20.3411064620515));
#41700=CARTESIAN_POINT('Ctrl Pts',(128.07264436121,32.2101942251539,20.335760233844));
#41701=CARTESIAN_POINT('Ctrl Pts',(127.848305813625,32.3736878745157,20.3181572849215));
#41702=CARTESIAN_POINT('Ctrl Pts',(127.702966406556,32.4998118061851,20.3056452067832));
#41703=CARTESIAN_POINT('Ctrl Pts',(127.453505989063,32.756502987286,20.2827775880254));
#41704=CARTESIAN_POINT('Ctrl Pts',(127.346793561227,32.8837725196323,20.2723879688226));
#41705=CARTESIAN_POINT('Ctrl Pts',(127.223880129731,33.0543556399103,20.2596804544436));
#41706=CARTESIAN_POINT('Ctrl Pts',(127.198651510759,33.090858718767,20.2570250430092));
#41707=CARTESIAN_POINT('Ctrl Pts',(127.158487004763,33.1514836200856,20.2527163680742));
#41708=CARTESIAN_POINT('Ctrl Pts',(127.143124962111,33.1753153697732,20.2510475468043));
#41709=CARTESIAN_POINT('Ctrl Pts',(127.113710024129,33.2222302374069,20.2478096195621));
#41710=CARTESIAN_POINT('Ctrl Pts',(127.099630619469,33.2452941351801,20.2462396326081));
#41711=CARTESIAN_POINT('Ctrl Pts',(127.06671350127,33.300695515867,20.2425186396044));
#41712=CARTESIAN_POINT('Ctrl Pts',(127.048132349975,33.3331817892836,20.2403768604267));
#41713=CARTESIAN_POINT('Ctrl Pts',(126.983557705921,33.450548501849,20.2327741049604));
#41714=CARTESIAN_POINT('Ctrl Pts',(126.940654870642,33.5370804321079,20.2274191296354));
#41715=CARTESIAN_POINT('Ctrl Pts',(126.795984085469,33.8631679062537,20.207957924295));
#41716=CARTESIAN_POINT('Ctrl Pts',(126.718206510932,34.1123465852793,20.1945374888264));
#41717=CARTESIAN_POINT('Ctrl Pts',(126.651263973486,34.4650764323385,20.1751129278367));
#41718=CARTESIAN_POINT('Ctrl Pts',(126.637091299803,34.5629439251915,20.1696701320848));
#41719=CARTESIAN_POINT('Ctrl Pts',(126.62457323614,34.687592483876,20.1625187030953));
#41720=CARTESIAN_POINT('Ctrl Pts',(126.622238986294,34.7139322864057,20.1609951523383));
#41721=CARTESIAN_POINT('Ctrl Pts',(126.618977841705,34.7563727802128,20.1585166094253));
#41722=CARTESIAN_POINT('Ctrl Pts',(126.617857237686,34.7724579839795,20.1575717579423));
#41723=CARTESIAN_POINT('Ctrl Pts',(126.615979814494,34.8024963275471,20.1557960863792));
#41724=CARTESIAN_POINT('Ctrl Pts',(126.615194436786,34.8164472993528,20.1549668525351));
#41725=CARTESIAN_POINT('Ctrl Pts',(126.613711945883,34.8460407510556,20.1531987661108));
#41726=CARTESIAN_POINT('Ctrl Pts',(126.613036918084,34.8616840679095,20.1522587723144));
#41727=CARTESIAN_POINT('Ctrl Pts',(126.611002638902,34.9178611839555,20.1488652024303));
#41728=CARTESIAN_POINT('Ctrl Pts',(126.610262545954,34.9584121894217,20.1463820977784));
#41729=CARTESIAN_POINT('Ctrl Pts',(126.610250158159,34.9989645099258,20.1438717258877));
#41730=CARTESIAN_POINT('Ctrl Pts',(126.610250159371,34.9989605517602,20.1438719709159));
#41731=CARTESIAN_POINT('Ctrl Pts',(126.610184366452,35.2135181673577,20.1305898943176));
#41732=CARTESIAN_POINT('Ctrl Pts',(126.630489346633,35.4275956772245,20.1166108704707));
#41733=CARTESIAN_POINT('Ctrl Pts',(126.705189704235,35.817192544607,20.0911256084591));
#41734=CARTESIAN_POINT('Ctrl Pts',(126.753851883876,35.9930339018189,20.0796019086335));
#41735=CARTESIAN_POINT('Ctrl Pts',(126.818016155968,36.1685056986385,20.068223916931));
#41736=CARTESIAN_POINT('Ctrl Pts',(126.819624542574,36.1728762511695,20.06794058377));
#41737=CARTESIAN_POINT('Ctrl Pts',(126.821241918282,36.1772434414401,20.0676575318486));
#41738=CARTESIAN_POINT('Ctrl Pts',(126.821241918623,36.1772434423597,20.4155867593643));
#41739=CARTESIAN_POINT('Ctrl Pts',(126.820287669406,36.174666806722,20.4157584005415));
#41740=CARTESIAN_POINT('Ctrl Pts',(126.819336531962,36.1720889539246,20.4159299649612));
#41741=CARTESIAN_POINT('Ctrl Pts',(126.785050662335,36.0788154230474,20.4221319007212));
#41742=CARTESIAN_POINT('Ctrl Pts',(126.755603836689,35.9867310859727,20.4280573351828));
#41743=CARTESIAN_POINT('Ctrl Pts',(126.720262772976,35.8573972608461,20.4361063917783));
#41744=CARTESIAN_POINT('Ctrl Pts',(126.710994149601,35.8211254629107,20.4383348157629));
#41745=CARTESIAN_POINT('Ctrl Pts',(126.69607245493,35.7584181214976,20.442139148177));
#41746=CARTESIAN_POINT('Ctrl Pts',(126.690131386026,35.7320553881174,20.4437240062198));
#41747=CARTESIAN_POINT('Ctrl Pts',(126.678604941951,35.6778964257731,20.446951220593));
#41748=CARTESIAN_POINT('Ctrl Pts',(126.673051753982,35.6500954814279,20.4485924542259));
#41749=CARTESIAN_POINT('Ctrl Pts',(126.659707162139,35.5786325369141,20.452773846614));
#41750=CARTESIAN_POINT('Ctrl Pts',(126.652422551288,35.5348806749159,20.4552981377726));
#41751=CARTESIAN_POINT('Ctrl Pts',(126.622062486016,35.3274909900031,20.4671126870272));
#41752=CARTESIAN_POINT('Ctrl Pts',(126.610113320875,35.1624456778701,20.4760587111048));
#41753=CARTESIAN_POINT('Ctrl Pts',(126.610434020872,34.7779706240709,20.4965624622672));
#41754=CARTESIAN_POINT('Ctrl Pts',(126.631878457629,34.5593210766636,20.507961576881));
#41755=CARTESIAN_POINT('Ctrl Pts',(126.686426682109,34.2826552361581,20.5235152352456));
#41756=CARTESIAN_POINT('Ctrl Pts',(126.70028919491,34.221373477112,20.5270361444065));
#41757=CARTESIAN_POINT('Ctrl Pts',(126.721539855484,34.1382385085309,20.5319594782805));
#41758=CARTESIAN_POINT('Ctrl Pts',(126.727460770062,34.1160199585576,20.533289798393));
#41759=CARTESIAN_POINT('Ctrl Pts',(126.737685091135,34.0791638455968,20.5355233342974));
#41760=CARTESIAN_POINT('Ctrl Pts',(126.74186223254,34.064491545674,20.536419620563));
#41761=CARTESIAN_POINT('Ctrl Pts',(126.750734768655,34.0341069269045,20.5382914133885));
#41762=CARTESIAN_POINT('Ctrl Pts',(126.755445343906,34.0183997599718,20.5392676946189));
#41763=CARTESIAN_POINT('Ctrl Pts',(126.768423535529,33.9762389134624,20.5419104104396));
#41764=CARTESIAN_POINT('Ctrl Pts',(126.776901763124,33.9498519837033,20.5435880158197));
#41765=CARTESIAN_POINT('Ctrl Pts',(126.8284236133,33.7960036005473,20.553496121321));
#41766=CARTESIAN_POINT('Ctrl Pts',(126.878697867504,33.6711017771715,20.5620484131386));
#41767=CARTESIAN_POINT('Ctrl Pts',(127.060272604103,33.28757172159,20.5893018313336));
#41768=CARTESIAN_POINT('Ctrl Pts',(127.217403944963,33.0425469118861,20.6080877805358));
#41769=CARTESIAN_POINT('Ctrl Pts',(127.436521563445,32.7815387563258,20.6288048290108));
#41770=CARTESIAN_POINT('Ctrl Pts',(127.470097988527,32.7433236350366,20.631863060392));
#41771=CARTESIAN_POINT('Ctrl Pts',(127.524804312639,32.6838157681659,20.6366677502469));
#41772=CARTESIAN_POINT('Ctrl Pts',(127.545377605051,32.6620239370128,20.6384367326263));
#41773=CARTESIAN_POINT('Ctrl Pts',(127.584692459151,32.6214715722403,20.6417478041207));
#41774=CARTESIAN_POINT('Ctrl Pts',(127.603370306727,32.6026526804182,20.6432924218791));
#41775=CARTESIAN_POINT('Ctrl Pts',(127.646331362137,32.5603711392118,20.6467825642812));
#41776=CARTESIAN_POINT('Ctrl Pts',(127.670748388758,32.5370480954941,20.6487220199996));
#41777=CARTESIAN_POINT('Ctrl Pts',(127.748548846851,32.4649253843845,20.6547693392371));
#41778=CARTESIAN_POINT('Ctrl Pts',(127.803149466954,32.4174655174925,20.6588222590061));
#41779=CARTESIAN_POINT('Ctrl Pts',(127.938265608477,32.3074087680611,20.6684502553522));
#41780=CARTESIAN_POINT('Ctrl Pts',(128.020168665936,32.2466264303729,20.6739631819367));
#41781=CARTESIAN_POINT('Ctrl Pts',(128.144183891671,32.1629908780481,20.6819651990938));
#41782=CARTESIAN_POINT('Ctrl Pts',(128.184234826507,32.1371917433332,20.6845000248636));
#41783=CARTESIAN_POINT('Ctrl Pts',(128.402268225455,32.0031605395511,20.6980894910399));
#41784=CARTESIAN_POINT('Ctrl Pts',(128.589380262871,31.9106748871943,20.7089910326984));
#41785=CARTESIAN_POINT('Ctrl Pts',(128.827680218912,31.8190749870077,20.7232378679673));
#41786=CARTESIAN_POINT('Ctrl Pts',(128.87193031137,31.8031146505917,20.725899008975));
#41787=CARTESIAN_POINT('Ctrl Pts',(128.934229248945,31.7820988161614,20.7296857708342));
#41788=CARTESIAN_POINT('Ctrl Pts',(128.952011469793,31.7762637624649,20.7307711629529));
#41789=CARTESIAN_POINT('Ctrl Pts',(128.98425221572,31.765979231962,20.7327487512041));
#41790=CARTESIAN_POINT('Ctrl Pts',(128.998694184847,31.7614786478996,20.733638100551));
#41791=CARTESIAN_POINT('Ctrl Pts',(129.029098164828,31.752226603529,20.7355185633058));
#41792=CARTESIAN_POINT('Ctrl Pts',(129.045065670042,31.7474959172843,20.7365107268351));
#41793=CARTESIAN_POINT('Ctrl Pts',(129.088842768182,31.7348762404121,20.7392421568406));
#41794=CARTESIAN_POINT('Ctrl Pts',(129.116718823208,31.727225197413,20.7409938469677));
#41795=CARTESIAN_POINT('Ctrl Pts',(129.325058703135,31.6728984170947,20.7541603296649));
#41796=CARTESIAN_POINT('Ctrl Pts',(129.508986324946,31.6408267906926,20.7661819326654));
#41797=CARTESIAN_POINT('Ctrl Pts',(129.926976852332,31.603013975896,20.7932358590426));
#41798=CARTESIAN_POINT('Ctrl Pts',(130.160937842385,31.6060383054034,20.8081622060412));
#41799=CARTESIAN_POINT('Ctrl Pts',(130.444559696523,31.6391233791211,20.8255380488592));
#41800=CARTESIAN_POINT('Ctrl Pts',(130.496216949364,31.6463610546961,20.8286762925382));
#41801=CARTESIAN_POINT('Ctrl Pts',(130.577535758621,31.6596748321647,20.8335765730972));
#41802=CARTESIAN_POINT('Ctrl Pts',(130.607316618918,31.6649608109426,20.8353626776652));
#41803=CARTESIAN_POINT('Ctrl Pts',(130.662778275836,31.6755725888658,20.8386741440546));
#41804=CARTESIAN_POINT('Ctrl Pts',(130.688475529499,31.6807991689149,20.8402024715004));
#41805=CARTESIAN_POINT('Ctrl Pts',(130.74656647488,31.6933179922378,20.8436449407203));
#41806=CARTESIAN_POINT('Ctrl Pts',(130.778919122243,31.7007891073026,20.8455533183412));
#41807=CARTESIAN_POINT('Ctrl Pts',(130.878248844127,31.7252696793858,20.8513891928279));
#41808=CARTESIAN_POINT('Ctrl Pts',(130.944821585727,31.7438530789242,20.8552673151768));
#41809=CARTESIAN_POINT('Ctrl Pts',(131.101938643297,31.7929364568094,20.8643792360567));
#41810=CARTESIAN_POINT('Ctrl Pts',(131.191853802399,31.8252541049068,20.8695600737131));
#41811=CARTESIAN_POINT('Ctrl Pts',(131.404081399756,31.9118233395886,20.8818533413628));
#41812=CARTESIAN_POINT('Ctrl Pts',(131.524780047811,31.9695997064192,20.8888964031794));
#41813=CARTESIAN_POINT('Ctrl Pts',(131.77439522822,32.1077840022079,20.9040647518095));
#41814=CARTESIAN_POINT('Ctrl Pts',(131.901952122942,32.1900246943164,20.9121919779557));
#41815=CARTESIAN_POINT('Ctrl Pts',(132.052479283903,32.3020317102068,20.9227817179465));
#41816=CARTESIAN_POINT('Ctrl Pts',(132.081048559259,32.324006580663,20.9248397193474));
#41817=CARTESIAN_POINT('Ctrl Pts',(132.123442417569,32.3577044918861,20.9279757442792));
#41818=CARTESIAN_POINT('Ctrl Pts',(132.137533085632,32.3690903609842,20.929032073311));
#41819=CARTESIAN_POINT('Ctrl Pts',(132.162966379457,32.3899807513462,20.9309656897006));
#41820=CARTESIAN_POINT('Ctrl Pts',(132.174339003062,32.3994473833754,20.9318403911967));
#41821=CARTESIAN_POINT('Ctrl Pts',(132.200642199068,32.4216354573315,20.933886879027));
#41822=CARTESIAN_POINT('Ctrl Pts',(132.215524654352,32.434412295685,20.9350624661483));
#41823=CARTESIAN_POINT('Ctrl Pts',(132.263607093785,32.4764222253639,20.9389161380733));
#41824=CARTESIAN_POINT('Ctrl Pts',(132.29634464679,32.5061750806288,20.9416274153544));
#41825=CARTESIAN_POINT('Ctrl Pts',(132.375493863726,32.5809883328067,20.948381507485));
#41826=CARTESIAN_POINT('Ctrl Pts',(132.421215260218,32.6267523580759,20.9524589968842));
#41827=CARTESIAN_POINT('Ctrl Pts',(132.638672508756,32.8572400759333,20.9726242675964));
#41828=CARTESIAN_POINT('Ctrl Pts',(132.790754797264,33.0594537018878,20.9891203864687));
#41829=CARTESIAN_POINT('Ctrl Pts',(132.972198604104,33.3667846683902,21.0114902674266));
#41830=CARTESIAN_POINT('Ctrl Pts',(133.021204514989,33.4593236646684,21.0179317523213));
#41831=CARTESIAN_POINT('Ctrl Pts',(133.082695836451,33.5896985382098,21.0266040484989));
#41832=CARTESIAN_POINT('Ctrl Pts',(133.098913237366,33.6256998951742,21.0289584376606));
#41833=CARTESIAN_POINT('Ctrl Pts',(133.124229154205,33.6846274451366,21.032748565642));
#41834=CARTESIAN_POINT('Ctrl Pts',(133.133712615707,33.7073832524177,21.0341970572899));
#41835=CARTESIAN_POINT('Ctrl Pts',(133.153173107556,33.7555524684059,21.0372322118983));
#41836=CARTESIAN_POINT('Ctrl Pts',(133.163093099845,33.7809871163205,21.038816898363));
#41837=CARTESIAN_POINT('Ctrl Pts',(133.186437348435,33.8430456479946,21.0426415025806));
#41838=CARTESIAN_POINT('Ctrl Pts',(133.199539002191,33.8797872082199,21.0448707648528));
#41839=CARTESIAN_POINT('Ctrl Pts',(133.24697040297,34.0204283734803,21.0532802494469));
#41840=CARTESIAN_POINT('Ctrl Pts',(133.276898129637,34.1257465454927,21.0593204917051));
#41841=CARTESIAN_POINT('Ctrl Pts',(133.347709550343,34.4303023991381,21.0762830157843));
#41842=CARTESIAN_POINT('Ctrl Pts',(133.375839675054,34.6320037613424,21.0868954548715));
#41843=CARTESIAN_POINT('Ctrl Pts',(133.392343664284,34.9706808097004,21.1050193267405));
#41844=CARTESIAN_POINT('Ctrl Pts',(133.390793642338,35.1066127959693,21.112384072702));
#41845=CARTESIAN_POINT('Ctrl Pts',(133.379085931659,35.2701393055838,21.1217219058544));
#41846=CARTESIAN_POINT('Ctrl Pts',(133.376726926689,35.2981813731623,21.1233403616281));
#41847=CARTESIAN_POINT('Ctrl Pts',(133.372432363392,35.342603170114,21.1259359640332));
#41848=CARTESIAN_POINT('Ctrl Pts',(133.370725863199,35.359004328886,21.1269011884282));
#41849=CARTESIAN_POINT('Ctrl Pts',(133.367195944092,35.3906830635239,21.1287799559407));
#41850=CARTESIAN_POINT('Ctrl Pts',(133.365388065386,35.405961719006,21.1296926790283));
#41851=CARTESIAN_POINT('Ctrl Pts',(133.360633906574,35.4439234314898,21.1319760699028));
#41852=CARTESIAN_POINT('Ctrl Pts',(133.357561939875,35.4665897816774,21.133353311651));
#41853=CARTESIAN_POINT('Ctrl Pts',(133.344577054242,35.5556181563419,21.1388128579982));
#41854=CARTESIAN_POINT('Ctrl Pts',(133.332924560987,35.6217072160312,21.1429751290883));
#41855=CARTESIAN_POINT('Ctrl Pts',(133.294650135896,35.8065262997047,21.1548467295322));
#41856=CARTESIAN_POINT('Ctrl Pts',(133.263586818616,35.9242308620343,21.1626769769337));
#41857=CARTESIAN_POINT('Ctrl Pts',(133.151264191168,36.2726739904816,21.1862746419526));
#41858=CARTESIAN_POINT('Ctrl Pts',(133.051301348161,36.4965828054287,21.2019464876325));
#41859=CARTESIAN_POINT('Ctrl Pts',(132.90227437232,36.7520949652057,21.2199339447609));
#41860=CARTESIAN_POINT('Ctrl Pts',(132.875443286598,36.7957894181399,21.2230172403244));
#41861=CARTESIAN_POINT('Ctrl Pts',(132.831326582747,36.8641078543573,21.2278518923955));
#41862=CARTESIAN_POINT('Ctrl Pts',(132.81468751178,36.8891380598049,21.2296262519872));
#41863=CARTESIAN_POINT('Ctrl Pts',(132.784251648261,36.9336278309288,21.2327866148261));
#41864=CARTESIAN_POINT('Ctrl Pts',(132.77057835594,36.9531690776478,21.234177062109));
#41865=CARTESIAN_POINT('Ctrl Pts',(132.73790686114,36.9988281614496,21.2374323043555));
#41866=CARTESIAN_POINT('Ctrl Pts',(132.718739210369,37.0248222658681,21.2392905478241));
#41867=CARTESIAN_POINT('Ctrl Pts',(132.660423487591,37.1015854657769,21.2447967908453));
#41868=CARTESIAN_POINT('Ctrl Pts',(132.620202665668,37.1515234883054,21.2484034836183));
#41869=CARTESIAN_POINT('Ctrl Pts',(132.472626587217,37.3244722121546,21.2610287433338));
#41870=CARTESIAN_POINT('Ctrl Pts',(132.35782780728,37.4408415255019,21.269763344948));
#41871=CARTESIAN_POINT('Ctrl Pts',(132.077113861039,37.6870340645996,21.289586796411));
#41872=CARTESIAN_POINT('Ctrl Pts',(131.906619338272,37.8105764631581,21.3005838628485));
#41873=CARTESIAN_POINT('Ctrl Pts',(131.687006581584,37.9404840054754,21.3148470834164));
#41874=CARTESIAN_POINT('Ctrl Pts',(131.647753259046,37.9626586356544,21.3174009936397));
#41875=CARTESIAN_POINT('Ctrl Pts',(131.591879926439,37.9927682268302,21.3210589503074));
#41876=CARTESIAN_POINT('Ctrl Pts',(131.575618084752,38.0013615207472,21.3221262512647));
#41877=CARTESIAN_POINT('Ctrl Pts',(131.545787996981,38.0168154863686,21.3240903603761));
#41878=CARTESIAN_POINT('Ctrl Pts',(131.532241812037,38.0237181142276,21.3249846571824));
#41879=CARTESIAN_POINT('Ctrl Pts',(131.503551296207,38.0380954173613,21.3268845100766));
#41880=CARTESIAN_POINT('Ctrl Pts',(131.488397027897,38.0455483128494,21.3278912299232));
#41881=CARTESIAN_POINT('Ctrl Pts',(131.446160455547,38.0659298089003,21.330704669029));
#41882=CARTESIAN_POINT('Ctrl Pts',(131.418961832046,38.0786121615635,21.3325250179129));
#41883=CARTESIAN_POINT('Ctrl Pts',(131.356681694553,38.1066519328712,21.3367068885165));
#41884=CARTESIAN_POINT('Ctrl Pts',(131.321501375593,38.1217791943306,21.3390787615205));
#41885=CARTESIAN_POINT('Ctrl Pts',(131.202648939869,38.1705158194699,21.347106767073));
#41886=CARTESIAN_POINT('Ctrl Pts',(131.117896505443,38.2013810699406,21.3528550837187));
#41887=CARTESIAN_POINT('Ctrl Pts',(130.753003320304,38.3180105961848,21.3774516244916));
#41888=CARTESIAN_POINT('Ctrl Pts',(130.463543951183,38.3706665408219,21.3964461136882));
#41889=CARTESIAN_POINT('Ctrl Pts',(130.120162223955,38.3880003854235,21.4173366391746));
#41890=CARTESIAN_POINT('Ctrl Pts',(130.06937504214,38.3894207607509,21.4203894802327));
#41891=CARTESIAN_POINT('Ctrl Pts',(129.988896230471,38.3898617235049,21.4251706978793));
#41892=CARTESIAN_POINT('Ctrl Pts',(129.959217953193,38.3896345978137,21.4269217621508));
#41893=CARTESIAN_POINT('Ctrl Pts',(129.90298658836,38.3884656048035,21.4302175802166));
#41894=CARTESIAN_POINT('Ctrl Pts',(129.876434289955,38.3876012651165,21.4317645907531));
#41895=CARTESIAN_POINT('Ctrl Pts',(129.815667605839,38.3849077389183,21.4352850277209));
#41896=CARTESIAN_POINT('Ctrl Pts',(129.781465008626,38.3828717699949,21.4372519642436));
#41897=CARTESIAN_POINT('Ctrl Pts',(129.672243050639,38.3747066847006,21.443491326659));
#41898=CARTESIAN_POINT('Ctrl Pts',(129.59739225161,38.3665973862088,21.4477034772471));
#41899=CARTESIAN_POINT('Ctrl Pts',(129.415917493554,38.3407967056482,21.4578131898332));
#41900=CARTESIAN_POINT('Ctrl Pts',(129.30974910089,38.3204865320446,21.4636392133884));
#41901=CARTESIAN_POINT('Ctrl Pts',(129.00959545413,38.2480452890874,21.480122175672));
#41902=CARTESIAN_POINT('Ctrl Pts',(128.819043973823,38.1837139111959,21.4905852867816));
#41903=CARTESIAN_POINT('Ctrl Pts',(128.560090377842,38.069823851479,21.5060108365125));
#41904=CARTESIAN_POINT('Ctrl Pts',(128.486100203053,38.0340177310372,21.5105706512268));
#41905=CARTESIAN_POINT('Ctrl Pts',(128.391282482039,37.9838003465354,21.5167069468011));
#41906=CARTESIAN_POINT('Ctrl Pts',(128.369207311317,37.971792672351,21.5181569856169));
#41907=CARTESIAN_POINT('Ctrl Pts',(128.334804793392,37.9525808662684,21.5204537150655));
#41908=CARTESIAN_POINT('Ctrl Pts',(128.322385539367,37.9455421492811,21.5212904833712));
#41909=CARTESIAN_POINT('Ctrl Pts',(128.296577701063,37.9306991812168,21.5230461253651));
#41910=CARTESIAN_POINT('Ctrl Pts',(128.28319766692,37.9228812729825,21.5239659273597));
#41911=CARTESIAN_POINT('Ctrl Pts',(128.249701909015,37.9030004845914,21.5262919114362));
#41912=CARTESIAN_POINT('Ctrl Pts',(128.229657099984,37.8908201552578,21.5277051883446));
#41913=CARTESIAN_POINT('Ctrl Pts',(128.148395497582,37.840279005941,21.5335171321417));
#41914=CARTESIAN_POINT('Ctrl Pts',(128.088289628102,37.800176073527,21.5380088262062));
#41915=CARTESIAN_POINT('Ctrl Pts',(127.917054047593,37.6778431338006,21.5512788691473));
#41916=CARTESIAN_POINT('Ctrl Pts',(127.809616123247,37.590699415582,21.5602085555482));
#41917=CARTESIAN_POINT('Ctrl Pts',(127.546608694519,37.3492872954638,21.5832138659074));
#41918=CARTESIAN_POINT('Ctrl Pts',(127.40009855453,37.1860507072318,21.5971685226719));
#41919=CARTESIAN_POINT('Ctrl Pts',(127.239068679673,36.9673444094585,21.6137026321429));
#41920=CARTESIAN_POINT('Ctrl Pts',(127.208797091498,36.9241550278903,21.6168768179205));
#41921=CARTESIAN_POINT('Ctrl Pts',(127.16269914587,36.8550070492302,21.6218199817447));
#41922=CARTESIAN_POINT('Ctrl Pts',(127.146194008049,36.8295132521392,21.6236137343507));
#41923=CARTESIAN_POINT('Ctrl Pts',(127.11608736585,36.7816115783088,21.6269321404692));
#41924=CARTESIAN_POINT('Ctrl Pts',(127.102398969492,36.7592612717466,21.6284598716567));
#41925=CARTESIAN_POINT('Ctrl Pts',(127.072051513625,36.7083949263889,21.6318917102578));
#41926=CARTESIAN_POINT('Ctrl Pts',(127.055547070627,36.6797894570398,21.6337902039268));
#41927=CARTESIAN_POINT('Ctrl Pts',(127.006297779011,36.5914738478518,21.6395600208409));
#41928=CARTESIAN_POINT('Ctrl Pts',(126.974930943181,36.5310127555541,21.6433836457532));
#41929=CARTESIAN_POINT('Ctrl Pts',(126.899435868449,36.3740994249191,21.6530287941239));
#41930=CARTESIAN_POINT('Ctrl Pts',(126.858009975527,36.2765234378314,21.6587653597668));
#41931=CARTESIAN_POINT('Ctrl Pts',(126.821242031451,36.1772437470164,21.6644319010721));
#41932=CARTESIAN_POINT('Origin',(130.,35.,23.));
#41933=CARTESIAN_POINT('',(126.821241918358,36.1772434416445,22.9104377666251));
#41934=CARTESIAN_POINT('',(126.821241895364,36.1772433795577,22.5700842967619));
#41935=CARTESIAN_POINT('',(126.821241918358,36.1772434416438,23.));
#41936=CARTESIAN_POINT('Ctrl Pts',(126.821241895364,36.1772433795577,22.5700842967619));
#41937=CARTESIAN_POINT('Ctrl Pts',(126.875225501832,36.3230083331407,22.5618217349734));
#41938=CARTESIAN_POINT('Ctrl Pts',(126.939183478084,36.4649200608349,22.5536544970183));
#41939=CARTESIAN_POINT('Ctrl Pts',(127.04434190883,36.6610177047732,22.5416107837619));
#41940=CARTESIAN_POINT('Ctrl Pts',(127.077749652317,36.7191121465268,22.537939604011));
#41941=CARTESIAN_POINT('Ctrl Pts',(127.13662180678,36.8148078998927,22.5316542712977));
#41942=CARTESIAN_POINT('Ctrl Pts',(127.161160408686,36.8529575700016,22.5290823090787));
#41943=CARTESIAN_POINT('Ctrl Pts',(127.197501754479,36.9070398211168,22.5253227374369));
#41944=CARTESIAN_POINT('Ctrl Pts',(127.208691300128,36.9233806166307,22.5241715278098));
#41945=CARTESIAN_POINT('Ctrl Pts',(127.228576270911,36.9518808912746,22.5221349878048));
#41946=CARTESIAN_POINT('Ctrl Pts',(127.237209935267,36.9640823674703,22.5212536651132));
#41947=CARTESIAN_POINT('Ctrl Pts',(127.25644081933,36.990882587254,22.5192965508899));
#41948=CARTESIAN_POINT('Ctrl Pts',(127.267073906163,37.0054539106027,22.5182184934474));
#41949=CARTESIAN_POINT('Ctrl Pts',(127.29906426764,37.0485658205786,22.5149887532843));
#41950=CARTESIAN_POINT('Ctrl Pts',(127.320755364013,37.0768542835653,22.5128165804459));
#41951=CARTESIAN_POINT('Ctrl Pts',(127.432680584142,37.2181497589344,22.5017178884316));
#41952=CARTESIAN_POINT('Ctrl Pts',(127.529628601901,37.3256345071104,22.4924602846372));
#41953=CARTESIAN_POINT('Ctrl Pts',(127.721878273514,37.5131523681107,22.4751668518684));
#41954=CARTESIAN_POINT('Ctrl Pts',(127.815307407623,37.5947819406969,22.4671568954737));
#41955=CARTESIAN_POINT('Ctrl Pts',(127.996097781847,37.7360375827837,22.4525313924841));
#41956=CARTESIAN_POINT('Ctrl Pts',(128.082185171625,37.797054698561,22.4458932087927));
#41957=CARTESIAN_POINT('Ctrl Pts',(128.233316088329,37.8939098397905,22.4348186512555));
#41958=CARTESIAN_POINT('Ctrl Pts',(128.296944042274,37.9318062479353,22.4303179910704));
#41959=CARTESIAN_POINT('Ctrl Pts',(128.391579325192,37.9840488775618,22.4238539947896));
#41960=CARTESIAN_POINT('Ctrl Pts',(128.421639769832,38.0000573130537,22.4218333253232));
#41961=CARTESIAN_POINT('Ctrl Pts',(128.475550057008,38.0277321439586,22.4182657481259));
#41962=CARTESIAN_POINT('Ctrl Pts',(128.499304954907,38.0395762871399,22.4167127952853));
#41963=CARTESIAN_POINT('Ctrl Pts',(128.550014494159,38.0641205515884,22.4134368923964));
#41964=CARTESIAN_POINT('Ctrl Pts',(128.577002510905,38.0767468127269,22.4117165598567));
#41965=CARTESIAN_POINT('Ctrl Pts',(128.650963668166,38.1101679342132,22.4070621615483));
#41966=CARTESIAN_POINT('Ctrl Pts',(128.69824954404,38.1302539422821,22.4041518421853));
#41967=CARTESIAN_POINT('Ctrl Pts',(128.977648396678,38.2415096665208,22.3872995504473));
#41968=CARTESIAN_POINT('Ctrl Pts',(129.218791812696,38.3079166523496,22.374198100807));
#41969=CARTESIAN_POINT('Ctrl Pts',(129.582428971256,38.3660315475674,22.3546418414912));
#41970=CARTESIAN_POINT('Ctrl Pts',(129.70070353675,38.3786021360902,22.34829738838));
#41971=CARTESIAN_POINT('Ctrl Pts',(129.885466481718,38.3884607355536,22.33810705976));
#41972=CARTESIAN_POINT('Ctrl Pts',(129.951631511365,38.3900506531305,22.3344018227716));
#41973=CARTESIAN_POINT('Ctrl Pts',(130.040559845929,38.3895837741391,22.3292975034845));
#41974=CARTESIAN_POINT('Ctrl Pts',(130.063321105859,38.389234963834,22.3279800893559));
#41975=CARTESIAN_POINT('Ctrl Pts',(130.101436401956,38.3882667839256,22.3257530956019));
#41976=CARTESIAN_POINT('Ctrl Pts',(130.116793321593,38.3877721965517,22.3248501250248));
#41977=CARTESIAN_POINT('Ctrl Pts',(130.148661475368,38.3865289004955,22.3229636064933));
#41978=CARTESIAN_POINT('Ctrl Pts',(130.165171323603,38.3857638188142,22.3219792789654));
#41979=CARTESIAN_POINT('Ctrl Pts',(130.209951597913,38.3833603539918,22.3192916976235));
#41980=CARTESIAN_POINT('Ctrl Pts',(130.238207546472,38.3814884310336,22.3175766460016));
#41981=CARTESIAN_POINT('Ctrl Pts',(130.417174789027,38.367377879468,22.3066057982526));
#41982=CARTESIAN_POINT('Ctrl Pts',(130.566936597936,38.3454212194724,22.2969459503887));
#41983=CARTESIAN_POINT('Ctrl Pts',(130.901919672664,38.2731668387252,22.2748900726358));
#41984=CARTESIAN_POINT('Ctrl Pts',(131.085379166613,38.2169928459768,22.2625034731648));
#41985=CARTESIAN_POINT('Ctrl Pts',(131.361744336801,38.1060187485805,22.2438387105796));
#41986=CARTESIAN_POINT('Ctrl Pts',(131.458458241516,38.061797390988,22.2372999180053));
#41987=CARTESIAN_POINT('Ctrl Pts',(131.587288169342,37.9953988565946,22.2285878548181));
#41988=CARTESIAN_POINT('Ctrl Pts',(131.621329746082,37.9771106936778,22.2262852851839));
#41989=CARTESIAN_POINT('Ctrl Pts',(131.678818464032,37.9449474112908,22.2223943749332));
#41990=CARTESIAN_POINT('Ctrl Pts',(131.702424041903,37.9313647225282,22.2207960070167));
#41991=CARTESIAN_POINT('Ctrl Pts',(131.7499680119,37.9032398015578,22.2175742984434));
#41992=CARTESIAN_POINT('Ctrl Pts',(131.773894996457,37.8886823982747,22.2159516618953));
#41993=CARTESIAN_POINT('Ctrl Pts',(131.833805184936,37.8512073493534,22.2118837861877));
#41994=CARTESIAN_POINT('Ctrl Pts',(131.86954181389,37.8279035415976,22.209452697161));
#41995=CARTESIAN_POINT('Ctrl Pts',(132.017179617188,37.72760685592,22.1993764829358));
#41996=CARTESIAN_POINT('Ctrl Pts',(132.124846239559,37.6445957052157,22.1919544186748));
#41997=CARTESIAN_POINT('Ctrl Pts',(132.392861901169,37.4109917086358,22.1728582887691));
#41998=CARTESIAN_POINT('Ctrl Pts',(132.54403999127,37.2508935064661,22.1614542791697));
#41999=CARTESIAN_POINT('Ctrl Pts',(132.716289259051,37.0287799853229,22.1461834313152));
#42000=CARTESIAN_POINT('Ctrl Pts',(132.752591867791,36.9792455248811,22.1428062646297));
#42001=CARTESIAN_POINT('Ctrl Pts',(132.811778717054,36.8937059116401,22.1369729486467));
#42002=CARTESIAN_POINT('Ctrl Pts',(132.835365711525,36.8582041250205,22.1345515047984));
#42003=CARTESIAN_POINT('Ctrl Pts',(132.868670118405,36.8059652979876,22.1309735325103));
#42004=CARTESIAN_POINT('Ctrl Pts',(132.878924333038,36.789573567079,22.1298487260907));
#42005=CARTESIAN_POINT('Ctrl Pts',(132.89684151262,36.7603797613966,22.1278401021512));
#42006=CARTESIAN_POINT('Ctrl Pts',(132.904561037384,36.7476134636984,22.1269598753378));
#42007=CARTESIAN_POINT('Ctrl Pts',(132.921618874079,36.7189785353462,22.1249811132792));
#42008=CARTESIAN_POINT('Ctrl Pts',(132.930912256793,36.7030846600515,22.1238799647535));
#42009=CARTESIAN_POINT('Ctrl Pts',(132.958777235811,36.6545253861387,22.1205089946005));
#42010=CARTESIAN_POINT('Ctrl Pts',(132.976934989941,36.6216272071616,22.1182160662738));
#42011=CARTESIAN_POINT('Ctrl Pts',(133.096953143681,36.3953672704998,22.1024187225744));
#42012=CARTESIAN_POINT('Ctrl Pts',(133.180447730085,36.1928585939215,22.0881808117108));
#42013=CARTESIAN_POINT('Ctrl Pts',(133.30225564042,35.7911972523882,22.0612069892058));
#42014=CARTESIAN_POINT('Ctrl Pts',(133.343394346909,35.5938191217872,22.0484946449271));
#42015=CARTESIAN_POINT('Ctrl Pts',(133.372016799823,35.349194261321,22.0336000612373));
#42016=CARTESIAN_POINT('Ctrl Pts',(133.376359310997,35.3043550987991,22.0309029574918));
#42017=CARTESIAN_POINT('Ctrl Pts',(133.381987590566,35.2310340089054,22.0265446647513));
#42018=CARTESIAN_POINT('Ctrl Pts',(133.383809995617,35.2026000090199,22.0248672164181));
#42019=CARTESIAN_POINT('Ctrl Pts',(133.386658259316,35.1472317184419,22.0216244942526));
#42020=CARTESIAN_POINT('Ctrl Pts',(133.38772179104,35.1203015890409,22.0200581806794));
#42021=CARTESIAN_POINT('Ctrl Pts',(133.389483011235,35.0563795253591,22.0163647799393));
#42022=CARTESIAN_POINT('Ctrl Pts',(133.389896487049,35.0193828208012,22.0142465428893));
#42023=CARTESIAN_POINT('Ctrl Pts',(133.389250356096,34.8950410974227,22.0071861394184));
#42024=CARTESIAN_POINT('Ctrl Pts',(133.385420668719,34.8077425342614,22.002327584243));
#42025=CARTESIAN_POINT('Ctrl Pts',(133.355757611513,34.4489787566194,21.9826170830355));
#42026=CARTESIAN_POINT('Ctrl Pts',(133.300599176495,34.1809950061153,21.968585924795));
#42027=CARTESIAN_POINT('Ctrl Pts',(133.192848435691,33.859592772917,21.9502308017877));
#42028=CARTESIAN_POINT('Ctrl Pts',(133.169909921302,33.7973030358979,21.9465929370727));
#42029=CARTESIAN_POINT('Ctrl Pts',(133.128355978564,33.6939281494664,21.9403585656468));
#42030=CARTESIAN_POINT('Ctrl Pts',(133.110721862331,33.6524674769688,21.9378033659265));
#42031=CARTESIAN_POINT('Ctrl Pts',(133.084175508649,33.593352675142,21.9340639779516));
#42032=CARTESIAN_POINT('Ctrl Pts',(133.075926228343,33.575404246216,21.9329156532463));
#42033=CARTESIAN_POINT('Ctrl Pts',(133.061161522789,33.5440060039617,21.9308822090732));
#42034=CARTESIAN_POINT('Ctrl Pts',(133.054713295202,33.5305255847754,21.9300010518782));
#42035=CARTESIAN_POINT('Ctrl Pts',(133.04026788089,33.5008325489308,21.9280417733783));
#42036=CARTESIAN_POINT('Ctrl Pts',(133.032230115397,33.4846411880798,21.9269613502632));
#42037=CARTESIAN_POINT('Ctrl Pts',(133.007870204435,33.4365402075092,21.9237173050272));
#42038=CARTESIAN_POINT('Ctrl Pts',(132.991171536618,33.4048253049535,21.9215329345346));
#42039=CARTESIAN_POINT('Ctrl Pts',(132.902689487806,33.2430519876629,21.9101775712375));
#42040=CARTESIAN_POINT('Ctrl Pts',(132.822920210585,33.1175582039464,21.9006576360235));
#42041=CARTESIAN_POINT('Ctrl Pts',(132.660088279477,32.8951249345666,21.8829012537954));
#42042=CARTESIAN_POINT('Ctrl Pts',(132.579275751378,32.7968415221911,21.8746901964973));
#42043=CARTESIAN_POINT('Ctrl Pts',(132.424597550314,32.6289320037647,21.8601615863824));
#42044=CARTESIAN_POINT('Ctrl Pts',(132.35276416376,32.5576363565423,21.8538060371207));
#42045=CARTESIAN_POINT('Ctrl Pts',(132.224571216312,32.4413162128416,21.8431393918312));
#42046=CARTESIAN_POINT('Ctrl Pts',(132.169769836736,32.3946823919707,21.8387702700472));
#42047=CARTESIAN_POINT('Ctrl Pts',(132.087177638633,32.3288148588872,21.8324560743247));
#42048=CARTESIAN_POINT('Ctrl Pts',(132.060520106401,32.3081980816888,21.8304573818686));
#42049=CARTESIAN_POINT('Ctrl Pts',(132.012351936533,32.2720800341061,21.8269140471918));
#42050=CARTESIAN_POINT('Ctrl Pts',(131.990958816923,32.2564273828991,21.8253636606872));
#42051=CARTESIAN_POINT('Ctrl Pts',(131.944959874856,32.2235928568047,21.8220783379534));
#42052=CARTESIAN_POINT('Ctrl Pts',(131.920304944633,32.2064834808644,21.8203462197528));
#42053=CARTESIAN_POINT('Ctrl Pts',(131.853100366146,32.1611568530082,21.8156993653701));
#42054=CARTESIAN_POINT('Ctrl Pts',(131.810134328719,32.1335692100242,21.812807748968));
#42055=CARTESIAN_POINT('Ctrl Pts',(131.556048120684,31.9784179696819,21.7961286814565));
#42056=CARTESIAN_POINT('Ctrl Pts',(131.332136474049,31.873233737867,21.7831603941922));
#42057=CARTESIAN_POINT('Ctrl Pts',(130.984876951053,31.7542459941395,21.7636706808566));
#42058=CARTESIAN_POINT('Ctrl Pts',(130.868983640072,31.721316445292,21.7572480507225));
#42059=CARTESIAN_POINT('Ctrl Pts',(130.686566189901,31.6798375212574,21.7469483223157));
#42060=CARTESIAN_POINT('Ctrl Pts',(130.621122555579,31.6669747039963,21.7432154948441));
#42061=CARTESIAN_POINT('Ctrl Pts',(130.532830222228,31.6523115449429,21.7380788432203));
#42062=CARTESIAN_POINT('Ctrl Pts',(130.510277200969,31.6487997441104,21.7367580134896));
#42063=CARTESIAN_POINT('Ctrl Pts',(130.472474911686,31.6433038644206,21.7345269381371));
#42064=CARTESIAN_POINT('Ctrl Pts',(130.457244039303,31.6411952467991,21.7336233569919));
#42065=CARTESIAN_POINT('Ctrl Pts',(130.425633760551,31.6370379974408,21.7317375219648));
#42066=CARTESIAN_POINT('Ctrl Pts',(130.409253005887,31.6350052777425,21.730754511883));
#42067=CARTESIAN_POINT('Ctrl Pts',(130.364829611908,31.629821855153,21.7280742865907));
#42068=CARTESIAN_POINT('Ctrl Pts',(130.33676201517,31.6269016311466,21.7263653772958));
#42069=CARTESIAN_POINT('Ctrl Pts',(130.169927402457,31.6116467093522,21.7161285458181));
#42070=CARTESIAN_POINT('Ctrl Pts',(130.030554460559,31.6075270525656,21.7072577501609));
#42071=CARTESIAN_POINT('Ctrl Pts',(129.690943783304,31.6184192464574,21.685417818628));
#42072=CARTESIAN_POINT('Ctrl Pts',(129.491497665301,31.6426139686564,21.672422138017));
#42073=CARTESIAN_POINT('Ctrl Pts',(129.189019170228,31.7068962072239,21.6530221978412));
#42074=CARTESIAN_POINT('Ctrl Pts',(129.083826876762,31.734597552331,21.6463285350691));
#42075=CARTESIAN_POINT('Ctrl Pts',(128.943019836274,31.7790198771942,21.6374507415542));
#42076=CARTESIAN_POINT('Ctrl Pts',(128.906104177428,31.7913691180207,21.6351307402485));
#42077=CARTESIAN_POINT('Ctrl Pts',(128.843686304791,31.8134520040832,21.6312193777857));
#42078=CARTESIAN_POINT('Ctrl Pts',(128.818074673809,31.8228625965841,21.6296177321195));
#42079=CARTESIAN_POINT('Ctrl Pts',(128.769531151717,31.8413674059478,21.6265873791212));
#42080=CARTESIAN_POINT('Ctrl Pts',(128.74657957293,31.8504046719075,21.6251569239996));
#42081=CARTESIAN_POINT('Ctrl Pts',(128.692955641821,31.8721983003785,21.6218191680345));
#42082=CARTESIAN_POINT('Ctrl Pts',(128.662367820567,31.8851567151857,21.6199186555321));
#42083=CARTESIAN_POINT('Ctrl Pts',(128.553199972666,31.9333100016939,21.6131428853398));
#42084=CARTESIAN_POINT('Ctrl Pts',(128.475774026608,31.9710472649369,21.6083517238278));
#42085=CARTESIAN_POINT('Ctrl Pts',(128.158333326709,32.1410258953333,21.5886249461558));
#42086=CARTESIAN_POINT('Ctrl Pts',(127.933389135964,32.2991521472882,21.5745270887007));
#42087=CARTESIAN_POINT('Ctrl Pts',(127.680569579761,32.527134068082,21.556094768226));
#42088=CARTESIAN_POINT('Ctrl Pts',(127.632528014676,32.5730886075578,21.5524515315607));
#42089=CARTESIAN_POINT('Ctrl Pts',(127.55420970803,32.6525441222596,21.5462089383984));
#42090=CARTESIAN_POINT('Ctrl Pts',(127.523194271577,32.6852921932327,21.5436510307822));
#42091=CARTESIAN_POINT('Ctrl Pts',(127.479542962563,32.7332640393114,21.5399083815639));
#42092=CARTESIAN_POINT('Ctrl Pts',(127.466371364697,32.7479961166553,21.5387595898787));
#42093=CARTESIAN_POINT('Ctrl Pts',(127.443466587,32.7740697873581,21.5367256452948));
#42094=CARTESIAN_POINT('Ctrl Pts',(127.433678426781,32.7853618864472,21.5358444620217));
#42095=CARTESIAN_POINT('Ctrl Pts',(127.412219366511,32.8104514159602,21.5338855369812));
#42096=CARTESIAN_POINT('Ctrl Pts',(127.400584067443,32.824277502484,21.5328054992466));
#42097=CARTESIAN_POINT('Ctrl Pts',(127.366922243548,32.8649328908504,21.5296298020527));
#42098=CARTESIAN_POINT('Ctrl Pts',(127.345197240853,32.8920075566197,21.5275151123006));
#42099=CARTESIAN_POINT('Ctrl Pts',(127.209834375424,33.0661146729589,21.5139426893951));
#42100=CARTESIAN_POINT('Ctrl Pts',(127.108040904296,33.2219394164598,21.5019310810867));
#42101=CARTESIAN_POINT('Ctrl Pts',(126.943989974793,33.5247509189535,21.4797356075034));
#42102=CARTESIAN_POINT('Ctrl Pts',(126.878318044167,33.6693360963235,21.4695663874464));
#42103=CARTESIAN_POINT('Ctrl Pts',(126.789542813604,33.9079467108937,21.4536824040873));
#42104=CARTESIAN_POINT('Ctrl Pts',(126.759910304147,33.9992816673109,21.4477985235872));
#42105=CARTESIAN_POINT('Ctrl Pts',(126.724185335262,34.1277396397894,21.4397947847223));
#42106=CARTESIAN_POINT('Ctrl Pts',(126.714773733107,34.1638849382873,21.4375716957518));
#42107=CARTESIAN_POINT('Ctrl Pts',(126.699588558702,34.2264246655947,21.433773566213));
#42108=CARTESIAN_POINT('Ctrl Pts',(126.69352977043,34.2527455830424,21.4321896525567));
#42109=CARTESIAN_POINT('Ctrl Pts',(126.681751704066,34.3068632978764,21.4289618683418));
#42110=CARTESIAN_POINT('Ctrl Pts',(126.676065601162,34.3346651785275,21.4273191523017));
#42111=CARTESIAN_POINT('Ctrl Pts',(126.662363998139,34.4062242534203,21.4231287783674));
#42112=CARTESIAN_POINT('Ctrl Pts',(126.654859365269,34.4500744502077,21.4205971266899));
#42113=CARTESIAN_POINT('Ctrl Pts',(126.622801559386,34.6624533174749,21.4084917881885));
#42114=CARTESIAN_POINT('Ctrl Pts',(126.61010777198,34.8325294876978,21.3992862819136));
#42115=CARTESIAN_POINT('Ctrl Pts',(126.610452581497,35.2419956021854,21.37746966976));
#42116=CARTESIAN_POINT('Ctrl Pts',(126.635959427902,35.4804181016502,21.3650622408845));
#42117=CARTESIAN_POINT('Ctrl Pts',(126.695861190542,35.758365398044,21.3491546717281));
#42118=CARTESIAN_POINT('Ctrl Pts',(126.706275144155,35.8023886319201,21.3465894054795));
#42119=CARTESIAN_POINT('Ctrl Pts',(126.722452815536,35.8651431615641,21.3428499875696));
#42120=CARTESIAN_POINT('Ctrl Pts',(126.727503279873,35.8840550964243,21.3417121992618));
#42121=CARTESIAN_POINT('Ctrl Pts',(126.736701095165,35.9173380081169,21.3396889132985));
#42122=CARTESIAN_POINT('Ctrl Pts',(126.740780200762,35.9317269194778,21.3388072003617));
#42123=CARTESIAN_POINT('Ctrl Pts',(126.749966795925,35.9633336605928,21.3368545829451));
#42124=CARTESIAN_POINT('Ctrl Pts',(126.755115896357,35.9805379602028,21.335781488118));
#42125=CARTESIAN_POINT('Ctrl Pts',(126.770773350142,36.0313787552242,21.3325816397422));
#42126=CARTESIAN_POINT('Ctrl Pts',(126.781669494679,36.0648922204941,21.3304349308154));
#42127=CARTESIAN_POINT('Ctrl Pts',(126.802146327224,36.1246862090647,21.3265448387815));
#42128=CARTESIAN_POINT('Ctrl Pts',(126.811532577294,36.1510265641211,21.3248100025831));
#42129=CARTESIAN_POINT('Ctrl Pts',(126.821241909055,36.1772434165241,21.3230640339373));
#42130=CARTESIAN_POINT('',(126.610250132112,35.0009463898671,21.731083596192));
#42131=CARTESIAN_POINT('Ctrl Pts',(126.821242031451,36.1772437470164,21.6644319010721));
#42132=CARTESIAN_POINT('Ctrl Pts',(126.771125806647,36.0419214321994,21.6721556306702));
#42133=CARTESIAN_POINT('Ctrl Pts',(126.729663516346,35.9034336601396,21.6797462668355));
#42134=CARTESIAN_POINT('Ctrl Pts',(126.685081021759,35.7103480487699,21.690316211781));
#42135=CARTESIAN_POINT('Ctrl Pts',(126.674256076812,35.6578064126016,21.6931920485904));
#42136=CARTESIAN_POINT('Ctrl Pts',(126.647643771163,35.5111024721233,21.7012705643072));
#42137=CARTESIAN_POINT('Ctrl Pts',(126.63458172262,35.4165031357547,21.7065348522985));
#42138=CARTESIAN_POINT('Ctrl Pts',(126.623044385766,35.2954021725561,21.7134815653526));
#42139=CARTESIAN_POINT('Ctrl Pts',(126.620861883431,35.2692901106178,21.7149916946813));
#42140=CARTESIAN_POINT('Ctrl Pts',(126.617829448891,35.2271249790515,21.71745369822));
#42141=CARTESIAN_POINT('Ctrl Pts',(126.616790571976,35.2110860863636,21.7183956746774));
#42142=CARTESIAN_POINT('Ctrl Pts',(126.615063214498,35.1811148686936,21.7201671196711));
#42143=CARTESIAN_POINT('Ctrl Pts',(126.614346598988,35.1671845235815,21.7209950205717));
#42144=CARTESIAN_POINT('Ctrl Pts',(126.613006261138,35.1375678885332,21.7227642901828));
#42145=CARTESIAN_POINT('Ctrl Pts',(126.612405492064,35.1218808444769,21.7237068444695));
#42146=CARTESIAN_POINT('Ctrl Pts',(126.610814474486,35.0711182665403,21.7267732381405));
#42147=CARTESIAN_POINT('Ctrl Pts',(126.6102599279,35.0360326396975,21.728917842519));
#42148=CARTESIAN_POINT('Ctrl Pts',(126.610250132112,35.0009463898671,21.731083596192));
#42149=CARTESIAN_POINT('Ctrl Pts',(126.610250133166,35.0009501562718,21.7310833637049));
#42150=CARTESIAN_POINT('Ctrl Pts',(126.610185136217,34.7690689316006,21.7453965851487));
#42151=CARTESIAN_POINT('Ctrl Pts',(126.633913061281,34.5377934983256,21.7605470636322));
#42152=CARTESIAN_POINT('Ctrl Pts',(126.716100312233,34.1420372335761,21.7864708213844));
#42153=CARTESIAN_POINT('Ctrl Pts',(126.763954461802,33.9762227578437,21.7973414354496));
#42154=CARTESIAN_POINT('Ctrl Pts',(126.842599677253,33.765499429003,21.811026118617));
#42155=CARTESIAN_POINT('Ctrl Pts',(126.862124328879,33.7166819594367,21.8141885434586));
#42156=CARTESIAN_POINT('Ctrl Pts',(126.894578255613,33.6407122464022,21.8190995686375));
#42157=CARTESIAN_POINT('Ctrl Pts',(126.906746049075,33.6132456996012,21.8208729997598));
#42158=CARTESIAN_POINT('Ctrl Pts',(126.930333074148,33.5618580123141,21.8241879615392));
#42159=CARTESIAN_POINT('Ctrl Pts',(126.941670812141,33.537902174995,21.8257320873769));
#42160=CARTESIAN_POINT('Ctrl Pts',(126.968038171882,33.4838388311011,21.8292152256595));
#42161=CARTESIAN_POINT('Ctrl Pts',(126.983237604426,33.4538169636571,21.8311482672978));
#42162=CARTESIAN_POINT('Ctrl Pts',(127.032192968928,33.3605915734959,21.8371514658501));
#42163=CARTESIAN_POINT('Ctrl Pts',(127.067508237429,33.2982269201851,21.8411678669521));
#42164=CARTESIAN_POINT('Ctrl Pts',(127.258034536226,32.9853373475992,21.8614154016649));
#42165=CARTESIAN_POINT('Ctrl Pts',(127.44344388813,32.7547269176752,21.8765394219163));
#42166=CARTESIAN_POINT('Ctrl Pts',(127.705398385339,32.5040389620112,21.8961530042115));
#42167=CARTESIAN_POINT('Ctrl Pts',(127.755865992799,32.4585673920826,21.8998721234481));
#42168=CARTESIAN_POINT('Ctrl Pts',(127.842590023496,32.3850268828863,21.9062306761191));
#42169=CARTESIAN_POINT('Ctrl Pts',(127.878112364205,32.3561212867045,21.9088266313155));
#42170=CARTESIAN_POINT('Ctrl Pts',(127.929876783607,32.3157142356581,21.9126150773015));
#42171=CARTESIAN_POINT('Ctrl Pts',(127.94565295177,32.3036212507069,21.9137703940878));
#42172=CARTESIAN_POINT('Ctrl Pts',(127.973481738142,32.2826755056885,21.9158113613552));
#42173=CARTESIAN_POINT('Ctrl Pts',(127.985488004876,32.2737626509971,21.9166929395694));
#42174=CARTESIAN_POINT('Ctrl Pts',(128.012064958381,32.2543046774915,21.9186470586094));
#42175=CARTESIAN_POINT('Ctrl Pts',(128.026660646407,32.2437960348655,21.9197218150898));
#42176=CARTESIAN_POINT('Ctrl Pts',(128.070211164312,32.2129636638088,21.9229316467005));
#42177=CARTESIAN_POINT('Ctrl Pts',(128.099400434427,32.1929770986787,21.9250868550094));
#42178=CARTESIAN_POINT('Ctrl Pts',(128.277882386406,32.0748265122162,21.9382628217981));
#42179=CARTESIAN_POINT('Ctrl Pts',(128.434422509681,31.9881423050445,21.9497938095468));
#42180=CARTESIAN_POINT('Ctrl Pts',(128.745650283263,31.8466433242713,21.9718310495977));
#42181=CARTESIAN_POINT('Ctrl Pts',(128.898947753035,31.7898997732664,21.9823118455692));
#42182=CARTESIAN_POINT('Ctrl Pts',(129.149452635028,31.7172429949641,21.998596902524));
#42183=CARTESIAN_POINT('Ctrl Pts',(129.244293575863,31.6941211468368,22.0045819160143));
#42184=CARTESIAN_POINT('Ctrl Pts',(129.376845565108,31.6678094100864,22.0126958534776));
#42185=CARTESIAN_POINT('Ctrl Pts',(129.413803670408,31.6611095240125,22.0149318517724));
#42186=CARTESIAN_POINT('Ctrl Pts',(129.477552619862,31.6506440721136,22.0187449940313));
#42187=CARTESIAN_POINT('Ctrl Pts',(129.504290622375,31.6465825382578,22.0203311965248));
#42188=CARTESIAN_POINT('Ctrl Pts',(129.55911303108,31.6389249912598,22.0235576350993));
#42189=CARTESIAN_POINT('Ctrl Pts',(129.587199658606,31.6353599772693,22.0251967932837));
#42190=CARTESIAN_POINT('Ctrl Pts',(129.659204632036,31.6271356640919,22.0293656135273));
#42191=CARTESIAN_POINT('Ctrl Pts',(129.703176048789,31.6229819209446,22.0318796012494));
#42192=CARTESIAN_POINT('Ctrl Pts',(129.906611045155,31.6077688869603,22.0433805957766));
#42193=CARTESIAN_POINT('Ctrl Pts',(130.066655911016,31.6071372037975,22.0520479730548));
#42194=CARTESIAN_POINT('Ctrl Pts',(130.423029488387,31.6309673075347,22.0711159478476));
#42195=CARTESIAN_POINT('Ctrl Pts',(130.618361038132,31.6612940092652,22.0814055127796));
#42196=CARTESIAN_POINT('Ctrl Pts',(130.893989806104,31.7291163042595,22.0968578131764));
#42197=CARTESIAN_POINT('Ctrl Pts',(130.977214478109,31.7530094763389,22.1016545409279));
#42198=CARTESIAN_POINT('Ctrl Pts',(131.083028570371,31.787824486902,22.1080279089504));
#42199=CARTESIAN_POINT('Ctrl Pts',(131.106543561795,31.7958489923484,22.1094620890962));
#42200=CARTESIAN_POINT('Ctrl Pts',(131.144846209414,31.80939170831,22.1118306449235));
#42201=CARTESIAN_POINT('Ctrl Pts',(131.159687739289,31.81475614083,22.1127564590557));
#42202=CARTESIAN_POINT('Ctrl Pts',(131.18943990428,31.8257454836426,22.1146296188666));
#42203=CARTESIAN_POINT('Ctrl Pts',(131.204349367739,31.8313722847083,22.1155770442873));
#42204=CARTESIAN_POINT('Ctrl Pts',(131.24307597267,31.8463004335149,22.1180597315593));
#42205=CARTESIAN_POINT('Ctrl Pts',(131.266828093659,31.8557663374046,22.1196040350218));
#42206=CARTESIAN_POINT('Ctrl Pts',(131.371109441346,31.8986988450281,22.1264727344473));
#42207=CARTESIAN_POINT('Ctrl Pts',(131.450431645843,31.9349950042574,22.1319315290125));
#42208=CARTESIAN_POINT('Ctrl Pts',(131.723538170903,32.0729394316787,22.1513542509982));
#42209=CARTESIAN_POINT('Ctrl Pts',(131.908811211507,32.1902467193027,22.1656400187615));
#42210=CARTESIAN_POINT('Ctrl Pts',(132.155889216488,32.3824760425944,22.1855028250328));
#42211=CARTESIAN_POINT('Ctrl Pts',(132.227842605618,32.4434379493351,22.1914069512509));
#42212=CARTESIAN_POINT('Ctrl Pts',(132.347511495781,32.5537207462146,22.2014142791882));
#42213=CARTESIAN_POINT('Ctrl Pts',(132.39644239102,32.6016344557052,22.2055661635953));
#42214=CARTESIAN_POINT('Ctrl Pts',(132.466820776393,32.6748558788899,22.2116316019938));
#42215=CARTESIAN_POINT('Ctrl Pts',(132.489400375891,32.6990467602028,22.2135928873867));
#42216=CARTESIAN_POINT('Ctrl Pts',(132.529389047945,32.7431668255357,22.2170954949322));
#42217=CARTESIAN_POINT('Ctrl Pts',(132.546925606437,32.7629763194571,22.2186420499808));
#42218=CARTESIAN_POINT('Ctrl Pts',(132.584119253654,32.805995070664,22.2219461469238));
#42219=CARTESIAN_POINT('Ctrl Pts',(132.603699613965,32.8292677838951,22.2237005014157));
#42220=CARTESIAN_POINT('Ctrl Pts',(132.656497312567,32.8937641444607,22.2284752524685));
#42221=CARTESIAN_POINT('Ctrl Pts',(132.689067020178,32.9355081897514,22.2314702366486));
#42222=CARTESIAN_POINT('Ctrl Pts',(132.844777895187,33.1450206681745,22.2460733612258));
#42223=CARTESIAN_POINT('Ctrl Pts',(132.953268749604,33.3231208749942,22.2571329321252));
#42224=CARTESIAN_POINT('Ctrl Pts',(133.108862974259,33.6410835689277,22.2759002461628));
#42225=CARTESIAN_POINT('Ctrl Pts',(133.164451006296,33.7761012828577,22.2836121177139));
#42226=CARTESIAN_POINT('Ctrl Pts',(133.235008555733,33.9847832069708,22.2956830777815));
#42227=CARTESIAN_POINT('Ctrl Pts',(133.256518973634,34.0560571499957,22.2998326282347));
#42228=CARTESIAN_POINT('Ctrl Pts',(133.281758803934,34.1508678579977,22.3054558379164));
#42229=CARTESIAN_POINT('Ctrl Pts',(133.287612612132,34.173822363689,22.306825153783));
#42230=CARTESIAN_POINT('Ctrl Pts',(133.296907886937,34.2119358986912,22.3091146074694));
#42231=CARTESIAN_POINT('Ctrl Pts',(133.300486646168,34.2270611083601,22.310027283591));
#42232=CARTESIAN_POINT('Ctrl Pts',(133.307141211445,34.2560749947266,22.3117867817737));
#42233=CARTESIAN_POINT('Ctrl Pts',(133.310233832377,34.2699593403977,22.3126325494457));
#42234=CARTESIAN_POINT('Ctrl Pts',(133.318492379371,34.3081678375939,22.3149696093761));
#42235=CARTESIAN_POINT('Ctrl Pts',(133.323478071746,34.3325295209846,22.316470354316));
#42236=CARTESIAN_POINT('Ctrl Pts',(133.343231493596,34.4347650116555,22.322806569415));
#42237=CARTESIAN_POINT('Ctrl Pts',(133.355532632564,34.5130849098086,22.327752716831));
#42238=CARTESIAN_POINT('Ctrl Pts',(133.389570346978,34.7936523774992,22.3456386592823));
#42239=CARTESIAN_POINT('Ctrl Pts',(133.395844665388,34.9973401507769,22.3589026368601));
#42240=CARTESIAN_POINT('Ctrl Pts',(133.377410047656,35.3086717116608,22.3788060385034));
#42241=CARTESIAN_POINT('Ctrl Pts',(133.365800204845,35.4166161332438,22.3856444539914));
#42242=CARTESIAN_POINT('Ctrl Pts',(133.337366225192,35.5984063675791,22.3970057762071));
#42243=CARTESIAN_POINT('Ctrl Pts',(133.323212233505,35.6725810677805,22.4015975956624));
#42244=CARTESIAN_POINT('Ctrl Pts',(133.299041897516,35.7796819470606,22.4081650495854));
#42245=CARTESIAN_POINT('Ctrl Pts',(133.290984059915,35.8130224026534,22.4102006582429));
#42246=CARTESIAN_POINT('Ctrl Pts',(133.275788524362,35.8719636014081,22.4137848342835));
#42247=CARTESIAN_POINT('Ctrl Pts',(133.268853283851,35.8976130830391,22.415339651587));
#42248=CARTESIAN_POINT('Ctrl Pts',(133.25354022307,35.9517145561435,22.4186097633576));
#42249=CARTESIAN_POINT('Ctrl Pts',(133.245089091695,35.9801435849834,22.420322570466));
#42250=CARTESIAN_POINT('Ctrl Pts',(133.221182757798,36.0568618965568,22.4249319711405));
#42251=CARTESIAN_POINT('Ctrl Pts',(133.205015236119,36.1049222319788,22.4278056216876));
#42252=CARTESIAN_POINT('Ctrl Pts',(133.101020619476,36.3925418740706,22.4449531645621));
#42253=CARTESIAN_POINT('Ctrl Pts',(132.987456783248,36.6219169825006,22.4583380015484));
#42254=CARTESIAN_POINT('Ctrl Pts',(132.786553059797,36.93362593827,22.4780418999169));
#42255=CARTESIAN_POINT('Ctrl Pts',(132.718949908545,37.0275836869717,22.4842242586241));
#42256=CARTESIAN_POINT('Ctrl Pts',(132.606008170176,37.1687241021567,22.4941869821473));
#42257=CARTESIAN_POINT('Ctrl Pts',(132.563882135444,37.2183665425879,22.4978341145279));
#42258=CARTESIAN_POINT('Ctrl Pts',(132.505220196106,37.2835912821238,22.5028702924944));
#42259=CARTESIAN_POINT('Ctrl Pts',(132.489916645425,37.3002679005011,22.504180427774));
#42260=CARTESIAN_POINT('Ctrl Pts',(132.463962465363,37.3279882696322,22.5063987403585));
#42261=CARTESIAN_POINT('Ctrl Pts',(132.453401477663,37.3391155587159,22.5073004264546));
#42262=CARTESIAN_POINT('Ctrl Pts',(132.43127439494,37.3621144281745,22.5091884801486));
#42263=CARTESIAN_POINT('Ctrl Pts',(132.41969628198,37.3739733850324,22.5101756778734));
#42264=CARTESIAN_POINT('Ctrl Pts',(132.387949990605,37.4060162185056,22.5128792947267));
#42265=CARTESIAN_POINT('Ctrl Pts',(132.367613620259,37.4260306737635,22.514607738994));
#42266=CARTESIAN_POINT('Ctrl Pts',(132.228178273114,37.5598358087644,22.5264204747788));
#42267=CARTESIAN_POINT('Ctrl Pts',(132.101183941304,37.6650617429714,22.5369827699567));
#42268=CARTESIAN_POINT('Ctrl Pts',(131.857631240868,37.8386026935512,22.5562500815089));
#42269=CARTESIAN_POINT('Ctrl Pts',(131.743659762656,37.9100021336918,22.5649240664566));
#42270=CARTESIAN_POINT('Ctrl Pts',(131.501289119615,38.0424748851552,22.5824549145191));
#42271=CARTESIAN_POINT('Ctrl Pts',(131.372672852509,38.102627893106,22.5912768848468));
#42272=CARTESIAN_POINT('Ctrl Pts',(131.2014989398,38.1699488019296,22.6023707342677));
#42273=CARTESIAN_POINT('Ctrl Pts',(131.162061675625,38.184617404044,22.6048846454384));
#42274=CARTESIAN_POINT('Ctrl Pts',(131.096044621136,38.2077825716159,22.6090251267297));
#42275=CARTESIAN_POINT('Ctrl Pts',(131.069615551006,38.2166916981156,22.6106649514572));
#42276=CARTESIAN_POINT('Ctrl Pts',(131.017385630406,38.2335832653519,22.6138717852138));
#42277=CARTESIAN_POINT('Ctrl Pts',(130.991593427256,38.2415855366864,22.6154393351417));
#42278=CARTESIAN_POINT('Ctrl Pts',(130.934351213932,38.2585983118098,22.6188842563285));
#42279=CARTESIAN_POINT('Ctrl Pts',(130.902860639959,38.267463529833,22.6207568927906));
#42280=CARTESIAN_POINT('Ctrl Pts',(130.792270079824,38.2968760272587,22.6272596072203));
#42281=CARTESIAN_POINT('Ctrl Pts',(130.712556942729,38.3150184661321,22.6318149187634));
#42282=CARTESIAN_POINT('Ctrl Pts',(130.402005222193,38.3739777361348,22.6491692540504));
#42283=CARTESIAN_POINT('Ctrl Pts',(130.167842092549,38.3936948931545,22.6613789063015));
#42284=CARTESIAN_POINT('Ctrl Pts',(129.794137748322,38.3863636728052,22.6813432456586));
#42285=CARTESIAN_POINT('Ctrl Pts',(129.655076647279,38.3750345481003,22.688893227768));
#42286=CARTESIAN_POINT('Ctrl Pts',(129.489518099407,38.3512074144264,22.6984232142029));
#42287=CARTESIAN_POINT('Ctrl Pts',(129.46196371905,38.3468940466031,22.700027642007));
#42288=CARTESIAN_POINT('Ctrl Pts',(129.418261066098,38.3394992162868,22.7026059371517));
#42289=CARTESIAN_POINT('Ctrl Pts',(129.402076003878,38.3366393381747,22.7035681527394));
#42290=CARTESIAN_POINT('Ctrl Pts',(129.370929901212,38.33090197641,22.7054351061322));
#42291=CARTESIAN_POINT('Ctrl Pts',(129.355966417397,38.328041147202,22.7063389490415));
#42292=CARTESIAN_POINT('Ctrl Pts',(129.318578288807,38.3206314270518,22.708613824594));
#42293=CARTESIAN_POINT('Ctrl Pts',(129.29617966386,38.3159561961234,22.7099915478526));
#42294=CARTESIAN_POINT('Ctrl Pts',(129.213279648547,38.2977748473846,22.7151416779097));
#42295=CARTESIAN_POINT('Ctrl Pts',(129.153107918049,38.282837291225,22.7189808451553));
#42296=CARTESIAN_POINT('Ctrl Pts',(128.881368540787,38.2074105303201,22.7366819321574));
#42297=CARTESIAN_POINT('Ctrl Pts',(128.675591133847,38.1280600251235,22.7510597703895));
#42298=CARTESIAN_POINT('Ctrl Pts',(128.379428464306,37.9793549700602,22.7722300759681));
#42299=CARTESIAN_POINT('Ctrl Pts',(128.282417992703,37.9245039862599,22.7792576601911));
#42300=CARTESIAN_POINT('Ctrl Pts',(128.123336891405,37.8239058718173,22.7908882365194));
#42301=CARTESIAN_POINT('Ctrl Pts',(128.05980787254,37.7806410619385,22.7955646577103));
#42302=CARTESIAN_POINT('Ctrl Pts',(127.96994586295,37.714862217285,22.8022278624333));
#42303=CARTESIAN_POINT('Ctrl Pts',(127.942403788916,37.6940479993052,22.8042771196634));
#42304=CARTESIAN_POINT('Ctrl Pts',(127.894213733997,37.6564594001493,22.8078765330194));
#42305=CARTESIAN_POINT('Ctrl Pts',(127.873436587783,37.6398561431246,22.8094331265583));
#42306=CARTESIAN_POINT('Ctrl Pts',(127.830000583806,37.6043002963895,22.812698331685));
#42307=CARTESIAN_POINT('Ctrl Pts',(127.807389644208,37.5852925187517,22.8144045709163));
#42308=CARTESIAN_POINT('Ctrl Pts',(127.747091646594,37.5332431249565,22.8189747654545));
#42309=CARTESIAN_POINT('Ctrl Pts',(127.709883451692,37.4996566438239,22.8218164680694));
#42310=CARTESIAN_POINT('Ctrl Pts',(127.484500890073,37.2869534792309,22.839199694401));
#42311=CARTESIAN_POINT('Ctrl Pts',(127.316693390111,37.0875268759518,22.8528117594899));
#42312=CARTESIAN_POINT('Ctrl Pts',(127.110822079402,36.7764772119614,22.8726394952216));
#42313=CARTESIAN_POINT('Ctrl Pts',(127.05311350517,36.6790108527592,22.878695607623));
#42314=CARTESIAN_POINT('Ctrl Pts',(126.970468729821,36.5219962967475,22.8884803264613));
#42315=CARTESIAN_POINT('Ctrl Pts',(126.942169542937,36.4643101739823,22.8920813498675));
#42316=CARTESIAN_POINT('Ctrl Pts',(126.906184228397,36.3853579421258,22.8970634009128));
#42317=CARTESIAN_POINT('Ctrl Pts',(126.897045130289,36.364765061904,22.8983676727469));
#42318=CARTESIAN_POINT('Ctrl Pts',(126.882036745769,36.3300169098345,22.9005790065444));
#42319=CARTESIAN_POINT('Ctrl Pts',(126.876056766035,36.3159097612529,22.9014796719121));
#42320=CARTESIAN_POINT('Ctrl Pts',(126.863793174131,36.2864244106126,22.9033690317465));
#42321=CARTESIAN_POINT('Ctrl Pts',(126.857526691458,36.2710399279242,22.9043585977638));
#42322=CARTESIAN_POINT('Ctrl Pts',(126.841006255287,36.2296125222993,22.9070321642731));
#42323=CARTESIAN_POINT('Ctrl Pts',(126.830961582237,36.2034881918925,22.9087274645162));
#42324=CARTESIAN_POINT('Ctrl Pts',(126.821241918358,36.1772434416451,22.910437766625));
#42325=CARTESIAN_POINT('Origin',(130.,35.,23.));
#42326=CARTESIAN_POINT('',(126.821241956411,36.1772435443955,24.1659079080442));
#42327=CARTESIAN_POINT('',(126.821241887301,36.1772433577858,23.8178898623416));
#42328=CARTESIAN_POINT('',(126.821241918358,36.1772434416438,23.));
#42329=CARTESIAN_POINT('',(126.610250686301,34.9978429702395,22.6387451035351));
#42330=CARTESIAN_POINT('Ctrl Pts',(126.821241887301,36.1772433577858,23.8178898623416));
#42331=CARTESIAN_POINT('Ctrl Pts',(126.830547905651,36.2023711965905,23.8162403472402));
#42332=CARTESIAN_POINT('Ctrl Pts',(126.840153832804,36.2273939784003,23.8145991736083));
#42333=CARTESIAN_POINT('Ctrl Pts',(126.869647398543,36.3015795205453,23.8097380037057));
#42334=CARTESIAN_POINT('Ctrl Pts',(126.890390921278,36.3503882810981,23.806545709812));
#42335=CARTESIAN_POINT('Ctrl Pts',(126.924828261293,36.4264115288566,23.8015809576627));
#42336=CARTESIAN_POINT('Ctrl Pts',(126.937757562149,36.453960939806,23.7997833655218));
#42337=CARTESIAN_POINT('Ctrl Pts',(126.962616510146,36.5051266937263,23.7964466480327));
#42338=CARTESIAN_POINT('Ctrl Pts',(126.974454965761,36.5287845279524,23.7949045717327));
#42339=CARTESIAN_POINT('Ctrl Pts',(127.001710040821,36.5816938744458,23.7914563267144));
#42340=CARTESIAN_POINT('Ctrl Pts',(127.017280253988,36.610863500984,23.7895556341927));
#42341=CARTESIAN_POINT('Ctrl Pts',(127.066324063279,36.6995934450194,23.7837711528408));
#42342=CARTESIAN_POINT('Ctrl Pts',(127.10117437948,36.7583751788372,23.7799354319769));
#42343=CARTESIAN_POINT('Ctrl Pts',(127.272238822473,37.0279821809498,23.762251831542));
#42344=CARTESIAN_POINT('Ctrl Pts',(127.429812642212,37.2243053300573,23.7491758856208));
#42345=CARTESIAN_POINT('Ctrl Pts',(127.709945733416,37.5033815381431,23.728081293334));
#42346=CARTESIAN_POINT('Ctrl Pts',(127.818673349209,37.5986675706755,23.7202757994235));
#42347=CARTESIAN_POINT('Ctrl Pts',(127.955551895266,37.7039669215246,23.710441410592));
#42348=CARTESIAN_POINT('Ctrl Pts',(127.978185716253,37.7209322036546,23.7088148520134));
#42349=CARTESIAN_POINT('Ctrl Pts',(128.014370949682,37.7473542324302,23.7062092541366));
#42350=CARTESIAN_POINT('Ctrl Pts',(128.027784243159,37.7569989095818,23.7052422944716));
#42351=CARTESIAN_POINT('Ctrl Pts',(128.053810544193,37.7754257094152,23.7033628262939));
#42352=CARTESIAN_POINT('Ctrl Pts',(128.066413627713,37.7842207119801,23.702451173637));
#42353=CARTESIAN_POINT('Ctrl Pts',(128.097847731293,37.8058404969463,23.7001743599675));
#42354=CARTESIAN_POINT('Ctrl Pts',(128.116748914716,37.8185615898077,23.6988027053274));
#42355=CARTESIAN_POINT('Ctrl Pts',(128.191180318661,37.8675733649739,23.6933955439765));
#42356=CARTESIAN_POINT('Ctrl Pts',(128.247639746503,37.9024193366012,23.6892819250367));
#42357=CARTESIAN_POINT('Ctrl Pts',(128.408440789845,37.9952610783694,23.6776074624184));
#42358=CARTESIAN_POINT('Ctrl Pts',(128.514875751083,38.0494348778509,23.6699297970736));
#42359=CARTESIAN_POINT('Ctrl Pts',(128.851015294822,38.1987460251132,23.6462237163329));
#42360=CARTESIAN_POINT('Ctrl Pts',(129.088528564994,38.2743546591568,23.6302831421948));
#42361=CARTESIAN_POINT('Ctrl Pts',(129.382064297564,38.333338764372,23.6120820566831));
#42362=CARTESIAN_POINT('Ctrl Pts',(129.432149098051,38.3422354230369,23.6090239068376));
#42363=CARTESIAN_POINT('Ctrl Pts',(129.512032589675,38.354577599804,23.604219317334));
#42364=CARTESIAN_POINT('Ctrl Pts',(129.541707973085,38.3587604218032,23.6024503552779));
#42365=CARTESIAN_POINT('Ctrl Pts',(129.597735815717,38.3659012943057,23.5991393061216));
#42366=CARTESIAN_POINT('Ctrl Pts',(129.624074926968,38.3689447005368,23.5975946906248));
#42367=CARTESIAN_POINT('Ctrl Pts',(129.68403140195,38.3751605742381,23.5941045326031));
#42368=CARTESIAN_POINT('Ctrl Pts',(129.717666169719,38.3781404325842,23.5921650593183));
#42369=CARTESIAN_POINT('Ctrl Pts',(129.82347051327,38.3859228070902,23.5861176012113));
#42370=CARTESIAN_POINT('Ctrl Pts',(129.895754711126,38.3889186846575,23.5820645640413));
#42371=CARTESIAN_POINT('Ctrl Pts',(130.070020260236,38.3905595878107,23.5724362132522));
#42372=CARTESIAN_POINT('Ctrl Pts',(130.17195295865,38.3869206098284,23.5669230563533));
#42373=CARTESIAN_POINT('Ctrl Pts',(130.321069444576,38.3748467142612,23.5589198326161));
#42374=CARTESIAN_POINT('Ctrl Pts',(130.368481742101,38.3699995893997,23.5563840398085));
#42375=CARTESIAN_POINT('Ctrl Pts',(130.622548086591,38.3385994770582,23.542791210834));
#42376=CARTESIAN_POINT('Ctrl Pts',(130.8265038965,38.2940382507515,23.5318872718909));
#42377=CARTESIAN_POINT('Ctrl Pts',(131.069845818878,38.2168373985469,23.5176400665579));
#42378=CARTESIAN_POINT('Ctrl Pts',(131.114331281821,38.2016992789401,23.5149816532573));
#42379=CARTESIAN_POINT('Ctrl Pts',(131.176066206146,38.1792488579611,23.5111981605724));
#42380=CARTESIAN_POINT('Ctrl Pts',(131.193593337823,38.172710187193,23.5101132193481));
#42381=CARTESIAN_POINT('Ctrl Pts',(131.225191884207,38.1606231471985,23.508136190163));
#42382=CARTESIAN_POINT('Ctrl Pts',(131.239282227988,38.1551249397208,23.5072469433335));
#42383=CARTESIAN_POINT('Ctrl Pts',(131.268812697216,38.1433734881624,23.5053663292103));
#42384=CARTESIAN_POINT('Ctrl Pts',(131.284244114081,38.1371005046665,23.5043739073764));
#42385=CARTESIAN_POINT('Ctrl Pts',(131.326344230695,38.1196238204367,23.5016410214345));
#42386=CARTESIAN_POINT('Ctrl Pts',(131.352916149311,38.108192331765,23.4998881126267));
#42387=CARTESIAN_POINT('Ctrl Pts',(131.412672445447,38.0815731933556,23.495887621898));
#42388=CARTESIAN_POINT('Ctrl Pts',(131.445764155099,38.0661869790508,23.4936308696321));
#42389=CARTESIAN_POINT('Ctrl Pts',(131.553727501971,38.0138524095655,23.4861457701705));
#42390=CARTESIAN_POINT('Ctrl Pts',(131.627480454689,37.9746733292204,23.4808367979217));
#42391=CARTESIAN_POINT('Ctrl Pts',(131.928332473327,37.8003150156067,23.4585491224898));
#42392=CARTESIAN_POINT('Ctrl Pts',(132.140716566043,37.6415141943275,23.4413574051443));
#42393=CARTESIAN_POINT('Ctrl Pts',(132.38691259932,37.4080440285661,23.420413188827));
#42394=CARTESIAN_POINT('Ctrl Pts',(132.439598327208,37.3546526529745,23.415852934522));
#42395=CARTESIAN_POINT('Ctrl Pts',(132.513434973223,37.2746857799418,23.4093431375153));
#42396=CARTESIAN_POINT('Ctrl Pts',(132.53602388301,37.2494741055551,23.4073342022896));
#42397=CARTESIAN_POINT('Ctrl Pts',(132.575672454448,37.2038654966798,23.4037753068264));
#42398=CARTESIAN_POINT('Ctrl Pts',(132.592876651251,37.1835985096205,23.4022195207993));
#42399=CARTESIAN_POINT('Ctrl Pts',(132.62872346103,37.140348940527,23.3989521733954));
#42400=CARTESIAN_POINT('Ctrl Pts',(132.647307193935,37.1173203165586,23.3972430353738));
#42401=CARTESIAN_POINT('Ctrl Pts',(132.696706429265,37.0544383733391,23.392655528209));
#42402=CARTESIAN_POINT('Ctrl Pts',(132.726939589997,37.014135903102,23.3897997155891));
#42403=CARTESIAN_POINT('Ctrl Pts',(132.847162076772,36.8462008286175,23.3782171813563));
#42404=CARTESIAN_POINT('Ctrl Pts',(132.929181780527,36.7130937255067,23.3697791330597));
#42405=CARTESIAN_POINT('Ctrl Pts',(133.10783028303,36.372569395749,23.3492808596052));
#42406=CARTESIAN_POINT('Ctrl Pts',(133.193206456312,36.1601597270009,23.3374180636593));
#42407=CARTESIAN_POINT('Ctrl Pts',(133.271582899674,35.8888608463141,23.321743558704));
#42408=CARTESIAN_POINT('Ctrl Pts',(133.285343064003,35.8365695243158,23.3186975522804));
#42409=CARTESIAN_POINT('Ctrl Pts',(133.302866097039,35.7628576105985,23.3143411163534));
#42410=CARTESIAN_POINT('Ctrl Pts',(133.307683006941,35.7416935092293,23.3130831286661));
#42411=CARTESIAN_POINT('Ctrl Pts',(133.315523124015,35.7056500351109,23.3109263262032));
#42412=CARTESIAN_POINT('Ctrl Pts',(133.318650288667,35.6907936116608,23.3100331696896));
#42413=CARTESIAN_POINT('Ctrl Pts',(133.325056645912,35.6593106548338,23.308130896282));
#42414=CARTESIAN_POINT('Ctrl Pts',(133.328311078969,35.6426799924452,23.3071205554749));
#42415=CARTESIAN_POINT('Ctrl Pts',(133.337033955339,35.5962606050892,23.304286584668));
#42416=CARTESIAN_POINT('Ctrl Pts',(133.342227933832,35.5664226592599,23.3024490157616));
#42417=CARTESIAN_POINT('Ctrl Pts',(133.374400550104,35.3657174218867,23.2899998445854));
#42418=CARTESIAN_POINT('Ctrl Pts',(133.388663002471,35.1930834819671,23.2788744273161));
#42419=CARTESIAN_POINT('Ctrl Pts',(133.391152529776,34.7739231627998,23.2518569552887));
#42420=CARTESIAN_POINT('Ctrl Pts',(133.365785569443,34.5282486079279,23.2360675279682));
#42421=CARTESIAN_POINT('Ctrl Pts',(133.303275536915,34.2375130499535,23.21798619962));
#42422=CARTESIAN_POINT('Ctrl Pts',(133.291407094403,34.1878082825827,23.2149136047277));
#42423=CARTESIAN_POINT('Ctrl Pts',(133.270789250371,34.1093576719016,23.2100917453265));
#42424=CARTESIAN_POINT('Ctrl Pts',(133.26277406109,34.0804285835136,23.2083196827582));
#42425=CARTESIAN_POINT('Ctrl Pts',(133.24695981027,34.0261624493708,23.2050059264274));
#42426=CARTESIAN_POINT('Ctrl Pts',(133.239245800273,34.0008031781776,23.203461657858));
#42427=CARTESIAN_POINT('Ctrl Pts',(133.221055268759,33.9434288755988,23.1999764020385));
#42428=CARTESIAN_POINT('Ctrl Pts',(133.210397314652,33.9114740316752,23.1980414153903));
#42429=CARTESIAN_POINT('Ctrl Pts',(133.175517156584,33.8118675768563,23.1920248474812));
#42430=CARTESIAN_POINT('Ctrl Pts',(133.149618535503,33.7448219467027,23.1879973806875));
#42431=CARTESIAN_POINT('Ctrl Pts',(133.082242563894,33.5856508050343,23.1784453312118));
#42432=CARTESIAN_POINT('Ctrl Pts',(133.038740474553,33.4944565624926,23.1729814907204));
#42433=CARTESIAN_POINT('Ctrl Pts',(132.93131867709,33.2929574500799,23.1607615617631));
#42434=CARTESIAN_POINT('Ctrl Pts',(132.865122594727,33.1840439979205,23.1540517333381));
#42435=CARTESIAN_POINT('Ctrl Pts',(132.708732522234,32.9566539985611,23.1393728012354));
#42436=CARTESIAN_POINT('Ctrl Pts',(132.616554587467,32.8398776552014,23.1313965047221));
#42437=CARTESIAN_POINT('Ctrl Pts',(132.493011915511,32.7029188610765,23.1209841801166));
#42438=CARTESIAN_POINT('Ctrl Pts',(132.468580821941,32.6766836889493,23.11893692044));
#42439=CARTESIAN_POINT('Ctrl Pts',(132.431210834953,32.637809119185,23.1158140339933));
#42440=CARTESIAN_POINT('Ctrl Pts',(132.418578608063,32.6248769787422,23.1147598324543));
#42441=CARTESIAN_POINT('Ctrl Pts',(132.395316354249,32.6014404428891,23.1128197272405));
#42442=CARTESIAN_POINT('Ctrl Pts',(132.384719448506,32.5909044204095,23.1119362689814));
#42443=CARTESIAN_POINT('Ctrl Pts',(132.359954649903,32.5666054068545,23.1098725721881));
#42444=CARTESIAN_POINT('Ctrl Pts',(132.345735802835,32.5528958548086,23.1086885123181));
#42445=CARTESIAN_POINT('Ctrl Pts',(132.298701197794,32.5083325507467,23.1047768897899));
#42446=CARTESIAN_POINT('Ctrl Pts',(132.265391460201,32.478009716113,23.1020148030263));
#42447=CARTESIAN_POINT('Ctrl Pts',(132.181546914975,32.4046849973098,23.0951031576372));
#42448=CARTESIAN_POINT('Ctrl Pts',(132.130335470072,32.3624866248943,23.0909169836351));
#42449=CARTESIAN_POINT('Ctrl Pts',(131.862779027798,32.1548973696357,23.0693496036981));
#42450=CARTESIAN_POINT('Ctrl Pts',(131.628269995534,32.0144812308314,23.0515299962715));
#42451=CARTESIAN_POINT('Ctrl Pts',(131.299464897008,31.8679926929895,23.0291444801164));
#42452=CARTESIAN_POINT('Ctrl Pts',(131.218090485511,31.8354563651473,23.02378555024));
#42453=CARTESIAN_POINT('Ctrl Pts',(131.100659059866,31.7937053700561,23.0163067535523));
#42454=CARTESIAN_POINT('Ctrl Pts',(131.065575255356,31.7818755216247,23.0141037029132));
#42455=CARTESIAN_POINT('Ctrl Pts',(131.004625045332,31.7624299100802,23.0103288184475));
#42456=CARTESIAN_POINT('Ctrl Pts',(130.978849142318,31.7545437935648,23.0087483980022));
#42457=CARTESIAN_POINT('Ctrl Pts',(130.925648073195,31.7389584589469,23.0055181939572));
#42458=CARTESIAN_POINT('Ctrl Pts',(130.898214379346,31.7312957783666,23.0038696869105));
#42459=CARTESIAN_POINT('Ctrl Pts',(130.827195331541,31.712420638472,22.9996443693254));
#42460=CARTESIAN_POINT('Ctrl Pts',(130.783476719666,31.7017285327599,22.9970841078204));
#42461=CARTESIAN_POINT('Ctrl Pts',(130.544738045398,31.6483561138424,22.9833029529771));
#42462=CARTESIAN_POINT('Ctrl Pts',(130.346445874397,31.6220948758561,22.9726074116107));
#42463=CARTESIAN_POINT('Ctrl Pts',(129.931890220432,31.6041031151512,22.9505824317376));
#42464=CARTESIAN_POINT('Ctrl Pts',(129.716425650023,31.6152812506665,22.9393132303251));
#42465=CARTESIAN_POINT('Ctrl Pts',(129.463150866573,31.6527829477532,22.9249304985064));
#42466=CARTESIAN_POINT('Ctrl Pts',(129.422912539357,31.6594852576506,22.9226099237233));
#42467=CARTESIAN_POINT('Ctrl Pts',(129.364115777614,31.6703727456152,22.9191541130007));
#42468=CARTESIAN_POINT('Ctrl Pts',(129.345454626718,31.6739908726697,22.9180476369328));
#42469=CARTESIAN_POINT('Ctrl Pts',(129.312212399634,31.6807266479543,22.9160577735641));
#42470=CARTESIAN_POINT('Ctrl Pts',(129.297619999223,31.6837838300989,22.9151776850011));
#42471=CARTESIAN_POINT('Ctrl Pts',(129.264765924357,31.6908935041108,22.9131811625249));
#42472=CARTESIAN_POINT('Ctrl Pts',(129.246517414978,31.6950009219945,22.9120618461793));
#42473=CARTESIAN_POINT('Ctrl Pts',(129.190196259282,31.7081685089321,22.9085771179016));
#42474=CARTESIAN_POINT('Ctrl Pts',(129.152247076564,31.7177368533767,22.9061863826025));
#42475=CARTESIAN_POINT('Ctrl Pts',(129.061776074907,31.7422214033854,22.9003976787353));
#42476=CARTESIAN_POINT('Ctrl Pts',(129.009432914097,31.7577535863735,22.8969758089811));
#42477=CARTESIAN_POINT('Ctrl Pts',(128.796644150592,31.8265296703261,22.8828236366041));
#42478=CARTESIAN_POINT('Ctrl Pts',(128.63991552364,31.8904746514034,22.8718441817082));
#42479=CARTESIAN_POINT('Ctrl Pts',(128.329335624545,32.0451819352462,22.849567343045));
#42480=CARTESIAN_POINT('Ctrl Pts',(128.176536004306,32.1369486958906,22.8383220110877));
#42481=CARTESIAN_POINT('Ctrl Pts',(127.98867194196,32.2709435508528,22.8242737343379));
#42482=CARTESIAN_POINT('Ctrl Pts',(127.946430570228,32.3025859189739,22.8210972684933));
#42483=CARTESIAN_POINT('Ctrl Pts',(127.881063779893,32.3539771243669,22.816151388328));
#42484=CARTESIAN_POINT('Ctrl Pts',(127.857437065946,32.3730717697567,22.8143571542829));
#42485=CARTESIAN_POINT('Ctrl Pts',(127.813910549841,32.409226994761,22.8110383123983));
#42486=CARTESIAN_POINT('Ctrl Pts',(127.793945945349,32.4262056388246,22.8095106198039));
#42487=CARTESIAN_POINT('Ctrl Pts',(127.74928218921,32.4650908973408,22.8060794495788));
#42488=CARTESIAN_POINT('Ctrl Pts',(127.724701934007,32.4871303966919,22.8041815762958));
#42489=CARTESIAN_POINT('Ctrl Pts',(127.650462825326,32.5556783007006,22.7984158708846));
#42490=CARTESIAN_POINT('Ctrl Pts',(127.601877412958,32.6033268015824,22.7945956338806));
#42491=CARTESIAN_POINT('Ctrl Pts',(127.381317544598,32.8330611337664,22.7769546290891));
#42492=CARTESIAN_POINT('Ctrl Pts',(127.228435384902,33.0323729753638,22.7639032732564));
#42493=CARTESIAN_POINT('Ctrl Pts',(127.02369088658,33.3711564030175,22.7427901419689));
#42494=CARTESIAN_POINT('Ctrl Pts',(126.956575650725,33.5002977236927,22.7349353508669));
#42495=CARTESIAN_POINT('Ctrl Pts',(126.886557478309,33.6592236657159,22.7250457464277));
#42496=CARTESIAN_POINT('Ctrl Pts',(126.875475691326,33.68525544379,22.7234188436114));
#42497=CARTESIAN_POINT('Ctrl Pts',(126.858440665005,33.7267038866486,22.7208128210263));
#42498=CARTESIAN_POINT('Ctrl Pts',(126.852271858339,33.7420311733536,22.7198457875952));
#42499=CARTESIAN_POINT('Ctrl Pts',(126.84058188203,33.7717010133015,22.7179662888178));
#42500=CARTESIAN_POINT('Ctrl Pts',(126.835045811053,33.7860369888344,22.7170546808426));
#42501=CARTESIAN_POINT('Ctrl Pts',(126.821546146027,33.8217151985876,22.7147781430227));
#42502=CARTESIAN_POINT('Ctrl Pts',(126.813699917688,33.8431008260554,22.7134067229216));
#42503=CARTESIAN_POINT('Ctrl Pts',(126.783860381062,33.9270380335679,22.7080017489805));
#42504=CARTESIAN_POINT('Ctrl Pts',(126.763489976588,33.9901469809117,22.7038901598557));
#42505=CARTESIAN_POINT('Ctrl Pts',(126.711696343838,34.1683233903572,22.6922238737635));
#42506=CARTESIAN_POINT('Ctrl Pts',(126.684476017317,34.284510585506,22.6845525239304));
#42507=CARTESIAN_POINT('Ctrl Pts',(126.628177866672,34.5985676272096,22.6639883048161));
#42508=CARTESIAN_POINT('Ctrl Pts',(126.610377855726,34.7979975720025,22.6511321729077));
#42509=CARTESIAN_POINT('Ctrl Pts',(126.610250686301,34.9978429702395,22.6387451035351));
#42510=CARTESIAN_POINT('Ctrl Pts',(126.610250683863,34.9978468054472,22.6387448658165));
#42511=CARTESIAN_POINT('Ctrl Pts',(126.610218691457,35.0482120802422,22.6356230633535));
#42512=CARTESIAN_POINT('Ctrl Pts',(126.611309197226,35.0985740946989,22.6325308277824));
#42513=CARTESIAN_POINT('Ctrl Pts',(126.615250243622,35.1882091841631,22.6270804172804));
#42514=CARTESIAN_POINT('Ctrl Pts',(126.617663277397,35.2274908769275,22.6247100370017));
#42515=CARTESIAN_POINT('Ctrl Pts',(126.622844397037,35.2931329588712,22.6207786219727));
#42516=CARTESIAN_POINT('Ctrl Pts',(126.62523851526,35.3195181983972,22.6192063880327));
#42517=CARTESIAN_POINT('Ctrl Pts',(126.630507067345,35.3708834463182,22.6161606738392));
#42518=CARTESIAN_POINT('Ctrl Pts',(126.633350590916,35.3958648266516,22.61468634392));
#42519=CARTESIAN_POINT('Ctrl Pts',(126.639972341806,35.4487920358022,22.6115766609327));
#42520=CARTESIAN_POINT('Ctrl Pts',(126.643821894405,35.4767271217682,22.6099436367488));
#42521=CARTESIAN_POINT('Ctrl Pts',(126.654511193208,35.5477328674716,22.6058120864575));
#42522=CARTESIAN_POINT('Ctrl Pts',(126.661834417446,35.5907261954345,22.6033286663749));
#42523=CARTESIAN_POINT('Ctrl Pts',(126.699004962162,35.7860935711715,22.5921112890358));
#42524=CARTESIAN_POINT('Ctrl Pts',(126.738470652228,35.9364532919305,22.5836777855363));
#42525=CARTESIAN_POINT('Ctrl Pts',(126.798698710943,36.1149763763543,22.5736078810968));
#42526=CARTESIAN_POINT('Ctrl Pts',(126.809744069168,36.1461972859097,22.571844118041));
#42527=CARTESIAN_POINT('Ctrl Pts',(126.821241895364,36.1772433795577,22.5700842967619));
#42528=CARTESIAN_POINT('Ctrl Pts',(126.821241918358,36.1772434416451,22.910437766625));
#42529=CARTESIAN_POINT('Ctrl Pts',(126.820991045024,36.1765660408554,22.9104819110725));
#42530=CARTESIAN_POINT('Ctrl Pts',(126.820740388213,36.1758885598419,22.910526065518));
#42531=CARTESIAN_POINT('Ctrl Pts',(126.762030801805,36.0170509380546,22.9208793282995));
#42532=CARTESIAN_POINT('Ctrl Pts',(126.715459346813,35.8547629778948,22.9317036025874));
#42533=CARTESIAN_POINT('Ctrl Pts',(126.652004445497,35.5494179881511,22.951800467092));
#42534=CARTESIAN_POINT('Ctrl Pts',(126.631773956849,35.4074205119328,22.9610436925096));
#42535=CARTESIAN_POINT('Ctrl Pts',(126.613747492658,35.1771592767367,22.9756515719051));
#42536=CARTESIAN_POINT('Ctrl Pts',(126.610297959855,35.0895173841033,22.9811257237269));
#42537=CARTESIAN_POINT('Ctrl Pts',(126.61021530294,34.936818897916,22.990495850361));
#42538=CARTESIAN_POINT('Ctrl Pts',(126.612050631336,34.8718123052779,22.9944323613035));
#42539=CARTESIAN_POINT('Ctrl Pts',(126.617604134971,34.7744847340311,23.0002494805929));
#42540=CARTESIAN_POINT('Ctrl Pts',(126.619919012245,34.7421016690371,23.0021722891916));
#42541=CARTESIAN_POINT('Ctrl Pts',(126.624960740196,34.6834357428838,23.0056338348393));
#42542=CARTESIAN_POINT('Ctrl Pts',(126.627530341423,34.6571423114836,23.0071772781116));
#42543=CARTESIAN_POINT('Ctrl Pts',(126.63377053995,34.6001771296514,23.0105049024812));
#42544=CARTESIAN_POINT('Ctrl Pts',(126.637553553801,34.5695199278666,23.0122854721365));
#42545=CARTESIAN_POINT('Ctrl Pts',(126.649479639371,34.4826574774102,23.017304110355));
#42546=CARTESIAN_POINT('Ctrl Pts',(126.65861696993,34.4265979281773,23.0205114836055));
#42547=CARTESIAN_POINT('Ctrl Pts',(126.682685970458,34.2991837440657,23.0277482056169));
#42548=CARTESIAN_POINT('Ctrl Pts',(126.698519210454,34.2280276787483,23.0317509489949));
#42549=CARTESIAN_POINT('Ctrl Pts',(126.765573149121,33.966727513005,23.0463955133786));
#42550=CARTESIAN_POINT('Ctrl Pts',(126.831032523688,33.7806496754215,23.0566936698902));
#42551=CARTESIAN_POINT('Ctrl Pts',(126.971708529375,33.4700968552031,23.074882759498));
#42552=CARTESIAN_POINT('Ctrl Pts',(127.039440357402,33.3428244037929,23.082667918556));
#42553=CARTESIAN_POINT('Ctrl Pts',(127.129901144472,33.196188050055,23.0924795150934));
#42554=CARTESIAN_POINT('Ctrl Pts',(127.145050913647,33.1723045672683,23.0941059015776));
#42555=CARTESIAN_POINT('Ctrl Pts',(127.169520150061,33.1347756697802,23.0967112886611));
#42556=CARTESIAN_POINT('Ctrl Pts',(127.178643912913,33.1210035157388,23.0976782129999));
#42557=CARTESIAN_POINT('Ctrl Pts',(127.19644938804,33.0945485456536,23.0995576704975));
#42558=CARTESIAN_POINT('Ctrl Pts',(127.205117267785,33.0818572113629,23.1004693485746));
#42559=CARTESIAN_POINT('Ctrl Pts',(127.226849289932,33.0504976586988,23.1027463106372));
#42560=CARTESIAN_POINT('Ctrl Pts',(127.240015820666,33.0319015503762,23.1041180900225));
#42561=CARTESIAN_POINT('Ctrl Pts',(127.292254821801,32.9596755409366,23.1095263979743));
#42562=CARTESIAN_POINT('Ctrl Pts',(127.332708979584,32.9070677793248,23.1136410789785));
#42563=CARTESIAN_POINT('Ctrl Pts',(127.450209079257,32.7632103827999,23.1253198157197));
#42564=CARTESIAN_POINT('Ctrl Pts',(127.530570304436,32.6747954991554,23.1330007812015));
#42565=CARTESIAN_POINT('Ctrl Pts',(127.791955440177,32.4160809980237,23.1567044337723));
#42566=CARTESIAN_POINT('Ctrl Pts',(127.987184945043,32.2612575279601,23.1726390998777));
#42567=CARTESIAN_POINT('Ctrl Pts',(128.24068915341,32.1021010800925,23.1908355258845));
#42568=CARTESIAN_POINT('Ctrl Pts',(128.284376938729,32.0760248400111,23.193894256953));
#42569=CARTESIAN_POINT('Ctrl Pts',(128.354709592771,32.0361641971151,23.198699544249));
#42570=CARTESIAN_POINT('Ctrl Pts',(128.380977642128,32.0217337456721,23.2004686338976));
#42571=CARTESIAN_POINT('Ctrl Pts',(128.430838663937,31.9951970638158,23.2037797986568));
#42572=CARTESIAN_POINT('Ctrl Pts',(128.454388872636,31.983015696808,23.2053244040204));
#42573=CARTESIAN_POINT('Ctrl Pts',(128.508246680073,31.9559538642707,23.208814374949));
#42574=CARTESIAN_POINT('Ctrl Pts',(128.53863878219,31.9412472554738,23.2107536739851));
#42575=CARTESIAN_POINT('Ctrl Pts',(128.634795826577,31.8964776820407,23.216799912662));
#42576=CARTESIAN_POINT('Ctrl Pts',(128.701307848315,31.8680624329588,23.2208519378052));
#42577=CARTESIAN_POINT('Ctrl Pts',(128.863624101897,31.8047786907942,23.2304772598761));
#42578=CARTESIAN_POINT('Ctrl Pts',(128.960191680524,31.7720610390162,23.235988456712));
#42579=CARTESIAN_POINT('Ctrl Pts',(129.103717917692,31.730544464895,23.2439814001364));
#42580=CARTESIAN_POINT('Ctrl Pts',(129.149617640359,31.718306686686,23.2465089516658));
#42581=CARTESIAN_POINT('Ctrl Pts',(129.397777717585,31.6576985568789,23.2600731109844));
#42582=CARTESIAN_POINT('Ctrl Pts',(129.603888448419,31.6270590688178,23.27095660855));
#42583=CARTESIAN_POINT('Ctrl Pts',(129.858824964905,31.6128592080461,23.2852007357883));
#42584=CARTESIAN_POINT('Ctrl Pts',(129.906213163451,31.6112160430695,23.2878824759269));
#42585=CARTESIAN_POINT('Ctrl Pts',(129.972391352175,31.6103104361192,23.2916938983876));
#42586=CARTESIAN_POINT('Ctrl Pts',(129.991166314496,31.6102095184953,23.292782664308));
#42587=CARTESIAN_POINT('Ctrl Pts',(130.02508178269,31.6103089784608,23.2947644288915));
#42588=CARTESIAN_POINT('Ctrl Pts',(130.040222210535,31.6104548262273,23.2956545382912));
#42589=CARTESIAN_POINT('Ctrl Pts',(130.071981331099,31.6109735830995,23.2975338471957));
#42590=CARTESIAN_POINT('Ctrl Pts',(130.088598903804,31.61136730006,23.2985240637229));
#42591=CARTESIAN_POINT('Ctrl Pts',(130.133958814,31.6127758791287,23.3012445796611));
#42592=CARTESIAN_POINT('Ctrl Pts',(130.162691565614,31.614034326185,23.3029871457164));
#42593=CARTESIAN_POINT('Ctrl Pts',(130.376229576136,31.6261111143128,23.3160641770337));
#42594=CARTESIAN_POINT('Ctrl Pts',(130.559873031074,31.6516861656024,23.3279985546282));
#42595=CARTESIAN_POINT('Ctrl Pts',(130.96989532433,31.7434725746539,23.355083154748));
#42596=CARTESIAN_POINT('Ctrl Pts',(131.193367220304,31.8185579226155,23.3701269114653));
#42597=CARTESIAN_POINT('Ctrl Pts',(131.454634121712,31.9377863027415,23.387601101697));
#42598=CARTESIAN_POINT('Ctrl Pts',(131.501474843771,31.9604791663651,23.3907323072274));
#42599=CARTESIAN_POINT('Ctrl Pts',(131.574662293488,31.9980411443712,23.3956241861937));
#42600=CARTESIAN_POINT('Ctrl Pts',(131.601362983871,32.0121989704975,23.3974087898721));
#42601=CARTESIAN_POINT('Ctrl Pts',(131.648772484437,32.0381556152005,23.4005783762225));
#42602=CARTESIAN_POINT('Ctrl Pts',(131.669552665223,32.0498191909558,23.4019679515779));
#42603=CARTESIAN_POINT('Ctrl Pts',(131.718007520089,32.0776920565041,23.4052097407483));
#42604=CARTESIAN_POINT('Ctrl Pts',(131.745578826942,32.0940770458146,23.4070555858349));
#42605=CARTESIAN_POINT('Ctrl Pts',(131.826530492941,32.143752700186,23.4124822725332));
#42606=CARTESIAN_POINT('Ctrl Pts',(131.879222682775,32.1781415561559,23.4160236447469));
#42607=CARTESIAN_POINT('Ctrl Pts',(132.057432311223,32.3016546988483,23.428073826773));
#42608=CARTESIAN_POINT('Ctrl Pts',(132.177823293654,32.3978496884418,23.4363342755972));
#42609=CARTESIAN_POINT('Ctrl Pts',(132.432127201846,32.63109801115,23.4546769479585));
#42610=CARTESIAN_POINT('Ctrl Pts',(132.56179911577,32.771970541328,23.4646804442863));
#42611=CARTESIAN_POINT('Ctrl Pts',(132.720457988631,32.9766084235078,23.47891602236));
#42612=CARTESIAN_POINT('Ctrl Pts',(132.760394783603,33.0314409913902,23.482706807058));
#42613=CARTESIAN_POINT('Ctrl Pts',(132.811993998189,33.1069459781343,23.4879486872838));
#42614=CARTESIAN_POINT('Ctrl Pts',(132.825125672649,33.1265997111924,23.4893150808563));
#42615=CARTESIAN_POINT('Ctrl Pts',(132.845703569156,33.1581063717356,23.4915113048036));
#42616=CARTESIAN_POINT('Ctrl Pts',(132.853284004639,33.1698712299973,23.4923326570048));
#42617=CARTESIAN_POINT('Ctrl Pts',(132.869269014327,33.1950207291062,23.4940918737467));
#42618=CARTESIAN_POINT('Ctrl Pts',(132.877653218377,33.2084178011201,23.4950310599182));
#42619=CARTESIAN_POINT('Ctrl Pts',(132.899033692813,33.243118823249,23.4974680142256));
#42620=CARTESIAN_POINT('Ctrl Pts',(132.911888725901,33.2645081995834,23.4989742465192));
#42621=CARTESIAN_POINT('Ctrl Pts',(132.968914712133,33.36181066487,23.5058379633032));
#42622=CARTESIAN_POINT('Ctrl Pts',(133.010358336426,33.4392760928862,23.511333584811));
#42623=CARTESIAN_POINT('Ctrl Pts',(133.137864867407,33.7016256654425,23.5298467141323));
#42624=CARTESIAN_POINT('Ctrl Pts',(133.210261002052,33.8926611336612,23.5431419976502));
#42625=CARTESIAN_POINT('Ctrl Pts',(133.306029671718,34.2359172180919,23.5658384522539));
#42626=CARTESIAN_POINT('Ctrl Pts',(133.33705384553,34.3853974850939,23.5753580462178));
#42627=CARTESIAN_POINT('Ctrl Pts',(133.363899805667,34.5798776584258,23.5872178965381));
#42628=CARTESIAN_POINT('Ctrl Pts',(133.369049152793,34.6233930960738,23.5898391577689));
#42629=CARTESIAN_POINT('Ctrl Pts',(133.376127783568,34.6951004868767,23.5941072072472));
#42630=CARTESIAN_POINT('Ctrl Pts',(133.378550736231,34.7232374322677,23.5957689864142));
#42631=CARTESIAN_POINT('Ctrl Pts',(133.382608107839,34.7784126162215,23.5990033198744));
#42632=CARTESIAN_POINT('Ctrl Pts',(133.384270617865,34.8054465952889,23.6005766217203));
#42633=CARTESIAN_POINT('Ctrl Pts',(133.387476474141,34.8702445546798,23.6043217909962));
#42634=CARTESIAN_POINT('Ctrl Pts',(133.388712628199,34.9080205246988,23.6064841005087));
#42635=CARTESIAN_POINT('Ctrl Pts',(133.390905763929,35.0451912823862,23.6142670098139));
#42636=CARTESIAN_POINT('Ctrl Pts',(133.388123031745,35.1445990175517,23.6197744850507));
#42637=CARTESIAN_POINT('Ctrl Pts',(133.368841502354,35.4120495621755,23.6343835536587));
#42638=CARTESIAN_POINT('Ctrl Pts',(133.344157514212,35.5792162243197,23.6432824012548));
#42639=CARTESIAN_POINT('Ctrl Pts',(133.26969183767,35.9102871861453,23.6612890226236));
#42640=CARTESIAN_POINT('Ctrl Pts',(133.219749184025,36.0736437526889,23.6703765168606));
#42641=CARTESIAN_POINT('Ctrl Pts',(133.144827057556,36.2655937969484,23.6820129487764));
#42642=CARTESIAN_POINT('Ctrl Pts',(133.1314032994,36.2984521743423,23.6840405581058));
#42643=CARTESIAN_POINT('Ctrl Pts',(133.110394990774,36.3476543971864,23.6871394033429));
#42644=CARTESIAN_POINT('Ctrl Pts',(133.103191638882,36.3641594458443,23.6881897026809));
#42645=CARTESIAN_POINT('Ctrl Pts',(133.089767837894,36.3942608468924,23.6901263775985));
#42646=CARTESIAN_POINT('Ctrl Pts',(133.0835884648,36.4078745519811,23.6910103733047));
#42647=CARTESIAN_POINT('Ctrl Pts',(133.068997150984,36.4394635833291,23.6930803427733));
#42648=CARTESIAN_POINT('Ctrl Pts',(133.060517211234,36.4574063531588,23.6942702211598));
#42649=CARTESIAN_POINT('Ctrl Pts',(133.032033595689,36.5163300782826,23.6982220130355));
#42650=CARTESIAN_POINT('Ctrl Pts',(133.011361259614,36.5569802718885,23.7010193888895));
#42651=CARTESIAN_POINT('Ctrl Pts',(132.958064203014,36.6567496917963,23.7080412184183));
#42652=CARTESIAN_POINT('Ctrl Pts',(132.924481529621,36.7153338540979,23.7123036745727));
#42653=CARTESIAN_POINT('Ctrl Pts',(132.738283491129,37.0187726811197,23.7349893323835));
#42654=CARTESIAN_POINT('Ctrl Pts',(132.556585850692,37.2444488319313,23.7538714155686));
#42655=CARTESIAN_POINT('Ctrl Pts',(132.293511631862,37.4972028835449,23.7764070360628));
#42656=CARTESIAN_POINT('Ctrl Pts',(132.236763711803,37.5481576332396,23.7810461544241));
#42657=CARTESIAN_POINT('Ctrl Pts',(132.152250731834,37.6190420965966,23.7876451362553));
#42658=CARTESIAN_POINT('Ctrl Pts',(132.125830511446,37.6405320448692,23.7896667089465));
#42659=CARTESIAN_POINT('Ctrl Pts',(132.078197381649,37.678097965243,23.7932398168382));
#42660=CARTESIAN_POINT('Ctrl Pts',(132.057110854539,37.6943288701668,23.7947973476644));
#42661=CARTESIAN_POINT('Ctrl Pts',(132.012265725829,37.7280140481446,23.7980601752366));
#42662=CARTESIAN_POINT('Ctrl Pts',(131.98846606496,37.7454101307536,23.799763157209));
#42663=CARTESIAN_POINT('Ctrl Pts',(131.923833722239,37.7913709500654,23.8043139224174));
#42664=CARTESIAN_POINT('Ctrl Pts',(131.88259235047,37.8193499907959,23.8071397917898));
#42665=CARTESIAN_POINT('Ctrl Pts',(131.789320868149,37.8796677994977,23.8133717403897));
#42666=CARTESIAN_POINT('Ctrl Pts',(131.73700060635,37.9115262766809,23.8167612185983));
#42667=CARTESIAN_POINT('Ctrl Pts',(131.561399150871,38.0120328562038,23.8278361040226));
#42668=CARTESIAN_POINT('Ctrl Pts',(131.434694004551,38.0744048953099,23.8353450126785));
#42669=CARTESIAN_POINT('Ctrl Pts',(131.10572997947,38.2115616680426,23.8542478941376));
#42670=CARTESIAN_POINT('Ctrl Pts',(130.899573310751,38.2752883140285,23.8655532104072));
#42671=CARTESIAN_POINT('Ctrl Pts',(130.65672521931,38.3256863741634,23.8795955671347));
#42672=CARTESIAN_POINT('Ctrl Pts',(130.624561217351,38.331876497226,23.8814701677594));
#42673=CARTESIAN_POINT('Ctrl Pts',(130.574928707429,38.3406846312721,23.8843924439984));
#42674=CARTESIAN_POINT('Ctrl Pts',(130.557520153186,38.3436339621925,23.8854229991198));
#42675=CARTESIAN_POINT('Ctrl Pts',(130.526769470808,38.3485968761796,23.8872544429829));
#42676=CARTESIAN_POINT('Ctrl Pts',(130.513437148415,38.3506670065454,23.8880522249649));
#42677=CARTESIAN_POINT('Ctrl Pts',(130.480884563198,38.3555226519605,23.8900090586031));
#42678=CARTESIAN_POINT('Ctrl Pts',(130.461652481773,38.3582226217893,23.8911726467208));
#42679=CARTESIAN_POINT('Ctrl Pts',(130.399655828344,38.3663836529264,23.8949453846792));
#42680=CARTESIAN_POINT('Ctrl Pts',(130.356811493864,38.3711939828922,23.8975859109875));
#42681=CARTESIAN_POINT('Ctrl Pts',(130.251766331356,38.3809630900562,23.9041227367526));
#42682=CARTESIAN_POINT('Ctrl Pts',(130.189498662944,38.3850239569588,23.9080511176068));
#42683=CARTESIAN_POINT('Ctrl Pts',(129.898612138814,38.3959434993859,23.9265542163559));
#42684=CARTESIAN_POINT('Ctrl Pts',(129.669781057678,38.3813720790272,23.9414957920195));
#42685=CARTESIAN_POINT('Ctrl Pts',(129.318781102657,38.3230253186719,23.9639851571508));
#42686=CARTESIAN_POINT('Ctrl Pts',(129.194674386032,38.2951499315762,23.9718618640757));
#42687=CARTESIAN_POINT('Ctrl Pts',(129.032287390868,38.2489502747913,23.9820412920123));
#42688=CARTESIAN_POINT('Ctrl Pts',(128.992373167529,38.2367937811066,23.9845334932294));
#42689=CARTESIAN_POINT('Ctrl Pts',(128.926234481771,38.2153081587685,23.9886482177712));
#42690=CARTESIAN_POINT('Ctrl Pts',(128.899883057568,38.2063876443464,23.9902836527663));
#42691=CARTESIAN_POINT('Ctrl Pts',(128.84782491827,38.1880475212083,23.9935075624008));
#42692=CARTESIAN_POINT('Ctrl Pts',(128.822116604895,38.1786388892469,23.9950962482949));
#42693=CARTESIAN_POINT('Ctrl Pts',(128.759680990087,38.1549274230296,23.9989477398151));
#42694=CARTESIAN_POINT('Ctrl Pts',(128.723083265356,38.1402933185247,24.0011995144406));
#42695=CARTESIAN_POINT('Ctrl Pts',(128.582512723536,38.0812203131108,24.009835081339));
#42696=CARTESIAN_POINT('Ctrl Pts',(128.480528833962,38.0322268266604,24.0160683901573));
#42697=CARTESIAN_POINT('Ctrl Pts',(128.189384764534,37.8739745551613,24.0340189001853));
#42698=CARTESIAN_POINT('Ctrl Pts',(128.008117640186,37.7514467796381,24.0453716552373));
#42699=CARTESIAN_POINT('Ctrl Pts',(127.749340308102,37.5374676319088,24.0634136231478));
#42700=CARTESIAN_POINT('Ctrl Pts',(127.662751094931,37.4579409069669,24.0698319668873));
#42701=CARTESIAN_POINT('Ctrl Pts',(127.561244346807,37.3544913931816,24.078094280142));
#42702=CARTESIAN_POINT('Ctrl Pts',(127.542254843493,37.3346621811819,24.0796744303567));
#42703=CARTESIAN_POINT('Ctrl Pts',(127.512349870862,37.3026656238794,24.0822227743127));
#42704=CARTESIAN_POINT('Ctrl Pts',(127.501277537835,37.2906457982934,24.0831797785276));
#42705=CARTESIAN_POINT('Ctrl Pts',(127.479892913285,37.2670916849648,24.0850556278928));
#42706=CARTESIAN_POINT('Ctrl Pts',(127.469571957248,37.2555660761954,24.0859738261498));
#42707=CARTESIAN_POINT('Ctrl Pts',(127.443889210031,37.2264875442427,24.088290290962));
#42708=CARTESIAN_POINT('Ctrl Pts',(127.428629168646,37.2088461098056,24.08969553583));
#42709=CARTESIAN_POINT('Ctrl Pts',(127.367621990318,37.1368295411859,24.0954266649304));
#42710=CARTESIAN_POINT('Ctrl Pts',(127.323410459365,37.0811827145054,24.0998424907736));
#42711=CARTESIAN_POINT('Ctrl Pts',(127.200823775203,36.9165168970774,24.1127799937611));
#42712=CARTESIAN_POINT('Ctrl Pts',(127.127134082419,36.8041793887822,24.1214455738092));
#42713=CARTESIAN_POINT('Ctrl Pts',(126.966564982019,36.5245064497519,24.1422305717618));
#42714=CARTESIAN_POINT('Ctrl Pts',(126.886606077617,36.3537378025582,24.1542830667824));
#42715=CARTESIAN_POINT('Ctrl Pts',(126.821241956411,36.1772435443955,24.1659079080442));
#42716=CARTESIAN_POINT('Origin',(130.,35.,23.));
#42717=CARTESIAN_POINT('',(126.821241938915,36.1772434971514,25.4139333020124));
#42718=CARTESIAN_POINT('',(126.821241918346,36.177243441613,25.0733700900595));
#42719=CARTESIAN_POINT('',(126.821241918358,36.1772434416438,23.));
#42720=CARTESIAN_POINT('Ctrl Pts',(126.821241918346,36.177243441613,25.0733700900595));
#42721=CARTESIAN_POINT('Ctrl Pts',(126.82271653249,36.1812251513086,25.0731092436031));
#42722=CARTESIAN_POINT('Ctrl Pts',(126.82419862865,36.1852040924822,25.0728480699998));
#42723=CARTESIAN_POINT('Ctrl Pts',(126.878017473958,36.3288642286552,25.0634002377664));
#42724=CARTESIAN_POINT('Ctrl Pts',(126.939505830955,36.4649312183301,25.0538394440563));
#42725=CARTESIAN_POINT('Ctrl Pts',(127.070403672287,36.710104269745,25.0359364811992));
#42726=CARTESIAN_POINT('Ctrl Pts',(127.137487035384,36.820168375137,25.0276193832681));
#42727=CARTESIAN_POINT('Ctrl Pts',(127.295509549523,37.0490064349424,25.0099311780473));
#42728=CARTESIAN_POINT('Ctrl Pts',(127.388378504628,37.1661344711245,25.0006253155994));
#42729=CARTESIAN_POINT('Ctrl Pts',(127.517304576101,37.3083424273972,24.9890422439931));
#42730=CARTESIAN_POINT('Ctrl Pts',(127.546523102162,37.3393744227889,24.9864947018794));
#42731=CARTESIAN_POINT('Ctrl Pts',(127.59589385837,37.3898666469458,24.9823142908905));
#42732=CARTESIAN_POINT('Ctrl Pts',(127.615715302454,37.4096421895552,24.9806676307273));
#42733=CARTESIAN_POINT('Ctrl Pts',(127.655076205008,37.4479506745823,24.9774581674764));
#42734=CARTESIAN_POINT('Ctrl Pts',(127.674595955637,37.4665008009705,24.9758946841886));
#42735=CARTESIAN_POINT('Ctrl Pts',(127.718082686967,37.5068521989489,24.9724715083904));
#42736=CARTESIAN_POINT('Ctrl Pts',(127.742145505016,37.5285465692299,24.9706163286446));
#42737=CARTESIAN_POINT('Ctrl Pts',(127.8271058803,37.602964438754,24.9641957456165));
#42738=CARTESIAN_POINT('Ctrl Pts',(127.889570604981,37.6538616862496,24.9597028966585));
#42739=CARTESIAN_POINT('Ctrl Pts',(128.177804786523,37.8721001522049,24.9398385771984));
#42740=CARTESIAN_POINT('Ctrl Pts',(128.422018362977,38.0131908377763,24.9253936572409));
#42741=CARTESIAN_POINT('Ctrl Pts',(128.74253862518,38.1486001980156,24.9065604790743));
#42742=CARTESIAN_POINT('Ctrl Pts',(128.805001103423,38.1728329696394,24.9028901796026));
#42743=CARTESIAN_POINT('Ctrl Pts',(128.910884003884,38.2103407931495,24.8966061926021));
#42744=CARTESIAN_POINT('Ctrl Pts',(128.95392840177,38.2246233056361,24.8940346723486));
#42745=CARTESIAN_POINT('Ctrl Pts',(129.016161331327,38.2438956080628,24.8902756327486));
#42746=CARTESIAN_POINT('Ctrl Pts',(129.035129000958,38.2495878440407,24.88912449901));
#42747=CARTESIAN_POINT('Ctrl Pts',(129.068498970997,38.2592843278496,24.8870880405747));
#42748=CARTESIAN_POINT('Ctrl Pts',(129.082879577217,38.2633600192156,24.8862067223702));
#42749=CARTESIAN_POINT('Ctrl Pts',(129.114675297002,38.2721446576098,24.8842495518035));
#42750=CARTESIAN_POINT('Ctrl Pts',(129.132101114727,38.2768097263735,24.8831714325921));
#42751=CARTESIAN_POINT('Ctrl Pts',(129.18302160838,38.2900069988382,24.8800067532311));
#42752=CARTESIAN_POINT('Ctrl Pts',(129.216609628911,38.2981660165721,24.8779013511822));
#42753=CARTESIAN_POINT('Ctrl Pts',(129.434296841521,38.3475326872473,24.8641660483345));
#42754=CARTESIAN_POINT('Ctrl Pts',(129.621427295724,38.3738209592561,24.8519643974789));
#42755=CARTESIAN_POINT('Ctrl Pts',(129.966342192234,38.3932091969743,24.8297023463993));
#42756=CARTESIAN_POINT('Ctrl Pts',(130.123361105058,38.3911341618485,24.8196512098367));
#42757=CARTESIAN_POINT('Ctrl Pts',(130.37471179684,38.3703247082056,24.8039201482275));
#42758=CARTESIAN_POINT('Ctrl Pts',(130.469373115477,38.3584503993726,24.7980754131398));
#42759=CARTESIAN_POINT('Ctrl Pts',(130.600161296829,38.3364052710126,24.7901144095479));
#42760=CARTESIAN_POINT('Ctrl Pts',(130.636803982012,38.329605767872,24.7878963804327));
#42761=CARTESIAN_POINT('Ctrl Pts',(130.699784311125,38.316841216531,24.7841041267788));
#42762=CARTESIAN_POINT('Ctrl Pts',(130.726175947379,38.3111632840996,24.7825211016516));
#42763=CARTESIAN_POINT('Ctrl Pts',(130.780190833074,38.2988655624278,24.7792927435839));
#42764=CARTESIAN_POINT('Ctrl Pts',(130.807804390822,38.2922126104616,24.7776485956208));
#42765=CARTESIAN_POINT('Ctrl Pts',(130.878566618735,38.274219887414,24.7734495688047));
#42766=CARTESIAN_POINT('Ctrl Pts',(130.921581629802,38.2623737883231,24.7709108300149));
#42767=CARTESIAN_POINT('Ctrl Pts',(131.133354568796,38.1995296011032,24.7584622212581));
#42768=CARTESIAN_POINT('Ctrl Pts',(131.298195476021,38.1362684816494,24.7489501108485));
#42769=CARTESIAN_POINT('Ctrl Pts',(131.599920151667,37.9925883482364,24.7311617706115));
#42770=CARTESIAN_POINT('Ctrl Pts',(131.737537901828,37.9148393853149,24.7228771968075));
#42771=CARTESIAN_POINT('Ctrl Pts',(131.928961773157,37.7883037979966,24.7104917956709));
#42772=CARTESIAN_POINT('Ctrl Pts',(131.987422597113,37.7469404722855,24.7065802556947));
#42773=CARTESIAN_POINT('Ctrl Pts',(132.082431684908,37.6750965760221,24.6999291392002));
#42774=CARTESIAN_POINT('Ctrl Pts',(132.119727775011,37.6456411525219,24.6972383960315));
#42775=CARTESIAN_POINT('Ctrl Pts',(132.171946472495,37.6025871892222,24.6933360809495));
#42776=CARTESIAN_POINT('Ctrl Pts',(132.187387391413,37.5896231219281,24.6921648189547));
#42777=CARTESIAN_POINT('Ctrl Pts',(132.213995416233,37.5668754846209,24.6901142944988));
#42778=CARTESIAN_POINT('Ctrl Pts',(132.225215371392,37.5571550594972,24.6892394510666));
#42779=CARTESIAN_POINT('Ctrl Pts',(132.249693458435,37.5356653301166,24.6873079026262));
#42780=CARTESIAN_POINT('Ctrl Pts',(132.262923138087,37.5238657182528,24.6862491201064));
#42781=CARTESIAN_POINT('Ctrl Pts',(132.300576563752,37.4897484064354,24.683194423011));
#42782=CARTESIAN_POINT('Ctrl Pts',(132.324766285672,37.4671767659435,24.6811814997411));
#42783=CARTESIAN_POINT('Ctrl Pts',(132.532109292819,37.2679463388249,24.6635128909466));
#42784=CARTESIAN_POINT('Ctrl Pts',(132.695153236213,37.0715453116095,24.6468253878137));
#42785=CARTESIAN_POINT('Ctrl Pts',(132.922736348147,36.7244721202652,24.6202722312554));
#42786=CARTESIAN_POINT('Ctrl Pts',(133.001146238963,36.584084636616,24.6101776743207));
#42787=CARTESIAN_POINT('Ctrl Pts',(133.090956575874,36.3924772576549,24.5973181859773));
#42788=CARTESIAN_POINT('Ctrl Pts',(133.111555251576,36.3458193810396,24.5942532448596));
#42789=CARTESIAN_POINT('Ctrl Pts',(133.142479748108,36.2712628408236,24.5894576821353));
#42790=CARTESIAN_POINT('Ctrl Pts',(133.153504098035,36.2436640083246,24.5877041399732));
#42791=CARTESIAN_POINT('Ctrl Pts',(133.173690469567,36.191133550113,24.5844062592439));
#42792=CARTESIAN_POINT('Ctrl Pts',(133.182925124096,36.1662324143684,24.5828596258703));
#42793=CARTESIAN_POINT('Ctrl Pts',(133.203376567791,36.1090322236372,24.5793436065871));
#42794=CARTESIAN_POINT('Ctrl Pts',(133.214399340973,36.0766665715583,24.5773806495906));
#42795=CARTESIAN_POINT('Ctrl Pts',(133.247981639246,35.9729441667907,24.5711693902981));
#42796=CARTESIAN_POINT('Ctrl Pts',(133.268669534253,35.9010025931604,24.5669805668041));
#42797=CARTESIAN_POINT('Ctrl Pts',(133.357935429193,35.546823039581,24.5468302647766));
#42798=CARTESIAN_POINT('Ctrl Pts',(133.39242406578,35.257283833085,24.5319176245196));
#42799=CARTESIAN_POINT('Ctrl Pts',(133.388927898805,34.8992632458069,24.5125464010006));
#42800=CARTESIAN_POINT('Ctrl Pts',(133.386243137713,34.8316649530008,24.5088419110364));
#42801=CARTESIAN_POINT('Ctrl Pts',(133.378361933162,34.7186449031059,24.5025056889307));
#42802=CARTESIAN_POINT('Ctrl Pts',(133.374265627533,34.6731650266735,24.4999170401894));
#42803=CARTESIAN_POINT('Ctrl Pts',(133.367071915915,34.6080484395856,24.496137386194));
#42804=CARTESIAN_POINT('Ctrl Pts',(133.364718325639,34.5883328281089,24.4949833183686));
#42805=CARTESIAN_POINT('Ctrl Pts',(133.36028904894,34.5538093163656,24.4929437010232));
#42806=CARTESIAN_POINT('Ctrl Pts',(133.358288384133,34.5389926941861,24.4920622041559));
#42807=CARTESIAN_POINT('Ctrl Pts',(133.353662891379,34.5063662071838,24.490107189215));
#42808=CARTESIAN_POINT('Ctrl Pts',(133.350994216694,34.4885639452007,24.4890314403384));
#42809=CARTESIAN_POINT('Ctrl Pts',(133.342648310382,34.4357619861346,24.485815625139));
#42810=CARTESIAN_POINT('Ctrl Pts',(133.336563743955,34.4008302144195,24.4836553186297));
#42811=CARTESIAN_POINT('Ctrl Pts',(133.297838333236,34.197433709356,24.4709089808406));
#42812=CARTESIAN_POINT('Ctrl Pts',(133.25299285538,34.0315585005043,24.4598527647854));
#42813=CARTESIAN_POINT('Ctrl Pts',(133.140866228321,33.7145042549144,24.4381747162702));
#42814=CARTESIAN_POINT('Ctrl Pts',(133.074692391641,33.5634017689105,24.4275826689688));
#42815=CARTESIAN_POINT('Ctrl Pts',(132.965566413778,33.3566540262536,24.4129593814519));
#42816=CARTESIAN_POINT('Ctrl Pts',(132.931485431608,33.2966021409348,24.4086928614946));
#42817=CARTESIAN_POINT('Ctrl Pts',(132.86723814407,33.1910431817702,24.4011634332219));
#42818=CARTESIAN_POINT('Ctrl Pts',(132.837762450489,33.1451457912991,24.3978789274453));
#42819=CARTESIAN_POINT('Ctrl Pts',(132.79012974431,33.0747707846583,24.3928236838606));
#42820=CARTESIAN_POINT('Ctrl Pts',(132.772729620079,33.0497943528555,24.3910256360486));
#42821=CARTESIAN_POINT('Ctrl Pts',(132.739583274734,33.0035560940002,24.3876884986761));
#42822=CARTESIAN_POINT('Ctrl Pts',(132.723920105334,32.9822378467044,24.3861464515368));
#42823=CARTESIAN_POINT('Ctrl Pts',(132.688128175638,32.9346999204486,24.382698816871));
#42824=CARTESIAN_POINT('Ctrl Pts',(132.667862083083,32.9085867163374,24.3807986967854));
#42825=CARTESIAN_POINT('Ctrl Pts',(132.604581925559,32.8294660892734,24.3750180314103));
#42826=CARTESIAN_POINT('Ctrl Pts',(132.56034486121,32.7774565196872,24.3711854577915));
#42827=CARTESIAN_POINT('Ctrl Pts',(132.346586833336,32.5410003276086,24.3535313387853));
#42828=CARTESIAN_POINT('Ctrl Pts',(132.158535095543,32.3743800774479,24.3404784790741));
#42829=CARTESIAN_POINT('Ctrl Pts',(131.835025983022,32.14619138228,24.3193613756595));
#42830=CARTESIAN_POINT('Ctrl Pts',(131.710958647749,32.0701270076269,24.3115058145515));
#42831=CARTESIAN_POINT('Ctrl Pts',(131.557574337656,31.9891602907802,24.3016262553113));
#42832=CARTESIAN_POINT('Ctrl Pts',(131.532580304157,31.9763612856899,24.3000111829602));
#42833=CARTESIAN_POINT('Ctrl Pts',(131.492673083546,31.9565474187759,24.2974197564617));
#42834=CARTESIAN_POINT('Ctrl Pts',(131.477862251687,31.9493279939051,24.2964552591049));
#42835=CARTESIAN_POINT('Ctrl Pts',(131.449276575382,31.9356511449311,24.2945873789926));
#42836=CARTESIAN_POINT('Ctrl Pts',(131.43550994076,31.9291780132069,24.2936849377532));
#42837=CARTESIAN_POINT('Ctrl Pts',(131.401037847122,31.9132515330251,24.2914187854233));
#42838=CARTESIAN_POINT('Ctrl Pts',(131.380280042599,31.903913746401,24.2900484906706));
#42839=CARTESIAN_POINT('Ctrl Pts',(131.303443130607,31.8702753452325,24.2849595064262));
#42840=CARTESIAN_POINT('Ctrl Pts',(131.246806599505,31.8472848570331,24.2811759951212));
#42841=CARTESIAN_POINT('Ctrl Pts',(131.005583057582,31.7568812676487,24.2650145874468));
#42842=CARTESIAN_POINT('Ctrl Pts',(130.815941005054,31.7040549936868,24.2522197029305));
#42843=CARTESIAN_POINT('Ctrl Pts',(130.436574000226,31.6331470951516,24.2274589048701));
#42844=CARTESIAN_POINT('Ctrl Pts',(130.247740163927,31.6140085097161,24.2155244208395));
#42845=CARTESIAN_POINT('Ctrl Pts',(130.013592473202,31.6099827098066,24.2013666635207));
#42846=CARTESIAN_POINT('Ctrl Pts',(129.968899838689,31.6100980767917,24.1986915279217));
#42847=CARTESIAN_POINT('Ctrl Pts',(129.895810393906,31.6117324266804,24.1943593804851));
#42848=CARTESIAN_POINT('Ctrl Pts',(129.86740838946,31.6127249652942,24.1926864803077));
#42849=CARTESIAN_POINT('Ctrl Pts',(129.812066056633,31.6153561284719,24.1894463349443));
#42850=CARTESIAN_POINT('Ctrl Pts',(129.785126268043,31.616959556081,24.1878781331347));
#42851=CARTESIAN_POINT('Ctrl Pts',(129.721086394716,31.6215392087954,24.1841704405491));
#42852=CARTESIAN_POINT('Ctrl Pts',(129.684010130816,31.6248050908958,24.1820399948799));
#42853=CARTESIAN_POINT('Ctrl Pts',(129.558348289526,31.6379629592714,24.1748674863531));
#42854=CARTESIAN_POINT('Ctrl Pts',(129.470098812605,31.6507380196447,24.1699130175832));
#42855=CARTESIAN_POINT('Ctrl Pts',(129.116410617838,31.7162701641653,24.1502345285996));
#42856=CARTESIAN_POINT('Ctrl Pts',(128.857248031665,31.7972323911606,24.1363057336784));
#42857=CARTESIAN_POINT('Ctrl Pts',(128.550083144372,31.9352765604378,24.1180691868218));
#42858=CARTESIAN_POINT('Ctrl Pts',(128.490503849463,31.9641789997478,24.1144396757732));
#42859=CARTESIAN_POINT('Ctrl Pts',(128.391938584734,32.0156128959156,24.108218092932));
#42860=CARTESIAN_POINT('Ctrl Pts',(128.352484978957,32.0372104769931,24.10566710795));
#42861=CARTESIAN_POINT('Ctrl Pts',(128.296350899884,32.069407142396,24.1019327964897));
#42862=CARTESIAN_POINT('Ctrl Pts',(128.279313635703,32.0793779518064,24.1007851993323));
#42863=CARTESIAN_POINT('Ctrl Pts',(128.249534501907,32.0971567563929,24.0987525342358));
#42864=CARTESIAN_POINT('Ctrl Pts',(128.236755665565,32.1049010791081,24.0978714171118));
#42865=CARTESIAN_POINT('Ctrl Pts',(128.208622571135,32.1222058633255,24.0959115854776));
#42866=CARTESIAN_POINT('Ctrl Pts',(128.19329354969,32.1318047563406,24.0948305600288));
#42867=CARTESIAN_POINT('Ctrl Pts',(128.148705735776,32.1602244980731,24.091649182839));
#42868=CARTESIAN_POINT('Ctrl Pts',(128.119659811271,32.1793731323099,24.0895297033442));
#42869=CARTESIAN_POINT('Ctrl Pts',(127.938698375858,32.302709938872,24.0760511504062));
#42870=CARTESIAN_POINT('Ctrl Pts',(127.795202818095,32.4186829466646,24.06414825003));
#42871=CARTESIAN_POINT('Ctrl Pts',(127.546283476208,32.6558248076775,24.0419901982629));
#42872=CARTESIAN_POINT('Ctrl Pts',(127.438629656662,32.7739560411853,24.0317524860668));
#42873=CARTESIAN_POINT('Ctrl Pts',(127.279997535091,32.9748406075572,24.0157800362342));
#42874=CARTESIAN_POINT('Ctrl Pts',(127.223545612863,33.0529541029085,24.0098736573249));
#42875=CARTESIAN_POINT('Ctrl Pts',(127.149901930039,33.1645860521701,24.0018453776311));
#42876=CARTESIAN_POINT('Ctrl Pts',(127.129827604531,33.1961391526485,23.9996193968764));
#42877=CARTESIAN_POINT('Ctrl Pts',(127.096156545385,33.2510494297626,23.9958179073234));
#42878=CARTESIAN_POINT('Ctrl Pts',(127.082309752074,33.274248399653,23.9942334839521));
#42879=CARTESIAN_POINT('Ctrl Pts',(127.054498206573,33.3221357080055,23.9910060166966));
#42880=CARTESIAN_POINT('Ctrl Pts',(127.040562983593,33.3468387814902,23.9893641100284));
#42881=CARTESIAN_POINT('Ctrl Pts',(127.005606839114,33.4106646518103,23.9851786309603));
#42882=CARTESIAN_POINT('Ctrl Pts',(126.985041410932,33.4500315441084,23.982650989225));
#42883=CARTESIAN_POINT('Ctrl Pts',(126.890677085338,33.6396556115579,23.9707127367289));
#42884=CARTESIAN_POINT('Ctrl Pts',(126.827298718546,33.7948441014666,23.9616564167831));
#42885=CARTESIAN_POINT('Ctrl Pts',(126.716773322046,34.1355760686435,23.9425609732444));
#42886=CARTESIAN_POINT('Ctrl Pts',(126.673334989371,34.3216938884895,23.9325965252199));
#42887=CARTESIAN_POINT('Ctrl Pts',(126.633473070127,34.5948223413107,23.9175604296236));
#42888=CARTESIAN_POINT('Ctrl Pts',(126.62434924651,34.6796060877563,23.9128334293433));
#42889=CARTESIAN_POINT('Ctrl Pts',(126.616713754069,34.7893085292808,23.9065406226926));
#42890=CARTESIAN_POINT('Ctrl Pts',(126.615266654413,34.8139977935598,23.9051128761941));
#42891=CARTESIAN_POINT('Ctrl Pts',(126.613340085274,34.8544391205199,23.9027522086949));
#42892=CARTESIAN_POINT('Ctrl Pts',(126.612700057938,34.8701830829695,23.9018277383581));
#42893=CARTESIAN_POINT('Ctrl Pts',(126.611697666212,34.8999538572098,23.9000683741713));
#42894=CARTESIAN_POINT('Ctrl Pts',(126.611312583221,34.9139795863136,23.8992347927287));
#42895=CARTESIAN_POINT('Ctrl Pts',(126.610508420011,34.9518346299784,23.8969730259222));
#42896=CARTESIAN_POINT('Ctrl Pts',(126.610253568627,34.9756661873626,23.895536357727));
#42897=CARTESIAN_POINT('Ctrl Pts',(126.610238801927,35.0753183644395,23.8894809500956));
#42898=CARTESIAN_POINT('Ctrl Pts',(126.612771473415,35.1511127742874,23.8847595611865));
#42899=CARTESIAN_POINT('Ctrl Pts',(126.627938181166,35.3773337443965,23.8704393478627));
#42900=CARTESIAN_POINT('Ctrl Pts',(126.648078376497,35.5270679312864,23.8606650076194));
#42901=CARTESIAN_POINT('Ctrl Pts',(126.712847935603,35.8458382130121,23.8397261393574));
#42902=CARTESIAN_POINT('Ctrl Pts',(126.760697643102,36.0137635588549,23.828621481531));
#42903=CARTESIAN_POINT('Ctrl Pts',(126.821241887301,36.1772433577858,23.8178898623416));
#42904=CARTESIAN_POINT('',(126.61025139839,34.9970473867279,24.2343657983436));
#42905=CARTESIAN_POINT('Ctrl Pts',(126.821241956411,36.1772435443955,24.1659079080442));
#42906=CARTESIAN_POINT('Ctrl Pts',(126.81168092342,36.151427127163,24.1676083132325));
#42907=CARTESIAN_POINT('Ctrl Pts',(126.80243217331,36.1254882379945,24.1693001454415));
#42908=CARTESIAN_POINT('Ctrl Pts',(126.776459846116,36.0497397820318,24.174192253994));
#42909=CARTESIAN_POINT('Ctrl Pts',(126.760578224573,35.9996558173652,24.1773663332289));
#42910=CARTESIAN_POINT('Ctrl Pts',(126.73662887044,35.9175522658716,24.1824734265101));
#42911=CARTESIAN_POINT('Ctrl Pts',(126.72785381004,35.8857498048348,24.184428534445));
#42912=CARTESIAN_POINT('Ctrl Pts',(126.71288235402,35.828228310642,24.1879244880184));
#42913=CARTESIAN_POINT('Ctrl Pts',(126.706520203129,35.8025555678061,24.1894704820985));
#42914=CARTESIAN_POINT('Ctrl Pts',(126.693473213447,35.7471378305393,24.1927780457357));
#42915=CARTESIAN_POINT('Ctrl Pts',(126.686887822117,35.7173716694405,24.1945363630827));
#42916=CARTESIAN_POINT('Ctrl Pts',(126.674196589676,35.6560993459167,24.198120409506));
#42917=CARTESIAN_POINT('Ctrl Pts',(126.668134808744,35.6245871594675,24.1999446350986));
#42918=CARTESIAN_POINT('Ctrl Pts',(126.650875049431,35.5274458934978,24.2055140255797));
#42919=CARTESIAN_POINT('Ctrl Pts',(126.641161920763,35.4615675591525,24.2092152021343));
#42920=CARTESIAN_POINT('Ctrl Pts',(126.617863520246,35.2632165309681,24.2201815224655));
#42921=CARTESIAN_POINT('Ctrl Pts',(126.610135275629,35.1301874299042,24.2272962254604));
#42922=CARTESIAN_POINT('Ctrl Pts',(126.610251286806,34.9970463750651,24.2343660470093));
#42923=CARTESIAN_POINT('Ctrl Pts',(126.610251285916,34.9970473969534,24.2343659927468));
#42924=CARTESIAN_POINT('Ctrl Pts',(126.610447429808,34.7718635519805,24.2463233086417));
#42925=CARTESIAN_POINT('Ctrl Pts',(126.633081622873,34.5472763101012,24.258087103762));
#42926=CARTESIAN_POINT('Ctrl Pts',(126.683070643506,34.3006529531977,24.2722722320412));
#42927=CARTESIAN_POINT('Ctrl Pts',(126.688636419679,34.2747567277788,24.2737780767598));
#42928=CARTESIAN_POINT('Ctrl Pts',(126.699512643886,34.2268899970247,24.2765962743958));
#42929=CARTESIAN_POINT('Ctrl Pts',(126.704740505068,34.2049021026687,24.2779045359552));
#42930=CARTESIAN_POINT('Ctrl Pts',(126.713883912621,34.1680857684514,24.2801206168535));
#42931=CARTESIAN_POINT('Ctrl Pts',(126.717681038701,34.1532282136674,24.2810219752463));
#42932=CARTESIAN_POINT('Ctrl Pts',(126.725794642887,34.1223557468768,24.282910439008));
#42933=CARTESIAN_POINT('Ctrl Pts',(126.730128017045,34.1063460707788,24.2838983876695));
#42934=CARTESIAN_POINT('Ctrl Pts',(126.742250537134,34.0628282642698,24.2866062056763));
#42935=CARTESIAN_POINT('Ctrl Pts',(126.750270319019,34.0353864460355,24.288338160018));
#42936=CARTESIAN_POINT('Ctrl Pts',(126.807231399905,33.8492564327964,24.3002372164349));
#42937=CARTESIAN_POINT('Ctrl Pts',(126.867425924522,33.6942619355829,24.3108897090073));
#42938=CARTESIAN_POINT('Ctrl Pts',(127.016163420946,33.3814697637651,24.3332060381767));
#42939=CARTESIAN_POINT('Ctrl Pts',(127.106477103547,33.2250476844012,24.3448367477163));
#42940=CARTESIAN_POINT('Ctrl Pts',(127.248450231542,33.0190258451249,24.3604960373607));
#42941=CARTESIAN_POINT('Ctrl Pts',(127.289858387392,32.9627424904563,24.3648156908691));
#42942=CARTESIAN_POINT('Ctrl Pts',(127.366940528956,32.8644835421773,24.372427768452));
#42943=CARTESIAN_POINT('Ctrl Pts',(127.401953026644,32.8220226875458,24.3757425007528));
#42944=CARTESIAN_POINT('Ctrl Pts',(127.457979813729,32.7573518180865,24.3808333863997));
#42945=CARTESIAN_POINT('Ctrl Pts',(127.478285687131,32.7345432003817,24.3826374785126));
#42946=CARTESIAN_POINT('Ctrl Pts',(127.516745830408,32.6925006985616,24.3859802204642));
#42947=CARTESIAN_POINT('Ctrl Pts',(127.534822209134,32.673199016931,24.3875219154788));
#42948=CARTESIAN_POINT('Ctrl Pts',(127.575903451376,32.6303492816788,24.3909616223566));
#42949=CARTESIAN_POINT('Ctrl Pts',(127.599029364226,32.6069206617977,24.3928542809879));
#42950=CARTESIAN_POINT('Ctrl Pts',(127.670611620867,32.5364838035046,24.3985853569239));
#42951=CARTESIAN_POINT('Ctrl Pts',(127.720135416407,32.4905816229533,24.4023770449682));
#42952=CARTESIAN_POINT('Ctrl Pts',(127.997305819603,32.2486637775179,24.4227624606193));
#42953=CARTESIAN_POINT('Ctrl Pts',(128.248842370753,32.0821117198644,24.4381693914244));
#42954=CARTESIAN_POINT('Ctrl Pts',(128.58044252669,31.9210515451339,24.4581065741255));
#42955=CARTESIAN_POINT('Ctrl Pts',(128.642744017878,31.8930847670628,24.4618445005339));
#42956=CARTESIAN_POINT('Ctrl Pts',(128.748327533255,31.8494708530255,24.4682317414877));
#42957=CARTESIAN_POINT('Ctrl Pts',(128.791161440821,31.8327888003664,24.4708370675807));
#42958=CARTESIAN_POINT('Ctrl Pts',(128.853011371577,31.8101381829686,24.4746367848401));
#42959=CARTESIAN_POINT('Ctrl Pts',(128.871763127689,31.8034576737053,24.475793697469));
#42960=CARTESIAN_POINT('Ctrl Pts',(128.90470436756,31.7920479710327,24.4778363896447));
#42961=CARTESIAN_POINT('Ctrl Pts',(128.918868015395,31.7872469184201,24.4787180718346));
#42962=CARTESIAN_POINT('Ctrl Pts',(128.950115208986,31.7768850897746,24.4806710483873));
#42963=CARTESIAN_POINT('Ctrl Pts',(128.967211247072,31.7713663634649,24.4817445391054));
#42964=CARTESIAN_POINT('Ctrl Pts',(129.018001302014,31.7554156315153,24.4849467582556));
#42965=CARTESIAN_POINT('Ctrl Pts',(129.051814192271,31.7453736573283,24.4870954841807));
#42966=CARTESIAN_POINT('Ctrl Pts',(129.261689925548,31.6865914069688,24.5005106610348));
#42967=CARTESIAN_POINT('Ctrl Pts',(129.441285970382,31.651626172727,24.5123110674619));
#42968=CARTESIAN_POINT('Ctrl Pts',(129.78239976852,31.613431849617,24.5344343467374));
#42969=CARTESIAN_POINT('Ctrl Pts',(129.943070853665,31.6069246258301,24.5447373374876));
#42970=CARTESIAN_POINT('Ctrl Pts',(130.200226190926,31.6147882949694,24.5607939471277));
#42971=CARTESIAN_POINT('Ctrl Pts',(130.296679788106,31.6218743863781,24.5667216304026));
#42972=CARTESIAN_POINT('Ctrl Pts',(130.429892341415,31.6374118203363,24.5747731379311));
#42973=CARTESIAN_POINT('Ctrl Pts',(130.467005237902,31.6423649740295,24.5770018493834));
#42974=CARTESIAN_POINT('Ctrl Pts',(130.530752354692,31.6519502317445,24.5808065160665));
#42975=CARTESIAN_POINT('Ctrl Pts',(130.557426643587,31.6562878543893,24.5823914250385));
#42976=CARTESIAN_POINT('Ctrl Pts',(130.611969832366,31.6658282082056,24.5856186092044));
#42977=CARTESIAN_POINT('Ctrl Pts',(130.639831091482,31.6710625031052,24.5872597634095));
#42978=CARTESIAN_POINT('Ctrl Pts',(130.71109690653,31.6853789944296,24.5914406746976));
#42979=CARTESIAN_POINT('Ctrl Pts',(130.754395544021,31.694964623461,24.5939645715964));
#42980=CARTESIAN_POINT('Ctrl Pts',(130.957874859001,31.7442190484277,24.6057654217752));
#42981=CARTESIAN_POINT('Ctrl Pts',(131.115213722613,31.7947012189676,24.6146992424365));
#42982=CARTESIAN_POINT('Ctrl Pts',(131.447080315978,31.9285925129293,24.6337843744378));
#42983=CARTESIAN_POINT('Ctrl Pts',(131.619406117166,32.015858205226,24.6438502027838));
#42984=CARTESIAN_POINT('Ctrl Pts',(131.856220968248,32.1623623893905,24.659016375288));
#42985=CARTESIAN_POINT('Ctrl Pts',(131.927331681797,32.2101731566946,24.6637654562619));
#42986=CARTESIAN_POINT('Ctrl Pts',(132.016565812746,32.2752099431086,24.6700837818974));
#42987=CARTESIAN_POINT('Ctrl Pts',(132.036420849003,32.2900168671208,24.6715135810462));
#42988=CARTESIAN_POINT('Ctrl Pts',(132.068644763198,32.3146019967338,24.6738767655178));
#42989=CARTESIAN_POINT('Ctrl Pts',(132.08111121167,32.3242515629454,24.6748016648582));
#42990=CARTESIAN_POINT('Ctrl Pts',(132.104540416444,32.3426495515891,24.6765610933071));
#42991=CARTESIAN_POINT('Ctrl Pts',(132.115517084681,32.3513797518478,24.6773943015001));
#42992=CARTESIAN_POINT('Ctrl Pts',(132.144974007505,32.3751079964873,24.6796537077394));
#42993=CARTESIAN_POINT('Ctrl Pts',(132.163350650214,32.3902326890632,24.681088358577));
#42994=CARTESIAN_POINT('Ctrl Pts',(132.234507324077,32.4500653799052,24.6867373980346));
#42995=CARTESIAN_POINT('Ctrl Pts',(132.286070274267,32.4961887161915,24.6910355061395));
#42996=CARTESIAN_POINT('Ctrl Pts',(132.4904374177,32.6905740973933,24.7088047143256));
#42997=CARTESIAN_POINT('Ctrl Pts',(132.630525463145,32.8514975107663,24.7227046782548));
#42998=CARTESIAN_POINT('Ctrl Pts',(132.818794666682,33.1140156765076,24.7433331048796));
#42999=CARTESIAN_POINT('Ctrl Pts',(132.878596442633,33.2066160340188,24.7502809841382));
#43000=CARTESIAN_POINT('Ctrl Pts',(132.971992707294,33.3679823369029,24.7617983077101));
#43001=CARTESIAN_POINT('Ctrl Pts',(133.007962346652,33.4352680080159,24.766439260946));
#43002=CARTESIAN_POINT('Ctrl Pts',(133.056829933331,33.5346055044568,24.7730623541747));
#43003=CARTESIAN_POINT('Ctrl Pts',(133.071555357095,33.5657273312423,24.775105914292));
#43004=CARTESIAN_POINT('Ctrl Pts',(133.096806917742,33.6212691781546,24.7786989589256));
#43005=CARTESIAN_POINT('Ctrl Pts',(133.107524465589,33.645598464111,24.7802548025497));
#43006=CARTESIAN_POINT('Ctrl Pts',(133.129562955564,33.6972659053719,24.7835220116048));
#43007=CARTESIAN_POINT('Ctrl Pts',(133.140814443324,33.7246313760677,24.7852309571184));
#43008=CARTESIAN_POINT('Ctrl Pts',(133.170244114801,33.7989616552292,24.789817301271));
#43009=CARTESIAN_POINT('Ctrl Pts',(133.187736762664,33.8461908507874,24.792672163936));
#43010=CARTESIAN_POINT('Ctrl Pts',(133.288335586404,34.1375795050371,24.8099602120246));
#43011=CARTESIAN_POINT('Ctrl Pts',(133.344404117157,34.3901704856982,24.8234804305214));
#43012=CARTESIAN_POINT('Ctrl Pts',(133.383190034256,34.7602679168404,24.8432575552909));
#43013=CARTESIAN_POINT('Ctrl Pts',(133.389345019598,34.8743668732681,24.8493643286174));
#43014=CARTESIAN_POINT('Ctrl Pts',(133.389948807836,35.053139882388,24.8592205563777));
#43015=CARTESIAN_POINT('Ctrl Pts',(133.388320874856,35.1177172293669,24.8628401733385));
#43016=CARTESIAN_POINT('Ctrl Pts',(133.383636288177,35.2047438232886,24.8678440567895));
#43017=CARTESIAN_POINT('Ctrl Pts',(133.382197932421,35.2272699951454,24.8691507022791));
#43018=CARTESIAN_POINT('Ctrl Pts',(133.379405152333,35.2650676990335,24.8713648595265));
#43019=CARTESIAN_POINT('Ctrl Pts',(133.378171860723,35.2803478939223,24.8722659364183));
#43020=CARTESIAN_POINT('Ctrl Pts',(133.375387592872,35.3121523688025,24.8741547593598));
#43021=CARTESIAN_POINT('Ctrl Pts',(133.373818855669,35.328674317659,24.8751433601113));
#43022=CARTESIAN_POINT('Ctrl Pts',(133.369212581616,35.3736734011228,24.8778548276226));
#43023=CARTESIAN_POINT('Ctrl Pts',(133.365935442272,35.4021240002849,24.8795898314739));
#43024=CARTESIAN_POINT('Ctrl Pts',(133.341072275835,35.59629781435,24.8915573087641));
#43025=CARTESIAN_POINT('Ctrl Pts',(133.307617858633,35.7602559971378,24.9022809968109));
#43026=CARTESIAN_POINT('Ctrl Pts',(133.225151470969,36.0523352079134,24.9218370378831));
#43027=CARTESIAN_POINT('Ctrl Pts',(133.180195955434,36.1812569971406,24.9306394596573));
#43028=CARTESIAN_POINT('Ctrl Pts',(133.074427855882,36.434331530677,24.9480273139767));
#43029=CARTESIAN_POINT('Ctrl Pts',(133.013547358119,36.5581891518807,24.9565929592968));
#43030=CARTESIAN_POINT('Ctrl Pts',(132.924612389499,36.714290312089,24.9674255855323));
#43031=CARTESIAN_POINT('Ctrl Pts',(132.90327116899,36.7501901770647,24.969920237475));
#43032=CARTESIAN_POINT('Ctrl Pts',(132.866612505062,36.8093402465385,24.9740378686356));
#43033=CARTESIAN_POINT('Ctrl Pts',(132.851662718574,36.8328118262213,24.9756737981008));
#43034=CARTESIAN_POINT('Ctrl Pts',(132.821613487206,36.8787320502932,24.9788793047147));
#43035=CARTESIAN_POINT('Ctrl Pts',(132.806530999555,36.9011892589982,24.9804493412534));
#43036=CARTESIAN_POINT('Ctrl Pts',(132.772511337284,36.9505559401192,24.9839073559653));
#43037=CARTESIAN_POINT('Ctrl Pts',(132.753447802503,36.9773752544277,24.9857904655089));
#43038=CARTESIAN_POINT('Ctrl Pts',(132.684941748547,37.0708400197813,24.9923738442464));
#43039=CARTESIAN_POINT('Ctrl Pts',(132.633443984725,37.1359458861149,24.9969967699041));
#43040=CARTESIAN_POINT('Ctrl Pts',(132.399556463027,37.4103024955336,25.0167766399029));
#43041=CARTESIAN_POINT('Ctrl Pts',(132.194265716785,37.5985799501043,25.0310506831749));
#43042=CARTESIAN_POINT('Ctrl Pts',(131.913997413708,37.7984768509725,25.0496866726311));
#43043=CARTESIAN_POINT('Ctrl Pts',(131.858534996384,37.835613788992,25.0533438338818));
#43044=CARTESIAN_POINT('Ctrl Pts',(131.763706638497,37.8951320644387,25.0596077317867));
#43045=CARTESIAN_POINT('Ctrl Pts',(131.724922074287,37.918406107543,25.0621726507204));
#43046=CARTESIAN_POINT('Ctrl Pts',(131.668521724666,37.950734094796,25.0659237444595));
#43047=CARTESIAN_POINT('Ctrl Pts',(131.651272630055,37.9604214402965,25.0670737452924));
#43048=CARTESIAN_POINT('Ctrl Pts',(131.620844925697,37.977161429794,25.0691089889572));
#43049=CARTESIAN_POINT('Ctrl Pts',(131.607702929539,37.9842787622033,25.0699902431549));
#43050=CARTESIAN_POINT('Ctrl Pts',(131.578581429694,37.9998019438753,25.071948266341));
#43051=CARTESIAN_POINT('Ctrl Pts',(131.562581772992,38.0081670836478,25.0730273162781));
#43052=CARTESIAN_POINT('Ctrl Pts',(131.515695209553,38.0322059215152,25.0761973307467));
#43053=CARTESIAN_POINT('Ctrl Pts',(131.484634832915,38.0475340739827,25.0783072282422));
#43054=CARTESIAN_POINT('Ctrl Pts',(131.284116212006,38.1426962452932,25.0919658861486));
#43055=CARTESIAN_POINT('Ctrl Pts',(131.108532214178,38.2088378816644,25.1040779219534));
#43056=CARTESIAN_POINT('Ctrl Pts',(130.776768232748,38.3033154241358,25.1263084250582));
#43057=CARTESIAN_POINT('Ctrl Pts',(130.62229795282,38.335867860018,25.1364150119625));
#43058=CARTESIAN_POINT('Ctrl Pts',(130.371375341455,38.370702226433,25.1522179494702));
#43059=CARTESIAN_POINT('Ctrl Pts',(130.276118010768,38.3798394411623,25.1580811255089));
#43060=CARTESIAN_POINT('Ctrl Pts',(130.143343824484,38.3869232590374,25.1660622703433));
#43061=CARTESIAN_POINT('Ctrl Pts',(130.106061964611,38.3882956838372,25.1682826909218));
#43062=CARTESIAN_POINT('Ctrl Pts',(130.041768923691,38.3896001899669,25.1720777242948));
#43063=CARTESIAN_POINT('Ctrl Pts',(130.014767816664,38.3898253738495,25.1736611718897));
#43064=CARTESIAN_POINT('Ctrl Pts',(129.959376883647,38.3896254652524,25.1768892647164));
#43065=CARTESIAN_POINT('Ctrl Pts',(129.930989268454,38.3891663609864,25.1785327393529));
#43066=CARTESIAN_POINT('Ctrl Pts',(129.858078550014,38.387070720279,25.1827276839961));
#43067=CARTESIAN_POINT('Ctrl Pts',(129.813575176762,38.3849129688725,25.1852630772148));
#43068=CARTESIAN_POINT('Ctrl Pts',(129.596160792958,38.3700705132298,25.1975443971339));
#43069=CARTESIAN_POINT('Ctrl Pts',(129.424348479733,38.3450105578429,25.2069071459543));
#43070=CARTESIAN_POINT('Ctrl Pts',(129.098003392692,38.2715086729099,25.2247214112106));
#43071=CARTESIAN_POINT('Ctrl Pts',(128.94354396535,38.2249441057969,25.2331719602147));
#43072=CARTESIAN_POINT('Ctrl Pts',(128.726198435116,38.1421239681673,25.2457269512349));
#43073=CARTESIAN_POINT('Ctrl Pts',(128.660234936429,38.1145693093006,25.2496318737395));
#43074=CARTESIAN_POINT('Ctrl Pts',(128.55199965517,38.0652818529753,25.2562729645903));
#43075=CARTESIAN_POINT('Ctrl Pts',(128.509224142083,38.0447076566642,25.2589604887549));
#43076=CARTESIAN_POINT('Ctrl Pts',(128.448923614584,38.0141289324193,25.2628589435286));
#43077=CARTESIAN_POINT('Ctrl Pts',(128.431032401559,38.0048547064027,25.2640296727719));
#43078=CARTESIAN_POINT('Ctrl Pts',(128.399989746438,37.9884103790362,25.2660874213966));
#43079=CARTESIAN_POINT('Ctrl Pts',(128.386801440671,37.9813117588307,25.2669701264422));
#43080=CARTESIAN_POINT('Ctrl Pts',(128.35804723808,37.9655881109694,25.2689137524011));
#43081=CARTESIAN_POINT('Ctrl Pts',(128.342502171476,37.9569279047334,25.2699767081016));
#43082=CARTESIAN_POINT('Ctrl Pts',(128.297976550915,37.9316611133745,25.2730549741757));
#43083=CARTESIAN_POINT('Ctrl Pts',(128.269173098016,37.9147484899942,25.2750876788226));
#43084=CARTESIAN_POINT('Ctrl Pts',(128.02455975007,37.7662137832415,25.2926776380643));
#43085=CARTESIAN_POINT('Ctrl Pts',(127.823857573102,37.6112640181542,25.309249756168));
#43086=CARTESIAN_POINT('Ctrl Pts',(127.558342291236,37.3542200632127,25.3328981072242));
#43087=CARTESIAN_POINT('Ctrl Pts',(127.478681851734,37.2687007430472,25.3402833524193));
#43088=CARTESIAN_POINT('Ctrl Pts',(127.352596733101,37.1184788012222,25.3524186677325));
#43089=CARTESIAN_POINT('Ctrl Pts',(127.303749046362,37.0559496179156,25.3572510919676));
#43090=CARTESIAN_POINT('Ctrl Pts',(127.236618535366,36.9635038497255,25.3640902051661));
#43091=CARTESIAN_POINT('Ctrl Pts',(127.216537287754,36.9349315112926,25.3661640994209));
#43092=CARTESIAN_POINT('Ctrl Pts',(127.181918583736,36.8840201973484,25.3697911851142));
#43093=CARTESIAN_POINT('Ctrl Pts',(127.16719660003,36.8618109275741,25.3713511534022));
#43094=CARTESIAN_POINT('Ctrl Pts',(127.136819849693,36.8147906109674,25.3746083817646));
#43095=CARTESIAN_POINT('Ctrl Pts',(127.121222169293,36.7899451987181,25.3763034682859));
#43096=CARTESIAN_POINT('Ctrl Pts',(127.080368322498,36.7229537876915,25.3808071650417));
#43097=CARTESIAN_POINT('Ctrl Pts',(127.055702169725,36.6804551515435,25.38359467332));
#43098=CARTESIAN_POINT('Ctrl Pts',(126.950289583187,36.489383015487,25.3958449719673));
#43099=CARTESIAN_POINT('Ctrl Pts',(126.879871236484,36.3355525918427,25.404949309684));
#43100=CARTESIAN_POINT('Ctrl Pts',(126.821241938915,36.1772434971515,25.4139333020124));
#43101=CARTESIAN_POINT('Origin',(130.,35.,23.));
#43102=CARTESIAN_POINT('',(126.821241918426,36.1772434418289,26.660716603687));
#43103=CARTESIAN_POINT('',(126.821241849252,36.1772432550457,26.31957821124));
#43104=CARTESIAN_POINT('',(126.821241918358,36.1772434416438,23.));
#43105=CARTESIAN_POINT('',(126.610251050396,35.0026685497381,25.1397300250475));
#43106=CARTESIAN_POINT('Ctrl Pts',(126.821241849252,36.1772432550457,26.31957821124));
#43107=CARTESIAN_POINT('Ctrl Pts',(126.87264245335,36.3160336779512,26.3116710105479));
#43108=CARTESIAN_POINT('Ctrl Pts',(126.933098780024,36.4513660671469,26.3038949611646));
#43109=CARTESIAN_POINT('Ctrl Pts',(127.064471806615,36.7002495766796,26.2888430195471));
#43110=CARTESIAN_POINT('Ctrl Pts',(127.133591949016,36.8143517529012,26.2816081672139));
#43111=CARTESIAN_POINT('Ctrl Pts',(127.225173264532,36.9471850152158,26.2724176359797));
#43112=CARTESIAN_POINT('Ctrl Pts',(127.241391176002,36.9700939427004,26.2708032366146));
#43113=CARTESIAN_POINT('Ctrl Pts',(127.267576166349,37.0061247360562,26.2682126403952));
#43114=CARTESIAN_POINT('Ctrl Pts',(127.27735800387,37.0193803503733,26.267248287326));
#43115=CARTESIAN_POINT('Ctrl Pts',(127.296466527679,37.0448835682806,26.2653698664562));
#43116=CARTESIAN_POINT('Ctrl Pts',(127.305780647298,37.0571397836088,26.2644566006722));
#43117=CARTESIAN_POINT('Ctrl Pts',(127.329169140659,37.0874848214385,26.2621698788389));
#43118=CARTESIAN_POINT('Ctrl Pts',(127.343343989076,37.1054949858957,26.2607898080824));
#43119=CARTESIAN_POINT('Ctrl Pts',(127.399974450612,37.1759657061189,26.2553034920362));
#43120=CARTESIAN_POINT('Ctrl Pts',(127.443807805546,37.2272942873035,26.2511163237943));
#43121=CARTESIAN_POINT('Ctrl Pts',(127.571667889857,37.3682691100777,26.2391429553349));
#43122=CARTESIAN_POINT('Ctrl Pts',(127.659076980421,37.4547041023452,26.2312337022798));
#43123=CARTESIAN_POINT('Ctrl Pts',(127.932364382142,37.697046514249,26.207689429004));
#43124=CARTESIAN_POINT('Ctrl Pts',(128.130508809315,37.8379946657421,26.1921535343798));
#43125=CARTESIAN_POINT('Ctrl Pts',(128.386902116052,37.9817726221802,26.17427543981));
#43126=CARTESIAN_POINT('Ctrl Pts',(128.432351729646,38.0059161811603,26.1711804082734));
#43127=CARTESIAN_POINT('Ctrl Pts',(128.505227450478,38.0425262169856,26.1663317351438));
#43128=CARTESIAN_POINT('Ctrl Pts',(128.532298880287,38.0556773825983,26.1645548646702));
#43129=CARTESIAN_POINT('Ctrl Pts',(128.581126138749,38.0785987951777,26.1613922612648));
#43130=CARTESIAN_POINT('Ctrl Pts',(128.602816443469,38.0885031533155,26.1600020477003));
#43131=CARTESIAN_POINT('Ctrl Pts',(128.654075073801,38.1112586612751,26.1567501975345));
#43132=CARTESIAN_POINT('Ctrl Pts',(128.683726081199,38.1239186029037,26.1548950665848));
#43133=CARTESIAN_POINT('Ctrl Pts',(128.772584280695,38.1603681150139,26.1494088484061));
#43134=CARTESIAN_POINT('Ctrl Pts',(128.832288854038,38.1829117749427,26.1458186016252));
#43135=CARTESIAN_POINT('Ctrl Pts',(129.048071606726,38.2574987101007,26.1331377740165));
#43136=CARTESIAN_POINT('Ctrl Pts',(129.207260332334,38.2998538543804,26.124337407227));
#43137=CARTESIAN_POINT('Ctrl Pts',(129.576723672592,38.3698638535487,26.1043741331663));
#43138=CARTESIAN_POINT('Ctrl Pts',(129.787753451535,38.3897019476663,26.0933033377676));
#43139=CARTESIAN_POINT('Ctrl Pts',(130.043946239876,38.389760054611,26.0789633544154));
#43140=CARTESIAN_POINT('Ctrl Pts',(130.088654952422,38.3888854223028,26.0764267098409));
#43141=CARTESIAN_POINT('Ctrl Pts',(130.152803922758,38.3863602592305,26.072721704868));
#43142=CARTESIAN_POINT('Ctrl Pts',(130.17226935427,38.3854258335599,26.071588795585));
#43143=CARTESIAN_POINT('Ctrl Pts',(130.206650590422,38.3834781039575,26.0695707861939));
#43144=CARTESIAN_POINT('Ctrl Pts',(130.221569413043,38.3825338919106,26.0686893954738));
#43145=CARTESIAN_POINT('Ctrl Pts',(130.254461787232,38.3802335889637,26.0667331211767));
#43146=CARTESIAN_POINT('Ctrl Pts',(130.272430842172,38.3788328341725,26.0656559857006));
#43147=CARTESIAN_POINT('Ctrl Pts',(130.325827559845,38.3742416559427,26.0624318107928));
#43148=CARTESIAN_POINT('Ctrl Pts',(130.361216056157,38.370636897761,26.0602643813034));
#43149=CARTESIAN_POINT('Ctrl Pts',(130.537586020666,38.349862148799,26.0493305542498));
#43150=CARTESIAN_POINT('Ctrl Pts',(130.677438050956,38.3244016636897,26.0402448634844));
#43151=CARTESIAN_POINT('Ctrl Pts',(131.08246708357,38.2240422492453,26.0133805593485));
#43152=CARTESIAN_POINT('Ctrl Pts',(131.34065662137,38.1255196558237,25.9956390174097));
#43153=CARTESIAN_POINT('Ctrl Pts',(131.626504695175,37.9744221904537,25.9760379551903));
#43154=CARTESIAN_POINT('Ctrl Pts',(131.668423574384,37.951113013679,25.9731609197076));
#43155=CARTESIAN_POINT('Ctrl Pts',(131.734954666002,37.9122471864839,25.9685885124051));
#43156=CARTESIAN_POINT('Ctrl Pts',(131.759884553984,37.897250041651,25.9668737298206));
#43157=CARTESIAN_POINT('Ctrl Pts',(131.807330599159,37.8678693813019,25.9636063651761));
#43158=CARTESIAN_POINT('Ctrl Pts',(131.829875725273,37.8535370284893,25.962052101296));
#43159=CARTESIAN_POINT('Ctrl Pts',(131.881932201038,37.8195730820643,25.9584580536347));
#43160=CARTESIAN_POINT('Ctrl Pts',(131.91131004776,37.7997419899689,25.9564257681728));
#43161=CARTESIAN_POINT('Ctrl Pts',(132.008143089599,37.7321415902902,25.9497080831998));
#43162=CARTESIAN_POINT('Ctrl Pts',(132.074163993074,37.6823649142129,25.9450973998106));
#43163=CARTESIAN_POINT('Ctrl Pts',(132.234788411982,37.551781361527,25.9337265155938));
#43164=CARTESIAN_POINT('Ctrl Pts',(132.326888494108,37.468088325903,25.9270663574183));
#43165=CARTESIAN_POINT('Ctrl Pts',(132.54821820058,37.2435342966165,25.9103062668759));
#43166=CARTESIAN_POINT('Ctrl Pts',(132.670513129399,37.0964761975298,25.9003133042839));
#43167=CARTESIAN_POINT('Ctrl Pts',(132.818732974382,36.8840872040139,25.8860769683793));
#43168=CARTESIAN_POINT('Ctrl Pts',(132.856002022722,36.8270991760439,25.8822723042224));
#43169=CARTESIAN_POINT('Ctrl Pts',(132.903879701195,36.7488418879926,25.8770140992347));
#43170=CARTESIAN_POINT('Ctrl Pts',(132.916019656605,36.728523810385,25.8756459362484));
#43171=CARTESIAN_POINT('Ctrl Pts',(132.93500069655,36.6959870315647,25.8734476026125));
#43172=CARTESIAN_POINT('Ctrl Pts',(132.94198077563,36.6838498152629,25.8726259399405));
#43173=CARTESIAN_POINT('Ctrl Pts',(132.956675522467,36.657927758442,25.8708668952331));
#43174=CARTESIAN_POINT('Ctrl Pts',(132.964369373089,36.6441316226644,25.8699282004673));
#43175=CARTESIAN_POINT('Ctrl Pts',(132.983950690853,36.6084353461604,25.8674939828363));
#43176=CARTESIAN_POINT('Ctrl Pts',(132.995693410953,36.5864573414299,25.8659900298847));
#43177=CARTESIAN_POINT('Ctrl Pts',(133.047525731707,36.4868188324965,25.8591551186033));
#43178=CARTESIAN_POINT('Ctrl Pts',(133.084842396766,36.4077600312121,25.8536873818405));
#43179=CARTESIAN_POINT('Ctrl Pts',(133.198004361153,36.1418484801708,25.8353488398284));
#43180=CARTESIAN_POINT('Ctrl Pts',(133.260242317555,35.9496697544995,25.8222045439304));
#43181=CARTESIAN_POINT('Ctrl Pts',(133.339466945969,35.6019848610798,25.7994791137931));
#43182=CARTESIAN_POINT('Ctrl Pts',(133.363499014095,35.4486758660495,25.7897966691731));
#43183=CARTESIAN_POINT('Ctrl Pts',(133.38076981964,35.2504630202239,25.7777759482062));
#43184=CARTESIAN_POINT('Ctrl Pts',(133.383732882833,35.2066115861234,25.7751465260161));
#43185=CARTESIAN_POINT('Ctrl Pts',(133.387199324183,35.134479668877,25.7708687715386));
#43186=CARTESIAN_POINT('Ctrl Pts',(133.388202975418,35.1062295286911,25.7692053134859));
#43187=CARTESIAN_POINT('Ctrl Pts',(133.389475774857,35.0509087774348,25.7659701546745));
#43188=CARTESIAN_POINT('Ctrl Pts',(133.389774240179,35.0238410326868,25.7643976741705));
#43189=CARTESIAN_POINT('Ctrl Pts',(133.389712560619,34.9590702896442,25.7606584272523));
#43190=CARTESIAN_POINT('Ctrl Pts',(133.389047667075,34.9213707692248,25.758501137612));
#43191=CARTESIAN_POINT('Ctrl Pts',(133.384367769555,34.785060766706,25.7507627341517));
#43192=CARTESIAN_POINT('Ctrl Pts',(133.376676014068,34.6866223889589,25.7452929607711));
#43193=CARTESIAN_POINT('Ctrl Pts',(133.344483636244,34.4232978212859,25.7308350784544));
#43194=CARTESIAN_POINT('Ctrl Pts',(133.312105683326,34.2596519708269,25.7220438641197));
#43195=CARTESIAN_POINT('Ctrl Pts',(133.221735544961,33.9318720038138,25.70400576397));
#43196=CARTESIAN_POINT('Ctrl Pts',(133.162888210715,33.768495518124,25.6947779792037));
#43197=CARTESIAN_POINT('Ctrl Pts',(133.077193733931,33.5778343586207,25.6829752559101));
#43198=CARTESIAN_POINT('Ctrl Pts',(133.062064917946,33.5455466266999,25.6809386802711));
#43199=CARTESIAN_POINT('Ctrl Pts',(133.038519091335,33.4972916953319,25.6778288643346));
#43200=CARTESIAN_POINT('Ctrl Pts',(133.030478800909,33.4811422967099,25.6767767829516));
#43201=CARTESIAN_POINT('Ctrl Pts',(133.015541542629,33.4517307391704,25.674838548748));
#43202=CARTESIAN_POINT('Ctrl Pts',(133.008685216209,33.4384489305471,25.6739548057915));
#43203=CARTESIAN_POINT('Ctrl Pts',(132.992541568739,33.4076771178906,25.6718877323408));
#43204=CARTESIAN_POINT('Ctrl Pts',(132.983188613403,33.3902227307331,25.6707005355786));
#43205=CARTESIAN_POINT('Ctrl Pts',(132.951917647127,33.3330736923022,25.6667672911804));
#43206=CARTESIAN_POINT('Ctrl Pts',(132.929356903163,33.2937383487556,25.6639862159263));
#43207=CARTESIAN_POINT('Ctrl Pts',(132.871535182112,33.197452829823,25.6570153590091));
#43208=CARTESIAN_POINT('Ctrl Pts',(132.835362746079,33.1410734830857,25.6527882195708));
#43209=CARTESIAN_POINT('Ctrl Pts',(132.639006079875,32.8541032393692,25.6306365285972));
#43210=CARTESIAN_POINT('Ctrl Pts',(132.452264181817,32.6429546375871,25.6122624390381));
#43211=CARTESIAN_POINT('Ctrl Pts',(132.181292258157,32.4040731323764,25.589875439973));
#43212=CARTESIAN_POINT('Ctrl Pts',(132.119091277369,32.353053460872,25.5849683325483));
#43213=CARTESIAN_POINT('Ctrl Pts',(132.029276026751,32.2845809144214,25.578198178467));
#43214=CARTESIAN_POINT('Ctrl Pts',(132.003138992895,32.2652429196206,25.5762635710107));
#43215=CARTESIAN_POINT('Ctrl Pts',(131.954830320327,32.2305650364201,25.5727512295535));
#43216=CARTESIAN_POINT('Ctrl Pts',(131.932746386482,32.2151080690904,25.5711691474748));
#43217=CARTESIAN_POINT('Ctrl Pts',(131.887386013099,32.1841589696634,25.5679661862652));
#43218=CARTESIAN_POINT('Ctrl Pts',(131.864097545566,32.1686880992406,25.5663461775516));
#43219=CARTESIAN_POINT('Ctrl Pts',(131.805001488225,32.1304749837513,25.5622945397053));
#43220=CARTESIAN_POINT('Ctrl Pts',(131.768952950445,32.1081130942001,25.5598768199138));
#43221=CARTESIAN_POINT('Ctrl Pts',(131.606607890169,32.0115779258518,25.5492113476853));
#43222=CARTESIAN_POINT('Ctrl Pts',(131.475997249499,31.9449560043203,25.5412291398559));
#43223=CARTESIAN_POINT('Ctrl Pts',(131.22132791832,31.8352126308915,25.5263711250156));
#43224=CARTESIAN_POINT('Ctrl Pts',(131.098283021394,31.7904368309098,25.5194787483502));
#43225=CARTESIAN_POINT('Ctrl Pts',(130.828997171191,31.7097485671671,25.5045305015377));
#43226=CARTESIAN_POINT('Ctrl Pts',(130.68233902518,31.6762377148937,25.4964703057189));
#43227=CARTESIAN_POINT('Ctrl Pts',(130.498456122186,31.6469060568909,25.4859596860316));
#43228=CARTESIAN_POINT('Ctrl Pts',(130.462868124912,31.6418084658141,25.4839067701749));
#43229=CARTESIAN_POINT('Ctrl Pts',(130.409253524055,31.634997153606,25.4807769658108));
#43230=CARTESIAN_POINT('Ctrl Pts',(130.391282202642,31.6328601441163,25.479721644142));
#43231=CARTESIAN_POINT('Ctrl Pts',(130.358443858445,31.6292217027729,25.4777805449679));
#43232=CARTESIAN_POINT('Ctrl Pts',(130.343582797286,31.6276745168874,25.4768972316233));
#43233=CARTESIAN_POINT('Ctrl Pts',(130.309079654235,31.6243128229454,25.4748352944844));
#43234=CARTESIAN_POINT('Ctrl Pts',(130.289431510769,31.6225714649622,25.4736528728346));
#43235=CARTESIAN_POINT('Ctrl Pts',(130.22502662722,31.6174295582927,25.4697525053143));
#43236=CARTESIAN_POINT('Ctrl Pts',(130.180219119405,31.614746621804,25.4670002959944));
#43237=CARTESIAN_POINT('Ctrl Pts',(130.069405707223,31.6103176152723,25.4601193795781));
#43238=CARTESIAN_POINT('Ctrl Pts',(130.003377710681,31.6096089405565,25.4559544395889));
#43239=CARTESIAN_POINT('Ctrl Pts',(129.66928852897,31.6157822573266,25.4346767409217));
#43240=CARTESIAN_POINT('Ctrl Pts',(129.402695369103,31.6525300271691,25.417131426605));
#43241=CARTESIAN_POINT('Ctrl Pts',(129.055215597889,31.7433052671798,25.3947593741147));
#43242=CARTESIAN_POINT('Ctrl Pts',(128.968168005087,31.769829234072,25.3891878459411));
#43243=CARTESIAN_POINT('Ctrl Pts',(128.846812310557,31.8122146970748,25.3814696405325));
#43244=CARTESIAN_POINT('Ctrl Pts',(128.811545657411,31.8251939538447,25.3792324901097));
#43245=CARTESIAN_POINT('Ctrl Pts',(128.75152771164,31.8484227609361,25.3754338206403));
#43246=CARTESIAN_POINT('Ctrl Pts',(128.726669315714,31.8583839861758,25.3738630281188));
#43247=CARTESIAN_POINT('Ctrl Pts',(128.67584405608,31.8794530011107,25.3706557048513));
#43248=CARTESIAN_POINT('Ctrl Pts',(128.64989269087,31.8905928442706,25.3690203893503));
#43249=CARTESIAN_POINT('Ctrl Pts',(128.584039948951,31.9198405991372,25.3648748877376));
#43250=CARTESIAN_POINT('Ctrl Pts',(128.544344296766,31.9384004961606,25.3623800196358));
#43251=CARTESIAN_POINT('Ctrl Pts',(128.353189201532,32.0323346100762,25.3503687049164));
#43252=CARTESIAN_POINT('Ctrl Pts',(128.207150797338,32.1182081988254,25.3412166055121));
#43253=CARTESIAN_POINT('Ctrl Pts',(127.879500123245,32.3454607097316,25.3199622793837));
#43254=CARTESIAN_POINT('Ctrl Pts',(127.704672406112,32.4950945088724,25.3080395430783));
#43255=CARTESIAN_POINT('Ctrl Pts',(127.509777659561,32.6995646204442,25.2923472407908));
#43256=CARTESIAN_POINT('Ctrl Pts',(127.474140499753,32.7387518038192,25.2893613295922));
#43257=CARTESIAN_POINT('Ctrl Pts',(127.425326040319,32.795023163629,25.285076797935));
#43258=CARTESIAN_POINT('Ctrl Pts',(127.411369829445,32.8114245190411,25.2838283451315));
#43259=CARTESIAN_POINT('Ctrl Pts',(127.387860111398,32.8395926419919,25.281682635137));
#43260=CARTESIAN_POINT('Ctrl Pts',(127.378227311552,32.8512927806164,25.2807908857807));
#43261=CARTESIAN_POINT('Ctrl Pts',(127.357941376522,32.8762718880977,25.2788853008936));
#43262=CARTESIAN_POINT('Ctrl Pts',(127.347309469444,32.8895669200587,25.2778701625419));
#43263=CARTESIAN_POINT('Ctrl Pts',(127.3178144485,32.9270249898117,25.2750089145093));
#43264=CARTESIAN_POINT('Ctrl Pts',(127.29917875787,32.9513640632801,25.2731484505139));
#43265=CARTESIAN_POINT('Ctrl Pts',(127.257364293247,33.0075379643608,25.2688578647804));
#43266=CARTESIAN_POINT('Ctrl Pts',(127.234405232973,33.0395304332064,25.2664166500125));
#43267=CARTESIAN_POINT('Ctrl Pts',(127.134668923196,33.1837480192524,25.2554472395178));
#43268=CARTESIAN_POINT('Ctrl Pts',(127.064131195399,33.3001282548846,25.2466936191634));
#43269=CARTESIAN_POINT('Ctrl Pts',(126.894262048728,33.622667376736,25.2231960739732));
#43270=CARTESIAN_POINT('Ctrl Pts',(126.808462737676,33.8351950907283,25.2085328572233));
#43271=CARTESIAN_POINT('Ctrl Pts',(126.729578014188,34.1068658890098,25.1912280096834));
#43272=CARTESIAN_POINT('Ctrl Pts',(126.715701777672,34.1593251541287,25.1879466538432));
#43273=CARTESIAN_POINT('Ctrl Pts',(126.695310049173,34.2446525507826,25.1827045223549));
#43274=CARTESIAN_POINT('Ctrl Pts',(126.688012340768,34.2773221286277,25.1807196649533));
#43275=CARTESIAN_POINT('Ctrl Pts',(126.675808923711,34.3360269163641,25.17719147766));
#43276=CARTESIAN_POINT('Ctrl Pts',(126.670722329536,34.36202130172,25.1756425926482));
#43277=CARTESIAN_POINT('Ctrl Pts',(126.661453128464,34.4125241800118,25.1726583184754));
#43278=CARTESIAN_POINT('Ctrl Pts',(126.657234468223,34.4370242459116,25.171221895726));
#43279=CARTESIAN_POINT('Ctrl Pts',(126.64856716605,34.4908974144687,25.1680870208185));
#43280=CARTESIAN_POINT('Ctrl Pts',(126.644234333626,34.5202872178922,25.1663922073998));
#43281=CARTESIAN_POINT('Ctrl Pts',(126.632668429241,34.6065869431955,25.1614574667667));
#43282=CARTESIAN_POINT('Ctrl Pts',(126.626492777579,34.6636292772607,25.158249059291));
#43283=CARTESIAN_POINT('Ctrl Pts',(126.614019374351,34.8145552517435,25.1498746786886));
#43284=CARTESIAN_POINT('Ctrl Pts',(126.610176989097,34.9085915285476,25.1447743661338));
#43285=CARTESIAN_POINT('Ctrl Pts',(126.610251050396,35.0026685497381,25.1397300250475));
#43286=CARTESIAN_POINT('Ctrl Pts',(126.610251047997,35.0026655008656,25.1397301885258));
#43287=CARTESIAN_POINT('Ctrl Pts',(126.610411758205,35.2070425715522,25.1287716367825));
#43288=CARTESIAN_POINT('Ctrl Pts',(126.629055404885,35.410984343521,25.1181316552081));
#43289=CARTESIAN_POINT('Ctrl Pts',(126.677916805914,35.6771690046066,25.1034765027583));
#43290=CARTESIAN_POINT('Ctrl Pts',(126.691785958565,35.7419660293238,25.0998446330445));
#43291=CARTESIAN_POINT('Ctrl Pts',(126.71824746432,35.8500177327797,25.0936194389212));
#43292=CARTESIAN_POINT('Ctrl Pts',(126.729819636648,35.8935042484559,25.0910672634323));
#43293=CARTESIAN_POINT('Ctrl Pts',(126.74770960057,35.9557206995766,25.0873315179809));
#43294=CARTESIAN_POINT('Ctrl Pts',(126.75333139516,35.9746475401143,25.0861837152293));
#43295=CARTESIAN_POINT('Ctrl Pts',(126.763497891763,36.0078107303777,25.0841508300451));
#43296=CARTESIAN_POINT('Ctrl Pts',(126.767971885647,36.0220678160657,25.0832697016655));
#43297=CARTESIAN_POINT('Ctrl Pts',(126.778068619525,36.0535132963877,25.0813100266379));
#43298=CARTESIAN_POINT('Ctrl Pts',(126.783734654622,36.0706863601936,25.0802291716339));
#43299=CARTESIAN_POINT('Ctrl Pts',(126.799688454388,36.1177708137905,25.0772380051815));
#43300=CARTESIAN_POINT('Ctrl Pts',(126.81025760997,36.1475839355275,25.0753131189722));
#43301=CARTESIAN_POINT('Ctrl Pts',(126.821241918346,36.177243441613,25.0733700900595));
#43302=CARTESIAN_POINT('Ctrl Pts',(126.821241938915,36.1772434971515,25.4139333020124));
#43303=CARTESIAN_POINT('Ctrl Pts',(126.78724614494,36.0854490600593,25.4191426080237));
#43304=CARTESIAN_POINT('Ctrl Pts',(126.75721423552,35.9921489540796,25.424315204267));
#43305=CARTESIAN_POINT('Ctrl Pts',(126.688840915227,35.743156357095,25.4380512485099));
#43306=CARTESIAN_POINT('Ctrl Pts',(126.65743459532,35.5859191685083,25.446654728435));
#43307=CARTESIAN_POINT('Ctrl Pts',(126.633676918287,35.3988522521441,25.4573909038189));
#43308=CARTESIAN_POINT('Ctrl Pts',(126.63044856704,35.3705903905907,25.4590263632019));
#43309=CARTESIAN_POINT('Ctrl Pts',(126.625904666717,35.3258217551147,25.4616429440096));
#43310=CARTESIAN_POINT('Ctrl Pts',(126.624353675026,35.3093396156075,25.4626118119845));
#43311=CARTESIAN_POINT('Ctrl Pts',(126.62161264969,35.2777304569417,25.4644816173911));
#43312=CARTESIAN_POINT('Ctrl Pts',(126.62040335581,35.2626057591035,25.4653815253128));
#43313=CARTESIAN_POINT('Ctrl Pts',(126.617650048713,35.2249932407246,25.4676316781336));
#43314=CARTESIAN_POINT('Ctrl Pts',(126.616228744797,35.202497367276,25.4689883103746));
#43315=CARTESIAN_POINT('Ctrl Pts',(126.611870211821,35.1205288024494,25.4739668504102));
#43316=CARTESIAN_POINT('Ctrl Pts',(126.610275975868,35.0609985004644,25.4776501540227));
#43317=CARTESIAN_POINT('Ctrl Pts',(126.610205881451,34.8983686986595,25.4878439336558));
#43318=CARTESIAN_POINT('Ctrl Pts',(126.614864496924,34.7953329491614,25.494445207943));
#43319=CARTESIAN_POINT('Ctrl Pts',(126.648420604002,34.426737769577,25.5182664324351));
#43320=CARTESIAN_POINT('Ctrl Pts',(126.703976256081,34.1645450672507,25.5355023094875));
#43321=CARTESIAN_POINT('Ctrl Pts',(126.806981197994,33.8607384048183,25.5550453529368));
#43322=CARTESIAN_POINT('Ctrl Pts',(126.825421485116,33.810320296512,25.5582779957451));
#43323=CARTESIAN_POINT('Ctrl Pts',(126.856231288907,33.731907809254,25.5632908257431));
#43324=CARTESIAN_POINT('Ctrl Pts',(126.867794988551,33.7036083265279,25.5650969549421));
#43325=CARTESIAN_POINT('Ctrl Pts',(126.89007157606,33.6511303474066,25.5684415969058));
#43326=CARTESIAN_POINT('Ctrl Pts',(126.900687553983,33.6269134906624,25.5699831842844));
#43327=CARTESIAN_POINT('Ctrl Pts',(126.925135318675,33.5728725153561,25.5734202769261));
#43328=CARTESIAN_POINT('Ctrl Pts',(126.939119898247,33.5431201912837,25.5753104667458));
#43329=CARTESIAN_POINT('Ctrl Pts',(126.983029030392,33.4531273314043,25.581025207538));
#43330=CARTESIAN_POINT('Ctrl Pts',(127.014316419729,33.3935681546972,25.5848034347772));
#43331=CARTESIAN_POINT('Ctrl Pts',(127.16968743093,33.1180434245127,25.6023333111695));
#43332=CARTESIAN_POINT('Ctrl Pts',(127.315548531494,32.9152565506276,25.61532180848));
#43333=CARTESIAN_POINT('Ctrl Pts',(127.581383438689,32.620380279568,25.6364865904468));
#43334=CARTESIAN_POINT('Ctrl Pts',(127.687531554942,32.5171031700493,25.6444715927467));
#43335=CARTESIAN_POINT('Ctrl Pts',(127.821605590945,32.4027314406696,25.6545069939703));
#43336=CARTESIAN_POINT('Ctrl Pts',(127.843367457853,32.3846334601348,25.6561345442673));
#43337=CARTESIAN_POINT('Ctrl Pts',(127.878189226834,32.3564044989029,25.6587413672163));
#43338=CARTESIAN_POINT('Ctrl Pts',(127.891101451538,32.3460925001281,25.6597085409375));
#43339=CARTESIAN_POINT('Ctrl Pts',(127.916165700065,32.3263740320514,25.6615881019812));
#43340=CARTESIAN_POINT('Ctrl Pts',(127.928307110233,32.3169551359925,25.6624996291));
#43341=CARTESIAN_POINT('Ctrl Pts',(127.958599424219,32.2937835737672,25.6647756590725));
#43342=CARTESIAN_POINT('Ctrl Pts',(127.976825522163,32.2801307702699,25.6661466459358));
#43343=CARTESIAN_POINT('Ctrl Pts',(128.048605097628,32.2274828122752,25.6715475648451));
#43344=CARTESIAN_POINT('Ctrl Pts',(128.103156590736,32.1898794462459,25.6756553895023));
#43345=CARTESIAN_POINT('Ctrl Pts',(128.258751584076,32.0892202447363,25.687306516073));
#43346=CARTESIAN_POINT('Ctrl Pts',(128.362066891044,32.0298556554298,25.6949661579377));
#43347=CARTESIAN_POINT('Ctrl Pts',(128.690371120084,31.8635603569447,25.7186854876994));
#43348=CARTESIAN_POINT('Ctrl Pts',(128.924208690513,31.7758580474907,25.7346583254899));
#43349=CARTESIAN_POINT('Ctrl Pts',(129.215397055654,31.7019026503466,25.7529212870196));
#43350=CARTESIAN_POINT('Ctrl Pts',(129.2655070823,31.6903824246386,25.7560118907501));
#43351=CARTESIAN_POINT('Ctrl Pts',(129.345050879154,31.6739911476349,25.7608378746362));
#43352=CARTESIAN_POINT('Ctrl Pts',(129.374318569061,31.6683613538053,25.7625966722292));
#43353=CARTESIAN_POINT('Ctrl Pts',(129.429784426982,31.6584489102964,25.7658989883642));
#43354=CARTESIAN_POINT('Ctrl Pts',(129.455965899989,31.654086605747,25.7674448818136));
#43355=CARTESIAN_POINT('Ctrl Pts',(129.515836767469,31.6448323836095,25.7709518161791));
#43356=CARTESIAN_POINT('Ctrl Pts',(129.549554307204,31.6401395017706,25.7729065542013));
#43357=CARTESIAN_POINT('Ctrl Pts',(129.656724476378,31.6268656692521,25.7790600552336));
#43358=CARTESIAN_POINT('Ctrl Pts',(129.730392212804,31.6201795876266,25.7832009591173));
#43359=CARTESIAN_POINT('Ctrl Pts',(129.909322388081,31.6098281225146,25.793093700157));
#43360=CARTESIAN_POINT('Ctrl Pts',(130.014651704467,31.6086470070153,25.7987783263936));
#43361=CARTESIAN_POINT('Ctrl Pts',(130.243975894216,31.6167615507051,25.8110391674679));
#43362=CARTESIAN_POINT('Ctrl Pts',(130.367746273111,31.6279695479897,25.8175819437801));
#43363=CARTESIAN_POINT('Ctrl Pts',(130.633803766805,31.6668877327694,25.8318930272458));
#43364=CARTESIAN_POINT('Ctrl Pts',(130.775484295209,31.6969770022114,25.8396704604642));
#43365=CARTESIAN_POINT('Ctrl Pts',(130.949123581928,31.7456428349665,25.8498525113236));
#43366=CARTESIAN_POINT('Ctrl Pts',(130.983297479166,31.7558048782406,25.8518888877336));
#43367=CARTESIAN_POINT('Ctrl Pts',(131.034511431215,31.7719175054613,25.8549984614742));
#43368=CARTESIAN_POINT('Ctrl Pts',(131.051675652803,31.7774685754146,25.856050504868));
#43369=CARTESIAN_POINT('Ctrl Pts',(131.082979776073,31.7878693508187,25.8579887083869));
#43370=CARTESIAN_POINT('Ctrl Pts',(131.097133066253,31.7926759578876,25.8588724593206));
#43371=CARTESIAN_POINT('Ctrl Pts',(131.129963235379,31.8040681594395,25.8609396042834));
#43372=CARTESIAN_POINT('Ctrl Pts',(131.148614640574,31.8107239679616,25.8621268654764));
#43373=CARTESIAN_POINT('Ctrl Pts',(131.209782591993,31.8331580813246,25.8660605443639));
#43374=CARTESIAN_POINT('Ctrl Pts',(131.252039247815,31.8496255845609,25.8688419997517));
#43375=CARTESIAN_POINT('Ctrl Pts',(131.355864826834,31.8925053731902,25.8758140411302));
#43376=CARTESIAN_POINT('Ctrl Pts',(131.417004491463,31.9199042791809,25.8800419997484));
#43377=CARTESIAN_POINT('Ctrl Pts',(131.730132241768,32.0715249194986,25.9022057181325));
#43378=CARTESIAN_POINT('Ctrl Pts',(131.966819487439,32.2249357559728,25.9205912344941));
#43379=CARTESIAN_POINT('Ctrl Pts',(132.243507293534,32.457645169772,25.9429954439113));
#43380=CARTESIAN_POINT('Ctrl Pts',(132.303287253762,32.5116747601661,25.9479099168073));
#43381=CARTESIAN_POINT('Ctrl Pts',(132.384334489616,32.590351967441,25.9546800141562));
#43382=CARTESIAN_POINT('Ctrl Pts',(132.407255554415,32.6132500331549,25.9566075982063));
#43383=CARTESIAN_POINT('Ctrl Pts',(132.448620379695,32.6557755324814,25.9601112378114));
#43384=CARTESIAN_POINT('Ctrl Pts',(132.467165044618,32.6753007026878,25.9616915620214));
#43385=CARTESIAN_POINT('Ctrl Pts',(132.504513233249,32.7155739469466,25.9648949990808));
#43386=CARTESIAN_POINT('Ctrl Pts',(132.523296304224,32.7363381973103,25.9665171906052));
#43387=CARTESIAN_POINT('Ctrl Pts',(132.570016032277,32.789289959578,25.9705823052299));
#43388=CARTESIAN_POINT('Ctrl Pts',(132.597607346055,32.8217765052163,25.9730111193099));
#43389=CARTESIAN_POINT('Ctrl Pts',(132.719063148581,32.9703718918971,25.9838461330538));
#43390=CARTESIAN_POINT('Ctrl Pts',(132.805811734546,33.0920896922729,25.9919753845479));
#43391=CARTESIAN_POINT('Ctrl Pts',(132.951925418626,33.3287338390268,26.0068656823502));
#43392=CARTESIAN_POINT('Ctrl Pts',(133.013290750971,33.4420932688901,26.0136513860237));
#43393=CARTESIAN_POINT('Ctrl Pts',(133.131482263418,33.6936791587142,26.0284347397644));
#43394=CARTESIAN_POINT('Ctrl Pts',(133.185921183258,33.8327154831244,26.0364383115737));
#43395=CARTESIAN_POINT('Ctrl Pts',(133.241874225197,34.0090691483376,26.0468825065732));
#43396=CARTESIAN_POINT('Ctrl Pts',(133.252180978407,34.0434378672002,26.0489315242536));
#43397=CARTESIAN_POINT('Ctrl Pts',(133.266858912297,34.0953647398473,26.052056562586));
#43398=CARTESIAN_POINT('Ctrl Pts',(133.271638534392,34.1128058977298,26.0531111140671));
#43399=CARTESIAN_POINT('Ctrl Pts',(133.280112330254,34.1447272539749,26.0550515320572));
#43400=CARTESIAN_POINT('Ctrl Pts',(133.283850635073,34.1591948207184,26.0559349473256));
#43401=CARTESIAN_POINT('Ctrl Pts',(133.292306025392,34.192834646471,26.0579981028226));
#43402=CARTESIAN_POINT('Ctrl Pts',(133.296951381128,34.2120238443578,26.0591816571156));
#43403=CARTESIAN_POINT('Ctrl Pts',(133.311632672507,34.2750734231234,26.0630897934203));
#43404=CARTESIAN_POINT('Ctrl Pts',(133.320962611913,34.3190914771046,26.0658488186212));
#43405=CARTESIAN_POINT('Ctrl Pts',(133.341856562497,34.4283460588573,26.0727509315481));
#43406=CARTESIAN_POINT('Ctrl Pts',(133.352389240764,34.4937599307751,26.0769305157319));
#43407=CARTESIAN_POINT('Ctrl Pts',(133.396219226552,34.8281330854671,26.098407060591));
#43408=CARTESIAN_POINT('Ctrl Pts',(133.399095152849,35.1001269397107,26.1161406110915));
#43409=CARTESIAN_POINT('Ctrl Pts',(133.359869795336,35.4577713463583,26.1385272932438));
#43410=CARTESIAN_POINT('Ctrl Pts',(133.346734566545,35.5455726577009,26.1439580288845));
#43411=CARTESIAN_POINT('Ctrl Pts',(133.323231154039,35.6692686246362,26.15151456168));
#43412=CARTESIAN_POINT('Ctrl Pts',(133.315694867736,35.7056582062518,26.1537260469566));
#43413=CARTESIAN_POINT('Ctrl Pts',(133.301657185491,35.7682399477624,26.1575107106607));
#43414=CARTESIAN_POINT('Ctrl Pts',(133.295438710376,35.7944913823401,26.1590925960401));
#43415=CARTESIAN_POINT('Ctrl Pts',(133.282022805055,35.848257043926,26.1623217419977));
#43416=CARTESIAN_POINT('Ctrl Pts',(133.274791165663,35.8757605827778,26.1639677778107));
#43417=CARTESIAN_POINT('Ctrl Pts',(133.255282939054,35.9463314819004,26.1681781856861));
#43418=CARTESIAN_POINT('Ctrl Pts',(133.24249730694,35.9892531347847,26.1707262411519));
#43419=CARTESIAN_POINT('Ctrl Pts',(133.170354094127,36.214990446809,26.184079251524));
#43420=CARTESIAN_POINT('Ctrl Pts',(133.096376796749,36.3927700589008,26.19440126684));
#43421=CARTESIAN_POINT('Ctrl Pts',(132.914834846855,36.742040773895,26.2153105494072));
#43422=CARTESIAN_POINT('Ctrl Pts',(132.806214736876,36.9120967792971,26.2258502858973));
#43423=CARTESIAN_POINT('Ctrl Pts',(132.649393039,37.1152243554,26.2400812804722));
#43424=CARTESIAN_POINT('Ctrl Pts',(132.614567679247,37.1581224950231,26.2431916057995));
#43425=CARTESIAN_POINT('Ctrl Pts',(132.564499063996,37.2168060593527,26.2476256048923));
#43426=CARTESIAN_POINT('Ctrl Pts',(132.55012574811,37.2333255849865,26.2488943656532));
#43427=CARTESIAN_POINT('Ctrl Pts',(132.525497139745,37.2610839658848,26.2510637652774));
#43428=CARTESIAN_POINT('Ctrl Pts',(132.515324144737,37.2723954200347,26.2519585752976));
#43429=CARTESIAN_POINT('Ctrl Pts',(132.49371508611,37.2960998415725,26.2538573993943));
#43430=CARTESIAN_POINT('Ctrl Pts',(132.482262300063,37.3084763936837,26.2548625510395));
#43431=CARTESIAN_POINT('Ctrl Pts',(132.450253642737,37.3425532199807,26.2576671177802));
#43432=CARTESIAN_POINT('Ctrl Pts',(132.429502839985,37.3640673256111,26.2594800297852));
#43433=CARTESIAN_POINT('Ctrl Pts',(132.381665254242,37.4123695417553,26.2636418140288));
#43434=CARTESIAN_POINT('Ctrl Pts',(132.354406133022,37.4389808782852,26.2660009032943));
#43435=CARTESIAN_POINT('Ctrl Pts',(132.261683280735,37.5264971981452,26.2739676947997));
#43436=CARTESIAN_POINT('Ctrl Pts',(132.194261612193,37.5852685887009,26.2796662504711));
#43437=CARTESIAN_POINT('Ctrl Pts',(131.894836912965,37.8261185135034,26.3043348915966));
#43438=CARTESIAN_POINT('Ctrl Pts',(131.641889943307,37.9802028589468,26.3234608454401));
#43439=CARTESIAN_POINT('Ctrl Pts',(131.326104938872,38.1199981527272,26.3444371791626));
#43440=CARTESIAN_POINT('Ctrl Pts',(131.279590474274,38.1393616242839,26.3474638417174));
#43441=CARTESIAN_POINT('Ctrl Pts',(131.205095240521,38.1684422212339,26.3522140059146));
#43442=CARTESIAN_POINT('Ctrl Pts',(131.177390408656,38.178841385905,26.3539596947402));
#43443=CARTESIAN_POINT('Ctrl Pts',(131.124544550547,38.1978916919145,26.3572510773682));
#43444=CARTESIAN_POINT('Ctrl Pts',(131.099431131877,38.2066123814533,26.3587989449796));
#43445=CARTESIAN_POINT('Ctrl Pts',(131.041571751205,38.2259445205204,26.3623291770914));
#43446=CARTESIAN_POINT('Ctrl Pts',(131.008761267519,38.2363545218863,26.3643049165404));
#43447=CARTESIAN_POINT('Ctrl Pts',(130.902797165338,38.2682063615257,26.3706068726379));
#43448=CARTESIAN_POINT('Ctrl Pts',(130.829074669472,38.2876818444433,26.3748710192081));
#43449=CARTESIAN_POINT('Ctrl Pts',(130.647451032434,38.3291630761976,26.3851405980968));
#43450=CARTESIAN_POINT('Ctrl Pts',(130.539013511112,38.3484304156418,26.3910711980922));
#43451=CARTESIAN_POINT('Ctrl Pts',(130.21919651251,38.3893137478553,26.4082716381633));
#43452=CARTESIAN_POINT('Ctrl Pts',(130.006518337483,38.3963864385934,26.4193233749639));
#43453=CARTESIAN_POINT('Ctrl Pts',(129.7249755408,38.3792944430617,26.4348116122454));
#43454=CARTESIAN_POINT('Ctrl Pts',(129.655510574254,38.3729208588594,26.4387057544104));
#43455=CARTESIAN_POINT('Ctrl Pts',(129.562606193132,38.361496904243,26.4440690797105));
#43456=CARTESIAN_POINT('Ctrl Pts',(129.538948023096,38.3583337810692,26.4454484618425));
#43457=CARTESIAN_POINT('Ctrl Pts',(129.501432476822,38.3529140377692,26.4476602002746));
#43458=CARTESIAN_POINT('Ctrl Pts',(129.487551875624,38.3508206493504,26.4484838590039));
#43459=CARTESIAN_POINT('Ctrl Pts',(129.458127069433,38.3461958724362,26.4502419541585));
#43460=CARTESIAN_POINT('Ctrl Pts',(129.442586827947,38.3436422684019,26.4511776476971));
#43461=CARTESIAN_POINT('Ctrl Pts',(129.402728566306,38.3368070956997,26.4535950378974));
#43462=CARTESIAN_POINT('Ctrl Pts',(129.378438869474,38.3323679933103,26.4550849553129));
#43463=CARTESIAN_POINT('Ctrl Pts',(129.270951786874,38.3115079878682,26.4617461553046));
#43464=CARTESIAN_POINT('Ctrl Pts',(129.188344702409,38.2922347877404,26.4670461697472));
#43465=CARTESIAN_POINT('Ctrl Pts',(128.924599016786,38.2201703551241,26.4843793302038));
#43466=CARTESIAN_POINT('Ctrl Pts',(128.747112982166,38.1553540329263,26.4966611666724));
#43467=CARTESIAN_POINT('Ctrl Pts',(128.421636549016,38.0046773507659,26.5195942091316));
#43468=CARTESIAN_POINT('Ctrl Pts',(128.272911156707,37.9217280443934,26.5302566622879));
#43469=CARTESIAN_POINT('Ctrl Pts',(128.093959684016,37.803460196987,26.5432216317841));
#43470=CARTESIAN_POINT('Ctrl Pts',(128.057380166286,37.7782381512113,26.5458806918995));
#43471=CARTESIAN_POINT('Ctrl Pts',(127.998275293459,37.7357462962776,26.5501937125388));
#43472=CARTESIAN_POINT('Ctrl Pts',(127.975453123062,37.718900442189,26.5518632917375));
#43473=CARTESIAN_POINT('Ctrl Pts',(127.931313403305,37.6854553758177,26.5551016323908));
#43474=CARTESIAN_POINT('Ctrl Pts',(127.909977604473,37.6688838976175,26.5566712888612));
#43475=CARTESIAN_POINT('Ctrl Pts',(127.859594084819,37.6287763458617,26.5603898069537));
#43476=CARTESIAN_POINT('Ctrl Pts',(127.830732824561,37.6050110627055,26.5625294756689));
#43477=CARTESIAN_POINT('Ctrl Pts',(127.728993602701,37.518372134899,26.5701139594879));
#43478=CARTESIAN_POINT('Ctrl Pts',(127.658404608437,37.4528761678907,26.5754534819271));
#43479=CARTESIAN_POINT('Ctrl Pts',(127.478579338137,37.2711771729287,26.5894012819383));
#43480=CARTESIAN_POINT('Ctrl Pts',(127.374589810402,37.150123819047,26.5978315907567));
#43481=CARTESIAN_POINT('Ctrl Pts',(127.169380576106,36.8740526380048,26.616071228891));
#43482=CARTESIAN_POINT('Ctrl Pts',(127.071555795253,36.7171720423548,26.6258582397219));
#43483=CARTESIAN_POINT('Ctrl Pts',(126.971064171271,36.522222677682,26.6382482074251));
#43484=CARTESIAN_POINT('Ctrl Pts',(126.955609467031,36.4910735132362,26.6402348019939));
#43485=CARTESIAN_POINT('Ctrl Pts',(126.932850421994,36.4433729667018,26.6432955881083));
#43486=CARTESIAN_POINT('Ctrl Pts',(126.92519446344,36.4269908672716,26.6443500590425));
#43487=CARTESIAN_POINT('Ctrl Pts',(126.911451779634,36.3969603658288,26.6462904054207));
#43488=CARTESIAN_POINT('Ctrl Pts',(126.905323713077,36.3833318568459,26.6471738309701));
#43489=CARTESIAN_POINT('Ctrl Pts',(126.891307580864,36.3516014172279,26.6492371126788));
#43490=CARTESIAN_POINT('Ctrl Pts',(126.88348738244,36.3334706637344,26.65042078459));
#43491=CARTESIAN_POINT('Ctrl Pts',(126.85836361659,36.2737940769975,26.6543297314844));
#43492=CARTESIAN_POINT('Ctrl Pts',(126.841729660886,36.2319734444147,26.6570894684764));
#43493=CARTESIAN_POINT('Ctrl Pts',(126.824361661966,36.1856417146286,26.6601597368587));
#43494=CARTESIAN_POINT('Ctrl Pts',(126.822797614578,36.1814440867763,26.6604380167156));
#43495=CARTESIAN_POINT('Ctrl Pts',(126.821241918426,36.1772434418289,26.660716603687));
#43496=CARTESIAN_POINT('Origin',(130.,35.,23.));
#43497=CARTESIAN_POINT('',(126.821241918358,36.1772434416438,27.913420165303));
#43498=CARTESIAN_POINT('',(126.821241849407,36.1772432554656,27.5681926079129));
#43499=CARTESIAN_POINT('',(126.821241918358,36.1772434416438,23.));
#43500=CARTESIAN_POINT('Ctrl Pts',(126.821241849407,36.1772432554656,27.5681926079129));
#43501=CARTESIAN_POINT('Ctrl Pts',(126.84174973112,36.2326180438488,27.5645149152729));
#43502=CARTESIAN_POINT('Ctrl Pts',(126.863708823237,36.2874684205701,27.560875143329));
#43503=CARTESIAN_POINT('Ctrl Pts',(126.908094792219,36.3904461959036,27.5540501120195));
#43504=CARTESIAN_POINT('Ctrl Pts',(126.930230872951,36.4386578534972,27.5508583571272));
#43505=CARTESIAN_POINT('Ctrl Pts',(126.966703979077,36.513416152388,27.545912642408));
#43506=CARTESIAN_POINT('Ctrl Pts',(126.980278559587,36.5403232488672,27.5441332650874));
#43507=CARTESIAN_POINT('Ctrl Pts',(127.006455704018,36.5905342607911,27.5408130429875));
#43508=CARTESIAN_POINT('Ctrl Pts',(127.018976054374,36.6138782423286,27.5392695146579));
#43509=CARTESIAN_POINT('Ctrl Pts',(127.047946222346,36.6664049900041,27.5357954366995));
#43510=CARTESIAN_POINT('Ctrl Pts',(127.064557704424,36.6954957212301,27.5338707303769));
#43511=CARTESIAN_POINT('Ctrl Pts',(127.117602918107,36.7852736030098,27.5279244917695));
#43512=CARTESIAN_POINT('Ctrl Pts',(127.155509017487,36.8450709425282,27.5239552016483));
#43513=CARTESIAN_POINT('Ctrl Pts',(127.334377706038,37.1086080224966,27.5063419690037));
#43514=CARTESIAN_POINT('Ctrl Pts',(127.495538001034,37.2977041148758,27.493434436482));
#43515=CARTESIAN_POINT('Ctrl Pts',(127.772738451284,37.5587924450687,27.4731179030451));
#43516=CARTESIAN_POINT('Ctrl Pts',(127.874886671473,37.644238972395,27.4659315126575));
#43517=CARTESIAN_POINT('Ctrl Pts',(128.009569288014,37.7440457123043,27.4564556370403));
#43518=CARTESIAN_POINT('Ctrl Pts',(128.037669831768,37.7642108109722,27.4544783598304));
#43519=CARTESIAN_POINT('Ctrl Pts',(128.080715429515,37.7941133962775,27.451441159174));
#43520=CARTESIAN_POINT('Ctrl Pts',(128.095437694628,37.8041692759178,27.4504009441274));
#43521=CARTESIAN_POINT('Ctrl Pts',(128.122668895766,37.8224558793165,27.4484729153796));
#43522=CARTESIAN_POINT('Ctrl Pts',(128.135154008266,37.8307205203255,27.4475873106595));
#43523=CARTESIAN_POINT('Ctrl Pts',(128.164237610395,37.8496967816733,27.4455208008625));
#43524=CARTESIAN_POINT('Ctrl Pts',(128.180875448037,37.8603463289733,27.4443360901591));
#43525=CARTESIAN_POINT('Ctrl Pts',(128.235281704718,37.8945040111036,27.4404563256271));
#43526=CARTESIAN_POINT('Ctrl Pts',(128.273418600079,37.9174133068107,27.4377279023964));
#43527=CARTESIAN_POINT('Ctrl Pts',(128.495145996398,38.044737393464,27.4218620742426));
#43528=CARTESIAN_POINT('Ctrl Pts',(128.687718191046,38.13255820633,27.408103943716));
#43529=CARTESIAN_POINT('Ctrl Pts',(128.933002366131,38.2178055231709,27.3914238318584));
#43530=CARTESIAN_POINT('Ctrl Pts',(128.979142033192,38.2327396305289,27.388319323848));
#43531=CARTESIAN_POINT('Ctrl Pts',(129.172328257359,38.2907198498557,27.3754769024027));
#43532=CARTESIAN_POINT('Ctrl Pts',(129.321900194696,38.3247659190711,27.3659172352249));
#43533=CARTESIAN_POINT('Ctrl Pts',(129.515640425054,38.355240633082,27.3540795555603));
#43534=CARTESIAN_POINT('Ctrl Pts',(129.558125279094,38.361099654519,27.3515157407274));
#43535=CARTESIAN_POINT('Ctrl Pts',(129.628566802088,38.3694553393505,27.3473159959942));
#43536=CARTESIAN_POINT('Ctrl Pts',(129.656462760342,38.3724136964487,27.3456660127627));
#43537=CARTESIAN_POINT('Ctrl Pts',(129.711167767749,38.3775292993976,27.342455137609));
#43538=CARTESIAN_POINT('Ctrl Pts',(129.737972055596,38.3797144323193,27.3408934994096));
#43539=CARTESIAN_POINT('Ctrl Pts',(129.796972160738,38.3838180814644,27.3374803530737));
#43540=CARTESIAN_POINT('Ctrl Pts',(129.829175272596,38.3855965686326,27.3356332552991));
#43541=CARTESIAN_POINT('Ctrl Pts',(129.94093078705,38.3901698603592,27.3292736917755));
#43542=CARTESIAN_POINT('Ctrl Pts',(130.020555456256,38.3906223087319,27.3248318949768));
#43543=CARTESIAN_POINT('Ctrl Pts',(130.33685043225,38.3812754888362,27.3074366036708));
#43544=CARTESIAN_POINT('Ctrl Pts',(130.572183542738,38.3494925762648,27.2950988421214));
#43545=CARTESIAN_POINT('Ctrl Pts',(130.928065421479,38.2627992155865,27.2755386718988));
#43546=CARTESIAN_POINT('Ctrl Pts',(131.051974902345,38.2249817013313,27.2685364923311));
#43547=CARTESIAN_POINT('Ctrl Pts',(131.205466811719,38.1683469882307,27.2592840484598));
#43548=CARTESIAN_POINT('Ctrl Pts',(131.237345259842,38.1560338072496,27.2573297118351));
#43549=CARTESIAN_POINT('Ctrl Pts',(131.285486515758,38.1365975849077,27.2543206405524));
#43550=CARTESIAN_POINT('Ctrl Pts',(131.301889403412,38.1298249060935,27.2532850659268));
#43551=CARTESIAN_POINT('Ctrl Pts',(131.332043859615,38.1170962101829,27.2513609024119));
#43552=CARTESIAN_POINT('Ctrl Pts',(131.345810180136,38.1111773586945,27.2504744430772));
#43553=CARTESIAN_POINT('Ctrl Pts',(131.377742144528,38.0971965742605,27.248399785386));
#43554=CARTESIAN_POINT('Ctrl Pts',(131.395876669298,38.0890659297726,27.247207677887));
#43555=CARTESIAN_POINT('Ctrl Pts',(131.45498571281,38.061937531507,27.2432789150226));
#43556=CARTESIAN_POINT('Ctrl Pts',(131.495650617758,38.042281000395,27.2405077789005));
#43557=CARTESIAN_POINT('Ctrl Pts',(131.723618261122,37.926411238217,27.2246313732063));
#43558=CARTESIAN_POINT('Ctrl Pts',(131.902021006087,37.8137256473614,27.2109148855617));
#43559=CARTESIAN_POINT('Ctrl Pts',(132.198835336501,37.5850474743562,27.1868480067767));
#43560=CARTESIAN_POINT('Ctrl Pts',(132.321425233059,37.4755490232633,27.1764468694824));
#43561=CARTESIAN_POINT('Ctrl Pts',(132.479909235462,37.3118201369169,27.1624757311334));
#43562=CARTESIAN_POINT('Ctrl Pts',(132.522912922333,37.2648119928417,27.1586216003407));
#43563=CARTESIAN_POINT('Ctrl Pts',(132.585636553301,37.1922423855049,27.1528999137642));
#43564=CARTESIAN_POINT('Ctrl Pts',(132.606356417777,37.1675676214481,27.1509921928415));
#43565=CARTESIAN_POINT('Ctrl Pts',(132.64179178201,37.1241256241629,27.1476972723839));
#43566=CARTESIAN_POINT('Ctrl Pts',(132.656666605396,37.1054918849347,27.1463038006724));
#43567=CARTESIAN_POINT('Ctrl Pts',(132.68987902583,37.062974180349,27.14316791993));
#43568=CARTESIAN_POINT('Ctrl Pts',(132.708097606682,37.0389995290249,27.1414302166747));
#43569=CARTESIAN_POINT('Ctrl Pts',(132.756619633286,36.9733494435621,27.1367513058747));
#43570=CARTESIAN_POINT('Ctrl Pts',(132.786296829381,36.9312198733415,27.1338337838781));
#43571=CARTESIAN_POINT('Ctrl Pts',(132.949650735728,36.6877148789652,27.1174122987796));
#43572=CARTESIAN_POINT('Ctrl Pts',(133.062447115473,36.4731767677177,27.1046881559627));
#43573=CARTESIAN_POINT('Ctrl Pts',(133.21675677284,36.0836520442633,27.082451282347));
#43574=CARTESIAN_POINT('Ctrl Pts',(133.269007399097,35.9140035793927,27.072999501741));
#43575=CARTESIAN_POINT('Ctrl Pts',(133.314309057919,35.7118007230369,27.0612244768151));
#43576=CARTESIAN_POINT('Ctrl Pts',(133.320477697972,35.6824459887214,27.0595025402855));
#43577=CARTESIAN_POINT('Ctrl Pts',(133.329508525208,35.6364457110599,27.0567793039032));
#43578=CARTESIAN_POINT('Ctrl Pts',(133.332637380287,35.6198533920223,27.0557919994136));
#43579=CARTESIAN_POINT('Ctrl Pts',(133.33834797022,35.5882763702048,27.0539023255508));
#43580=CARTESIAN_POINT('Ctrl Pts',(133.340953034992,35.5732966434007,27.0530012148235));
#43581=CARTESIAN_POINT('Ctrl Pts',(133.346487347797,35.5401536598437,27.0509977372896));
#43582=CARTESIAN_POINT('Ctrl Pts',(133.349369667537,35.5219830861987,27.0498929230021));
#43583=CARTESIAN_POINT('Ctrl Pts',(133.358808397105,35.4591799805184,27.0460543286177));
#43584=CARTESIAN_POINT('Ctrl Pts',(133.364621407311,35.414442367759,27.0432851332842));
#43585=CARTESIAN_POINT('Ctrl Pts',(133.392445744273,35.160778735379,27.0274360881326));
#43586=CARTESIAN_POINT('Ctrl Pts',(133.395888667287,34.9502857097828,27.0137514169556));
#43587=CARTESIAN_POINT('Ctrl Pts',(133.364771354037,34.5444732602922,26.9876098975294));
#43588=CARTESIAN_POINT('Ctrl Pts',(133.332628556801,34.3497707699144,26.9751797635475));
#43589=CARTESIAN_POINT('Ctrl Pts',(133.27260388089,34.1154168988314,26.9605512346294));
#43590=CARTESIAN_POINT('Ctrl Pts',(133.260592348471,34.0721200230522,26.9578613367002));
#43591=CARTESIAN_POINT('Ctrl Pts',(133.239569500702,34.0017991874978,26.9535116197802));
#43592=CARTESIAN_POINT('Ctrl Pts',(133.23107237707,33.9746284673449,26.9518356634807));
#43593=CARTESIAN_POINT('Ctrl Pts',(133.21386297266,33.9219384204237,26.9485937975823));
#43594=CARTESIAN_POINT('Ctrl Pts',(133.205186507776,33.8964097280512,26.9470268753813));
#43595=CARTESIAN_POINT('Ctrl Pts',(133.183860361694,33.8360359828586,26.943328843921));
#43596=CARTESIAN_POINT('Ctrl Pts',(133.170941748151,33.8012891845922,26.9412066479099));
#43597=CARTESIAN_POINT('Ctrl Pts',(133.125432144514,33.6847712507651,26.93410440991));
#43598=CARTESIAN_POINT('Ctrl Pts',(133.090226025618,33.6040567386323,26.9292094912048));
#43599=CARTESIAN_POINT('Ctrl Pts',(132.933596450339,33.2800192882011,26.9095095461876));
#43600=CARTESIAN_POINT('Ctrl Pts',(132.786268353647,33.0503792664814,26.8955158725032));
#43601=CARTESIAN_POINT('Ctrl Pts',(132.570862613999,32.7896906343086,26.8772041577259));
#43602=CARTESIAN_POINT('Ctrl Pts',(132.527135925704,32.739826288371,26.8735693367992));
#43603=CARTESIAN_POINT('Ctrl Pts',(132.451311606521,32.6583117844775,26.8673396245334));
#43604=CARTESIAN_POINT('Ctrl Pts',(132.419993456021,32.625960496851,26.8647859598575));
#43605=CARTESIAN_POINT('Ctrl Pts',(132.374025847732,32.5803313547091,26.8610484204164));
#43606=CARTESIAN_POINT('Ctrl Pts',(132.359888859941,32.5665416365412,26.859900360259));
#43607=CARTESIAN_POINT('Ctrl Pts',(132.334844466412,32.5425359224136,26.8578671991929));
#43608=CARTESIAN_POINT('Ctrl Pts',(132.323988747155,32.5322673026014,26.8569860563863));
#43609=CARTESIAN_POINT('Ctrl Pts',(132.299848281481,32.5097329773295,26.8550265762205));
#43610=CARTESIAN_POINT('Ctrl Pts',(132.286533243774,32.4975017173244,26.8539459337305));
#43611=CARTESIAN_POINT('Ctrl Pts',(132.246519414397,32.461330760321,26.8507005602657));
#43612=CARTESIAN_POINT('Ctrl Pts',(132.219538703033,32.4377083083858,26.8485150568652));
#43613=CARTESIAN_POINT('Ctrl Pts',(132.078643979194,32.3182458249101,26.837138995158));
#43614=CARTESIAN_POINT('Ctrl Pts',(131.958888328919,32.2295639714867,26.827598065087));
#43615=CARTESIAN_POINT('Ctrl Pts',(131.726048860069,32.0798040275783,26.8097653438476));
#43616=CARTESIAN_POINT('Ctrl Pts',(131.614554581721,32.0167124264297,26.8014987711256));
#43617=CARTESIAN_POINT('Ctrl Pts',(131.36499186427,31.8935898024786,26.7837941281575));
#43618=CARTESIAN_POINT('Ctrl Pts',(131.22594259457,31.8361318853769,26.7744251611541));
#43619=CARTESIAN_POINT('Ctrl Pts',(131.043077614443,31.7744432822549,26.7627786588056));
#43620=CARTESIAN_POINT('Ctrl Pts',(131.002376853114,31.7615639665268,26.7602269846072));
#43621=CARTESIAN_POINT('Ctrl Pts',(130.934581474045,31.7415115233497,26.7560416649428));
#43622=CARTESIAN_POINT('Ctrl Pts',(130.907622680837,31.7338997529692,26.7543941617961));
#43623=CARTESIAN_POINT('Ctrl Pts',(130.854578436878,31.7196303075117,26.7511843481561));
#43624=CARTESIAN_POINT('Ctrl Pts',(130.828501964309,31.7129474935023,26.7496213406051));
#43625=CARTESIAN_POINT('Ctrl Pts',(130.7709090476,31.6989166354121,26.7462007406769));
#43626=CARTESIAN_POINT('Ctrl Pts',(130.739361214378,31.6917078066846,26.7443476347643));
#43627=CARTESIAN_POINT('Ctrl Pts',(130.629182261354,31.6681862162432,26.7379427701141));
#43628=CARTESIAN_POINT('Ctrl Pts',(130.550075814619,31.6542158839966,26.7334630773457));
#43629=CARTESIAN_POINT('Ctrl Pts',(130.19197226452,31.6040202769227,26.7135922502048));
#43630=CARTESIAN_POINT('Ctrl Pts',(129.909645010857,31.5998003012233,26.6991317310287));
#43631=CARTESIAN_POINT('Ctrl Pts',(129.563438593948,31.6378118020697,26.6802805678334));
#43632=CARTESIAN_POINT('Ctrl Pts',(129.497064085396,31.6470982858762,26.6766090862874));
#43633=CARTESIAN_POINT('Ctrl Pts',(129.386294991413,31.6659590879004,26.6703232922234));
#43634=CARTESIAN_POINT('Ctrl Pts',(129.341737581999,31.6744695429726,26.6677511785052));
#43635=CARTESIAN_POINT('Ctrl Pts',(129.27799144348,31.6879763047251,26.6639914245659));
#43636=CARTESIAN_POINT('Ctrl Pts',(129.258653113571,31.6922512086516,26.6628401890118));
#43637=CARTESIAN_POINT('Ctrl Pts',(129.224787208086,31.7000494506515,26.6608036212264));
#43638=CARTESIAN_POINT('Ctrl Pts',(129.210243746969,31.7034998028508,26.6599222970913));
#43639=CARTESIAN_POINT('Ctrl Pts',(129.178199947378,31.7113262376537,26.6579652024416));
#43640=CARTESIAN_POINT('Ctrl Pts',(129.160711643262,31.71574582839,26.656887166339));
#43641=CARTESIAN_POINT('Ctrl Pts',(129.10877219126,31.7293137387408,26.6536575548113));
#43642=CARTESIAN_POINT('Ctrl Pts',(129.074430190552,31.7388658510306,26.6514854915809));
#43643=CARTESIAN_POINT('Ctrl Pts',(128.901591763817,31.7898901724134,26.6403893903998));
#43644=CARTESIAN_POINT('Ctrl Pts',(128.76570803256,31.8396483629176,26.6311344485386));
#43645=CARTESIAN_POINT('Ctrl Pts',(128.520060699034,31.947864531237,26.6138494102096));
#43646=CARTESIAN_POINT('Ctrl Pts',(128.409513671725,32.0039849627096,26.6058452079918));
#43647=CARTESIAN_POINT('Ctrl Pts',(128.210942693684,32.1188863209674,26.5912200509964));
#43648=CARTESIAN_POINT('Ctrl Pts',(128.122112945259,32.175980658667,26.5845767806013));
#43649=CARTESIAN_POINT('Ctrl Pts',(127.975712420424,32.2800456771507,26.5734949155237));
#43650=CARTESIAN_POINT('Ctrl Pts',(127.916758582053,32.3249302465901,26.5689919189262));
#43651=CARTESIAN_POINT('Ctrl Pts',(127.83290980495,32.3932232000597,26.5625252675083));
#43652=CARTESIAN_POINT('Ctrl Pts',(127.806825363361,32.4151304987645,26.5605042123048));
#43653=CARTESIAN_POINT('Ctrl Pts',(127.761008829871,32.4548029271644,26.556936207825));
#43654=CARTESIAN_POINT('Ctrl Pts',(127.741147217858,32.4724134500349,26.5553832081525));
#43655=CARTESIAN_POINT('Ctrl Pts',(127.699437805256,32.5102799165774,26.5521074612325));
#43656=CARTESIAN_POINT('Ctrl Pts',(127.677645973352,32.5305943301381,26.5503873280708));
#43657=CARTESIAN_POINT('Ctrl Pts',(127.619028944112,32.5866996423387,26.5457341222069));
#43658=CARTESIAN_POINT('Ctrl Pts',(127.582743943563,32.6230449453872,26.5428247744739));
#43659=CARTESIAN_POINT('Ctrl Pts',(127.375060425673,32.8407500318552,26.5259642020765));
#43660=CARTESIAN_POINT('Ctrl Pts',(127.223285073611,33.0397618764855,26.5128548293274));
#43661=CARTESIAN_POINT('Ctrl Pts',(127.033530045413,33.3554427869589,26.4932945514482));
#43662=CARTESIAN_POINT('Ctrl Pts',(126.977735037592,33.4603819487298,26.486954707205));
#43663=CARTESIAN_POINT('Ctrl Pts',(126.899623357417,33.6279778617142,26.4767708357208));
#43664=CARTESIAN_POINT('Ctrl Pts',(126.873443912479,33.6887311621582,26.4730672340935));
#43665=CARTESIAN_POINT('Ctrl Pts',(126.840668297963,33.7713640512458,26.4679648317604));
#43666=CARTESIAN_POINT('Ctrl Pts',(126.832490137436,33.7926043282475,26.4666476209584));
#43667=CARTESIAN_POINT('Ctrl Pts',(126.819150775209,33.8283177344914,26.4644208700565));
#43668=CARTESIAN_POINT('Ctrl Pts',(126.813872808196,33.8427469452109,26.4635179357086));
#43669=CARTESIAN_POINT('Ctrl Pts',(126.803120702062,33.8727728602793,26.4616313758305));
#43670=CARTESIAN_POINT('Ctrl Pts',(126.797662294472,33.8883744044702,26.4606469693287));
#43671=CARTESIAN_POINT('Ctrl Pts',(126.783160624375,33.9308172629002,26.4579589469619));
#43672=CARTESIAN_POINT('Ctrl Pts',(126.774339525068,33.957732433461,26.4562435270594));
#43673=CARTESIAN_POINT('Ctrl Pts',(126.720193774909,34.1302178169966,26.4451955018039));
#43674=CARTESIAN_POINT('Ctrl Pts',(126.684400452344,34.2785839766073,26.4354521072505));
#43675=CARTESIAN_POINT('Ctrl Pts',(126.626604614875,34.6166890551896,26.4133729314832));
#43676=CARTESIAN_POINT('Ctrl Pts',(126.610389780316,34.8069278845278,26.4010494746156));
#43677=CARTESIAN_POINT('Ctrl Pts',(126.610175022935,35.1016647330484,26.3825795547791));
#43678=CARTESIAN_POINT('Ctrl Pts',(126.614897715772,35.2057547114801,26.3761709170851));
#43679=CARTESIAN_POINT('Ctrl Pts',(126.62800535707,35.3487281028196,26.3675337610334));
#43680=CARTESIAN_POINT('Ctrl Pts',(126.63228909971,35.3879209332811,26.3651830153553));
#43681=CARTESIAN_POINT('Ctrl Pts',(126.64035998537,35.4514767387727,26.3613971096362));
#43682=CARTESIAN_POINT('Ctrl Pts',(126.643730796172,35.4758879624845,26.3599492528049));
#43683=CARTESIAN_POINT('Ctrl Pts',(126.651397953111,35.5272714839633,26.3569141535342));
#43684=CARTESIAN_POINT('Ctrl Pts',(126.65575469729,35.5542330785541,26.3553289021937));
#43685=CARTESIAN_POINT('Ctrl Pts',(126.667133689455,35.6196233185677,26.3515004563569));
#43686=CARTESIAN_POINT('Ctrl Pts',(126.674495371031,35.6579893932487,26.3492679709382));
#43687=CARTESIAN_POINT('Ctrl Pts',(126.705097587925,35.8038084756085,26.340826609284));
#43688=CARTESIAN_POINT('Ctrl Pts',(126.732897811005,35.9102397376974,26.3347591677512));
#43689=CARTESIAN_POINT('Ctrl Pts',(126.782934923845,36.0696551455584,26.3256969442815));
#43690=CARTESIAN_POINT('Ctrl Pts',(126.801414675095,36.1237064934745,26.322628320241));
#43691=CARTESIAN_POINT('Ctrl Pts',(126.821241849252,36.1772432550457,26.31957821124));
#43692=CARTESIAN_POINT('',(126.610250231881,35.0012538096501,26.7339821967504));
#43693=CARTESIAN_POINT('Ctrl Pts',(126.821241918426,36.1772434418289,26.660716603687));
#43694=CARTESIAN_POINT('Ctrl Pts',(126.799783544056,36.1193021711248,26.6645592714981));
#43695=CARTESIAN_POINT('Ctrl Pts',(126.779914062806,36.0607868592372,26.6684601693087));
#43696=CARTESIAN_POINT('Ctrl Pts',(126.717623530252,35.8594237440769,26.681883581533));
#43697=CARTESIAN_POINT('Ctrl Pts',(126.683024607012,35.7143375892325,26.6915468822929));
#43698=CARTESIAN_POINT('Ctrl Pts',(126.626333159024,35.380459596025,26.7132883205415));
#43699=CARTESIAN_POINT('Ctrl Pts',(126.610329828592,35.1911214548352,26.7252549797204));
#43700=CARTESIAN_POINT('Ctrl Pts',(126.6102502979,35.0014211316691,26.7367447340574));
#43701=CARTESIAN_POINT('Ctrl Pts',(126.610250231881,35.0012538096501,26.7339821967504));
#43702=CARTESIAN_POINT('Ctrl Pts',(126.610210918892,34.8949687788819,26.740189865272));
#43703=CARTESIAN_POINT('Ctrl Pts',(126.615174777716,34.7887128757728,26.7463975337937));
#43704=CARTESIAN_POINT('Ctrl Pts',(126.625107297087,34.6829758584513,26.7526052023153));
#43705=CARTESIAN_POINT('Ctrl Pts',(126.635045153883,34.5771820213633,26.7588162066439));
#43706=CARTESIAN_POINT('Ctrl Pts',(126.649956949819,34.4719080254279,26.7650272109724));
#43707=CARTESIAN_POINT('Ctrl Pts',(126.669756487626,34.367636804686,26.771238215301));
#43708=CARTESIAN_POINT('Ctrl Pts',(126.689810650005,34.2620246427923,26.7775290939347));
#43709=CARTESIAN_POINT('Ctrl Pts',(126.714879066246,34.1574416454979,26.7838199725683));
#43710=CARTESIAN_POINT('Ctrl Pts',(126.744819612016,34.0543754951455,26.790110851202));
#43711=CARTESIAN_POINT('Ctrl Pts',(126.774450142089,33.9523765305604,26.7963365917072));
#43712=CARTESIAN_POINT('Ctrl Pts',(126.808852175928,33.8518635051602,26.8025623322124));
#43713=CARTESIAN_POINT('Ctrl Pts',(126.847839093271,33.7532896565007,26.8087880727176));
#43714=CARTESIAN_POINT('Ctrl Pts',(126.887437873932,33.6531687831915,26.8151115204155));
#43715=CARTESIAN_POINT('Ctrl Pts',(126.931766482537,33.5550488623061,26.8214349681134));
#43716=CARTESIAN_POINT('Ctrl Pts',(126.980581021143,33.4593786666999,26.8277584158113));
#43717=CARTESIAN_POINT('Ctrl Pts',(127.029395559749,33.3637084710937,26.8340818635091));
#43718=CARTESIAN_POINT('Ctrl Pts',(127.082695759614,33.2704883394357,26.840405311207));
#43719=CARTESIAN_POINT('Ctrl Pts',(127.140192688397,33.1801353888262,26.8467287589049));
#43720=CARTESIAN_POINT('Ctrl Pts',(127.195672875846,33.0929516254072,26.8528304076542));
#43721=CARTESIAN_POINT('Ctrl Pts',(127.255237266495,33.0081598841338,26.8589320564036));
#43722=CARTESIAN_POINT('Ctrl Pts',(127.318653174024,32.9261667710911,26.8650337051529));
#43723=CARTESIAN_POINT('Ctrl Pts',(127.381985666382,32.8442815090561,26.8711273279969));
#43724=CARTESIAN_POINT('Ctrl Pts',(127.449159344413,32.7651878923461,26.8772209508408));
#43725=CARTESIAN_POINT('Ctrl Pts',(127.519897363508,32.689265057397,26.8833145736848));
#43726=CARTESIAN_POINT('Ctrl Pts',(127.590562576428,32.6134203650273,26.8894019247476));
#43727=CARTESIAN_POINT('Ctrl Pts',(127.66478454543,32.5407402762669,26.8954892758104));
#43728=CARTESIAN_POINT('Ctrl Pts',(127.742245693163,32.4715715251444,26.9015766268732));
#43729=CARTESIAN_POINT('Ctrl Pts',(127.819651737303,32.4024519786474,26.9076596475725));
#43730=CARTESIAN_POINT('Ctrl Pts',(127.900292059834,32.3368390866557,26.9137426682719));
#43731=CARTESIAN_POINT('Ctrl Pts',(127.983812297817,32.2750427137171,26.9198256889713));
#43732=CARTESIAN_POINT('Ctrl Pts',(128.067301613316,32.2132692202315,26.9259064574966));
#43733=CARTESIAN_POINT('Ctrl Pts',(128.153668381654,32.1553096916414,26.9319872260219));
#43734=CARTESIAN_POINT('Ctrl Pts',(128.242525864334,32.1014331601695,26.9380679945473));
#43735=CARTESIAN_POINT('Ctrl Pts',(128.331373469526,32.0475626176675,26.9441480871282));
#43736=CARTESIAN_POINT('Ctrl Pts',(128.422710872735,31.9977743915357,26.9502281797091));
#43737=CARTESIAN_POINT('Ctrl Pts',(128.51612389788,31.9522931938821,26.9563082722901));
#43738=CARTESIAN_POINT('Ctrl Pts',(128.609550740106,31.9068052689289,26.962389264201));
#43739=CARTESIAN_POINT('Ctrl Pts',(128.705053429597,31.8656258254152,26.9684702561119));
#43740=CARTESIAN_POINT('Ctrl Pts',(128.802195670932,31.8289323798183,26.9745512480228));
#43741=CARTESIAN_POINT('Ctrl Pts',(128.899438741757,31.7922008479942,26.9806385517432));
#43742=CARTESIAN_POINT('Ctrl Pts',(128.998324362099,31.7599647645011,26.9867258554636));
#43743=CARTESIAN_POINT('Ctrl Pts',(129.098398877822,31.7323524549017,26.992813159184));
#43744=CARTESIAN_POINT('Ctrl Pts',(129.198527160446,31.7047253100735,26.998903733422));
#43745=CARTESIAN_POINT('Ctrl Pts',(129.299845193589,31.681726982188,27.0049943076599));
#43746=CARTESIAN_POINT('Ctrl Pts',(129.401888827003,31.6634346871018,27.0110848818979));
#43747=CARTESIAN_POINT('Ctrl Pts',(129.504099053315,31.6451125286487,27.0171853993963));
#43748=CARTESIAN_POINT('Ctrl Pts',(129.607036821974,31.6315118072128,27.0232859168946));
#43749=CARTESIAN_POINT('Ctrl Pts',(129.710232315187,31.6226578865419,27.029386434393));
#43750=CARTESIAN_POINT('Ctrl Pts',(129.791551230574,31.6156809226893,27.0341936934198));
#43751=CARTESIAN_POINT('Ctrl Pts',(129.873030044137,31.6116504793404,27.0390009524466));
#43752=CARTESIAN_POINT('Ctrl Pts',(129.95444001818,31.610556188612,27.0438082114734));
#43753=CARTESIAN_POINT('Ctrl Pts',(130.057770259625,31.6091672516112,27.0499098623063));
#43754=CARTESIAN_POINT('Ctrl Pts',(130.161338693267,31.6125054473483,27.0560115131392));
#43755=CARTESIAN_POINT('Ctrl Pts',(130.264677695029,31.6205990500897,27.0621131639721));
#43756=CARTESIAN_POINT('Ctrl Pts',(130.367880768537,31.6286820068093,27.068206788922));
#43757=CARTESIAN_POINT('Ctrl Pts',(130.470854587276,31.6415079020645,27.0743004138719));
#43758=CARTESIAN_POINT('Ctrl Pts',(130.573130296056,31.6590530195404,27.0803940388219));
#43759=CARTESIAN_POINT('Ctrl Pts',(130.675300739269,31.6765800789967,27.0864813920099));
#43760=CARTESIAN_POINT('Ctrl Pts',(130.77677408194,31.6988166302027,27.092568745198));
#43761=CARTESIAN_POINT('Ctrl Pts',(130.877086241145,31.7256871273358,27.0986560983861));
#43762=CARTESIAN_POINT('Ctrl Pts',(130.977327041571,31.752538509679,27.1047391212308));
#43763=CARTESIAN_POINT('Ctrl Pts',(131.076407889174,31.7840171723514,27.1108221440756));
#43764=CARTESIAN_POINT('Ctrl Pts',(131.173875373105,31.8199965926247,27.1169051669204));
#43765=CARTESIAN_POINT('Ctrl Pts',(131.271306770929,31.8559626919715,27.1229859376027));
#43766=CARTESIAN_POINT('Ctrl Pts',(131.367125591384,31.8964260891807,27.1290667082849));
#43767=CARTESIAN_POINT('Ctrl Pts',(131.460894827519,31.9412108007533,27.1351474789672));
#43768=CARTESIAN_POINT('Ctrl Pts',(131.554653640311,31.985990534079,27.141227573714));
#43769=CARTESIAN_POINT('Ctrl Pts',(131.646362935839,32.035090442233,27.1473076684607));
#43770=CARTESIAN_POINT('Ctrl Pts',(131.735607734947,32.0882872990467,27.1533877632075));
#43771=CARTESIAN_POINT('Ctrl Pts',(131.824865734684,32.1414920244646,27.1594687572904));
#43772=CARTESIAN_POINT('Ctrl Pts',(131.911658146298,32.1987946834705,27.1655497513734));
#43773=CARTESIAN_POINT('Ctrl Pts',(131.995597338689,32.2599276789989,27.1716307454564));
#43774=CARTESIAN_POINT('Ctrl Pts',(132.079623656287,32.3211241279004,27.177718051345));
#43775=CARTESIAN_POINT('Ctrl Pts',(132.160790493824,32.3861586008612,27.1838053572336));
#43776=CARTESIAN_POINT('Ctrl Pts',(132.238741846655,32.4547220178269,27.1898926631222));
#43777=CARTESIAN_POINT('Ctrl Pts',(132.316735080305,32.5233222717677,27.1959832395295));
#43778=CARTESIAN_POINT('Ctrl Pts',(132.39150908014,32.5954549493437,27.2020738159367));
#43779=CARTESIAN_POINT('Ctrl Pts',(132.462744834613,32.6707741753775,27.208164392344));
#43780=CARTESIAN_POINT('Ctrl Pts',(132.534096885825,32.7462163646678,27.2142649119909));
#43781=CARTESIAN_POINT('Ctrl Pts',(132.601898872626,32.824855170724,27.2203654316377));
#43782=CARTESIAN_POINT('Ctrl Pts',(132.665872044335,32.90631155476,27.2264659512846));
#43783=CARTESIAN_POINT('Ctrl Pts',(132.716283198355,32.9704995606356,27.2312731888703));
#43784=CARTESIAN_POINT('Ctrl Pts',(132.764317638959,33.0364364599261,27.2360804264561));
#43785=CARTESIAN_POINT('Ctrl Pts',(132.809858653429,33.1039252624829,27.2408876640418));
#43786=CARTESIAN_POINT('Ctrl Pts',(132.86766209271,33.1895861759738,27.2469893038304));
#43787=CARTESIAN_POINT('Ctrl Pts',(132.921642478837,33.2780375419525,27.253090943619));
#43788=CARTESIAN_POINT('Ctrl Pts',(132.971519829651,33.3689037537619,27.2591925834075));
#43789=CARTESIAN_POINT('Ctrl Pts',(133.021331573391,33.4596504430609,27.2652861972941));
#43790=CARTESIAN_POINT('Ctrl Pts',(133.067050807172,33.5528052915461,27.2713798111808));
#43791=CARTESIAN_POINT('Ctrl Pts',(133.10844035734,33.6479631634594,27.2774734250674));
#43792=CARTESIAN_POINT('Ctrl Pts',(133.149787307896,33.7430230954735,27.2835607671878));
#43793=CARTESIAN_POINT('Ctrl Pts',(133.186813266437,33.8400815612675,27.2896481093081));
#43794=CARTESIAN_POINT('Ctrl Pts',(133.219327023952,33.9387090053368,27.2957354514285));
#43795=CARTESIAN_POINT('Ctrl Pts',(133.251817652411,34.0372662895778,27.3018184632442));
#43796=CARTESIAN_POINT('Ctrl Pts',(133.279802329281,34.1373899275475,27.30790147506));
#43797=CARTESIAN_POINT('Ctrl Pts',(133.303138331179,34.2386313458034,27.3139844868757));
#43798=CARTESIAN_POINT('Ctrl Pts',(133.326465693307,34.3398352810896,27.3200652465564));
#43799=CARTESIAN_POINT('Ctrl Pts',(133.345147705063,34.4421557578086,27.326146006237));
#43800=CARTESIAN_POINT('Ctrl Pts',(133.359092002632,34.5451308096242,27.3322267659177));
#43801=CARTESIAN_POINT('Ctrl Pts',(133.37303475025,34.6480944154463,27.3383068497033));
#43802=CARTESIAN_POINT('Ctrl Pts',(133.38224077345,34.7517120278049,27.3443869334888));
#43803=CARTESIAN_POINT('Ctrl Pts',(133.386669295655,34.8555142070427,27.3504670172744));
#43804=CARTESIAN_POINT('Ctrl Pts',(133.391098472945,34.959331741101,27.3565480004494));
#43805=CARTESIAN_POINT('Ctrl Pts',(133.390748726961,35.063333468874,27.3626289836245));
#43806=CARTESIAN_POINT('Ctrl Pts',(133.385631382875,35.1670485013206,27.3687099667996));
#43807=CARTESIAN_POINT('Ctrl Pts',(133.380508727074,35.2708711881793,27.3747972619302));
#43808=CARTESIAN_POINT('Ctrl Pts',(133.370608611354,35.3744061573462,27.3808845570608));
#43809=CARTESIAN_POINT('Ctrl Pts',(133.355994392532,35.4771862317753,27.3869718521914));
#43810=CARTESIAN_POINT('Ctrl Pts',(133.341372321774,35.5800215279423,27.3930624179074));
#43811=CARTESIAN_POINT('Ctrl Pts',(133.322031182432,35.6821007011185,27.3991529836234));
#43812=CARTESIAN_POINT('Ctrl Pts',(133.298085383964,35.7829673445205,27.4052435493394));
#43813=CARTESIAN_POINT('Ctrl Pts',(133.274100491576,35.8839986628428,27.4113440585154));
#43814=CARTESIAN_POINT('Ctrl Pts',(133.245496040138,35.9838130852854,27.4174445676913));
#43815=CARTESIAN_POINT('Ctrl Pts',(133.212436245724,36.0819696990494,27.4235450768672));
#43816=CARTESIAN_POINT('Ctrl Pts',(133.186384340044,36.1593194493689,27.4283524234482));
#43817=CARTESIAN_POINT('Ctrl Pts',(133.157566756941,36.2356400196643,27.4331597700292));
#43818=CARTESIAN_POINT('Ctrl Pts',(133.126084283164,36.310725797813,27.4379671166102));
#43819=CARTESIAN_POINT('Ctrl Pts',(133.086125603402,36.4060273482895,27.4440687725315));
#43820=CARTESIAN_POINT('Ctrl Pts',(133.041737391433,36.499661019544,27.4501704284528));
#43821=CARTESIAN_POINT('Ctrl Pts',(132.993080319361,36.5911867471649,27.4562720843741));
#43822=CARTESIAN_POINT('Ctrl Pts',(132.944487249499,36.682592084295,27.4623657143406));
#43823=CARTESIAN_POINT('Ctrl Pts',(132.891636681759,36.7718946155797,27.4684593443072));
#43824=CARTESIAN_POINT('Ctrl Pts',(132.834737451556,36.8586738937331,27.4745529742737));
#43825=CARTESIAN_POINT('Ctrl Pts',(132.77789678461,36.9453638547353,27.4806403324011));
#43826=CARTESIAN_POINT('Ctrl Pts',(132.717015974739,37.0295353710263,27.4867276905286));
#43827=CARTESIAN_POINT('Ctrl Pts',(132.652349477433,37.1107930528741,27.492815048656));
#43828=CARTESIAN_POINT('Ctrl Pts',(132.587728983149,37.1919929289171,27.498898076305));
#43829=CARTESIAN_POINT('Ctrl Pts',(132.519328422461,37.2702827588664,27.5049811039541));
#43830=CARTESIAN_POINT('Ctrl Pts',(132.44744473493,37.3452972800827,27.5110641316031));
#43831=CARTESIAN_POINT('Ctrl Pts',(132.375587662402,37.4202840271022,27.5171449070055));
#43832=CARTESIAN_POINT('Ctrl Pts',(132.300250321725,37.4919975670229,27.5232256824078));
#43833=CARTESIAN_POINT('Ctrl Pts',(132.221768459159,37.5601074150091,27.5293064578102));
#43834=CARTESIAN_POINT('Ctrl Pts',(132.143295321744,37.6282096909439,27.5353865571877));
#43835=CARTESIAN_POINT('Ctrl Pts',(132.061678680655,37.6927087912504,27.5414666565653));
#43836=CARTESIAN_POINT('Ctrl Pts',(131.977288810877,37.7533132805549,27.5475467559429));
#43837=CARTESIAN_POINT('Ctrl Pts',(131.892886459905,37.8139267332147,27.5536277545623));
#43838=CARTESIAN_POINT('Ctrl Pts',(131.805710412839,37.8706441809512,27.5597087531817));
#43839=CARTESIAN_POINT('Ctrl Pts',(131.716160717207,37.9232169702598,27.5657897518011));
#43840=CARTESIAN_POINT('Ctrl Pts',(131.626518075536,37.9758443262817,27.5718770620526));
#43841=CARTESIAN_POINT('Ctrl Pts',(131.534497234732,38.0243182157326,27.5779643723042));
#43842=CARTESIAN_POINT('Ctrl Pts',(131.440523659614,38.0684355376302,27.5840516825558));
#43843=CARTESIAN_POINT('Ctrl Pts',(131.346499596856,38.1125765617171,27.5901422632366));
#43844=CARTESIAN_POINT('Ctrl Pts',(131.250521105259,38.1523561921926,27.5962328439174));
#43845=CARTESIAN_POINT('Ctrl Pts',(131.153032627016,38.1876199308476,27.6023234245982));
#43846=CARTESIAN_POINT('Ctrl Pts',(131.055384996012,38.222941238576,27.6084239483281));
#43847=CARTESIAN_POINT('Ctrl Pts',(130.956222862647,38.2537317998478,27.614524472058));
#43848=CARTESIAN_POINT('Ctrl Pts',(130.856005012664,38.2798872664763,27.620624995788));
#43849=CARTESIAN_POINT('Ctrl Pts',(130.777033701207,38.3004976817045,27.6254321869182));
#43850=CARTESIAN_POINT('Ctrl Pts',(130.697407166111,38.3182309901524,27.6302393780484));
#43851=CARTESIAN_POINT('Ctrl Pts',(130.617352600307,38.3330587797688,27.6350465691787));
#43852=CARTESIAN_POINT('Ctrl Pts',(130.515741023488,38.3518793812989,27.6411482357845));
#43853=CARTESIAN_POINT('Ctrl Pts',(130.413096307233,38.3660809580804,27.6472499023904));
#43854=CARTESIAN_POINT('Ctrl Pts',(130.309874585369,38.3755566657727,27.6533515689962));
#43855=CARTESIAN_POINT('Ctrl Pts',(130.206788634955,38.3850199097069,27.6594452098483));
#43856=CARTESIAN_POINT('Ctrl Pts',(130.103127610138,38.3897696036588,27.6655388507005));
#43857=CARTESIAN_POINT('Ctrl Pts',(129.999357638686,38.3897499391359,27.6716324915526));
#43858=CARTESIAN_POINT('Ctrl Pts',(129.895694468648,38.389730294852,27.6777198607497));
#43859=CARTESIAN_POINT('Ctrl Pts',(129.791923000431,38.3849510531249,27.6838072299467));
#43860=CARTESIAN_POINT('Ctrl Pts',(129.688513411436,38.3754082964354,27.6898945991438));
#43861=CARTESIAN_POINT('Ctrl Pts',(129.585177382847,38.3658723279853,27.6959776380911));
#43862=CARTESIAN_POINT('Ctrl Pts',(129.482203146275,38.3515796221331,27.7020606770384));
#43863=CARTESIAN_POINT('Ctrl Pts',(129.380058969734,38.3325783083813,27.7081437159857));
#43864=CARTESIAN_POINT('Ctrl Pts',(129.277952609821,38.3135840294466,27.7142245028221));
#43865=CARTESIAN_POINT('Ctrl Pts',(129.176676119256,38.2898846853788,27.7203052896585));
#43866=CARTESIAN_POINT('Ctrl Pts',(129.076689951158,38.2615799263866,27.7263860764948));
#43867=CARTESIAN_POINT('Ctrl Pts',(128.976714896919,38.2332783135805,27.7324661874277));
#43868=CARTESIAN_POINT('Ctrl Pts',(128.878030291518,38.2003724202943,27.7385462983605));
#43869=CARTESIAN_POINT('Ctrl Pts',(128.781082855486,38.1630121810245,27.7446264092933));
#43870=CARTESIAN_POINT('Ctrl Pts',(128.684121079331,38.1256464155598,27.7507074195747));
#43871=CARTESIAN_POINT('Ctrl Pts',(128.588897382226,38.0838251489321,27.7567884298561));
#43872=CARTESIAN_POINT('Ctrl Pts',(128.495839023297,38.0377466679536,27.7628694401375));
#43873=CARTESIAN_POINT('Ctrl Pts',(128.402684075371,37.9916203602747,27.768956762143));
#43874=CARTESIAN_POINT('Ctrl Pts',(128.311699338125,37.9412282038409,27.7750440841484));
#43875=CARTESIAN_POINT('Ctrl Pts',(128.223287904622,37.8868147139431,27.7811314061539));
#43876=CARTESIAN_POINT('Ctrl Pts',(128.134828970858,37.8323719896477,27.787221998657));
#43877=CARTESIAN_POINT('Ctrl Pts',(128.048946448402,37.7739038690723,27.7933125911601));
#43878=CARTESIAN_POINT('Ctrl Pts',(127.966013183012,37.7116973818659,27.7994031836632));
#43879=CARTESIAN_POINT('Ctrl Pts',(127.882944527085,37.6493893410834,27.805503719204));
#43880=CARTESIAN_POINT('Ctrl Pts',(127.802835076882,37.5833310140908,27.8116042547449));
#43881=CARTESIAN_POINT('Ctrl Pts',(127.726023596702,37.5138489174461,27.8177047902857));
#43882=CARTESIAN_POINT('Ctrl Pts',(127.665497974148,37.4590986750873,27.8225118674395));
#43883=CARTESIAN_POINT('Ctrl Pts',(127.60701941582,37.4022234011004,27.8273189445933));
#43884=CARTESIAN_POINT('Ctrl Pts',(127.550736212838,37.3433975256871,27.8321260217471));
#43885=CARTESIAN_POINT('Ctrl Pts',(127.480210871469,37.2696861033617,27.8381495019205));
#43886=CARTESIAN_POINT('Ctrl Pts',(127.412881596586,37.1926473030203,27.8441729820939));
#43887=CARTESIAN_POINT('Ctrl Pts',(127.349084150531,37.1125932456429,27.8501964622673));
#43888=CARTESIAN_POINT('Ctrl Pts',(127.285385720088,37.0326634346403,27.8562105938131));
#43889=CARTESIAN_POINT('Ctrl Pts',(127.225208489255,36.9497280139285,27.8622247253588));
#43890=CARTESIAN_POINT('Ctrl Pts',(127.168851230835,36.8641356467162,27.8682388569045));
#43891=CARTESIAN_POINT('Ctrl Pts',(127.112544511846,36.7786200360664,27.8742475951649));
#43892=CARTESIAN_POINT('Ctrl Pts',(127.060051203334,36.6904525754194,27.8802563334252));
#43893=CARTESIAN_POINT('Ctrl Pts',(127.011629290659,36.6000142393288,27.8862650716856));
#43894=CARTESIAN_POINT('Ctrl Pts',(126.963239521667,36.5096359384768,27.8922698211946));
#43895=CARTESIAN_POINT('Ctrl Pts',(126.918915984628,36.4169901445685,27.8982745707036));
#43896=CARTESIAN_POINT('Ctrl Pts',(126.878872253773,36.3224850298713,27.9042793202126));
#43897=CARTESIAN_POINT('Ctrl Pts',(126.858553141375,36.2745309554951,27.907326268576));
#43898=CARTESIAN_POINT('Ctrl Pts',(126.839335262965,36.2260985580622,27.9103732169395));
#43899=CARTESIAN_POINT('Ctrl Pts',(126.821241918358,36.1772434416438,27.913420165303));
#43900=CARTESIAN_POINT('Origin',(130.,35.,23.));
#43901=CARTESIAN_POINT('',(126.821241934448,36.17724348509,29.1634527466974));
#43902=CARTESIAN_POINT('',(126.821241918358,36.1772434416436,28.8235740826546));
#43903=CARTESIAN_POINT('',(126.821241918358,36.1772434416438,23.));
#43904=CARTESIAN_POINT('',(132.573234427015,37.2065515280923,30.));
#43905=CARTESIAN_POINT('Ctrl Pts',(132.573234427015,37.2065515280921,29.9999999999999));
#43906=CARTESIAN_POINT('Ctrl Pts',(132.579543502806,37.1991940153298,29.999431170887));
#43907=CARTESIAN_POINT('Ctrl Pts',(132.585821065603,37.1918093942846,29.9988641961783));
#43908=CARTESIAN_POINT('Ctrl Pts',(132.599714029705,37.1753236187309,29.9976069824885));
#43909=CARTESIAN_POINT('Ctrl Pts',(132.60731351268,37.166209162608,29.9969176352125));
#43910=CARTESIAN_POINT('Ctrl Pts',(132.636602405948,37.1307040370924,29.9942536828936));
#43911=CARTESIAN_POINT('Ctrl Pts',(132.657940874235,37.1040252846207,29.9922974533084));
#43912=CARTESIAN_POINT('Ctrl Pts',(132.773829252144,36.9545567649187,29.9815615504326));
#43913=CARTESIAN_POINT('Ctrl Pts',(132.860282271052,36.8257089538147,29.9731252601069));
#43914=CARTESIAN_POINT('Ctrl Pts',(133.018347198056,36.5511804425255,29.9559328731301));
#43915=CARTESIAN_POINT('Ctrl Pts',(133.088931743976,36.405374905407,29.9471969570919));
#43916=CARTESIAN_POINT('Ctrl Pts',(133.170151634526,36.2016068031044,29.9350254270888));
#43917=CARTESIAN_POINT('Ctrl Pts',(133.190103632595,36.147588212588,29.9318033302057));
#43918=CARTESIAN_POINT('Ctrl Pts',(133.224142504401,36.0476700300939,29.9258303603832));
#43919=CARTESIAN_POINT('Ctrl Pts',(133.238648741697,36.001928852775,29.9230911528992));
#43920=CARTESIAN_POINT('Ctrl Pts',(133.260934604744,35.9261072468255,29.9185337556719));
#43921=CARTESIAN_POINT('Ctrl Pts',(133.26928051528,35.896199730786,29.9167318836821));
#43922=CARTESIAN_POINT('Ctrl Pts',(133.284811176684,35.8374392397412,29.9131811344762));
#43923=CARTESIAN_POINT('Ctrl Pts',(133.292029485041,35.8085980084427,29.9114334138339));
#43924=CARTESIAN_POINT('Ctrl Pts',(133.307087210171,35.7448868470315,29.9075600154555));
#43925=CARTESIAN_POINT('Ctrl Pts',(133.314756329506,35.709980682258,29.905429579274));
#43926=CARTESIAN_POINT('Ctrl Pts',(133.335889145256,35.6059738755283,29.8990540301905));
#43927=CARTESIAN_POINT('Ctrl Pts',(133.347753148856,35.5365710943665,29.8947632501768));
#43928=CARTESIAN_POINT('Ctrl Pts',(133.393624784718,35.2066777904556,29.8741797628565));
#43929=CARTESIAN_POINT('Ctrl Pts',(133.399432763104,34.9432083554542,29.8570994967609));
#43930=CARTESIAN_POINT('Ctrl Pts',(133.364495018107,34.5727113607211,29.8329906909243));
#43931=CARTESIAN_POINT('Ctrl Pts',(133.348931797021,34.464219511136,29.8259340540569));
#43932=CARTESIAN_POINT('Ctrl Pts',(133.316043421954,34.2940788387603,29.8150230129187));
#43933=CARTESIAN_POINT('Ctrl Pts',(133.302181190938,34.2318404201251,29.8110657881638));
#43934=CARTESIAN_POINT('Ctrl Pts',(133.281033934727,34.1481004927447,29.8058179643617));
#43935=CARTESIAN_POINT('Ctrl Pts',(133.275277526079,34.126230213497,29.8044545666945));
#43936=CARTESIAN_POINT('Ctrl Pts',(133.265239119605,34.0895852082588,29.8021839383872));
#43937=CARTESIAN_POINT('Ctrl Pts',(133.261074734494,34.0747793786584,29.8012703447512));
#43938=CARTESIAN_POINT('Ctrl Pts',(133.252321869158,34.0444533368971,29.7994076076095));
#43939=CARTESIAN_POINT('Ctrl Pts',(133.247722751505,34.0289367111117,29.7984591779236));
#43940=CARTESIAN_POINT('Ctrl Pts',(133.234924289306,33.9868651321377,29.7958987887815));
#43941=CARTESIAN_POINT('Ctrl Pts',(133.226509004075,33.9603764271592,29.7942988807161));
#43942=CARTESIAN_POINT('Ctrl Pts',(133.171839494331,33.7953551080938,29.7843900347279));
#43943=CARTESIAN_POINT('Ctrl Pts',(133.116993251934,33.6598144652685,29.7765061627368));
#43944=CARTESIAN_POINT('Ctrl Pts',(132.944979851788,33.3029298753189,29.7553956919803));
#43945=CARTESIAN_POINT('Ctrl Pts',(132.8118011791,33.090360633968,29.7423721876542));
#43946=CARTESIAN_POINT('Ctrl Pts',(132.61715667909,32.8447974239,29.7249895683762));
#43947=CARTESIAN_POINT('Ctrl Pts',(132.576481306061,32.7963324679505,29.7214339043033));
#43948=CARTESIAN_POINT('Ctrl Pts',(132.5136286147,32.7255634100047,29.7160314421877));
#43949=CARTESIAN_POINT('Ctrl Pts',(132.492457221272,32.702382208203,29.7142263747315));
#43950=CARTESIAN_POINT('Ctrl Pts',(132.453571716938,32.6609752824088,29.7109350850109));
#43951=CARTESIAN_POINT('Ctrl Pts',(132.435968644666,32.6426482001669,29.7094537467989));
#43952=CARTESIAN_POINT('Ctrl Pts',(132.397479758546,32.6034677445963,29.7062321106564));
#43953=CARTESIAN_POINT('Ctrl Pts',(132.376524444496,32.582685886613,29.7044887499999));
#43954=CARTESIAN_POINT('Ctrl Pts',(132.317919073489,32.5260642611729,29.699640583135));
#43955=CARTESIAN_POINT('Ctrl Pts',(132.27971316248,32.4908140165465,29.6965103205222));
#43956=CARTESIAN_POINT('Ctrl Pts',(132.016355063005,32.2588107922306,29.6751229616274));
#43957=CARTESIAN_POINT('Ctrl Pts',(131.766862907665,32.0917469731511,29.6556014388477));
#43958=CARTESIAN_POINT('Ctrl Pts',(131.382402485095,31.9022262470931,29.6278695643384));
#43959=CARTESIAN_POINT('Ctrl Pts',(131.262819949973,31.8515828266004,29.6195591923214));
#43960=CARTESIAN_POINT('Ctrl Pts',(131.108994411807,31.7966167501559,29.6094932214696));
#43961=CARTESIAN_POINT('Ctrl Pts',(131.077202575661,31.7857866191262,29.6074455889445));
#43962=CARTESIAN_POINT('Ctrl Pts',(131.029020014237,31.7701681009778,29.6043970460613));
#43963=CARTESIAN_POINT('Ctrl Pts',(131.012746418862,31.7650284381931,29.6033767382018));
#43964=CARTESIAN_POINT('Ctrl Pts',(130.982367034029,31.7556854841539,29.6014903155602));
#43965=CARTESIAN_POINT('Ctrl Pts',(130.968271440575,31.7514507694914,29.6006223258154));
#43966=CARTESIAN_POINT('Ctrl Pts',(130.935695117675,31.7418947937145,29.5986321345464));
#43967=CARTESIAN_POINT('Ctrl Pts',(130.917195616119,31.7366386764378,29.5975136270731));
#43968=CARTESIAN_POINT('Ctrl Pts',(130.856792604257,31.7200310738578,29.593896562386));
#43969=CARTESIAN_POINT('Ctrl Pts',(130.814714011916,31.7093266393166,29.5914314007824));
#43970=CARTESIAN_POINT('Ctrl Pts',(130.564651183838,31.6508038505701,29.5770410367168));
#43971=CARTESIAN_POINT('Ctrl Pts',(130.352714136749,31.6219004168492,29.5658760995767));
#43972=CARTESIAN_POINT('Ctrl Pts',(129.973225695019,31.6062755965984,29.5457252523382));
#43973=CARTESIAN_POINT('Ctrl Pts',(129.806733774014,31.6116782805812,29.5368323813005));
#43974=CARTESIAN_POINT('Ctrl Pts',(129.577290737996,31.6360932864945,29.524020356432));
#43975=CARTESIAN_POINT('Ctrl Pts',(129.51346969133,31.6447296648041,29.5203980037632));
#43976=CARTESIAN_POINT('Ctrl Pts',(129.417834692579,31.6604570704717,29.5148625070593));
#43977=CARTESIAN_POINT('Ctrl Pts',(129.38581191603,31.6661979188677,29.5129907465977));
#43978=CARTESIAN_POINT('Ctrl Pts',(129.330246921808,31.6769870096695,29.5097090662008));
#43979=CARTESIAN_POINT('Ctrl Pts',(129.306666354747,31.681826868247,29.5083057153445));
#43980=CARTESIAN_POINT('Ctrl Pts',(129.253415977728,31.6933487896156,29.5051115664288));
#43981=CARTESIAN_POINT('Ctrl Pts',(129.223780830528,31.7001797562397,29.5033162244936));
#43982=CARTESIAN_POINT('Ctrl Pts',(129.143587570761,31.7198045211257,29.4984082845861));
#43983=CARTESIAN_POINT('Ctrl Pts',(129.093227870037,31.7333674084522,29.4952720645511));
#43984=CARTESIAN_POINT('Ctrl Pts',(128.832936408414,31.8099518695685,29.4787729543286));
#43985=CARTESIAN_POINT('Ctrl Pts',(128.629193389014,31.89205713254,29.4648217502512));
#43986=CARTESIAN_POINT('Ctrl Pts',(128.318101573545,32.0539959479666,29.4422922916578));
#43987=CARTESIAN_POINT('Ctrl Pts',(128.205008187947,32.1215057671064,29.4338247481737));
#43988=CARTESIAN_POINT('Ctrl Pts',(128.038062758905,32.2348360296538,29.4211366806577));
#43989=CARTESIAN_POINT('Ctrl Pts',(127.981236338199,32.2760462332199,29.4167826496236));
#43990=CARTESIAN_POINT('Ctrl Pts',(127.907173516086,32.3333480456181,29.4111016653535));
#43991=CARTESIAN_POINT('Ctrl Pts',(127.888769205194,32.3478951878976,29.4096894529985));
#43992=CARTESIAN_POINT('Ctrl Pts',(127.858313202438,32.3724862045089,29.4073536973156));
#43993=CARTESIAN_POINT('Ctrl Pts',(127.846177734222,32.3824246407634,29.4064233263937));
#43994=CARTESIAN_POINT('Ctrl Pts',(127.821321495395,32.4030707606196,29.4045191623325));
#43995=CARTESIAN_POINT('Ctrl Pts',(127.808609715539,32.4137884566159,29.4035460945967));
#43996=CARTESIAN_POINT('Ctrl Pts',(127.774413908781,32.4430531646311,29.4009288994761));
#43997=CARTESIAN_POINT('Ctrl Pts',(127.753082663019,32.4617775590151,29.3992967791197));
#43998=CARTESIAN_POINT('Ctrl Pts',(127.627027030361,32.575262808709,29.3896373875369));
#43999=CARTESIAN_POINT('Ctrl Pts',(127.528062719975,32.6762346833468,29.3819902458382));
#44000=CARTESIAN_POINT('Ctrl Pts',(127.306067691046,32.9330191558556,29.3638553958639));
#44001=CARTESIAN_POINT('Ctrl Pts',(127.189856811042,33.094015857445,29.35348307448));
#44002=CARTESIAN_POINT('Ctrl Pts',(127.050934312555,33.3270495162919,29.3387478273863));
#44003=CARTESIAN_POINT('Ctrl Pts',(127.015535652641,33.3910489645016,29.3347302675267));
#44004=CARTESIAN_POINT('Ctrl Pts',(126.956287582004,33.5068604929344,29.3274676792414));
#44005=CARTESIAN_POINT('Ctrl Pts',(126.931623655667,33.5582243718561,29.3242492696531));
#44006=CARTESIAN_POINT('Ctrl Pts',(126.895545594211,33.6384822601704,29.3192112457515));
#44007=CARTESIAN_POINT('Ctrl Pts',(126.883213953513,33.6669537283064,29.3174223195902));
#44008=CARTESIAN_POINT('Ctrl Pts',(126.861052524359,33.7201095638191,29.3140773917719));
#44009=CARTESIAN_POINT('Ctrl Pts',(126.851118702481,33.7447481135677,29.3125249957522));
#44010=CARTESIAN_POINT('Ctrl Pts',(126.829609147711,33.7999601996466,29.3090407659347));
#44011=CARTESIAN_POINT('Ctrl Pts',(126.818184154466,33.8305892543389,29.3071041588329));
#44012=CARTESIAN_POINT('Ctrl Pts',(126.785147744064,33.923226239808,29.3012338234429));
#44013=CARTESIAN_POINT('Ctrl Pts',(126.764894271259,33.985698863947,29.2972571783176));
#44014=CARTESIAN_POINT('Ctrl Pts',(126.661228848593,34.3402503030917,29.274580814602));
#44015=CARTESIAN_POINT('Ctrl Pts',(126.615569582305,34.6418953961436,29.2547104726883));
#44016=CARTESIAN_POINT('Ctrl Pts',(126.60958560063,35.0140739890281,29.230981199355));
#44017=CARTESIAN_POINT('Ctrl Pts',(126.610564120949,35.0826634886745,29.2266490881475));
#44018=CARTESIAN_POINT('Ctrl Pts',(126.615680867445,35.1972773075019,29.2195242613778));
#44019=CARTESIAN_POINT('Ctrl Pts',(126.618680020258,35.2433309753297,29.2166924126869));
#44020=CARTESIAN_POINT('Ctrl Pts',(126.624323894424,35.3092167976886,29.2126986865175));
#44021=CARTESIAN_POINT('Ctrl Pts',(126.62620501545,35.3291073421322,29.2115005575774));
#44022=CARTESIAN_POINT('Ctrl Pts',(126.629803075381,35.3638706358091,29.209421125578));
#44023=CARTESIAN_POINT('Ctrl Pts',(126.631442850777,35.3787504627889,29.2085357966238));
#44024=CARTESIAN_POINT('Ctrl Pts',(126.635258912827,35.411391072945,29.2066044350555));
#44025=CARTESIAN_POINT('Ctrl Pts',(126.63747730604,35.4291460850888,29.2055606746302));
#44026=CARTESIAN_POINT('Ctrl Pts',(126.644464772336,35.4816856185259,29.2024900568527));
#44027=CARTESIAN_POINT('Ctrl Pts',(126.649633917006,35.5164155420274,29.2004837357089));
#44028=CARTESIAN_POINT('Ctrl Pts',(126.68544509628,35.7337713432637,29.188039763442));
#44029=CARTESIAN_POINT('Ctrl Pts',(126.730472684173,35.9137287668374,29.1782253639928));
#44030=CARTESIAN_POINT('Ctrl Pts',(126.799998047657,36.1186440237703,29.1667563461289));
#44031=CARTESIAN_POINT('Ctrl Pts',(126.810419332266,36.148020614536,29.165105224614));
#44032=CARTESIAN_POINT('Ctrl Pts',(126.821241934448,36.17724348509,29.1634527466974));
#44033=CARTESIAN_POINT('',(127.462900812983,37.2480064007332,30.));
#44034=CARTESIAN_POINT('Origin',(130.,35.,30.));
#44035=CARTESIAN_POINT('Ctrl Pts',(127.462900812983,37.2480064007329,29.9999999999999));
#44036=CARTESIAN_POINT('Ctrl Pts',(127.478117849802,37.2651803428221,29.9985918573257));
#44037=CARTESIAN_POINT('Ctrl Pts',(127.493508854484,37.2821993118563,29.9971740439912));
#44038=CARTESIAN_POINT('Ctrl Pts',(127.658101727054,37.4605282678587,29.9820908018274));
#44039=CARTESIAN_POINT('Ctrl Pts',(127.822472262042,37.6071160583103,29.9677449542209));
#44040=CARTESIAN_POINT('Ctrl Pts',(128.101798222967,37.8112586652844,29.9455445514229));
#44041=CARTESIAN_POINT('Ctrl Pts',(128.207820718677,37.8800075148949,29.937532612846));
#44042=CARTESIAN_POINT('Ctrl Pts',(128.390146127328,37.9842570301074,29.9245087482649));
#44043=CARTESIAN_POINT('Ctrl Pts',(128.464372478913,38.0231224647332,29.9193981623304));
#44044=CARTESIAN_POINT('Ctrl Pts',(128.572286864749,38.0746256244688,29.9122349161533));
#44045=CARTESIAN_POINT('Ctrl Pts',(128.604849527171,38.0895376404814,29.9101068158507));
#44046=CARTESIAN_POINT('Ctrl Pts',(128.662342021915,38.1147718598676,29.9064061054776));
#44047=CARTESIAN_POINT('Ctrl Pts',(128.6871697164,38.1253174740691,29.9048261741106));
#44048=CARTESIAN_POINT('Ctrl Pts',(128.739289134993,38.1467246134861,29.901546238517));
#44049=CARTESIAN_POINT('Ctrl Pts',(128.766601553822,38.1575300519343,29.8998481808724));
#44050=CARTESIAN_POINT('Ctrl Pts',(128.839348796321,38.1852225998621,29.8953777787254));
#44051=CARTESIAN_POINT('Ctrl Pts',(128.88501206646,38.2014928486645,29.8926253785995));
#44052=CARTESIAN_POINT('Ctrl Pts',(129.181085841966,38.2998831524024,29.8750894211646));
#44053=CARTESIAN_POINT('Ctrl Pts',(129.439994122515,38.3535432528616,29.8612585804505));
#44054=CARTESIAN_POINT('Ctrl Pts',(129.844770929947,38.3892037207016,29.8395615335009));
#44055=CARTESIAN_POINT('Ctrl Pts',(129.987661194082,38.3927331741491,29.8318668538269));
#44056=CARTESIAN_POINT('Ctrl Pts',(130.166121615511,38.3858664096661,29.8217768437165));
#44057=CARTESIAN_POINT('Ctrl Pts',(130.201884035525,38.3839223339755,29.8197304548625));
#44058=CARTESIAN_POINT('Ctrl Pts',(130.25582799341,38.380131761888,29.8165979455674));
#44059=CARTESIAN_POINT('Ctrl Pts',(130.274037449334,38.3787042093047,29.8155326381145));
#44060=CARTESIAN_POINT('Ctrl Pts',(130.307341319321,38.3758223168553,29.8135683816065));
#44061=CARTESIAN_POINT('Ctrl Pts',(130.322438762146,38.3744137598175,29.8126718443432));
#44062=CARTESIAN_POINT('Ctrl Pts',(130.357305303917,38.370924666362,29.8105872841581));
#44063=CARTESIAN_POINT('Ctrl Pts',(130.377065932835,38.3687715011547,29.8093955407772));
#44064=CARTESIAN_POINT('Ctrl Pts',(130.442981566568,38.3610019644911,29.805388279165));
#44065=CARTESIAN_POINT('Ctrl Pts',(130.489037976877,38.3546100044673,29.8025359538501));
#44066=CARTESIAN_POINT('Ctrl Pts',(130.741906137056,38.3141977742004,29.7866376125801));
#44067=CARTESIAN_POINT('Ctrl Pts',(130.945343166554,38.2620011290399,29.772997467042));
#44068=CARTESIAN_POINT('Ctrl Pts',(131.295610522636,38.1365897490847,29.7491192806637));
#44069=CARTESIAN_POINT('Ctrl Pts',(131.444450934583,38.0708913578075,29.7388296333424));
#44070=CARTESIAN_POINT('Ctrl Pts',(131.644653186378,37.9647310777899,29.7249343755634));
#44071=CARTESIAN_POINT('Ctrl Pts',(131.700427393834,37.9330976748062,29.7210549320412));
#44072=CARTESIAN_POINT('Ctrl Pts',(131.782990151824,37.8831234489878,29.7152972335149));
#44073=CARTESIAN_POINT('Ctrl Pts',(131.81046522756,37.8659501865912,29.7133785464316));
#44074=CARTESIAN_POINT('Ctrl Pts',(131.857834388023,37.8353890598971,29.7100648297688));
#44075=CARTESIAN_POINT('Ctrl Pts',(131.877840107333,37.822179354524,29.7086634942706));
#44076=CARTESIAN_POINT('Ctrl Pts',(131.922792188439,37.7918080111974,29.7055097554022));
#44077=CARTESIAN_POINT('Ctrl Pts',(131.947652310103,37.7745220012697,29.7037620873418));
#44078=CARTESIAN_POINT('Ctrl Pts',(132.014435168709,37.7267458256772,29.6990550485609));
#44079=CARTESIAN_POINT('Ctrl Pts',(132.055896373624,37.6956228119713,29.6961195437228));
#44080=CARTESIAN_POINT('Ctrl Pts',(132.285675537508,37.5147514640486,29.6797402903712));
#44081=CARTESIAN_POINT('Ctrl Pts',(132.458343912125,37.3462403951417,29.6670640870943));
#44082=CARTESIAN_POINT('Ctrl Pts',(132.691009760089,37.0650279231619,29.6476875016497));
#44083=CARTESIAN_POINT('Ctrl Pts',(132.764955498168,36.9649151355708,29.6410602893032));
#44084=CARTESIAN_POINT('Ctrl Pts',(132.87058883755,36.8040941486077,29.6304724136616));
#44085=CARTESIAN_POINT('Ctrl Pts',(132.906225027213,36.7461073381031,29.626664916079));
#44086=CARTESIAN_POINT('Ctrl Pts',(132.951554711617,36.6671114233039,29.6214382482017));
#44087=CARTESIAN_POINT('Ctrl Pts',(132.962815444465,36.6470155716039,29.6201052809632));
#44088=CARTESIAN_POINT('Ctrl Pts',(132.981281728464,36.6132584466571,29.6178579851844));
#44089=CARTESIAN_POINT('Ctrl Pts',(132.98860052641,36.5996594770144,29.6169504770649));
#44090=CARTESIAN_POINT('Ctrl Pts',(133.00349885901,36.5715179256244,29.6150670479207));
#44091=CARTESIAN_POINT('Ctrl Pts',(133.01106620254,36.5569695840981,29.6140904680651));
#44092=CARTESIAN_POINT('Ctrl Pts',(133.031221032418,36.517525081759,29.6114360571237));
#44093=CARTESIAN_POINT('Ctrl Pts',(133.043606956059,36.4925280260277,29.6097468025566));
#44094=CARTESIAN_POINT('Ctrl Pts',(133.111976697401,36.3501545721132,29.6000974754614));
#44095=CARTESIAN_POINT('Ctrl Pts',(133.161473464185,36.2297949978379,29.5918371166948));
#44096=CARTESIAN_POINT('Ctrl Pts',(133.271856857366,35.9102901768983,29.5701329181773));
#44097=CARTESIAN_POINT('Ctrl Pts',(133.321546649492,35.7078245061683,29.5566221564843));
#44098=CARTESIAN_POINT('Ctrl Pts',(133.368732334231,35.3927647529445,29.5366175010145));
#44099=CARTESIAN_POINT('Ctrl Pts',(133.379748476982,35.2827118151283,29.529806863054));
#44100=CARTESIAN_POINT('Ctrl Pts',(133.387350997142,35.1333432881135,29.5208120952739));
#44101=CARTESIAN_POINT('Ctrl Pts',(133.38866140773,35.0943465197464,29.5184862352233));
#44102=CARTESIAN_POINT('Ctrl Pts',(133.389742338794,35.0281383747375,29.5145740616786));
#44103=CARTESIAN_POINT('Ctrl Pts',(133.389859005575,35.0009372713536,29.5129772495642));
#44104=CARTESIAN_POINT('Ctrl Pts',(133.389433506699,34.9460198171519,29.509773562024));
#44105=CARTESIAN_POINT('Ctrl Pts',(133.388878790023,34.9183056313543,29.5081671970383));
#44106=CARTESIAN_POINT('Ctrl Pts',(133.386638238652,34.848918021057,29.504169709681));
#44107=CARTESIAN_POINT('Ctrl Pts',(133.384523125122,34.8072624702924,29.5017919413971));
#44108=CARTESIAN_POINT('Ctrl Pts',(133.372795943351,34.638037008602,29.4922100853011));
#44109=CARTESIAN_POINT('Ctrl Pts',(133.356734698258,34.5110149166854,29.4852030982287));
#44110=CARTESIAN_POINT('Ctrl Pts',(133.291922423045,34.1595968896442,29.4659731802995));
#44111=CARTESIAN_POINT('Ctrl Pts',(133.227524837606,33.9388188216643,29.4541002424322));
#44112=CARTESIAN_POINT('Ctrl Pts',(133.106664216691,33.6407526985984,29.4366497275216));
#44113=CARTESIAN_POINT('Ctrl Pts',(133.068525500484,33.5567175384529,29.4315533664364));
#44114=CARTESIAN_POINT('Ctrl Pts',(133.015654636829,33.4518175726498,29.4248379527263));
#44115=CARTESIAN_POINT('Ctrl Pts',(133.004047409048,33.429413867341,29.4233824938021));
#44116=CARTESIAN_POINT('Ctrl Pts',(132.984765846177,33.3931933448236,29.4209913413125));
#44117=CARTESIAN_POINT('Ctrl Pts',(132.977242832909,33.3792964860299,29.4200646774961));
#44118=CARTESIAN_POINT('Ctrl Pts',(132.962911506226,33.3532595244232,29.418310096787));
#44119=CARTESIAN_POINT('Ctrl Pts',(132.95612505258,33.3411077654539,29.4174836166903));
#44120=CARTESIAN_POINT('Ctrl Pts',(132.937807246257,33.3087774265661,29.4152650857196));
#44121=CARTESIAN_POINT('Ctrl Pts',(132.926143087348,33.2886754323102,29.4138650891572));
#44122=CARTESIAN_POINT('Ctrl Pts',(132.881232139369,33.213077643167,29.4085263680866));
#44123=CARTESIAN_POINT('Ctrl Pts',(132.846607438647,33.1584204749311,29.404514713979));
#44124=CARTESIAN_POINT('Ctrl Pts',(132.702154559927,32.9442084447895,29.3882742934291));
#44125=CARTESIAN_POINT('Ctrl Pts',(132.580305908436,32.7932066257174,29.3756642189649));
#44126=CARTESIAN_POINT('Ctrl Pts',(132.326575404897,32.5286987145862,29.3521543999739));
#44127=CARTESIAN_POINT('Ctrl Pts',(132.197539714227,32.4132808873563,29.3412484409462));
#44128=CARTESIAN_POINT('Ctrl Pts',(132.018417709447,32.2761847322142,29.3275238950633));
#44129=CARTESIAN_POINT('Ctrl Pts',(131.975846736311,32.2451479526931,29.3243549625648));
#44130=CARTESIAN_POINT('Ctrl Pts',(131.907849366188,32.1979612603903,29.3194346321943));
#44131=CARTESIAN_POINT('Ctrl Pts',(131.882903049924,32.1811373757809,29.3176583229723));
#44132=CARTESIAN_POINT('Ctrl Pts',(131.835536862737,32.15010284226,29.3143382953861));
#44133=CARTESIAN_POINT('Ctrl Pts',(131.813167807197,32.1358191492085,29.3127919737489));
#44134=CARTESIAN_POINT('Ctrl Pts',(131.762026658838,32.1040023894909,29.309304123544));
#44135=CARTESIAN_POINT('Ctrl Pts',(131.733156058135,32.0866324809796,29.3073685690024));
#44136=CARTESIAN_POINT('Ctrl Pts',(131.64200786455,32.0336279892345,29.3013570985733));
#44137=CARTESIAN_POINT('Ctrl Pts',(131.578853086716,31.9995372597811,29.2973349803857));
#44138=CARTESIAN_POINT('Ctrl Pts',(131.252041653444,31.8363041766667,29.2771424565233));
#44139=CARTESIAN_POINT('Ctrl Pts',(130.973518179817,31.7398110085746,29.2620654744137));
#44140=CARTESIAN_POINT('Ctrl Pts',(130.619654923719,31.6666788248659,29.242512375996));
#44141=CARTESIAN_POINT('Ctrl Pts',(130.552861772203,31.6549521350261,29.238798627151));
#44142=CARTESIAN_POINT('Ctrl Pts',(130.440488724307,31.6386806582955,29.232448062967));
#44143=CARTESIAN_POINT('Ctrl Pts',(130.395086070095,31.6330422318763,29.229854401965));
#44144=CARTESIAN_POINT('Ctrl Pts',(130.329794477347,31.6262726009943,29.2260672936508));
#44145=CARTESIAN_POINT('Ctrl Pts',(130.309986230686,31.6243949497358,29.2249108177791));
#44146=CARTESIAN_POINT('Ctrl Pts',(130.275238890605,31.6214096145749,29.2228671719588));
#44147=CARTESIAN_POINT('Ctrl Pts',(130.26030718412,31.6202263983687,29.2219840665314));
#44148=CARTESIAN_POINT('Ctrl Pts',(130.22738442505,31.6178370109096,29.2200256982347));
#44149=CARTESIAN_POINT('Ctrl Pts',(130.209391533693,31.61667540501,29.2189482036346));
#44150=CARTESIAN_POINT('Ctrl Pts',(130.156968170767,31.6137107692029,29.2157895394178));
#44151=CARTESIAN_POINT('Ctrl Pts',(130.122519361727,31.6122894795468,29.2136896584942));
#44152=CARTESIAN_POINT('Ctrl Pts',(129.895418420125,31.6063880329707,29.1997124205796));
#44153=CARTESIAN_POINT('Ctrl Pts',(129.702718164474,31.6178183357135,29.1872387209001));
#44154=CARTESIAN_POINT('Ctrl Pts',(129.359552834562,31.6677365880789,29.1648974729263));
#44155=CARTESIAN_POINT('Ctrl Pts',(129.208736362133,31.70029380636,29.1550298705524));
#44156=CARTESIAN_POINT('Ctrl Pts',(128.969964925965,31.7691579384153,29.1395374135534));
#44157=CARTESIAN_POINT('Ctrl Pts',(128.880407081276,31.7990896708485,29.1337544714835));
#44158=CARTESIAN_POINT('Ctrl Pts',(128.757503538842,31.8459570095804,29.1258603909076));
#44159=CARTESIAN_POINT('Ctrl Pts',(128.723017450146,31.8597610961331,29.1236498622348));
#44160=CARTESIAN_POINT('Ctrl Pts',(128.663881751335,31.8845672586581,29.1198657557421));
#44161=CARTESIAN_POINT('Ctrl Pts',(128.639124357407,31.8953018362051,29.1182834958549));
#44162=CARTESIAN_POINT('Ctrl Pts',(128.588523152817,31.9179636373577,29.115052625006));
#44163=CARTESIAN_POINT('Ctrl Pts',(128.562696050417,31.9299230532415,29.1134052517419));
#44164=CARTESIAN_POINT('Ctrl Pts',(128.496561847067,31.9615644589303,29.1091893537274));
#44165=CARTESIAN_POINT('Ctrl Pts',(128.456488609414,31.9817240569353,29.1066372099883));
#44166=CARTESIAN_POINT('Ctrl Pts',(128.25432265732,32.0885071927156,29.0937551582498));
#44167=CARTESIAN_POINT('Ctrl Pts',(128.099061540752,32.1874170745686,29.0838614437335));
#44168=CARTESIAN_POINT('Ctrl Pts',(127.811353682883,32.4054616617986,29.0646669692373));
#44169=CARTESIAN_POINT('Ctrl Pts',(127.678752245693,32.523388502055,29.0553820673352));
#44170=CARTESIAN_POINT('Ctrl Pts',(127.498935769655,32.7104890326141,29.0412242664885));
#44171=CARTESIAN_POINT('Ctrl Pts',(127.444074420526,32.7719010017034,29.0366527478963));
#44172=CARTESIAN_POINT('Ctrl Pts',(127.375879876727,32.85407422525,29.0305396321504));
#44173=CARTESIAN_POINT('Ctrl Pts',(127.360457615728,32.873072690533,29.0291265128249));
#44174=CARTESIAN_POINT('Ctrl Pts',(127.335478339087,32.9045344236397,29.0267836639857));
#44175=CARTESIAN_POINT('Ctrl Pts',(127.325799554906,32.9169004762236,29.0258621324421));
#44176=CARTESIAN_POINT('Ctrl Pts',(127.307612713588,32.9404724540948,29.024103316386));
#44177=CARTESIAN_POINT('Ctrl Pts',(127.299087827608,32.9516649605973,29.0232672841928));
#44178=CARTESIAN_POINT('Ctrl Pts',(127.276172125178,32.9821432638267,29.0209889823996));
#44179=CARTESIAN_POINT('Ctrl Pts',(127.261916869223,33.0015293857175,29.019538010938));
#44180=CARTESIAN_POINT('Ctrl Pts',(127.206137571674,33.0791023721337,29.0137301344299));
#44181=CARTESIAN_POINT('Ctrl Pts',(127.166254566074,33.1384414168332,29.0092836109307));
#44182=CARTESIAN_POINT('Ctrl Pts',(127.02823455371,33.3585153431092,28.9928991426864));
#44183=CARTESIAN_POINT('Ctrl Pts',(126.941657351632,33.5260935052429,28.9806427878136));
#44184=CARTESIAN_POINT('Ctrl Pts',(126.798563933177,33.8706771973782,28.9567221888633));
#44185=CARTESIAN_POINT('Ctrl Pts',(126.741753844291,34.0468935515748,28.9450928169622));
#44186=CARTESIAN_POINT('Ctrl Pts',(126.68944108561,34.2702156167127,28.9312282178701));
#44187=CARTESIAN_POINT('Ctrl Pts',(126.680145061556,34.3137427290265,28.9285644142146));
#44188=CARTESIAN_POINT('Ctrl Pts',(126.666330871604,34.3852968031259,28.9242464007384));
#44189=CARTESIAN_POINT('Ctrl Pts',(126.661302993951,34.4132187351067,28.9225764757834));
#44190=CARTESIAN_POINT('Ctrl Pts',(126.652177297309,34.467819090193,28.9193393158131));
#44191=CARTESIAN_POINT('Ctrl Pts',(126.648046417002,34.4944897541941,28.9177711615604));
#44192=CARTESIAN_POINT('Ctrl Pts',(126.638966772336,34.5581272555422,28.914059226215));
#44193=CARTESIAN_POINT('Ctrl Pts',(126.634308647977,34.5951324183887,28.9119245724412));
#44194=CARTESIAN_POINT('Ctrl Pts',(126.620540178399,34.7212801693608,28.9047218423056));
#44195=CARTESIAN_POINT('Ctrl Pts',(126.614353322164,34.8107070684153,28.899742453578));
#44196=CARTESIAN_POINT('Ctrl Pts',(126.603771081865,35.1702684500139,28.8800694472354));
#44197=CARTESIAN_POINT('Ctrl Pts',(126.628122353902,35.4402203034712,28.8661653493926));
#44198=CARTESIAN_POINT('Ctrl Pts',(126.697999968844,35.7691423114793,28.8479565103754));
#44199=CARTESIAN_POINT('Ctrl Pts',(126.713643286946,35.8334523266386,28.8443289963956));
#44200=CARTESIAN_POINT('Ctrl Pts',(126.743057386354,35.9406119691821,28.8381106137182));
#44201=CARTESIAN_POINT('Ctrl Pts',(126.755817688955,35.9837208943478,28.8355608235598));
#44202=CARTESIAN_POINT('Ctrl Pts',(126.775405856459,36.0453645009853,28.8318283427567));
#44203=CARTESIAN_POINT('Ctrl Pts',(126.781544802124,36.0641148570927,28.8306813769202));
#44204=CARTESIAN_POINT('Ctrl Pts',(126.792618524998,36.0969650256828,28.8286496727444));
#44205=CARTESIAN_POINT('Ctrl Pts',(126.797483360558,36.1110874651656,28.8277688806398));
#44206=CARTESIAN_POINT('Ctrl Pts',(126.808444365314,36.1422367254611,28.8258095158838));
#44207=CARTESIAN_POINT('Ctrl Pts',(126.814583471908,36.1592470040824,28.8247286292288));
#44208=CARTESIAN_POINT('Ctrl Pts',(126.820986075039,36.1765524481033,28.823618425201));
#44209=CARTESIAN_POINT('Ctrl Pts',(126.821113968604,36.1768979554873,28.8235962553991));
#44210=CARTESIAN_POINT('Ctrl Pts',(126.821241918358,36.1772434416436,28.8235740826546));
#44211=CARTESIAN_POINT('Origin',(-10.,35.,32.7603849714045));
#44212=CARTESIAN_POINT('',(-7.51282733495085,38.2405550657615,18.0469656644349));
#44213=CARTESIAN_POINT('',(-7.51282733495087,38.2405550657615,17.9425398374177));
#44214=CARTESIAN_POINT('',(-7.51282733495086,38.2405550657615,32.7603849714045));
#44215=CARTESIAN_POINT('',(-14.0827629539364,34.9944901030589,17.1353849829093));
#44216=CARTESIAN_POINT('Ctrl Pts',(-7.51282733495087,38.2405550657615,17.9425398374177));
#44217=CARTESIAN_POINT('Ctrl Pts',(-7.4183033415916,38.1680065400603,17.9367380921735));
#44218=CARTESIAN_POINT('Ctrl Pts',(-7.32687001393603,38.0912526206094,17.9309363469293));
#44219=CARTESIAN_POINT('Ctrl Pts',(-7.23891909304243,38.0105908432124,17.925134601685));
#44220=CARTESIAN_POINT('Ctrl Pts',(-7.15101721148065,37.929974040895,17.9193360913553));
#44221=CARTESIAN_POINT('Ctrl Pts',(-7.0665941758643,37.8454539901771,17.9135375810256));
#44222=CARTESIAN_POINT('Ctrl Pts',(-6.98600847518456,37.7573683265644,17.9077390706959));
#44223=CARTESIAN_POINT('Ctrl Pts',(-6.9054455566571,37.669307565397,17.9019421996465));
#44224=CARTESIAN_POINT('Ctrl Pts',(-6.82871809216569,37.5776834973517,17.896145328597));
#44225=CARTESIAN_POINT('Ctrl Pts',(-6.75614709878714,37.482869983566,17.8903484575475));
#44226=CARTESIAN_POINT('Ctrl Pts',(-6.68357939025863,37.3880607614147,17.8845518488873));
#44227=CARTESIAN_POINT('Ctrl Pts',(-6.61516802742511,37.2900627057404,17.8787552402272));
#44228=CARTESIAN_POINT('Ctrl Pts',(-6.55119276284196,37.1892815353276,17.872958631567));
#44229=CARTESIAN_POINT('Ctrl Pts',(-6.48720520356606,37.0884809969054,17.8671609089212));
#44230=CARTESIAN_POINT('Ctrl Pts',(-6.42765565715021,36.984896625763,17.8613631862754));
#44231=CARTESIAN_POINT('Ctrl Pts',(-6.37277934104189,36.8789612266429,17.8555654636297));
#44232=CARTESIAN_POINT('Ctrl Pts',(-6.31784510984411,36.7729140259561,17.8497616222127));
#44233=CARTESIAN_POINT('Ctrl Pts',(-6.26759414824649,36.6645112056742,17.8439577807956));
#44234=CARTESIAN_POINT('Ctrl Pts',(-6.22221477081377,36.5542084037034,17.8381539393786));
#44235=CARTESIAN_POINT('Ctrl Pts',(-6.17681086915101,36.4438459911465,17.8323469614104));
#44236=CARTESIAN_POINT('Ctrl Pts',(-6.13628393538455,36.3315819363009,17.8265399834421));
#44237=CARTESIAN_POINT('Ctrl Pts',(-6.10077276455028,36.2178883226007,17.8207330054739));
#44238=CARTESIAN_POINT('Ctrl Pts',(-6.06520417671164,36.104010880923,17.8149166383677));
#44239=CARTESIAN_POINT('Ctrl Pts',(-6.03466765964787,35.988699658222,17.8091002712616));
#44240=CARTESIAN_POINT('Ctrl Pts',(-6.00925125311316,35.8724387882374,17.8032839041555));
#44241=CARTESIAN_POINT('Ctrl Pts',(-5.98745160169316,35.7727218421778,17.7982952061949));
#44242=CARTESIAN_POINT('Ctrl Pts',(-5.96941771976481,35.6723065937043,17.7933065082343));
#44243=CARTESIAN_POINT('Ctrl Pts',(-5.95517468308408,35.571500792332,17.7883178102738));
#44244=CARTESIAN_POINT('Ctrl Pts',(-5.93851904215847,35.4536196642752,17.7824840850802));
#44245=CARTESIAN_POINT('Ctrl Pts',(-5.92699445772989,35.3348226640355,17.7766503598866));
#44246=CARTESIAN_POINT('Ctrl Pts',(-5.92069312782201,35.2155932341272,17.770816634693));
#44247=CARTESIAN_POINT('Ctrl Pts',(-5.91439975786786,35.0965144169879,17.7649902787665));
#44248=CARTESIAN_POINT('Ctrl Pts',(-5.91331653925813,34.9770046594567,17.7591639228399));
#44249=CARTESIAN_POINT('Ctrl Pts',(-5.91748428809018,34.8575554072299,17.7533375669133));
#44250=CARTESIAN_POINT('Ctrl Pts',(-5.92164784806494,34.7382262092316,17.7475170668515));
#44251=CARTESIAN_POINT('Ctrl Pts',(-5.93105186156511,34.6189577997927,17.7416965667897));
#44252=CARTESIAN_POINT('Ctrl Pts',(-5.94568515168971,34.5002439487403,17.7358760667279));
#44253=CARTESIAN_POINT('Ctrl Pts',(-5.96083652425654,34.3773271083836,17.7298494955186));
#44254=CARTESIAN_POINT('Ctrl Pts',(-5.98159433369207,34.2550052647982,17.7238229243093));
#44255=CARTESIAN_POINT('Ctrl Pts',(-6.00788729115695,34.1338238516942,17.7177963531001));
#44256=CARTESIAN_POINT('Ctrl Pts',(-6.03325201513153,34.016920566914,17.7119825409627));
#44257=CARTESIAN_POINT('Ctrl Pts',(-6.06376758361259,33.9010789832808,17.7061687288253));
#44258=CARTESIAN_POINT('Ctrl Pts',(-6.09931768119087,33.7867801321566,17.700354916688));
#44259=CARTESIAN_POINT('Ctrl Pts',(-6.13486209666282,33.6724995498494,17.6945420337942));
#44260=CARTESIAN_POINT('Ctrl Pts',(-6.17543931998105,33.5597615979302,17.6887291509004));
#44261=CARTESIAN_POINT('Ctrl Pts',(-6.22088303717803,33.4490325660056,17.6829162680066));
#44262=CARTESIAN_POINT('Ctrl Pts',(-6.26633011389279,33.3382953482156,17.6771029553837));
#44263=CARTESIAN_POINT('Ctrl Pts',(-6.31664424526961,33.2295677220171,17.6712896427609));
#44264=CARTESIAN_POINT('Ctrl Pts',(-6.37161104484388,33.1232958171035,17.6654763301381));
#44265=CARTESIAN_POINT('Ctrl Pts',(-6.42659475686175,33.0169912139501,17.6596612288479));
#44266=CARTESIAN_POINT('Ctrl Pts',(-6.48623379744393,32.9131441959916,17.6538461275577));
#44267=CARTESIAN_POINT('Ctrl Pts',(-6.55026823437055,32.8121755680112,17.6480310262675));
#44268=CARTESIAN_POINT('Ctrl Pts',(-6.61437141346114,32.7110985483229,17.6422096823575));
#44269=CARTESIAN_POINT('Ctrl Pts',(-6.6828791897496,32.6129064304381,17.6363883384474));
#44270=CARTESIAN_POINT('Ctrl Pts',(-6.75548868636104,32.5179904642269,17.6305669945374));
#44271=CARTESIAN_POINT('Ctrl Pts',(-6.82814457559643,32.4230138530458,17.624741931177));
#44272=CARTESIAN_POINT('Ctrl Pts',(-6.90490714451128,32.3313178741207,17.6189168678166));
#44273=CARTESIAN_POINT('Ctrl Pts',(-6.98543474817405,32.2432589271962,17.6130918044561));
#44274=CARTESIAN_POINT('Ctrl Pts',(-7.06607455930401,32.1550772786023,17.6072586244304));
#44275=CARTESIAN_POINT('Ctrl Pts',(-7.1504895902578,32.0705430644841,17.6014254444047));
#44276=CARTESIAN_POINT('Ctrl Pts',(-7.23830297666916,31.9899743271318,17.595592264379));
#44277=CARTESIAN_POINT('Ctrl Pts',(-7.26015105310161,31.9699287281215,17.5941409621545));
#44278=CARTESIAN_POINT('Ctrl Pts',(-7.28220934456464,31.9501283972475,17.5926896599299));
#44279=CARTESIAN_POINT('Ctrl Pts',(-7.30447175887145,31.9305778228992,17.5912383577053));
#44280=CARTESIAN_POINT('Ctrl Pts',(-7.39387101201482,31.8520685147364,17.5854103584069));
#44281=CARTESIAN_POINT('Ctrl Pts',(-7.48684416404283,31.7773442700337,17.5795823591084));
#44282=CARTESIAN_POINT('Ctrl Pts',(-7.58303761970974,31.706746615843,17.57375435981));
#44283=CARTESIAN_POINT('Ctrl Pts',(-7.67911152471163,31.6362367014725,17.5679336036362));
#44284=CARTESIAN_POINT('Ctrl Pts',(-7.77839744686426,31.56984341552,17.5621128474624));
#44285=CARTESIAN_POINT('Ctrl Pts',(-7.8805069604902,31.5078696680293,17.5562920912886));
#44286=CARTESIAN_POINT('Ctrl Pts',(-7.9825160475301,31.44595687286,17.5504770599357));
#44287=CARTESIAN_POINT('Ctrl Pts',(-8.0873428547323,31.3884551787733,17.5446620285827));
#44288=CARTESIAN_POINT('Ctrl Pts',(-8.19456855147211,31.3356252532435,17.5388469972298));
#44289=CARTESIAN_POINT('Ctrl Pts',(-8.30573362625101,31.2808544025926,17.5328183267259));
#44290=CARTESIAN_POINT('Ctrl Pts',(-8.41947687947959,31.2311054465056,17.526789656222));
#44291=CARTESIAN_POINT('Ctrl Pts',(-8.53530150854896,31.1866178621674,17.5207609857182));
#44292=CARTESIAN_POINT('Ctrl Pts',(-8.64690001636399,31.1437535070787,17.5149522847731));
#44293=CARTESIAN_POINT('Ctrl Pts',(-8.76043025743789,31.1057734553835,17.509143583828));
#44294=CARTESIAN_POINT('Ctrl Pts',(-8.87542649629038,31.0728433396725,17.5033348828829));
#44295=CARTESIAN_POINT('Ctrl Pts',(-8.99040711539206,31.0399176968052,17.4975269709241));
#44296=CARTESIAN_POINT('Ctrl Pts',(-9.10685294459492,31.0120407379528,17.4917190589654));
#44297=CARTESIAN_POINT('Ctrl Pts',(-9.22428325402143,30.9893281697441,17.4859111470066));
#44298=CARTESIAN_POINT('Ctrl Pts',(-9.34172518549361,30.9666133536786,17.4801026602404));
#44299=CARTESIAN_POINT('Ctrl Pts',(-9.46015139082179,30.9490640219931,17.4742941734742));
#44300=CARTESIAN_POINT('Ctrl Pts',(-9.57907174529857,30.9367446050742,17.468485686708));
#44301=CARTESIAN_POINT('Ctrl Pts',(-9.69803179132901,30.9244210763545,17.4626752612672));
#44302=CARTESIAN_POINT('Ctrl Pts',(-9.81748590941725,30.9173309761372,17.4568648358264));
#44303=CARTESIAN_POINT('Ctrl Pts',(-9.93694029613936,30.915486751919,17.4510544103857));
#44304=CARTESIAN_POINT('Ctrl Pts',(-10.0565280337012,30.913640468933,17.4452374985769));
#44305=CARTESIAN_POINT('Ctrl Pts',(-10.1761156328021,30.9170517577107,17.4394205867682));
#44306=CARTESIAN_POINT('Ctrl Pts',(-10.2952105629053,30.9256809497108,17.4336036749594));
#44307=CARTESIAN_POINT('Ctrl Pts',(-10.4143844498564,30.9343158626414,17.427782906689));
#44308=CARTESIAN_POINT('Ctrl Pts',(-10.5330646134808,30.9481755212524,17.4219621384187));
#44309=CARTESIAN_POINT('Ctrl Pts',(-10.6507665506426,30.9671687493072,17.4161413701484));
#44310=CARTESIAN_POINT('Ctrl Pts',(-10.7686372902992,30.9861892165421,17.4103122540103));
#44311=CARTESIAN_POINT('Ctrl Pts',(-10.8855266056535,31.0103578659512,17.4044831378722));
#44312=CARTESIAN_POINT('Ctrl Pts',(-11.0009628848836,31.0395330700679,17.3986540217341));
#44313=CARTESIAN_POINT('Ctrl Pts',(-11.0306357387891,31.0470325457544,17.397155649535));
#44314=CARTESIAN_POINT('Ctrl Pts',(-11.0602126778042,31.0548625757694,17.395657277336));
#44315=CARTESIAN_POINT('Ctrl Pts',(-11.0896858991661,31.0630202386654,17.3941589051369));
#44316=CARTESIAN_POINT('Ctrl Pts',(-11.2031708726653,31.0944308587056,17.3883895076483));
#44317=CARTESIAN_POINT('Ctrl Pts',(-11.3154990757746,31.1308085462832,17.3826201101598));
#44318=CARTESIAN_POINT('Ctrl Pts',(-11.4261981271612,31.1720522597504,17.3768507126713));
#44319=CARTESIAN_POINT('Ctrl Pts',(-11.5367558093482,31.2132433025696,17.3710886830427));
#44320=CARTESIAN_POINT('Ctrl Pts',(-11.6456880894902,31.2592878728293,17.3653266534141));
#44321=CARTESIAN_POINT('Ctrl Pts',(-11.7525351267066,31.3100344676868,17.3595646237854));
#44322=CARTESIAN_POINT('Ctrl Pts',(-11.8592748935706,31.3607301148975,17.3538083790149));
#44323=CARTESIAN_POINT('Ctrl Pts',(-11.963933206448,31.4161182219792,17.3480521342444));
#44324=CARTESIAN_POINT('Ctrl Pts',(-12.0660683609068,31.4759985062347,17.3422958894739));
#44325=CARTESIAN_POINT('Ctrl Pts',(-12.1734278736667,31.5389417521295,17.3362452046029));
#44326=CARTESIAN_POINT('Ctrl Pts',(-12.2779988274438,31.6068487403076,17.3301945197318));
#44327=CARTESIAN_POINT('Ctrl Pts',(-12.3792952275086,31.6794308890862,17.3241438348608));
#44328=CARTESIAN_POINT('Ctrl Pts',(-12.4755596833424,31.7484074869806,17.3183937204819));
#44329=CARTESIAN_POINT('Ctrl Pts',(-12.5688667050551,31.8216056715209,17.3126436061031));
#44330=CARTESIAN_POINT('Ctrl Pts',(-12.6588281203624,31.8987328353768,17.3068934917243));
#44331=CARTESIAN_POINT('Ctrl Pts',(-12.7487797405037,31.9758516014838,17.3011440034286));
#44332=CARTESIAN_POINT('Ctrl Pts',(-12.8353861617372,32.0568982255982,17.2953945151329));
#44333=CARTESIAN_POINT('Ctrl Pts',(-12.9182926742957,32.1415401232216,17.2896450268373));
#44334=CARTESIAN_POINT('Ctrl Pts',(-13.0012106444888,32.2261937183089,17.2838947439654));
#44335=CARTESIAN_POINT('Ctrl Pts',(-13.0804273978305,32.3144432769193,17.2781444610936));
#44336=CARTESIAN_POINT('Ctrl Pts',(-13.1556259804814,32.4059202650437,17.2723941782218));
#44337=CARTESIAN_POINT('Ctrl Pts',(-13.2308535373257,32.4974324994701,17.2666416797523));
#44338=CARTESIAN_POINT('Ctrl Pts',(-13.3020595810806,32.5921743139375,17.2608891812828));
#44339=CARTESIAN_POINT('Ctrl Pts',(-13.3689687108363,32.6897457227816,17.2551366828132));
#44340=CARTESIAN_POINT('Ctrl Pts',(-13.4359614234129,32.7874390177363,17.2493769983281));
#44341=CARTESIAN_POINT('Ctrl Pts',(-13.498646273364,32.8879686178449,17.243617313843));
#44342=CARTESIAN_POINT('Ctrl Pts',(-13.5567922492037,32.990907195771,17.2378576293579));
#44343=CARTESIAN_POINT('Ctrl Pts',(-13.6149804832775,33.0939205854527,17.232093758958));
#44344=CARTESIAN_POINT('Ctrl Pts',(-13.6686230900308,33.1993460671065,17.2263298885582));
#44345=CARTESIAN_POINT('Ctrl Pts',(-13.7175367147721,33.3067351730099,17.2205660181584));
#44346=CARTESIAN_POINT('Ctrl Pts',(-13.7665291072191,33.414297212192,17.2147928659511));
#44347=CARTESIAN_POINT('Ctrl Pts',(-13.81077716563,33.5238288013093,17.2090197137437));
#44348=CARTESIAN_POINT('Ctrl Pts',(-13.8501469330714,33.6348649906472,17.2032465615364));
#44349=CARTESIAN_POINT('Ctrl Pts',(-13.8641657127107,33.6744027367777,17.2011908585471));
#44350=CARTESIAN_POINT('Ctrl Pts',(-13.877566430735,33.7141311528221,17.1991351555578));
#44351=CARTESIAN_POINT('Ctrl Pts',(-13.8903446080909,33.7540289608912,17.1970794525685));
#44352=CARTESIAN_POINT('Ctrl Pts',(-13.9364896150878,33.8981093395885,17.189655825068));
#44353=CARTESIAN_POINT('Ctrl Pts',(-13.9746373453614,34.0447885994859,17.1822321975675));
#44354=CARTESIAN_POINT('Ctrl Pts',(-14.004551758706,34.193284305443,17.174808570067));
#44355=CARTESIAN_POINT('Ctrl Pts',(-14.033969026612,34.3393121721674,17.1675083152867));
#44356=CARTESIAN_POINT('Ctrl Pts',(-14.0554244147101,34.4870967690664,17.1602080605065));
#44357=CARTESIAN_POINT('Ctrl Pts',(-14.0687390147019,34.6358738814061,17.1529078057263));
#44358=CARTESIAN_POINT('Ctrl Pts',(-14.0793920292548,34.7549104836218,17.1470668701773));
#44359=CARTESIAN_POINT('Ctrl Pts',(-14.0848344524003,34.8745821123516,17.1412259346282));
#44360=CARTESIAN_POINT('Ctrl Pts',(-14.0849962795766,34.9944867572603,17.1353849990792));
#44361=CARTESIAN_POINT('',(-13.1750507821943,37.570267988068,17.));
#44362=CARTESIAN_POINT('Ctrl Pts',(-14.0811739487135,34.9944924835857,17.1353849714045));
#44363=CARTESIAN_POINT('Ctrl Pts',(-14.0735484049167,35.9200466893068,17.090256647603));
#44364=CARTESIAN_POINT('Ctrl Pts',(-13.7580895933996,36.8500404311904,17.0451283238015));
#44365=CARTESIAN_POINT('Ctrl Pts',(-13.1750507821943,37.570267988068,17.));
#44366=CARTESIAN_POINT('',(-11.4626270635503,38.8141771160986,17.0000001028261));
#44367=CARTESIAN_POINT('Origin',(-10.,35.,17.));
#44368=CARTESIAN_POINT('',(-14.0849987342305,35.0032157946179,17.2396150285694));
#44369=CARTESIAN_POINT('Ctrl Pts',(-14.0849987342305,35.0032157946178,17.2396150285694));
#44370=CARTESIAN_POINT('Ctrl Pts',(-14.0848793000589,35.1549320880902,17.2322291681083));
#44371=CARTESIAN_POINT('Ctrl Pts',(-14.0763041428688,35.3062908916574,17.2248433076472));
#44372=CARTESIAN_POINT('Ctrl Pts',(-14.059414157619,35.4564884411704,17.2174574471862));
#44373=CARTESIAN_POINT('Ctrl Pts',(-14.0421962898582,35.6096017510568,17.2099282062284));
#44374=CARTESIAN_POINT('Ctrl Pts',(-14.0163376314483,35.7615085205179,17.2023989652706));
#44375=CARTESIAN_POINT('Ctrl Pts',(-13.9820359968326,35.9113804474144,17.1948697243128));
#44376=CARTESIAN_POINT('Ctrl Pts',(-13.9743911680411,35.9447825063723,17.1931916772256));
#44377=CARTESIAN_POINT('Ctrl Pts',(-13.9663271537708,35.9780835733154,17.1915136301384));
#44378=CARTESIAN_POINT('Ctrl Pts',(-13.9578464672157,36.0112746125304,17.1898355830512));
#44379=CARTESIAN_POINT('Ctrl Pts',(-13.9285721977973,36.1258459291263,17.1840431743579));
#44380=CARTESIAN_POINT('Ctrl Pts',(-13.8942697521635,36.2393372344149,17.1782507656646));
#44381=CARTESIAN_POINT('Ctrl Pts',(-13.855034425663,36.3512714667873,17.1724583569712));
#44382=CARTESIAN_POINT('Ctrl Pts',(-13.8158480556437,36.463066031502,17.1666731758448));
#44383=CARTESIAN_POINT('Ctrl Pts',(-13.7717411799201,36.5733070003613,17.1608879947184));
#44384=CARTESIAN_POINT('Ctrl Pts',(-13.7228597190487,36.6815292183857,17.155102813592));
#44385=CARTESIAN_POINT('Ctrl Pts',(-13.6740261466227,36.789645412701,17.1493233001222));
#44386=CARTESIAN_POINT('Ctrl Pts',(-13.6204274618174,36.8957464154687,17.1435437866523));
#44387=CARTESIAN_POINT('Ctrl Pts',(-13.5622586122089,36.9993845502413,17.1377642731824));
#44388=CARTESIAN_POINT('Ctrl Pts',(-13.5041295541281,37.1029517893414,17.1319887133006));
#44389=CARTESIAN_POINT('Ctrl Pts',(-13.4414367513126,37.2040591524435,17.1262131534188));
#44390=CARTESIAN_POINT('Ctrl Pts',(-13.3744219785508,37.3022817617905,17.120437593537));
#44391=CARTESIAN_POINT('Ctrl Pts',(-13.3074313226107,37.4004690234514,17.1146641121245));
#44392=CARTESIAN_POINT('Ctrl Pts',(-13.2361220211795,37.4957732542151,17.108890630712));
#44393=CARTESIAN_POINT('Ctrl Pts',(-13.1607799203636,37.5877973829158,17.1031171492995));
#44394=CARTESIAN_POINT('Ctrl Pts',(-13.0854466514282,37.6798107242069,17.097344344676));
#44395=CARTESIAN_POINT('Ctrl Pts',(-13.0060817849086,37.7685444084177,17.0915715400524));
#44396=CARTESIAN_POINT('Ctrl Pts',(-12.9230118657337,37.8536339346139,17.0857987354288));
#44397=CARTESIAN_POINT('Ctrl Pts',(-12.8399315271689,37.9387341335176,17.0800252067272));
#44398=CARTESIAN_POINT('Ctrl Pts',(-12.7531455009603,38.020188970308,17.0742516780256));
#44399=CARTESIAN_POINT('Ctrl Pts',(-12.6630171327591,38.0976708589893,17.068478149324));
#44400=CARTESIAN_POINT('Ctrl Pts',(-12.5727996533326,38.1752293551381,17.0626989122508));
#44401=CARTESIAN_POINT('Ctrl Pts',(-12.4792335449056,38.2488067870086,17.0569196751776));
#44402=CARTESIAN_POINT('Ctrl Pts',(-12.3827153287825,38.3181158301037,17.0511404381044));
#44403=CARTESIAN_POINT('Ctrl Pts',(-12.2861497208749,38.3874589049015,17.0453583633455));
#44404=CARTESIAN_POINT('Ctrl Pts',(-12.1866294636243,38.452529189814,17.0395762885867));
#44405=CARTESIAN_POINT('Ctrl Pts',(-12.0845786339523,38.5130836766108,17.0337942138278));
#44406=CARTESIAN_POINT('Ctrl Pts',(-11.982363678535,38.5737355516436,17.0280028399057));
#44407=CARTESIAN_POINT('Ctrl Pts',(-11.8776103833025,38.6298569217935,17.0222114659835));
#44408=CARTESIAN_POINT('Ctrl Pts',(-11.7707663916904,38.6812513342693,17.0164200920614));
#44409=CARTESIAN_POINT('Ctrl Pts',(-11.6697899385664,38.7298233260482,17.0109467623163));
#44410=CARTESIAN_POINT('Ctrl Pts',(-11.5669465668444,38.7741735913199,17.0054734325712));
#44411=CARTESIAN_POINT('Ctrl Pts',(-11.4626270635503,38.8141771160986,17.0000001028261));
#44412=CARTESIAN_POINT('Ctrl Pts',(-7.51282733495085,38.2405550657615,18.0469656644349));
#44413=CARTESIAN_POINT('Ctrl Pts',(-7.41799580939191,38.1677705046697,18.0411565278969));
#44414=CARTESIAN_POINT('Ctrl Pts',(-7.32640791336297,38.0908551206141,18.035347391359));
#44415=CARTESIAN_POINT('Ctrl Pts',(-7.23842896479515,38.0101412620536,18.029538254821));
#44416=CARTESIAN_POINT('Ctrl Pts',(-7.15040477028745,37.9293858938541,18.0237261307519));
#44417=CARTESIAN_POINT('Ctrl Pts',(-7.06599350988609,37.8448284480232,18.0179140066829));
#44418=CARTESIAN_POINT('Ctrl Pts',(-6.98552275644513,37.7568373089629,18.0121018826139));
#44419=CARTESIAN_POINT('Ctrl Pts',(-6.90492115276495,37.6687030910684,18.0062803076848));
#44420=CARTESIAN_POINT('Ctrl Pts',(-6.82827312247758,37.5771243363809,18.0004587327558));
#44421=CARTESIAN_POINT('Ctrl Pts',(-6.75586553378204,37.4825020775614,17.9946371578267));
#44422=CARTESIAN_POINT('Ctrl Pts',(-6.68752494125946,37.3931945705715,17.9891425696595));
#44423=CARTESIAN_POINT('Ctrl Pts',(-6.6229615963789,37.3011763603051,17.9836479814922));
#44424=CARTESIAN_POINT('Ctrl Pts',(-6.56237959198754,37.2068055941601,17.978153393325));
#44425=CARTESIAN_POINT('Ctrl Pts',(-6.49815823619039,37.1067656794967,17.9723287279777));
#44426=CARTESIAN_POINT('Ctrl Pts',(-6.43820405998836,37.0037589441355,17.9665040626304));
#44427=CARTESIAN_POINT('Ctrl Pts',(-6.38280233067359,36.8981849280351,17.9606793972832));
#44428=CARTESIAN_POINT('Ctrl Pts',(-6.32747052185801,36.7927441530446,17.9548620830333));
#44429=CARTESIAN_POINT('Ctrl Pts',(-6.2766799202222,36.6847429000424,17.9490447687834));
#44430=CARTESIAN_POINT('Ctrl Pts',(-6.2306724747935,36.5746094778454,17.9432274545335));
#44431=CARTESIAN_POINT('Ctrl Pts',(-6.18471111391979,36.4645863736569,17.9374159673478));
#44432=CARTESIAN_POINT('Ctrl Pts',(-6.14352353417009,36.3524357235726,17.9316044801622));
#44433=CARTESIAN_POINT('Ctrl Pts',(-6.10730542645452,36.2386096871451,17.9257929929765));
#44434=CARTESIAN_POINT('Ctrl Pts',(-6.06972575841709,36.1205045476785,17.9197630324673));
#44435=CARTESIAN_POINT('Ctrl Pts',(-6.03749674247662,36.0005959791163,17.9137330719582));
#44436=CARTESIAN_POINT('Ctrl Pts',(-6.01078195992056,35.879411410379,17.907703111449));
#44437=CARTESIAN_POINT('Ctrl Pts',(-5.9850641472194,35.7627493325756,17.9018981832358));
#44438=CARTESIAN_POINT('Ctrl Pts',(-5.96445646557269,35.6449052207303,17.8960932550225));
#44439=CARTESIAN_POINT('Ctrl Pts',(-5.94905364667441,35.5263636029192,17.8902883268093));
#44440=CARTESIAN_POINT('Ctrl Pts',(-5.93365312577556,35.407839670739,17.8844842646533));
#44441=CARTESIAN_POINT('Ctrl Pts',(-5.92345597590759,35.2886188442069,17.8786802024972));
#44442=CARTESIAN_POINT('Ctrl Pts',(-5.91850533560985,35.1691930984252,17.8728761403411));
#44443=CARTESIAN_POINT('Ctrl Pts',(-5.91355426670033,35.0497570131161,17.8670715756866));
#44444=CARTESIAN_POINT('Ctrl Pts',(-5.91385062737332,34.930116381129,17.861267011032));
#44445=CARTESIAN_POINT('Ctrl Pts',(-5.91938545454085,34.8107648780294,17.8554624463774));
#44446=CARTESIAN_POINT('Ctrl Pts',(-5.92492206583707,34.6913749024654,17.8496560106454));
#44447=CARTESIAN_POINT('Ctrl Pts',(-5.93570048298359,34.5722746486728,17.8438495749133));
#44448=CARTESIAN_POINT('Ctrl Pts',(-5.95165978867681,34.4539537259685,17.8380431391813));
#44449=CARTESIAN_POINT('Ctrl Pts',(-5.9676367064291,34.3355022289698,17.8322302956962));
#44450=CARTESIAN_POINT('Ctrl Pts',(-5.98880587063381,34.2178321845306,17.8264174522112));
#44451=CARTESIAN_POINT('Ctrl Pts',(-6.01505501390461,34.1014242058717,17.8206046087261));
#44452=CARTESIAN_POINT('Ctrl Pts',(-6.04132134427662,33.9849400069838,17.8147879591767));
#44453=CARTESIAN_POINT('Ctrl Pts',(-6.07267417110744,33.8697199125778,17.8089713096273));
#44454=CARTESIAN_POINT('Ctrl Pts',(-6.10895148188831,33.7562289480371,17.8031546600778));
#44455=CARTESIAN_POINT('Ctrl Pts',(-6.14528059883978,33.6425759116079,17.7973297040048));
#44456=CARTESIAN_POINT('Ctrl Pts',(-6.186548095489,33.5306573152795,17.7915047479317));
#44457=CARTESIAN_POINT('Ctrl Pts',(-6.23254398375756,33.4209179357365,17.7856797918587));
#44458=CARTESIAN_POINT('Ctrl Pts',(-6.24466712025368,33.3919939269331,17.784144508158));
#44459=CARTESIAN_POINT('Ctrl Pts',(-6.25711848824365,33.3632211702652,17.7826092244573));
#44460=CARTESIAN_POINT('Ctrl Pts',(-6.26989372335423,33.3346075042418,17.7810739407566));
#44461=CARTESIAN_POINT('Ctrl Pts',(-6.31836100253144,33.2260516516537,17.7752493102826));
#44462=CARTESIAN_POINT('Ctrl Pts',(-6.37164897662962,33.1194389214489,17.7694246798086));
#44463=CARTESIAN_POINT('Ctrl Pts',(-6.42957975018663,33.0152269047262,17.7636000493346));
#44464=CARTESIAN_POINT('Ctrl Pts',(-6.48743758471783,32.9111460984555,17.7577827524908));
#44465=CARTESIAN_POINT('Ctrl Pts',(-6.54992639521803,32.809460347201,17.7519654556471));
#44466=CARTESIAN_POINT('Ctrl Pts',(-6.61682048404191,32.710606769731,17.7461481588033));
#44467=CARTESIAN_POINT('Ctrl Pts',(-6.68364776473429,32.611851918814,17.7403366717813));
#44468=CARTESIAN_POINT('Ctrl Pts',(-6.75487134372906,32.5159239507107,17.7345251847593));
#44469=CARTESIAN_POINT('Ctrl Pts',(-6.83022022433124,32.4232343580059,17.7287136977373));
#44470=CARTESIAN_POINT('Ctrl Pts',(-6.90840180963993,32.3270601449139,17.7226837306727));
#44471=CARTESIAN_POINT('Ctrl Pts',(-6.99102474449253,32.2343729681636,17.7166537636082));
#44472=CARTESIAN_POINT('Ctrl Pts',(-7.07773747670501,32.1455987063929,17.7106237965436));
#44473=CARTESIAN_POINT('Ctrl Pts',(-7.16121469147295,32.0601368840445,17.7048188260064));
#44474=CARTESIAN_POINT('Ctrl Pts',(-7.24848165424397,31.9783015195646,17.6990138554693));
#44475=CARTESIAN_POINT('Ctrl Pts',(-7.33918496830152,31.9004373910038,17.6932088849321));
#44476=CARTESIAN_POINT('Ctrl Pts',(-7.4298749923951,31.8225846711933,17.6874047649465));
#44477=CARTESIAN_POINT('Ctrl Pts',(-7.52400005685096,31.7487022959226,17.681600644961));
#44478=CARTESIAN_POINT('Ctrl Pts',(-7.62117226406248,31.6790959660456,17.6757965249754));
#44479=CARTESIAN_POINT('Ctrl Pts',(-7.71835314130074,31.609483425661,17.669991887127));
#44480=CARTESIAN_POINT('Ctrl Pts',(-7.81858137002927,31.5441479269376,17.6641872492786));
#44481=CARTESIAN_POINT('Ctrl Pts',(-7.9214390800406,31.4833525195127,17.6583826114302));
#44482=CARTESIAN_POINT('Ctrl Pts',(-8.02433021534186,31.4225373556289,17.6525760872701));
#44483=CARTESIAN_POINT('Ctrl Pts',(-8.12985218014831,31.3662654248431,17.64676956311));
#44484=CARTESIAN_POINT('Ctrl Pts',(-8.23756203615051,31.3147540891303,17.6409630389498));
#44485=CARTESIAN_POINT('Ctrl Pts',(-8.34539116131664,31.2631857139396,17.6351500851155));
#44486=CARTESIAN_POINT('Ctrl Pts',(-8.45541264515805,31.2163886324068,17.6293371312812));
#44487=CARTESIAN_POINT('Ctrl Pts',(-8.56716293433242,31.1745323235911,17.6235241774469));
#44488=CARTESIAN_POINT('Ctrl Pts',(-8.67898664029595,31.1326485163607,17.6177074046658));
#44489=CARTESIAN_POINT('Ctrl Pts',(-8.79254102629172,31.0957120722684,17.6118906318847));
#44490=CARTESIAN_POINT('Ctrl Pts',(-8.90734831928826,31.0638423171019,17.6060738591037));
#44491=CARTESIAN_POINT('Ctrl Pts',(-9.02231991125934,31.0319269536125,17.6002487620273));
#44492=CARTESIAN_POINT('Ctrl Pts',(-9.13854759271531,31.0050928429122,17.594423664951));
#44493=CARTESIAN_POINT('Ctrl Pts',(-9.25554423799079,30.9834080841575,17.5885985678747));
#44494=CARTESIAN_POINT('Ctrl Pts',(-9.28636843833458,30.9776949686516,17.5870638746458));
#44495=CARTESIAN_POINT('Ctrl Pts',(-9.31724599351994,30.9723390017576,17.585529181417));
#44496=CARTESIAN_POINT('Ctrl Pts',(-9.34816796603897,30.9673408277537,17.5839944881881));
#44497=CARTESIAN_POINT('Ctrl Pts',(-9.4653745462179,30.9483957594282,17.5781773901725));
#44498=CARTESIAN_POINT('Ctrl Pts',(-9.58359933606191,30.9345337715468,17.572360292157));
#44499=CARTESIAN_POINT('Ctrl Pts',(-9.70236334270299,30.9258574619642,17.5665431941414));
#44500=CARTESIAN_POINT('Ctrl Pts',(-9.8209770473109,30.917192132703,17.5607334579662));
#44501=CARTESIAN_POINT('Ctrl Pts',(-9.94012820689428,30.9136994588333,17.5549237217911));
#44502=CARTESIAN_POINT('Ctrl Pts',(-10.0593286541284,30.915430853713,17.5491139856159));
#44503=CARTESIAN_POINT('Ctrl Pts',(-10.1784095075453,30.9171605114842,17.5433100783494));
#44504=CARTESIAN_POINT('Ctrl Pts',(-10.2975391433226,30.9241038056909,17.5375061710829));
#44505=CARTESIAN_POINT('Ctrl Pts',(-10.4162259165701,30.9362602216215,17.5317022638165));
#44506=CARTESIAN_POINT('Ctrl Pts',(-10.53959344679,30.9488960610554,17.5256694626416));
#44507=CARTESIAN_POINT('Ctrl Pts',(-10.6624820156081,30.9671646983021,17.5196366614667));
#44508=CARTESIAN_POINT('Ctrl Pts',(-10.7843409195185,30.9910058216594,17.5136038602919));
#44509=CARTESIAN_POINT('Ctrl Pts',(-10.9014446806331,31.0139166236176,17.5078064693343));
#44510=CARTESIAN_POINT('Ctrl Pts',(-11.0175971881947,31.0419730899628,17.5020090783767));
#44511=CARTESIAN_POINT('Ctrl Pts',(-11.1323173311832,31.0750691137929,17.4962116874191));
#44512=CARTESIAN_POINT('Ctrl Pts',(-11.2470208997623,31.1081603560126,17.4904151340505));
#44513=CARTESIAN_POINT('Ctrl Pts',(-11.3602921220666,31.146289594431,17.4846185806819));
#44514=CARTESIAN_POINT('Ctrl Pts',(-11.4716636378013,31.1893004399227,17.4788220273133));
#44515=CARTESIAN_POINT('Ctrl Pts',(-11.5830455072493,31.2323152839409,17.473024935065));
#44516=CARTESIAN_POINT('Ctrl Pts',(-11.692526937101,31.2802124898519,17.4672278428167));
#44517=CARTESIAN_POINT('Ctrl Pts',(-11.7996598050395,31.3327872183189,17.4614307505684));
#44518=CARTESIAN_POINT('Ctrl Pts',(-11.9068280705152,31.3853793178872,17.4556317429154));
#44519=CARTESIAN_POINT('Ctrl Pts',(-12.0116458635929,31.4426518332669,17.4498327352625));
#44520=CARTESIAN_POINT('Ctrl Pts',(-12.1136895424318,31.5043539197719,17.4440337276096));
#44521=CARTESIAN_POINT('Ctrl Pts',(-12.2158477829119,31.5661252775181,17.4382282095698));
#44522=CARTESIAN_POINT('Ctrl Pts',(-12.3152253421021,31.6323359207464,17.4324226915299));
#44523=CARTESIAN_POINT('Ctrl Pts',(-12.4114273401869,31.7026915244401,17.4266171734901));
#44524=CARTESIAN_POINT('Ctrl Pts',(-12.5076932531773,31.7730938711522,17.4208077983667));
#44525=CARTESIAN_POINT('Ctrl Pts',(-12.600779084965,31.8476464069538,17.4149984232434));
#44526=CARTESIAN_POINT('Ctrl Pts',(-12.6903241425304,31.926015450898,17.4091890481201));
#44527=CARTESIAN_POINT('Ctrl Pts',(-12.7799992418815,32.0044983062651,17.4033712363333));
#44528=CARTESIAN_POINT('Ctrl Pts',(-12.8661230090778,32.0868084503061,17.3975534245465));
#44529=CARTESIAN_POINT('Ctrl Pts',(-12.948372500504,32.1725763320168,17.3917356127597));
#44530=CARTESIAN_POINT('Ctrl Pts',(-12.9710895192435,32.1962651177136,17.390128753713));
#44531=CARTESIAN_POINT('Ctrl Pts',(-12.9935112341829,32.220217488981,17.3885218946664));
#44532=CARTESIAN_POINT('Ctrl Pts',(-13.0156314083634,32.2444252489014,17.3869150356197));
#44533=CARTESIAN_POINT('Ctrl Pts',(-13.0950954777897,32.3313887194088,17.3811425874553));
#44534=CARTESIAN_POINT('Ctrl Pts',(-13.1709349916773,32.4219460065299,17.3753701392909));
#44535=CARTESIAN_POINT('Ctrl Pts',(-13.2428036170308,32.515759733566,17.3695976911265));
#44536=CARTESIAN_POINT('Ctrl Pts',(-13.3145580842969,32.6094244443158,17.3638344120765));
#44537=CARTESIAN_POINT('Ctrl Pts',(-13.3823539658873,32.7063349721867,17.3580711330264));
#44538=CARTESIAN_POINT('Ctrl Pts',(-13.4458827470682,32.8061182590081,17.3523078539764));
#44539=CARTESIAN_POINT('Ctrl Pts',(-13.5093535973036,32.9058105549425,17.3465498303743));
#44540=CARTESIAN_POINT('Ctrl Pts',(-13.5685648588005,33.0083700540876,17.3407918067722));
#44541=CARTESIAN_POINT('Ctrl Pts',(-13.6232492660118,33.1133919971692,17.3350337831701));
#44542=CARTESIAN_POINT('Ctrl Pts',(-13.6778973144575,33.2183441128832,17.3292795879835));
#44543=CARTESIAN_POINT('Ctrl Pts',(-13.728024301,33.3257550493138,17.3235253927969));
#44544=CARTESIAN_POINT('Ctrl Pts',(-13.7734075587941,33.4351931763838,17.3177711976103));
#44545=CARTESIAN_POINT('Ctrl Pts',(-13.8187718496968,33.5445855662994,17.3120194072575));
#44546=CARTESIAN_POINT('Ctrl Pts',(-13.859396196102,33.6560030774838,17.3062676169047));
#44547=CARTESIAN_POINT('Ctrl Pts',(-13.8951052977852,33.768992396788,17.300515826552));
#44548=CARTESIAN_POINT('Ctrl Pts',(-13.93081740448,33.8819912244305,17.2947635521715));
#44549=CARTESIAN_POINT('Ctrl Pts',(-13.9616133050997,33.9965617302525,17.2890112777909));
#44550=CARTESIAN_POINT('Ctrl Pts',(-13.9873671243155,34.11223403088,17.2832590034104));
#44551=CARTESIAN_POINT('Ctrl Pts',(-14.0131218752288,34.227910516191,17.2775065209295));
#44552=CARTESIAN_POINT('Ctrl Pts',(-14.033834098558,34.3446884673207,17.2717540384486));
#44553=CARTESIAN_POINT('Ctrl Pts',(-14.0494289930285,34.4620875253162,17.2660015559677));
#44554=CARTESIAN_POINT('Ctrl Pts',(-14.0650344310494,34.5795659556281,17.2602451842916));
#44555=CARTESIAN_POINT('Ctrl Pts',(-14.0755155851035,34.6976659171536,17.2544888126154));
#44556=CARTESIAN_POINT('Ctrl Pts',(-14.0808495272278,34.815901830198,17.2487324409393));
#44557=CARTESIAN_POINT('Ctrl Pts',(-14.0836656385158,34.8783257338717,17.2456933034914));
#44558=CARTESIAN_POINT('Ctrl Pts',(-14.0850478790537,34.9407874999945,17.2426541660434));
#44559=CARTESIAN_POINT('Ctrl Pts',(-14.0849987342309,35.0032157940822,17.2396150285955));
#44560=CARTESIAN_POINT('Origin',(-10.,35.,32.7603849714045));
#44561=CARTESIAN_POINT('',(-7.51282733495084,38.2405550657615,19.2967866609659));
#44562=CARTESIAN_POINT('',(-7.51282733495087,38.2405550657615,19.1927507857623));
#44563=CARTESIAN_POINT('',(-7.51282733495086,38.2405550657615,32.7603849714045));
#44564=CARTESIAN_POINT('',(-14.0849999333317,35.0007380241213,18.3853849714444));
#44565=CARTESIAN_POINT('Ctrl Pts',(-7.51282733495087,38.2405550657615,19.1927507857623));
#44566=CARTESIAN_POINT('Ctrl Pts',(-7.41816085919388,38.1678971827688,19.1869271965536));
#44567=CARTESIAN_POINT('Ctrl Pts',(-7.32679476472752,38.0911750994162,19.1811036073449));
#44568=CARTESIAN_POINT('Ctrl Pts',(-7.23907757352064,38.0107361815615,19.1752800181361));
#44569=CARTESIAN_POINT('Ctrl Pts',(-7.20189334496105,37.9766372886826,19.1728113381751));
#44570=CARTESIAN_POINT('Ctrl Pts',(-7.16536434784443,37.941870910604,19.170342658214));
#44571=CARTESIAN_POINT('Ctrl Pts',(-7.12951495706164,37.9064653134464,19.1678739782529));
#44572=CARTESIAN_POINT('Ctrl Pts',(-7.04494813906446,37.8229453811538,19.1620504927095));
#44573=CARTESIAN_POINT('Ctrl Pts',(-6.96389310497571,37.7355968276586,19.1562270071662));
#44574=CARTESIAN_POINT('Ctrl Pts',(-6.88671567260117,37.6447468114685,19.1504035216228));
#44575=CARTESIAN_POINT('Ctrl Pts',(-6.80963561420458,37.5540114198157,19.1445873835116));
#44576=CARTESIAN_POINT('Ctrl Pts',(-6.73642368884896,37.459783660754,19.1387712454005));
#44577=CARTESIAN_POINT('Ctrl Pts',(-6.66740975917089,37.3624282606527,19.1329551072893));
#44578=CARTESIAN_POINT('Ctrl Pts',(-6.59846491381403,37.2651703152503,19.1271447912485));
#44579=CARTESIAN_POINT('Ctrl Pts',(-6.53370993903152,37.1647912884284,19.1213344752077));
#44580=CARTESIAN_POINT('Ctrl Pts',(-6.47343479399331,37.0616893189283,19.1155241591669));
#44581=CARTESIAN_POINT('Ctrl Pts',(-6.41087652415465,36.9546820139306,19.1094937577718));
#44582=CARTESIAN_POINT('Ctrl Pts',(-6.35314446173313,36.8447417480414,19.1034633563767));
#44583=CARTESIAN_POINT('Ctrl Pts',(-6.3005139448485,36.7323475193331,19.0974329549816));
#44584=CARTESIAN_POINT('Ctrl Pts',(-6.24986130149476,36.6241771056878,19.0916291782143));
#44585=CARTESIAN_POINT('Ctrl Pts',(-6.20393387604689,36.5137342455091,19.085825401447));
#44586=CARTESIAN_POINT('Ctrl Pts',(-6.16293020497594,36.401470794599,19.0800216246797));
#44587=CARTESIAN_POINT('Ctrl Pts',(-6.12193258746479,36.2892239176565,19.0742187047505));
#44588=CARTESIAN_POINT('Ctrl Pts',(-6.08585741878447,36.1751573679706,19.0684157848214));
#44589=CARTESIAN_POINT('Ctrl Pts',(-6.05485452695307,36.0597415706187,19.0626128648922));
#44590=CARTESIAN_POINT('Ctrl Pts',(-6.02384889478502,35.9443155716977,19.0568094320447));
#44591=CARTESIAN_POINT('Ctrl Pts',(-5.99791653680995,35.8275404823864,19.0510059991971));
#44592=CARTESIAN_POINT('Ctrl Pts',(-5.97715681697477,35.7098997991177,19.0452025663495));
#44593=CARTESIAN_POINT('Ctrl Pts',(-5.95639036242527,35.5922209517313,19.0393972507953));
#44594=CARTESIAN_POINT('Ctrl Pts',(-5.94079995424183,35.4736763538543,19.0335919352411));
#44595=CARTESIAN_POINT('Ctrl Pts',(-5.93043337277146,35.3547569119097,19.0277866196869));
#44596=CARTESIAN_POINT('Ctrl Pts',(-5.92005530830509,35.2357057436598,19.0219748736218));
#44597=CARTESIAN_POINT('Ctrl Pts',(-5.91491265618143,35.1162793095952,19.0161631275567));
#44598=CARTESIAN_POINT('Ctrl Pts',(-5.91500112300383,34.9969709836484,19.0103513814916));
#44599=CARTESIAN_POINT('Ctrl Pts',(-5.91508964794459,34.8775842779968,19.004535817395));
#44600=CARTESIAN_POINT('Ctrl Pts',(-5.92041611769691,34.7583162419962,18.9987202532984));
#44601=CARTESIAN_POINT('Ctrl Pts',(-5.93092428797763,34.6396559285493,18.9929046892019));
#44602=CARTESIAN_POINT('Ctrl Pts',(-5.94144751381989,34.5208256047578,18.9870807928666));
#44603=CARTESIAN_POINT('Ctrl Pts',(-5.95716720459475,34.4026051447689,18.9812568965313));
#44604=CARTESIAN_POINT('Ctrl Pts',(-5.97797587157177,34.2854743459181,18.9754330001961));
#44605=CARTESIAN_POINT('Ctrl Pts',(-5.98350026428286,34.2543778546277,18.9738868420255));
#44606=CARTESIAN_POINT('Ctrl Pts',(-5.98938306682778,34.2233580850842,18.972340683855));
#44607=CARTESIAN_POINT('Ctrl Pts',(-5.99562168069339,34.1924238265853,18.9707945256844));
#44608=CARTESIAN_POINT('Ctrl Pts',(-6.01911980050726,34.0759080542969,18.9649708265863));
#44609=CARTESIAN_POINT('Ctrl Pts',(-6.04774543487043,33.9602308548337,18.9591471274881));
#44610=CARTESIAN_POINT('Ctrl Pts',(-6.08142546695665,33.8458775502642,18.95332342839));
#44611=CARTESIAN_POINT('Ctrl Pts',(-6.1150630040176,33.7316685284126,18.9475070772136));
#44612=CARTESIAN_POINT('Ctrl Pts',(-6.15374214020114,33.6187804673103,18.9416907260373));
#44613=CARTESIAN_POINT('Ctrl Pts',(-6.19733862899554,33.5076892088206,18.9358743748609));
#44614=CARTESIAN_POINT('Ctrl Pts',(-6.24089147294573,33.3967091648072,18.9300638464869));
#44615=CARTESIAN_POINT('Ctrl Pts',(-6.28935172787708,33.2875227228382,18.924253318113));
#44616=CARTESIAN_POINT('Ctrl Pts',(-6.34254532887773,33.1805906648899,18.918442789739));
#44617=CARTESIAN_POINT('Ctrl Pts',(-6.3977510686166,33.0696137193591,18.9124124682131));
#44618=CARTESIAN_POINT('Ctrl Pts',(-6.45805519237411,32.9610655072652,18.9063821466871));
#44619=CARTESIAN_POINT('Ctrl Pts',(-6.52320802882969,32.8554388352846,18.9003518251611));
#44620=CARTESIAN_POINT('Ctrl Pts',(-6.58591548917144,32.7537766405961,18.8945478392028));
#44621=CARTESIAN_POINT('Ctrl Pts',(-6.65311401549713,32.6548210093335,18.8887438532444));
#44622=CARTESIAN_POINT('Ctrl Pts',(-6.72453450385764,32.5589857059859,18.882939867286));
#44623=CARTESIAN_POINT('Ctrl Pts',(-6.7959444298385,32.4631645757263,18.8771367396794));
#44624=CARTESIAN_POINT('Ctrl Pts',(-6.87157483221681,32.370463182986,18.8713336120728));
#44625=CARTESIAN_POINT('Ctrl Pts',(-6.95111437587402,32.2812647331897,18.8655304844662));
#44626=CARTESIAN_POINT('Ctrl Pts',(-7.0306609260148,32.1920584260756,18.8597268456733));
#44627=CARTESIAN_POINT('Ctrl Pts',(-7.11411703031398,32.1063559801816,18.8539232068805));
#44628=CARTESIAN_POINT('Ctrl Pts',(-7.20113275808643,32.0245055600551,18.8481195680877));
#44629=CARTESIAN_POINT('Ctrl Pts',(-7.28817668458438,31.9426286150969,18.8423140485404));
#44630=CARTESIAN_POINT('Ctrl Pts',(-7.37878223143703,31.8646064581257,18.8365085289932));
#44631=CARTESIAN_POINT('Ctrl Pts',(-7.4725649933112,31.7907481733332,18.8307030094459));
#44632=CARTESIAN_POINT('Ctrl Pts',(-7.56645157108528,31.7168081286933,18.8248910632886));
#44633=CARTESIAN_POINT('Ctrl Pts',(-7.66352206338473,31.6470414096444,18.8190791171313));
#44634=CARTESIAN_POINT('Ctrl Pts',(-7.76336145521262,31.5817149007183,18.8132671709741));
#44635=CARTESIAN_POINT('Ctrl Pts',(-7.86326639937157,31.5163454998548,18.8074514088218));
#44636=CARTESIAN_POINT('Ctrl Pts',(-7.96594351330009,31.4554223229835,18.8016356466695));
#44637=CARTESIAN_POINT('Ctrl Pts',(-8.07095291650907,31.3991664368267,18.7958198845173));
#44638=CARTESIAN_POINT('Ctrl Pts',(-8.17611268573994,31.3428299962286,18.7899957946058));
#44639=CARTESIAN_POINT('Ctrl Pts',(-8.28361104332895,31.2911743619366,18.7841717046944));
#44640=CARTESIAN_POINT('Ctrl Pts',(-8.39298775763767,31.2443726685283,18.778347614783));
#44641=CARTESIAN_POINT('Ctrl Pts',(-8.42198754954446,31.2319638173545,18.7768034342273));
#44642=CARTESIAN_POINT('Ctrl Pts',(-8.45111930268121,31.2198959143175,18.7752592536717));
#44643=CARTESIAN_POINT('Ctrl Pts',(-8.48037427561966,31.2081715943622,18.773715073116));
#44644=CARTESIAN_POINT('Ctrl Pts',(-8.59070780167218,31.1639539646294,18.7678912808354));
#44645=CARTESIAN_POINT('Ctrl Pts',(-8.70315069552679,31.1244847482118,18.7620674885548));
#44646=CARTESIAN_POINT('Ctrl Pts',(-8.81725694322182,31.089968815771,18.7562436962742));
#44647=CARTESIAN_POINT('Ctrl Pts',(-8.93121926730304,31.0554964187004,18.7504272496145));
#44648=CARTESIAN_POINT('Ctrl Pts',(-9.04684038495362,31.0259649963554,18.7446108029547));
#44649=CARTESIAN_POINT('Ctrl Pts',(-9.16365418619704,31.0015314582037,18.738794356295));
#44650=CARTESIAN_POINT('Ctrl Pts',(-9.28035108931023,30.977122371229,18.7329837302808));
#44651=CARTESIAN_POINT('Ctrl Pts',(-9.39823790424308,30.9578011026136,18.7271731042667));
#44652=CARTESIAN_POINT('Ctrl Pts',(-9.51683381037535,30.9436746391341,18.7213624782525));
#44653=CARTESIAN_POINT('Ctrl Pts',(-9.63991301037189,30.9290141514282,18.7153321925148));
#44654=CARTESIAN_POINT('Ctrl Pts',(-9.76375554226951,30.9199491087418,18.7093019067771));
#44655=CARTESIAN_POINT('Ctrl Pts',(-9.88781239446962,30.9165408118649,18.7032716210394));
#44656=CARTESIAN_POINT('Ctrl Pts',(-10.0072158449064,30.913260361007,18.6974675327409));
#44657=CARTESIAN_POINT('Ctrl Pts',(-10.1268173820277,30.9152199397431,18.6916634444424));
#44658=CARTESIAN_POINT('Ctrl Pts',(-10.2461234163943,30.9224212743465,18.685859356144));
#44659=CARTESIAN_POINT('Ctrl Pts',(-10.3654118386774,30.9296215458811,18.6800561246511));
#44660=CARTESIAN_POINT('Ctrl Pts',(-10.4844044375049,30.9420620098548,18.6742528931583));
#44661=CARTESIAN_POINT('Ctrl Pts',(-10.6026100342064,30.9596923202962,18.6684496616655));
#44662=CARTESIAN_POINT('Ctrl Pts',(-10.7208260722507,30.977324188059,18.6626459175614));
#44663=CARTESIAN_POINT('Ctrl Pts',(-10.8382545660942,31.0001467535251,18.6568421734572));
#44664=CARTESIAN_POINT('Ctrl Pts',(-10.9544124889484,31.0280581825838,18.6510384293531));
#44665=CARTESIAN_POINT('Ctrl Pts',(-11.0706080799226,31.0559786628638,18.6452328031894));
#44666=CARTESIAN_POINT('Ctrl Pts',(-11.1855318836809,31.0889911933418,18.6394271770257));
#44667=CARTESIAN_POINT('Ctrl Pts',(-11.2987146624959,31.1269436841923,18.633621550862));
#44668=CARTESIAN_POINT('Ctrl Pts',(-11.4120227572256,31.1649381960212,18.6278094967119));
#44669=CARTESIAN_POINT('Ctrl Pts',(-11.5235855918826,31.207883455975,18.6219974425619));
#44670=CARTESIAN_POINT('Ctrl Pts',(-11.6329524450306,31.2555786411959,18.6161853884119));
#44671=CARTESIAN_POINT('Ctrl Pts',(-11.7423911221245,31.303305149037,18.6103695173406));
#44672=CARTESIAN_POINT('Ctrl Pts',(-11.8496305797145,31.3557876154431,18.6045536462694));
#44673=CARTESIAN_POINT('Ctrl Pts',(-11.9542447873468,31.412779305489,18.5987377751982));
#44674=CARTESIAN_POINT('Ctrl Pts',(-12.0590088014886,31.4698526070708,18.5929135758571));
#44675=CARTESIAN_POINT('Ctrl Pts',(-12.1611397138472,31.5314478103286,18.5870893765161));
#44676=CARTESIAN_POINT('Ctrl Pts',(-12.2602404277346,31.5972748849144,18.5812651771751));
#44677=CARTESIAN_POINT('Ctrl Pts',(-12.2864982496202,31.6147164908517,18.5797219916326));
#44678=CARTESIAN_POINT('Ctrl Pts',(-12.3125435203847,31.6324549745908,18.5781788060901));
#44679=CARTESIAN_POINT('Ctrl Pts',(-12.3383692581764,31.6504844809412,18.5766356205475));
#44680=CARTESIAN_POINT('Ctrl Pts',(-12.4353485371795,31.7181878139787,18.5708407417144));
#44681=CARTESIAN_POINT('Ctrl Pts',(-12.529549225962,31.7902211139549,18.5650458628812));
#44682=CARTESIAN_POINT('Ctrl Pts',(-12.6205578142079,31.8663277544718,18.559250984048));
#44683=CARTESIAN_POINT('Ctrl Pts',(-12.7114512408163,31.9423380901725,18.5534634380144));
#44684=CARTESIAN_POINT('Ctrl Pts',(-12.7991602853564,32.0224112542013,18.5476758919808));
#44685=CARTESIAN_POINT('Ctrl Pts',(-12.8833003257636,32.1062473790161,18.5418883459472));
#44686=CARTESIAN_POINT('Ctrl Pts',(-12.9673564177595,32.1899998586429,18.5361065742784));
#44687=CARTESIAN_POINT('Ctrl Pts',(-13.047850297363,32.2775075419245,18.5303248026097));
#44688=CARTESIAN_POINT('Ctrl Pts',(-13.1244308869851,32.3684307661675,18.524543030941));
#44689=CARTESIAN_POINT('Ctrl Pts',(-13.2012297678581,32.4596131650193,18.518744778462));
#44690=CARTESIAN_POINT('Ctrl Pts',(-13.274092698496,32.5542303324158,18.5129465259829));
#44691=CARTESIAN_POINT('Ctrl Pts',(-13.342703073328,32.6519026503223,18.5071482735039));
#44692=CARTESIAN_POINT('Ctrl Pts',(-13.4110440602726,32.7491914731751,18.5013727869548));
#44693=CARTESIAN_POINT('Ctrl Pts',(-13.4751655872742,32.849511157776,18.4955973004057));
#44694=CARTESIAN_POINT('Ctrl Pts',(-13.5347959679208,32.9524545267148,18.4898218138566));
#44695=CARTESIAN_POINT('Ctrl Pts',(-13.5944183664386,33.0553841156436,18.4840471004147));
#44696=CARTESIAN_POINT('Ctrl Pts',(-13.6495506071614,33.1609363333146,18.4782723869729));
#44697=CARTESIAN_POINT('Ctrl Pts',(-13.6999657706881,33.2686772987867,18.472497673531));
#44698=CARTESIAN_POINT('Ctrl Pts',(-13.7503864001868,33.3764299454487,18.4667223339993));
#44699=CARTESIAN_POINT('Ctrl Pts',(-13.7960887610852,33.4863714375386,18.4609469944676));
#44700=CARTESIAN_POINT('Ctrl Pts',(-13.8368934036505,33.598046359888,18.4551716549359));
#44701=CARTESIAN_POINT('Ctrl Pts',(-13.8779821953434,33.7104989469777,18.4493560979783));
#44702=CARTESIAN_POINT('Ctrl Pts',(-13.9141046401688,33.8247088036354,18.4435405410206));
#44703=CARTESIAN_POINT('Ctrl Pts',(-13.9451284266687,33.9401949721339,18.437724984063));
#44704=CARTESIAN_POINT('Ctrl Pts',(-13.9759825901072,34.0550497181122,18.4319412237584));
#44705=CARTESIAN_POINT('Ctrl Pts',(-14.0017936775757,34.1711664361819,18.4261574634538));
#44706=CARTESIAN_POINT('Ctrl Pts',(-14.0224830443867,34.2880623920447,18.4203737031492));
#44707=CARTESIAN_POINT('Ctrl Pts',(-14.0433430232002,34.4059223142426,18.4145422478651));
#44708=CARTESIAN_POINT('Ctrl Pts',(-14.0589963762885,34.5245739590227,18.408710792581));
#44709=CARTESIAN_POINT('Ctrl Pts',(-14.069415969644,34.6435190523933,18.4028793372968));
#44710=CARTESIAN_POINT('Ctrl Pts',(-14.0798355629994,34.7624641457639,18.3970478820127));
#44711=CARTESIAN_POINT('Ctrl Pts',(-14.0850214391494,34.8817022618907,18.3912164267285));
#44712=CARTESIAN_POINT('Ctrl Pts',(-14.0849999333317,35.0007380241213,18.3853849714444));
#44713=CARTESIAN_POINT('Ctrl Pts',(-14.0849999333316,35.0007380249352,18.3853849714045));
#44714=CARTESIAN_POINT('Ctrl Pts',(-14.0849927679777,35.0403985684774,18.3834420369294));
#44715=CARTESIAN_POINT('Ctrl Pts',(-14.0844080310192,35.0800533014694,18.3814991024543));
#44716=CARTESIAN_POINT('Ctrl Pts',(-14.0832461438359,35.119690972297,18.3795561679791));
#44717=CARTESIAN_POINT('Ctrl Pts',(-14.0797629567325,35.2385195692697,18.3737315023802));
#44718=CARTESIAN_POINT('Ctrl Pts',(-14.071082720807,35.3573873330334,18.3679068367812));
#44719=CARTESIAN_POINT('Ctrl Pts',(-14.0571955944118,35.475803434924,18.3620821711823));
#44720=CARTESIAN_POINT('Ctrl Pts',(-14.043325994456,35.5940700881394,18.3562648566829));
#44721=CARTESIAN_POINT('Ctrl Pts',(-14.0242626216709,35.7118858114284,18.3504475421835));
#44722=CARTESIAN_POINT('Ctrl Pts',(-14.0000476306313,35.828760491747,18.3446302276842));
#44723=CARTESIAN_POINT('Ctrl Pts',(-13.9758568951768,35.9455181014567,18.3388187402515));
#44724=CARTESIAN_POINT('Ctrl Pts',(-13.9465248895661,36.0613361460438,18.3330072528187));
#44725=CARTESIAN_POINT('Ctrl Pts',(-13.9121454139528,36.1757309471506,18.327195765386));
#44726=CARTESIAN_POINT('Ctrl Pts',(-13.8764735004439,36.2944262261845,18.3211658049704));
#44727=CARTESIAN_POINT('Ctrl Pts',(-13.8353672182095,36.4115887078271,18.3151358445547));
#44728=CARTESIAN_POINT('Ctrl Pts',(-13.7889893690839,36.5266907221075,18.3091058841391));
#44729=CARTESIAN_POINT('Ctrl Pts',(-13.7443422939109,36.6374972467962,18.3033009556863));
#44730=CARTESIAN_POINT('Ctrl Pts',(-13.6948102278603,36.7463939255093,18.2974960272336));
#44731=CARTESIAN_POINT('Ctrl Pts',(-13.6405885728166,36.8529273713444,18.2916910987808));
#44732=CARTESIAN_POINT('Ctrl Pts',(-13.5863750073168,36.9594449230317,18.2858870363884));
#44733=CARTESIAN_POINT('Ctrl Pts',(-13.5274734293382,37.0635995793517,18.2800829739959));
#44734=CARTESIAN_POINT('Ctrl Pts',(-13.4641260272299,37.1649609390167,18.2742789116035));
#44735=CARTESIAN_POINT('Ctrl Pts',(-13.4007731407284,37.2663310741887,18.2684743467159));
#44736=CARTESIAN_POINT('Ctrl Pts',(-13.3329738811572,37.3649070857318,18.2626697818283));
#44737=CARTESIAN_POINT('Ctrl Pts',(-13.2610143982138,37.4602865879085,18.2568652169407));
#44738=CARTESIAN_POINT('Ctrl Pts',(-13.1890317194737,37.5556968352134,18.2510587809793));
#44739=CARTESIAN_POINT('Ctrl Pts',(-13.112886396056,37.6479081982739,18.2452523450179));
#44740=CARTESIAN_POINT('Ctrl Pts',(-13.0329051611896,37.7365509831227,18.2394459090565));
#44741=CARTESIAN_POINT('Ctrl Pts',(-12.9528356622855,37.8252915905434,18.2336330653485));
#44742=CARTESIAN_POINT('Ctrl Pts',(-12.868922075769,37.9104554556389,18.2278202216405));
#44743=CARTESIAN_POINT('Ctrl Pts',(-12.7815284361686,37.9917093038572,18.2220073779326));
#44744=CARTESIAN_POINT('Ctrl Pts',(-12.694077574057,38.073016354451,18.2161907281637));
#44745=CARTESIAN_POINT('Ctrl Pts',(-12.6031424309925,38.150408025542,18.2103740783949));
#44746=CARTESIAN_POINT('Ctrl Pts',(-12.5091192961749,38.2235919961376,18.204557428626));
#44747=CARTESIAN_POINT('Ctrl Pts',(-12.4149618908088,38.2968804777337,18.1987324723403));
#44748=CARTESIAN_POINT('Ctrl Pts',(-12.3177080234843,38.365949029947,18.1929075160545));
#44749=CARTESIAN_POINT('Ctrl Pts',(-12.2177821458632,38.4305491329363,18.1870825597688));
#44750=CARTESIAN_POINT('Ctrl Pts',(-12.1914447213347,38.4475757568452,18.1855472783161));
#44751=CARTESIAN_POINT('Ctrl Pts',(-12.1649218010831,38.4642922135478,18.1840119968634));
#44752=CARTESIAN_POINT('Ctrl Pts',(-12.1382214131198,38.4806944980098,18.1824767154107));
#44753=CARTESIAN_POINT('Ctrl Pts',(-12.0369240773754,38.5429223472234,18.1766520839113));
#44754=CARTESIAN_POINT('Ctrl Pts',(-11.9327452401376,38.6008244834567,18.1708274524119));
#44755=CARTESIAN_POINT('Ctrl Pts',(-11.8260901017685,38.6541236897816,18.1650028209125));
#44756=CARTESIAN_POINT('Ctrl Pts',(-11.7195692497886,38.7073557886228,18.1591855230376));
#44757=CARTESIAN_POINT('Ctrl Pts',(-11.6105786599547,38.7559963037591,18.1533682251627));
#44758=CARTESIAN_POINT('Ctrl Pts',(-11.4995514257018,38.7998119060916,18.1475509272877));
#44759=CARTESIAN_POINT('Ctrl Pts',(-11.38863507591,38.8435837491656,18.14173943923));
#44760=CARTESIAN_POINT('Ctrl Pts',(-11.2756865056747,38.8825401167798,18.1359279511724));
#44761=CARTESIAN_POINT('Ctrl Pts',(-11.1611617254819,38.9164944079209,18.1301164631147));
#44762=CARTESIAN_POINT('Ctrl Pts',(-11.042331470388,38.9517251856709,18.1240864964367));
#44763=CARTESIAN_POINT('Ctrl Pts',(-10.9218045669189,38.9815702060192,18.1180565297586));
#44764=CARTESIAN_POINT('Ctrl Pts',(-10.8001116333098,39.0058764801529,18.1120265630806));
#44765=CARTESIAN_POINT('Ctrl Pts',(-10.6829594070215,39.0292758184964,18.1062215915032));
#44766=CARTESIAN_POINT('Ctrl Pts',(-10.5647270436356,39.0475422523483,18.1004166199258));
#44767=CARTESIAN_POINT('Ctrl Pts',(-10.4459008909407,39.0605907692672,18.0946116483484));
#44768=CARTESIAN_POINT('Ctrl Pts',(-10.3270921488026,39.0736373743011,18.0888075273226));
#44769=CARTESIAN_POINT('Ctrl Pts',(-10.2076901959899,39.081467538296,18.0830034062969));
#44770=CARTESIAN_POINT('Ctrl Pts',(-10.0881877902054,39.084047981312,18.0771992852712));
#44771=CARTESIAN_POINT('Ctrl Pts',(-9.96867472204712,39.0866286545631,18.0713946463839));
#44772=CARTESIAN_POINT('Ctrl Pts',(-9.84906159118034,39.0839586667239,18.0655900074966));
#44773=CARTESIAN_POINT('Ctrl Pts',(-9.72984180982053,39.0760568632293,18.0597853686093));
#44774=CARTESIAN_POINT('Ctrl Pts',(-9.61058328610529,39.0681524919187,18.0539788434127));
#44775=CARTESIAN_POINT('Ctrl Pts',(-9.49171877317047,39.055012950657,18.048172318216));
#44776=CARTESIAN_POINT('Ctrl Pts',(-9.37373657538421,39.0367089470246,18.0423657930194));
#44777=CARTESIAN_POINT('Ctrl Pts',(-9.25562373387619,39.0183846750534,18.0365528381573));
#44778=CARTESIAN_POINT('Ctrl Pts',(-9.13839556127501,38.9948845882849,18.0307398832953));
#44779=CARTESIAN_POINT('Ctrl Pts',(-9.02253033929591,38.9663305538499,18.0249269284332));
#44780=CARTESIAN_POINT('Ctrl Pts',(-8.90658899722417,38.9377577602418,18.0191101546282));
#44781=CARTESIAN_POINT('Ctrl Pts',(-8.79201277977996,38.9041245211396,18.0132933808233));
#44782=CARTESIAN_POINT('Ctrl Pts',(-8.67926338579312,38.8656021259169,18.0074766070184));
#44783=CARTESIAN_POINT('Ctrl Pts',(-8.56635263814957,38.8270246019781,18.0016515089317));
#44784=CARTESIAN_POINT('Ctrl Pts',(-8.45527431078127,38.7835441049257,17.9958264108449));
#44785=CARTESIAN_POINT('Ctrl Pts',(-8.34646889662311,38.7353794840906,17.9900013127582));
#44786=CARTESIAN_POINT('Ctrl Pts',(-8.31780296685609,38.7226900085825,17.9884666294529));
#44787=CARTESIAN_POINT('Ctrl Pts',(-8.28929466225861,38.7096756441621,17.9869319461476));
#44788=CARTESIAN_POINT('Ctrl Pts',(-8.26095172288859,38.6963409055275,17.9853972628422));
#44789=CARTESIAN_POINT('Ctrl Pts',(-8.15351046874027,38.6457921242617,17.9795796482013));
#44790=CARTESIAN_POINT('Ctrl Pts',(-8.04809935594169,38.5904723324018,17.9737620335603));
#44791=CARTESIAN_POINT('Ctrl Pts',(-7.94517176492508,38.530567365784,17.9679444189194));
#44792=CARTESIAN_POINT('Ctrl Pts',(-7.8423892622281,38.470746842131,17.9621350048778));
#44793=CARTESIAN_POINT('Ctrl Pts',(-7.74208366574298,38.4063542092715,17.9563255908361));
#44794=CARTESIAN_POINT('Ctrl Pts',(-7.64468683351894,38.3376226401139,17.9505161767945));
#44795=CARTESIAN_POINT('Ctrl Pts',(-7.60011147230471,38.3061664371548,17.9478573970022));
#44796=CARTESIAN_POINT('Ctrl Pts',(-7.55614507346746,38.2738020536891,17.9451986172099));
#44797=CARTESIAN_POINT('Ctrl Pts',(-7.51282733495087,38.2405550657615,17.9425398374177));
#44798=CARTESIAN_POINT('',(-14.0849995332602,34.9980472419391,18.4896150286338));
#44799=CARTESIAN_POINT('Ctrl Pts',(-14.0849995332606,34.9980472427294,18.4896150285955));
#44800=CARTESIAN_POINT('Ctrl Pts',(-14.0850575831595,35.1194826169903,18.4837275467034));
#44801=CARTESIAN_POINT('Ctrl Pts',(-14.079696394968,35.2409097711324,18.4778400648113));
#44802=CARTESIAN_POINT('Ctrl Pts',(-14.0689446252189,35.3618212775702,18.4719525829192));
#44803=CARTESIAN_POINT('Ctrl Pts',(-14.0581894988055,35.4827705321505,18.4660632629762));
#44804=CARTESIAN_POINT('Ctrl Pts',(-14.0420404743837,35.6032034284576,18.4601739430332));
#44805=CARTESIAN_POINT('Ctrl Pts',(-14.0205780237788,35.7226184018604,18.4542846230902));
#44806=CARTESIAN_POINT('Ctrl Pts',(-13.9991044168668,35.8420954478629,18.4483922418444));
#44807=CARTESIAN_POINT('Ctrl Pts',(-13.9723119534402,35.9605531323285,18.4424998605985));
#44808=CARTESIAN_POINT('Ctrl Pts',(-13.9403319792833,36.0775012264666,18.4366074793527));
#44809=CARTESIAN_POINT('Ctrl Pts',(-13.9083066364416,36.1946152300958,18.4307067388259));
#44810=CARTESIAN_POINT('Ctrl Pts',(-13.8710791873055,36.3102149878166,18.4248059982991));
#44811=CARTESIAN_POINT('Ctrl Pts',(-13.8288307107525,36.4238259684381,18.4189052577723));
#44812=CARTESIAN_POINT('Ctrl Pts',(-13.7865496276371,36.5375246318313,18.4129999631674));
#44813=CARTESIAN_POINT('Ctrl Pts',(-13.7392399463767,36.6492310991074,18.4070946685624));
#44814=CARTESIAN_POINT('Ctrl Pts',(-13.6871299964566,36.7584929312426,18.4011893739575));
#44815=CARTESIAN_POINT('Ctrl Pts',(-13.6349282140381,36.867947313688,18.3952736725501));
#44816=CARTESIAN_POINT('Ctrl Pts',(-13.5779094458923,36.9749481085648,18.3893579711426));
#44817=CARTESIAN_POINT('Ctrl Pts',(-13.5163472182928,37.0790688397464,18.3834422697352));
#44818=CARTESIAN_POINT('Ctrl Pts',(-13.4777389013461,37.1443674221228,18.3797322793107));
#44819=CARTESIAN_POINT('Ctrl Pts',(-13.4373444700697,37.2085338354459,18.3760222888863));
#44820=CARTESIAN_POINT('Ctrl Pts',(-13.3952395715432,37.271469403674,18.3723122984619));
#44821=CARTESIAN_POINT('Ctrl Pts',(-13.3291450141728,37.3702630991931,18.3664885063728));
#44822=CARTESIAN_POINT('Ctrl Pts',(-13.2586283516628,37.4663288203657,18.3606647142837));
#44823=CARTESIAN_POINT('Ctrl Pts',(-13.183942014477,37.5592456405058,18.3548409221946));
#44824=CARTESIAN_POINT('Ctrl Pts',(-13.1093498801037,37.652045263497,18.3490244757274));
#44825=CARTESIAN_POINT('Ctrl Pts',(-13.0305987851725,37.7417035697452,18.3432080292603));
#44826=CARTESIAN_POINT('Ctrl Pts',(-12.9479848271691,37.8278278693692,18.3373915827931));
#44827=CARTESIAN_POINT('Ctrl Pts',(-12.8654535427777,37.9138659825047,18.3315809569723));
#44828=CARTESIAN_POINT('Ctrl Pts',(-12.7790673665881,37.9963768316084,18.3257703311515));
#44829=CARTESIAN_POINT('Ctrl Pts',(-12.6891627259359,38.075000623323,18.3199597053308));
#44830=CARTESIAN_POINT('Ctrl Pts',(-12.5958594062092,38.1565966424302,18.3139294195209));
#44831=CARTESIAN_POINT('Ctrl Pts',(-12.4987666351617,38.2340055693401,18.307899133711));
#44832=CARTESIAN_POINT('Ctrl Pts',(-12.3983029168726,38.306866813,18.3018688479011));
#44833=CARTESIAN_POINT('Ctrl Pts',(-12.3016076207253,38.3769950110533,18.2960647597967));
#44834=CARTESIAN_POINT('Ctrl Pts',(-12.2017900731062,38.4429102895892,18.2902606716924));
#44835=CARTESIAN_POINT('Ctrl Pts',(-12.0992566748516,38.5043325203369,18.2844565835881));
#44836=CARTESIAN_POINT('Ctrl Pts',(-11.9967384126859,38.56574568387,18.2786533522893));
#44837=CARTESIAN_POINT('Ctrl Pts',(-11.8915054473537,38.6226669088808,18.2728501209906));
#44838=CARTESIAN_POINT('Ctrl Pts',(-11.7839915924143,38.6748604052664,18.2670468896919));
#44839=CARTESIAN_POINT('Ctrl Pts',(-11.6764682405506,38.7270585120131,18.2612431457816));
#44840=CARTESIAN_POINT('Ctrl Pts',(-11.5666639658243,38.7745278815008,18.2554394018713));
#44841=CARTESIAN_POINT('Ctrl Pts',(-11.4550349263738,38.8170798214122,18.249635657961));
#44842=CARTESIAN_POINT('Ctrl Pts',(-11.3433696874364,38.8596455602276,18.2438300319907));
#44843=CARTESIAN_POINT('Ctrl Pts',(-11.2298788882609,38.897290552718,18.2380244060204));
#44844=CARTESIAN_POINT('Ctrl Pts',(-11.1150356831317,38.9298753702049,18.2322187800501));
#44845=CARTESIAN_POINT('Ctrl Pts',(-11.0000653236272,38.9624962655956,18.2264067260918));
#44846=CARTESIAN_POINT('Ctrl Pts',(-10.8837399622936,38.9900456911426,18.2205946721334));
#44847=CARTESIAN_POINT('Ctrl Pts',(-10.7665449882451,39.0124348943,18.2147826181751));
#44848=CARTESIAN_POINT('Ctrl Pts',(-10.6492730493103,39.0348388010101,18.2089667472949));
#44849=CARTESIAN_POINT('Ctrl Pts',(-10.5311307634036,39.052075677528,18.2031508764146));
#44850=CARTESIAN_POINT('Ctrl Pts',(-10.4126090654447,39.0641086057231,18.1973350055343));
#44851=CARTESIAN_POINT('Ctrl Pts',(-10.2939176455307,39.0761587649581,18.1915108063817));
#44852=CARTESIAN_POINT('Ctrl Pts',(-10.1748461353257,39.0829900787603,18.1856866072291));
#44853=CARTESIAN_POINT('Ctrl Pts',(-10.0558860363671,39.0846176994841,18.1798624080765));
#44854=CARTESIAN_POINT('Ctrl Pts',(-10.0243662135838,39.0850489559914,18.1783192206821));
#44855=CARTESIAN_POINT('Ctrl Pts',(-9.99285418524738,39.0851151723714,18.1767760332878));
#44856=CARTESIAN_POINT('Ctrl Pts',(-9.96135901985522,39.0848172388313,18.1752328458934));
#44857=CARTESIAN_POINT('Ctrl Pts',(-9.84254219543945,39.0836932721311,18.1694111071156));
#44858=CARTESIAN_POINT('Ctrl Pts',(-9.72358255591783,39.0773790740118,18.1635893683379));
#44859=CARTESIAN_POINT('Ctrl Pts',(-9.60497011596792,39.0658549397048,18.1577676295601));
#44860=CARTESIAN_POINT('Ctrl Pts',(-9.48649786732683,39.0543444260894,18.1519527716557));
#44861=CARTESIAN_POINT('Ctrl Pts',(-9.36837240499521,39.0376362587188,18.1461379137513));
#44862=CARTESIAN_POINT('Ctrl Pts',(-9.25108419494506,39.0157627067518,18.1403230558469));
#44863=CARTESIAN_POINT('Ctrl Pts',(-9.13390689647571,38.9939098391335,18.1345136966629));
#44864=CARTESIAN_POINT('Ctrl Pts',(-9.0175656748106,38.9669013755368,18.128704337479));
#44865=CARTESIAN_POINT('Ctrl Pts',(-8.90254568416089,38.934821345963,18.1228949782951));
#44866=CARTESIAN_POINT('Ctrl Pts',(-8.78760728663151,38.9027640733873,18.1170897401665));
#44867=CARTESIAN_POINT('Ctrl Pts',(-8.67398864760348,38.8656425013601,18.1112845020378));
#44868=CARTESIAN_POINT('Ctrl Pts',(-8.56216390622729,38.8235915534278,18.1054792639092));
#44869=CARTESIAN_POINT('Ctrl Pts',(-8.45038395661472,38.7815574491394,18.0996763510876));
#44870=CARTESIAN_POINT('Ctrl Pts',(-8.34039685749402,38.7345980387547,18.093873438266));
#44871=CARTESIAN_POINT('Ctrl Pts',(-8.23266026355598,38.6828976711261,18.0880705254443));
#44872=CARTESIAN_POINT('Ctrl Pts',(-8.12494841703871,38.6312091792279,18.0822689455693));
#44873=CARTESIAN_POINT('Ctrl Pts',(-8.01948641360687,38.5747820767256,18.0764673656943));
#44874=CARTESIAN_POINT('Ctrl Pts',(-7.91670996681592,38.5138479815774,18.0706657858192));
#44875=CARTESIAN_POINT('Ctrl Pts',(-7.81391316543473,38.4529018186007,18.0648630569574));
#44876=CARTESIAN_POINT('Ctrl Pts',(-7.71380333385899,38.3874470893049,18.0590603280956));
#44877=CARTESIAN_POINT('Ctrl Pts',(-7.61678939141035,38.3177601171733,18.0532575992337));
#44878=CARTESIAN_POINT('Ctrl Pts',(-7.58172511877826,38.2925727788583,18.0511602876341));
#44879=CARTESIAN_POINT('Ctrl Pts',(-7.54706499785715,38.2668329649385,18.0490629760345));
#44880=CARTESIAN_POINT('Ctrl Pts',(-7.51282733495085,38.2405550657615,18.0469656644349));
#44881=CARTESIAN_POINT('Ctrl Pts',(-7.51282733495083,38.2405550657615,19.2967866609659));
#44882=CARTESIAN_POINT('Ctrl Pts',(-7.41811218255726,38.1678598227495,19.2909817422586));
#44883=CARTESIAN_POINT('Ctrl Pts',(-7.3265292139763,38.0909644348317,19.2851768235514));
#44884=CARTESIAN_POINT('Ctrl Pts',(-7.23846551527048,38.0101747938699,19.2793719048441));
#44885=CARTESIAN_POINT('Ctrl Pts',(-7.1504261827437,37.9294075064418,19.2735685922889));
#44886=CARTESIAN_POINT('Ctrl Pts',(-7.06590448452307,37.8447483843177,19.2677652797336));
#44887=CARTESIAN_POINT('Ctrl Pts',(-6.98525330733249,37.7565426495976,19.2619619671784));
#44888=CARTESIAN_POINT('Ctrl Pts',(-6.90460541135285,37.6683405034379,19.2561588907251));
#44889=CARTESIAN_POINT('Ctrl Pts',(-6.82782799866911,37.576592333092,19.2503558142717));
#44890=CARTESIAN_POINT('Ctrl Pts',(-6.75523561031701,37.4816786769131,19.2445527378183));
#44891=CARTESIAN_POINT('Ctrl Pts',(-6.68262904333245,37.3867464823464,19.2387485279171));
#44892=CARTESIAN_POINT('Ctrl Pts',(-6.61420937421198,37.2886478967719,19.2329443180158));
#44893=CARTESIAN_POINT('Ctrl Pts',(-6.55024913470335,37.187794315603,19.2271401081146));
#44894=CARTESIAN_POINT('Ctrl Pts',(-6.4862220837446,37.0868353850162,19.2213298352642));
#44895=CARTESIAN_POINT('Ctrl Pts',(-6.42666398505913,36.9831160565537,19.2155195624138));
#44896=CARTESIAN_POINT('Ctrl Pts',(-6.37180263230093,36.8770745486052,19.2097092895634));
#44897=CARTESIAN_POINT('Ctrl Pts',(-6.31691159195473,36.7709756575184,19.2038958725509));
#44898=CARTESIAN_POINT('Ctrl Pts',(-6.26672253250245,36.6625524538866,19.1980824555384));
#44899=CARTESIAN_POINT('Ctrl Pts',(-6.22141536100894,36.5522638712477,19.1922690385259));
#44900=CARTESIAN_POINT('Ctrl Pts',(-6.17603640724264,36.4418005532443,19.1864464110447));
#44901=CARTESIAN_POINT('Ctrl Pts',(-6.13555493258404,36.3294663360085,19.1806237835634));
#44902=CARTESIAN_POINT('Ctrl Pts',(-6.10010133507654,36.2157365682286,19.1748011560822));
#44903=CARTESIAN_POINT('Ctrl Pts',(-6.07133914191992,36.123471811518,19.1700774736334));
#44904=CARTESIAN_POINT('Ctrl Pts',(-6.04588509371599,36.0302889351828,19.1653537911845));
#44905=CARTESIAN_POINT('Ctrl Pts',(-6.0237839425562,35.9364458684441,19.1606301087357));
#44906=CARTESIAN_POINT('Ctrl Pts',(-5.99653648737942,35.8207512271955,19.1548065059349));
#44907=CARTESIAN_POINT('Ctrl Pts',(-5.97429877800222,35.7036798183631,19.1489829031342));
#44908=CARTESIAN_POINT('Ctrl Pts',(-5.95720681326372,35.5857032092099,19.1431593003334));
#44909=CARTESIAN_POINT('Ctrl Pts',(-5.94013641280084,35.4678754466144,19.1373430449487));
#44910=CARTESIAN_POINT('Ctrl Pts',(-5.92819890219626,35.3491451557764,19.131526789564));
#44911=CARTESIAN_POINT('Ctrl Pts',(-5.92147985708011,35.2299966169245,19.1257105341793));
#44912=CARTESIAN_POINT('Ctrl Pts',(-5.91476753786673,35.1109673482181,19.1199001009862));
#44913=CARTESIAN_POINT('Ctrl Pts',(-5.91326331491296,34.9915210697442,19.1140896677931));
#44914=CARTESIAN_POINT('Ctrl Pts',(-5.91700120477437,34.8721491564906,19.1082792346001));
#44915=CARTESIAN_POINT('Ctrl Pts',(-5.92088057334584,34.7482590297715,19.1022488771654));
#44916=CARTESIAN_POINT('Ctrl Pts',(-5.9304067859898,34.6244494525114,19.0962185197307));
#44917=CARTESIAN_POINT('Ctrl Pts',(-5.94555850207841,34.5012724792722,19.090188162296));
#44918=CARTESIAN_POINT('Ctrl Pts',(-5.96014120934238,34.3827213044808,19.0843842694133));
#44919=CARTESIAN_POINT('Ctrl Pts',(-5.97993446366303,34.2647565185023,19.0785803765306));
#44920=CARTESIAN_POINT('Ctrl Pts',(-6.00486629199975,34.1478664100036,19.0727764836479));
#44921=CARTESIAN_POINT('Ctrl Pts',(-6.029794437115,34.0309935698797,19.0669734481841));
#44922=CARTESIAN_POINT('Ctrl Pts',(-6.05985956141968,33.9151954907488,19.0611704127204));
#44923=CARTESIAN_POINT('Ctrl Pts',(-6.09493856300208,33.8009503040859,19.0553673772567));
#44924=CARTESIAN_POINT('Ctrl Pts',(-6.13002066089168,33.686695033379,19.0495638295783));
#44925=CARTESIAN_POINT('Ctrl Pts',(-6.17011739610909,33.573993318034,19.0437602818999));
#44926=CARTESIAN_POINT('Ctrl Pts',(-6.21505597259766,33.4633075423393,19.0379567342214));
#44927=CARTESIAN_POINT('Ctrl Pts',(-6.26000912103195,33.3525858752737,19.0321513046636));
#44928=CARTESIAN_POINT('Ctrl Pts',(-6.30980707965028,33.2438818260596,19.0263458751058));
#44929=CARTESIAN_POINT('Ctrl Pts',(-6.36422941860888,33.1376366413906,19.020540445548));
#44930=CARTESIAN_POINT('Ctrl Pts',(-6.41871202285655,33.0312738047264,19.0147285872717));
#44931=CARTESIAN_POINT('Ctrl Pts',(-6.47782904286411,32.9273756313071,19.0089167289955));
#44932=CARTESIAN_POINT('Ctrl Pts',(-6.54131462650677,32.8263577830784,19.0031048707193));
#44933=CARTESIAN_POINT('Ctrl Pts',(-6.60484190628768,32.7252735882254,18.9972891953238));
#44934=CARTESIAN_POINT('Ctrl Pts',(-6.67274323206694,32.6270738211096,18.9914735199283));
#44935=CARTESIAN_POINT('Ctrl Pts',(-6.74471104103503,32.5321428741435,18.9856578445328));
#44936=CARTESIAN_POINT('Ctrl Pts',(-6.81678193279979,32.4370759532239,18.9798338390785));
#44937=CARTESIAN_POINT('Ctrl Pts',(-6.89293067356589,32.345287510785,18.9740098336241));
#44938=CARTESIAN_POINT('Ctrl Pts',(-6.97281121072416,32.2571268651134,18.9681858281698));
#44939=CARTESIAN_POINT('Ctrl Pts',(-6.99400281343857,32.2337386225629,18.9666407708356));
#44940=CARTESIAN_POINT('Ctrl Pts',(-7.01545686912637,32.2106054893505,18.9650957135014));
#44941=CARTESIAN_POINT('Ctrl Pts',(-7.03716652042704,32.1877335168371,18.9635506561672));
#44942=CARTESIAN_POINT('Ctrl Pts',(-7.1189944886594,32.1015245301369,18.9577270295825));
#44943=CARTESIAN_POINT('Ctrl Pts',(-7.20472013130725,32.0187508998506,18.9519034029978));
#44944=CARTESIAN_POINT('Ctrl Pts',(-7.29402358738557,31.9397848679587,18.9460797764131));
#44945=CARTESIAN_POINT('Ctrl Pts',(-7.38321437769467,31.8609184600804,18.9402634969502));
#44946=CARTESIAN_POINT('Ctrl Pts',(-7.47597370040877,31.785850364272,18.9344472174873));
#44947=CARTESIAN_POINT('Ctrl Pts',(-7.57194342192194,31.7149176184376,18.9286309380244));
#44948=CARTESIAN_POINT('Ctrl Pts',(-7.66781708048372,31.6440558742567,18.9228204804912));
#44949=CARTESIAN_POINT('Ctrl Pts',(-7.76689441846199,31.5773214865998,18.917010022958));
#44950=CARTESIAN_POINT('Ctrl Pts',(-7.86878310589314,31.5150122596667,18.9111995654248));
#44951=CARTESIAN_POINT('Ctrl Pts',(-7.97452766743188,31.4503450031931,18.9051692170154));
#44952=CARTESIAN_POINT('Ctrl Pts',(-8.08330023142771,31.390444752136,18.899138868606));
#44953=CARTESIAN_POINT('Ctrl Pts',(-8.19462738046408,31.3355962688822,18.8931085201966));
#44954=CARTESIAN_POINT('Ctrl Pts',(-8.30177435914308,31.2828072653315,18.8873046024816));
#44955=CARTESIAN_POINT('Ctrl Pts',(-8.41128714073893,31.2346976934736,18.8815006847666));
#44956=CARTESIAN_POINT('Ctrl Pts',(-8.52271787763656,31.1914750189942,18.8756967670516));
#44957=CARTESIAN_POINT('Ctrl Pts',(-8.63413215539231,31.1482587288227,18.8698937066181));
#44958=CARTESIAN_POINT('Ctrl Pts',(-8.74746344447043,31.1099280481632,18.8640906461846));
#44959=CARTESIAN_POINT('Ctrl Pts',(-8.86224436564803,31.076642112106,18.8582875857511));
#44960=CARTESIAN_POINT('Ctrl Pts',(-8.97703542028208,31.0433532373933,18.8524840129932));
#44961=CARTESIAN_POINT('Ctrl Pts',(-9.09327596927955,31.015110106533,18.8466804402353));
#44962=CARTESIAN_POINT('Ctrl Pts',(-9.21048456353993,30.9920216597902,18.8408768674775));
#44963=CARTESIAN_POINT('Ctrl Pts',(-9.32773116577276,30.9689257260106,18.8350714127583));
#44964=CARTESIAN_POINT('Ctrl Pts',(-9.44594603714658,30.9509878795476,18.8292659580392));
#44965=CARTESIAN_POINT('Ctrl Pts',(-9.56463929642827,30.9382656342659,18.8234605033201));
#44966=CARTESIAN_POINT('Ctrl Pts',(-9.68346399152251,30.9255293009167,18.81764861989));
#44967=CARTESIAN_POINT('Ctrl Pts',(-9.80276772569672,30.918020140751,18.8118367364599));
#44968=CARTESIAN_POINT('Ctrl Pts',(-9.92205711728293,30.9157436531195,18.8060248530298));
#44969=CARTESIAN_POINT('Ctrl Pts',(-10.0414248560725,30.9134656703303,18.8002091524555));
#44970=CARTESIAN_POINT('Ctrl Pts',(-10.1607778262462,30.9164271943039,18.7943934518811));
#44971=CARTESIAN_POINT('Ctrl Pts',(-10.2796259347861,30.9245816979609,18.7885777513068));
#44972=CARTESIAN_POINT('Ctrl Pts',(-10.3986442709859,30.9327478814175,18.7827537208305));
#44973=CARTESIAN_POINT('Ctrl Pts',(-10.5171558979279,30.9461218447179,18.7769296903541));
#44974=CARTESIAN_POINT('Ctrl Pts',(-10.6346789588496,30.9646056426672,18.7711056598778));
#44975=CARTESIAN_POINT('Ctrl Pts',(-10.6658518433224,30.9695084531758,18.7695608411181));
#44976=CARTESIAN_POINT('Ctrl Pts',(-10.6969552497768,30.9747705023045,18.7680160223585));
#44977=CARTESIAN_POINT('Ctrl Pts',(-10.7279803621977,30.9803893730543,18.7664712035988));
#44978=CARTESIAN_POINT('Ctrl Pts',(-10.8449353738875,31.0015707658987,18.7606477179771));
#44979=CARTESIAN_POINT('Ctrl Pts',(-10.9611538121788,31.0278949622146,18.7548242323554));
#44980=CARTESIAN_POINT('Ctrl Pts',(-11.0761490267025,31.0592985050467,18.7490007467337));
#44981=CARTESIAN_POINT('Ctrl Pts',(-11.190999152942,31.0906624263504,18.7431846085442));
#44982=CARTESIAN_POINT('Ctrl Pts',(-11.3046287346005,31.1270928410789,18.7373684703546));
#44983=CARTESIAN_POINT('Ctrl Pts',(-11.4165595837332,31.1684749843263,18.7315523321651));
#44984=CARTESIAN_POINT('Ctrl Pts',(-11.5283783878524,31.2098157032224,18.7257420160459));
#44985=CARTESIAN_POINT('Ctrl Pts',(-11.6385014614945,31.2560981489563,18.7199316999268));
#44986=CARTESIAN_POINT('Ctrl Pts',(-11.7464646841815,31.3071574489417,18.7141213838077));
#44987=CARTESIAN_POINT('Ctrl Pts',(-11.8585173767009,31.3601507914812,18.7080909824419));
#44988=CARTESIAN_POINT('Ctrl Pts',(-11.9682429275002,31.4182899039562,18.7020605810762));
#44989=CARTESIAN_POINT('Ctrl Pts',(-12.0751436264263,31.4813349222038,18.6960301797105));
#44990=CARTESIAN_POINT('Ctrl Pts',(-12.1780269609712,31.5420106873665,18.6902264028654));
#44991=CARTESIAN_POINT('Ctrl Pts',(-12.2782935465882,31.6072300550486,18.6844226260203));
#44992=CARTESIAN_POINT('Ctrl Pts',(-12.3755243858113,31.6767321967052,18.6786188491753));
#44993=CARTESIAN_POINT('Ctrl Pts',(-12.4727408703948,31.7462240774383,18.6728159291687));
#44994=CARTESIAN_POINT('Ctrl Pts',(-12.566922167756,31.8199972373276,18.6670130091621));
#44995=CARTESIAN_POINT('Ctrl Pts',(-12.6576789960419,31.8977480189389,18.6612100891555));
#44996=CARTESIAN_POINT('Ctrl Pts',(-12.7484438462911,31.9755056729138,18.6554066562309));
#44997=CARTESIAN_POINT('Ctrl Pts',(-12.8357833155193,32.057241381952,18.6496032233063));
#44998=CARTESIAN_POINT('Ctrl Pts',(-12.9193423908359,32.1426122060406,18.6437997903818));
#44999=CARTESIAN_POINT('Ctrl Pts',(-13.0029285737598,32.2280107254902,18.6379944747511));
#45000=CARTESIAN_POINT('Ctrl Pts',(-13.0827316382375,32.3170464136244,18.6321891591204));
#45001=CARTESIAN_POINT('Ctrl Pts',(-13.1584349609951,32.4093410882241,18.6263838434897));
#45002=CARTESIAN_POINT('Ctrl Pts',(-13.2342221398235,32.5017379970255,18.6205720973492));
#45003=CARTESIAN_POINT('Ctrl Pts',(-13.3059002530701,32.5974007821578,18.6147603512088));
#45004=CARTESIAN_POINT('Ctrl Pts',(-13.3731942623637,32.6959198216302,18.6089486050683));
#45005=CARTESIAN_POINT('Ctrl Pts',(-13.4405324805062,32.7945035832581,18.6031330408969));
#45006=CARTESIAN_POINT('Ctrl Pts',(-13.5034806440173,32.8959469899746,18.5973174767255));
#45007=CARTESIAN_POINT('Ctrl Pts',(-13.5618090311546,32.9998146521921,18.5915019125542));
#45008=CARTESIAN_POINT('Ctrl Pts',(-13.6202209881655,33.1038311305834,18.5856780161455));
#45009=CARTESIAN_POINT('Ctrl Pts',(-13.6739997742077,33.2102784338999,18.5798541197368));
#45010=CARTESIAN_POINT('Ctrl Pts',(-13.7229631873897,33.3186998764821,18.5740302233282));
#45011=CARTESIAN_POINT('Ctrl Pts',(-13.7359622416147,33.3474841486495,18.5724840658956));
#45012=CARTESIAN_POINT('Ctrl Pts',(-13.7486221680768,33.3764074745468,18.570937908463));
#45013=CARTESIAN_POINT('Ctrl Pts',(-13.7609401485724,33.4054611328486,18.5693917510304));
#45014=CARTESIAN_POINT('Ctrl Pts',(-13.8139041444415,33.5303840322502,18.5627436908306));
#45015=CARTESIAN_POINT('Ctrl Pts',(-13.8606921381242,33.6580718198479,18.5560956306309));
#45016=CARTESIAN_POINT('Ctrl Pts',(-13.9010386252039,33.7879263039455,18.5494475704312));
#45017=CARTESIAN_POINT('Ctrl Pts',(-13.9400043430179,33.913336805589,18.543027025385));
#45018=CARTESIAN_POINT('Ctrl Pts',(-13.9729620170383,34.040767878319,18.5366064803388));
#45019=CARTESIAN_POINT('Ctrl Pts',(-13.999719495407,34.1696573249187,18.5301859352926));
#45020=CARTESIAN_POINT('Ctrl Pts',(-14.0264024485984,34.2981877874345,18.5237832728081));
#45021=CARTESIAN_POINT('Ctrl Pts',(-14.0469195731717,34.428168277178,18.5173806103235));
#45022=CARTESIAN_POINT('Ctrl Pts',(-14.0611283268584,34.5590218681288,18.510977947839));
#45023=CARTESIAN_POINT('Ctrl Pts',(-14.0752785381356,34.6893363206963,18.5046016653803));
#45024=CARTESIAN_POINT('Ctrl Pts',(-14.0831721555653,34.8205164481573,18.4982253829215));
#45025=CARTESIAN_POINT('Ctrl Pts',(-14.0847177095373,34.9519767411296,18.4918491004628));
#45026=CARTESIAN_POINT('Ctrl Pts',(-14.0848982158961,34.9673300831989,18.4911044098531));
#45027=CARTESIAN_POINT('Ctrl Pts',(-14.0849921906929,34.9826872315731,18.4903597192435));
#45028=CARTESIAN_POINT('Ctrl Pts',(-14.0849995332602,34.9980472419391,18.4896150286338));
#45029=CARTESIAN_POINT('Origin',(-10.,35.,32.7603849714045));
#45030=CARTESIAN_POINT('',(-7.51282733495085,38.2405550657615,20.5469196478657));
#45031=CARTESIAN_POINT('',(-7.51282733495086,38.2405550657615,20.4426717868481));
#45032=CARTESIAN_POINT('',(-7.51282733495086,38.2405550657615,32.7603849714045));
#45033=CARTESIAN_POINT('',(-14.0849992317297,35.0025053477764,19.6353849713615));
#45034=CARTESIAN_POINT('Ctrl Pts',(-7.51282733495086,38.2405550657615,20.4426717868481));
#45035=CARTESIAN_POINT('Ctrl Pts',(-7.41801445252157,38.1677848135401,20.4368682809325));
#45036=CARTESIAN_POINT('Ctrl Pts',(-7.32640760621858,38.090857480237,20.4310647750169));
#45037=CARTESIAN_POINT('Ctrl Pts',(-7.2383799075348,38.0100962550876,20.4252612691014));
#45038=CARTESIAN_POINT('Ctrl Pts',(-7.15032426427737,37.9293093921215,20.4194559208509));
#45039=CARTESIAN_POINT('Ctrl Pts',(-7.06585032903301,37.8446864927464,20.4136505726005));
#45040=CARTESIAN_POINT('Ctrl Pts',(-6.98529479736551,37.7565880252966,20.4078452243501));
#45041=CARTESIAN_POINT('Ctrl Pts',(-6.90465031166474,37.6683922744717,20.4020334655015));
#45042=CARTESIAN_POINT('Ctrl Pts',(-6.82793314244132,37.576713596073,20.3962217066529));
#45043=CARTESIAN_POINT('Ctrl Pts',(-6.75544017465018,37.4819461194244,20.3904099478043));
#45044=CARTESIAN_POINT('Ctrl Pts',(-6.68290003758068,37.3871169800571,20.3845944073963));
#45045=CARTESIAN_POINT('Ctrl Pts',(-6.61458980900607,37.289195373977,20.3787788669882));
#45046=CARTESIAN_POINT('Ctrl Pts',(-6.5507625249852,37.1886036281048,20.3729633265801));
#45047=CARTESIAN_POINT('Ctrl Pts',(-6.48684332500794,37.0878670227628,20.3671394113686));
#45048=CARTESIAN_POINT('Ctrl Pts',(-6.42742015841111,36.9844529552749,20.3613154961571));
#45049=CARTESIAN_POINT('Ctrl Pts',(-6.3726997764162,36.8788076239969,20.3554915809455));
#45050=CARTESIAN_POINT('Ctrl Pts',(-6.35659884856678,36.8477225366031,20.3537779518515));
#45051=CARTESIAN_POINT('Ctrl Pts',(-6.34090475411754,36.8164443971796,20.3520643227575));
#45052=CARTESIAN_POINT('Ctrl Pts',(-6.32562195112683,36.7849848609887,20.3503506936635));
#45053=CARTESIAN_POINT('Ctrl Pts',(-6.27368491836625,36.6780728656717,20.3445271015875));
#45054=CARTESIAN_POINT('Ctrl Pts',(-6.22633417317533,36.5687197963928,20.3387035095116));
#45055=CARTESIAN_POINT('Ctrl Pts',(-6.18380574208759,36.4573559571623,20.3328799174356));
#45056=CARTESIAN_POINT('Ctrl Pts',(-6.14133096694234,36.3461326199818,20.3270636726874));
#45057=CARTESIAN_POINT('Ctrl Pts',(-6.10366654922815,36.23290393676,20.3212474279392));
#45058=CARTESIAN_POINT('Ctrl Pts',(-6.07100210351602,36.1181236646384,20.315431183191));
#45059=CARTESIAN_POINT('Ctrl Pts',(-6.03837035508901,36.003458288184,20.3096207605349));
#45060=CARTESIAN_POINT('Ctrl Pts',(-6.01072873296436,35.8872448031128,20.3038103378788));
#45061=CARTESIAN_POINT('Ctrl Pts',(-5.98821810037733,35.7699551869167,20.2979999152228));
#45062=CARTESIAN_POINT('Ctrl Pts',(-5.96485538506858,35.6482258707249,20.2919695538008));
#45063=CARTESIAN_POINT('Ctrl Pts',(-5.94701993537065,35.5253377640211,20.2859391923788));
#45064=CARTESIAN_POINT('Ctrl Pts',(-5.93481189990426,35.4018341832646,20.2799088309568));
#45065=CARTESIAN_POINT('Ctrl Pts',(-5.92306235450141,35.2829689544154,20.2741049482995));
#45066=CARTESIAN_POINT('Ctrl Pts',(-5.91652519884472,35.1635340907011,20.2683010656422));
#45067=CARTESIAN_POINT('Ctrl Pts',(-5.9152372060822,35.0440217835264,20.2624971829849));
#45068=CARTESIAN_POINT('Ctrl Pts',(-5.9139494035681,34.9245271294228,20.2566941576146));
#45069=CARTESIAN_POINT('Ctrl Pts',(-5.91790922642153,34.8049554628107,20.2508911322444));
#45070=CARTESIAN_POINT('Ctrl Pts',(-5.92710133581934,34.6858002684352,20.2450881068741));
#45071=CARTESIAN_POINT('Ctrl Pts',(-5.93629425680091,34.5666345536865,20.2392845691469));
#45072=CARTESIAN_POINT('Ctrl Pts',(-5.95072035141718,34.4478857914314,20.2334810314197));
#45073=CARTESIAN_POINT('Ctrl Pts',(-5.9703123438196,34.3300429912097,20.2276774936925));
#45074=CARTESIAN_POINT('Ctrl Pts',(-5.98991068971902,34.2121619756874,20.2218720739331));
#45075=CARTESIAN_POINT('Ctrl Pts',(-6.01467819816725,34.0951879090913,20.2160666541737));
#45076=CARTESIAN_POINT('Ctrl Pts',(-6.04449648540219,33.9795996148548,20.2102612344144));
#45077=CARTESIAN_POINT('Ctrl Pts',(-6.0743477937702,33.863883316739,20.2044493856627));
#45078=CARTESIAN_POINT('Ctrl Pts',(-6.10926094355822,33.7495562498452,20.1986375369111));
#45079=CARTESIAN_POINT('Ctrl Pts',(-6.1490676263635,33.6370822278368,20.1928256881595));
#45080=CARTESIAN_POINT('Ctrl Pts',(-6.1889004545081,33.5245343320147,20.1870100221403));
#45081=CARTESIAN_POINT('Ctrl Pts',(-6.23363306400828,33.4138422826733,20.1811943561211));
#45082=CARTESIAN_POINT('Ctrl Pts',(-6.28304959755292,33.3054485237242,20.175378690102));
#45083=CARTESIAN_POINT('Ctrl Pts',(-6.33253691522382,33.1968995018101,20.1695546937365));
#45084=CARTESIAN_POINT('Ctrl Pts',(-6.38672136336078,33.0906557035423,20.163730697371));
#45085=CARTESIAN_POINT('Ctrl Pts',(-6.44534184466881,32.9871337851865,20.1579067010056));
#45086=CARTESIAN_POINT('Ctrl Pts',(-6.46089433211237,32.9596685836147,20.1563615477021));
#45087=CARTESIAN_POINT('Ctrl Pts',(-6.47675883397401,32.9323948043757,20.1548163943986));
#45088=CARTESIAN_POINT('Ctrl Pts',(-6.49292998453718,32.9053198557676,20.1532712410951));
#45089=CARTESIAN_POINT('Ctrl Pts',(-6.55387812436898,32.8032759259147,20.1474476468347));
#45090=CARTESIAN_POINT('Ctrl Pts',(-6.61938194651444,32.7037297289456,20.1416240525744));
#45091=CARTESIAN_POINT('Ctrl Pts',(-6.68921093804276,32.6071145478263,20.1358004583141));
#45092=CARTESIAN_POINT('Ctrl Pts',(-6.75895182978661,32.5106212613019,20.1299842113945));
#45093=CARTESIAN_POINT('Ctrl Pts',(-6.83300680027765,32.4170519635853,20.124167964475));
#45094=CARTESIAN_POINT('Ctrl Pts',(-6.91110027972097,32.3268139761588,20.1183517175555));
#45095=CARTESIAN_POINT('Ctrl Pts',(-6.98911558699545,32.2366663176463,20.1125412927435));
#45096=CARTESIAN_POINT('Ctrl Pts',(-7.07116109533737,32.1498436425087,20.1067308679315));
#45097=CARTESIAN_POINT('Ctrl Pts',(-7.1569192722743,32.0667224857449,20.1009204431196));
#45098=CARTESIAN_POINT('Ctrl Pts',(-7.24592356176301,31.9804550327335,20.0948900825115));
#45099=CARTESIAN_POINT('Ctrl Pts',(-7.33892687398621,31.8981752172698,20.0888597219035));
#45100=CARTESIAN_POINT('Ctrl Pts',(-7.43552969293926,31.8202646267018,20.0828293612954));
#45101=CARTESIAN_POINT('Ctrl Pts',(-7.52850450245564,31.7452800414084,20.0770254765339));
#45102=CARTESIAN_POINT('Ctrl Pts',(-7.6248129822553,31.6743426980231,20.0712215917723));
#45103=CARTESIAN_POINT('Ctrl Pts',(-7.72406363515827,31.6077531541483,20.0654177070107));
#45104=CARTESIAN_POINT('Ctrl Pts',(-7.82329962744296,31.5411734464191,20.0596146795587));
#45105=CARTESIAN_POINT('Ctrl Pts',(-7.92547658955635,31.4789404884555,20.0538116521068));
#45106=CARTESIAN_POINT('Ctrl Pts',(-8.03017337671437,31.4213119618783,20.0480086246548));
#45107=CARTESIAN_POINT('Ctrl Pts',(-8.13487940724463,31.3636783474476,20.0422050848705));
#45108=CARTESIAN_POINT('Ctrl Pts',(-8.24210534739603,31.3106501695605,20.0364015450863));
#45109=CARTESIAN_POINT('Ctrl Pts',(-8.35140532531963,31.2624392180708,20.0305980053021));
#45110=CARTESIAN_POINT('Ctrl Pts',(-8.46074074766888,31.2142126324563,20.0247925835126));
#45111=CARTESIAN_POINT('Ctrl Pts',(-8.57215117198729,31.1708065447275,20.0189871617231));
#45112=CARTESIAN_POINT('Ctrl Pts',(-8.6851712302782,31.1323844159079,20.0131817399336));
#45113=CARTESIAN_POINT('Ctrl Pts',(-8.79831644733963,31.0939197383012,20.0073698892016));
#45114=CARTESIAN_POINT('Ctrl Pts',(-8.91307446958729,31.0604501680115,20.0015580384696));
#45115=CARTESIAN_POINT('Ctrl Pts',(-9.02896511587748,31.0320891827289,19.9957461877376));
#45116=CARTESIAN_POINT('Ctrl Pts',(-9.14493187948949,31.0037095698666,19.9899305197647));
#45117=CARTESIAN_POINT('Ctrl Pts',(-9.26203234907246,30.9804453036296,19.9841148517919));
#45118=CARTESIAN_POINT('Ctrl Pts',(-9.37977815191968,30.9623583790579,19.978299183819));
#45119=CARTESIAN_POINT('Ctrl Pts',(-9.49769261243319,30.9442455469938,19.9724751855536));
#45120=CARTESIAN_POINT('Ctrl Pts',(-9.61625384670567,30.9313249025324,19.9666511872881));
#45121=CARTESIAN_POINT('Ctrl Pts',(-9.73497025113626,30.9236064674498,19.9608271890227));
#45122=CARTESIAN_POINT('Ctrl Pts',(-9.76646625868438,30.9215587311594,19.959282055524));
#45123=CARTESIAN_POINT('Ctrl Pts',(-9.79797320078038,30.9198768761249,19.9577369220253));
#45124=CARTESIAN_POINT('Ctrl Pts',(-9.82948194040127,30.918560475598,19.9561917885266));
#45125=CARTESIAN_POINT('Ctrl Pts',(-9.94823818743541,30.9135989700585,19.9503681898147));
#45126=CARTESIAN_POINT('Ctrl Pts',(-10.0674026600072,30.9138168806141,19.9445445911028));
#45127=CARTESIAN_POINT('Ctrl Pts',(-10.186486613217,30.9192589223168,19.9387209923909));
#45128=CARTESIAN_POINT('Ctrl Pts',(-10.3054203249576,30.9246940981042,19.9329047409832));
#45129=CARTESIAN_POINT('Ctrl Pts',(-10.4242733150749,30.9353402772369,19.9270884895754));
#45130=CARTESIAN_POINT('Ctrl Pts',(-10.5425538536446,30.9511902593607,19.9212722381677));
#45131=CARTESIAN_POINT('Ctrl Pts',(-10.6607159932118,30.9670243756279,19.9154618088366));
#45132=CARTESIAN_POINT('Ctrl Pts',(-10.7783064188011,30.988051878274,19.9096513795056));
#45133=CARTESIAN_POINT('Ctrl Pts',(-10.8948361470651,31.0142135945455,19.9038409501745));
#45134=CARTESIAN_POINT('Ctrl Pts',(-11.0157766227005,31.0413655535902,19.8978105912488));
#45135=CARTESIAN_POINT('Ctrl Pts',(-11.1355740702196,31.0740480535646,19.8917802323231));
#45136=CARTESIAN_POINT('Ctrl Pts',(-11.2536903419425,31.1121361229436,19.8857498733975));
#45137=CARTESIAN_POINT('Ctrl Pts',(-11.3673707675015,31.1487937982373,19.8799459840692));
#45138=CARTESIAN_POINT('Ctrl Pts',(-11.4794935894149,31.1904582166419,19.874142094741));
#45139=CARTESIAN_POINT('Ctrl Pts',(-11.5895928249534,31.2369666954893,19.8683382054127));
#45140=CARTESIAN_POINT('Ctrl Pts',(-11.69967579759,31.2834683045085,19.8625351733846));
#45141=CARTESIAN_POINT('Ctrl Pts',(-11.8077354022319,31.3348123921697,19.8567321413564));
#45142=CARTESIAN_POINT('Ctrl Pts',(-11.9133252646715,31.3907879763625,19.8509291093282));
#45143=CARTESIAN_POINT('Ctrl Pts',(-12.018924449405,31.446768502515,19.8451255649633));
#45144=CARTESIAN_POINT('Ctrl Pts',(-12.1220530976098,31.507381146935,19.8393220205983));
#45145=CARTESIAN_POINT('Ctrl Pts',(-12.2222896631662,31.5723690903214,19.8335184762334));
#45146=CARTESIAN_POINT('Ctrl Pts',(-12.3225587339777,31.637378108349,19.8277130498637));
#45147=CARTESIAN_POINT('Ctrl Pts',(-12.4199335144992,31.7067650250812,19.821907623494));
#45148=CARTESIAN_POINT('Ctrl Pts',(-12.5140221923776,31.7802302231009,19.8161021971244));
#45149=CARTESIAN_POINT('Ctrl Pts',(-12.6082150638857,31.8537767763464,19.8102903418361));
#45150=CARTESIAN_POINT('Ctrl Pts',(-12.6991142469081,31.9314103743132,19.8044784865479));
#45151=CARTESIAN_POINT('Ctrl Pts',(-12.7863616136823,32.0127916112535,19.7986666312597));
#45152=CARTESIAN_POINT('Ctrl Pts',(-12.8736662846126,32.09422629947,19.7928509587393));
#45153=CARTESIAN_POINT('Ctrl Pts',(-12.9573140771527,32.1794132380182,19.7870352862188));
#45154=CARTESIAN_POINT('Ctrl Pts',(-13.036985431817,32.2679779490401,19.7812196136983));
#45155=CARTESIAN_POINT('Ctrl Pts',(-13.1167709060288,32.3566695182632,19.7753956109327));
#45156=CARTESIAN_POINT('Ctrl Pts',(-13.1925683153322,32.4487482027003,19.7695716081671));
#45157=CARTESIAN_POINT('Ctrl Pts',(-13.2640997981118,32.5438083324043,19.7637476054014));
#45158=CARTESIAN_POINT('Ctrl Pts',(-13.2830768779487,32.5690274890693,19.762202515587));
#45159=CARTESIAN_POINT('Ctrl Pts',(-13.3017539560937,32.5944563419323,19.7606574257726));
#45160=CARTESIAN_POINT('Ctrl Pts',(-13.3201263812762,32.620087015802,19.7591123359582));
#45161=CARTESIAN_POINT('Ctrl Pts',(-13.3898878288234,32.7174085666047,19.7532455164733));
#45162=CARTESIAN_POINT('Ctrl Pts',(-13.4554778687479,32.8179551023663,19.7473786969884));
#45163=CARTESIAN_POINT('Ctrl Pts',(-13.5165873049546,32.9213372744401,19.7415118775035));
#45164=CARTESIAN_POINT('Ctrl Pts',(-13.5776176330624,33.0245856150207,19.7356526528021));
#45165=CARTESIAN_POINT('Ctrl Pts',(-13.6341786926365,33.130661949438,19.7297934281007));
#45166=CARTESIAN_POINT('Ctrl Pts',(-13.6860029530911,33.2391458806011,19.7239342033993));
#45167=CARTESIAN_POINT('Ctrl Pts',(-13.7377717246662,33.3475136566716,19.7180812522426));
#45168=CARTESIAN_POINT('Ctrl Pts',(-13.7848136157239,33.4582835422107,19.7122283010859));
#45169=CARTESIAN_POINT('Ctrl Pts',(-13.8269059407739,33.5710087752301,19.7063753499291));
#45170=CARTESIAN_POINT('Ctrl Pts',(-13.869450718731,33.6849456984881,19.7004594850521));
#45171=CARTESIAN_POINT('Ctrl Pts',(-13.9069386738898,33.8008799030811,19.694543620175));
#45172=CARTESIAN_POINT('Ctrl Pts',(-13.9391887239996,33.9183266682058,19.688627755298));
#45173=CARTESIAN_POINT('Ctrl Pts',(-13.9710477411261,34.0343493872042,19.682783620489));
#45174=CARTESIAN_POINT('Ctrl Pts',(-13.9977950631134,34.1518477927289,19.6769394856801));
#45175=CARTESIAN_POINT('Ctrl Pts',(-14.019305630051,34.270337576519,19.6710953508711));
#45176=CARTESIAN_POINT('Ctrl Pts',(-14.0412122233848,34.3910088500948,19.66514362096));
#45177=CARTESIAN_POINT('Ctrl Pts',(-14.0576872012397,34.512707961776,19.6591918910489));
#45178=CARTESIAN_POINT('Ctrl Pts',(-14.0686527748495,34.6349115207107,19.6532401611378));
#45179=CARTESIAN_POINT('Ctrl Pts',(-14.0796183484592,34.7571150796453,19.6472884312267));
#45180=CARTESIAN_POINT('Ctrl Pts',(-14.0850744735353,34.8798226489189,19.6413367013156));
#45181=CARTESIAN_POINT('Ctrl Pts',(-14.0849992317303,35.0025053468896,19.6353849714045));
#45182=CARTESIAN_POINT('Ctrl Pts',(-14.0849992317297,35.0025053477764,19.6353849713615));
#45183=CARTESIAN_POINT('Ctrl Pts',(-14.0849166368293,35.1371773114109,19.6288516038417));
#45184=CARTESIAN_POINT('Ctrl Pts',(-14.0781702966957,35.2716029408522,19.622318236322));
#45185=CARTESIAN_POINT('Ctrl Pts',(-14.0648574523362,35.4051652652772,19.6157848688022));
#45186=CARTESIAN_POINT('Ctrl Pts',(-14.0514920356939,35.5392550259205,19.6092257010827));
#45187=CARTESIAN_POINT('Ctrl Pts',(-14.0315082634781,35.6724744539174,19.6026665333631));
#45188=CARTESIAN_POINT('Ctrl Pts',(-14.0050544117836,35.8042164874292,19.5961073656435));
#45189=CARTESIAN_POINT('Ctrl Pts',(-13.9784604826347,35.9366561164707,19.5895134660623));
#45190=CARTESIAN_POINT('Ctrl Pts',(-13.9453278743482,36.0676024707254,19.5829195664811));
#45191=CARTESIAN_POINT('Ctrl Pts',(-13.9058559320516,36.1964591251094,19.5763256668999));
#45192=CARTESIAN_POINT('Ctrl Pts',(-13.8773364437467,36.2895613550451,19.5715614057298));
#45193=CARTESIAN_POINT('Ctrl Pts',(-13.8455085704644,36.3815730886471,19.5667971445598));
#45194=CARTESIAN_POINT('Ctrl Pts',(-13.8104627254334,36.4722767464314,19.5620328833897));
#45195=CARTESIAN_POINT('Ctrl Pts',(-13.7676243767153,36.5831485179276,19.5562092805859));
#45196=CARTESIAN_POINT('Ctrl Pts',(-13.7198739330841,36.6923278457604,19.550385677782));
#45197=CARTESIAN_POINT('Ctrl Pts',(-13.6673654190107,36.7993487386953,19.5445620749782));
#45198=CARTESIAN_POINT('Ctrl Pts',(-13.6149231529138,36.9062346074779,19.5387458195904));
#45199=CARTESIAN_POINT('Ctrl Pts',(-13.5577349346273,37.0109670944149,19.5329295642026));
#45200=CARTESIAN_POINT('Ctrl Pts',(-13.4960035828856,37.1130981871298,19.5271133088149));
#45201=CARTESIAN_POINT('Ctrl Pts',(-13.4343340255014,37.2151270445124,19.5213028756188));
#45202=CARTESIAN_POINT('Ctrl Pts',(-13.3681305918992,37.3145593406558,19.5154924424228));
#45203=CARTESIAN_POINT('Ctrl Pts',(-13.2976426602438,37.4109703202943,19.5096820092268));
#45204=CARTESIAN_POINT('Ctrl Pts',(-13.2244867683692,37.5110304445784,19.5036516517932));
#45205=CARTESIAN_POINT('Ctrl Pts',(-13.1467158323389,37.6078356182348,19.4976212943596));
#45206=CARTESIAN_POINT('Ctrl Pts',(-13.0646591809277,37.7009422623884,19.4915909369261));
#45207=CARTESIAN_POINT('Ctrl Pts',(-12.9856840918765,37.790552371829,19.4857870440407));
#45208=CARTESIAN_POINT('Ctrl Pts',(-12.9027396693396,37.8767363983482,19.4799831511552));
#45209=CARTESIAN_POINT('Ctrl Pts',(-12.8161610255012,37.9591319805726,19.4741792582698));
#45210=CARTESIAN_POINT('Ctrl Pts',(-12.7295951720748,38.0415153903561,19.4683762228035));
#45211=CARTESIAN_POINT('Ctrl Pts',(-12.6393964607655,38.1201111874317,19.4625731873371));
#45212=CARTESIAN_POINT('Ctrl Pts',(-12.545936466874,38.1945942632267,19.4567701518708));
#45213=CARTESIAN_POINT('Ctrl Pts',(-12.4524682235801,38.2690839133948,19.4509666041898));
#45214=CARTESIAN_POINT('Ctrl Pts',(-12.3557384447104,38.3394598660146,19.4451630565089));
#45215=CARTESIAN_POINT('Ctrl Pts',(-12.2561508281849,38.4054380688071,19.4393595088279));
#45216=CARTESIAN_POINT('Ctrl Pts',(-12.1565309190185,38.4714376659303,19.4335540792676));
#45217=CARTESIAN_POINT('Ctrl Pts',(-12.0540516694452,38.5330364517656,19.4277486497073));
#45218=CARTESIAN_POINT('Ctrl Pts',(-11.949144155848,38.5899947158351,19.4219432201469));
#45219=CARTESIAN_POINT('Ctrl Pts',(-11.8441204715464,38.6470160533816,19.4161313618684));
#45220=CARTESIAN_POINT('Ctrl Pts',(-11.7366635148745,38.6993864168409,19.4103195035899));
#45221=CARTESIAN_POINT('Ctrl Pts',(-11.6272274043801,38.7469128591995,19.4045076453114));
#45222=CARTESIAN_POINT('Ctrl Pts',(-11.5177194183068,38.7944705160314,19.3986919699137));
#45223=CARTESIAN_POINT('Ctrl Pts',(-11.406230070125,38.8371777701989,19.392876294516));
#45224=CARTESIAN_POINT('Ctrl Pts',(-11.2932302473512,38.8748910342532,19.3870606191183));
#45225=CARTESIAN_POINT('Ctrl Pts',(-11.1800685697464,38.912658316746,19.3812366136618));
#45226=CARTESIAN_POINT('Ctrl Pts',(-11.0653924905132,38.9454172201218,19.3754126082054));
#45227=CARTESIAN_POINT('Ctrl Pts',(-10.9496848595851,38.97307483789,19.369588602749));
#45228=CARTESIAN_POINT('Ctrl Pts',(-10.9189886450579,38.9804121600832,19.3680435454397));
#45229=CARTESIAN_POINT('Ctrl Pts',(-10.8882198660469,38.9873907390189,19.3664984881305));
#45230=CARTESIAN_POINT('Ctrl Pts',(-10.8573875990365,38.9940094522946,19.3649534308213));
#45231=CARTESIAN_POINT('Ctrl Pts',(-10.7411646735354,39.0189588411828,19.3591293024663));
#45232=CARTESIAN_POINT('Ctrl Pts',(-10.6236644106922,39.0388712407908,19.3533051741113));
#45233=CARTESIAN_POINT('Ctrl Pts',(-10.5053611106736,39.0536200053556,19.3474810457563));
#45234=CARTESIAN_POINT('Ctrl Pts',(-10.3872094693508,39.0683498627689,19.3416643836318));
#45235=CARTESIAN_POINT('Ctrl Pts',(-10.2682572403599,39.0779292021587,19.3358477215073));
#45236=CARTESIAN_POINT('Ctrl Pts',(-10.1489904075468,39.0822820650292,19.3300310593828));
#45237=CARTESIAN_POINT('Ctrl Pts',(-10.0298630210115,39.0866298385508,19.3242211980752));
#45238=CARTESIAN_POINT('Ctrl Pts',(-9.91042216868238,39.085763286278,19.3184113367675));
#45239=CARTESIAN_POINT('Ctrl Pts',(-9.79115965652278,39.0796581610395,19.3126014754599));
#45240=CARTESIAN_POINT('Ctrl Pts',(-9.67197560514657,39.0735570522593,19.3067954363614));
#45241=CARTESIAN_POINT('Ctrl Pts',(-9.55297006689244,39.0622242445947,19.3009893972629));
#45242=CARTESIAN_POINT('Ctrl Pts',(-9.43463532006182,39.0456875532693,19.2951833581645));
#45243=CARTESIAN_POINT('Ctrl Pts',(-9.31635049644983,39.029157838465,19.2893797685254));
#45244=CARTESIAN_POINT('Ctrl Pts',(-9.19873630501614,39.0074286634322,19.2835761788864));
#45245=CARTESIAN_POINT('Ctrl Pts',(-9.08227973382074,38.9805796704807,19.2777725892473));
#45246=CARTESIAN_POINT('Ctrl Pts',(-8.96584481065281,38.9537356684689,19.2719700784333));
#45247=CARTESIAN_POINT('Ctrl Pts',(-8.85056747696325,38.9217738347375,19.2661675676193));
#45248=CARTESIAN_POINT('Ctrl Pts',(-8.73692373103594,38.884824750073,19.2603650568053));
#45249=CARTESIAN_POINT('Ctrl Pts',(-8.62322683247863,38.8478583838502,19.254559832083));
#45250=CARTESIAN_POINT('Ctrl Pts',(-8.51116543836122,38.8059002282797,19.2487546073606));
#45251=CARTESIAN_POINT('Ctrl Pts',(-8.40119956722646,38.7591305079982,19.2429493826383));
#45252=CARTESIAN_POINT('Ctrl Pts',(-8.29121019275929,38.7123507914855,19.237142917148));
#45253=CARTESIAN_POINT('Ctrl Pts',(-8.18331760511866,38.6607576315025,19.2313364516578));
#45254=CARTESIAN_POINT('Ctrl Pts',(-8.07795978764544,38.6045785359861,19.2255299861675));
#45255=CARTESIAN_POINT('Ctrl Pts',(-7.97248665224614,38.5483379504262,19.2197171652916));
#45256=CARTESIAN_POINT('Ctrl Pts',(-7.86955418587233,38.4875016023944,19.2139043444157));
#45257=CARTESIAN_POINT('Ctrl Pts',(-7.76957405592466,38.4223420501165,19.2080915235398));
#45258=CARTESIAN_POINT('Ctrl Pts',(-7.68162083497658,38.3650207353575,19.2029779442807));
#45259=CARTESIAN_POINT('Ctrl Pts',(-7.59595210725508,38.304354525196,19.1978643650215));
#45260=CARTESIAN_POINT('Ctrl Pts',(-7.51282733495087,38.2405550657615,19.1927507857623));
#45261=CARTESIAN_POINT('',(-14.0849997388207,34.9985392348549,19.7396150285601));
#45262=CARTESIAN_POINT('Ctrl Pts',(-14.0849997388207,34.9985392348549,19.7396150285601));
#45263=CARTESIAN_POINT('Ctrl Pts',(-14.0850418772222,35.1163784095191,19.7338448932763));
#45264=CARTESIAN_POINT('Ctrl Pts',(-14.0799808576043,35.2344196440369,19.7280747579925));
#45265=CARTESIAN_POINT('Ctrl Pts',(-14.0697904347134,35.3521800924462,19.7223046227086));
#45266=CARTESIAN_POINT('Ctrl Pts',(-14.0596124124487,35.4697972393143,19.7165415090461));
#45267=CARTESIAN_POINT('Ctrl Pts',(-14.0443174331508,35.5871338681316,19.7107783953837));
#45268=CARTESIAN_POINT('Ctrl Pts',(-14.0239312542512,35.7037060899698,19.7050152817212));
#45269=CARTESIAN_POINT('Ctrl Pts',(-14.0035643215084,35.8201682584586,19.6992576088914));
#45270=CARTESIAN_POINT('Ctrl Pts',(-13.9781158193346,35.9358670471083,19.6934999360617));
#45271=CARTESIAN_POINT('Ctrl Pts',(-13.947663338309,36.0503233632415,19.6877422632319));
#45272=CARTESIAN_POINT('Ctrl Pts',(-13.9172299732922,36.1647078314375,19.6819882046799));
#45273=CARTESIAN_POINT('Ctrl Pts',(-13.8817989825304,36.2778509767239,19.6762341461279));
#45274=CARTESIAN_POINT('Ctrl Pts',(-13.8414989711434,36.3892842238738,19.6704800875759));
#45275=CARTESIAN_POINT('Ctrl Pts',(-13.8012118049636,36.5006819528411,19.6647278630699));
#45276=CARTESIAN_POINT('Ctrl Pts',(-13.7560588443521,36.6103704756653,19.6589756385639));
#45277=CARTESIAN_POINT('Ctrl Pts',(-13.706218251875,36.7178973396186,19.6532234140579));
#45278=CARTESIAN_POINT('Ctrl Pts',(-13.6563812420875,36.825416474222,19.6474716030389));
#45279=CARTESIAN_POINT('Ctrl Pts',(-13.6018574457932,36.9307738811283,19.6417197920198));
#45280=CARTESIAN_POINT('Ctrl Pts',(-13.5428724623509,37.0335387174862,19.6359679810008));
#45281=CARTESIAN_POINT('Ctrl Pts',(-13.4838771575834,37.1363215358666,19.6302151635169));
#45282=CARTESIAN_POINT('Ctrl Pts',(-13.4204193217302,37.2365105209835,19.624462346033));
#45283=CARTESIAN_POINT('Ctrl Pts',(-13.3527692484885,37.3337016446816,19.6187095285492));
#45284=CARTESIAN_POINT('Ctrl Pts',(-13.2850503482449,37.4309916503666,19.6129508581643));
#45285=CARTESIAN_POINT('Ctrl Pts',(-13.2131309324407,37.5252773621647,19.6071921877795));
#45286=CARTESIAN_POINT('Ctrl Pts',(-13.1373232309764,37.6161857625894,19.6014335173946));
#45287=CARTESIAN_POINT('Ctrl Pts',(-13.0614743853006,37.7071435030467,19.5956717215232));
#45288=CARTESIAN_POINT('Ctrl Pts',(-12.9817333321907,37.7947199746858,19.5899099256517));
#45289=CARTESIAN_POINT('Ctrl Pts',(-12.8984497566299,37.8785784700599,19.5841481297803));
#45290=CARTESIAN_POINT('Ctrl Pts',(-12.8150375635516,37.9625664708187,19.5783774357813));
#45291=CARTESIAN_POINT('Ctrl Pts',(-12.7280722283443,38.0428247465532,19.5726067417823));
#45292=CARTESIAN_POINT('Ctrl Pts',(-12.6379373774227,38.1190561701894,19.5668360477833));
#45293=CARTESIAN_POINT('Ctrl Pts',(-12.5752148460843,38.1721036630193,19.562820369813));
#45294=CARTESIAN_POINT('Ctrl Pts',(-12.5109581858319,38.2232020492989,19.5588046918428));
#45295=CARTESIAN_POINT('Ctrl Pts',(-12.4453045396966,38.2722638506299,19.5547890138725));
#45296=CARTESIAN_POINT('Ctrl Pts',(-12.3500926000171,38.343414038683,19.5489654151666));
#45297=CARTESIAN_POINT('Ctrl Pts',(-12.2516191994198,38.4105199874075,19.5431418164606));
#45298=CARTESIAN_POINT('Ctrl Pts',(-12.1502624669472,38.4732688239234,19.5373182177547));
#45299=CARTESIAN_POINT('Ctrl Pts',(-12.0490336105157,38.535938493791,19.5315019663529));
#45300=CARTESIAN_POINT('Ctrl Pts',(-11.9449290017087,38.5942617720503,19.5256857149512));
#45301=CARTESIAN_POINT('Ctrl Pts',(-11.8383585470582,38.6479669478297,19.5198694635494));
#45302=CARTESIAN_POINT('Ctrl Pts',(-11.7318947695989,38.7016183646445,19.5140590342244));
#45303=CARTESIAN_POINT('Ctrl Pts',(-11.6229704192588,38.7506606926182,19.5082486048994));
#45304=CARTESIAN_POINT('Ctrl Pts',(-11.5120224817609,38.7948666662545,19.5024381755743));
#45305=CARTESIAN_POINT('Ctrl Pts',(-11.3968750721636,38.8407458729144,19.4964078166464));
#45306=CARTESIAN_POINT('Ctrl Pts',(-11.2795482409027,38.8814151354747,19.4903774577185));
#45307=CARTESIAN_POINT('Ctrl Pts',(-11.1605567036874,38.9166737338622,19.4843470987906));
#45308=CARTESIAN_POINT('Ctrl Pts',(-11.0460338833157,38.9506081986502,19.4785432094683));
#45309=CARTESIAN_POINT('Ctrl Pts',(-10.929969564689,38.9795309383138,19.4727393201461));
#45310=CARTESIAN_POINT('Ctrl Pts',(-10.8128401968705,39.0033131047111,19.4669354308239));
#45311=CARTESIAN_POINT('Ctrl Pts',(-10.6957281303837,39.0270917582136,19.4611323988017));
#45312=CARTESIAN_POINT('Ctrl Pts',(-10.5775517276272,39.0457312672697,19.4553293667795));
#45313=CARTESIAN_POINT('Ctrl Pts',(-10.4587985262156,39.0591537187377,19.4495263347574));
#45314=CARTESIAN_POINT('Ctrl Pts',(-10.3400348403481,39.0725773552441,19.4437227903984));
#45315=CARTESIAN_POINT('Ctrl Pts',(-10.2206946603482,39.0807829725099,19.4379192460395));
#45316=CARTESIAN_POINT('Ctrl Pts',(-10.1012709142005,39.0837445074266,19.4321157016805));
#45317=CARTESIAN_POINT('Ctrl Pts',(-9.98180844067378,39.0867070027259,19.4263102753168));
#45318=CARTESIAN_POINT('Ctrl Pts',(-9.86226275510547,39.0844220234896,19.4205048489531));
#45319=CARTESIAN_POINT('Ctrl Pts',(-9.74312641102951,39.0769156183676,19.4146994225893));
#45320=CARTESIAN_POINT('Ctrl Pts',(-9.62385813558292,39.0694009006662,19.408887567307));
#45321=CARTESIAN_POINT('Ctrl Pts',(-9.50500051423202,39.05665324101,19.4030757120247));
#45322=CARTESIAN_POINT('Ctrl Pts',(-9.38704076585035,39.0387505465516,19.3972638567424));
#45323=CARTESIAN_POINT('Ctrl Pts',(-9.26900354139001,39.0208360935859,19.3914481842278));
#45324=CARTESIAN_POINT('Ctrl Pts',(-9.15186576406399,38.9977599415919,19.3856325117132));
#45325=CARTESIAN_POINT('Ctrl Pts',(-9.0361026244213,38.9696507213296,19.3798168391986));
#45326=CARTESIAN_POINT('Ctrl Pts',(-8.92017366812708,38.9415012380198,19.3739928364388));
#45327=CARTESIAN_POINT('Ctrl Pts',(-8.80562367034322,38.9083044104079,19.368168833679));
#45328=CARTESIAN_POINT('Ctrl Pts',(-8.69291101949768,38.8702381576654,19.3623448309191));
#45329=CARTESIAN_POINT('Ctrl Pts',(-8.66300870275553,38.8601392988581,19.3607997410475));
#45330=CARTESIAN_POINT('Ctrl Pts',(-8.63323558306982,38.8496979759635,19.3592546511758));
#45331=CARTESIAN_POINT('Ctrl Pts',(-8.60359994598701,38.8389180623129,19.3577095613041));
#45332=CARTESIAN_POINT('Ctrl Pts',(-8.49191615552896,38.7982932694686,19.3518867914752));
#45333=CARTESIAN_POINT('Ctrl Pts',(-8.38182657469041,38.7527251855687,19.3460640216462));
#45334=CARTESIAN_POINT('Ctrl Pts',(-8.27379996102366,38.7023584949918,19.3402412518173));
#45335=CARTESIAN_POINT('Ctrl Pts',(-8.16589302847115,38.6520476049389,19.3344249329503));
#45336=CARTESIAN_POINT('Ctrl Pts',(-8.06004488713174,38.5969488455534,19.3286086140834));
#45337=CARTESIAN_POINT('Ctrl Pts',(-7.95670750458039,38.5372561086472,19.3227922952165));
#45338=CARTESIAN_POINT('Ctrl Pts',(-7.85348150833941,38.4776277139331,19.3169822457003));
#45339=CARTESIAN_POINT('Ctrl Pts',(-7.75276123655803,38.4134153993639,19.3111721961842));
#45340=CARTESIAN_POINT('Ctrl Pts',(-7.65497622910664,38.344860014103,19.305362146668));
#45341=CARTESIAN_POINT('Ctrl Pts',(-7.60686683227912,38.3111313442369,19.3025036514339));
#45342=CARTESIAN_POINT('Ctrl Pts',(-7.55946757667728,38.2763521227345,19.2996451561999));
#45343=CARTESIAN_POINT('Ctrl Pts',(-7.51282733495083,38.2405550657615,19.2967866609659));
#45344=CARTESIAN_POINT('Ctrl Pts',(-7.51282733495085,38.2405550657615,20.5469196478657));
#45345=CARTESIAN_POINT('Ctrl Pts',(-7.47644404336342,38.2126303656825,20.5446751908154));
#45346=CARTESIAN_POINT('Ctrl Pts',(-7.44055209258124,38.1841089670783,20.5424307337651));
#45347=CARTESIAN_POINT('Ctrl Pts',(-7.40517161095562,38.1550104011571,20.5401862767148));
#45348=CARTESIAN_POINT('Ctrl Pts',(-7.31337143935251,38.0795096385265,20.5343626832275));
#45349=CARTESIAN_POINT('Ctrl Pts',(-7.22472119485878,37.9998771861964,20.5285390897402));
#45350=CARTESIAN_POINT('Ctrl Pts',(-7.1396148866694,37.9164056651016,20.5227154962529));
#45351=CARTESIAN_POINT('Ctrl Pts',(-7.05461595272924,37.8330394557293,20.5168992500938));
#45352=CARTESIAN_POINT('Ctrl Pts',(-6.97315235093204,37.7458440947145,20.5110830039347));
#45353=CARTESIAN_POINT('Ctrl Pts',(-6.89558569271732,37.6551528786001,20.5052667577756));
#45354=CARTESIAN_POINT('Ctrl Pts',(-6.81809667915196,37.5645524448894,20.4994563337107));
#45355=CARTESIAN_POINT('Ctrl Pts',(-6.74449711277133,37.4704634261763,20.4936459096458));
#45356=CARTESIAN_POINT('Ctrl Pts',(-6.67511189832342,37.3732560147042,20.4878354855809));
#45357=CARTESIAN_POINT('Ctrl Pts',(-6.60310030689818,37.2723690973092,20.4818051246878));
#45358=CARTESIAN_POINT('Ctrl Pts',(-6.53562873547309,37.1681233610124,20.4757747637947));
#45359=CARTESIAN_POINT('Ctrl Pts',(-6.47301484400611,37.0609708172118,20.4697444029016));
#45360=CARTESIAN_POINT('Ctrl Pts',(-6.41275248615357,36.9578425051387,20.4639405188496));
#45361=CARTESIAN_POINT('Ctrl Pts',(-6.35698974174589,36.852022169106,20.4581366347976));
#45362=CARTESIAN_POINT('Ctrl Pts',(-6.30596534635692,36.7439417930894,20.4523327507455));
#45363=CARTESIAN_POINT('Ctrl Pts',(-6.25494848780699,36.6358773816795,20.4465297239881));
#45364=CARTESIAN_POINT('Ctrl Pts',(-6.20866876066544,36.5255539633277,20.4407266972307));
#45365=CARTESIAN_POINT('Ctrl Pts',(-6.1673180785442,36.4134264356329,20.4349236704733));
#45366=CARTESIAN_POINT('Ctrl Pts',(-6.12596374558054,36.3012890082239,20.429120131368));
#45367=CARTESIAN_POINT('Ctrl Pts',(-6.08953946418185,36.1873475379103,20.4233165922627));
#45368=CARTESIAN_POINT('Ctrl Pts',(-6.05818807868422,36.0720745202516,20.4175130531573));
#45369=CARTESIAN_POINT('Ctrl Pts',(-6.02682652628934,35.9567641208663,20.4117076320304));
#45370=CARTESIAN_POINT('Ctrl Pts',(-6.00054124860252,35.8401217091931,20.4059022109034));
#45371=CARTESIAN_POINT('Ctrl Pts',(-5.979424391948,35.7226318425985,20.4000967897765));
#45372=CARTESIAN_POINT('Ctrl Pts',(-5.95828415031718,35.605011866784,20.3942849396796));
#45373=CARTESIAN_POINT('Ctrl Pts',(-5.94232382669346,35.4865429649003,20.3884730895828));
#45374=CARTESIAN_POINT('Ctrl Pts',(-5.93158393263372,35.3677168785845,20.3826612394859));
#45375=CARTESIAN_POINT('Ctrl Pts',(-5.9208369845507,35.2488127466218,20.376845572133));
#45376=CARTESIAN_POINT('Ctrl Pts',(-5.9153173134238,35.1295513699764,20.3710299047801));
#45377=CARTESIAN_POINT('Ctrl Pts',(-5.91501330217704,35.0104249033315,20.3652142374271));
#45378=CARTESIAN_POINT('Ctrl Pts',(-5.91470885546679,34.8911278008061,20.3593902397548));
#45379=CARTESIAN_POINT('Ctrl Pts',(-5.91963496328685,34.7719664005263,20.3535662420825));
#45380=CARTESIAN_POINT('Ctrl Pts',(-5.92972813547437,34.6534282919063,20.3477422444101));
#45381=CARTESIAN_POINT('Ctrl Pts',(-5.93240591212172,34.6219794497397,20.3461971043222));
#45382=CARTESIAN_POINT('Ctrl Pts',(-5.93544710453927,34.5905744243414,20.3446519642342));
#45383=CARTESIAN_POINT('Ctrl Pts',(-5.93884992652121,34.5592221867163,20.3431068241463));
#45384=CARTESIAN_POINT('Ctrl Pts',(-5.95167507597917,34.4410564009306,20.3372832304742));
#45385=CARTESIAN_POINT('Ctrl Pts',(-5.9696825270576,34.3232602815359,20.3314596368022));
#45386=CARTESIAN_POINT('Ctrl Pts',(-5.99284352153456,34.2063237706139,20.3256360431301));
#45387=CARTESIAN_POINT('Ctrl Pts',(-6.01597529497003,34.0895347925038,20.3198197967882));
#45388=CARTESIAN_POINT('Ctrl Pts',(-6.04424760091767,33.9736036627986,20.3140035504462));
#45389=CARTESIAN_POINT('Ctrl Pts',(-6.07757990198118,33.8590155239189,20.3081873041043));
#45390=CARTESIAN_POINT('Ctrl Pts',(-6.11087883721793,33.7445420884311,20.3023768798587));
#45391=CARTESIAN_POINT('Ctrl Pts',(-6.14922757781491,33.6314093591995,20.2965664556131));
#45392=CARTESIAN_POINT('Ctrl Pts',(-6.19249460660536,33.520092003106,20.2907560313675));
#45393=CARTESIAN_POINT('Ctrl Pts',(-6.23739938195125,33.4045610547785,20.2847256705429));
#45394=CARTESIAN_POINT('Ctrl Pts',(-6.28760204991982,33.2909860659518,20.2786953097183));
#45395=CARTESIAN_POINT('Ctrl Pts',(-6.34289869086028,33.1798804943937,20.2726649488938));
#45396=CARTESIAN_POINT('Ctrl Pts',(-6.39611860778833,33.0729476104427,20.2668610646673));
#45397=CARTESIAN_POINT('Ctrl Pts',(-6.45405658031249,32.9683024039722,20.2610571804409));
#45398=CARTESIAN_POINT('Ctrl Pts',(-6.51648217564307,32.8663813444321,20.2552532962144));
#45399=CARTESIAN_POINT('Ctrl Pts',(-6.57889855002973,32.7644753397483,20.2494502692853));
#45400=CARTESIAN_POINT('Ctrl Pts',(-6.64580101576262,32.6652930298942,20.2436472423561));
#45401=CARTESIAN_POINT('Ctrl Pts',(-6.71691430966396,32.5692442841966,20.2378442154269));
#45402=CARTESIAN_POINT('Ctrl Pts',(-6.78803388210761,32.4731870584234,20.2320406761525));
#45403=CARTESIAN_POINT('Ctrl Pts',(-6.8633647788998,32.3802642750675,20.2262371368782));
#45404=CARTESIAN_POINT('Ctrl Pts',(-6.94259012044536,32.290854409892,20.2204335976039));
#45405=CARTESIAN_POINT('Ctrl Pts',(-7.0218411538256,32.201415550162,20.2146281763109));
#45406=CARTESIAN_POINT('Ctrl Pts',(-7.104988872959,32.1154921796808,20.2088227550179));
#45407=CARTESIAN_POINT('Ctrl Pts',(-7.19167851929846,32.0334269837015,20.2030173337249));
#45408=CARTESIAN_POINT('Ctrl Pts',(-7.27846416636655,31.9512709081427,20.1972054834672));
#45409=CARTESIAN_POINT('Ctrl Pts',(-7.36879927328299,31.8729818163873,20.1913936332096));
#45410=CARTESIAN_POINT('Ctrl Pts',(-7.46229476848371,31.798863146016,20.1855817829519));
#45411=CARTESIAN_POINT('Ctrl Pts',(-7.55585167200815,31.7246957941194,20.179766115441));
#45412=CARTESIAN_POINT('Ctrl Pts',(-7.6525727676968,31.6547045575369,20.1739504479301));
#45413=CARTESIAN_POINT('Ctrl Pts',(-7.75204006350553,31.589149501383,20.1681347804191));
#45414=CARTESIAN_POINT('Ctrl Pts',(-7.85164983544689,31.5235005447083,20.1623107825941));
#45415=CARTESIAN_POINT('Ctrl Pts',(-7.95401330959738,31.46230066019,20.1564867847691));
#45416=CARTESIAN_POINT('Ctrl Pts',(-8.05868787723299,31.4057640252763,20.1506627869441));
#45417=CARTESIAN_POINT('Ctrl Pts',(-8.08645861215048,31.3907645470193,20.1491176484887));
#45418=CARTESIAN_POINT('Ctrl Pts',(-8.11439191093491,31.3760930372918,20.1475725100333));
#45419=CARTESIAN_POINT('Ctrl Pts',(-8.14247929139104,31.3617529197306,20.1460273715779));
#45420=CARTESIAN_POINT('Ctrl Pts',(-8.24834003867474,31.3077053176931,20.1402037771774));
#45421=CARTESIAN_POINT('Ctrl Pts',(-8.35673235697298,31.2581946822142,20.134380182777));
#45422=CARTESIAN_POINT('Ctrl Pts',(-8.46723070851764,31.2134655291297,20.1285565883766));
#45423=CARTESIAN_POINT('Ctrl Pts',(-8.57758965004794,31.1687928084878,20.1227403413018));
#45424=CARTESIAN_POINT('Ctrl Pts',(-8.69004896480404,31.1288897235107,20.1169240942271));
#45425=CARTESIAN_POINT('Ctrl Pts',(-8.80415874586783,31.0939548524223,20.1111078471524));
#45426=CARTESIAN_POINT('Ctrl Pts',(-8.91815430246159,31.0590549513171,20.1052974221705));
#45427=CARTESIAN_POINT('Ctrl Pts',(-9.03379665046037,31.02911348937,20.0994869971886));
#45428=CARTESIAN_POINT('Ctrl Pts',(-9.15061669913917,31.0042806644837,20.0936765722067));
#45429=CARTESIAN_POINT('Ctrl Pts',(-9.27185860746496,30.9785078702384,20.0876462116568));
#45430=CARTESIAN_POINT('Ctrl Pts',(-9.39436871897362,30.9582382657709,20.0816158511069));
#45431=CARTESIAN_POINT('Ctrl Pts',(-9.51760581123321,30.9435827573283,20.075585490557));
#45432=CARTESIAN_POINT('Ctrl Pts',(-9.63621462428657,30.9294776496112,20.0697816055903));
#45433=CARTESIAN_POINT('Ctrl Pts',(-9.75549635605137,30.9205726101855,20.0639777206236));
#45434=CARTESIAN_POINT('Ctrl Pts',(-9.87495964110511,30.9169141683468,20.0581738356569));
#45435=CARTESIAN_POINT('Ctrl Pts',(-9.99440528012957,30.9132562668997,20.0523708079873));
#45436=CARTESIAN_POINT('Ctrl Pts',(-10.1140320110764,30.9148434343454,20.0465677803176));
#45437=CARTESIAN_POINT('Ctrl Pts',(-10.2333461417158,30.9216701239176,20.040764752648));
#45438=CARTESIAN_POINT('Ctrl Pts',(-10.3526708065008,30.9284974162125,20.0349612126339));
#45439=CARTESIAN_POINT('Ctrl Pts',(-10.4716824084144,30.9405651270542,20.0291576726197));
#45440=CARTESIAN_POINT('Ctrl Pts',(-10.589890699295,30.9578156940974,20.0233541326056));
#45441=CARTESIAN_POINT('Ctrl Pts',(-10.7081373236823,30.9750718552891,20.0175487105742));
#45442=CARTESIAN_POINT('Ctrl Pts',(-10.825579715104,30.9975141563537,20.0117432885429));
#45443=CARTESIAN_POINT('Ctrl Pts',(-10.9417367956866,31.0250337350299,20.0059378665115));
#45444=CARTESIAN_POINT('Ctrl Pts',(-11.0580225093099,31.052583789051,20.0001260155213));
#45445=CARTESIAN_POINT('Ctrl Pts',(-11.1730196733704,31.0852222496975,19.9943141645311));
#45446=CARTESIAN_POINT('Ctrl Pts',(-11.2862612264689,31.1227900421459,19.9885023135409));
#45447=CARTESIAN_POINT('Ctrl Pts',(-11.3995771571447,31.1603825092947,19.9826866453));
#45448=CARTESIAN_POINT('Ctrl Pts',(-11.5111347997691,31.2029106109023,19.9768709770592));
#45449=CARTESIAN_POINT('Ctrl Pts',(-11.620487515265,31.2501673086829,19.9710553088183));
#45450=CARTESIAN_POINT('Ctrl Pts',(-11.7299968664924,31.2974916964829,19.9652313102726));
#45451=CARTESIAN_POINT('Ctrl Pts',(-11.8372946207,31.3495580217486,19.959407311727));
#45452=CARTESIAN_POINT('Ctrl Pts',(-11.9419590239602,31.4061135035648,19.9535833131813));
#45453=CARTESIAN_POINT('Ctrl Pts',(-11.9697269318143,31.4211179115468,19.9520381817907));
#45454=CARTESIAN_POINT('Ctrl Pts',(-11.9973096495272,31.4364380607679,19.9504930504001));
#45455=CARTESIAN_POINT('Ctrl Pts',(-12.0246996641409,31.4520687337509,19.9489479190094));
#45456=CARTESIAN_POINT('Ctrl Pts',(-12.1279324850377,31.5109806579436,19.9431243269318));
#45457=CARTESIAN_POINT('Ctrl Pts',(-12.2287584357382,31.5744969117993,19.9373007348541));
#45458=CARTESIAN_POINT('Ctrl Pts',(-12.3267397461459,31.642395622813,19.9314771427765));
#45459=CARTESIAN_POINT('Ctrl Pts',(-12.4245974385545,31.710208669502,19.9256608980266));
#45460=CARTESIAN_POINT('Ctrl Pts',(-12.5196172963132,31.7823929455247,19.9198446532766));
#45461=CARTESIAN_POINT('Ctrl Pts',(-12.6113866119169,31.8586810153852,19.9140284085267));
#45462=CARTESIAN_POINT('Ctrl Pts',(-12.7030640659445,31.9348927204794,19.9082179858689));
#45463=CARTESIAN_POINT('Ctrl Pts',(-12.7914971386674,32.0151997876799,19.9024075632112));
#45464=CARTESIAN_POINT('Ctrl Pts',(-12.8763030706051,32.0992922163672,19.8965971405534));
#45465=CARTESIAN_POINT('Ctrl Pts',(-12.9643191152854,32.1865677499473,19.890566779132));
#45466=CARTESIAN_POINT('Ctrl Pts',(-13.0484276328377,32.2779206224034,19.8845364177107));
#45467=CARTESIAN_POINT('Ctrl Pts',(-13.1282391855969,32.3729589653574,19.8785060562893));
#45468=CARTESIAN_POINT('Ctrl Pts',(-13.2050533024765,32.4644280087644,19.8727021736304));
#45469=CARTESIAN_POINT('Ctrl Pts',(-13.2778871049818,32.5593103479768,19.8668982909714));
#45470=CARTESIAN_POINT('Ctrl Pts',(-13.3464323288902,32.6572205250688,19.8610944083124));
#45471=CARTESIAN_POINT('Ctrl Pts',(-13.414967428036,32.7551162399235,19.8552913829405));
#45472=CARTESIAN_POINT('Ctrl Pts',(-13.4792149742207,32.8560385688199,19.8494883575686));
#45473=CARTESIAN_POINT('Ctrl Pts',(-13.5389089826654,32.9595715615562,19.8436853321967));
#45474=CARTESIAN_POINT('Ctrl Pts',(-13.5986082615749,33.0631136953605,19.8378817944678));
#45475=CARTESIAN_POINT('Ctrl Pts',(-13.6537529994241,33.1692665975251,19.8320782567389));
#45476=CARTESIAN_POINT('Ctrl Pts',(-13.7041226036779,33.2775886853244,19.82627471901));
#45477=CARTESIAN_POINT('Ctrl Pts',(-13.7545085423157,33.3859459009474,19.820469299249));
#45478=CARTESIAN_POINT('Ctrl Pts',(-13.8001160955967,33.4964733311269,19.814663879488));
#45479=CARTESIAN_POINT('Ctrl Pts',(-13.8407726035764,33.6087089421631,19.808858459727));
#45480=CARTESIAN_POINT('Ctrl Pts',(-13.881474135066,33.7210688442758,19.8030466109737));
#45481=CARTESIAN_POINT('Ctrl Pts',(-13.9172135378649,33.8351403190091,19.7972347622205));
#45482=CARTESIAN_POINT('Ctrl Pts',(-13.9478678316903,33.9504455309489,19.7914229134673));
#45483=CARTESIAN_POINT('Ctrl Pts',(-13.9785422594946,34.06582647625,19.7856072474465));
#45484=CARTESIAN_POINT('Ctrl Pts',(-14.0041248394553,34.1824423746108,19.7797915814257));
#45485=CARTESIAN_POINT('Ctrl Pts',(-14.0245439013221,34.2998061794537,19.773975915405));
#45486=CARTESIAN_POINT('Ctrl Pts',(-14.0449922114049,34.4173380959335,19.7681519190379));
#45487=CARTESIAN_POINT('Ctrl Pts',(-14.0602621888624,34.5356196536117,19.7623279226709));
#45488=CARTESIAN_POINT('Ctrl Pts',(-14.0703340623937,34.6541595447062,19.7565039263038));
#45489=CARTESIAN_POINT('Ctrl Pts',(-14.0730062118111,34.6856091354846,19.7549587730162));
#45490=CARTESIAN_POINT('Ctrl Pts',(-14.0753127595328,34.7170769169523,19.7534136197286));
#45491=CARTESIAN_POINT('Ctrl Pts',(-14.0772539509919,34.7485537450649,19.751868466441));
#45492=CARTESIAN_POINT('Ctrl Pts',(-14.0823853229795,34.8317600219526,19.7477839871591));
#45493=CARTESIAN_POINT('Ctrl Pts',(-14.0849699104881,34.9151249563342,19.7436995078773));
#45494=CARTESIAN_POINT('Ctrl Pts',(-14.0849997388204,34.9985392341328,19.7396150285955));
#45495=CARTESIAN_POINT('Origin',(-10.,35.,32.7603849714045));
#45496=CARTESIAN_POINT('',(-7.51282733495087,38.2405550657615,21.796951697066));
#45497=CARTESIAN_POINT('',(-7.51282733495086,38.2405550657615,21.6925401826178));
#45498=CARTESIAN_POINT('',(-7.51282733495086,38.2405550657615,32.7603849714045));
#45499=CARTESIAN_POINT('',(-14.084998525967,34.996529719382,20.8853849714301));
#45500=CARTESIAN_POINT('Ctrl Pts',(-7.51282733495086,38.2405550657615,21.6925401826178));
#45501=CARTESIAN_POINT('Ctrl Pts',(-7.4182381975729,38.1679565410881,21.6867304536884));
#45502=CARTESIAN_POINT('Ctrl Pts',(-7.32673645481531,38.0911410533406,21.680920724759));
#45503=CARTESIAN_POINT('Ctrl Pts',(-7.23871595880767,38.0104045315965,21.6751109958296));
#45504=CARTESIAN_POINT('Ctrl Pts',(-7.14889627851993,37.9280177137584,21.6691825130481));
#45505=CARTESIAN_POINT('Ctrl Pts',(-7.06270208366081,37.8415480444578,21.6632540302666));
#45506=CARTESIAN_POINT('Ctrl Pts',(-6.98051717086134,37.7513539293477,21.6573255474852));
#45507=CARTESIAN_POINT('Ctrl Pts',(-6.90006201646432,37.6630581435434,21.6515218423856));
#45508=CARTESIAN_POINT('Ctrl Pts',(-6.82344932057546,37.5711934669989,21.645718137286));
#45509=CARTESIAN_POINT('Ctrl Pts',(-6.75100187895214,37.4761333181853,21.6399144321864));
#45510=CARTESIAN_POINT('Ctrl Pts',(-6.67856303800499,37.3810844545399,21.6341114160799));
#45511=CARTESIAN_POINT('Ctrl Pts',(-6.61028871537809,37.2828411977853,21.6283083999734));
#45512=CARTESIAN_POINT('Ctrl Pts',(-6.54646060282584,37.1818090274279,21.622505383867));
#45513=CARTESIAN_POINT('Ctrl Pts',(-6.482625004261,37.0807650076194,21.6167016871599));
#45514=CARTESIAN_POINT('Ctrl Pts',(-6.42323687074606,36.9769317690469,21.6108979904528));
#45515=CARTESIAN_POINT('Ctrl Pts',(-6.36853349851039,36.870742111719,21.6050942937457));
#45516=CARTESIAN_POINT('Ctrl Pts',(-6.31177021911534,36.7605537825278,21.5990720533564));
#45517=CARTESIAN_POINT('Ctrl Pts',(-6.26005167499529,36.647828502816,21.5930498129671));
#45518=CARTESIAN_POINT('Ctrl Pts',(-6.21358909714194,36.533074517014,21.5870275725778));
#45519=CARTESIAN_POINT('Ctrl Pts',(-6.16874563957074,36.4223194592623,21.5812151942325));
#45520=CARTESIAN_POINT('Ctrl Pts',(-6.12879802966201,36.3096751367095,21.5754028158873));
#45521=CARTESIAN_POINT('Ctrl Pts',(-6.09388551090899,36.1956147364905,21.569590437542));
#45522=CARTESIAN_POINT('Ctrl Pts',(-6.05894887807914,36.0814755547527,21.563774044587));
#45523=CARTESIAN_POINT('Ctrl Pts',(-6.02905436381748,35.9659187417862,21.5579576516319));
#45524=CARTESIAN_POINT('Ctrl Pts',(-6.00429025138867,35.8494283988968,21.5521412586769));
#45525=CARTESIAN_POINT('Ctrl Pts',(-5.97949170059666,35.7327760580053,21.5463167771197));
#45526=CARTESIAN_POINT('Ctrl Pts',(-5.9598378545568,35.6151879976554,21.5404922955625));
#45527=CARTESIAN_POINT('Ctrl Pts',(-5.94536528078422,35.4971541951246,21.5346678140054));
#45528=CARTESIAN_POINT('Ctrl Pts',(-5.94384094504857,35.4847221877954,21.534054345695));
#45529=CARTESIAN_POINT('Ctrl Pts',(-5.94237404025469,35.4722852357941,21.5334408773846));
#45530=CARTESIAN_POINT('Ctrl Pts',(-5.94096457550343,35.4598439112155,21.5328274090742));
#45531=CARTESIAN_POINT('Ctrl Pts',(-5.92758466681423,35.3417396544853,21.5270038154232));
#45532=CARTESIAN_POINT('Ctrl Pts',(-5.91934211447414,35.2228604957279,21.5211802217721));
#45533=CARTESIAN_POINT('Ctrl Pts',(-5.91631621890921,35.1036907713156,21.5153566281211));
#45534=CARTESIAN_POINT('Ctrl Pts',(-5.91329414096098,34.9846713972114,21.5095403817985));
#45535=CARTESIAN_POINT('Ctrl Pts',(-5.91547563943873,34.8653625912019,21.5037241354758));
#45536=CARTESIAN_POINT('Ctrl Pts',(-5.92288844228433,34.7462553528815,21.4979078891532));
#45537=CARTESIAN_POINT('Ctrl Pts',(-5.93029382487344,34.6272673415628,21.4920974649252));
#45538=CARTESIAN_POINT('Ctrl Pts',(-5.94292006911531,34.5084809017419,21.4862870406972));
#45539=CARTESIAN_POINT('Ctrl Pts',(-5.96074286670309,34.3903879831318,21.4804766164691));
#45540=CARTESIAN_POINT('Ctrl Pts',(-5.97924029413158,34.2678250027103,21.4744462556373));
#45541=CARTESIAN_POINT('Ctrl Pts',(-6.00333545989573,34.1460095313729,21.4684158948055));
#45542=CARTESIAN_POINT('Ctrl Pts',(-6.03294191299889,34.0254872323263,21.4623855339737));
#45543=CARTESIAN_POINT('Ctrl Pts',(-6.06143646424841,33.9094912764808,21.4565816497605));
#45544=CARTESIAN_POINT('Ctrl Pts',(-6.09503569745824,33.7946935438724,21.4507777655472));
#45545=CARTESIAN_POINT('Ctrl Pts',(-6.13361042261505,33.6815703902411,21.444973881334));
#45546=CARTESIAN_POINT('Ctrl Pts',(-6.17217944987339,33.5684639461066,21.4391708544164));
#45547=CARTESIAN_POINT('Ctrl Pts',(-6.21572237577386,33.4570319754221,21.4333678274988));
#45548=CARTESIAN_POINT('Ctrl Pts',(-6.26406044064626,33.3477347038518,21.4275648005812));
#45549=CARTESIAN_POINT('Ctrl Pts',(-6.31240277326573,33.2384277824721,21.4217612613168));
#45550=CARTESIAN_POINT('Ctrl Pts',(-6.36554092143188,33.1312563083968,21.4159577220525));
#45551=CARTESIAN_POINT('Ctrl Pts',(-6.42324864130282,33.0266589960025,21.4101541827881));
#45552=CARTESIAN_POINT('Ctrl Pts',(-6.48097507511621,32.9220277639161,21.4043487615034));
#45553=CARTESIAN_POINT('Ctrl Pts',(-6.54327383056353,32.8199727110296,21.3985433402188));
#45554=CARTESIAN_POINT('Ctrl Pts',(-6.6098738627712,32.720905931367,21.3927379189341));
#45555=CARTESIAN_POINT('Ctrl Pts',(-6.67654764835466,32.6217294444087,21.3869260686823));
#45556=CARTESIAN_POINT('Ctrl Pts',(-6.74753199063213,32.5255481752715,21.3811142184305));
#45557=CARTESIAN_POINT('Ctrl Pts',(-6.8225137654087,32.4327434430928,21.3753023681788));
#45558=CARTESIAN_POINT('Ctrl Pts',(-6.89754478862016,32.3398777562645,21.3694867006723));
#45559=CARTESIAN_POINT('Ctrl Pts',(-6.97657820346002,32.2503933284084,21.3636710331659));
#45560=CARTESIAN_POINT('Ctrl Pts',(-7.0592631640353,32.164635497577,21.3578553656594));
#45561=CARTESIAN_POINT('Ctrl Pts',(-7.14206656189467,32.0787548279065,21.3520313678368));
#45562=CARTESIAN_POINT('Ctrl Pts',(-7.22853165018271,31.9966116897609,21.3462073700142));
#45563=CARTESIAN_POINT('Ctrl Pts',(-7.31827350936087,31.9185120429565,21.3403833721916));
#45564=CARTESIAN_POINT('Ctrl Pts',(-7.34208251675777,31.8977917783498,21.3388382336296));
#45565=CARTESIAN_POINT('Ctrl Pts',(-7.36612200402485,31.8773558892563,21.3372930950677));
#45566=CARTESIAN_POINT('Ctrl Pts',(-7.39038444532685,31.8572095747874,21.3357479565057));
#45567=CARTESIAN_POINT('Ctrl Pts',(-7.48182905933954,31.78127855336,21.3299243628436));
#45568=CARTESIAN_POINT('Ctrl Pts',(-7.57673789068907,31.7092194954885,21.3241007691814));
#45569=CARTESIAN_POINT('Ctrl Pts',(-7.67474932401372,31.6413642213206,21.3182771755193));
#45570=CARTESIAN_POINT('Ctrl Pts',(-7.77263710135293,31.5735945566628,21.3124609291858));
#45571=CARTESIAN_POINT('Ctrl Pts',(-7.87361936226054,31.5100183571618,21.3066446828523));
#45572=CARTESIAN_POINT('Ctrl Pts',(-7.97730064829077,31.4509279617631,21.3008284365188));
#45573=CARTESIAN_POINT('Ctrl Pts',(-8.08087814877779,31.3918967161785,21.2950180122802));
#45574=CARTESIAN_POINT('Ctrl Pts',(-8.18714894688558,31.337342542798,21.2892075880416));
#45575=CARTESIAN_POINT('Ctrl Pts',(-8.29568826514029,31.2875147797709,21.283397163803));
#45576=CARTESIAN_POINT('Ctrl Pts',(-8.40833602134445,31.2358009327344,21.2773668029753));
#45577=CARTESIAN_POINT('Ctrl Pts',(-8.52342705878339,31.1891786297618,21.2713364421475));
#45578=CARTESIAN_POINT('Ctrl Pts',(-8.64045761121134,31.1478746784292,21.2653060813198));
#45579=CARTESIAN_POINT('Ctrl Pts',(-8.7530929569649,31.1081219408507,21.2595021970967));
#45580=CARTESIAN_POINT('Ctrl Pts',(-8.86752434410631,31.0732954343172,21.2536983128737));
#45581=CARTESIAN_POINT('Ctrl Pts',(-8.98328254517895,31.0435482288972,21.2478944286506));
#45582=CARTESIAN_POINT('Ctrl Pts',(-9.09902364752437,31.0138054174584,21.2420914017235));
#45583=CARTESIAN_POINT('Ctrl Pts',(-9.21609077866904,30.9891405166922,21.2362883747964));
#45584=CARTESIAN_POINT('Ctrl Pts',(-9.33400102960615,30.9696562961164,21.2304853478693));
#45585=CARTESIAN_POINT('Ctrl Pts',(-9.45192169078268,30.950170355288,21.2246818085957));
#45586=CARTESIAN_POINT('Ctrl Pts',(-9.57068521686028,30.9358660706478,21.2188782693221));
#45587=CARTESIAN_POINT('Ctrl Pts',(-9.68980066115883,30.9267947056179,21.2130747300485));
#45588=CARTESIAN_POINT('Ctrl Pts',(-9.80895473320445,30.9177203988502,21.2072693087549));
#45589=CARTESIAN_POINT('Ctrl Pts',(-9.92846054348736,30.9138824175841,21.2014638874613));
#45590=CARTESIAN_POINT('Ctrl Pts',(-10.0478248515278,30.9152799626442,21.1956584661677));
#45591=CARTESIAN_POINT('Ctrl Pts',(-10.1673213444887,30.9166790553559,21.1898466159075));
#45592=CARTESIAN_POINT('Ctrl Pts',(-10.2866756138682,30.9233252426369,21.1840347656473));
#45593=CARTESIAN_POINT('Ctrl Pts',(-10.4053970920624,30.9351656617093,21.1782229153871));
#45594=CARTESIAN_POINT('Ctrl Pts',(-10.5241965471592,30.9470138576323,21.1724072478726));
#45595=CARTESIAN_POINT('Ctrl Pts',(-10.6423619801288,30.964063021455,21.166591580358));
#45596=CARTESIAN_POINT('Ctrl Pts',(-10.7594122392473,30.9862090175395,21.1607759128434));
#45597=CARTESIAN_POINT('Ctrl Pts',(-10.8766301602221,31.0083867353719,21.1549519150132));
#45598=CARTESIAN_POINT('Ctrl Pts',(-10.992729322997,31.0356757640889,21.1491279171829));
#45599=CARTESIAN_POINT('Ctrl Pts',(-11.1072428327368,31.0679218841237,21.1433039193526));
#45600=CARTESIAN_POINT('Ctrl Pts',(-11.1376238930657,31.0764769561007,21.1417587808808));
#45601=CARTESIAN_POINT('Ctrl Pts',(-11.1678934506043,31.0853806790487,21.1402136424091));
#45602=CARTESIAN_POINT('Ctrl Pts',(-11.1980430315782,31.0946296085407,21.1386685039373));
#45603=CARTESIAN_POINT('Ctrl Pts',(-11.3116761558715,31.129488625502,21.1328449101644));
#45604=CARTESIAN_POINT('Ctrl Pts',(-11.4239698392315,31.1693674834581,21.1270213163916));
#45605=CARTESIAN_POINT('Ctrl Pts',(-11.5344483324783,31.2141456294577,21.1211977226187));
#45606=CARTESIAN_POINT('Ctrl Pts',(-11.6447874407038,31.2588672811781,21.115381476174));
#45607=CARTESIAN_POINT('Ctrl Pts',(-11.7533155387359,31.3084757746901,21.1095652297293));
#45608=CARTESIAN_POINT('Ctrl Pts',(-11.8595713467884,31.3628006095069,21.1037489832845));
#45609=CARTESIAN_POINT('Ctrl Pts',(-11.9657207921956,31.4170710648668,21.0979385589343));
#45610=CARTESIAN_POINT('Ctrl Pts',(-12.0696021111229,31.4760482847061,21.0921281345841));
#45611=CARTESIAN_POINT('Ctrl Pts',(-12.1707739167872,31.539513675479,21.0863177102339));
#45612=CARTESIAN_POINT('Ctrl Pts',(-12.2757752820505,31.6053813609906,21.0802873494479));
#45613=CARTESIAN_POINT('Ctrl Pts',(-12.3778575445559,31.6760835353256,21.0742569886618));
#45614=CARTESIAN_POINT('Ctrl Pts',(-12.4765548627097,31.7513231905915,21.0682266278758));
#45615=CARTESIAN_POINT('Ctrl Pts',(-12.5715455007581,31.8237371426009,21.0624227435409));
#45616=CARTESIAN_POINT('Ctrl Pts',(-12.6634005056374,31.9003536323609,21.056618859206));
#45617=CARTESIAN_POINT('Ctrl Pts',(-12.7517346405485,31.9808641189895,21.0508149748711));
#45618=CARTESIAN_POINT('Ctrl Pts',(-12.8400557275596,32.0613627133548,21.0450119478323));
#45619=CARTESIAN_POINT('Ctrl Pts',(-12.9248566771465,32.1457538857377,21.0392089207934));
#45620=CARTESIAN_POINT('Ctrl Pts',(-13.0057868227125,32.2336900794726,21.0334058937545));
#45621=CARTESIAN_POINT('Ctrl Pts',(-13.0867241135586,32.3216340370481,21.0276023543695));
#45622=CARTESIAN_POINT('Ctrl Pts',(-13.1637896443656,32.413123337798,21.0217988149844));
#45623=CARTESIAN_POINT('Ctrl Pts',(-13.2366714207888,32.5077754688132,21.0159952755993));
#45624=CARTESIAN_POINT('Ctrl Pts',(-13.3095768319158,32.6024582944024,21.0101898541946));
#45625=CARTESIAN_POINT('Ctrl Pts',(-13.3782955414098,32.7003056667091,21.0043844327899));
#45626=CARTESIAN_POINT('Ctrl Pts',(-13.4425578412034,32.8009046155364,20.9985790113851));
#45627=CARTESIAN_POINT('Ctrl Pts',(-13.5068913055313,32.9016149683654,20.9927671610149));
#45628=CARTESIAN_POINT('Ctrl Pts',(-13.5667582894038,33.0050826356966,20.9869553106446));
#45629=CARTESIAN_POINT('Ctrl Pts',(-13.6219340944211,33.1108683434789,20.9811434602744));
#45630=CARTESIAN_POINT('Ctrl Pts',(-13.6771461391971,33.2167235318701,20.9753277926502));
#45631=CARTESIAN_POINT('Ctrl Pts',(-13.7276606964746,33.324899423677,20.9695121250261));
#45632=CARTESIAN_POINT('Ctrl Pts',(-13.7733011124365,33.4349365141039,20.963696457402));
#45633=CARTESIAN_POINT('Ctrl Pts',(-13.8190069033523,33.5451312207478,20.9578724594637));
#45634=CARTESIAN_POINT('Ctrl Pts',(-13.8598244786433,33.6571920648184,20.9520484615254));
#45635=CARTESIAN_POINT('Ctrl Pts',(-13.8956268883525,33.7706440113843,20.9462244635872));
#45636=CARTESIAN_POINT('Ctrl Pts',(-13.9051254566996,33.8007434118807,20.9446793261811));
#45637=CARTESIAN_POINT('Ctrl Pts',(-13.9142713021519,33.8309406722877,20.943134188775));
#45638=CARTESIAN_POINT('Ctrl Pts',(-13.923062660518,33.8612268172943,20.9415890513689));
#45639=CARTESIAN_POINT('Ctrl Pts',(-13.9640196809555,34.0023233587344,20.9343905933279));
#45640=CARTESIAN_POINT('Ctrl Pts',(-13.9973850464633,34.1457148908331,20.927192135287));
#45641=CARTESIAN_POINT('Ctrl Pts',(-14.0229437095927,34.2906700982983,20.9199936772461));
#45642=CARTESIAN_POINT('Ctrl Pts',(-14.0481513699598,34.4336346039029,20.9128940772184));
#45643=CARTESIAN_POINT('Ctrl Pts',(-14.0657652702748,34.5781201849237,20.9057944771907));
#45644=CARTESIAN_POINT('Ctrl Pts',(-14.0756251114016,34.7234047156716,20.898694877163));
#45645=CARTESIAN_POINT('Ctrl Pts',(-14.0817866583163,34.8141949668195,20.8942582419187));
#45646=CARTESIAN_POINT('Ctrl Pts',(-14.0849210219501,34.9052968107325,20.8898216066744));
#45647=CARTESIAN_POINT('Ctrl Pts',(-14.084998525967,34.996529719382,20.8853849714301));
#45648=CARTESIAN_POINT('Ctrl Pts',(-14.0849985259674,34.9965297199084,20.8853849714045));
#45649=CARTESIAN_POINT('Ctrl Pts',(-14.0851010661903,35.1172337115238,20.8795151642127));
#45650=CARTESIAN_POINT('Ctrl Pts',(-14.0798491529871,35.2380430359988,20.8736453570208));
#45651=CARTESIAN_POINT('Ctrl Pts',(-14.0692436282635,35.3584428738826,20.867775549829));
#45652=CARTESIAN_POINT('Ctrl Pts',(-14.0588381189791,35.4765720248277,20.862016444568));
#45653=CARTESIAN_POINT('Ctrl Pts',(-14.0432792039204,35.594306568102,20.8562573393069));
#45654=CARTESIAN_POINT('Ctrl Pts',(-14.0226202175485,35.7111621371884,20.8504982340459));
#45655=CARTESIAN_POINT('Ctrl Pts',(-14.0019643520335,35.8280000534476,20.8447399987861));
#45656=CARTESIAN_POINT('Ctrl Pts',(-13.9762100192018,35.9439588506284,20.8389817635263));
#45657=CARTESIAN_POINT('Ctrl Pts',(-13.9454620141955,36.058562466055,20.8332235282666));
#45658=CARTESIAN_POINT('Ctrl Pts',(-13.9147111095653,36.1731768889268,20.8274647499889));
#45659=CARTESIAN_POINT('Ctrl Pts',(-13.8789657046316,36.2864354749415,20.8217059717112));
#45660=CARTESIAN_POINT('Ctrl Pts',(-13.8383807969595,36.3978761953523,20.8159471934336));
#45661=CARTESIAN_POINT('Ctrl Pts',(-13.79642617796,36.5130779596051,20.8099940605475));
#45662=CARTESIAN_POINT('Ctrl Pts',(-13.7492997768768,36.6263365341239,20.8040409276614));
#45663=CARTESIAN_POINT('Ctrl Pts',(-13.6972267955671,36.7371640746171,20.7980877947753));
#45664=CARTESIAN_POINT('Ctrl Pts',(-13.6467793219885,36.8445320278283,20.7923204946049));
#45665=CARTESIAN_POINT('Ctrl Pts',(-13.5916897459076,36.9496181183724,20.7865531944344));
#45666=CARTESIAN_POINT('Ctrl Pts',(-13.5322089943319,37.0520050244482,20.780785894264));
#45667=CARTESIAN_POINT('Ctrl Pts',(-13.4698533786252,37.1593405640898,20.7747398450201));
#45668=CARTESIAN_POINT('Ctrl Pts',(-13.4026717823633,37.2637090316623,20.7686937957761));
#45669=CARTESIAN_POINT('Ctrl Pts',(-13.3310026043533,37.3646662871939,20.7626477465322));
#45670=CARTESIAN_POINT('Ctrl Pts',(-13.2593334263433,37.4656235427255,20.7566016972883));
#45671=CARTESIAN_POINT('Ctrl Pts',(-13.1831770448823,37.563169225137,20.7505556480444));
#45672=CARTESIAN_POINT('Ctrl Pts',(-13.102917086446,37.6569024360412,20.7445095988004));
#45673=CARTESIAN_POINT('Ctrl Pts',(-13.0256101762298,37.7471868700332,20.7386860051284));
#45674=CARTESIAN_POINT('Ctrl Pts',(-12.9442348728705,37.8342400379334,20.7328624114565));
#45675=CARTESIAN_POINT('Ctrl Pts',(-12.8590915555362,37.9176738126566,20.7270388177845));
#45676=CARTESIAN_POINT('Ctrl Pts',(-12.7740556591683,38.0010023232557,20.7212225714426));
#45677=CARTESIAN_POINT('Ctrl Pts',(-12.6852614933218,38.0807202398707,20.7154063251008));
#45678=CARTESIAN_POINT('Ctrl Pts',(-12.5930494621087,38.1564726336621,20.7095900787589));
#45679=CARTESIAN_POINT('Ctrl Pts',(-12.5009297356738,38.2321491988679,20.7037796545134));
#45680=CARTESIAN_POINT('Ctrl Pts',(-12.4053992638386,38.3038678803899,20.6979692302679));
#45681=CARTESIAN_POINT('Ctrl Pts',(-12.3068346110207,38.3713111807421,20.6921588060223));
#45682=CARTESIAN_POINT('Ctrl Pts',(-12.2045390821698,38.4413073495485,20.6861284451977));
#45683=CARTESIAN_POINT('Ctrl Pts',(-12.0989754539081,38.5066977643392,20.6800980843731));
#45684=CARTESIAN_POINT('Ctrl Pts',(-11.9906019499406,38.567173794041,20.6740677235485));
#45685=CARTESIAN_POINT('Ctrl Pts',(-11.8862985278857,38.6253785822895,20.6682638393222));
#45686=CARTESIAN_POINT('Ctrl Pts',(-11.7793928683705,38.6790312416888,20.6624599550958));
#45687=CARTESIAN_POINT('Ctrl Pts',(-11.6703216060842,38.727901652706,20.6566560708695));
#45688=CARTESIAN_POINT('Ctrl Pts',(-11.5612664548177,38.7767648450285,20.6508530439404));
#45689=CARTESIAN_POINT('Ctrl Pts',(-11.4500467094675,38.820847026836,20.6450500170113));
#45690=CARTESIAN_POINT('Ctrl Pts',(-11.3371209850514,38.8599653458723,20.6392469900822));
#45691=CARTESIAN_POINT('Ctrl Pts',(-11.2241852905032,38.8990871186373,20.6334434508079));
#45692=CARTESIAN_POINT('Ctrl Pts',(-11.1095437032821,38.933244023607,20.6276399115337));
#45693=CARTESIAN_POINT('Ctrl Pts',(-10.9936714595392,38.9623026172287,20.6218363722595));
#45694=CARTESIAN_POINT('Ctrl Pts',(-10.8777616398077,38.9913706342062,20.6160309509666));
#45695=CARTESIAN_POINT('Ctrl Pts',(-10.7606207657281,39.0153369524756,20.6102255296737));
#45696=CARTESIAN_POINT('Ctrl Pts',(-10.6427351272116,39.0341190557851,20.6044201083808));
#45697=CARTESIAN_POINT('Ctrl Pts',(-10.5247189413039,39.0529219585288,20.5986082581232));
#45698=CARTESIAN_POINT('Ctrl Pts',(-10.4059567481628,39.0665291224263,20.5927964078656));
#45699=CARTESIAN_POINT('Ctrl Pts',(-10.2869409963013,39.0749097983442,20.586984557608));
#45700=CARTESIAN_POINT('Ctrl Pts',(-10.1678470742798,39.0832959787333,20.5811688900972));
#45701=CARTESIAN_POINT('Ctrl Pts',(-10.0484996691281,39.0864488239077,20.5753532225864));
#45702=CARTESIAN_POINT('Ctrl Pts',(-9.92939060827338,39.0843897113033,20.5695375550756));
#45703=CARTESIAN_POINT('Ctrl Pts',(-9.81011093658415,39.0823276492429,20.5637135572507));
#45704=CARTESIAN_POINT('Ctrl Pts',(-9.69107069673944,39.0750387534088,20.5578895594258));
#45705=CARTESIAN_POINT('Ctrl Pts',(-9.57275612281357,39.0625961735578,20.5520655616009));
#45706=CARTESIAN_POINT('Ctrl Pts',(-9.54136661965563,39.0592950891135,20.5505204231446));
#45707=CARTESIAN_POINT('Ctrl Pts',(-9.51002813346101,39.0556315303432,20.5489752846882));
#45708=CARTESIAN_POINT('Ctrl Pts',(-9.47874959800879,39.0516074610485,20.5474301462319));
#45709=CARTESIAN_POINT('Ctrl Pts',(-9.36086616727409,39.0364414346629,20.541606784634));
#45710=CARTESIAN_POINT('Ctrl Pts',(-9.2434550920497,39.016101871959,20.5357834230361));
#45711=CARTESIAN_POINT('Ctrl Pts',(-9.12700558900731,38.9906272387152,20.5299600614382));
#45712=CARTESIAN_POINT('Ctrl Pts',(-9.01069687684402,38.9651834050533,20.5241437404559));
#45713=CARTESIAN_POINT('Ctrl Pts',(-8.8953478203895,38.9346169330401,20.5183274194737));
#45714=CARTESIAN_POINT('Ctrl Pts',(-8.78144188777357,38.8990179695825,20.5125110984915));
#45715=CARTESIAN_POINT('Ctrl Pts',(-8.66746502923026,38.8633968396807,20.5066911558545));
#45716=CARTESIAN_POINT('Ctrl Pts',(-8.55493349871637,38.822737008394,20.5008712132176));
#45717=CARTESIAN_POINT('Ctrl Pts',(-8.44432157315873,38.7771801164706,20.4950512705806));
#45718=CARTESIAN_POINT('Ctrl Pts',(-8.33397535865273,38.7317326609357,20.4892453085617));
#45719=CARTESIAN_POINT('Ctrl Pts',(-8.22553992374258,38.6814117788916,20.4834393465427));
#45720=CARTESIAN_POINT('Ctrl Pts',(-8.11947015931623,38.626407660247,20.4776333845238));
#45721=CARTESIAN_POINT('Ctrl Pts',(-8.01301727469707,38.5712048686944,20.4718064515778));
#45722=CARTESIAN_POINT('Ctrl Pts',(-7.90894757308101,38.5112850853853,20.4659795186319));
#45723=CARTESIAN_POINT('Ctrl Pts',(-7.80769890231647,38.4468885820542,20.4601525856859));
#45724=CARTESIAN_POINT('Ctrl Pts',(-7.70645023155192,38.3824920787231,20.45432565274));
#45725=CARTESIAN_POINT('Ctrl Pts',(-7.60802294883767,38.3136190698864,20.448498719794));
#45726=CARTESIAN_POINT('Ctrl Pts',(-7.51282733495086,38.2405550657615,20.4426717868481));
#45727=CARTESIAN_POINT('',(-14.0849985032409,35.0034969300359,20.9896150285484));
#45728=CARTESIAN_POINT('Ctrl Pts',(-14.0849985032409,35.0034969300359,20.9896150285484));
#45729=CARTESIAN_POINT('Ctrl Pts',(-14.0848731076928,35.149979879647,20.982490506098));
#45730=CARTESIAN_POINT('Ctrl Pts',(-14.0768649533832,35.2961228114989,20.9753659836477));
#45731=CARTESIAN_POINT('Ctrl Pts',(-14.0611057921048,35.4411856132435,20.9682414611973));
#45732=CARTESIAN_POINT('Ctrl Pts',(-14.0451084213706,35.5884411288293,20.9610092471899));
#45733=CARTESIAN_POINT('Ctrl Pts',(-14.0211239958759,35.7345836848413,20.9537770331826));
#45734=CARTESIAN_POINT('Ctrl Pts',(-13.9893392113713,35.8788615685165,20.9465448191752));
#45735=CARTESIAN_POINT('Ctrl Pts',(-13.9714671903015,35.9599864657635,20.9424782734007));
#45736=CARTESIAN_POINT('Ctrl Pts',(-13.9511298671922,36.0405222226871,20.9384117276261));
#45737=CARTESIAN_POINT('Ctrl Pts',(-13.9283670284786,36.120338113947,20.9343451818516));
#45738=CARTESIAN_POINT('Ctrl Pts',(-13.8957689635322,36.2346403606827,20.9285215881894));
#45739=CARTESIAN_POINT('Ctrl Pts',(-13.8581254755738,36.3477030066093,20.9226979945273));
#45740=CARTESIAN_POINT('Ctrl Pts',(-13.8155476565826,36.4590480048124,20.9168744008651));
#45741=CARTESIAN_POINT('Ctrl Pts',(-13.7730235558362,36.5702525247569,20.9110581545316));
#45742=CARTESIAN_POINT('Ctrl Pts',(-13.7255776507761,36.6797433291843,20.9052419081981));
#45743=CARTESIAN_POINT('Ctrl Pts',(-13.6733712581126,36.7870558469371,20.8994256618646));
#45744=CARTESIAN_POINT('Ctrl Pts',(-13.6212171243382,36.8942609442635,20.8936152376259));
#45745=CARTESIAN_POINT('Ctrl Pts',(-13.5643121604916,36.9992917276244,20.8878048133873));
#45746=CARTESIAN_POINT('Ctrl Pts',(-13.5028661614887,37.1017025609485,20.8819943891487));
#45747=CARTESIAN_POINT('Ctrl Pts',(-13.439094304187,37.2079898563765,20.875964028321));
#45748=CARTESIAN_POINT('Ctrl Pts',(-13.3704310041989,37.3114545231373,20.8699336674932));
#45749=CARTESIAN_POINT('Ctrl Pts',(-13.29716397028,37.4116249196522,20.8639033066655));
#45750=CARTESIAN_POINT('Ctrl Pts',(-13.2266485576238,37.5080333105528,20.8580994224424));
#45751=CARTESIAN_POINT('Ctrl Pts',(-13.151869234024,37.6013900493696,20.8522955382194));
#45752=CARTESIAN_POINT('Ctrl Pts',(-13.0731268378601,37.6913038547187,20.8464916539963));
#45753=CARTESIAN_POINT('Ctrl Pts',(-12.9943960727923,37.781204378835,20.8406886270691));
#45754=CARTESIAN_POINT('Ctrl Pts',(-12.9117036682631,37.8676626737381,20.834885600142));
#45755=CARTESIAN_POINT('Ctrl Pts',(-12.8253901565136,37.9503212475044,20.8290825732148));
#45756=CARTESIAN_POINT('Ctrl Pts',(-12.7390690241855,38.0329871191566,20.8232790339412));
#45757=CARTESIAN_POINT('Ctrl Pts',(-12.6491264439136,38.1118523202253,20.8174754946676));
#45758=CARTESIAN_POINT('Ctrl Pts',(-12.5559386644293,38.1865973300176,20.811671955394));
#45759=CARTESIAN_POINT('Ctrl Pts',(-12.4627206652368,38.2613665787434,20.8058665341004));
#45760=CARTESIAN_POINT('Ctrl Pts',(-12.3662556922538,38.3320127235715,20.8000611128068));
#45761=CARTESIAN_POINT('Ctrl Pts',(-12.2669512843216,38.3982579175973,20.7942556915132));
#45762=CARTESIAN_POINT('Ctrl Pts',(-12.1675369059512,38.4645764720424,20.7884438412529));
#45763=CARTESIAN_POINT('Ctrl Pts',(-12.0652771560088,38.5264841207323,20.7826319909927));
#45764=CARTESIAN_POINT('Ctrl Pts',(-11.9606067648518,38.5837474957951,20.7768201407325));
#45765=CARTESIAN_POINT('Ctrl Pts',(-11.8558676256214,38.6410484817492,20.7710044732179));
#45766=CARTESIAN_POINT('Ctrl Pts',(-11.7487150575937,38.6936989394978,20.7651888057033));
#45767=CARTESIAN_POINT('Ctrl Pts',(-11.6396049709297,38.74151313499,20.7593731381887));
#45768=CARTESIAN_POINT('Ctrl Pts',(-11.5303385958489,38.7893958191539,20.7535491403584));
#45769=CARTESIAN_POINT('Ctrl Pts',(-11.4191094851098,38.8324282674881,20.7477251425281));
#45770=CARTESIAN_POINT('Ctrl Pts',(-11.3063900619071,38.8704741319573,20.7419011446978));
#45771=CARTESIAN_POINT('Ctrl Pts',(-11.2764849825518,38.8805679078458,20.7403560062263));
#45772=CARTESIAN_POINT('Ctrl Pts',(-11.2464750655801,38.8903109709657,20.7388108677547));
#45773=CARTESIAN_POINT('Ctrl Pts',(-11.2163692495601,38.8997013794295,20.7372657292832));
#45774=CARTESIAN_POINT('Ctrl Pts',(-11.1028985208678,38.9350944240956,20.7314420044528));
#45775=CARTESIAN_POINT('Ctrl Pts',(-10.9876987634882,38.965587897618,20.7256182796223));
#45776=CARTESIAN_POINT('Ctrl Pts',(-10.8712307299976,38.991012655343,20.7197945547919));
#45777=CARTESIAN_POINT('Ctrl Pts',(-10.7549102795949,39.016405195951,20.7139782095253));
#45778=CARTESIAN_POINT('Ctrl Pts',(-10.6373251451083,39.0367417096102,20.7081618642587));
#45779=CARTESIAN_POINT('Ctrl Pts',(-10.5189523331906,39.0519024514265,20.7023455189922));
#45780=CARTESIAN_POINT('Ctrl Pts',(-10.4006986643615,39.0670479338469,20.6965350279191));
#45781=CARTESIAN_POINT('Ctrl Pts',(-10.28165929806,39.0770279566943,20.6907245368459));
#45782=CARTESIAN_POINT('Ctrl Pts',(-10.1623219706014,39.0817737048813,20.6849140457728));
#45783=CARTESIAN_POINT('Ctrl Pts',(-10.0430738621129,39.086515905052,20.6791078987389));
#45784=CARTESIAN_POINT('Ctrl Pts',(-9.92352864238431,39.0860316015774,20.673301751705));
#45785=CARTESIAN_POINT('Ctrl Pts',(-9.80417911357673,39.0803038098211,20.6674956046711));
#45786=CARTESIAN_POINT('Ctrl Pts',(-9.6848774062533,39.074578313101,20.6616917840692));
#45787=CARTESIAN_POINT('Ctrl Pts',(-9.56577164113457,39.0636135255086,20.6558879634673));
#45788=CARTESIAN_POINT('Ctrl Pts',(-9.44735408749383,39.0474445635969,20.6500841428655));
#45789=CARTESIAN_POINT('Ctrl Pts',(-9.32895603525967,39.031278264445,20.6442812780565));
#45790=CARTESIAN_POINT('Ctrl Pts',(-9.21124637345403,39.0099095510758,20.6384784132476));
#45791=CARTESIAN_POINT('Ctrl Pts',(-9.09471107987942,38.9834252812256,20.6326755484387));
#45792=CARTESIAN_POINT('Ctrl Pts',(-8.97816747571492,38.956939122678,20.6268722698047));
#45793=CARTESIAN_POINT('Ctrl Pts',(-8.86279880429894,38.9253367733678,20.6210689911707));
#45794=CARTESIAN_POINT('Ctrl Pts',(-8.74907907106665,38.8887558202536,20.6152657125367));
#45795=CARTESIAN_POINT('Ctrl Pts',(-8.6352596005273,38.8521427840028,20.609457344167));
#45796=CARTESIAN_POINT('Ctrl Pts',(-8.52309234671557,38.810542545988,20.6036489757974));
#45797=CARTESIAN_POINT('Ctrl Pts',(-8.41303458850368,38.7641421044794,20.5978406074277));
#45798=CARTESIAN_POINT('Ctrl Pts',(-8.3029290834294,38.7177215328542,20.5920297191869));
#45799=CARTESIAN_POINT('Ctrl Pts',(-8.1949352672077,38.6664967819516,20.5862188309461));
#45800=CARTESIAN_POINT('Ctrl Pts',(-8.0894874175106,38.6107016869508,20.5804079427053));
#45801=CARTESIAN_POINT('Ctrl Pts',(-7.98388384687261,38.554824196105,20.5745884731896));
#45802=CARTESIAN_POINT('Ctrl Pts',(-7.88083410901292,38.4943630802427,20.568769003674));
#45803=CARTESIAN_POINT('Ctrl Pts',(-7.78074545011815,38.429596804703,20.5629495341583));
#45804=CARTESIAN_POINT('Ctrl Pts',(-7.6888464767986,38.3701299850496,20.5576062387274));
#45805=CARTESIAN_POINT('Ctrl Pts',(-7.59944368418054,38.3070343607522,20.5522629432965));
#45806=CARTESIAN_POINT('Ctrl Pts',(-7.51282733495085,38.2405550657615,20.5469196478657));
#45807=CARTESIAN_POINT('Ctrl Pts',(-7.51282733495087,38.2405550657615,21.796951697066));
#45808=CARTESIAN_POINT('Ctrl Pts',(-7.4180311178499,38.1677976044195,21.7911462584032));
#45809=CARTESIAN_POINT('Ctrl Pts',(-7.32646749484719,38.0909057833876,21.7853408197403));
#45810=CARTESIAN_POINT('Ctrl Pts',(-7.23850323443017,38.0102093969934,21.7795353810774));
#45811=CARTESIAN_POINT('Ctrl Pts',(-7.15044149746005,37.9294235878546,21.7737235091864));
#45812=CARTESIAN_POINT('Ctrl Pts',(-7.06598738566451,37.8448250741453,21.7679116372954));
#45813=CARTESIAN_POINT('Ctrl Pts',(-6.98547092660869,37.7567806343049,21.7620997654045));
#45814=CARTESIAN_POINT('Ctrl Pts',(-6.90490146889063,37.6686782406302,21.7562840679425));
#45815=CARTESIAN_POINT('Ctrl Pts',(-6.82827508719332,37.5771257160173,21.7504683704804));
#45816=CARTESIAN_POINT('Ctrl Pts',(-6.75588057567389,37.4825217341868,21.7446526730184));
#45817=CARTESIAN_POINT('Ctrl Pts',(-6.68338249601108,37.3877824111744,21.738828655575));
#45818=CARTESIAN_POINT('Ctrl Pts',(-6.61512860297032,37.2899832515262,21.7330046381316));
#45819=CARTESIAN_POINT('Ctrl Pts',(-6.55136364389892,37.1895507035412,21.7271806206882));
#45820=CARTESIAN_POINT('Ctrl Pts',(-6.53487637640687,37.1635825494382,21.7256747445006));
#45821=CARTESIAN_POINT('Ctrl Pts',(-6.51868897258072,37.1374384598219,21.724168868313));
#45822=CARTESIAN_POINT('Ctrl Pts',(-6.50280514828385,37.1111260429283,21.7226629921254));
#45823=CARTESIAN_POINT('Ctrl Pts',(-6.44137849223954,37.0093694538341,21.7168393984561));
#45824=CARTESIAN_POINT('Ctrl Pts',(-6.38429762830083,36.9047655862678,21.7110158047867));
#45825=CARTESIAN_POINT('Ctrl Pts',(-6.33183666579976,36.7977215450756,21.7051922111174));
#45826=CARTESIAN_POINT('Ctrl Pts',(-6.27944189059542,36.6908125558416,21.6993759647765));
#45827=CARTESIAN_POINT('Ctrl Pts',(-6.23165560181378,36.5814698797651,21.6935597184356));
#45828=CARTESIAN_POINT('Ctrl Pts',(-6.18870781714492,36.4701281906377,21.6877434720948));
#45829=CARTESIAN_POINT('Ctrl Pts',(-6.14580302344537,36.3588979551552,21.6819330478485));
#45830=CARTESIAN_POINT('Ctrl Pts',(-6.10772724468464,36.2456730661968,21.6761226236023));
#45831=CARTESIAN_POINT('Ctrl Pts',(-6.07466360223744,36.1309107676561,21.6703121993561));
#45832=CARTESIAN_POINT('Ctrl Pts',(-6.04034843251919,36.0118044786872,21.6642818385311));
#45833=CARTESIAN_POINT('Ctrl Pts',(-6.01143253294929,35.8910424947053,21.6582514777062));
#45834=CARTESIAN_POINT('Ctrl Pts',(-5.98806495335441,35.7691567990318,21.6522211168812));
#45835=CARTESIAN_POINT('Ctrl Pts',(-5.9655749679841,35.6518486498751,21.64641723265));
#45836=CARTESIAN_POINT('Ctrl Pts',(-5.94822415578516,35.5335001083631,21.6406133484189));
#45837=CARTESIAN_POINT('Ctrl Pts',(-5.93609381245957,35.4145979967035,21.6348094641877));
#45838=CARTESIAN_POINT('Ctrl Pts',(-5.92396526091538,35.2957134481571,21.6290064372523));
#45839=CARTESIAN_POINT('Ctrl Pts',(-5.91705568616431,35.1762758981931,21.6232034103169));
#45840=CARTESIAN_POINT('Ctrl Pts',(-5.91539460443507,35.0567781870249,21.6174003833815));
#45841=CARTESIAN_POINT('Ctrl Pts',(-5.91373337604967,34.9372699254579,21.6115968440995));
#45842=CARTESIAN_POINT('Ctrl Pts',(-5.91732156768735,34.8177019004437,21.6057933048175));
#45843=CARTESIAN_POINT('Ctrl Pts',(-5.92613656673833,34.6985672095915,21.5999897655354));
#45844=CARTESIAN_POINT('Ctrl Pts',(-5.93495442439076,34.5793938847476,21.5941843442333));
#45845=CARTESIAN_POINT('Ctrl Pts',(-5.94900243029866,34.460654580553,21.5883789229311));
#45846=CARTESIAN_POINT('Ctrl Pts',(-5.96820615034577,34.3428368894328,21.5825735016289));
#45847=CARTESIAN_POINT('Ctrl Pts',(-5.98743113673544,34.2248887261243,21.57676165136));
#45848=CARTESIAN_POINT('Ctrl Pts',(-6.01182316813872,34.1078646163548,21.5709498010911));
#45849=CARTESIAN_POINT('Ctrl Pts',(-6.0412567294953,33.9922417362116,21.5651379508221));
#45850=CARTESIAN_POINT('Ctrl Pts',(-6.07070962297316,33.8765429143393,21.5593222832987));
#45851=CARTESIAN_POINT('Ctrl Pts',(-6.10521052322021,33.7622475449808,21.5535066157753));
#45852=CARTESIAN_POINT('Ctrl Pts',(-6.1445846228837,33.649815838526,21.5476909482518));
#45853=CARTESIAN_POINT('Ctrl Pts',(-6.18401512169361,33.5372230857914,21.5418669504126));
#45854=CARTESIAN_POINT('Ctrl Pts',(-6.22833260108606,33.4264997018816,21.5360429525734));
#45855=CARTESIAN_POINT('Ctrl Pts',(-6.2773148598132,33.3180843222586,21.5302189547342));
#45856=CARTESIAN_POINT('Ctrl Pts',(-6.29031012021587,33.2893211307181,21.5286738163418));
#45857=CARTESIAN_POINT('Ctrl Pts',(-6.30363347546003,33.2607202478935,21.5271286779494));
#45858=CARTESIAN_POINT('Ctrl Pts',(-6.31728025454018,33.2322895383009,21.525583539557));
#45859=CARTESIAN_POINT('Ctrl Pts',(-6.36871467403732,33.1251347997945,21.5197599458878));
#45860=CARTESIAN_POINT('Ctrl Pts',(-6.42491268003554,33.0200539820572,21.5139363522187));
#45861=CARTESIAN_POINT('Ctrl Pts',(-6.48568403854052,32.9174995022735,21.5081127585496));
#45862=CARTESIAN_POINT('Ctrl Pts',(-6.54637872494952,32.8150744101999,21.5022965122089));
#45863=CARTESIAN_POINT('Ctrl Pts',(-6.61163508121126,32.7151696647093,21.4964802658682));
#45864=CARTESIAN_POINT('Ctrl Pts',(-6.68121564602866,32.6182159183009,21.4906640195275));
#45865=CARTESIAN_POINT('Ctrl Pts',(-6.75072656031655,32.521359223128,21.4848535952816));
#45866=CARTESIAN_POINT('Ctrl Pts',(-6.82455283531785,32.4274479803262,21.4790431710356));
#45867=CARTESIAN_POINT('Ctrl Pts',(-6.90241242590131,32.3368859917778,21.4732327467896));
#45868=CARTESIAN_POINT('Ctrl Pts',(-6.98321916307439,32.2428960445964,21.4672023859646));
#45869=CARTESIAN_POINT('Ctrl Pts',(-7.06837035901901,32.1525142994728,21.4611720251395));
#45870=CARTESIAN_POINT('Ctrl Pts',(-7.15750278192142,32.0661570312616,21.4551416643145));
#45871=CARTESIAN_POINT('Ctrl Pts',(-7.24328774218274,31.9830430018149,21.4493377800837));
#45872=CARTESIAN_POINT('Ctrl Pts',(-7.33275996413731,31.9036569233247,21.4435338958528));
#45873=CARTESIAN_POINT('Ctrl Pts',(-7.42555684708045,31.8283336473731,21.437730011622));
#45874=CARTESIAN_POINT('Ctrl Pts',(-7.51834002293136,31.7530214974751,21.431926984687));
#45875=CARTESIAN_POINT('Ctrl Pts',(-7.61444656619753,31.6817712139399,21.4261239577519));
#45876=CARTESIAN_POINT('Ctrl Pts',(-7.71348045926666,31.6148776403438,21.4203209308169));
#45877=CARTESIAN_POINT('Ctrl Pts',(-7.81252309599266,31.5479781607448,21.4145173915353));
#45878=CARTESIAN_POINT('Ctrl Pts',(-7.91449325799753,31.4854363844379,21.4087138522537));
#45879=CARTESIAN_POINT('Ctrl Pts',(-8.01896613726001,31.427503697038,21.4029103129721));
#45880=CARTESIAN_POINT('Ctrl Pts',(-8.12347289585904,31.369552222743,21.3971048916703));
#45881=CARTESIAN_POINT('Ctrl Pts',(-8.2304836288856,31.3162130078463,21.3912994703686));
#45882=CARTESIAN_POINT('Ctrl Pts',(-8.33954972603321,31.2676910782086,21.3854940490669));
#45883=CARTESIAN_POINT('Ctrl Pts',(-8.44873660378823,31.2191154150251,21.3796821987984));
#45884=CARTESIAN_POINT('Ctrl Pts',(-8.55998301570261,31.1753678516908,21.3738703485299));
#45885=CARTESIAN_POINT('Ctrl Pts',(-8.6728210626815,31.1366049815819,21.3680584982614));
#45886=CARTESIAN_POINT('Ctrl Pts',(-8.78573322229546,31.0978166518117,21.3622428307385));
#45887=CARTESIAN_POINT('Ctrl Pts',(-8.90023870816946,31.0640196507947,21.3564271632156));
#45888=CARTESIAN_POINT('Ctrl Pts',(-9.01585679058879,31.0353200452786,21.3506114956926));
#45889=CARTESIAN_POINT('Ctrl Pts',(-9.13164048342669,31.0065793306766,21.344787497854));
#45890=CARTESIAN_POINT('Ctrl Pts',(-9.24853955487536,30.9829506655232,21.3389635000153));
#45891=CARTESIAN_POINT('Ctrl Pts',(-9.36606534026051,30.9644886510901,21.3331395021766));
#45892=CARTESIAN_POINT('Ctrl Pts',(-9.39724557221665,30.9595905779522,21.3315943637806));
#45893=CARTESIAN_POINT('Ctrl Pts',(-9.42846990348814,30.9550558856007,21.3300492253845));
#45894=CARTESIAN_POINT('Ctrl Pts',(-9.45972919594568,30.9508849783827,21.3285040869885));
#45895=CARTESIAN_POINT('Ctrl Pts',(-9.57754480302819,30.9351649179674,21.3226804933035));
#45896=CARTESIAN_POINT('Ctrl Pts',(-9.69623706723345,30.9245658317069,21.3168568996184));
#45897=CARTESIAN_POINT('Ctrl Pts',(-9.81532332053317,30.9191766119984,21.3110333059334));
#45898=CARTESIAN_POINT('Ctrl Pts',(-9.93425932883662,30.913794191591,21.3052170595767));
#45899=CARTESIAN_POINT('Ctrl Pts',(-10.0535879332387,30.9136085824498,21.2994008132201));
#45900=CARTESIAN_POINT('Ctrl Pts',(-10.1728187807789,30.9186572468108,21.2935845668634));
#45901=CARTESIAN_POINT('Ctrl Pts',(-10.2919302775845,30.923700857431,21.2877741426014));
#45902=CARTESIAN_POINT('Ctrl Pts',(-10.4109438065726,30.9339683009686,21.2819637183394));
#45903=CARTESIAN_POINT('Ctrl Pts',(-10.5293670326301,30.9494450324969,21.2761532940774));
#45904=CARTESIAN_POINT('Ctrl Pts',(-10.6522728223415,30.9655075902734,21.2701229332583));
#45905=CARTESIAN_POINT('Ctrl Pts',(-10.7745422900183,30.9871816129408,21.2640925724392));
#45906=CARTESIAN_POINT('Ctrl Pts',(-10.8956281649368,31.0143914906037,21.2580622116202));
#45907=CARTESIAN_POINT('Ctrl Pts',(-11.0121665318834,31.0405794725611,21.2522583273734));
#45908=CARTESIAN_POINT('Ctrl Pts',(-11.1276081707663,31.0718949007598,21.2464544431266));
#45909=CARTESIAN_POINT('Ctrl Pts',(-11.2414742568829,31.1082180598732,21.2406505588797));
#45910=CARTESIAN_POINT('Ctrl Pts',(-11.3553235237601,31.1445358536673,21.2348475319287));
#45911=CARTESIAN_POINT('Ctrl Pts',(-11.4675973117717,31.185859783291,21.2290445049777));
#45912=CARTESIAN_POINT('Ctrl Pts',(-11.5778319398252,31.2320202535487,21.2232414780267));
#45913=CARTESIAN_POINT('Ctrl Pts',(-11.6880763004424,31.2781847992926,21.2174379387292));
#45914=CARTESIAN_POINT('Ctrl Pts',(-11.7962807664794,31.3291865769534,21.2116343994316));
#45915=CARTESIAN_POINT('Ctrl Pts',(-11.9020022219751,31.3848080897964,21.2058308601341));
#45916=CARTESIAN_POINT('Ctrl Pts',(-12.007757961704,31.4404476400463,21.2000254388166));
#45917=CARTESIAN_POINT('Ctrl Pts',(-12.1110287283191,31.5007097148868,21.194220017499));
#45918=CARTESIAN_POINT('Ctrl Pts',(-12.2113971322741,31.5653314973101,21.1884145961814));
#45919=CARTESIAN_POINT('Ctrl Pts',(-12.3118766849435,31.6300248423742,21.1826027458973));
#45920=CARTESIAN_POINT('Ctrl Pts',(-12.4094471158047,31.699087310885,21.1767908956131));
#45921=CARTESIAN_POINT('Ctrl Pts',(-12.5037209694331,31.7722134043247,21.170979045329));
#45922=CARTESIAN_POINT('Ctrl Pts',(-12.5980567426327,31.8453875273736,21.1651633777905));
#45923=CARTESIAN_POINT('Ctrl Pts',(-12.6890913158874,31.9226303271731,21.159347710252));
#45924=CARTESIAN_POINT('Ctrl Pts',(-12.7764724595077,32.0035978771875,21.1535320427135));
#45925=CARTESIAN_POINT('Ctrl Pts',(-12.8639787671778,32.0846814044716,21.1477080448594));
#45926=CARTESIAN_POINT('Ctrl Pts',(-12.9478209141016,32.1695000415701,21.1418840470054));
#45927=CARTESIAN_POINT('Ctrl Pts',(-13.0276853651733,32.2576750138768,21.1360600491513));
#45928=CARTESIAN_POINT('Ctrl Pts',(-13.0488738375526,32.2810683126499,21.1345149109076));
#45929=CARTESIAN_POINT('Ctrl Pts',(-13.0697825624206,32.3046976868828,21.1329697726638));
#45930=CARTESIAN_POINT('Ctrl Pts',(-13.0904061924051,32.3285557153585,21.1314246344201));
#45931=CARTESIAN_POINT('Ctrl Pts',(-13.1692726209863,32.4197907452863,21.125515900844));
#45932=CARTESIAN_POINT('Ctrl Pts',(-13.2442376687111,32.5146859736304,21.119607167268));
#45933=CARTESIAN_POINT('Ctrl Pts',(-13.3149406608934,32.6128692087036,21.113698433692));
#45934=CARTESIAN_POINT('Ctrl Pts',(-13.3839459164557,32.7086948452011,21.1079315819948));
#45935=CARTESIAN_POINT('Ctrl Pts',(-13.4488911827402,32.8076520351367,21.1021647302976));
#45936=CARTESIAN_POINT('Ctrl Pts',(-13.5094788137178,32.9093581234305,21.0963978786004));
#45937=CARTESIAN_POINT('Ctrl Pts',(-13.5700104610616,33.0109702341862,21.0906363555373));
#45938=CARTESIAN_POINT('Ctrl Pts',(-13.6261922654222,33.1153258395129,21.0848748324742));
#45939=CARTESIAN_POINT('Ctrl Pts',(-13.6777687647287,33.2220118354765,21.079113309411));
#45940=CARTESIAN_POINT('Ctrl Pts',(-13.7293102997805,33.3286255078743,21.0733556921454));
#45941=CARTESIAN_POINT('Ctrl Pts',(-13.7762525571435,33.4375660566901,21.0675980748797));
#45942=CARTESIAN_POINT('Ctrl Pts',(-13.8183854556803,33.5483948498821,21.061840457614));
#45943=CARTESIAN_POINT('Ctrl Pts',(-13.8624295242045,33.6642508942395,21.0558216718625));
#45944=CARTESIAN_POINT('Ctrl Pts',(-13.9012174237266,33.7821701041747,21.0498028861109));
#45945=CARTESIAN_POINT('Ctrl Pts',(-13.9345650358086,33.901627122061,21.0437841003594));
#45946=CARTESIAN_POINT('Ctrl Pts',(-13.9664521067653,34.0158522244831,21.0380289222117));
#45947=CARTESIAN_POINT('Ctrl Pts',(-13.9933652579045,34.1314828387702,21.032273744064));
#45948=CARTESIAN_POINT('Ctrl Pts',(-14.0151946311385,34.2480444999362,21.0265185659163));
#45949=CARTESIAN_POINT('Ctrl Pts',(-14.0370247942147,34.364610378599,21.0207631795317));
#45950=CARTESIAN_POINT('Ctrl Pts',(-14.0537707443973,34.4821069611363,21.015007793147));
#45951=CARTESIAN_POINT('Ctrl Pts',(-14.0653740111759,34.6000510666906,21.0092524067624));
#45952=CARTESIAN_POINT('Ctrl Pts',(-14.0769833472086,34.7180568645902,21.0034940099409));
#45953=CARTESIAN_POINT('Ctrl Pts',(-14.0834446009016,34.8365102381816,20.9977356131194));
#45954=CARTESIAN_POINT('Ctrl Pts',(-14.0847513050874,34.9549247785714,20.9919772162979));
#45955=CARTESIAN_POINT('Ctrl Pts',(-14.0849299821656,34.9711166331078,20.9911898203971));
#45956=CARTESIAN_POINT('Ctrl Pts',(-14.0850123618426,34.9873077634264,20.9904024244963));
#45957=CARTESIAN_POINT('Ctrl Pts',(-14.0849985032417,35.0034969290672,20.9896150285955));
#45958=CARTESIAN_POINT('Origin',(-10.,35.,32.7603849714045));
#45959=CARTESIAN_POINT('',(-7.51282733495086,38.2405550657615,23.0467784846721));
#45960=CARTESIAN_POINT('',(-7.51282733495087,38.2405550657615,22.942760002634));
#45961=CARTESIAN_POINT('',(-7.51282733495086,38.2405550657615,32.7603849714045));
#45962=CARTESIAN_POINT('',(-14.084999774902,35.0013561158978,22.1353849714381));
#45963=CARTESIAN_POINT('Ctrl Pts',(-7.51282733495087,38.2405550657615,22.942760002634));
#45964=CARTESIAN_POINT('Ctrl Pts',(-7.41810510545334,38.1678543909703,22.9369372088697));
#45965=CARTESIAN_POINT('Ctrl Pts',(-7.32667850440273,38.0910780862914,22.9311144151054));
#45966=CARTESIAN_POINT('Ctrl Pts',(-7.23889853618177,38.0105719899217,22.9252916213411));
#45967=CARTESIAN_POINT('Ctrl Pts',(-7.17403461442627,37.9510830057991,22.9209889399118));
#45968=CARTESIAN_POINT('Ctrl Pts',(-7.11116111779867,37.8895582518679,22.9166862584826));
#45969=CARTESIAN_POINT('Ctrl Pts',(-7.05040557842172,37.8261489253389,22.9123835770533));
#45970=CARTESIAN_POINT('Ctrl Pts',(-6.968174165185,37.7403256640143,22.9065599833816));
#45971=CARTESIAN_POINT('Ctrl Pts',(-6.88955900838778,37.6507720416984,22.9007363897099));
#45972=CARTESIAN_POINT('Ctrl Pts',(-6.8149167632981,37.5578252042078,22.8949127960382));
#45973=CARTESIAN_POINT('Ctrl Pts',(-6.74036869048772,37.4649956329587,22.889096549695));
#45974=CARTESIAN_POINT('Ctrl Pts',(-6.66978381322939,37.3687816770076,22.8832803033517));
#45975=CARTESIAN_POINT('Ctrl Pts',(-6.60348180785171,37.2695570427741,22.8774640570085));
#45976=CARTESIAN_POINT('Ctrl Pts',(-6.53724617114725,37.1704317329471,22.8716536327599));
#45977=CARTESIAN_POINT('Ctrl Pts',(-6.47528510307411,37.0683020777964,22.8658432085113));
#45978=CARTESIAN_POINT('Ctrl Pts',(-6.41787746912869,36.9635740815727,22.8600327842627));
#45979=CARTESIAN_POINT('Ctrl Pts',(-6.35829683750226,36.8548819140831,22.8540024234387));
#45980=CARTESIAN_POINT('Ctrl Pts',(-6.30362144545678,36.7433911632484,22.8479720626146));
#45981=CARTESIAN_POINT('Ctrl Pts',(-6.25411329246119,36.6295882223077,22.8419417017905));
#45982=CARTESIAN_POINT('Ctrl Pts',(-6.20646447061094,36.5200592714014,22.836137817557));
#45983=CARTESIAN_POINT('Ctrl Pts',(-6.16360194235753,36.4083890800178,22.8303339333236));
#45984=CARTESIAN_POINT('Ctrl Pts',(-6.12571170368778,36.2950348246507,22.8245300490901));
#45985=CARTESIAN_POINT('Ctrl Pts',(-6.08782706181148,36.1816973129194,22.8187270221524));
#45986=CARTESIAN_POINT('Ctrl Pts',(-6.05491337832601,36.0666766190678,22.8129239952147));
#45987=CARTESIAN_POINT('Ctrl Pts',(-6.02710744688957,35.9504471376356,22.807120968277));
#45988=CARTESIAN_POINT('Ctrl Pts',(-5.99929906048016,35.8342073943556,22.8013174289927));
#45989=CARTESIAN_POINT('Ctrl Pts',(-5.97659941775083,35.7167590484535,22.7955138897084));
#45990=CARTESIAN_POINT('Ctrl Pts',(-5.95909450684949,35.5985881684648,22.7897103504241));
#45991=CARTESIAN_POINT('Ctrl Pts',(-5.94158391930968,35.4803789670377,22.7839049291197));
#45992=CARTESIAN_POINT('Ctrl Pts',(-5.92927147367316,35.361447169257,22.7780995078153));
#45993=CARTESIAN_POINT('Ctrl Pts',(-5.92219138970121,35.2422848277813,22.7722940865109));
#45994=CARTESIAN_POINT('Ctrl Pts',(-5.9151034651916,35.1229905250422,22.7664822362397));
#45995=CARTESIAN_POINT('Ctrl Pts',(-5.91325949261094,35.0034655768557,22.7606703859686));
#45996=CARTESIAN_POINT('Ctrl Pts',(-5.91664156972959,34.8842030659318,22.7548585356974));
#45997=CARTESIAN_POINT('Ctrl Pts',(-5.92002586821465,34.7648622227506,22.7490428681718));
#45998=CARTESIAN_POINT('Ctrl Pts',(-5.92864302289951,34.6457845664473,22.7432272006462));
#45999=CARTESIAN_POINT('Ctrl Pts',(-5.94242331960044,34.5274574276558,22.7374115331206));
#46000=CARTESIAN_POINT('Ctrl Pts',(-5.95622335508837,34.4089607980151,22.7315875352793));
#46001=CARTESIAN_POINT('Ctrl Pts',(-5.97520122914806,34.2912172333013,22.7257635374379));
#46002=CARTESIAN_POINT('Ctrl Pts',(-5.99923625789207,34.1747033988713,22.7199395395966));
#46003=CARTESIAN_POINT('Ctrl Pts',(-6.00561288201908,34.1437916435466,22.718394401226));
#46004=CARTESIAN_POINT('Ctrl Pts',(-6.01234519332935,34.1129663576641,22.7168492628554));
#46005=CARTESIAN_POINT('Ctrl Pts',(-6.01943035767116,34.0822362381473,22.7153041244848));
#46006=CARTESIAN_POINT('Ctrl Pts',(-6.04613419145458,33.9664150709686,22.7094805308136));
#46007=CARTESIAN_POINT('Ctrl Pts',(-6.07794029159737,33.8515735883069,22.7036569371423));
#46008=CARTESIAN_POINT('Ctrl Pts',(-6.11476218449409,33.7381948973939,22.697833343471));
#46009=CARTESIAN_POINT('Ctrl Pts',(-6.15153762110351,33.6249592505404,22.6920170971282));
#46010=CARTESIAN_POINT('Ctrl Pts',(-6.19331613887171,33.513183109667,22.6862008507854));
#46011=CARTESIAN_POINT('Ctrl Pts',(-6.23996041545217,33.4033386950786,22.6803846044426));
#46012=CARTESIAN_POINT('Ctrl Pts',(-6.28655800085442,33.2936042353552,22.6745741801944));
#46013=CARTESIAN_POINT('Ctrl Pts',(-6.33801149682608,33.1857980288159,22.6687637559463));
#46014=CARTESIAN_POINT('Ctrl Pts',(-6.39413419703502,33.0803758672574,22.6629533316981));
#46015=CARTESIAN_POINT('Ctrl Pts',(-6.45238125753126,32.9709632588284,22.6569229708739));
#46016=CARTESIAN_POINT('Ctrl Pts',(-6.51565784605973,32.8641191697906,22.6508926100497));
#46017=CARTESIAN_POINT('Ctrl Pts',(-6.58370077591595,32.7603293519978,22.6448622492254));
#46018=CARTESIAN_POINT('Ctrl Pts',(-6.64918828143558,32.6604374707993,22.6390583649924));
#46019=CARTESIAN_POINT('Ctrl Pts',(-6.71909033052302,32.5633749574202,22.6332544807593));
#46020=CARTESIAN_POINT('Ctrl Pts',(-6.79312651017594,32.469547981039,22.6274505965263));
#46021=CARTESIAN_POINT('Ctrl Pts',(-6.86715175389342,32.3757348639056,22.621647569589));
#46022=CARTESIAN_POINT('Ctrl Pts',(-6.94530966090001,32.2851566538041,22.6158445426517));
#46023=CARTESIAN_POINT('Ctrl Pts',(-7.02727844659217,32.1981878068107,22.6100415157144));
#46024=CARTESIAN_POINT('Ctrl Pts',(-7.10925446927096,32.1112112813775,22.6042379764306));
#46025=CARTESIAN_POINT('Ctrl Pts',(-7.19504175951734,32.0278450498116,22.5984344371467));
#46026=CARTESIAN_POINT('Ctrl Pts',(-7.28428091920428,31.9484274751856,22.5926308978628));
#46027=CARTESIAN_POINT('Ctrl Pts',(-7.37354901811011,31.8689841463663,22.5868254765588));
#46028=CARTESIAN_POINT('Ctrl Pts',(-7.46627090781391,31.7934922924429,22.5810200552548));
#46029=CARTESIAN_POINT('Ctrl Pts',(-7.56205380769659,31.7222502591819,22.5752146339508));
#46030=CARTESIAN_POINT('Ctrl Pts',(-7.65794277827528,31.6509293319631,22.5694027836801));
#46031=CARTESIAN_POINT('Ctrl Pts',(-7.75689919749645,31.5838678633924,22.5635909334093));
#46032=CARTESIAN_POINT('Ctrl Pts',(-7.85850085185887,31.5213211705432,22.5577790831386));
#46033=CARTESIAN_POINT('Ctrl Pts',(-7.96016923873341,31.4587333966904,22.5519634156134));
#46034=CARTESIAN_POINT('Ctrl Pts',(-8.06448596486822,31.4006665022316,22.5461477480882));
#46035=CARTESIAN_POINT('Ctrl Pts',(-8.17100522620662,31.3473293171384,22.540332080563));
#46036=CARTESIAN_POINT('Ctrl Pts',(-8.27767706488483,31.293915732287,22.534508082722));
#46037=CARTESIAN_POINT('Ctrl Pts',(-8.38655736429865,31.2452455449764,22.5286840848811));
#46038=CARTESIAN_POINT('Ctrl Pts',(-8.49718130078616,31.2014791092725,22.5228600870401));
#46039=CARTESIAN_POINT('Ctrl Pts',(-8.52653043416175,31.1898676353037,22.5213149486655));
#46040=CARTESIAN_POINT('Ctrl Pts',(-8.55600222175017,31.1786010472323,22.519769810291));
#46041=CARTESIAN_POINT('Ctrl Pts',(-8.58558783611666,31.1676817419923,22.5182246719164));
#46042=CARTESIAN_POINT('Ctrl Pts',(-8.69709538742306,31.1265271127798,22.5124010782454));
#46043=CARTESIAN_POINT('Ctrl Pts',(-8.81058043544496,31.0901768992956,22.5065774845743));
#46044=CARTESIAN_POINT('Ctrl Pts',(-8.92559152155267,31.0588235992993,22.5007538909033));
#46045=CARTESIAN_POINT('Ctrl Pts',(-9.04045750409172,31.027509856148,22.4949376445607));
#46046=CARTESIAN_POINT('Ctrl Pts',(-9.15684530480516,31.0011805937347,22.4891213982181));
#46047=CARTESIAN_POINT('Ctrl Pts',(-9.27428469714716,30.9799798135824,22.4833051518755));
#46048=CARTESIAN_POINT('Ctrl Pts',(-9.39160653200931,30.9588002555279,22.4774947276276));
#46049=CARTESIAN_POINT('Ctrl Pts',(-9.50997746485329,30.9427390391209,22.4716843033797));
#46050=CARTESIAN_POINT('Ctrl Pts',(-9.62891393896111,30.931889857034,22.4658738791318));
#46051=CARTESIAN_POINT('Ctrl Pts',(-9.7523524046294,30.920630010964,22.4598435183075));
#46052=CARTESIAN_POINT('Ctrl Pts',(-9.87639963886789,30.9149846857926,22.4538131574832));
#46053=CARTESIAN_POINT('Ctrl Pts',(-10.000505103477,30.9150000312276,22.4477827966588));
#46054=CARTESIAN_POINT('Ctrl Pts',(-10.1199496558401,30.9150148003486,22.441978912426));
#46055=CARTESIAN_POINT('Ctrl Pts',(-10.239447698591,30.9202727227138,22.4361750281932));
#46056=CARTESIAN_POINT('Ctrl Pts',(-10.3585058113543,30.9307619161291,22.4303711439604));
#46057=CARTESIAN_POINT('Ctrl Pts',(-10.4775463379612,30.9412495601784,22.4245681170234));
#46058=CARTESIAN_POINT('Ctrl Pts',(-10.5961466571583,30.9569669027656,22.4187650900864));
#46059=CARTESIAN_POINT('Ctrl Pts',(-10.7138171940892,30.9778500757154,22.4129620631493));
#46060=CARTESIAN_POINT('Ctrl Pts',(-10.8314981200979,30.998735092431,22.4071585238657));
#46061=CARTESIAN_POINT('Ctrl Pts',(-10.9482486985512,31.0247867749672,22.4013549845821));
#46062=CARTESIAN_POINT('Ctrl Pts',(-11.0635889233756,31.0558900114129,22.3955514452984));
#46063=CARTESIAN_POINT('Ctrl Pts',(-11.1789665516898,31.0870033342754,22.3897460239947));
#46064=CARTESIAN_POINT('Ctrl Pts',(-11.2929325227361,31.1231713627163,22.383940602691));
#46065=CARTESIAN_POINT('Ctrl Pts',(-11.4050220006952,31.1642291286415,22.3781351813872));
#46066=CARTESIAN_POINT('Ctrl Pts',(-11.5172356073763,31.2053323622422,22.3723233311168));
#46067=CARTESIAN_POINT('Ctrl Pts',(-11.6275681893683,31.2513360014652,22.3665114808463));
#46068=CARTESIAN_POINT('Ctrl Pts',(-11.7355747647748,31.3020268746411,22.3606996305758));
#46069=CARTESIAN_POINT('Ctrl Pts',(-11.8436522794798,31.3527510418545,22.3548839630509));
#46070=CARTESIAN_POINT('Ctrl Pts',(-11.9494003842287,31.4081683850273,22.3490682955259));
#46071=CARTESIAN_POINT('Ctrl Pts',(-12.052400046113,31.468020519494,22.343252628001));
#46072=CARTESIAN_POINT('Ctrl Pts',(-12.1555472438912,31.5279583856806,22.3374286301603));
#46073=CARTESIAN_POINT('Ctrl Pts',(-12.2559377985707,31.5923435024643,22.3316046323196));
#46074=CARTESIAN_POINT('Ctrl Pts',(-12.3531827952367,31.6608750050048,22.3257806344789));
#46075=CARTESIAN_POINT('Ctrl Pts',(-12.3789824229886,31.679056786232,22.3242354961019));
#46076=CARTESIAN_POINT('Ctrl Pts',(-12.4045608326988,31.6975302057917,22.3226903577249));
#46077=CARTESIAN_POINT('Ctrl Pts',(-12.4299111807625,31.716289194584,22.321145219348));
#46078=CARTESIAN_POINT('Ctrl Pts',(-12.5246533662665,31.7863974073616,22.3153705535969));
#46079=CARTESIAN_POINT('Ctrl Pts',(-12.6165244936635,31.860731942538,22.3095958878458));
#46080=CARTESIAN_POINT('Ctrl Pts',(-12.7051198634262,31.9390276831541,22.3038212220947));
#46081=CARTESIAN_POINT('Ctrl Pts',(-12.7936030129364,32.0172242496507,22.2980538708845));
#46082=CARTESIAN_POINT('Ctrl Pts',(-12.878818345861,32.099371772537,22.2922865196742));
#46083=CARTESIAN_POINT('Ctrl Pts',(-12.9603911014528,32.185162611013,22.286519168464));
#46084=CARTESIAN_POINT('Ctrl Pts',(-13.0418827354367,32.2708681331269,22.280757552708));
#46085=CARTESIAN_POINT('Ctrl Pts',(-13.1197387110857,32.3602094656816,22.2749959369519));
#46086=CARTESIAN_POINT('Ctrl Pts',(-13.1936188085977,32.4528400314524,22.2692343211959));
#46087=CARTESIAN_POINT('Ctrl Pts',(-13.2674469120447,32.5454054072761,22.2634767602507));
#46088=CARTESIAN_POINT('Ctrl Pts',(-13.3373044441081,32.6412550879758,22.2577191993055));
#46089=CARTESIAN_POINT('Ctrl Pts',(-13.402889872101,32.740007628696,22.2519616383604));
#46090=CARTESIAN_POINT('Ctrl Pts',(-13.4684512490792,32.8387239555972,22.2462061887864));
#46091=CARTESIAN_POINT('Ctrl Pts',(-13.5297434061291,32.9403406804837,22.2404507392124));
#46092=CARTESIAN_POINT('Ctrl Pts',(-13.5865071222819,33.0444459450527,22.2346952896385));
#46093=CARTESIAN_POINT('Ctrl Pts',(-13.6432640019236,33.1485386713869,22.2289405332396));
#46094=CARTESIAN_POINT('Ctrl Pts',(-13.6954933261924,33.2551189761469,22.2231857768408));
#46095=CARTESIAN_POINT('Ctrl Pts',(-13.7429813543268,33.3637495359323,22.2174310204419));
#46096=CARTESIAN_POINT('Ctrl Pts',(-13.7904753584471,33.4723937659988,22.2116755398533));
#46097=CARTESIAN_POINT('Ctrl Pts',(-13.8332267144456,33.5830883824799,22.2059200592647));
#46098=CARTESIAN_POINT('Ctrl Pts',(-13.8710697362886,33.6953758791166,22.2001645786761));
#46099=CARTESIAN_POINT('Ctrl Pts',(-13.9089487815488,33.8077702641347,22.1944036193474));
#46100=CARTESIAN_POINT('Ctrl Pts',(-13.9419100289843,33.9217601624649,22.1886426600188));
#46101=CARTESIAN_POINT('Ctrl Pts',(-13.9698376062264,34.0368726043817,22.1828817006901));
#46102=CARTESIAN_POINT('Ctrl Pts',(-13.9977791248236,34.1520425100522,22.1771178655095));
#46103=CARTESIAN_POINT('Ctrl Pts',(-14.0206818886159,34.2683356672832,22.1713540303288));
#46104=CARTESIAN_POINT('Ctrl Pts',(-14.0384814547986,34.3852703527179,22.1655901951481));
#46105=CARTESIAN_POINT('Ctrl Pts',(-14.0563077963079,34.5023809393155,22.1598176896118));
#46106=CARTESIAN_POINT('Ctrl Pts',(-14.0690155630161,34.6201345681094,22.1540451840755));
#46107=CARTESIAN_POINT('Ctrl Pts',(-14.0765923082487,34.7380455147783,22.1482726785391));
#46108=CARTESIAN_POINT('Ctrl Pts',(-14.0822309269687,34.8257949178241,22.1439767761721));
#46109=CARTESIAN_POINT('Ctrl Pts',(-14.085028897281,34.9136313781386,22.1396808738051));
#46110=CARTESIAN_POINT('Ctrl Pts',(-14.084999774902,35.0013561158978,22.1353849714381));
#46111=CARTESIAN_POINT('Ctrl Pts',(-14.0849997749018,35.0013561165845,22.1353849714045));
#46112=CARTESIAN_POINT('Ctrl Pts',(-14.0849741968583,35.0784042873399,22.1316119031962));
#46113=CARTESIAN_POINT('Ctrl Pts',(-14.0827689216963,35.1554131039001,22.1278388349879));
#46114=CARTESIAN_POINT('Ctrl Pts',(-14.0783897720535,35.2322969375804,22.1240657667795));
#46115=CARTESIAN_POINT('Ctrl Pts',(-14.0716307137146,35.3509643409699,22.1182421731102));
#46116=CARTESIAN_POINT('Ctrl Pts',(-14.0596772245188,35.4695278607971,22.1124185794409));
#46117=CARTESIAN_POINT('Ctrl Pts',(-14.0425329433293,35.5874967251799,22.1065949857716));
#46118=CARTESIAN_POINT('Ctrl Pts',(-14.0254102921972,35.7053167543175,22.1007787394307));
#46119=CARTESIAN_POINT('Ctrl Pts',(-14.0031099329979,35.8225432197027,22.0949624930898));
#46120=CARTESIAN_POINT('Ctrl Pts',(-13.9756874615848,35.9386874920855,22.0891462467489));
#46121=CARTESIAN_POINT('Ctrl Pts',(-13.9482924402167,36.054715503411,22.0833358225027));
#46122=CARTESIAN_POINT('Ctrl Pts',(-13.9157855999806,36.1696630816619,22.0775253982564));
#46123=CARTESIAN_POINT('Ctrl Pts',(-13.8782739859291,36.2830494495792,22.0717149740102));
#46124=CARTESIAN_POINT('Ctrl Pts',(-13.8393424796791,36.400727726104,22.0656846131852));
#46125=CARTESIAN_POINT('Ctrl Pts',(-13.7950198958781,36.5167238234022,22.0596542523603));
#46126=CARTESIAN_POINT('Ctrl Pts',(-13.7454836013012,36.6305145176857,22.0536238915353));
#46127=CARTESIAN_POINT('Ctrl Pts',(-13.6978076947825,36.7400316818114,22.0478200073042));
#46128=CARTESIAN_POINT('Ctrl Pts',(-13.6453028057693,36.8475057000283,22.042016123073));
#46129=CARTESIAN_POINT('Ctrl Pts',(-13.5881767206809,36.9524888786274,22.0362122388418));
#46130=CARTESIAN_POINT('Ctrl Pts',(-13.5310590737261,37.0574565500886,22.0304092119064));
#46131=CARTESIAN_POINT('Ctrl Pts',(-13.4693217832903,37.1599337550384,22.024606184971));
#46132=CARTESIAN_POINT('Ctrl Pts',(-13.4032187691411,37.259497070006,22.0188031580356));
#46133=CARTESIAN_POINT('Ctrl Pts',(-13.3371099187868,37.3590691753735,22.0129996187536));
#46134=CARTESIAN_POINT('Ctrl Pts',(-13.2666348042263,37.4557265390491,22.0071960794716));
#46135=CARTESIAN_POINT('Ctrl Pts',(-13.1920905142096,37.5490749594888,22.0013925401896));
#46136=CARTESIAN_POINT('Ctrl Pts',(-13.1175220503485,37.6424536517333,21.9955871188874));
#46137=CARTESIAN_POINT('Ctrl Pts',(-13.0388820413468,37.7325209477668,21.9897816975852));
#46138=CARTESIAN_POINT('Ctrl Pts',(-12.9565072374651,37.8189164504852,21.9839762762831));
#46139=CARTESIAN_POINT('Ctrl Pts',(-12.8740412111122,37.9054076282268,21.9781644260141));
#46140=CARTESIAN_POINT('Ctrl Pts',(-12.7878324161358,37.9882186005192,21.9723525757452));
#46141=CARTESIAN_POINT('Ctrl Pts',(-12.6982538800312,38.0670264098792,21.9665407254763));
#46142=CARTESIAN_POINT('Ctrl Pts',(-12.6086165082629,38.1458859806317,21.9607250579528));
#46143=CARTESIAN_POINT('Ctrl Pts',(-12.5156053049828,38.2207368967183,21.9549093904294));
#46144=CARTESIAN_POINT('Ctrl Pts',(-12.4196244006156,38.2912980357217,21.949093722906));
#46145=CARTESIAN_POINT('Ctrl Pts',(-12.3235060139662,38.361960245938,21.9432697250668));
#46146=CARTESIAN_POINT('Ctrl Pts',(-12.2244097740082,38.4283201883,21.9374457272276));
#46147=CARTESIAN_POINT('Ctrl Pts',(-12.1227667446997,38.4901413076833,21.9316217293883));
#46148=CARTESIAN_POINT('Ctrl Pts',(-12.0958002946353,38.5065427878449,21.9300765909959));
#46149=CARTESIAN_POINT('Ctrl Pts',(-12.0686547041497,38.5226250516946,21.9285314526035));
#46150=CARTESIAN_POINT('Ctrl Pts',(-12.0413382690484,38.5383842458555,21.9269863142111));
#46151=CARTESIAN_POINT('Ctrl Pts',(-11.9383832073534,38.5977803127684,21.9211627205419));
#46152=CARTESIAN_POINT('Ctrl Pts',(-11.8326676330745,38.6527749624113,21.9153391268728));
#46153=CARTESIAN_POINT('Ctrl Pts',(-11.7246040083451,38.7031022149544,21.9095155332037));
#46154=CARTESIAN_POINT('Ctrl Pts',(-11.6166767219304,38.7533659721925,21.903699286863));
#46155=CARTESIAN_POINT('Ctrl Pts',(-11.5064076441376,38.7989738737752,21.8978830405223));
#46156=CARTESIAN_POINT('Ctrl Pts',(-11.3942359259936,38.8397045697122,21.8920667941817));
#46157=CARTESIAN_POINT('Ctrl Pts',(-11.2821764923588,38.8803944939977,21.8862563699357));
#46158=CARTESIAN_POINT('Ctrl Pts',(-11.1682185888573,38.9162167864233,21.8804459456898));
#46159=CARTESIAN_POINT('Ctrl Pts',(-11.052823001915,38.9469974318004,21.8746355214438));
#46160=CARTESIAN_POINT('Ctrl Pts',(-10.9330594532611,38.978943188288,21.8686051606187));
#46161=CARTESIAN_POINT('Ctrl Pts',(-10.8117476384202,39.0054578936876,21.8625747997937));
#46162=CARTESIAN_POINT('Ctrl Pts',(-10.689422392677,39.0264030802287,21.8565444389686));
#46163=CARTESIAN_POINT('Ctrl Pts',(-10.5716912012283,39.046561648083,21.8507405547378));
#46164=CARTESIAN_POINT('Ctrl Pts',(-10.4530217657467,39.0615614161482,21.844936670507));
#46165=CARTESIAN_POINT('Ctrl Pts',(-10.3339024252795,39.0713307616052,21.8391327862762));
#46166=CARTESIAN_POINT('Ctrl Pts',(-10.2148006800129,39.0810986640253,21.8333297593412));
#46167=CARTESIAN_POINT('Ctrl Pts',(-10.0952495687809,39.0856376469056,21.8275267324061));
#46168=CARTESIAN_POINT('Ctrl Pts',(-9.97574242032439,39.0849279760882,21.8217237054711));
#46169=CARTESIAN_POINT('Ctrl Pts',(-9.85622472063662,39.0842182426144,21.8159201661895));
#46170=CARTESIAN_POINT('Ctrl Pts',(-9.73675139979158,39.0782589365143,21.8101166269079));
#46171=CARTESIAN_POINT('Ctrl Pts',(-9.6178150098177,39.0670824473177,21.8043130876263));
#46172=CARTESIAN_POINT('Ctrl Pts',(-9.49884005015977,39.0559023337159,21.7985076663245));
#46173=CARTESIAN_POINT('Ctrl Pts',(-9.38040277399597,39.0395017104503,21.7927022450228));
#46174=CARTESIAN_POINT('Ctrl Pts',(-9.26298920129247,39.0179646691563,21.7868968237211));
#46175=CARTESIAN_POINT('Ctrl Pts',(-9.14544560392483,38.9964037775826,21.7810849734526));
#46176=CARTESIAN_POINT('Ctrl Pts',(-9.02892837476783,38.969695187746,21.7752731231842));
#46177=CARTESIAN_POINT('Ctrl Pts',(-8.913912106228,38.9379738555508,21.7694612729157));
#46178=CARTESIAN_POINT('Ctrl Pts',(-8.79882029438557,38.9062316886144,21.7636456053928));
#46179=CARTESIAN_POINT('Ctrl Pts',(-8.68523179408831,38.8694703478723,21.7578299378699));
#46180=CARTESIAN_POINT('Ctrl Pts',(-8.57360325759354,38.8278737352808,21.7520142703469));
#46181=CARTESIAN_POINT('Ctrl Pts',(-8.46181482527368,38.7862175400332,21.7461902725083));
#46182=CARTESIAN_POINT('Ctrl Pts',(-8.35199233492593,38.7397124076678,21.7403662746696));
#46183=CARTESIAN_POINT('Ctrl Pts',(-8.24456992799178,38.6885891967376,21.7345422768309));
#46184=CARTESIAN_POINT('Ctrl Pts',(-8.21607017745062,38.6750259300044,21.7329971384348));
#46185=CARTESIAN_POINT('Ctrl Pts',(-8.1877392119687,38.6611378526349,21.7314520000387));
#46186=CARTESIAN_POINT('Ctrl Pts',(-8.15958480185777,38.6469297907208,21.7299068616426));
#46187=CARTESIAN_POINT('Ctrl Pts',(-8.0534531648498,38.5933706906114,21.7240822655408));
#46188=CARTESIAN_POINT('Ctrl Pts',(-7.9494902807754,38.535088453809,21.718257669439));
#46189=CARTESIAN_POINT('Ctrl Pts',(-7.84814493426046,38.4722823583417,21.7124330733371));
#46190=CARTESIAN_POINT('Ctrl Pts',(-7.74693946608145,38.40956294877,21.7066165164284));
#46191=CARTESIAN_POINT('Ctrl Pts',(-7.64834469092929,38.3423323182262,21.7007999595197));
#46192=CARTESIAN_POINT('Ctrl Pts',(-7.55278652960942,38.2708364725768,21.694983402611));
#46193=CARTESIAN_POINT('Ctrl Pts',(-7.53940692985026,38.2608259639398,21.6941689959466));
#46194=CARTESIAN_POINT('Ctrl Pts',(-7.52608682171778,38.2507319127429,21.6933545892822));
#46195=CARTESIAN_POINT('Ctrl Pts',(-7.51282733495086,38.2405550657615,21.6925401826178));
#46196=CARTESIAN_POINT('',(-14.0849992774348,34.997570317556,22.2396150286382));
#46197=CARTESIAN_POINT('Ctrl Pts',(-14.0849992774354,34.9975703184362,22.2396150285955));
#46198=CARTESIAN_POINT('Ctrl Pts',(-14.085070989627,35.1181393078928,22.233766442302));
#46199=CARTESIAN_POINT('Ctrl Pts',(-14.0798004648248,35.2387276668954,22.2279178560085));
#46200=CARTESIAN_POINT('Ctrl Pts',(-14.0692091476505,35.3588341018879,22.2220692697149));
#46201=CARTESIAN_POINT('Ctrl Pts',(-14.0586166826973,35.4789535527894,22.2162200496113));
#46202=CARTESIAN_POINT('Ctrl Pts',(-14.0427023124911,35.5985905779619,22.2103708295077));
#46203=CARTESIAN_POINT('Ctrl Pts',(-14.0215393834305,35.7172489020677,22.2045216094042));
#46204=CARTESIAN_POINT('Ctrl Pts',(-14.0003694708714,35.8359463819171,22.198670459132));
#46205=CARTESIAN_POINT('Ctrl Pts',(-13.9739476224999,35.9536641249992,22.1928193088599));
#46206=CARTESIAN_POINT('Ctrl Pts',(-13.9423982256983,36.0699164593606,22.1869681585878));
#46207=CARTESIAN_POINT('Ctrl Pts',(-13.9108091820569,36.186314883288,22.1811096554138));
#46208=CARTESIAN_POINT('Ctrl Pts',(-13.8740798226734,36.3012438337504,22.1752511522399));
#46209=CARTESIAN_POINT('Ctrl Pts',(-13.8323844851566,36.4142327099637,22.1693926490659));
#46210=CARTESIAN_POINT('Ctrl Pts',(-13.7906628672968,36.527292802447,22.1635304533095));
#46211=CARTESIAN_POINT('Ctrl Pts',(-13.7439691883516,36.6384100158729,22.157668257553));
#46212=CARTESIAN_POINT('Ctrl Pts',(-13.6925253126223,36.7471353169242,22.1518060617966));
#46213=CARTESIAN_POINT('Ctrl Pts',(-13.6409886366947,36.8560567487948,22.1459332911579));
#46214=CARTESIAN_POINT('Ctrl Pts',(-13.5846848248008,36.9625772912325,22.1400605205192));
#46215=CARTESIAN_POINT('Ctrl Pts',(-13.5238813533298,37.0662732654841,22.1341877498805));
#46216=CARTESIAN_POINT('Ctrl Pts',(-13.4639491572563,37.1684833418256,22.1283991323411));
#46217=CARTESIAN_POINT('Ctrl Pts',(-13.3996456789963,37.2679490084678,22.1226105148017));
#46218=CARTESIAN_POINT('Ctrl Pts',(-13.3312658119027,37.364295474438,22.1168218972623));
#46219=CARTESIAN_POINT('Ctrl Pts',(-13.2624727782426,37.4612240874675,22.1109983035913));
#46220=CARTESIAN_POINT('Ctrl Pts',(-13.1893348551766,37.5553040447086,22.1051747099203));
#46221=CARTESIAN_POINT('Ctrl Pts',(-13.1121159531809,37.6461215569125,22.0993511162492));
#46222=CARTESIAN_POINT('Ctrl Pts',(-13.0349944743,37.736824489335,22.0935348699066));
#46223=CARTESIAN_POINT('Ctrl Pts',(-12.9538025194293,37.8242728551197,22.087718623564));
#46224=CARTESIAN_POINT('Ctrl Pts',(-12.8688468720517,37.9080822933197,22.0819023772214));
#46225=CARTESIAN_POINT('Ctrl Pts',(-12.7839762657457,37.9918078378097,22.0760919529735));
#46226=CARTESIAN_POINT('Ctrl Pts',(-12.6953497508831,38.0719014160679,22.0702815287256));
#46227=CARTESIAN_POINT('Ctrl Pts',(-12.6033135194903,38.1480126618613,22.0644711044777));
#46228=CARTESIAN_POINT('Ctrl Pts',(-12.5077935263661,38.227004875741,22.0584407436534));
#46229=CARTESIAN_POINT('Ctrl Pts',(-12.4086008771728,38.3017069798914,22.052410382829));
#46230=CARTESIAN_POINT('Ctrl Pts',(-12.3061638909231,38.3717700259956,22.0463800220047));
#46231=CARTESIAN_POINT('Ctrl Pts',(-12.2075740342511,38.439201780153,22.0405761377719));
#46232=CARTESIAN_POINT('Ctrl Pts',(-12.1059795022868,38.50233639066,22.0347722535391));
#46233=CARTESIAN_POINT('Ctrl Pts',(-12.0017942403325,38.5609050562142,22.0289683693063));
#46234=CARTESIAN_POINT('Ctrl Pts',(-11.8976243676556,38.6194650705501,22.0231653423693));
#46235=CARTESIAN_POINT('Ctrl Pts',(-11.7908648818676,38.6734602811338,22.0173623154322));
#46236=CARTESIAN_POINT('Ctrl Pts',(-11.6819559081379,38.7226669637613,22.0115592884952));
#46237=CARTESIAN_POINT('Ctrl Pts',(-11.5730373188848,38.7718779908243,22.0057557492116));
#46238=CARTESIAN_POINT('Ctrl Pts',(-11.4619692365034,38.8162994812118,21.9999522099279));
#46239=CARTESIAN_POINT('Ctrl Pts',(-11.3492128233253,38.8557554068398,21.9941486706443));
#46240=CARTESIAN_POINT('Ctrl Pts',(-11.2364198445577,38.8952241275643,21.9883432493406));
#46241=CARTESIAN_POINT('Ctrl Pts',(-11.121937831351,38.9297239462582,21.9825378280369));
#46242=CARTESIAN_POINT('Ctrl Pts',(-11.0062435766446,38.9591285486154,21.9767324067331));
#46243=CARTESIAN_POINT('Ctrl Pts',(-10.8904212012593,38.9885657138481,21.9709205564627));
#46244=CARTESIAN_POINT('Ctrl Pts',(-10.773384300728,39.012896299226,21.9651087061922));
#46245=CARTESIAN_POINT('Ctrl Pts',(-10.6556204998727,39.0320449848863,21.9592968559217));
#46246=CARTESIAN_POINT('Ctrl Pts',(-10.5377793511207,39.0512062475061,21.9534811883967));
#46247=CARTESIAN_POINT('Ctrl Pts',(-10.4192107558254,39.0651787845738,21.9476655208718));
#46248=CARTESIAN_POINT('Ctrl Pts',(-10.3004064516139,39.0739392440031,21.9418498533468));
#46249=CARTESIAN_POINT('Ctrl Pts',(-10.1814319730652,39.0827122518446,21.9360258555061));
#46250=CARTESIAN_POINT('Ctrl Pts',(-10.0622215184218,39.086258268742,21.9302018576654));
#46251=CARTESIAN_POINT('Ctrl Pts',(-9.94326595422021,39.0846060089132,21.9243778598247));
#46252=CARTESIAN_POINT('Ctrl Pts',(-9.91170639454557,39.0841676553732,21.9228327214478));
#46253=CARTESIAN_POINT('Ctrl Pts',(-9.88016474084429,39.083363693142,21.9212875830708));
#46254=CARTESIAN_POINT('Ctrl Pts',(-9.8486500682641,39.0821952670302,21.9197424446939));
#46255=CARTESIAN_POINT('Ctrl Pts',(-9.72988906658912,39.077792128934,21.9139196908352));
#46256=CARTESIAN_POINT('Ctrl Pts',(-9.61112888814208,39.0681950209669,21.9080969369765));
#46257=CARTESIAN_POINT('Ctrl Pts',(-9.49286006791139,39.0533978449298,21.9022741831178));
#46258=CARTESIAN_POINT('Ctrl Pts',(-9.37473174465413,39.0386182471389,21.8964583463763));
#46259=CARTESIAN_POINT('Ctrl Pts',(-9.25709402035442,39.0186509142913,21.8906425096348));
#46260=CARTESIAN_POINT('Ctrl Pts',(-9.14043642794768,38.9935417195267,21.8848266728934));
#46261=CARTESIAN_POINT('Ctrl Pts',(-9.02388987407472,38.9684564245197,21.8790163718566));
#46262=CARTESIAN_POINT('Ctrl Pts',(-8.90832199345271,38.9382390867825,21.8732060708199));
#46263=CARTESIAN_POINT('Ctrl Pts',(-8.7942155633382,38.9029871755239,21.8673957697831));
#46264=CARTESIAN_POINT('Ctrl Pts',(-8.6789300613533,38.8673710031373,21.86152543039));
#46265=CARTESIAN_POINT('Ctrl Pts',(-8.56513680480514,38.8266156664125,21.8556550909969));
#46266=CARTESIAN_POINT('Ctrl Pts',(-8.4533218289518,38.7808744537743,21.8497847516038));
#46267=CARTESIAN_POINT('Ctrl Pts',(-8.34277846018579,38.7356534295073,21.8439811721874));
#46268=CARTESIAN_POINT('Ctrl Pts',(-8.23416899235596,38.6855595136954,21.838177592771));
#46269=CARTESIAN_POINT('Ctrl Pts',(-8.12794564672773,38.6307902030267,21.8323740133545));
#46270=CARTESIAN_POINT('Ctrl Pts',(-8.01988943187385,38.5750758554318,21.8264702939731));
#46271=CARTESIAN_POINT('Ctrl Pts',(-7.91430285340421,38.5145234231377,21.8205665745917));
#46272=CARTESIAN_POINT('Ctrl Pts',(-7.81163749354091,38.4493904592441,21.8146628552103));
#46273=CARTESIAN_POINT('Ctrl Pts',(-7.7089721336776,38.3842574953504,21.8087591358289));
#46274=CARTESIAN_POINT('Ctrl Pts',(-7.60922836451667,38.3145442437736,21.8028554164475));
#46275=CARTESIAN_POINT('Ctrl Pts',(-7.51282733495087,38.2405550657615,21.796951697066));
#46276=CARTESIAN_POINT('Ctrl Pts',(-7.51282733495086,38.2405550657615,23.0467784846721));
#46277=CARTESIAN_POINT('Ctrl Pts',(-7.41657395968785,38.1666792145524,23.0408768689581));
#46278=CARTESIAN_POINT('Ctrl Pts',(-7.3235466771998,38.0884588542002,23.0349752532441));
#46279=CARTESIAN_POINT('Ctrl Pts',(-7.23415348605168,38.0062132428156,23.0290736375301));
#46280=CARTESIAN_POINT('Ctrl Pts',(-7.14624403414103,37.9253327358551,23.0232699762429));
#46281=CARTESIAN_POINT('Ctrl Pts',(-7.06184926695299,37.8405598681496,23.0174663149557));
#46282=CARTESIAN_POINT('Ctrl Pts',(-6.98132337274585,37.7522384380844,23.0116626536685));
#46283=CARTESIAN_POINT('Ctrl Pts',(-6.9008064225061,37.6639268178326,23.0058596369908));
#46284=CARTESIAN_POINT('Ctrl Pts',(-6.82415776570052,37.5720677207802,23.0000566203132));
#46285=CARTESIAN_POINT('Ctrl Pts',(-6.75169343838683,37.4770404683373,22.9942536036355));
#46286=CARTESIAN_POINT('Ctrl Pts',(-6.67922005806772,37.3820013440913,22.988449861984));
#46287=CARTESIAN_POINT('Ctrl Pts',(-6.61093229428784,37.2837936021546,22.9826461203324));
#46288=CARTESIAN_POINT('Ctrl Pts',(-6.54710433902782,37.1828276511075,22.9768423786809));
#46289=CARTESIAN_POINT('Ctrl Pts',(-6.48139048348633,37.0788784975636,22.9708671560855));
#46290=CARTESIAN_POINT('Ctrl Pts',(-6.42040433136491,36.9720059953963,22.9648919334901));
#46291=CARTESIAN_POINT('Ctrl Pts',(-6.36439496966692,36.8626865177525,22.9589167108947));
#46292=CARTESIAN_POINT('Ctrl Pts',(-6.30991126876428,36.7563448358941,22.9531042497124));
#46293=CARTESIAN_POINT('Ctrl Pts',(-6.26013684913735,36.6476881651299,22.9472917885301));
#46294=CARTESIAN_POINT('Ctrl Pts',(-6.21525214167994,36.5371755426566,22.9414793273478));
#46295=CARTESIAN_POINT('Ctrl Pts',(-6.16848213171892,36.4220210335447,22.9354227240459));
#46296=CARTESIAN_POINT('Ctrl Pts',(-6.12702172979419,36.3048517336437,22.9293661207439));
#46297=CARTESIAN_POINT('Ctrl Pts',(-6.09101723354879,36.1862034950157,22.923309517442));
#46298=CARTESIAN_POINT('Ctrl Pts',(-6.05501273730338,36.0675552563876,22.91725291414));
#46299=CARTESIAN_POINT('Ctrl Pts',(-6.02446420208395,35.9474285749655,22.911196310838));
#46300=CARTESIAN_POINT('Ctrl Pts',(-5.99945759808047,35.8263688585879,22.9051397075361));
#46301=CARTESIAN_POINT('Ctrl Pts',(-5.97541304809779,35.7099665513844,22.8993161138646));
#46302=CARTESIAN_POINT('Ctrl Pts',(-5.95641431380094,35.592326242637,22.8934925201932));
#46303=CARTESIAN_POINT('Ctrl Pts',(-5.94258432963635,35.4739230716978,22.8876689265217));
#46304=CARTESIAN_POINT('Ctrl Pts',(-5.92877179405107,35.3556692839461,22.8818526801787));
#46305=CARTESIAN_POINT('Ctrl Pts',(-5.92011508514747,35.2366549503255,22.8760364338357));
#46306=CARTESIAN_POINT('Ctrl Pts',(-5.91668638256212,35.1173665269419,22.8702201874927));
#46307=CARTESIAN_POINT('Ctrl Pts',(-5.91326111212698,34.9981975119284,22.8644097632444));
#46308=CARTESIAN_POINT('Ctrl Pts',(-5.91505344874562,34.8787553587903,22.8585993389961));
#46309=CARTESIAN_POINT('Ctrl Pts',(-5.92208383683801,34.7595321929608,22.8527889147477));
#46310=CARTESIAN_POINT('Ctrl Pts',(-5.92938033966108,34.6357961837083,22.8467585539236));
#46311=CARTESIAN_POINT('Ctrl Pts',(-5.94231932317017,34.512296512764,22.8407281930994));
#46312=CARTESIAN_POINT('Ctrl Pts',(-5.96086422097439,34.3895844377842,22.8346978322752));
#46313=CARTESIAN_POINT('Ctrl Pts',(-5.97871264549011,34.2714809448146,22.828893948042));
#46314=CARTESIAN_POINT('Ctrl Pts',(-6.00175343918375,34.1541073967008,22.8230900638088));
#46315=CARTESIAN_POINT('Ctrl Pts',(-6.02990118229129,34.0379499089819,22.8172861795755));
#46316=CARTESIAN_POINT('Ctrl Pts',(-6.05804476767612,33.9218095789663,22.8114831526381));
#46317=CARTESIAN_POINT('Ctrl Pts',(-6.09129370616824,33.8068853488722,22.8056801257006));
#46318=CARTESIAN_POINT('Ctrl Pts',(-6.12951174889358,33.6936517699912,22.7998770987632));
#46319=CARTESIAN_POINT('Ctrl Pts',(-6.16773316587247,33.5804081937692,22.7940735594791));
#46320=CARTESIAN_POINT('Ctrl Pts',(-6.21092442877671,33.4688559524523,22.7882700201951));
#46321=CARTESIAN_POINT('Ctrl Pts',(-6.25890004806708,33.3594524847943,22.782466480911));
#46322=CARTESIAN_POINT('Ctrl Pts',(-6.30689122529137,33.2500135388675,22.7766610596068));
#46323=CARTESIAN_POINT('Ctrl Pts',(-6.35966968060203,33.14272512619,22.7708556383027));
#46324=CARTESIAN_POINT('Ctrl Pts',(-6.41700289212914,33.0380222414642,22.7650502169985));
#46325=CARTESIAN_POINT('Ctrl Pts',(-6.47439959488128,32.9332034079848,22.7592383667276));
#46326=CARTESIAN_POINT('Ctrl Pts',(-6.53636092581199,32.8309761760842,22.7534265164567));
#46327=CARTESIAN_POINT('Ctrl Pts',(-6.60260966410514,32.731748711988,22.7476146661858));
#46328=CARTESIAN_POINT('Ctrl Pts',(-6.66890191492497,32.6324560747611,22.7417989986604));
#46329=CARTESIAN_POINT('Ctrl Pts',(-6.73948694036518,32.5361674577396,22.7359833311351));
#46330=CARTESIAN_POINT('Ctrl Pts',(-6.81404668775278,32.4432586184401,22.7301676636097));
#46331=CARTESIAN_POINT('Ctrl Pts',(-6.88871323392784,32.3502166972602,22.7243436657686));
#46332=CARTESIAN_POINT('Ctrl Pts',(-6.96736559735073,32.2605645223719,22.7185196679275));
#46333=CARTESIAN_POINT('Ctrl Pts',(-7.0496482181394,32.1746417283339,22.7126956700863));
#46334=CARTESIAN_POINT('Ctrl Pts',(-7.07147824594366,32.1518459427246,22.7111505317134));
#46335=CARTESIAN_POINT('Ctrl Pts',(-7.09356361386295,32.1293124389546,22.7096053933405));
#46336=CARTESIAN_POINT('Ctrl Pts',(-7.11589729903296,32.1070470777639,22.7080602549676));
#46337=CARTESIAN_POINT('Ctrl Pts',(-7.20007248353149,32.0231294048904,22.7022366612962));
#46338=CARTESIAN_POINT('Ctrl Pts',(-7.28804902917342,31.9427532793078,22.6964130676248));
#46339=CARTESIAN_POINT('Ctrl Pts',(-7.37949693130055,31.8662819739267,22.6905894739534));
#46340=CARTESIAN_POINT('Ctrl Pts',(-7.47082945831563,31.7899071484562,22.6847732276105));
#46341=CARTESIAN_POINT('Ctrl Pts',(-7.56562432034542,31.7174276041097,22.6789569812675));
#46342=CARTESIAN_POINT('Ctrl Pts',(-7.66351422578696,31.6491703673717,22.6731407349246));
#46343=CARTESIAN_POINT('Ctrl Pts',(-7.7613061428933,31.580981456504,22.6673303106763));
#46344=CARTESIAN_POINT('Ctrl Pts',(-7.86218660699066,31.5170066772535,22.661519886428));
#46345=CARTESIAN_POINT('Ctrl Pts',(-7.96575522545295,31.4575328939808,22.6557094621797));
#46346=CARTESIAN_POINT('Ctrl Pts',(-8.07324413034226,31.3958079049975,22.6496791013556));
#46347=CARTESIAN_POINT('Ctrl Pts',(-8.18362837108477,31.3389316761016,22.6436487405314));
#46348=CARTESIAN_POINT('Ctrl Pts',(-8.29642684731927,31.2871758035876,22.6376183797072));
#46349=CARTESIAN_POINT('Ctrl Pts',(-8.40498905724828,31.2373636777106,22.631814495474));
#46350=CARTESIAN_POINT('Ctrl Pts',(-8.51578703002254,31.192294428774,22.6260106112408));
#46351=CARTESIAN_POINT('Ctrl Pts',(-8.62836736862838,31.1521630849844,22.6202067270077));
#46352=CARTESIAN_POINT('Ctrl Pts',(-8.74093107791437,31.1120376690235,22.6144037000702));
#46353=CARTESIAN_POINT('Ctrl Pts',(-8.8552762449359,31.0768488447719,22.6086006731328));
#46354=CARTESIAN_POINT('Ctrl Pts',(-8.97093128201541,31.0467427893362,22.6027976461954));
#46355=CARTESIAN_POINT('Ctrl Pts',(-9.08659653022548,31.0166340758505,22.5969941069114));
#46356=CARTESIAN_POINT('Ctrl Pts',(-9.20357148324194,30.9916091262857,22.5911905676274));
#46357=CARTESIAN_POINT('Ctrl Pts',(-9.32137187388096,30.9717635538067,22.5853870283434));
#46358=CARTESIAN_POINT('Ctrl Pts',(-9.43921046581253,30.95191154564,22.5795816070393));
#46359=CARTESIAN_POINT('Ctrl Pts',(-9.55787462526565,30.9372423227284,22.5737761857352));
#46360=CARTESIAN_POINT('Ctrl Pts',(-9.67687307520295,30.9277998587408,22.5679707644311));
#46361=CARTESIAN_POINT('Ctrl Pts',(-9.79600330490938,30.9183469380984,22.5621589141602));
#46362=CARTESIAN_POINT('Ctrl Pts',(-9.91546815674363,30.9141323623456,22.5563470638893));
#46363=CARTESIAN_POINT('Ctrl Pts',(-10.0347742898978,30.915148013849,22.5505352136185));
#46364=CARTESIAN_POINT('Ctrl Pts',(-10.1541587839607,30.9161643324377,22.5447195460931));
#46365=CARTESIAN_POINT('Ctrl Pts',(-10.2733839448934,30.9224176983138,22.5389038785678));
#46366=CARTESIAN_POINT('Ctrl Pts',(-10.3919611550605,30.9338480779829,22.5330882110425));
#46367=CARTESIAN_POINT('Ctrl Pts',(-10.5107082142768,30.9452948304366,22.5272642132014));
#46368=CARTESIAN_POINT('Ctrl Pts',(-10.6288050673429,30.9619333408792,22.5214402153604));
#46369=CARTESIAN_POINT('Ctrl Pts',(-10.7457727487375,30.9836524045794,22.5156162175193));
#46370=CARTESIAN_POINT('Ctrl Pts',(-10.7768049121928,30.989414590568,22.5140710791459));
#46371=CARTESIAN_POINT('Ctrl Pts',(-10.8077576788365,30.9955341090123,22.5125259407726));
#46372=CARTESIAN_POINT('Ctrl Pts',(-10.8386222972362,31.0020082988357,22.5109808023992));
#46373=CARTESIAN_POINT('Ctrl Pts',(-10.9549503876449,31.0264093826057,22.5051572087275));
#46374=CARTESIAN_POINT('Ctrl Pts',(-11.0704001978096,31.0559311623806,22.4993336150558));
#46375=CARTESIAN_POINT('Ctrl Pts',(-11.1844870002163,31.0904967647643,22.4935100213841));
#46376=CARTESIAN_POINT('Ctrl Pts',(-11.2984298651754,31.1250187575062,22.4876937750409));
#46377=CARTESIAN_POINT('Ctrl Pts',(-11.411012755344,31.1645717985846,22.4818775286976));
#46378=CARTESIAN_POINT('Ctrl Pts',(-11.5217608193279,31.2090279599081,22.4760612823544));
#46379=CARTESIAN_POINT('Ctrl Pts',(-11.6323980238884,31.2534396203687,22.4702508581059));
#46380=CARTESIAN_POINT('Ctrl Pts',(-11.7412036793263,31.3027444858749,22.4644404338573));
#46381=CARTESIAN_POINT('Ctrl Pts',(-11.8477183799133,31.3567649281812,22.4586300096088));
#46382=CARTESIAN_POINT('Ctrl Pts',(-11.9582648822224,31.4128301559596,22.4525996487847));
#46383=CARTESIAN_POINT('Ctrl Pts',(-12.0663431391599,31.4739748727744,22.4465692879606));
#46384=CARTESIAN_POINT('Ctrl Pts',(-12.1714622737273,31.5399455793616,22.4405389271365));
#46385=CARTESIAN_POINT('Ctrl Pts',(-12.2726335478101,31.6034386861594,22.434735042903));
#46386=CARTESIAN_POINT('Ctrl Pts',(-12.3710635802309,31.6714015928774,22.4289311586696));
#46387=CARTESIAN_POINT('Ctrl Pts',(-12.4663407192963,31.7435619986953,22.4231272744361));
#46388=CARTESIAN_POINT('Ctrl Pts',(-12.5616037849094,31.8157117456497,22.4173242474984));
#46389=CARTESIAN_POINT('Ctrl Pts',(-12.6537145579033,31.8920575122198,22.4115212205607));
#46390=CARTESIAN_POINT('Ctrl Pts',(-12.7422922727758,31.9722850050452,22.405718193623));
#46391=CARTESIAN_POINT('Ctrl Pts',(-12.830877808134,32.052519581119,22.3999146543387));
#46392=CARTESIAN_POINT('Ctrl Pts',(-12.9159293625088,32.1366362907165,22.3941111150544));
#46393=CARTESIAN_POINT('Ctrl Pts',(-12.9971015101764,32.2242825183931,22.3883075757702));
#46394=CARTESIAN_POINT('Ctrl Pts',(-13.0782999810246,32.3119571687189,22.3825021544658));
#46395=CARTESIAN_POINT('Ctrl Pts',(-13.1556162658772,32.4031633140018,22.3766967331614));
#46396=CARTESIAN_POINT('Ctrl Pts',(-13.228744286248,32.4975141690669,22.370891311857));
#46397=CARTESIAN_POINT('Ctrl Pts',(-13.3019532891329,32.5919695089712,22.3650794615859));
#46398=CARTESIAN_POINT('Ctrl Pts',(-13.3709645191639,32.6895761870393,22.3592676113147));
#46399=CARTESIAN_POINT('Ctrl Pts',(-13.4355143342332,32.7899171374634,22.3534557610436));
#46400=CARTESIAN_POINT('Ctrl Pts',(-13.5001065459675,32.8903239923622,22.347640093518));
#46401=CARTESIAN_POINT('Ctrl Pts',(-13.5602313018439,32.9934683442013,22.3418244259924));
#46402=CARTESIAN_POINT('Ctrl Pts',(-13.615670969754,33.0989086191143,22.3360087584668));
#46403=CARTESIAN_POINT('Ctrl Pts',(-13.6711900490022,33.2044999258359,22.3301847606255));
#46404=CARTESIAN_POINT('Ctrl Pts',(-13.7220104723443,33.3123933515242,22.3243607627841));
#46405=CARTESIAN_POINT('Ctrl Pts',(-13.7679626967556,33.4221273448537,22.3185367649427));
#46406=CARTESIAN_POINT('Ctrl Pts',(-13.7801540723517,33.4512403713825,22.3169916265721));
#46407=CARTESIAN_POINT('Ctrl Pts',(-13.7920030629533,33.4804828693455,22.3154464882014));
#46408=CARTESIAN_POINT('Ctrl Pts',(-13.8035070969918,33.5098460605921,22.3139013498308));
#46409=CARTESIAN_POINT('Ctrl Pts',(-13.8524065999432,33.6346584048717,22.3073335234437));
#46410=CARTESIAN_POINT('Ctrl Pts',(-13.8952013288733,33.7619885269329,22.3007656970566));
#46411=CARTESIAN_POINT('Ctrl Pts',(-13.9316569522712,33.8912626056376,22.2941978706695));
#46412=CARTESIAN_POINT('Ctrl Pts',(-13.9679980306452,34.020130500027,22.2876506806551));
#46413=CARTESIAN_POINT('Ctrl Pts',(-13.998039658383,34.1509299686843,22.2811034906407));
#46414=CARTESIAN_POINT('Ctrl Pts',(-14.0215963303964,34.2830704669619,22.2745563006263));
#46415=CARTESIAN_POINT('Ctrl Pts',(-14.045014957528,34.4144366063038,22.2680474779191));
#46416=CARTESIAN_POINT('Ctrl Pts',(-14.0620243166781,34.5471279040333,22.2615386552119));
#46417=CARTESIAN_POINT('Ctrl Pts',(-14.0724898512343,34.6805451337141,22.2550298325047));
#46418=CARTESIAN_POINT('Ctrl Pts',(-14.0807516711158,34.7858688622623,22.2498915645492));
#46419=CARTESIAN_POINT('Ctrl Pts',(-14.0849362747585,34.8916445871562,22.2447532965937));
#46420=CARTESIAN_POINT('Ctrl Pts',(-14.0849992774348,34.997570317556,22.2396150286382));
#46421=CARTESIAN_POINT('Origin',(-10.,35.,32.7603849714045));
#46422=CARTESIAN_POINT('',(-7.51282733495087,38.2405550657615,24.2969436900965));
#46423=CARTESIAN_POINT('',(-7.51282733495086,38.2405550657615,24.1926554110861));
#46424=CARTESIAN_POINT('',(-7.51282733495086,38.2405550657615,32.7603849714045));
#46425=CARTESIAN_POINT('',(-14.0849994926668,35.0020359057622,23.3853849713652));
#46426=CARTESIAN_POINT('Ctrl Pts',(-7.51282733495086,38.2405550657615,24.1926554110861));
#46427=CARTESIAN_POINT('Ctrl Pts',(-7.41801595757955,38.1677859686938,24.1868522021358));
#46428=CARTESIAN_POINT('Ctrl Pts',(-7.32640211884168,38.090853475721,24.1810489931854));
#46429=CARTESIAN_POINT('Ctrl Pts',(-7.23836078677592,38.0100787125893,24.175245784235));
#46430=CARTESIAN_POINT('Ctrl Pts',(-7.15029803900647,37.9292843013178,24.1694411636772));
#46431=CARTESIAN_POINT('Ctrl Pts',(-7.06580982687109,37.8446460372456,24.1636365431193));
#46432=CARTESIAN_POINT('Ctrl Pts',(-6.98523496836354,37.7565225926921,24.1578319225615));
#46433=CARTESIAN_POINT('Ctrl Pts',(-6.90457399469106,37.6683049653488,24.1520210982589));
#46434=CARTESIAN_POINT('Ctrl Pts',(-6.82783500204308,37.5765950215359,24.1462102739563));
#46435=CARTESIAN_POINT('Ctrl Pts',(-6.75531726620277,37.4817854373411,24.1403994496536));
#46436=CARTESIAN_POINT('Ctrl Pts',(-6.68275717128929,37.3869204729545,24.1345852311313));
#46437=CARTESIAN_POINT('Ctrl Pts',(-6.61442347813049,37.2889525962203,24.1287710126089));
#46438=CARTESIAN_POINT('Ctrl Pts',(-6.55057180331045,37.1883030219517,24.1229567940865));
#46439=CARTESIAN_POINT('Ctrl Pts',(-6.48662268280583,37.087499843777,24.1171337023356));
#46440=CARTESIAN_POINT('Ctrl Pts',(-6.42716944479547,36.9840071480697,24.1113106105847));
#46441=CARTESIAN_POINT('Ctrl Pts',(-6.3724216621271,36.8782705882261,24.1054875188338));
#46442=CARTESIAN_POINT('Ctrl Pts',(-6.3391164979892,36.8139470063507,24.1019451100438));
#46443=CARTESIAN_POINT('Ctrl Pts',(-6.30755177516101,36.7487934398425,24.0984027012539));
#46444=CARTESIAN_POINT('Ctrl Pts',(-6.27776578209767,36.6829133747989,24.0948602924639));
#46445=CARTESIAN_POINT('Ctrl Pts',(-6.22879867214834,36.5746088982081,24.0890366987924));
#46446=CARTESIAN_POINT('Ctrl Pts',(-6.18448346565953,36.4639908317763,24.0832131051209));
#46447=CARTESIAN_POINT('Ctrl Pts',(-6.14504422535157,36.3514958288891,24.0773895114494));
#46448=CARTESIAN_POINT('Ctrl Pts',(-6.1056547435035,36.2391427551579,24.0715732651064));
#46449=CARTESIAN_POINT('Ctrl Pts',(-6.07112912604364,36.1249178368807,24.0657570187633));
#46450=CARTESIAN_POINT('Ctrl Pts',(-6.04164439422485,36.0092798909264,24.0599407724203));
#46451=CARTESIAN_POINT('Ctrl Pts',(-6.01218917678531,35.8937576991942,24.0541303481719));
#46452=CARTESIAN_POINT('Ctrl Pts',(-5.98776490699338,35.7768256870582,24.0483199239235));
#46453=CARTESIAN_POINT('Ctrl Pts',(-5.96849937054938,35.6589595395312,24.0425094996752));
#46454=CARTESIAN_POINT('Ctrl Pts',(-5.94850459370311,35.536631914532,24.036479138851));
#46455=CARTESIAN_POINT('Ctrl Pts',(-5.93406695235358,35.413298461934,24.0304487780269));
#46456=CARTESIAN_POINT('Ctrl Pts',(-5.92527156445519,35.2895050544681,24.0244184172027));
#46457=CARTESIAN_POINT('Ctrl Pts',(-5.91680649666945,35.1703608395985,24.0186145329694));
#46458=CARTESIAN_POINT('Ctrl Pts',(-5.91356755497438,35.0507910389473,24.0128106487362));
#46459=CARTESIAN_POINT('Ctrl Pts',(-5.91557791684954,34.9312886714371,24.0070067645029));
#46460=CARTESIAN_POINT('Ctrl Pts',(-5.91758798177276,34.8118039557044,24.0012037375654));
#46461=CARTESIAN_POINT('Ctrl Pts',(-5.92484580141719,34.6923870614731,23.9954007106279));
#46462=CARTESIAN_POINT('Ctrl Pts',(-5.93732242544661,34.5735308625223,23.9895976836904));
#46463=CARTESIAN_POINT('Ctrl Pts',(-5.94980015103141,34.4546641698125,23.9837941444063));
#46464=CARTESIAN_POINT('Ctrl Pts',(-5.96749755448297,34.3363586769337,23.9779906051222));
#46465=CARTESIAN_POINT('Ctrl Pts',(-5.99033389170669,34.2191013510039,23.9721870658381));
#46466=CARTESIAN_POINT('Ctrl Pts',(-6.01317763448839,34.10180599989,23.9663816445339));
#46467=CARTESIAN_POINT('Ctrl Pts',(-6.04116354730872,33.9855598923264,23.9605762232297));
#46468=CARTESIAN_POINT('Ctrl Pts',(-6.07416007869768,33.870838402925,23.9547708019254));
#46469=CARTESIAN_POINT('Ctrl Pts',(-6.10719315069095,33.7559898700929,23.9489589516545));
#46470=CARTESIAN_POINT('Ctrl Pts',(-6.14524780418735,33.642669718221,23.9431471013835));
#46471=CARTESIAN_POINT('Ctrl Pts',(-6.18814299626849,33.5313369402402,23.9373352511126));
#46472=CARTESIAN_POINT('Ctrl Pts',(-6.231066362142,33.4199310382933,23.9315195835871));
#46473=CARTESIAN_POINT('Ctrl Pts',(-6.27883643523125,33.3105154831759,23.9257039160617));
#46474=CARTESIAN_POINT('Ctrl Pts',(-6.33122523149234,33.2035265941402,23.9198882485363));
#46475=CARTESIAN_POINT('Ctrl Pts',(-6.38368906904711,33.0963844550736,23.9140642506952));
#46476=CARTESIAN_POINT('Ctrl Pts',(-6.44078463980339,32.9916762771008,23.908240252854));
#46477=CARTESIAN_POINT('Ctrl Pts',(-6.50223944854455,32.8898113532951,23.9024162550128));
#46478=CARTESIAN_POINT('Ctrl Pts',(-6.51854374427875,32.8627860337687,23.9008711166404));
#46479=CARTESIAN_POINT('Ctrl Pts',(-6.53515464753998,32.8359606696416,23.8993259782679));
#46480=CARTESIAN_POINT('Ctrl Pts',(-6.5520665903944,32.809342518118,23.8977808398955));
#46481=CARTESIAN_POINT('Ctrl Pts',(-6.6158073434137,32.7090192710078,23.891957246224));
#46482=CARTESIAN_POINT('Ctrl Pts',(-6.68403312025836,32.6113185160413,23.8861336525526));
#46483=CARTESIAN_POINT('Ctrl Pts',(-6.75650153965819,32.5166670102944,23.8803100588811));
#46484=CARTESIAN_POINT('Ctrl Pts',(-6.82887852938271,32.4221349214811,23.8744938125381));
#46485=CARTESIAN_POINT('Ctrl Pts',(-6.90548726917439,32.3306447514965,23.8686775661951));
#46486=CARTESIAN_POINT('Ctrl Pts',(-6.98604105444614,32.2425960625045,23.862861319852));
#46487=CARTESIAN_POINT('Ctrl Pts',(-7.06651420493434,32.1546355107359,23.8570508956037));
#46488=CARTESIAN_POINT('Ctrl Pts',(-7.15092427078563,32.0701098862195,23.8512404713553));
#46489=CARTESIAN_POINT('Ctrl Pts',(-7.2389434502476,31.9893868184256,23.845430047107));
#46490=CARTESIAN_POINT('Ctrl Pts',(-7.33029433770718,31.9056082155517,23.8393996862828));
#46491=CARTESIAN_POINT('Ctrl Pts',(-7.42553268961834,31.825926082405,23.8333693254587));
#46492=CARTESIAN_POINT('Ctrl Pts',(-7.52424861234205,31.7507108367353,23.8273389646345));
#46493=CARTESIAN_POINT('Ctrl Pts',(-7.61925715398179,31.6783203793198,23.8215350804013));
#46494=CARTESIAN_POINT('Ctrl Pts',(-7.71748641525967,31.6100676123452,23.815731196168));
#46495=CARTESIAN_POINT('Ctrl Pts',(-7.81853675442483,31.5462421758026,23.8099273119348));
#46496=CARTESIAN_POINT('Ctrl Pts',(-7.91957216737421,31.4824261669596,23.8041242849973));
#46497=CARTESIAN_POINT('Ctrl Pts',(-8.0234274843748,31.423036406021,23.7983212580599));
#46498=CARTESIAN_POINT('Ctrl Pts',(-8.12967461049948,31.3683188552146,23.7925182311224));
#46499=CARTESIAN_POINT('Ctrl Pts',(-8.2359311171346,31.3135964734205,23.7867146918383));
#46500=CARTESIAN_POINT('Ctrl Pts',(-8.34457948971319,31.2635473088899,23.7809111525543));
#46501=CARTESIAN_POINT('Ctrl Pts',(-8.45516818201734,31.218370767229,23.7751076132702));
#46502=CARTESIAN_POINT('Ctrl Pts',(-8.5657927369445,31.1731795753425,23.769302191966));
#46503=CARTESIAN_POINT('Ctrl Pts',(-8.67835848516235,31.1328643031991,23.7634967706618));
#46504=CARTESIAN_POINT('Ctrl Pts',(-8.79239572533773,31.0975755079928,23.7576913493577));
#46505=CARTESIAN_POINT('Ctrl Pts',(-8.90655925120153,31.0622476337121,23.7518794990867));
#46506=CARTESIAN_POINT('Ctrl Pts',(-9.02219713140855,31.0319574680794,23.7460676488158));
#46507=CARTESIAN_POINT('Ctrl Pts',(-9.13882623638185,31.0068051952283,23.7402557985449));
#46508=CARTESIAN_POINT('Ctrl Pts',(-9.25553194397738,30.9816364022293,23.7344401310195));
#46509=CARTESIAN_POINT('Ctrl Pts',(-9.37322977127797,30.9616122909336,23.7286244634941));
#46510=CARTESIAN_POINT('Ctrl Pts',(-9.49142982090204,30.946781356387,23.7228087959687));
#46511=CARTESIAN_POINT('Ctrl Pts',(-9.60979917933367,30.9319291781281,23.7169847981276));
#46512=CARTESIAN_POINT('Ctrl Pts',(-9.72867179037554,30.9222850566915,23.7111608002865));
#46513=CARTESIAN_POINT('Ctrl Pts',(-9.8475559611583,30.9178454444961,23.7053368024454));
#46514=CARTESIAN_POINT('Ctrl Pts',(-9.87909657968253,30.9166675911811,23.7037916640726));
#46515=CARTESIAN_POINT('Ctrl Pts',(-9.91063803235893,30.9158557838219,23.7022465256998));
#46516=CARTESIAN_POINT('Ctrl Pts',(-9.94217119733301,30.915409343694,23.700701387327));
#46517=CARTESIAN_POINT('Ctrl Pts',(-10.0610190256046,30.9137267203452,23.6948777936556));
#46518=CARTESIAN_POINT('Ctrl Pts',(-10.1801320038198,30.9172327961846,23.6890541999841));
#46519=CARTESIAN_POINT('Ctrl Pts',(-10.2990203400902,30.9259587831967,23.6832306063126));
#46520=CARTESIAN_POINT('Ctrl Pts',(-10.4177586810649,30.93467376108,23.6774143599696));
#46521=CARTESIAN_POINT('Ctrl Pts',(-10.5362725401572,30.9485955217199,23.6715981136266));
#46522=CARTESIAN_POINT('Ctrl Pts',(-10.6540705740902,30.9677032990975,23.6657818672836));
#46523=CARTESIAN_POINT('Ctrl Pts',(-10.7717506915413,30.9867919494845,23.6599714430352));
#46524=CARTESIAN_POINT('Ctrl Pts',(-10.8887160085587,31.0110562242921,23.6541610187869));
#46525=CARTESIAN_POINT('Ctrl Pts',(-11.0044793614797,31.0404234806786,23.6483505945386));
#46526=CARTESIAN_POINT('Ctrl Pts',(-11.1246245967487,31.0709023484613,23.6423202337144));
#46527=CARTESIAN_POINT('Ctrl Pts',(-11.2434746293577,31.1068781148384,23.6362898728902));
#46528=CARTESIAN_POINT('Ctrl Pts',(-11.3604949638257,31.1482110061161,23.6302595120661));
#46529=CARTESIAN_POINT('Ctrl Pts',(-11.4731204756299,31.1879915968627,23.6244556278328));
#46530=CARTESIAN_POINT('Ctrl Pts',(-11.5840508237368,31.2327340357742,23.6186517435996));
#46531=CARTESIAN_POINT('Ctrl Pts',(-11.6928246925636,31.2822628441151,23.6128478593664));
#46532=CARTESIAN_POINT('Ctrl Pts',(-11.8015824943266,31.3317843365213,23.6070448324289));
#46533=CARTESIAN_POINT('Ctrl Pts',(-11.9081840787502,31.3860906231921,23.6012418054915));
#46534=CARTESIAN_POINT('Ctrl Pts',(-12.0121890640777,31.4449584854174,23.595438778554));
#46535=CARTESIAN_POINT('Ctrl Pts',(-12.1162032319578,31.5038315450593,23.58963523927));
#46536=CARTESIAN_POINT('Ctrl Pts',(-12.2176199895527,31.5672667798505,23.5838316999859));
#46537=CARTESIAN_POINT('Ctrl Pts',(-12.3160250385771,31.6349958364537,23.5780281607019));
#46538=CARTESIAN_POINT('Ctrl Pts',(-12.4144619992115,31.7027468568003,23.5722227393977));
#46539=CARTESIAN_POINT('Ctrl Pts',(-12.5098849727222,31.7747942368095,23.5664173180935));
#46540=CARTESIAN_POINT('Ctrl Pts',(-12.6019105642536,31.8508276618093,23.5606118967894));
#46541=CARTESIAN_POINT('Ctrl Pts',(-12.6940380656099,31.9269452867898,23.5548000465184));
#46542=CARTESIAN_POINT('Ctrl Pts',(-12.7827603601636,32.0070575075925,23.5489881962475));
#46543=CARTESIAN_POINT('Ctrl Pts',(-12.8677288227591,32.0908151658727,23.5431763459766));
#46544=CARTESIAN_POINT('Ctrl Pts',(-12.9527530930976,32.174627836633,23.5373606784512));
#46545=CARTESIAN_POINT('Ctrl Pts',(-13.0340183439925,32.2620904148114,23.5315450109258));
#46546=CARTESIAN_POINT('Ctrl Pts',(-13.1112154716859,32.3528197475914,23.5257293434004));
#46547=CARTESIAN_POINT('Ctrl Pts',(-13.1885231759283,32.4436790403428,23.5199053455592));
#46548=CARTESIAN_POINT('Ctrl Pts',(-13.2617508764709,32.5378141061121,23.5140813477181));
#46549=CARTESIAN_POINT('Ctrl Pts',(-13.3306320122865,32.6348117625161,23.508257349877));
#46550=CARTESIAN_POINT('Ctrl Pts',(-13.3489065530772,32.6605457694769,23.5067122115042));
#46551=CARTESIAN_POINT('Ctrl Pts',(-13.3668754008443,32.6864811271589,23.5051670731314));
#46552=CARTESIAN_POINT('Ctrl Pts',(-13.384534122985,32.7126098342542,23.5036219347586));
#46553=CARTESIAN_POINT('Ctrl Pts',(-13.4520539487645,32.8125154637139,23.4977139492936));
#46554=CARTESIAN_POINT('Ctrl Pts',(-13.5152498617656,32.9155658287591,23.4918059638286));
#46555=CARTESIAN_POINT('Ctrl Pts',(-13.5738211458682,33.0213571779258,23.4858979783635));
#46556=CARTESIAN_POINT('Ctrl Pts',(-13.632313063434,33.1270051753951,23.4799979984656));
#46557=CARTESIAN_POINT('Ctrl Pts',(-13.6861926320066,33.2353864267388,23.4740980185677));
#46558=CARTESIAN_POINT('Ctrl Pts',(-13.7352017518379,33.3460674520807,23.4681980386698));
#46559=CARTESIAN_POINT('Ctrl Pts',(-13.7841547944733,33.456621834023,23.4623048096446));
#46560=CARTESIAN_POINT('Ctrl Pts',(-13.8282483207179,33.5694703964324,23.4564115806194));
#46561=CARTESIAN_POINT('Ctrl Pts',(-13.8672698330022,33.6841546296196,23.4505183515942));
#46562=CARTESIAN_POINT('Ctrl Pts',(-13.9062483904797,33.7987126186204,23.4446316098243));
#46563=CARTESIAN_POINT('Ctrl Pts',(-13.9401659294038,33.9151018831737,23.4387448680545));
#46564=CARTESIAN_POINT('Ctrl Pts',(-13.9688580865625,34.0328441238729,23.4328581262846));
#46565=CARTESIAN_POINT('Ctrl Pts',(-13.9975315945566,34.150509835142,23.4269752107456));
#46566=CARTESIAN_POINT('Ctrl Pts',(-14.020986387276,34.2695263920299,23.4210922952066));
#46567=CARTESIAN_POINT('Ctrl Pts',(-14.0391079923919,34.3894006012155,23.4152093796675));
#46568=CARTESIAN_POINT('Ctrl Pts',(-14.0572220478135,34.5092248692604,23.409328915027));
#46569=CARTESIAN_POINT('Ctrl Pts',(-14.0700072787421,34.6299056907764,23.4034484503864));
#46570=CARTESIAN_POINT('Ctrl Pts',(-14.0774004327816,34.7509403469993,23.3975679857458));
#46571=CARTESIAN_POINT('Ctrl Pts',(-14.0825060895164,34.8345259728912,23.3935069809654));
#46572=CARTESIAN_POINT('Ctrl Pts',(-14.0850412353373,34.9182801351345,23.3894459761849));
#46573=CARTESIAN_POINT('Ctrl Pts',(-14.0849994926672,35.0020359049511,23.3853849714045));
#46574=CARTESIAN_POINT('Ctrl Pts',(-14.0849994926668,35.0020359057622,23.3853849713652));
#46575=CARTESIAN_POINT('Ctrl Pts',(-14.0849319581215,35.1375424641162,23.3788147639339));
#46576=CARTESIAN_POINT('Ctrl Pts',(-14.0781173618785,35.2728211146141,23.3722445565027));
#46577=CARTESIAN_POINT('Ctrl Pts',(-14.0646509392799,35.4072318035354,23.3656743490714));
#46578=CARTESIAN_POINT('Ctrl Pts',(-14.0514755036666,35.5387381011188,23.3592461128904));
#46579=CARTESIAN_POINT('Ctrl Pts',(-14.0319329338456,35.6694133588879,23.3528178767094));
#46580=CARTESIAN_POINT('Ctrl Pts',(-14.0061633244727,35.7986741623779,23.3463896405284));
#46581=CARTESIAN_POINT('Ctrl Pts',(-13.9795400103919,35.9322171633543,23.339748447472));
#46582=CARTESIAN_POINT('Ctrl Pts',(-13.9462701124894,36.0642500789004,23.3331072544156));
#46583=CARTESIAN_POINT('Ctrl Pts',(-13.9065621511343,36.1941512296711,23.3264660613593));
#46584=CARTESIAN_POINT('Ctrl Pts',(-13.8668541897792,36.3240523804417,23.3198248683029));
#46585=CARTESIAN_POINT('Ctrl Pts',(-13.8207083428048,36.451821524871,23.3131836752465));
#46586=CARTESIAN_POINT('Ctrl Pts',(-13.7683854637982,36.5768627068437,23.3065424821901));
#46587=CARTESIAN_POINT('Ctrl Pts',(-13.7225040710322,36.6865100292187,23.3007188885187));
#46588=CARTESIAN_POINT('Ctrl Pts',(-13.671759167446,36.7943300130207,23.2948952948473));
#46589=CARTESIAN_POINT('Ctrl Pts',(-13.6163175769508,36.8998610956163,23.2890717011758));
#46590=CARTESIAN_POINT('Ctrl Pts',(-13.5609459342572,37.005259035076,23.2832554548328));
#46591=CARTESIAN_POINT('Ctrl Pts',(-13.5008895787069,37.1083734587724,23.2774392084898));
#46592=CARTESIAN_POINT('Ctrl Pts',(-13.4363636137901,37.2087621225066,23.2716229621468));
#46593=CARTESIAN_POINT('Ctrl Pts',(-13.3719022397201,37.3090502966344,23.2658125378984));
#46594=CARTESIAN_POINT('Ctrl Pts',(-13.3029803764777,37.4066177972895,23.2600021136501));
#46595=CARTESIAN_POINT('Ctrl Pts',(-13.2298590274942,37.5010469132974,23.2541916894018));
#46596=CARTESIAN_POINT('Ctrl Pts',(-13.1539698842106,37.5990503666593,23.2481613285776));
#46597=CARTESIAN_POINT('Ctrl Pts',(-13.0735572636367,37.6936727555006,23.2421309677534));
#46598=CARTESIAN_POINT('Ctrl Pts',(-12.9889626109015,37.784479755831,23.2361006069293));
#46599=CARTESIAN_POINT('Ctrl Pts',(-12.9075449999921,37.8718764030386,23.230296722696));
#46600=CARTESIAN_POINT('Ctrl Pts',(-12.8222541168128,37.9557387498776,23.2244928384628));
#46601=CARTESIAN_POINT('Ctrl Pts',(-12.7334349445222,38.0357138211737,23.2186889542296));
#46602=CARTESIAN_POINT('Ctrl Pts',(-12.6446288917731,38.1156770792965,23.2128859272921));
#46603=CARTESIAN_POINT('Ctrl Pts',(-12.5522958897155,38.1917539306026,23.2070829003546));
#46604=CARTESIAN_POINT('Ctrl Pts',(-12.4568163427329,38.2636296447484,23.2012798734172));
#46605=CARTESIAN_POINT('Ctrl Pts',(-12.3613283659046,38.3355117047682,23.1954763341331));
#46606=CARTESIAN_POINT('Ctrl Pts',(-12.2626936180526,38.4031916445604,23.1896727948491));
#46607=CARTESIAN_POINT('Ctrl Pts',(-12.1613234809667,38.466396660889,23.183869255565));
#46608=CARTESIAN_POINT('Ctrl Pts',(-12.0599204707275,38.5296221738672,23.1780638342609));
#46609=CARTESIAN_POINT('Ctrl Pts',(-11.9557806534257,38.5883696614061,23.1722584129567));
#46610=CARTESIAN_POINT('Ctrl Pts',(-11.8493415552261,38.6424114007226,23.1664529916525));
#46611=CARTESIAN_POINT('Ctrl Pts',(-11.7427845855772,38.6965129862633,23.1606411413816));
#46612=CARTESIAN_POINT('Ctrl Pts',(-11.6339236168275,38.7458982366489,23.1548292911107));
#46613=CARTESIAN_POINT('Ctrl Pts',(-11.5232179180482,38.790386810622,23.1490174408398));
#46614=CARTESIAN_POINT('Ctrl Pts',(-11.4124395071716,38.8349046049292,23.1432017733144));
#46615=CARTESIAN_POINT('Ctrl Pts',(-11.299814337594,38.8745191825742,23.1373861057891));
#46616=CARTESIAN_POINT('Ctrl Pts',(-11.1858170787976,38.9091000058366,23.1315704382637));
#46617=CARTESIAN_POINT('Ctrl Pts',(-11.0716565312375,38.9437303623943,23.1257464404226));
#46618=CARTESIAN_POINT('Ctrl Pts',(-10.95612036586,38.9733124722587,23.1199224425815));
#46619=CARTESIAN_POINT('Ctrl Pts',(-10.8396938113804,38.9977667894875,23.1140984447403));
#46620=CARTESIAN_POINT('Ctrl Pts',(-10.8088052118554,39.0042546531447,23.1125533063675));
#46621=CARTESIAN_POINT('Ctrl Pts',(-10.7778539682479,39.0103818700821,23.1110081679946));
#46622=CARTESIAN_POINT('Ctrl Pts',(-10.7468491860047,39.0161475686738,23.1094630296217));
#46623=CARTESIAN_POINT('Ctrl Pts',(-10.6299803966617,39.0378806745165,23.1036388167764));
#46624=CARTESIAN_POINT('Ctrl Pts',(-10.5119736989003,39.0545433208812,23.0978146039311));
#46625=CARTESIAN_POINT('Ctrl Pts',(-10.3933067302697,39.0660219891098,23.0919903910859));
#46626=CARTESIAN_POINT('Ctrl Pts',(-10.27479242528,39.0774858901685,23.086173671021));
#46627=CARTESIAN_POINT('Ctrl Pts',(-10.1556199421426,39.0837790401271,23.0803569509561));
#46628=CARTESIAN_POINT('Ctrl Pts',(-10.0362771935645,39.0848389154564,23.0745402308913));
#46629=CARTESIAN_POINT('Ctrl Pts',(-9.91707555091006,39.085897537633,23.0687303882753));
#46630=CARTESIAN_POINT('Ctrl Pts',(-9.79770444963335,39.0817352006476,23.0629205456594));
#46631=CARTESIAN_POINT('Ctrl Pts',(-9.67865617647097,39.0723412365714,23.0571107030434));
#46632=CARTESIAN_POINT('Ctrl Pts',(-9.55968699036968,39.0629535131653,23.0513047200666));
#46633=CARTESIAN_POINT('Ctrl Pts',(-9.4410406114256,39.0483411063072,23.0454987370898));
#46634=CARTESIAN_POINT('Ctrl Pts',(-9.32320835254928,39.0285454032369,23.039692754113));
#46635=CARTESIAN_POINT('Ctrl Pts',(-9.20542656317161,39.0087581789925,23.0338892579345));
#46636=CARTESIAN_POINT('Ctrl Pts',(-9.08845860213525,38.9837921425446,23.0280857617559));
#46637=CARTESIAN_POINT('Ctrl Pts',(-8.97278905484733,38.953740339749,23.0222822655773));
#46638=CARTESIAN_POINT('Ctrl Pts',(-8.85714175273698,38.9236943164149,23.0164798855076));
#46639=CARTESIAN_POINT('Ctrl Pts',(-8.74279276211062,38.8885645766798,23.0106775054378));
#46640=CARTESIAN_POINT('Ctrl Pts',(-8.63021426868508,38.8484947772195,23.0048751253681));
#46641=CARTESIAN_POINT('Ctrl Pts',(-8.51759076243004,38.8084089564483,22.9990704253033));
#46642=CARTESIAN_POINT('Ctrl Pts',(-8.40673955369542,38.7633792637949,22.9932657252385));
#46643=CARTESIAN_POINT('Ctrl Pts',(-8.29811539405272,38.7135984958043,22.9874610251737));
#46644=CARTESIAN_POINT('Ctrl Pts',(-8.18946829494124,38.6638072150108,22.9816550992607));
#46645=CARTESIAN_POINT('Ctrl Pts',(-8.08304954841149,38.6092630402489,22.9758491733477));
#46646=CARTESIAN_POINT('Ctrl Pts',(-7.9792905795812,38.5502054078927,22.9700432474347));
#46647=CARTESIAN_POINT('Ctrl Pts',(-7.87543494651362,38.4910927560905,22.9642319125878));
#46648=CARTESIAN_POINT('Ctrl Pts',(-7.77424438905138,38.4274584610306,22.9584205777409));
#46649=CARTESIAN_POINT('Ctrl Pts',(-7.67612259923038,38.3595861093582,22.952609242894));
#46650=CARTESIAN_POINT('Ctrl Pts',(-7.62068926029576,38.3212420159472,22.9493261628073));
#46651=CARTESIAN_POINT('Ctrl Pts',(-7.56623480188463,38.2815460655043,22.9460430827206));
#46652=CARTESIAN_POINT('Ctrl Pts',(-7.51282733495087,38.2405550657615,22.942760002634));
#46653=CARTESIAN_POINT('',(-14.0849999165586,34.9991743389247,23.4896150285502));
#46654=CARTESIAN_POINT('Ctrl Pts',(-14.0849999165586,34.9991743389247,23.4896150285502));
#46655=CARTESIAN_POINT('Ctrl Pts',(-14.0850238118884,35.1173976913746,23.4838237303793));
#46656=CARTESIAN_POINT('Ctrl Pts',(-14.0799112176567,35.2358210967393,23.4780324322084));
#46657=CARTESIAN_POINT('Ctrl Pts',(-14.0696361080072,35.3539589642939,23.4722411340375));
#46658=CARTESIAN_POINT('Ctrl Pts',(-14.0593738341097,35.4719492530461,23.4664570704042));
#46659=CARTESIAN_POINT('Ctrl Pts',(-14.0439619044241,35.5896543051682,23.4606730067709));
#46660=CARTESIAN_POINT('Ctrl Pts',(-14.0234262888692,35.706587502038,23.4548889431377));
#46661=CARTESIAN_POINT('Ctrl Pts',(-14.0029108151614,35.8234060078938,23.4491105526591));
#46662=CARTESIAN_POINT('Ctrl Pts',(-13.9772817220657,35.9394537594224,23.4433321621806));
#46663=CARTESIAN_POINT('Ctrl Pts',(-13.9466168096246,36.054248907037,23.4375537717021));
#46664=CARTESIAN_POINT('Ctrl Pts',(-13.9159728587046,36.1689655844809,23.4317793311404));
#46665=CARTESIAN_POINT('Ctrl Pts',(-13.8803000416626,36.2824309629973,23.4260048905788));
#46666=CARTESIAN_POINT('Ctrl Pts',(-13.8397271776588,36.3941736624783,23.4202304500171));
#46667=CARTESIAN_POINT('Ctrl Pts',(-13.799168923569,36.5058761244445,23.4144580887782));
#46668=CARTESIAN_POINT('Ctrl Pts',(-13.753714270898,36.6158567524158,23.4086857275393));
#46669=CARTESIAN_POINT('Ctrl Pts',(-13.7035416294543,36.7236601750053,23.4029133663004));
#46670=CARTESIAN_POINT('Ctrl Pts',(-13.653374866864,36.8314509659989,23.3971416814234));
#46671=CARTESIAN_POINT('Ctrl Pts',(-13.598491389195,36.937064684168,23.3913699965464));
#46672=CARTESIAN_POINT('Ctrl Pts',(-13.5391171100778,37.0400674207375,23.3855983116695));
#46673=CARTESIAN_POINT('Ctrl Pts',(-13.4797353646703,37.1430831098572,23.3798259010056));
#46674=CARTESIAN_POINT('Ctrl Pts',(-13.4158619018823,37.243486806659,23.3740534903417));
#46675=CARTESIAN_POINT('Ctrl Pts',(-13.3477674386442,37.3408712430959,23.3682810796779));
#46676=CARTESIAN_POINT('Ctrl Pts',(-13.2796050587144,37.4383528097317,23.3625029116731));
#46677=CARTESIAN_POINT('Ctrl Pts',(-13.2072135061452,37.5328087612768,23.3567247436684));
#46678=CARTESIAN_POINT('Ctrl Pts',(-13.130905624707,37.6238626048591,23.3509465756636));
#46679=CARTESIAN_POINT('Ctrl Pts',(-13.0545602420002,37.7149611965668,23.3451655679964));
#46680=CARTESIAN_POINT('Ctrl Pts',(-12.9742949756232,37.8026540447818,23.3393845603291));
#46681=CARTESIAN_POINT('Ctrl Pts',(-12.8904603476387,37.8866007653862,23.3336035526619));
#46682=CARTESIAN_POINT('Ctrl Pts',(-12.8064891229373,37.9706842653466,23.327813125657));
#46683=CARTESIAN_POINT('Ctrl Pts',(-12.7189372206986,38.0510091615247,23.3220226986521));
#46684=CARTESIAN_POINT('Ctrl Pts',(-12.6281895523726,38.1272743206824,23.3162322716471));
#46685=CARTESIAN_POINT('Ctrl Pts',(-12.5397280240124,38.201618187188,23.3105877186557));
#46686=CARTESIAN_POINT('Ctrl Pts',(-12.4482301579863,38.2721042776266,23.3049431656643));
#46687=CARTESIAN_POINT('Ctrl Pts',(-12.3540776653063,38.3384941733821,23.2992986126729));
#46688=CARTESIAN_POINT('Ctrl Pts',(-12.2569387313004,38.4069899032228,23.2934750190015));
#46689=CARTESIAN_POINT('Ctrl Pts',(-12.1566511796999,38.4713529449552,23.28765142533));
#46690=CARTESIAN_POINT('Ctrl Pts',(-12.0536016281218,38.5312809790465,23.2818278316586));
#46691=CARTESIAN_POINT('Ctrl Pts',(-11.9506820888599,38.591133405021,23.2760115853155));
#46692=CARTESIAN_POINT('Ctrl Pts',(-11.8450078304294,38.6465617490465,23.2701953389725));
#46693=CARTESIAN_POINT('Ctrl Pts',(-11.7369961000549,38.6973057147596,23.2643790926295));
#46694=CARTESIAN_POINT('Ctrl Pts',(-11.6290924900184,38.7479988854831,23.2585686683812));
#46695=CARTESIAN_POINT('Ctrl Pts',(-11.5188564302833,38.7940168336229,23.2527582441328));
#46696=CARTESIAN_POINT('Ctrl Pts',(-11.4067310105654,38.8351444384682,23.2469478198845));
#46697=CARTESIAN_POINT('Ctrl Pts',(-11.290361411796,38.8778288082234,23.2409174590603));
#46698=CARTESIAN_POINT('Ctrl Pts',(-11.1719569820487,38.915245075191,23.2348870982362));
#46699=CARTESIAN_POINT('Ctrl Pts',(-11.0520377807438,38.9472067982166,23.228856737412));
#46700=CARTESIAN_POINT('Ctrl Pts',(-10.9366222721185,38.9779681648652,23.2230528531788));
#46701=CARTESIAN_POINT('Ctrl Pts',(-10.8198041478439,39.0036771868587,23.2172489689455));
#46702=CARTESIAN_POINT('Ctrl Pts',(-10.702063230289,39.0242182123583,23.2114450847123));
#46703=CARTESIAN_POINT('Ctrl Pts',(-10.5843397043267,39.0447562037287,23.2056420577748));
#46704=CARTESIAN_POINT('Ctrl Pts',(-10.465694058307,39.0601276465443,23.1998390308373));
#46705=CARTESIAN_POINT('Ctrl Pts',(-10.3466157934312,39.070268110548,23.1940360038999));
#46706=CARTESIAN_POINT('Ctrl Pts',(-10.2275270151899,39.0804094698486,23.1882324646158));
#46707=CARTESIAN_POINT('Ctrl Pts',(-10.1080059490346,39.0853188974369,23.1824289253317));
#46708=CARTESIAN_POINT('Ctrl Pts',(-9.98854605372726,39.0849839420878,23.1766253860477));
#46709=CARTESIAN_POINT('Ctrl Pts',(-9.86904741896912,39.0846488781165,23.1708199647435));
#46710=CARTESIAN_POINT('Ctrl Pts',(-9.74961040263544,39.0790660500592,23.1650145434394));
#46711=CARTESIAN_POINT('Ctrl Pts',(-9.63072665119051,39.0682750882726,23.1592091221352));
#46712=CARTESIAN_POINT('Ctrl Pts',(-9.51171124699446,39.0574721764945,23.1533972718643));
#46713=CARTESIAN_POINT('Ctrl Pts',(-9.39325073757442,39.0414496554457,23.1475854215933));
#46714=CARTESIAN_POINT('Ctrl Pts',(-9.2758300057599,39.0202988470314,23.1417735713224));
#46715=CARTESIAN_POINT('Ctrl Pts',(-9.15833215137831,38.9991341466526,23.135957903797));
#46716=CARTESIAN_POINT('Ctrl Pts',(-9.04187583206838,38.9728345406241,23.1301422362717));
#46717=CARTESIAN_POINT('Ctrl Pts',(-8.92693250720861,38.9415417232238,23.1243265687463));
#46718=CARTESIAN_POINT('Ctrl Pts',(-8.81182453844765,38.9102040822417,23.1185025709051));
#46719=CARTESIAN_POINT('Ctrl Pts',(-8.69823427728596,38.8738590784108,23.112678573064));
#46720=CARTESIAN_POINT('Ctrl Pts',(-8.58661502727579,38.8326972120006,23.1068545752229));
#46721=CARTESIAN_POINT('Ctrl Pts',(-8.55700183183216,38.8217767444763,23.1053094368501));
#46722=CARTESIAN_POINT('Ctrl Pts',(-8.52752724292257,38.8105174870963,23.1037642984773));
#46723=CARTESIAN_POINT('Ctrl Pts',(-8.49819943683015,38.7989235407498,23.1022191601045));
#46724=CARTESIAN_POINT('Ctrl Pts',(-8.38767210568014,38.7552295820833,23.0963960167005));
#46725=CARTESIAN_POINT('Ctrl Pts',(-8.27887501036345,38.7066375795626,23.0905728732964));
#46726=CARTESIAN_POINT('Ctrl Pts',(-8.1722728246637,38.6533051299525,23.0847497298924));
#46727=CARTESIAN_POINT('Ctrl Pts',(-8.06578901655625,38.600031903959,23.0789330528632));
#46728=CARTESIAN_POINT('Ctrl Pts',(-7.96149563552509,38.542028874668,23.0731163758341));
#46729=CARTESIAN_POINT('Ctrl Pts',(-7.85983920561452,38.4795023745035,23.0672996988049));
#46730=CARTESIAN_POINT('Ctrl Pts',(-7.75829239064119,38.4170432959314,23.0614892938305));
#46731=CARTESIAN_POINT('Ctrl Pts',(-7.65937721402651,38.3500706661944,23.055678888856));
#46732=CARTESIAN_POINT('Ctrl Pts',(-7.56351647808874,38.2788371486634,23.0498684838815));
#46733=CARTESIAN_POINT('Ctrl Pts',(-7.54652342283912,38.266209714843,23.048838484145));
#46734=CARTESIAN_POINT('Ctrl Pts',(-7.52962628560435,38.2534485022311,23.0478084844086));
#46735=CARTESIAN_POINT('Ctrl Pts',(-7.51282733495086,38.2405550657615,23.0467784846721));
#46736=CARTESIAN_POINT('Ctrl Pts',(-7.51282733495087,38.2405550657615,24.2969436900965));
#46737=CARTESIAN_POINT('Ctrl Pts',(-7.44658649974838,38.1897142711191,24.2928610852361));
#46738=CARTESIAN_POINT('Ctrl Pts',(-7.38197057038218,38.1368917967566,24.2887784803756));
#46739=CARTESIAN_POINT('Ctrl Pts',(-7.31909951636829,38.0822066116442,24.2846958755152));
#46740=CARTESIAN_POINT('Ctrl Pts',(-7.22941768704517,38.0042014387603,24.2788722818435));
#46741=CARTESIAN_POINT('Ctrl Pts',(-7.14299859653684,37.9221530692216,24.2730486881718));
#46742=CARTESIAN_POINT('Ctrl Pts',(-7.0602280293539,37.8363648849546,24.2672250945001));
#46743=CARTESIAN_POINT('Ctrl Pts',(-6.97756188953597,37.7506849352248,24.2614088481569));
#46744=CARTESIAN_POINT('Ctrl Pts',(-6.8985353985021,37.6612748466875,24.2555926018137));
#46745=CARTESIAN_POINT('Ctrl Pts',(-6.82350083292964,37.5684777673948,24.2497763554704));
#46746=CARTESIAN_POINT('Ctrl Pts',(-6.74854137737129,37.4757735784904,24.2439659312219));
#46747=CARTESIAN_POINT('Ctrl Pts',(-6.67756615311727,37.3796894593027,24.2381555069733));
#46748=CARTESIAN_POINT('Ctrl Pts',(-6.61088972602059,37.2806044266394,24.2323450827247));
#46749=CARTESIAN_POINT('Ctrl Pts',(-6.54168945825131,37.177768820552,24.2263147219006));
#46750=CARTESIAN_POINT('Ctrl Pts',(-6.47712016569852,37.0717009532391,24.2202843610766));
#46751=CARTESIAN_POINT('Ctrl Pts',(-6.41748691440689,36.9628614295345,24.2142540002525));
#46752=CARTESIAN_POINT('Ctrl Pts',(-6.36009325305589,36.8581094894707,24.208450116019));
#46753=CARTESIAN_POINT('Ctrl Pts',(-6.30727177640937,36.7507907139614,24.2026462317855));
#46754=CARTESIAN_POINT('Ctrl Pts',(-6.25924920886273,36.6413435102397,24.1968423475521));
#46755=CARTESIAN_POINT('Ctrl Pts',(-6.21123373476286,36.5319124730403,24.1910393206144));
#46756=CARTESIAN_POINT('Ctrl Pts',(-6.16801592410824,36.420354006679,24.1852362936767));
#46757=CARTESIAN_POINT('Ctrl Pts',(-6.12977506487738,36.3071281312691,24.179433266739));
#46758=CARTESIAN_POINT('Ctrl Pts',(-6.09153082937854,36.1938922591985,24.1736297274547));
#46759=CARTESIAN_POINT('Ctrl Pts',(-6.05826454962927,36.0789890722679,24.1678261881704));
#46760=CARTESIAN_POINT('Ctrl Pts',(-6.03010597741497,35.9628948278206,24.1620226488861));
#46761=CARTESIAN_POINT('Ctrl Pts',(-6.00193827370406,35.8467629353636,24.1562172275817));
#46762=CARTESIAN_POINT('Ctrl Pts',(-5.97888166787568,35.7294396138604,24.1504118062773));
#46763=CARTESIAN_POINT('Ctrl Pts',(-5.96101490017239,35.6114117788942,24.1446063849729));
#46764=CARTESIAN_POINT('Ctrl Pts',(-5.9431283466776,35.4932532390254,24.1387945347017));
#46765=CARTESIAN_POINT('Ctrl Pts',(-5.93044316449469,35.3743890323574,24.1329826844306));
#46766=CARTESIAN_POINT('Ctrl Pts',(-5.92298628051653,35.2553118311861,24.1271708341594));
#46767=CARTESIAN_POINT('Ctrl Pts',(-5.91552449881694,35.1361564194698,24.1213551666338));
#46768=CARTESIAN_POINT('Ctrl Pts',(-5.91329786176667,35.0167881419714,24.1155394991082));
#46769=CARTESIAN_POINT('Ctrl Pts',(-5.91628117607831,34.8976986454261,24.1097238315826));
#46770=CARTESIAN_POINT('Ctrl Pts',(-5.91926876366556,34.7784385660364,24.1038998337412));
#46771=CARTESIAN_POINT('Ctrl Pts',(-5.92748116972554,34.6594584705499,24.0980758358998));
#46772=CARTESIAN_POINT('Ctrl Pts',(-5.94084147361198,34.5412440107732,24.0922518380585));
#46773=CARTESIAN_POINT('Ctrl Pts',(-5.9443860350524,34.5098810702753,24.0907066996879));
#46774=CARTESIAN_POINT('Ctrl Pts',(-5.94829266398167,34.4785719579324,24.0891615613173));
#46775=CARTESIAN_POINT('Ctrl Pts',(-5.95255932733317,34.4473255920143,24.0876164229467));
#46776=CARTESIAN_POINT('Ctrl Pts',(-5.96864029080211,34.3295587031203,24.0817928292753));
#46777=CARTESIAN_POINT('Ctrl Pts',(-5.9898913818671,34.2123043416862,24.0759692356039));
#46778=CARTESIAN_POINT('Ctrl Pts',(-6.01627033365602,34.0960514696672,24.0701456419325));
#46779=CARTESIAN_POINT('Ctrl Pts',(-6.042616004479,33.9799452679141,24.0643293955896));
#46780=CARTESIAN_POINT('Ctrl Pts',(-6.07407657866468,33.864838437153,24.0585131492466));
#46781=CARTESIAN_POINT('Ctrl Pts',(-6.11055816232705,33.7512137126957,24.0526969029037));
#46782=CARTESIAN_POINT('Ctrl Pts',(-6.14700322772288,33.6377027272145,24.0468864786554));
#46783=CARTESIAN_POINT('Ctrl Pts',(-6.18845917976376,33.5256712831598,24.0410760544071));
#46784=CARTESIAN_POINT('Ctrl Pts',(-6.23478145327104,33.4155902375432,24.0352656301588));
#46785=CARTESIAN_POINT('Ctrl Pts',(-6.28285712064224,33.3013423966617,24.0292352693346));
#46786=CARTESIAN_POINT('Ctrl Pts',(-6.33617468997625,33.1891959619523,24.0232049085104));
#46787=CARTESIAN_POINT('Ctrl Pts',(-6.39451615077475,33.0796585686457,24.0171745476863));
#46788=CARTESIAN_POINT('Ctrl Pts',(-6.45066653618959,32.9742349682195,24.0113706634531));
#46789=CARTESIAN_POINT('Ctrl Pts',(-6.51147005382735,32.8712283654531,24.0055667792199));
#46790=CARTESIAN_POINT('Ctrl Pts',(-6.57668431458382,32.7710687049656,23.9997628949867));
#46791=CARTESIAN_POINT('Ctrl Pts',(-6.64188894249656,32.6709238391312,23.9939598680493));
#46792=CARTESIAN_POINT('Ctrl Pts',(-6.7115027951286,32.5736254213892,23.9881568411119));
#46793=CARTESIAN_POINT('Ctrl Pts',(-6.78523940407018,32.4795755693025,23.9823538141745));
#46794=CARTESIAN_POINT('Ctrl Pts',(-6.85898252318327,32.3855174135973,23.9765502748905));
#46795=CARTESIAN_POINT('Ctrl Pts',(-6.93684887036415,32.2947087151672,23.9707467356065));
#46796=CARTESIAN_POINT('Ctrl Pts',(-7.01851124291598,32.2075190615903,23.9649431963225));
#46797=CARTESIAN_POINT('Ctrl Pts',(-7.1002000976229,32.1203011334255,23.9591377750184));
#46798=CARTESIAN_POINT('Ctrl Pts',(-7.18568714690232,32.0367048820438,23.9533323537143));
#46799=CARTESIAN_POINT('Ctrl Pts',(-7.2746083111431,31.9570630728998,23.9475269324102));
#46800=CARTESIAN_POINT('Ctrl Pts',(-7.36362794734278,31.8773330678238,23.9417150821393));
#46801=CARTESIAN_POINT('Ctrl Pts',(-7.45608898519393,31.8015665187932,23.9359032318685));
#46802=CARTESIAN_POINT('Ctrl Pts',(-7.55159412814597,31.7300560116921,23.9300913815976));
#46803=CARTESIAN_POINT('Ctrl Pts',(-7.64716199938857,31.6584985361061,23.9242757140723));
#46804=CARTESIAN_POINT('Ctrl Pts',(-7.74577762104491,31.5912028991786,23.918460046547));
#46805=CARTESIAN_POINT('Ctrl Pts',(-7.84701598392935,31.5284175328038,23.9126443790217));
#46806=CARTESIAN_POINT('Ctrl Pts',(-7.94839935983682,31.4655422331712,23.9068203811806));
#46807=CARTESIAN_POINT('Ctrl Pts',(-8.05241262046835,31.4071902979273,23.9009963833395));
#46808=CARTESIAN_POINT('Ctrl Pts',(-8.15860741556952,31.3535636094943,23.8951723854985));
#46809=CARTESIAN_POINT('Ctrl Pts',(-8.18678147356946,31.3393361567381,23.8936272471251));
#46810=CARTESIAN_POINT('Ctrl Pts',(-8.21510898346396,31.3254410334175,23.8920821087517));
#46811=CARTESIAN_POINT('Ctrl Pts',(-8.2435813718164,31.311881427805,23.8905369703783));
#46812=CARTESIAN_POINT('Ctrl Pts',(-8.35089319804208,31.2607755626009,23.8847133767068));
#46813=CARTESIAN_POINT('Ctrl Pts',(-8.46061043672434,31.2142747918228,23.8788897830354));
#46814=CARTESIAN_POINT('Ctrl Pts',(-8.57230096503299,31.1726117958124,23.8730661893639));
#46815=CARTESIAN_POINT('Ctrl Pts',(-8.68385057914995,31.13100136386,23.8672499430209));
#46816=CARTESIAN_POINT('Ctrl Pts',(-8.79736815192766,31.09421670827,23.8614336966779));
#46817=CARTESIAN_POINT('Ctrl Pts',(-8.91239846827199,31.0624439168206,23.8556174503349));
#46818=CARTESIAN_POINT('Ctrl Pts',(-9.02731363863492,31.0307029301108,23.8498070260866));
#46819=CARTESIAN_POINT('Ctrl Pts',(-9.14373814878634,31.0039639351248,23.8439966018382));
#46820=CARTESIAN_POINT('Ctrl Pts',(-9.26119894214244,30.9823641283824,23.8381861775899));
#46821=CARTESIAN_POINT('Ctrl Pts',(-9.38310586947809,30.9599467242787,23.8321558167657));
#46822=CARTESIAN_POINT('Ctrl Pts',(-9.50612866105522,30.943065410048,23.8261254559415));
#46823=CARTESIAN_POINT('Ctrl Pts',(-9.62972324000001,30.9318161151438,23.8200950951174));
#46824=CARTESIAN_POINT('Ctrl Pts',(-9.74867609356314,30.9209892994302,23.8142912108841));
#46825=CARTESIAN_POINT('Ctrl Pts',(-9.86815811762731,30.9153791393267,23.8084873266509));
#46826=CARTESIAN_POINT('Ctrl Pts',(-9.98767685004044,30.9150185875606,23.8026834424177));
#46827=CARTESIAN_POINT('Ctrl Pts',(-10.1071779282586,30.9146580890519,23.7968804154802));
#46828=CARTESIAN_POINT('Ctrl Pts',(-10.2267152958179,30.9195456580402,23.7910773885428));
#46829=CARTESIAN_POINT('Ctrl Pts',(-10.3457956016436,30.929662126815,23.7852743616053));
#46830=CARTESIAN_POINT('Ctrl Pts',(-10.4648864210149,30.9397794887682,23.7794708223212));
#46831=CARTESIAN_POINT('Ctrl Pts',(-10.5835196915282,30.9551266338264,23.7736672830372));
#46832=CARTESIAN_POINT('Ctrl Pts',(-10.7012069401966,30.9756324935438,23.7678637437531));
#46833=CARTESIAN_POINT('Ctrl Pts',(-10.8189323534675,30.9961450030725,23.762058322449));
#46834=CARTESIAN_POINT('Ctrl Pts',(-10.9357107327005,31.0218194842462,23.7562529011448));
#46835=CARTESIAN_POINT('Ctrl Pts',(-11.0510641872895,31.0525338412853,23.7504474798406));
#46836=CARTESIAN_POINT('Ctrl Pts',(-11.1665453851523,31.0832822116319,23.7446356295697));
#46837=CARTESIAN_POINT('Ctrl Pts',(-11.2805981137804,31.1190814932624,23.7388237792988));
#46838=CARTESIAN_POINT('Ctrl Pts',(-11.3927598792845,31.1597597837303,23.7330119290279));
#46839=CARTESIAN_POINT('Ctrl Pts',(-11.5049953132384,31.2004647919177,23.7271962615025));
#46840=CARTESIAN_POINT('Ctrl Pts',(-11.6153369340792,31.2460550353328,23.7213805939771));
#46841=CARTESIAN_POINT('Ctrl Pts',(-11.7233439859837,31.2963112298718,23.7155649264518));
#46842=CARTESIAN_POINT('Ctrl Pts',(-11.8315057463272,31.3466394109827,23.7097409286107));
#46843=CARTESIAN_POINT('Ctrl Pts',(-11.9373259022321,31.4016466953953,23.7039169307695));
#46844=CARTESIAN_POINT('Ctrl Pts',(-12.0403898357864,31.4610687604844,23.6980929329284));
#46845=CARTESIAN_POINT('Ctrl Pts',(-12.0677332591423,31.4768337582521,23.6965477945556));
#46846=CARTESIAN_POINT('Ctrl Pts',(-12.094882848487,31.4929092696485,23.6950026561827));
#46847=CARTESIAN_POINT('Ctrl Pts',(-12.1218312375957,31.5092898717935,23.6934575178098));
#46848=CARTESIAN_POINT('Ctrl Pts',(-12.2233991431153,31.5710280129606,23.6876339241383));
#46849=CARTESIAN_POINT('Ctrl Pts',(-12.3224340400303,31.6373023167315,23.6818103304668));
#46850=CARTESIAN_POINT('Ctrl Pts',(-12.4185044472204,31.707878914928,23.6759867367953));
#46851=CARTESIAN_POINT('Ctrl Pts',(-12.5144536473217,31.7783664702627,23.6701704904523));
#46852=CARTESIAN_POINT('Ctrl Pts',(-12.607445470577,31.8531452842684,23.6643542441092));
#46853=CARTESIAN_POINT('Ctrl Pts',(-12.6970747462039,31.9319366347174,23.6585379977661));
#46854=CARTESIAN_POINT('Ctrl Pts',(-12.7866143024314,32.0106491145899,23.6527275735178));
#46855=CARTESIAN_POINT('Ctrl Pts',(-12.8727977022077,32.0933658723848,23.6469171492694));
#46856=CARTESIAN_POINT('Ctrl Pts',(-12.9552508859335,32.17976646336,23.641106725021));
#46857=CARTESIAN_POINT('Ctrl Pts',(-13.0408250932051,32.2694374954099,23.6350763641969));
#46858=CARTESIAN_POINT('Ctrl Pts',(-13.1223807507816,32.3630764869399,23.6290460033727));
#46859=CARTESIAN_POINT('Ctrl Pts',(-13.1995393829108,32.4602809727841,23.6230156425486));
#46860=CARTESIAN_POINT('Ctrl Pts',(-13.2738002408486,32.5538348411587,23.6172117583153));
#46861=CARTESIAN_POINT('Ctrl Pts',(-13.3439881105525,32.6506908730695,23.611407874082));
#46862=CARTESIAN_POINT('Ctrl Pts',(-13.4098054814972,32.7504552508671,23.6056039898487));
#46863=CARTESIAN_POINT('Ctrl Pts',(-13.4756131305124,32.8502048923992,23.5998009629112));
#46864=CARTESIAN_POINT('Ctrl Pts',(-13.5370513397982,32.9528616847393,23.5939979359737));
#46865=CARTESIAN_POINT('Ctrl Pts',(-13.5938657035848,33.0580024962433,23.5881949090362));
#46866=CARTESIAN_POINT('Ctrl Pts',(-13.6506850834856,33.1631525905815,23.5823913697521));
#46867=CARTESIAN_POINT('Ctrl Pts',(-13.7028796120812,33.2707867808696,23.576587830468));
#46868=CARTESIAN_POINT('Ctrl Pts',(-13.7502409658695,33.380457565263,23.5707842911839));
#46869=CARTESIAN_POINT('Ctrl Pts',(-13.7976176783924,33.4901639146125,23.5649788698797));
#46870=CARTESIAN_POINT('Ctrl Pts',(-13.8401579372118,33.601907796859,23.5591734485755));
#46871=CARTESIAN_POINT('Ctrl Pts',(-13.8777018974906,33.7152225896296,23.5533680272713));
#46872=CARTESIAN_POINT('Ctrl Pts',(-13.9152874342304,33.828662868045,23.5475561770004));
#46873=CARTESIAN_POINT('Ctrl Pts',(-13.9478654997087,33.9436771416056,23.5417443267294));
#46874=CARTESIAN_POINT('Ctrl Pts',(-13.9753263458668,34.0597843631074,23.5359324764584));
#46875=CARTESIAN_POINT('Ctrl Pts',(-14.0028052284561,34.1759678444556,23.530116808933));
#46876=CARTESIAN_POINT('Ctrl Pts',(-14.0251601218919,34.2932453031767,23.5243011414076));
#46877=CARTESIAN_POINT('Ctrl Pts',(-14.0423328227828,34.4111279002593,23.5184854738822));
#46878=CARTESIAN_POINT('Ctrl Pts',(-14.0595301217133,34.529179351433,23.512661476041));
#46879=CARTESIAN_POINT('Ctrl Pts',(-14.0715303713907,34.6478372662219,23.5068374781999));
#46880=CARTESIAN_POINT('Ctrl Pts',(-14.0783273651943,34.7666099781324,23.5010134803587));
#46881=CARTESIAN_POINT('Ctrl Pts',(-14.0801306446991,34.7981210260031,23.4994683419863));
#46882=CARTESIAN_POINT('Ctrl Pts',(-14.0815679668199,34.8296401689612,23.4979232036138));
#46883=CARTESIAN_POINT('Ctrl Pts',(-14.0826398292009,34.8611582734834,23.4963780652414));
#46884=CARTESIAN_POINT('Ctrl Pts',(-14.0842036685506,34.9071429567314,23.4941237196927));
#46885=CARTESIAN_POINT('Ctrl Pts',(-14.0849906149495,34.953154209098,23.4918693741441));
#46886=CARTESIAN_POINT('Ctrl Pts',(-14.0849999165584,34.9991743380006,23.4896150285955));
#46887=CARTESIAN_POINT('Origin',(-10.,35.,32.7603849714045));
#46888=CARTESIAN_POINT('',(-7.51282733495086,38.2405550657615,25.5469376052728));
#46889=CARTESIAN_POINT('',(-7.51282733495087,38.2405550657615,25.4425445275748));
#46890=CARTESIAN_POINT('',(-7.51282733495086,38.2405550657615,32.7603849714045));
#46891=CARTESIAN_POINT('',(-14.0849984277889,34.9964160131029,24.6353849714293));
#46892=CARTESIAN_POINT('Ctrl Pts',(-7.51282733495087,38.2405550657615,25.4425445275748));
#46893=CARTESIAN_POINT('Ctrl Pts',(-7.41827383907103,38.167983896451,25.4367331956948));
#46894=CARTESIAN_POINT('Ctrl Pts',(-7.32679683731213,38.0911923601983,25.4309218638148));
#46895=CARTESIAN_POINT('Ctrl Pts',(-7.23879170183744,38.0104740048966,25.4251105319348));
#46896=CARTESIAN_POINT('Ctrl Pts',(-7.15085573664087,37.9298190926094,25.4193037676456));
#46897=CARTESIAN_POINT('Ctrl Pts',(-7.06638650781902,37.8452437774452,25.4134970033563));
#46898=CARTESIAN_POINT('Ctrl Pts',(-6.98574662823781,37.7570820827136,25.4076902390671));
#46899=CARTESIAN_POINT('Ctrl Pts',(-6.90514174153435,37.668958644877,25.4018859945658));
#46900=CARTESIAN_POINT('Ctrl Pts',(-6.8283631753088,37.5772522224484,25.3960817500644));
#46901=CARTESIAN_POINT('Ctrl Pts',(-6.75573660684465,37.4823335867349,25.3902775055631));
#46902=CARTESIAN_POINT('Ctrl Pts',(-6.683124423063,37.3874337509518,25.3844744106716));
#46903=CARTESIAN_POINT('Ctrl Pts',(-6.61466284974465,37.2893232912073,25.37867131578));
#46904=CARTESIAN_POINT('Ctrl Pts',(-6.55063677423441,37.1884054324407,25.3728682208885));
#46905=CARTESIAN_POINT('Ctrl Pts',(-6.48660826976873,37.0874837451561,25.3670649058451));
#46906=CARTESIAN_POINT('Ctrl Pts',(-6.42701581633417,36.9837547919758,25.3612615908017));
#46907=CARTESIAN_POINT('Ctrl Pts',(-6.37210016940302,36.8776495464155,25.3554582757583));
#46908=CARTESIAN_POINT('Ctrl Pts',(-6.31716947910029,36.7715152348107,25.3496533709781));
#46909=CARTESIAN_POINT('Ctrl Pts',(-6.26691833075206,36.6630036988033,25.3438484661979));
#46910=CARTESIAN_POINT('Ctrl Pts',(-6.22154056228396,36.5525686063857,25.3380435614177));
#46911=CARTESIAN_POINT('Ctrl Pts',(-6.17611361638147,36.4420138316944,25.3322323656644));
#46912=CARTESIAN_POINT('Ctrl Pts',(-6.13557075027135,36.3295317166733,25.326421169911));
#46913=CARTESIAN_POINT('Ctrl Pts',(-6.10005692608878,36.2155941017675,25.3206099741577));
#46914=CARTESIAN_POINT('Ctrl Pts',(-6.06452138003439,36.1015867974288,25.3147952240124));
#46915=CARTESIAN_POINT('Ctrl Pts',(-6.03402110671144,35.9861226142386,25.3089804738671));
#46916=CARTESIAN_POINT('Ctrl Pts',(-6.00865023460705,35.8696850293627,25.3031657237219));
#46917=CARTESIAN_POINT('Ctrl Pts',(-5.98324156117036,35.7530739583009,25.2973423098893));
#46918=CARTESIAN_POINT('Ctrl Pts',(-5.96297761825259,35.635486991259,25.2915188960568));
#46919=CARTESIAN_POINT('Ctrl Pts',(-5.94790088227622,35.5174144761621,25.2856954822242));
#46920=CARTESIAN_POINT('Ctrl Pts',(-5.94068755835331,35.4609237808869,25.2829093241077));
#46921=CARTESIAN_POINT('Ctrl Pts',(-5.93466084598134,35.4043219717969,25.2801231659911));
#46922=CARTESIAN_POINT('Ctrl Pts',(-5.92982117855721,35.347662712235,25.2773370078746));
#46923=CARTESIAN_POINT('Ctrl Pts',(-5.91970536480494,35.2292342197704,25.2715134142015));
#46924=CARTESIAN_POINT('Ctrl Pts',(-5.91474633401455,35.1101728819247,25.2656898205283));
#46925=CARTESIAN_POINT('Ctrl Pts',(-5.91500999150824,34.9909650388779,25.2598662268552));
#46926=CARTESIAN_POINT('Ctrl Pts',(-5.91527331635883,34.8719075942315,25.2540499805105));
#46927=CARTESIAN_POINT('Ctrl Pts',(-5.92074622284017,34.7527044167591,25.2482337341658));
#46928=CARTESIAN_POINT('Ctrl Pts',(-5.93144287956206,34.6338470842206,25.2424174878211));
#46929=CARTESIAN_POINT('Ctrl Pts',(-5.9421288288716,34.5151087285273,25.236607063571));
#46930=CARTESIAN_POINT('Ctrl Pts',(-5.95802808957789,34.3967159334161,25.2307966393209));
#46931=CARTESIAN_POINT('Ctrl Pts',(-5.9791027876393,34.2791597905014,25.2249862150709));
#46932=CARTESIAN_POINT('Ctrl Pts',(-6.00097520660355,34.1571539044783,25.2189558542474));
#46933=CARTESIAN_POINT('Ctrl Pts',(-6.02842260533313,34.0360497083627,25.2129254934238));
#46934=CARTESIAN_POINT('Ctrl Pts',(-6.06134350857744,33.9163902720191,25.2068951326003));
#46935=CARTESIAN_POINT('Ctrl Pts',(-6.09302803242813,33.8012247725595,25.2010912483653));
#46936=CARTESIAN_POINT('Ctrl Pts',(-6.1297822303506,33.6873979000119,25.1952873641303));
#46937=CARTESIAN_POINT('Ctrl Pts',(-6.17146381683957,33.5753822638226,25.1894834798953));
#46938=CARTESIAN_POINT('Ctrl Pts',(-6.21313924651255,33.4633831735404,25.1836804529561));
#46939=CARTESIAN_POINT('Ctrl Pts',(-6.25974047496561,33.3531951701633,25.1778774260168));
#46940=CARTESIAN_POINT('Ctrl Pts',(-6.31107611101002,33.2452733713655,25.1720743990776));
#46941=CARTESIAN_POINT('Ctrl Pts',(-6.36241627945433,33.1373420442012,25.1662708597918));
#46942=CARTESIAN_POINT('Ctrl Pts',(-6.41849151116107,33.0316776881912,25.1604673205059));
#46943=CARTESIAN_POINT('Ctrl Pts',(-6.47906354243962,32.9287126076225,25.1546637812201));
#46944=CARTESIAN_POINT('Ctrl Pts',(-6.53965521652162,32.8257141366787,25.1488583599141));
#46945=CARTESIAN_POINT('Ctrl Pts',(-6.60474638338519,32.7254170338091,25.1430529386082));
#46946=CARTESIAN_POINT('Ctrl Pts',(-6.67405472993697,32.6282257568341,25.1372475173022));
#46947=CARTESIAN_POINT('Ctrl Pts',(-6.74343982906742,32.5309268495158,25.1314356670295));
#46948=CARTESIAN_POINT('Ctrl Pts',(-6.81705119265443,32.4367409661172,25.1256238167568));
#46949=CARTESIAN_POINT('Ctrl Pts',(-6.8945652935171,32.3460406401432,25.1198119664841));
#46950=CARTESIAN_POINT('Ctrl Pts',(-6.97213030605738,32.2552807417081,25.1139962989569));
#46951=CARTESIAN_POINT('Ctrl Pts',(-7.05360288281349,32.1680112577565,25.1081806314297));
#46952=CARTESIAN_POINT('Ctrl Pts',(-7.13862278214205,32.0845677135074,25.1023649639026));
#46953=CARTESIAN_POINT('Ctrl Pts',(-7.22376446329569,32.0010046453916,25.0965409660596));
#46954=CARTESIAN_POINT('Ctrl Pts',(-7.31246330612202,31.9212787272494,25.0907169682167));
#46955=CARTESIAN_POINT('Ctrl Pts',(-7.40432609492042,31.8456851808215,25.0848929703738));
#46956=CARTESIAN_POINT('Ctrl Pts',(-7.42869779324151,31.8256298011334,25.0833478320179));
#46957=CARTESIAN_POINT('Ctrl Pts',(-7.45329203647522,31.8058650485147,25.0818026936621));
#46958=CARTESIAN_POINT('Ctrl Pts',(-7.47810115818958,31.7863959124255,25.0802575553062));
#46959=CARTESIAN_POINT('Ctrl Pts',(-7.57160621141033,31.7130171516962,25.0744339616352));
#46960=CARTESIAN_POINT('Ctrl Pts',(-7.66846731883891,31.6436044726484,25.0686103679641));
#46961=CARTESIAN_POINT('Ctrl Pts',(-7.7683138464795,31.5784795905643,25.0627867742931));
#46962=CARTESIAN_POINT('Ctrl Pts',(-7.86803440289447,31.5134368731926,25.0569705279505));
#46963=CARTESIAN_POINT('Ctrl Pts',(-7.9707325489391,31.4526714141459,25.0511542816079));
#46964=CARTESIAN_POINT('Ctrl Pts',(-8.07600490987562,31.3964645286639,25.0453380352653));
#46965=CARTESIAN_POINT('Ctrl Pts',(-8.18117189259796,31.3403139065845,25.0395276110174));
#46966=CARTESIAN_POINT('Ctrl Pts',(-8.28890760584183,31.2887129714506,25.0337171867695));
#46967=CARTESIAN_POINT('Ctrl Pts',(-8.39878055358142,31.2418992450427,25.0279067625216));
#46968=CARTESIAN_POINT('Ctrl Pts',(-8.51281241966084,31.1933135222578,25.0218764016973));
#46969=CARTESIAN_POINT('Ctrl Pts',(-8.62914613917008,31.1498848252515,25.0158460408729));
#46970=CARTESIAN_POINT('Ctrl Pts',(-8.74727187910778,31.1118259741717,25.0098156800486));
#46971=CARTESIAN_POINT('Ctrl Pts',(-8.86096128169651,31.0751964635777,25.0040117958158));
#46972=CARTESIAN_POINT('Ctrl Pts',(-8.97631010603354,31.0435408686069,24.998207911583));
#46973=CARTESIAN_POINT('Ctrl Pts',(-9.09284507948373,31.0169992530527,24.9924040273502));
#46974=CARTESIAN_POINT('Ctrl Pts',(-9.20936283947211,30.9904615579789,24.9866010004132));
#46975=CARTESIAN_POINT('Ctrl Pts',(-9.3270660021089,30.9690364307456,24.9807979734761));
#46976=CARTESIAN_POINT('Ctrl Pts',(-9.44546900642545,30.952813276217,24.9749949465391));
#46977=CARTESIAN_POINT('Ctrl Pts',(-9.56388246448913,30.9365886893536,24.9691914072555));
#46978=CARTESIAN_POINT('Ctrl Pts',(-9.68299548250637,30.9255670437877,24.9633878679718));
#46979=CARTESIAN_POINT('Ctrl Pts',(-9.80231588616876,30.9197860361081,24.9575843286882));
#46980=CARTESIAN_POINT('Ctrl Pts',(-9.92167498404659,30.914003153715,24.9517789073845));
#46981=CARTESIAN_POINT('Ctrl Pts',(-10.0412411936714,30.9134643088361,24.9459734860807));
#46982=CARTESIAN_POINT('Ctrl Pts',(-10.1605214844378,30.9181550919916,24.940168064777));
#46983=CARTESIAN_POINT('Ctrl Pts',(-10.2799338670858,30.9228510697553,24.9343562145065));
#46984=CARTESIAN_POINT('Ctrl Pts',(-10.3990592905939,30.9327882194868,24.928544364236));
#46985=CARTESIAN_POINT('Ctrl Pts',(-10.5174088328717,30.9479001616858,24.9227325139655));
#46986=CARTESIAN_POINT('Ctrl Pts',(-10.6358361077642,30.9630220294894,24.9169168464406));
#46987=CARTESIAN_POINT('Ctrl Pts',(-10.7534860850753,30.9833253893368,24.9111011789156));
#46988=CARTESIAN_POINT('Ctrl Pts',(-10.8698806698456,31.0086928682161,24.9052855113907));
#46989=CARTESIAN_POINT('Ctrl Pts',(-10.9864419772903,31.0340966832697,24.89946151355));
#46990=CARTESIAN_POINT('Ctrl Pts',(-11.1017439096834,31.0645789915572,24.8936375157093));
#46991=CARTESIAN_POINT('Ctrl Pts',(-11.2153240055548,31.099972748618,24.8878135178686));
#46992=CARTESIAN_POINT('Ctrl Pts',(-11.2454574241771,31.1093629053171,24.8862683794916));
#46993=CARTESIAN_POINT('Ctrl Pts',(-11.2754697617164,31.119098503343,24.8847232411147));
#46994=CARTESIAN_POINT('Ctrl Pts',(-11.3053526426732,31.1291758657534,24.8831781027377));
#46995=CARTESIAN_POINT('Ctrl Pts',(-11.4179805852676,31.1671572302912,24.8773545090664));
#46996=CARTESIAN_POINT('Ctrl Pts',(-11.529131078261,31.2101195632519,24.8715309153951));
#46997=CARTESIAN_POINT('Ctrl Pts',(-11.6383318802172,31.2579292296559,24.8657073217238));
#46998=CARTESIAN_POINT('Ctrl Pts',(-11.7473949091412,31.3056785770641,24.859891075381));
#46999=CARTESIAN_POINT('Ctrl Pts',(-11.8545127688013,31.3582629317444,24.8540748290382));
#47000=CARTESIAN_POINT('Ctrl Pts',(-11.9592290599093,31.4154991294733,24.8482585826953));
#47001=CARTESIAN_POINT('Ctrl Pts',(-12.0638405294322,31.4726780334524,24.8424481584472));
#47002=CARTESIAN_POINT('Ctrl Pts',(-12.1660548565827,31.5344993221901,24.836637734199));
#47003=CARTESIAN_POINT('Ctrl Pts',(-12.2654368545924,31.6007323056496,24.8308273099508));
#47004=CARTESIAN_POINT('Ctrl Pts',(-12.3685806667885,31.6694723445293,24.8247969491266));
#47005=CARTESIAN_POINT('Ctrl Pts',(-12.4686730836359,31.7429644808949,24.8187665883024));
#47006=CARTESIAN_POINT('Ctrl Pts',(-12.5652566366221,31.8208989653888,24.8127362274781));
#47007=CARTESIAN_POINT('Ctrl Pts',(-12.6582128919254,31.8959065377296,24.8069323432451));
#47008=CARTESIAN_POINT('Ctrl Pts',(-12.7479187422818,31.9750285219178,24.8011284590121));
#47009=CARTESIAN_POINT('Ctrl Pts',(-12.8339976115554,32.0579458642475,24.795324574779));
#47010=CARTESIAN_POINT('Ctrl Pts',(-12.9200637660593,32.1408509587989,24.7895215478417));
#47011=CARTESIAN_POINT('Ctrl Pts',(-13.0025037108972,32.2275500133955,24.7837185209045));
#47012=CARTESIAN_POINT('Ctrl Pts',(-13.080976503583,32.3176859273438,24.7779154939672));
#47013=CARTESIAN_POINT('Ctrl Pts',(-13.1594562245957,32.4078297993508,24.7721119546833));
#47014=CARTESIAN_POINT('Ctrl Pts',(-13.2339678289211,32.5014108260291,24.7663084153994));
#47015=CARTESIAN_POINT('Ctrl Pts',(-13.3042099961909,32.5980380308856,24.7605048761156));
#47016=CARTESIAN_POINT('Ctrl Pts',(-13.3744749421764,32.6946965708177,24.7546994548116));
#47017=CARTESIAN_POINT('Ctrl Pts',(-13.4404674576145,32.7944029233995,24.7488940335076));
#47018=CARTESIAN_POINT('Ctrl Pts',(-13.5019293327583,32.896736833307,24.7430886122036));
#47019=CARTESIAN_POINT('Ctrl Pts',(-13.5634592712398,32.9991840685478,24.7372767619329));
#47020=CARTESIAN_POINT('Ctrl Pts',(-13.6204483441698,33.1042643190166,24.7314649116622));
#47021=CARTESIAN_POINT('Ctrl Pts',(-13.6726840601651,33.2115322775602,24.7256530613915));
#47022=CARTESIAN_POINT('Ctrl Pts',(-13.7249540848591,33.3188706902747,24.7198373938663));
#47023=CARTESIAN_POINT('Ctrl Pts',(-13.7724643728939,33.4283992989325,24.7140217263411));
#47024=CARTESIAN_POINT('Ctrl Pts',(-13.815051017427,33.5396538990948,24.7082060588159));
#47025=CARTESIAN_POINT('Ctrl Pts',(-13.8576986627298,33.6510678594582,24.702382060975));
#47026=CARTESIAN_POINT('Ctrl Pts',(-13.8954084592957,33.7642123598829,24.6965580631341));
#47027=CARTESIAN_POINT('Ctrl Pts',(-13.928066613758,33.8786090432503,24.6907340652932));
#47028=CARTESIAN_POINT('Ctrl Pts',(-13.936731000161,33.90895910694,24.6891889269185));
#47029=CARTESIAN_POINT('Ctrl Pts',(-13.9450400971673,33.9393972602586,24.6876437885439));
#47030=CARTESIAN_POINT('Ctrl Pts',(-13.9529923889216,33.9699144826142,24.6860986501693));
#47031=CARTESIAN_POINT('Ctrl Pts',(-13.9915465443551,34.1178675218693,24.6786075385625));
#47032=CARTESIAN_POINT('Ctrl Pts',(-14.0218101378451,34.2680627700932,24.6711164269557));
#47033=CARTESIAN_POINT('Ctrl Pts',(-14.0435706506767,34.4196885379504,24.6636253153489));
#47034=CARTESIAN_POINT('Ctrl Pts',(-14.0649246235171,34.5684815629024,24.6562741561629));
#47035=CARTESIAN_POINT('Ctrl Pts',(-14.0780902876873,34.7186523616395,24.6489229969768));
#47036=CARTESIAN_POINT('Ctrl Pts',(-14.0829121862387,34.8694125600844,24.6415718377907));
#47037=CARTESIAN_POINT('Ctrl Pts',(-14.084264918109,34.911706715187,24.6395095490036));
#47038=CARTESIAN_POINT('Ctrl Pts',(-14.0849612552969,34.9540471161242,24.6374472602165));
#47039=CARTESIAN_POINT('Ctrl Pts',(-14.0849984277889,34.9964160131029,24.6353849714293));
#47040=CARTESIAN_POINT('Ctrl Pts',(-14.0849984277894,34.9964160136128,24.6353849714045));
#47041=CARTESIAN_POINT('Ctrl Pts',(-14.0851020062225,35.1144738661964,24.6296385535608));
#47042=CARTESIAN_POINT('Ctrl Pts',(-14.0800834836686,35.2326545958956,24.6238921357172));
#47043=CARTESIAN_POINT('Ctrl Pts',(-14.0699376947858,35.3504741938599,24.6181457178735));
#47044=CARTESIAN_POINT('Ctrl Pts',(-14.0597976023172,35.4682276413016,24.6124025263907));
#47045=CARTESIAN_POINT('Ctrl Pts',(-14.0445360024406,35.5856199446743,24.606659334908));
#47046=CARTESIAN_POINT('Ctrl Pts',(-14.024199795063,35.7021687898326,24.6009161434252));
#47047=CARTESIAN_POINT('Ctrl Pts',(-14.003869129897,35.8186858720201,24.5951745171302));
#47048=CARTESIAN_POINT('Ctrl Pts',(-13.9784666777729,35.934359541358,24.5894328908351));
#47049=CARTESIAN_POINT('Ctrl Pts',(-13.9480909112641,36.0487150024645,24.5836912645401));
#47050=CARTESIAN_POINT('Ctrl Pts',(-13.9177158689797,36.1630677370876,24.577949775138));
#47051=CARTESIAN_POINT('Ctrl Pts',(-13.8823678558293,36.276101922028,24.5722082857358));
#47052=CARTESIAN_POINT('Ctrl Pts',(-13.842195744884,36.3873560674878,24.5664667963337));
#47053=CARTESIAN_POINT('Ctrl Pts',(-13.8020146008845,36.4986352294257,24.5607240159069));
#47054=CARTESIAN_POINT('Ctrl Pts',(-13.7570073454804,36.6081331633929,24.5549812354801));
#47055=CARTESIAN_POINT('Ctrl Pts',(-13.7073714148722,36.7154072962969,24.5492384550533));
#47056=CARTESIAN_POINT('Ctrl Pts',(-13.657683486109,36.8227938086187,24.5434896585413));
#47057=CARTESIAN_POINT('Ctrl Pts',(-13.6033573785645,36.9279514897564,24.5377408620293));
#47058=CARTESIAN_POINT('Ctrl Pts',(-13.5446370465652,37.03046132889,24.5319920655174));
#47059=CARTESIAN_POINT('Ctrl Pts',(-13.4858820406439,37.1330316993258,24.5262398743836));
#47060=CARTESIAN_POINT('Ctrl Pts',(-13.4227278681908,37.2329507627263,24.5204876832497));
#47061=CARTESIAN_POINT('Ctrl Pts',(-13.355461467923,37.3298290360634,24.5147354921159));
#47062=CARTESIAN_POINT('Ctrl Pts',(-13.288094569961,37.4268520479781,24.5089747070638));
#47063=CARTESIAN_POINT('Ctrl Pts',(-13.2166034327953,37.5208248695699,24.5032139220118));
#47064=CARTESIAN_POINT('Ctrl Pts',(-13.141314941821,37.6113914751128,24.4974531369597));
#47065=CARTESIAN_POINT('Ctrl Pts',(-13.1045735045831,37.6555887649024,24.4946418238401));
#47066=CARTESIAN_POINT('Ctrl Pts',(-13.0669282755439,37.6989754169976,24.4918305107205));
#47067=CARTESIAN_POINT('Ctrl Pts',(-13.0284202510578,37.7415134110529,24.4890191976008));
#47068=CARTESIAN_POINT('Ctrl Pts',(-12.9486514461779,37.8296302384692,24.4831956039294));
#47069=CARTESIAN_POINT('Ctrl Pts',(-12.8649049617742,37.9144047658744,24.477372010258));
#47070=CARTESIAN_POINT('Ctrl Pts',(-12.7774917727232,37.9954573027261,24.4715484165866));
#47071=CARTESIAN_POINT('Ctrl Pts',(-12.6901888683943,38.0764075797631,24.4657321702437));
#47072=CARTESIAN_POINT('Ctrl Pts',(-12.5992287573944,38.1536449309788,24.4599159239007));
#47073=CARTESIAN_POINT('Ctrl Pts',(-12.5049615082202,38.2268239558946,24.4540996775578));
#47074=CARTESIAN_POINT('Ctrl Pts',(-12.4107886210825,38.2999297282026,24.4482892533095));
#47075=CARTESIAN_POINT('Ctrl Pts',(-12.3133155022275,38.3689850069095,24.4424788290612));
#47076=CARTESIAN_POINT('Ctrl Pts',(-12.2129273337961,38.433682806454,24.4366684048129));
#47077=CARTESIAN_POINT('Ctrl Pts',(-12.1087392655496,38.5008295515304,24.4306380439888));
#47078=CARTESIAN_POINT('Ctrl Pts',(-12.0014114347734,38.5632821155977,24.4246076831646));
#47079=CARTESIAN_POINT('Ctrl Pts',(-11.8914104071374,38.6207446294612,24.4185773223404));
#47080=CARTESIAN_POINT('Ctrl Pts',(-11.7855405846603,38.6760490777246,24.4127734381072));
#47081=CARTESIAN_POINT('Ctrl Pts',(-11.6771951282994,38.7267313236942,24.406969553874));
#47082=CARTESIAN_POINT('Ctrl Pts',(-11.5668168564609,38.7725733840854,24.4011656696409));
#47083=CARTESIAN_POINT('Ctrl Pts',(-11.4564548886736,38.8184086731141,24.3953626427035));
#47084=CARTESIAN_POINT('Ctrl Pts',(-11.3440610795531,38.8594050417916,24.3895596157661));
#47085=CARTESIAN_POINT('Ctrl Pts',(-11.2300989151574,38.8953923626419,24.3837565888287));
#47086=CARTESIAN_POINT('Ctrl Pts',(-11.1161266890942,38.9313828607963,24.3779530495447));
#47087=CARTESIAN_POINT('Ctrl Pts',(-11.0005862218483,38.9623633088637,24.3721495102607));
#47088=CARTESIAN_POINT('Ctrl Pts',(-10.8839562508837,38.9882134279052,24.3663459709767));
#47089=CARTESIAN_POINT('Ctrl Pts',(-10.7672884581794,39.014071929839,24.3605405496725));
#47090=CARTESIAN_POINT('Ctrl Pts',(-10.6495308575529,39.0347967056966,24.3547351283684));
#47091=CARTESIAN_POINT('Ctrl Pts',(-10.531171830717,39.0503186894679,24.3489297070643));
#47092=CARTESIAN_POINT('Ctrl Pts',(-10.4126817322146,39.0658578623994,24.3431178567934));
#47093=CARTESIAN_POINT('Ctrl Pts',(-10.2935892831723,39.0761826894489,24.3373060065226));
#47094=CARTESIAN_POINT('Ctrl Pts',(-10.1743875930832,39.0812760219542,24.3314941562517));
#47095=CARTESIAN_POINT('Ctrl Pts',(-10.0551076106835,39.0863726997878,24.3256784887264));
#47096=CARTESIAN_POINT('Ctrl Pts',(-9.93571865174297,39.0862310405332,24.319862821201));
#47097=CARTESIAN_POINT('Ctrl Pts',(-9.81671176650951,39.0808859851096,24.3140471536757));
#47098=CARTESIAN_POINT('Ctrl Pts',(-9.69753441676378,39.0755332734713,24.3082231558346));
#47099=CARTESIAN_POINT('Ctrl Pts',(-9.57874063835108,39.064962325341,24.3023991579936));
#47100=CARTESIAN_POINT('Ctrl Pts',(-9.46081446167668,39.0492596798999,24.2965751601525));
#47101=CARTESIAN_POINT('Ctrl Pts',(-9.4295280041992,39.0450936824706,24.2950300217791));
#47102=CARTESIAN_POINT('Ctrl Pts',(-9.39830254646565,39.0405667565594,24.2934848834058));
#47103=CARTESIAN_POINT('Ctrl Pts',(-9.36714696466197,39.035681111741,24.2919397450324));
#47104=CARTESIAN_POINT('Ctrl Pts',(-9.24972281423343,39.0172673104611,24.2861161798706));
#47105=CARTESIAN_POINT('Ctrl Pts',(-9.1329136420351,38.9936946162266,24.2802926147089));
#47106=CARTESIAN_POINT('Ctrl Pts',(-9.01720746822139,38.9650149860348,24.2744690495471));
#47107=CARTESIAN_POINT('Ctrl Pts',(-8.90164192703478,38.9363702138941,24.2686525625147));
#47108=CARTESIAN_POINT('Ctrl Pts',(-8.78717711116186,38.9026309465696,24.2628360754823));
#47109=CARTESIAN_POINT('Ctrl Pts',(-8.67429385793938,38.8639006489431,24.2570195884499));
#47110=CARTESIAN_POINT('Ctrl Pts',(-8.56153930383042,38.8252145080434,24.2512097328416));
#47111=CARTESIAN_POINT('Ctrl Pts',(-8.45036310699467,38.7815487958191,24.2453998772333));
#47112=CARTESIAN_POINT('Ctrl Pts',(-8.34123302696642,38.7330573434081,24.239590021625));
#47113=CARTESIAN_POINT('Ctrl Pts',(-8.23217569907244,38.6845982180755,24.2337840391871));
#47114=CARTESIAN_POINT('Ctrl Pts',(-8.12516214703689,38.6313199156194,24.2279780567491));
#47115=CARTESIAN_POINT('Ctrl Pts',(-8.02064187898784,38.5734250277266,24.2221720743112));
#47116=CARTESIAN_POINT('Ctrl Pts',(-7.91616129548763,38.5155521215275,24.216368296305));
#47117=CARTESIAN_POINT('Ctrl Pts',(-7.81417247075485,38.4530663117817,24.2105645182988));
#47118=CARTESIAN_POINT('Ctrl Pts',(-7.71510143288208,38.3862166997968,24.2047607402926));
#47119=CARTESIAN_POINT('Ctrl Pts',(-7.6462217291788,38.3397391260772,24.2007256305571));
#47120=CARTESIAN_POINT('Ctrl Pts',(-7.57875194927019,38.2911531563236,24.1966905208216));
#47121=CARTESIAN_POINT('Ctrl Pts',(-7.51282733495086,38.2405550657615,24.1926554110861));
#47122=CARTESIAN_POINT('',(-14.084998667809,35.0032990905415,24.7396150285614));
#47123=CARTESIAN_POINT('Ctrl Pts',(-14.084998667809,35.0032990905415,24.7396150285614));
#47124=CARTESIAN_POINT('Ctrl Pts',(-14.0848838734084,35.145439770813,24.7327077308575));
#47125=CARTESIAN_POINT('Ctrl Pts',(-14.0773464015934,35.2872683007845,24.7258004331536));
#47126=CARTESIAN_POINT('Ctrl Pts',(-14.0625068059482,35.4280928072564,24.7188931354498));
#47127=CARTESIAN_POINT('Ctrl Pts',(-14.0474942948949,35.5705582430094,24.7119053518465));
#47128=CARTESIAN_POINT('Ctrl Pts',(-14.0250085659473,35.7119960749589,24.7049175682433));
#47129=CARTESIAN_POINT('Ctrl Pts',(-13.9952238380689,35.8517109155848,24.6979297846401));
#47130=CARTESIAN_POINT('Ctrl Pts',(-13.9681220732688,35.9788404554339,24.6915714499774));
#47131=CARTESIAN_POINT('Ctrl Pts',(-13.9349776994647,36.1045436836478,24.6852131153147));
#47132=CARTESIAN_POINT('Ctrl Pts',(-13.8959562242754,36.2283118897615,24.6788547806521));
#47133=CARTESIAN_POINT('Ctrl Pts',(-13.8602164861204,36.341671091508,24.673031186981));
#47134=CARTESIAN_POINT('Ctrl Pts',(-13.8194674520747,36.4536519397332,24.66720759331));
#47135=CARTESIAN_POINT('Ctrl Pts',(-13.7738333631693,36.5637796350606,24.661383999639));
#47136=CARTESIAN_POINT('Ctrl Pts',(-13.7282568484454,36.6737683879422,24.6555677532964));
#47137=CARTESIAN_POINT('Ctrl Pts',(-13.677807692304,36.7819082643004,24.6497515069538));
#47138=CARTESIAN_POINT('Ctrl Pts',(-13.6226599695283,36.8877393212987,24.6439352606112));
#47139=CARTESIAN_POINT('Ctrl Pts',(-13.5675674499273,36.9934644408251,24.6381248363633));
#47140=CARTESIAN_POINT('Ctrl Pts',(-13.5077859079211,37.0968849786803,24.6323144121154));
#47141=CARTESIAN_POINT('Ctrl Pts',(-13.4435373555386,37.1975612576241,24.6265039878675));
#47142=CARTESIAN_POINT('Ctrl Pts',(-13.3768568625528,37.3020483419707,24.6204736270431));
#47143=CARTESIAN_POINT('Ctrl Pts',(-13.3053646778811,37.4035788967282,24.6144432662188));
#47144=CARTESIAN_POINT('Ctrl Pts',(-13.2293614153235,37.5016893990301,24.6084129053945));
#47145=CARTESIAN_POINT('Ctrl Pts',(-13.1562125358369,37.596115257444,24.6026090211617));
#47146=CARTESIAN_POINT('Ctrl Pts',(-13.0788855771601,37.6873729663277,24.5968051369289));
#47147=CARTESIAN_POINT('Ctrl Pts',(-12.9976920602387,37.7750796947082,24.5910012526961));
#47148=CARTESIAN_POINT('Ctrl Pts',(-12.9165105364681,37.862773467867,24.585198225759));
#47149=CARTESIAN_POINT('Ctrl Pts',(-12.8314638675764,37.9469170040542,24.579395198822));
#47150=CARTESIAN_POINT('Ctrl Pts',(-12.7429023208599,38.0271623442131,24.573592171885));
#47151=CARTESIAN_POINT('Ctrl Pts',(-12.6543329550849,38.1074147691964,24.5677886326014));
#47152=CARTESIAN_POINT('Ctrl Pts',(-12.5622483970906,38.1837680396641,24.5619850933177));
#47153=CARTESIAN_POINT('Ctrl Pts',(-12.4670335692749,38.2559131389014,24.5561815540341));
#47154=CARTESIAN_POINT('Ctrl Pts',(-12.3717878644008,38.3280816339531,24.5503761327304));
#47155=CARTESIAN_POINT('Ctrl Pts',(-12.2734101961747,38.3960389972939,24.5445707114266));
#47156=CARTESIAN_POINT('Ctrl Pts',(-12.1723156152314,38.4595187335555,24.5387652901229));
#47157=CARTESIAN_POINT('Ctrl Pts',(-12.071109081397,38.5230687677495,24.5329534398524));
#47158=CARTESIAN_POINT('Ctrl Pts',(-11.9671799751829,38.5821310598852,24.5271415895819));
#47159=CARTESIAN_POINT('Ctrl Pts',(-11.8609693010198,38.63648432702,24.5213297393114));
#47160=CARTESIAN_POINT('Ctrl Pts',(-11.7546888671159,38.6908732936724,24.5155140717865));
#47161=CARTESIAN_POINT('Ctrl Pts',(-11.6461242513323,38.7405469062056,24.5096984042615));
#47162=CARTESIAN_POINT('Ctrl Pts',(-11.5357363154178,38.7853320818004,24.5038827367366));
#47163=CARTESIAN_POINT('Ctrl Pts',(-11.4251902607046,38.8301814073233,24.4980587388959));
#47164=CARTESIAN_POINT('Ctrl Pts',(-11.3128160564156,38.8701281836955,24.4922347410552));
#47165=CARTESIAN_POINT('Ctrl Pts',(-11.1990897082746,38.9050491509724,24.4864107432145));
#47166=CARTESIAN_POINT('Ctrl Pts',(-11.168917488128,38.9143138739643,24.4848656048375));
#47167=CARTESIAN_POINT('Ctrl Pts',(-11.1386501479591,38.9232251248635,24.4833204664606));
#47168=CARTESIAN_POINT('Ctrl Pts',(-11.1082966765157,38.9317812091753,24.4817753280836));
#47169=CARTESIAN_POINT('Ctrl Pts',(-10.993890353726,38.9640302435378,24.4759514933952));
#47170=CARTESIAN_POINT('Ctrl Pts',(-10.8778908004984,38.9913336744909,24.4701276587067));
#47171=CARTESIAN_POINT('Ctrl Pts',(-10.7607632878954,39.0135351275142,24.4643038240182));
#47172=CARTESIAN_POINT('Ctrl Pts',(-10.643784722252,39.0357083477265,24.4584873952966));
#47173=CARTESIAN_POINT('Ctrl Pts',(-10.5256814480422,39.0527924196243,24.4526709665749));
#47174=CARTESIAN_POINT('Ctrl Pts',(-10.406933615581,39.0646808032747,24.4468545378532));
#47175=CARTESIAN_POINT('Ctrl Pts',(-10.2883058386793,39.076557167619,24.4410439896145));
#47176=CARTESIAN_POINT('Ctrl Pts',(-10.1690352040094,39.0832482538052,24.4352334413758));
#47177=CARTESIAN_POINT('Ctrl Pts',(-10.0496111758125,39.0846987320039,24.4294228931371));
#47178=CARTESIAN_POINT('Ctrl Pts',(-9.93027871603207,39.086148098048,24.4236168001383));
#47179=CARTESIAN_POINT('Ctrl Pts',(-9.81079350372809,39.0823648482954,24.4178107071396));
#47180=CARTESIAN_POINT('Ctrl Pts',(-9.69164860839685,39.073345605187,24.4120046141408));
#47181=CARTESIAN_POINT('Ctrl Pts',(-9.5725522194164,39.064330033999,24.4062008849226));
#47182=CARTESIAN_POINT('Ctrl Pts',(-9.45379627835535,39.0500827395527,24.4003971557043));
#47183=CARTESIAN_POINT('Ctrl Pts',(-9.33587187472176,39.0306524078881,24.3945934264861));
#47184=CARTESIAN_POINT('Ctrl Pts',(-9.21796765035945,39.0112254011498,24.3887906904043));
#47185=CARTESIAN_POINT('Ctrl Pts',(-9.10089508299161,38.9866171882742,24.3829879543226));
#47186=CARTESIAN_POINT('Ctrl Pts',(-8.98513753636281,38.956927997816,24.3771852182408));
#47187=CARTESIAN_POINT('Ctrl Pts',(-8.86937247998411,38.927236881277,24.3713821057076));
#47188=CARTESIAN_POINT('Ctrl Pts',(-8.75492300913772,38.8924642342029,24.3655789931744));
#47189=CARTESIAN_POINT('Ctrl Pts',(-8.64225911211109,38.8527606571593,24.3597758806412));
#47190=CARTESIAN_POINT('Ctrl Pts',(-8.52950544821218,38.8130254456168,24.3539681443795));
#47191=CARTESIAN_POINT('Ctrl Pts',(-8.41854058513476,38.7683515933072,24.3481604081179));
#47192=CARTESIAN_POINT('Ctrl Pts',(-8.30981632197193,38.7189385763316,24.3423526718563));
#47193=CARTESIAN_POINT('Ctrl Pts',(-8.20104516969539,38.6695042491857,24.3365424309136));
#47194=CARTESIAN_POINT('Ctrl Pts',(-8.09451690726418,38.6153268687497,24.3307321899709));
#47195=CARTESIAN_POINT('Ctrl Pts',(-7.9906590570246,38.5566520739148,24.3249219490281));
#47196=CARTESIAN_POINT('Ctrl Pts',(-7.88666743955713,38.4979017068952,24.3191042245893));
#47197=CARTESIAN_POINT('Ctrl Pts',(-7.78535345100347,38.4346425708196,24.3132865001504));
#47198=CARTESIAN_POINT('Ctrl Pts',(-7.68711615239853,38.367163985835,24.3074687757115));
#47199=CARTESIAN_POINT('Ctrl Pts',(-7.62787443402184,38.3264712206136,24.3039604138398));
#47200=CARTESIAN_POINT('Ctrl Pts',(-7.56975099729801,38.2842447961043,24.3004520519682));
#47201=CARTESIAN_POINT('Ctrl Pts',(-7.51282733495087,38.2405550657615,24.2969436900965));
#47202=CARTESIAN_POINT('Ctrl Pts',(-7.51282733495086,38.2405550657615,25.5469376052728));
#47203=CARTESIAN_POINT('Ctrl Pts',(-7.41802255720225,38.1677910339992,25.5411329091515));
#47204=CARTESIAN_POINT('Ctrl Pts',(-7.3264425387479,38.0908854305494,25.5353282130303));
#47205=CARTESIAN_POINT('Ctrl Pts',(-7.23845601126725,38.0101660748693,25.529523516909));
#47206=CARTESIAN_POINT('Ctrl Pts',(-7.15037508265753,37.9293601150404,25.5237125929039));
#47207=CARTESIAN_POINT('Ctrl Pts',(-7.06589564461184,37.8447325091728,25.5179016688989));
#47208=CARTESIAN_POINT('Ctrl Pts',(-6.98534998547147,37.7566483798089,25.5120907448938));
#47209=CARTESIAN_POINT('Ctrl Pts',(-6.90475667042894,37.6685121343075,25.5062763827789));
#47210=CARTESIAN_POINT('Ctrl Pts',(-6.82810203213645,37.5769156044792,25.5004620206639));
#47211=CARTESIAN_POINT('Ctrl Pts',(-6.75567734419892,37.4822561320411,25.494647658549));
#47212=CARTESIAN_POINT('Ctrl Pts',(-6.68314285103467,37.3874531435573,25.4888244811065));
#47213=CARTESIAN_POINT('Ctrl Pts',(-6.61485134901944,37.2895782729125,25.483001303664));
#47214=CARTESIAN_POINT('Ctrl Pts',(-6.55105035391789,37.1890571803382,25.4771781262214));
#47215=CARTESIAN_POINT('Ctrl Pts',(-6.51450884287949,37.1314845263686,25.4738429477896));
#47216=CARTESIAN_POINT('Ctrl Pts',(-6.47943952189608,37.0730442819452,25.4705077693577));
#47217=CARTESIAN_POINT('Ctrl Pts',(-6.44588189144363,37.013819622119,25.4671725909258));
#47218=CARTESIAN_POINT('Ctrl Pts',(-6.38728652428229,36.9104067577203,25.4613489972415));
#47219=CARTESIAN_POINT('Ctrl Pts',(-6.33311386295598,36.8042676180022,25.4555254035571));
#47220=CARTESIAN_POINT('Ctrl Pts',(-6.28362667865849,36.6958167166357,25.4497018098728));
#47221=CARTESIAN_POINT('Ctrl Pts',(-6.23420192979309,36.5875026421868,25.4438855635167));
#47222=CARTESIAN_POINT('Ctrl Pts',(-6.18945106829059,36.4768829754139,25.4380693171607));
#47223=CARTESIAN_POINT('Ctrl Pts',(-6.14959202974776,36.364398571759,25.4322530708046));
#47224=CARTESIAN_POINT('Ctrl Pts',(-6.10977289032142,36.2520267656099,25.4264426465431));
#47225=CARTESIAN_POINT('Ctrl Pts',(-6.07483596799513,36.1377943186469,25.4206322222815));
#47226=CARTESIAN_POINT('Ctrl Pts',(-6.04495169710269,36.0221633537498,25.41482179802));
#47227=CARTESIAN_POINT('Ctrl Pts',(-6.01393624484118,35.9021555180351,25.4087914372007));
#47228=CARTESIAN_POINT('Ctrl Pts',(-5.98836369439253,35.7806416066818,25.4027610763815));
#47229=CARTESIAN_POINT('Ctrl Pts',(-5.96836835913579,35.6581575133526,25.3967307155622));
#47230=CARTESIAN_POINT('Ctrl Pts',(-5.94912396982272,35.5402734395715,25.3909268313155));
#47231=CARTESIAN_POINT('Ctrl Pts',(-5.93504550560123,35.4214911813111,25.3851229470688));
#47232=CARTESIAN_POINT('Ctrl Pts',(-5.92620079771532,35.3022996186976,25.379319062822));
#47233=CARTESIAN_POINT('Ctrl Pts',(-5.91735739628723,35.1831256619508,25.373516035871));
#47234=CARTESIAN_POINT('Ctrl Pts',(-5.91374624398912,35.0635429281912,25.36771300892));
#47235=CARTESIAN_POINT('Ctrl Pts',(-5.9153832462466,34.9440448844426,25.3619099819689));
#47236=CARTESIAN_POINT('Ctrl Pts',(-5.91702039303428,34.8245362902649,25.3561064426712));
#47237=CARTESIAN_POINT('Ctrl Pts',(-5.9239066100501,34.7051128092835,25.3503029033735));
#47238=CARTESIAN_POINT('Ctrl Pts',(-5.93600568662888,34.5862667273627,25.3444993640758));
#47239=CARTESIAN_POINT('Ctrl Pts',(-5.94810868679719,34.4673821050426,25.338693942758));
#47240=CARTESIAN_POINT('Ctrl Pts',(-5.96542786715539,34.349075660197,25.3328885214401));
#47241=CARTESIAN_POINT('Ctrl Pts',(-5.98787536717668,34.2318327456261,25.3270831001222));
#47242=CARTESIAN_POINT('Ctrl Pts',(-6.0103477257265,34.1144599953793,25.3212712498376));
#47243=CARTESIAN_POINT('Ctrl Pts',(-6.03795966315626,33.9981535276099,25.315459399553));
#47244=CARTESIAN_POINT('Ctrl Pts',(-6.0705725448776,33.8833868732053,25.3096475492684));
#47245=CARTESIAN_POINT('Ctrl Pts',(-6.10320684691488,33.7685448394454,25.3038318817293));
#47246=CARTESIAN_POINT('Ctrl Pts',(-6.14084850625437,33.6552450198145,25.2980162141902));
#47247=CARTESIAN_POINT('Ctrl Pts',(-6.18331008294142,33.543942625779,25.292200546651));
#47248=CARTESIAN_POINT('Ctrl Pts',(-6.22583248125123,33.4324808030847,25.2863765487963));
#47249=CARTESIAN_POINT('Ctrl Pts',(-6.27318841537602,33.3230224900152,25.2805525509415));
#47250=CARTESIAN_POINT('Ctrl Pts',(-6.32514366485763,33.2160000235247,25.2747285530867));
#47251=CARTESIAN_POINT('Ctrl Pts',(-6.33892767455449,33.1876063822544,25.2731834148436));
#47252=CARTESIAN_POINT('Ctrl Pts',(-6.35303517530403,33.1593840413966,25.2716382766005));
#47253=CARTESIAN_POINT('Ctrl Pts',(-6.36746128086535,33.1313407335772,25.2700931383574));
#47254=CARTESIAN_POINT('Ctrl Pts',(-6.42183297051189,33.0256460938884,25.2642695446884));
#47255=CARTESIAN_POINT('Ctrl Pts',(-6.48090920439752,32.9221560328926,25.2584459510193));
#47256=CARTESIAN_POINT('Ctrl Pts',(-6.54448733684888,32.8213175461297,25.2526223573503));
#47257=CARTESIAN_POINT('Ctrl Pts',(-6.60798525604231,32.7206062820963,25.2468061110097));
#47258=CARTESIAN_POINT('Ctrl Pts',(-6.67597356092362,32.6225402808324,25.2409898646691));
#47259=CARTESIAN_POINT('Ctrl Pts',(-6.74820299708105,32.5275434782777,25.2351736183285));
#47260=CARTESIAN_POINT('Ctrl Pts',(-6.82036013117396,32.4326417680469,25.2293631940827));
#47261=CARTESIAN_POINT('Ctrl Pts',(-6.89674970512732,32.3408034677767,25.2235527698368));
#47262=CARTESIAN_POINT('Ctrl Pts',(-6.97707863859544,32.2524244427561,25.2177423455909));
#47263=CARTESIAN_POINT('Ctrl Pts',(-7.0604481883922,32.1607000887864,25.2117119847658));
#47264=CARTESIAN_POINT('Ctrl Pts',(-7.14806097693785,32.0727024450321,25.2056816239407));
#47265=CARTESIAN_POINT('Ctrl Pts',(-7.23954242393711,31.9888376047186,25.1996512631157));
#47266=CARTESIAN_POINT('Ctrl Pts',(-7.32758818820413,31.908122397398,25.1938473788848));
#47267=CARTESIAN_POINT('Ctrl Pts',(-7.41921694001576,31.8312354687225,25.188043494654));
#47268=CARTESIAN_POINT('Ctrl Pts',(-7.51405697676075,31.7585015370653,25.1822396104232));
#47269=CARTESIAN_POINT('Ctrl Pts',(-7.60888300461805,31.6857783489877,25.1764365834882));
#47270=CARTESIAN_POINT('Ctrl Pts',(-7.70691905016106,31.6172071864138,25.1706335565532));
#47271=CARTESIAN_POINT('Ctrl Pts',(-7.80776111058734,31.5530718528309,25.1648305296181));
#47272=CARTESIAN_POINT('Ctrl Pts',(-7.90861207431313,31.4889308567686,25.1590269903365));
#47273=CARTESIAN_POINT('Ctrl Pts',(-8.01226920092046,31.4292266875141,25.1532234510548));
#47274=CARTESIAN_POINT('Ctrl Pts',(-8.11830090735156,31.3741989126917,25.1474199117732));
#47275=CARTESIAN_POINT('Ctrl Pts',(-8.22436699862915,31.3191532930033,25.1416144904714));
#47276=CARTESIAN_POINT('Ctrl Pts',(-8.33280883893436,31.2687872717215,25.1358090691696));
#47277=CARTESIAN_POINT('Ctrl Pts',(-8.44317233125128,31.2232934175636,25.1300036478679));
#47278=CARTESIAN_POINT('Ctrl Pts',(-8.55365804092114,31.1777491831729,25.1241917975993));
#47279=CARTESIAN_POINT('Ctrl Pts',(-8.66606927263243,31.1370880414473,25.1183799473308));
#47280=CARTESIAN_POINT('Ctrl Pts',(-8.77993398438469,31.101453614802,25.1125680970622));
#47281=CARTESIAN_POINT('Ctrl Pts',(-8.89387348309082,31.0657957832739,25.1067524295392));
#47282=CARTESIAN_POINT('Ctrl Pts',(-9.00926796928695,31.0351713464946,25.1009367620162));
#47283=CARTESIAN_POINT('Ctrl Pts',(-9.12563396948364,31.0096730654395,25.0951210944932));
#47284=CARTESIAN_POINT('Ctrl Pts',(-9.24216665141152,30.9841382608499,25.0892970966544));
#47285=CARTESIAN_POINT('Ctrl Pts',(-9.35967322398113,30.9637443371213,25.0834730988156));
#47286=CARTESIAN_POINT('Ctrl Pts',(-9.47766370191699,30.9485323903917,25.0776491009768));
#47287=CARTESIAN_POINT('Ctrl Pts',(-9.50896721933983,30.9444965779447,25.0761039625809));
#47288=CARTESIAN_POINT('Ctrl Pts',(-9.5403047920601,30.9408252247989,25.0745588241849));
#47289=CARTESIAN_POINT('Ctrl Pts',(-9.57166727427056,30.9375184829874,25.0730136857889));
#47290=CARTESIAN_POINT('Ctrl Pts',(-9.68987180102311,30.9250554436048,25.0671900921193));
#47291=CARTESIAN_POINT('Ctrl Pts',(-9.80881134156637,30.9177356190189,25.0613664984498));
#47292=CARTESIAN_POINT('Ctrl Pts',(-9.9280009587515,30.9156345489098,25.0555429047802));
#47293=CARTESIAN_POINT('Ctrl Pts',(-10.0470402005297,30.9135361296127,25.0497266584391));
#47294=CARTESIAN_POINT('Ctrl Pts',(-10.1663284867354,30.9166433760391,25.043910412098));
#47295=CARTESIAN_POINT('Ctrl Pts',(-10.2853746173911,30.9249802052323,25.0380941657569));
#47296=CARTESIAN_POINT('Ctrl Pts',(-10.4043015822122,30.9333086892133,25.0322837415105));
#47297=CARTESIAN_POINT('Ctrl Pts',(-10.5229864687082,30.9468563135307,25.0264733172642));
#47298=CARTESIAN_POINT('Ctrl Pts',(-10.640937530603,30.9655949531728,25.0206628930178));
#47299=CARTESIAN_POINT('Ctrl Pts',(-10.7633532842114,30.9850428890925,25.0146325321929));
#47300=CARTESIAN_POINT('Ctrl Pts',(-10.884978113858,31.0100825942663,25.008602171368));
#47301=CARTESIAN_POINT('Ctrl Pts',(-11.0052670436125,31.0406233860585,25.0025718105431));
#47302=CARTESIAN_POINT('Ctrl Pts',(-11.121038395089,31.0700171860381,24.9967679263119));
#47303=CARTESIAN_POINT('Ctrl Pts',(-11.235571948038,31.1045062163305,24.9909640420807));
#47304=CARTESIAN_POINT('Ctrl Pts',(-11.3483923635487,31.1439575943821,24.9851601578495));
#47305=CARTESIAN_POINT('Ctrl Pts',(-11.4611961142771,31.1834031450431,24.9793571309141));
#47306=CARTESIAN_POINT('Ctrl Pts',(-11.572286845455,31.227809451025,24.9735541039787));
#47307=CARTESIAN_POINT('Ctrl Pts',(-11.6812057324133,31.2769941867759,24.9677510770433));
#47308=CARTESIAN_POINT('Ctrl Pts',(-11.7901342357698,31.3261832650243,24.9619475377614));
#47309=CARTESIAN_POINT('Ctrl Pts',(-11.8968901414889,31.38015144379,24.9561439984794));
#47310=CARTESIAN_POINT('Ctrl Pts',(-12.0010365040093,31.4386690817024,24.9503404591974));
#47311=CARTESIAN_POINT('Ctrl Pts',(-12.1052166399804,31.4972056962023,24.9445350378953));
#47312=CARTESIAN_POINT('Ctrl Pts',(-12.2067851939559,31.5602945040393,24.9387296165933));
#47313=CARTESIAN_POINT('Ctrl Pts',(-12.3053321875728,31.627661270729,24.9329241952912));
#47314=CARTESIAN_POINT('Ctrl Pts',(-12.4039883128633,31.6951026398772,24.9271123450224));
#47315=CARTESIAN_POINT('Ctrl Pts',(-12.4996158613971,31.766831193643,24.9213004947536));
#47316=CARTESIAN_POINT('Ctrl Pts',(-12.5918359552986,31.8425308582947,24.9154886444848));
#47317=CARTESIAN_POINT('Ctrl Pts',(-12.6841166198525,31.9182802428921,24.9096729769616));
#47318=CARTESIAN_POINT('Ctrl Pts',(-12.7729850694209,31.9980056607131,24.9038573094384));
#47319=CARTESIAN_POINT('Ctrl Pts',(-12.858098698843,32.0813535966698,24.8980416419151));
#47320=CARTESIAN_POINT('Ctrl Pts',(-12.9433342443486,32.1648209195448,24.8922176440762));
#47321=CARTESIAN_POINT('Ctrl Pts',(-13.0248039568165,32.2519208200932,24.8863936462372));
#47322=CARTESIAN_POINT('Ctrl Pts',(-13.1022048725415,32.3422660161747,24.8805696483982));
#47323=CARTESIAN_POINT('Ctrl Pts',(-13.122739757652,32.366235089466,24.8790245100056));
#47324=CARTESIAN_POINT('Ctrl Pts',(-13.1429884873942,32.3904324289387,24.8774793716131));
#47325=CARTESIAN_POINT('Ctrl Pts',(-13.1629459212136,32.4148504686424,24.8759342332205));
#47326=CARTESIAN_POINT('Ctrl Pts',(-13.2378042578985,32.5064400915305,24.8701385737653));
#47327=CARTESIAN_POINT('Ctrl Pts',(-13.3088098080701,32.6014415259609,24.8643429143101));
#47328=CARTESIAN_POINT('Ctrl Pts',(-13.3756340199531,32.6994957154278,24.8585472548549));
#47329=CARTESIAN_POINT('Ctrl Pts',(-13.4423779072391,32.7974320409792,24.8527585619467));
#47330=CARTESIAN_POINT('Ctrl Pts',(-13.5049502169777,32.8984134904676,24.8469698690384));
#47331=CARTESIAN_POINT('Ctrl Pts',(-13.5630617794873,33.0020471087743,24.8411811761302));
#47332=CARTESIAN_POINT('Ctrl Pts',(-13.6211175348197,33.1055812030029,24.8353980423671));
#47333=CARTESIAN_POINT('Ctrl Pts',(-13.6747208597774,33.2117620448675,24.829614908604));
#47334=CARTESIAN_POINT('Ctrl Pts',(-13.723625557915,33.3201673582043,24.8238317748409));
#47335=CARTESIAN_POINT('Ctrl Pts',(-13.7724951073978,33.4284947587621,24.8180527975164));
#47336=CARTESIAN_POINT('Ctrl Pts',(-13.8166725773334,33.53904307673,24.8122738201918));
#47337=CARTESIAN_POINT('Ctrl Pts',(-13.8559577878752,33.6513656766476,24.8064948428672));
#47338=CARTESIAN_POINT('Ctrl Pts',(-13.8952293775642,33.763649332403,24.8007178692127));
#47339=CARTESIAN_POINT('Ctrl Pts',(-13.9296119399903,33.8777056600116,24.7949408955582));
#47340=CARTESIAN_POINT('Ctrl Pts',(-13.9589537101833,33.9930687607258,24.7891639219037));
#47341=CARTESIAN_POINT('Ctrl Pts',(-13.9882886312207,34.1084049326007,24.7833882967497));
#47342=CARTESIAN_POINT('Ctrl Pts',(-14.0125850024546,34.2250468704272,24.7776126715957));
#47343=CARTESIAN_POINT('Ctrl Pts',(-14.0317413883321,34.3425151122573,24.7718370464416));
#47344=CARTESIAN_POINT('Ctrl Pts',(-14.0509049499058,34.4600273559376,24.7660592578246));
#47345=CARTESIAN_POINT('Ctrl Pts',(-14.0649246106828,34.5783661150095,24.7602814692076));
#47346=CARTESIAN_POINT('Ctrl Pts',(-14.0737504068469,34.6970435300002,24.7545036805906));
#47347=CARTESIAN_POINT('Ctrl Pts',(-14.0813314046056,34.7989825732682,24.7495407965922));
#47348=CARTESIAN_POINT('Ctrl Pts',(-14.0850811474127,34.9011712045389,24.7445779125939));
#47349=CARTESIAN_POINT('Ctrl Pts',(-14.0849986678096,35.0032990898398,24.7396150285955));
#47350=CARTESIAN_POINT('Origin',(-10.,35.,32.7603849714045));
#47351=CARTESIAN_POINT('',(-7.51282733495086,38.2405550657615,26.7967727135811));
#47352=CARTESIAN_POINT('',(-7.51282733495086,38.2405550657615,26.6927653349501));
#47353=CARTESIAN_POINT('',(-7.51282733495086,38.2405550657615,32.7603849714045));
#47354=CARTESIAN_POINT('',(-14.0849995364304,35.0019461149621,25.8853849714457));
#47355=CARTESIAN_POINT('Ctrl Pts',(-7.51282733495086,38.2405550657615,26.6927653349501));
#47356=CARTESIAN_POINT('Ctrl Pts',(-7.41550399904621,38.1658580043565,26.6867866417674));
#47357=CARTESIAN_POINT('Ctrl Pts',(-7.32165086959052,38.08685124892,26.6808079485846));
#47358=CARTESIAN_POINT('Ctrl Pts',(-7.23165012498627,38.0039081160234,26.6748292554019));
#47359=CARTESIAN_POINT('Ctrl Pts',(-7.14164938038203,37.9209649831269,26.6688505622192));
#47360=CARTESIAN_POINT('Ctrl Pts',(-7.05550130075222,37.8340858473106,26.6628718690364));
#47361=CARTESIAN_POINT('Ctrl Pts',(-6.9735432720381,37.7436808622313,26.6568931758537));
#47362=CARTESIAN_POINT('Ctrl Pts',(-6.89371140427812,37.6556211696432,26.6510695823506));
#47363=CARTESIAN_POINT('Ctrl Pts',(-6.8175973521335,37.5639323246363,26.6452459888476));
#47364=CARTESIAN_POINT('Ctrl Pts',(-6.74554833177251,37.4689611862424,26.6394223953446));
#47365=CARTESIAN_POINT('Ctrl Pts',(-6.67359021199008,37.3741098680955,26.6336061491728));
#47366=CARTESIAN_POINT('Ctrl Pts',(-6.60568716786191,37.2759848155647,26.627789903001));
#47367=CARTESIAN_POINT('Ctrl Pts',(-6.542148441838,37.1749684139584,26.6219736568292));
#47368=CARTESIAN_POINT('Ctrl Pts',(-6.47867331845955,37.0740531303754,26.6161632327546));
#47369=CARTESIAN_POINT('Ctrl Pts',(-6.41955403834108,36.9702525991447,26.6103528086801));
#47370=CARTESIAN_POINT('Ctrl Pts',(-6.36505815740818,36.863980364965,26.6045423846056));
#47371=CARTESIAN_POINT('Ctrl Pts',(-6.30849949237123,36.7536855024396,26.5985120237172));
#47372=CARTESIAN_POINT('Ctrl Pts',(-6.25692142392517,36.6407284785424,26.5924816628289));
#47373=CARTESIAN_POINT('Ctrl Pts',(-6.21057243014792,36.5256027310034,26.5864513019405));
#47374=CARTESIAN_POINT('Ctrl Pts',(-6.16596412379834,36.4148006575079,26.5806474178865));
#47375=CARTESIAN_POINT('Ctrl Pts',(-6.12619937408759,36.3019902331726,26.5748435338324));
#47376=CARTESIAN_POINT('Ctrl Pts',(-6.09145149073612,36.1876335927933,26.5690396497783));
#47377=CARTESIAN_POINT('Ctrl Pts',(-6.05670874002877,36.0732938441461,26.5632366230217));
#47378=CARTESIAN_POINT('Ctrl Pts',(-6.0269815006576,35.95740872425,26.5574335962651));
#47379=CARTESIAN_POINT('Ctrl Pts',(-6.00239342363177,35.84045622169,26.5516305695084));
#47380=CARTESIAN_POINT('Ctrl Pts',(-5.97780317574206,35.7234933934766,26.5458270304067));
#47381=CARTESIAN_POINT('Ctrl Pts',(-5.95835307634472,35.6054633948514,26.5400234913049));
#47382=CARTESIAN_POINT('Ctrl Pts',(-5.94411566815009,35.4868544820112,26.5342199522032));
#47383=CARTESIAN_POINT('Ctrl Pts',(-5.92987364293303,35.3682071057088,26.5284145310826));
#47384=CARTESIAN_POINT('Ctrl Pts',(-5.92084771941127,35.2489808470468,26.5226091099621));
#47385=CARTESIAN_POINT('Ctrl Pts',(-5.91705852649427,35.1296685155574,26.5168036888415));
#47386=CARTESIAN_POINT('Ctrl Pts',(-5.91326513739736,35.0102240567207,26.5109918387552));
#47387=CARTESIAN_POINT('Ctrl Pts',(-5.91472006756182,34.8906937431675,26.5051799886689));
#47388=CARTESIAN_POINT('Ctrl Pts',(-5.92139181533038,34.771569975822,26.4993681385826));
#47389=CARTESIAN_POINT('Ctrl Pts',(-5.92806794513791,34.6523679673605,26.4935524712426));
#47390=CARTESIAN_POINT('Ctrl Pts',(-5.93996767577151,34.5335734422569,26.4877368039026));
#47391=CARTESIAN_POINT('Ctrl Pts',(-5.95700787207372,34.4156716218374,26.4819211365627));
#47392=CARTESIAN_POINT('Ctrl Pts',(-5.97407247661856,34.2976009197813,26.4760971389067));
#47393=CARTESIAN_POINT('Ctrl Pts',(-5.9962921674974,34.1804258743947,26.4702731412508));
#47394=CARTESIAN_POINT('Ctrl Pts',(-6.02353315355834,34.0646196393176,26.4644491435948));
#47395=CARTESIAN_POINT('Ctrl Pts',(-6.03076034396942,34.0338955785284,26.4629040034916));
#47396=CARTESIAN_POINT('Ctrl Pts',(-6.03834070085544,34.003267769391,26.4613588633884));
#47397=CARTESIAN_POINT('Ctrl Pts',(-6.0462711511481,33.9727448273402,26.4598137232852));
#47398=CARTESIAN_POINT('Ctrl Pts',(-6.07616081669262,33.8577046347074,26.453990129517));
#47399=CARTESIAN_POINT('Ctrl Pts',(-6.11112377218076,33.7437845469228,26.4481665357487));
#47400=CARTESIAN_POINT('Ctrl Pts',(-6.1510602459293,33.6314651010902,26.4423429419805));
#47401=CARTESIAN_POINT('Ctrl Pts',(-6.190946333893,33.5192873628972,26.4365266955395));
#47402=CARTESIAN_POINT('Ctrl Pts',(-6.23579332403263,33.4087066313721,26.4307104490985));
#47403=CARTESIAN_POINT('Ctrl Pts',(-6.28545091570393,33.3001911577018,26.4248942026575));
#47404=CARTESIAN_POINT('Ctrl Pts',(-6.33505879986176,33.191784308598,26.4190837783101));
#47405=CARTESIAN_POINT('Ctrl Pts',(-6.38946753689784,33.0854389738162,26.4132733539628));
#47406=CARTESIAN_POINT('Ctrl Pts',(-6.44847791432055,32.981605619575,26.4074629296154));
#47407=CARTESIAN_POINT('Ctrl Pts',(-6.50972195516655,32.8738419606042,26.401432568828));
#47408=CARTESIAN_POINT('Ctrl Pts',(-6.57592273232874,32.7687846290923,26.3954022080405));
#47409=CARTESIAN_POINT('Ctrl Pts',(-6.64680375535941,32.6669119294531,26.3893718472531));
#47410=CARTESIAN_POINT('Ctrl Pts',(-6.71502276806236,32.5688651646968,26.3835679629188));
#47411=CARTESIAN_POINT('Ctrl Pts',(-6.78757656909231,32.4737685065685,26.3777640785846));
#47412=CARTESIAN_POINT('Ctrl Pts',(-6.86417364427234,32.3820202317963,26.3719601942504));
#47413=CARTESIAN_POINT('Ctrl Pts',(-6.94075940525276,32.2902855092165,26.3661571672114));
#47414=CARTESIAN_POINT('Ctrl Pts',(-7.02138699104981,32.2018984997788,26.3603541401724));
#47415=CARTESIAN_POINT('Ctrl Pts',(-7.10572440673968,32.1172246375658,26.3545511131333));
#47416=CARTESIAN_POINT('Ctrl Pts',(-7.19006926854778,32.0325432995298,26.3487475737473));
#47417=CARTESIAN_POINT('Ctrl Pts',(-7.2781243232996,31.9515760498547,26.3429440343612));
#47418=CARTESIAN_POINT('Ctrl Pts',(-7.36952097283118,31.8746512054452,26.3371404949752));
#47419=CARTESIAN_POINT('Ctrl Pts',(-7.46094726123517,31.7977014152018,26.3313350735686));
#47420=CARTESIAN_POINT('Ctrl Pts',(-7.55571698728567,31.724796900126,26.3255296521621));
#47421=CARTESIAN_POINT('Ctrl Pts',(-7.65342928728698,31.6562250538893,26.3197242307556));
#47422=CARTESIAN_POINT('Ctrl Pts',(-7.75124979461412,31.5875772706814,26.3139123803824));
#47423=CARTESIAN_POINT('Ctrl Pts',(-7.85201904595084,31.523271968293,26.3081005300091));
#47424=CARTESIAN_POINT('Ctrl Pts',(-7.95530794327248,31.4635527159089,26.3022886796359));
#47425=CARTESIAN_POINT('Ctrl Pts',(-8.05866468129722,31.4037942395987,26.2964730120081));
#47426=CARTESIAN_POINT('Ctrl Pts',(-8.16454399981762,31.3486280002973,26.2906573443803));
#47427=CARTESIAN_POINT('Ctrl Pts',(-8.27249450201417,31.2982504468253,26.2848416767525));
#47428=CARTESIAN_POINT('Ctrl Pts',(-8.38059963163431,31.2478007329545,26.2790176788095));
#47429=CARTESIAN_POINT('Ctrl Pts',(-8.49078149049063,31.202153551386,26.2731936808666));
#47430=CARTESIAN_POINT('Ctrl Pts',(-8.60257100705781,31.1614563686621,26.2673696829236));
#47431=CARTESIAN_POINT('Ctrl Pts',(-8.63222935600017,31.1506591912231,26.2658245455214));
#47432=CARTESIAN_POINT('Ctrl Pts',(-8.66200079543199,31.1402101524658,26.2642794081191));
#47433=CARTESIAN_POINT('Ctrl Pts',(-8.69187643515535,31.1301114048208,26.2627342707168));
#47434=CARTESIAN_POINT('Ctrl Pts',(-8.80447715651746,31.0920494158489,26.2569106770561));
#47435=CARTESIAN_POINT('Ctrl Pts',(-8.9189220472593,31.0588445806593,26.2510870833955));
#47436=CARTESIAN_POINT('Ctrl Pts',(-9.0347545088317,31.0306768660414,26.2452634897348));
#47437=CARTESIAN_POINT('Ctrl Pts',(-9.15044083054925,31.0025446891792,26.2394472434025));
#47438=CARTESIAN_POINT('Ctrl Pts',(-9.26751084786546,30.9794370884277,26.2336309970703));
#47439=CARTESIAN_POINT('Ctrl Pts',(-9.38549053967956,30.9614850349198,26.227814750738));
#47440=CARTESIAN_POINT('Ctrl Pts',(-9.50335213317253,30.9435509515163,26.2220043265003));
#47441=CARTESIAN_POINT('Ctrl Pts',(-9.62212118828901,30.9307622097943,26.2161939022626));
#47442=CARTESIAN_POINT('Ctrl Pts',(-9.74131174706777,30.9231991233573,26.210383478025));
#47443=CARTESIAN_POINT('Ctrl Pts',(-9.86501391533451,30.9153497584358,26.2043531171968));
#47444=CARTESIAN_POINT('Ctrl Pts',(-9.98916969179079,30.9131295749646,26.1983227563686));
#47445=CARTESIAN_POINT('Ctrl Pts',(-10.1132274744092,30.9165695133823,26.1922923955404));
#47446=CARTESIAN_POINT('Ctrl Pts',(-10.2326261352478,30.9198802612593,26.1864885113176));
#47447=CARTESIAN_POINT('Ctrl Pts',(-10.3519335851551,30.9284336418294,26.1806846270947));
#47448=CARTESIAN_POINT('Ctrl Pts',(-10.4706569195293,30.942204161851,26.1748807428719));
#47449=CARTESIAN_POINT('Ctrl Pts',(-10.5893627171996,30.9559726478198,26.1690777159447));
#47450=CARTESIAN_POINT('Ctrl Pts',(-10.7074841654126,30.9749566936718,26.1632746890175));
#47451=CARTESIAN_POINT('Ctrl Pts',(-10.8245336381355,30.9990789460947,26.1574716620903));
#47452=CARTESIAN_POINT('Ctrl Pts',(-10.9415934451055,31.0232033282607,26.1516681228164));
#47453=CARTESIAN_POINT('Ctrl Pts',(-11.0575806884576,31.0524667365388,26.1458645835425));
#47454=CARTESIAN_POINT('Ctrl Pts',(-11.1720187213321,31.0867408574377,26.1400610442686));
#47455=CARTESIAN_POINT('Ctrl Pts',(-11.2864938651288,31.1210260930353,26.1342556229745));
#47456=CARTESIAN_POINT('Ctrl Pts',(-11.3994184083371,31.1603251557496,26.1284502016803));
#47457=CARTESIAN_POINT('Ctrl Pts',(-11.5103322443192,31.2044603135035,26.1226447803862));
#47458=CARTESIAN_POINT('Ctrl Pts',(-11.6213689071137,31.2486443468616,26.116832930125));
#47459=CARTESIAN_POINT('Ctrl Pts',(-11.730390038426,31.2976750142891,26.1110210798638));
#47460=CARTESIAN_POINT('Ctrl Pts',(-11.8369567081233,31.3513269463433,26.1052092296027));
#47461=CARTESIAN_POINT('Ctrl Pts',(-11.9435933713841,31.4050141172758,26.0993935620869));
#47462=CARTESIAN_POINT('Ctrl Pts',(-12.0477720069898,31.4633283986657,26.0935778945711));
#47463=CARTESIAN_POINT('Ctrl Pts',(-12.1490808715335,31.5259999413344,26.0877622270554));
#47464=CARTESIAN_POINT('Ctrl Pts',(-12.2505348500914,31.5887612542238,26.0819382292236));
#47465=CARTESIAN_POINT('Ctrl Pts',(-12.3491105166702,31.6558920566716,26.0761142313918));
#47466=CARTESIAN_POINT('Ctrl Pts',(-12.4444274065974,31.7270808665848,26.07029023356));
#47467=CARTESIAN_POINT('Ctrl Pts',(-12.4697154986905,31.7459676471171,26.0687450950895));
#47468=CARTESIAN_POINT('Ctrl Pts',(-12.4947744094078,31.7651398506132,26.0671999566189));
#47469=CARTESIAN_POINT('Ctrl Pts',(-12.5195974652219,31.7845912214389,26.0656548181484));
#47470=CARTESIAN_POINT('Ctrl Pts',(-12.6121091278205,31.8570834507757,26.0598963277382));
#47471=CARTESIAN_POINT('Ctrl Pts',(-12.7016553977115,31.9337015217862,26.054137837328));
#47472=CARTESIAN_POINT('Ctrl Pts',(-12.7878402403027,32.014171506173,26.0483793469178));
#47473=CARTESIAN_POINT('Ctrl Pts',(-12.8739158143967,32.0945394675823,26.0426281573459));
#47474=CARTESIAN_POINT('Ctrl Pts',(-12.9566381307581,32.1787493506631,26.0368769677739));
#47475=CARTESIAN_POINT('Ctrl Pts',(-13.0356421573526,32.2664854687594,26.031125778202));
#47476=CARTESIAN_POINT('Ctrl Pts',(-13.1145677909222,32.3541345292716,26.025380295341));
#47477=CARTESIAN_POINT('Ctrl Pts',(-13.1897821930166,32.4453025579342,26.0196348124801));
#47478=CARTESIAN_POINT('Ctrl Pts',(-13.260955868785,32.5396358355242,26.0138893296191));
#47479=CARTESIAN_POINT('Ctrl Pts',(-13.3320794864054,32.6339027662645,26.0081478876936));
#47480=CARTESIAN_POINT('Ctrl Pts',(-13.3991677787573,32.7313301853019,26.0024064457681));
#47481=CARTESIAN_POINT('Ctrl Pts',(-13.4619308537017,32.8315305480159,25.9966650038427));
#47482=CARTESIAN_POINT('Ctrl Pts',(-13.5246713353043,32.931694840779,25.9909256287114));
#47483=CARTESIAN_POINT('Ctrl Pts',(-13.5830894723143,33.0346297389846,25.9851862535801));
#47484=CARTESIAN_POINT('Ctrl Pts',(-13.6369384953871,33.139918447817,25.9794468784488));
#47485=CARTESIAN_POINT('Ctrl Pts',(-13.6907815551914,33.2451954969237,25.9737081388989));
#47486=CARTESIAN_POINT('Ctrl Pts',(-13.7400563170462,33.3528254656153,25.967969399349));
#47487=CARTESIAN_POINT('Ctrl Pts',(-13.784562181292,33.4623673728961,25.962230659799));
#47488=CARTESIAN_POINT('Ctrl Pts',(-13.8290742097634,33.5719244521334,25.9564911254126));
#47489=CARTESIAN_POINT('Ctrl Pts',(-13.8688158713915,33.6833936081926,25.9507515910262));
#47490=CARTESIAN_POINT('Ctrl Pts',(-13.903635172702,33.7963150584794,25.9450120566397));
#47491=CARTESIAN_POINT('Ctrl Pts',(-13.9384862376441,33.9093395204637,25.9392672864086));
#47492=CARTESIAN_POINT('Ctrl Pts',(-13.9684058548559,34.0238185210516,25.9335225161774));
#47493=CARTESIAN_POINT('Ctrl Pts',(-13.9932922830984,34.1392783598938,25.9277777459462));
#47494=CARTESIAN_POINT('Ctrl Pts',(-14.0181915929126,34.2547979624027,25.9220300021397));
#47495=CARTESIAN_POINT('Ctrl Pts',(-14.0380524566273,34.3712990019251,25.9162822583331));
#47496=CARTESIAN_POINT('Ctrl Pts',(-14.0528247789693,34.4883005657883,25.9105345145266));
#47497=CARTESIAN_POINT('Ctrl Pts',(-14.0676173085825,34.6054621777655,25.904778908299));
#47498=CARTESIAN_POINT('Ctrl Pts',(-14.0773073680087,34.7231252646438,25.8990233020715));
#47499=CARTESIAN_POINT('Ctrl Pts',(-14.0818969247286,34.8408067341535,25.8932676958439));
#47500=CARTESIAN_POINT('Ctrl Pts',(-14.0839921694519,34.8945311988609,25.8906401210445));
#47501=CARTESIAN_POINT('Ctrl Pts',(-14.0850251129975,34.948259530738,25.8880125462451));
#47502=CARTESIAN_POINT('Ctrl Pts',(-14.0849995364304,35.0019461149621,25.8853849714457));
#47503=CARTESIAN_POINT('Ctrl Pts',(-14.08499953643,35.0019461158033,25.8853849714045));
#47504=CARTESIAN_POINT('Ctrl Pts',(-14.0849449953633,35.1164306865273,25.879781769463));
#47505=CARTESIAN_POINT('Ctrl Pts',(-14.080078085778,35.2307950929958,25.8741785675215));
#47506=CARTESIAN_POINT('Ctrl Pts',(-14.0704266820106,35.3447486423126,25.8685753655799));
#47507=CARTESIAN_POINT('Ctrl Pts',(-14.0603956578548,35.4631843469393,25.8627517718956));
#47508=CARTESIAN_POINT('Ctrl Pts',(-14.0451750474133,35.5813728710574,25.8569281782112));
#47509=CARTESIAN_POINT('Ctrl Pts',(-14.0247820306547,35.6988237300772,25.8511045845269));
#47510=CARTESIAN_POINT('Ctrl Pts',(-14.0044147427152,35.8161264073961,25.8452883381708));
#47511=CARTESIAN_POINT('Ctrl Pts',(-13.9788880972782,35.9326928719345,25.8394720918147));
#47512=CARTESIAN_POINT('Ctrl Pts',(-13.9482711523926,36.048036214634,25.8336558454586));
#47513=CARTESIAN_POINT('Ctrl Pts',(-13.9176848552369,36.1632640980144,25.827845421197));
#47514=CARTESIAN_POINT('Ctrl Pts',(-13.8820184994948,36.2772709028511,25.8220349969355));
#47515=CARTESIAN_POINT('Ctrl Pts',(-13.8413923561535,36.3895789887896,25.8162245726739));
#47516=CARTESIAN_POINT('Ctrl Pts',(-13.7992284293876,36.5061381677141,25.8101942118546));
#47517=CARTESIAN_POINT('Ctrl Pts',(-13.7517218964731,36.6208670451566,25.8041638510354));
#47518=CARTESIAN_POINT('Ctrl Pts',(-13.6990644946204,36.733247490879,25.7981334902161));
#47519=CARTESIAN_POINT('Ctrl Pts',(-13.6483846971346,36.841407370216,25.7923296059694));
#47520=CARTESIAN_POINT('Ctrl Pts',(-13.5929341350882,36.9473916294299,25.7865257217226));
#47521=CARTESIAN_POINT('Ctrl Pts',(-13.5329328695572,37.0507584790028,25.7807218374759));
#47522=CARTESIAN_POINT('Ctrl Pts',(-13.472940466854,37.154110060188,25.7749188105248));
#47523=CARTESIAN_POINT('Ctrl Pts',(-13.4083989023735,37.2548446475391,25.7691157835738));
#47524=CARTESIAN_POINT('Ctrl Pts',(-13.3395736832524,37.3525459855501,25.7633127566227));
#47525=CARTESIAN_POINT('Ctrl Pts',(-13.2707423875834,37.4502559495688,25.757509217325));
#47526=CARTESIAN_POINT('Ctrl Pts',(-13.1976269204893,37.5449317979474,25.7517056780273));
#47527=CARTESIAN_POINT('Ctrl Pts',(-13.1205351352935,37.6361876771957,25.7459021387296));
#47528=CARTESIAN_POINT('Ctrl Pts',(-13.0434183501301,37.7274731496623,25.7400967174117));
#47529=CARTESIAN_POINT('Ctrl Pts',(-12.9623229457708,37.8153361355679,25.7342912960938));
#47530=CARTESIAN_POINT('Ctrl Pts',(-12.8775954891384,37.8994256674194,25.7284858747759));
#47531=CARTESIAN_POINT('Ctrl Pts',(-12.7927742046902,37.983608320644,25.7226740244913));
#47532=CARTESIAN_POINT('Ctrl Pts',(-12.7043131293883,38.0640088908545,25.7168621742066));
#47533=CARTESIAN_POINT('Ctrl Pts',(-12.6125940604571,38.1403148369653,25.711050323922));
#47534=CARTESIAN_POINT('Ctrl Pts',(-12.5208147499488,38.2166709012313,25.7052346563829));
#47535=CARTESIAN_POINT('Ctrl Pts',(-12.4257735085254,38.2889267388844,25.6994189888437));
#47536=CARTESIAN_POINT('Ctrl Pts',(-12.3278820700889,38.3568124862373,25.6936033213046));
#47537=CARTESIAN_POINT('Ctrl Pts',(-12.2298504127388,38.4247954725918,25.6877793234498));
#47538=CARTESIAN_POINT('Ctrl Pts',(-12.1289607539321,38.488395657677,25.681955325595));
#47539=CARTESIAN_POINT('Ctrl Pts',(-12.0256505210465,38.5473884713383,25.6761313277402));
#47540=CARTESIAN_POINT('Ctrl Pts',(-11.9982417555052,38.5630395850093,25.6745861894973));
#47541=CARTESIAN_POINT('Ctrl Pts',(-11.9706627263306,38.5783666607387,25.6730410512544));
#47542=CARTESIAN_POINT('Ctrl Pts',(-11.942921832498,38.5933660755346,25.6714959130115));
#47543=CARTESIAN_POINT('Ctrl Pts',(-11.8383669847759,38.6498985556834,25.6656723193424));
#47544=CARTESIAN_POINT('Ctrl Pts',(-11.7311741295247,38.7019551202848,25.6598487256734));
#47545=CARTESIAN_POINT('Ctrl Pts',(-11.6217629113322,38.7492812723811,25.6540251320044));
#47546=CARTESIAN_POINT('Ctrl Pts',(-11.5124897316433,38.7965477155066,25.6482088856638));
#47547=CARTESIAN_POINT('Ctrl Pts',(-11.4010041272243,38.8390954558911,25.6423926393232));
#47548=CARTESIAN_POINT('Ctrl Pts',(-11.287751189866,38.8767153458822,25.6365763929827));
#47549=CARTESIAN_POINT('Ctrl Pts',(-11.1746116193231,38.9142975781558,25.6307659687368));
#47550=CARTESIAN_POINT('Ctrl Pts',(-11.0597086205557,38.9469616452577,25.6249555444909));
#47551=CARTESIAN_POINT('Ctrl Pts',(-10.9435076063458,38.9745463133253,25.619145120245));
#47552=CARTESIAN_POINT('Ctrl Pts',(-10.8229081433339,39.0031751181505,25.6131147594199));
#47553=CARTESIAN_POINT('Ctrl Pts',(-10.7009108695603,39.026332216735,25.6070843985948));
#47554=CARTESIAN_POINT('Ctrl Pts',(-10.5780542375637,39.0438939524219,25.6010540377697));
#47555=CARTESIAN_POINT('Ctrl Pts',(-10.4598116166367,39.0607961385059,25.5952501535389));
#47556=CARTESIAN_POINT('Ctrl Pts',(-10.3407734622352,39.0725155990886,25.5894462693081));
#47557=CARTESIAN_POINT('Ctrl Pts',(-10.2214299038287,39.078994213981,25.5836423850773));
#47558=CARTESIAN_POINT('Ctrl Pts',(-10.1021039737419,39.0854718719127,25.5778393581423));
#47559=CARTESIAN_POINT('Ctrl Pts',(-9.98247313698898,39.0867102015237,25.5720363312073));
#47560=CARTESIAN_POINT('Ctrl Pts',(-9.86303107900381,39.0827030892144,25.5662333042722));
#47561=CARTESIAN_POINT('Ctrl Pts',(-9.74357847553385,39.0786956231191,25.5604297649906));
#47562=CARTESIAN_POINT('Ctrl Pts',(-9.62431509209752,39.0694418080057,25.554626225709));
#47563=CARTESIAN_POINT('Ctrl Pts',(-9.50573239939709,39.0549876126807,25.5488226864273));
#47564=CARTESIAN_POINT('Ctrl Pts',(-9.38711125171189,39.0405287300287,25.5430172651256));
#47565=CARTESIAN_POINT('Ctrl Pts',(-9.26917163889313,39.0208661626327,25.5372118438238));
#47566=CARTESIAN_POINT('Ctrl Pts',(-9.15239707538665,38.9960973814694,25.5314064225221));
#47567=CARTESIAN_POINT('Ctrl Pts',(-9.03549319485917,38.9713011711736,25.5255945722535));
#47568=CARTESIAN_POINT('Ctrl Pts',(-8.91975733864937,38.9413875447034,25.519782721985));
#47569=CARTESIAN_POINT('Ctrl Pts',(-8.80566019443292,38.9065045026005,25.5139708717165));
#47570=CARTESIAN_POINT('Ctrl Pts',(-8.69148811059923,38.8715985491282,25.5081552041935));
#47571=CARTESIAN_POINT('Ctrl Pts',(-8.57895726626273,38.8317168158974,25.5023395366704));
#47572=CARTESIAN_POINT('Ctrl Pts',(-8.46851906515115,38.7870557358183,25.4965238691474));
#47573=CARTESIAN_POINT('Ctrl Pts',(-8.357922673241,38.7423306835643,25.4906998713086));
#47574=CARTESIAN_POINT('Ctrl Pts',(-8.24942527753198,38.6928127893603,25.4848758734699));
#47575=CARTESIAN_POINT('Ctrl Pts',(-8.14345448377524,38.6387448036632,25.4790518756311));
#47576=CARTESIAN_POINT('Ctrl Pts',(-8.11533985413041,38.6244002721217,25.477506737235));
#47577=CARTESIAN_POINT('Ctrl Pts',(-8.0874029081827,38.6097357111295,25.475961598839));
#47578=CARTESIAN_POINT('Ctrl Pts',(-8.0596512801125,38.5947561593564,25.474416460443));
#47579=CARTESIAN_POINT('Ctrl Pts',(-7.95507361048059,38.5383080615151,25.4685938480793));
#47580=CARTESIAN_POINT('Ctrl Pts',(-7.85279263304946,38.477201648066,25.4627712357156));
#47581=CARTESIAN_POINT('Ctrl Pts',(-7.75325101345552,38.4116482807378,25.4569486233519));
#47582=CARTESIAN_POINT('Ctrl Pts',(-7.67116832542903,38.3575925337906,25.4521472580929));
#47583=CARTESIAN_POINT('Ctrl Pts',(-7.59094813059903,38.3005139010736,25.4473458928338));
#47584=CARTESIAN_POINT('Ctrl Pts',(-7.51282733495087,38.2405550657615,25.4425445275748));
#47585=CARTESIAN_POINT('',(-14.0849990113761,34.997157983738,25.9896150286377));
#47586=CARTESIAN_POINT('Ctrl Pts',(-14.0849990113767,34.9971579846073,25.9896150285955));
#47587=CARTESIAN_POINT('Ctrl Pts',(-14.0850823687406,35.1169725184056,25.9837992556083));
#47588=CARTESIAN_POINT('Ctrl Pts',(-14.0798901022421,35.2368329720402,25.9779834826211));
#47589=CARTESIAN_POINT('Ctrl Pts',(-14.0694367788927,35.3562433193698,25.9721677096339));
#47590=CARTESIAN_POINT('Ctrl Pts',(-14.0589841763782,35.4756454324611,25.9663523376878));
#47591=CARTESIAN_POINT('Ctrl Pts',(-14.0432712735987,35.5945970970668,25.9605369657417));
#47592=CARTESIAN_POINT('Ctrl Pts',(-14.0223646062367,35.7126064653753,25.9547215937957));
#47593=CARTESIAN_POINT('Ctrl Pts',(-14.0014545368501,35.8306350366852,25.9489052755468));
#47594=CARTESIAN_POINT('Ctrl Pts',(-13.9753490922683,35.9477206074002,25.9430889572979));
#47595=CARTESIAN_POINT('Ctrl Pts',(-13.9441660016536,36.0633811881917,25.937272639049));
#47596=CARTESIAN_POINT('Ctrl Pts',(-13.9129706122599,36.1790873861394,25.9314540268129));
#47597=CARTESIAN_POINT('Ctrl Pts',(-13.8766936982003,36.2933670848564,25.9256354145768));
#47598=CARTESIAN_POINT('Ctrl Pts',(-13.8355027712538,36.4057537094756,25.9198168023407));
#47599=CARTESIAN_POINT('Ctrl Pts',(-13.7942616422284,36.5182773070305,25.9139910985809));
#47600=CARTESIAN_POINT('Ctrl Pts',(-13.7480946838436,36.6289028436099,25.9081653948212));
#47601=CARTESIAN_POINT('Ctrl Pts',(-13.6972175586699,36.7371837334787,25.9023396910615));
#47602=CARTESIAN_POINT('Ctrl Pts',(-13.6463043683703,36.8455413801202,25.8965098576514));
#47603=CARTESIAN_POINT('Ctrl Pts',(-13.5906745491849,36.9515507116461,25.8906800242413));
#47604=CARTESIAN_POINT('Ctrl Pts',(-13.5305888844153,37.0547912617206,25.8848501908312));
#47605=CARTESIAN_POINT('Ctrl Pts',(-13.4704104787615,37.1581911612827,25.8790113592032));
#47606=CARTESIAN_POINT('Ctrl Pts',(-13.4057627161401,37.2588134079781,25.8731725275752));
#47607=CARTESIAN_POINT('Ctrl Pts',(-13.3369488313703,37.3562677048282,25.8673336959472));
#47608=CARTESIAN_POINT('Ctrl Pts',(-13.3133690744641,37.3896613816549,25.8653329626524));
#47609=CARTESIAN_POINT('Ctrl Pts',(-13.2893004869571,37.4226833896288,25.8633322293576));
#47610=CARTESIAN_POINT('Ctrl Pts',(-13.2647562933781,37.4553189904467,25.8613314960627));
#47611=CARTESIAN_POINT('Ctrl Pts',(-13.1933147821562,37.5503124003773,25.8555079024021));
#47612=CARTESIAN_POINT('Ctrl Pts',(-13.1176086426081,37.6423383452609,25.8496843087414));
#47613=CARTESIAN_POINT('Ctrl Pts',(-13.0379131029223,37.7309904758334,25.8438607150807));
#47614=CARTESIAN_POINT('Ctrl Pts',(-12.958318110997,37.8195307585757,25.8380444687484));
#47615=CARTESIAN_POINT('Ctrl Pts',(-12.8747440004759,37.9047053922272,25.8322282224161));
#47616=CARTESIAN_POINT('Ctrl Pts',(-12.7875080441765,37.986138627668,25.8264119760838));
#47617=CARTESIAN_POINT('Ctrl Pts',(-12.7003594115499,38.0674903479917,25.8206015518461));
#47618=CARTESIAN_POINT('Ctrl Pts',(-12.6095565220376,38.1451078435993,25.8147911276084));
#47619=CARTESIAN_POINT('Ctrl Pts',(-12.5154551039352,38.21865043459,25.8089807033707));
#47620=CARTESIAN_POINT('Ctrl Pts',(-12.4177917522782,38.2949767649528,25.8029503425425));
#47621=CARTESIAN_POINT('Ctrl Pts',(-12.3165755254885,38.3669132749912,25.7969199817143));
#47622=CARTESIAN_POINT('Ctrl Pts',(-12.2122442084511,38.4341229684119,25.7908896208861));
#47623=CARTESIAN_POINT('Ctrl Pts',(-12.1118311648279,38.4988085304176,25.7850857366633));
#47624=CARTESIAN_POINT('Ctrl Pts',(-12.0085331665974,38.5591156733134,25.7792818524404));
#47625=CARTESIAN_POINT('Ctrl Pts',(-11.9027714188067,38.6147871206715,25.7734779682176));
#47626=CARTESIAN_POINT('Ctrl Pts',(-11.7970252931551,38.6704503447625,25.7676749412904));
#47627=CARTESIAN_POINT('Ctrl Pts',(-11.6888165029063,38.7214790449011,25.7618719143631));
#47628=CARTESIAN_POINT('Ctrl Pts',(-11.5785911791359,38.7676617270071,25.7560688874359));
#47629=CARTESIAN_POINT('Ctrl Pts',(-11.4683561236196,38.813848486562,25.750265348162));
#47630=CARTESIAN_POINT('Ctrl Pts',(-11.3561045572319,38.8551882196057,25.7444618088881));
#47631=CARTESIAN_POINT('Ctrl Pts',(-11.2423023240607,38.8915176905204,25.7386582696141));
#47632=CARTESIAN_POINT('Ctrl Pts',(-11.1284631861493,38.9278589426599,25.7328528483199));
#47633=CARTESIAN_POINT('Ctrl Pts',(-11.0130727701695,38.9591865772534,25.7270474270257));
#47634=CARTESIAN_POINT('Ctrl Pts',(-10.8966111730493,38.9853874848455,25.7212420057315));
#47635=CARTESIAN_POINT('Ctrl Pts',(-10.7800206054849,39.0116174075187,25.7154301554704));
#47636=CARTESIAN_POINT('Ctrl Pts',(-10.6623568875714,39.0327091809837,25.7096183052092));
#47637=CARTESIAN_POINT('Ctrl Pts',(-10.5441095368408,39.0486009697078,25.703806454948));
#47638=CARTESIAN_POINT('Ctrl Pts',(-10.4257845206125,39.0645031962444,25.6979907874322));
#47639=CARTESIAN_POINT('Ctrl Pts',(-10.3068755139097,39.0751985997321,25.6921751199164));
#47640=CARTESIAN_POINT('Ctrl Pts',(-10.1878747114908,39.0806774061156,25.6863594524006));
#47641=CARTESIAN_POINT('Ctrl Pts',(-10.0687034532662,39.0861640602979,25.6805354545688));
#47642=CARTESIAN_POINT('Ctrl Pts',(-9.94944054377033,39.0864192023761,25.674711456737));
#47643=CARTESIAN_POINT('Ctrl Pts',(-9.83057587027134,39.0814850807354,25.6688874589052));
#47644=CARTESIAN_POINT('Ctrl Pts',(-9.79904042244212,39.0801760312844,25.6673423204349));
#47645=CARTESIAN_POINT('Ctrl Pts',(-9.76753296247365,39.0785020064223,25.6657971819646));
#47646=CARTESIAN_POINT('Ctrl Pts',(-9.73606253046936,39.0764644009457,25.6642520434943));
#47647=CARTESIAN_POINT('Ctrl Pts',(-9.61746471748885,39.0687855882367,25.6584291160142));
#47648=CARTESIAN_POINT('Ctrl Pts',(-9.49901105976693,39.0559144963217,25.652606188534));
#47649=CARTESIAN_POINT('Ctrl Pts',(-9.38119211768221,39.0378585667135,25.6467832610539));
#47650=CARTESIAN_POINT('Ctrl Pts',(-9.26351389264308,39.0198242022036,25.6409672881868));
#47651=CARTESIAN_POINT('Ctrl Pts',(-9.14646927575777,38.9966173744826,25.6351513153197));
#47652=CARTESIAN_POINT('Ctrl Pts',(-9.03054638182726,38.9682974538474,25.6293353424526));
#47653=CARTESIAN_POINT('Ctrl Pts',(-8.91473456847413,38.9400046701566,25.6235249426143));
#47654=CARTESIAN_POINT('Ctrl Pts',(-8.80004273458407,38.9066086345948,25.617714542776));
#47655=CARTESIAN_POINT('Ctrl Pts',(-8.68695080785641,38.8682201099486,25.6119041429377));
#47656=CARTESIAN_POINT('Ctrl Pts',(-8.57394311497465,38.8298601780868,25.6060980708383));
#47657=CARTESIAN_POINT('Ctrl Pts',(-8.46253334329489,38.7865152875142,25.6002919987388));
#47658=CARTESIAN_POINT('Ctrl Pts',(-8.35318755706752,38.7383463961761,25.5944859266393));
#47659=CARTESIAN_POINT('Ctrl Pts',(-8.24389061310108,38.6901990207797,25.5886824479795));
#47660=CARTESIAN_POINT('Ctrl Pts',(-8.13665619313469,38.6372320964834,25.5828789693196));
#47661=CARTESIAN_POINT('Ctrl Pts',(-8.03193111003031,38.5796549895672,25.5770754906597));
#47662=CARTESIAN_POINT('Ctrl Pts',(-7.92720867012837,38.522079335865,25.5712721584763));
#47663=CARTESIAN_POINT('Ctrl Pts',(-7.82499580309165,38.4598939198369,25.565468826293));
#47664=CARTESIAN_POINT('Ctrl Pts',(-7.72571506549868,38.3933542456838,25.5596654941096));
#47665=CARTESIAN_POINT('Ctrl Pts',(-7.6531341096041,38.3447092288151,25.5554228644974));
#47666=CARTESIAN_POINT('Ctrl Pts',(-7.58211977490954,38.2937380109861,25.5511802348851));
#47667=CARTESIAN_POINT('Ctrl Pts',(-7.51282733495086,38.2405550657615,25.5469376052728));
#47668=CARTESIAN_POINT('Ctrl Pts',(-7.51282733495086,38.2405550657615,26.7967727135811));
#47669=CARTESIAN_POINT('Ctrl Pts',(-7.41816743920586,38.1679022330228,26.7909660918651));
#47670=CARTESIAN_POINT('Ctrl Pts',(-7.3266191318822,38.0910411499093,26.7851594701491));
#47671=CARTESIAN_POINT('Ctrl Pts',(-7.23857267566336,38.0102730993063,26.7793528484331));
#47672=CARTESIAN_POINT('Ctrl Pts',(-7.15056331236747,37.9295390753206,26.7735486729777));
#47673=CARTESIAN_POINT('Ctrl Pts',(-7.06605316749299,37.8449016317536,26.7677444975222));
#47674=CARTESIAN_POINT('Ctrl Pts',(-6.98539889507687,37.7567018660342,26.7619403220667));
#47675=CARTESIAN_POINT('Ctrl Pts',(-6.90475988744046,37.6685187931688,26.7561372451205));
#47676=CARTESIAN_POINT('Ctrl Pts',(-6.82797557649666,37.5767750400944,26.7503341681742));
#47677=CARTESIAN_POINT('Ctrl Pts',(-6.75536479151172,37.4818475706292,26.744531091228));
#47678=CARTESIAN_POINT('Ctrl Pts',(-6.6827506127708,37.3869156643484,26.7387277430516));
#47679=CARTESIAN_POINT('Ctrl Pts',(-6.61431059584699,37.2888000702335,26.7329243948753));
#47680=CARTESIAN_POINT('Ctrl Pts',(-6.55032200867168,37.1879092202706,26.727121046699));
#47681=CARTESIAN_POINT('Ctrl Pts',(-6.48631532947053,37.0869898445979,26.7213160576938));
#47682=CARTESIAN_POINT('Ctrl Pts',(-6.42676280162494,36.9832939972967,26.7155110686885));
#47683=CARTESIAN_POINT('Ctrl Pts',(-6.3718969191612,36.8772567844618,26.7097060796833));
#47684=CARTESIAN_POINT('Ctrl Pts',(-6.31697134521963,36.7711042081688,26.7038947751253));
#47685=CARTESIAN_POINT('Ctrl Pts',(-6.26674278408351,36.6626055438139,26.6980834705674));
#47686=CARTESIAN_POINT('Ctrl Pts',(-6.22139661147764,36.5522182295822,26.6922721660094));
#47687=CARTESIAN_POINT('Ctrl Pts',(-6.17602234506711,36.4417625259041,26.6864572611111));
#47688=CARTESIAN_POINT('Ctrl Pts',(-6.13553663004733,36.3294162253693,26.6806423562128));
#47689=CARTESIAN_POINT('Ctrl Pts',(-6.10007521054347,36.2156527615164,26.6748274513145));
#47690=CARTESIAN_POINT('Ctrl Pts',(-6.06456131784517,36.1017209588761,26.6690039419486));
#47691=CARTESIAN_POINT('Ctrl Pts',(-6.03408666856618,35.9863681999291,26.6631804325827));
#47692=CARTESIAN_POINT('Ctrl Pts',(-6.00873614398522,35.8700792099976,26.6573569232168));
#47693=CARTESIAN_POINT('Ctrl Pts',(-5.99755204410615,35.8187750378067,26.65478771759));
#47694=CARTESIAN_POINT('Ctrl Pts',(-5.98736461721418,35.7672887225753,26.6522185119633));
#47695=CARTESIAN_POINT('Ctrl Pts',(-5.97817793785381,35.7156621412609,26.6496493063365));
#47696=CARTESIAN_POINT('Ctrl Pts',(-5.95735457763845,35.5986406520781,26.643825711963));
#47697=CARTESIAN_POINT('Ctrl Pts',(-5.94160927486657,35.4805208685255,26.6380021175896));
#47698=CARTESIAN_POINT('Ctrl Pts',(-5.93105180597031,35.3617811414413,26.6321785232162));
#47699=CARTESIAN_POINT('Ctrl Pts',(-5.92050765687337,35.2431912219815,26.6263622761633));
#47700=CARTESIAN_POINT('Ctrl Pts',(-5.91513835921745,35.123983317815,26.6205460291104));
#47701=CARTESIAN_POINT('Ctrl Pts',(-5.91500264167174,35.0046456916703,26.6147297820576));
#47702=CARTESIAN_POINT('Ctrl Pts',(-5.91486705997985,34.8854275229902,26.6089193570924));
#47703=CARTESIAN_POINT('Ctrl Pts',(-5.91995463684506,34.7660802966464,26.6031089321272));
#47704=CARTESIAN_POINT('Ctrl Pts',(-5.93027222897837,34.647096514929,26.5972985071621));
#47705=CARTESIAN_POINT('Ctrl Pts',(-5.94098036152084,34.523608971656,26.591268146604));
#47706=CARTESIAN_POINT('Ctrl Pts',(-5.95732230395538,34.4005133772377,26.5852377860459));
#47707=CARTESIAN_POINT('Ctrl Pts',(-5.97924629220264,34.2783597702222,26.5792074254878));
#47708=CARTESIAN_POINT('Ctrl Pts',(-6.00034690542287,34.1607937513929,26.5734035405249));
#47709=CARTESIAN_POINT('Ctrl Pts',(-6.02661776946005,34.0441006796139,26.567599655562));
#47710=CARTESIAN_POINT('Ctrl Pts',(-6.05796008300251,33.9287641283086,26.5617957705992));
#47711=CARTESIAN_POINT('Ctrl Pts',(-6.08929776696935,33.8134446133744,26.5559927429286));
#47712=CARTESIAN_POINT('Ctrl Pts',(-6.12570530365791,33.6994816143779,26.550189715258));
#47713=CARTESIAN_POINT('Ctrl Pts',(-6.16703340111029,33.5873457423007,26.5443866875875));
#47714=CARTESIAN_POINT('Ctrl Pts',(-6.20836514741999,33.4751999697485,26.5385831475676));
#47715=CARTESIAN_POINT('Ctrl Pts',(-6.25461817704179,33.3648820280153,26.5327796075478));
#47716=CARTESIAN_POINT('Ctrl Pts',(-6.30559444831266,33.2568440632973,26.526976067528));
#47717=CARTESIAN_POINT('Ctrl Pts',(-6.35658725060838,33.1487710630965,26.5211706454861));
#47718=CARTESIAN_POINT('Ctrl Pts',(-6.41230616658958,33.0429798794551,26.5153652234443));
#47719=CARTESIAN_POINT('Ctrl Pts',(-6.47250675950058,32.9398989252391,26.5095598014025));
#47720=CARTESIAN_POINT('Ctrl Pts',(-6.53277401897794,32.8367038184386,26.5037479503948));
#47721=CARTESIAN_POINT('Ctrl Pts',(-6.59753265599006,32.7362252847876,26.4979360993872));
#47722=CARTESIAN_POINT('Ctrl Pts',(-6.66649429216926,32.6388636854557,26.4921242483795));
#47723=CARTESIAN_POINT('Ctrl Pts',(-6.73550122271972,32.5414381385049,26.4863085801171));
#47724=CARTESIAN_POINT('Ctrl Pts',(-6.80871640031047,32.4471339247615,26.4804929118546));
#47725=CARTESIAN_POINT('Ctrl Pts',(-6.88581152455996,32.356317882302,26.4746772435922));
#47726=CARTESIAN_POINT('Ctrl Pts',(-6.96301707916817,32.2653717557645,26.4688532450191));
#47727=CARTESIAN_POINT('Ctrl Pts',(-7.04411339642909,32.1779240714469,26.463029246446));
#47728=CARTESIAN_POINT('Ctrl Pts',(-7.12873567982069,32.0943045232397,26.4572052478729));
#47729=CARTESIAN_POINT('Ctrl Pts',(-7.15118632826877,32.0721199046624,26.4556601165046));
#47730=CARTESIAN_POINT('Ctrl Pts',(-7.17388497986136,32.0502045115405,26.4541149851363));
#47731=CARTESIAN_POINT('Ctrl Pts',(-7.196824452785,32.0285640085144,26.452569853768));
#47732=CARTESIAN_POINT('Ctrl Pts',(-7.28328323015379,31.9470010432489,26.4467462601125));
#47733=CARTESIAN_POINT('Ctrl Pts',(-7.37344419471702,31.8690831724474,26.4409226664571));
#47734=CARTESIAN_POINT('Ctrl Pts',(-7.46696744322747,31.795164424447,26.4350990728016));
#47735=CARTESIAN_POINT('Ctrl Pts',(-7.56037269829168,31.7213389359083,26.429282826473));
#47736=CARTESIAN_POINT('Ctrl Pts',(-7.65713148249352,31.6515027857869,26.4234665801445));
#47737=CARTESIAN_POINT('Ctrl Pts',(-7.75686762003372,31.5859727408899,26.417650333816));
#47738=CARTESIAN_POINT('Ctrl Pts',(-7.85650392117553,31.5205082919126,26.4118399095807));
#47739=CARTESIAN_POINT('Ctrl Pts',(-7.95911130732079,31.4593415960198,26.4060294853453));
#47740=CARTESIAN_POINT('Ctrl Pts',(-8.06428162249677,31.4027483597896,26.40021906111));
#47741=CARTESIAN_POINT('Ctrl Pts',(-8.17343285197416,31.3440129523289,26.3941887002804));
#47742=CARTESIAN_POINT('Ctrl Pts',(-8.28534451679734,31.290204353265,26.3881583394508));
#47743=CARTESIAN_POINT('Ctrl Pts',(-8.39952820529889,31.2415807798536,26.3821279786212));
#47744=CARTESIAN_POINT('Ctrl Pts',(-8.50942360410989,31.1947833163823,26.3763240943971));
#47745=CARTESIAN_POINT('Ctrl Pts',(-8.62142303817242,31.1527886180174,26.370520210173));
#47746=CARTESIAN_POINT('Ctrl Pts',(-8.73506790146244,31.1157791275354,26.3647163259489));
#47747=CARTESIAN_POINT('Ctrl Pts',(-8.84869597821914,31.0787751037417,26.3589132990191));
#47748=CARTESIAN_POINT('Ctrl Pts',(-8.96396861269728,31.0467549498376,26.3531102720893));
#47749=CARTESIAN_POINT('Ctrl Pts',(-9.08041036314702,31.019851774143,26.3473072451596));
#47750=CARTESIAN_POINT('Ctrl Pts',(-9.19686239421507,30.9929462231726,26.3415037058817));
#47751=CARTESIAN_POINT('Ctrl Pts',(-9.31448334860745,30.9711586405803,26.3357001666039));
#47752=CARTESIAN_POINT('Ctrl Pts',(-9.43278650517214,30.9545712401174,26.3298966273261));
#47753=CARTESIAN_POINT('Ctrl Pts',(-9.551128026101,30.9379784605498,26.3240912060267));
#47754=CARTESIAN_POINT('Ctrl Pts',(-9.6701517850061,30.92658927357,26.3182857847272));
#47755=CARTESIAN_POINT('Ctrl Pts',(-9.78936547850621,30.9204340796655,26.3124803634278));
#47756=CARTESIAN_POINT('Ctrl Pts',(-9.90871119018325,30.914272069451,26.3066685131594));
#47757=CARTESIAN_POINT('Ctrl Pts',(-10.0282468482665,30.9133556430209,26.3008566628911));
#47758=CARTESIAN_POINT('Ctrl Pts',(-10.1474795238122,30.9176630724478,26.2950448126227));
#47759=CARTESIAN_POINT('Ctrl Pts',(-10.266790512046,30.9219733310185,26.2892291450985));
#47760=CARTESIAN_POINT('Ctrl Pts',(-10.3857977153321,30.9315142459272,26.2834134775744));
#47761=CARTESIAN_POINT('Ctrl Pts',(-10.5040143586819,30.9462123234878,26.2775978100502));
#47762=CARTESIAN_POINT('Ctrl Pts',(-10.6224003346473,30.9609314544622,26.2717738122084));
#47763=CARTESIAN_POINT('Ctrl Pts',(-10.7399930892949,30.9808224244376,26.2659498143666));
#47764=CARTESIAN_POINT('Ctrl Pts',(-10.8563169081083,31.0057608543193,26.2601258165248));
#47765=CARTESIAN_POINT('Ctrl Pts',(-10.8871782526725,31.0123771559962,26.2585806780831));
#47766=CARTESIAN_POINT('Ctrl Pts',(-10.9179503703238,31.0193484631904,26.2570355396413));
#47767=CARTESIAN_POINT('Ctrl Pts',(-10.9486245863916,31.0266718743485,26.2554904011996));
#47768=CARTESIAN_POINT('Ctrl Pts',(-11.0642350460018,31.0542736532507,26.2496668076964));
#47769=CARTESIAN_POINT('Ctrl Pts',(-11.1788262581777,31.0869699424238,26.2438432141931));
#47770=CARTESIAN_POINT('Ctrl Pts',(-11.2919158012722,31.1246705220816,26.2380196206899));
#47771=CARTESIAN_POINT('Ctrl Pts',(-11.4048626650515,31.1623235368387,26.2322033745179));
#47772=CARTESIAN_POINT('Ctrl Pts',(-11.5163112440597,31.2049681563606,26.2263871283459));
#47773=CARTESIAN_POINT('Ctrl Pts',(-11.6257903978218,31.2524633981307,26.2205708821739));
#47774=CARTESIAN_POINT('Ctrl Pts',(-11.7351599622947,31.299911096879,26.2147604580992));
#47775=CARTESIAN_POINT('Ctrl Pts',(-11.8425636509395,31.3521995968757,26.2089500340245));
#47776=CARTESIAN_POINT('Ctrl Pts',(-11.9475471345016,31.4091386605865,26.2031396099497));
#47777=CARTESIAN_POINT('Ctrl Pts',(-12.0565044644739,31.468232988023,26.1971092490615));
#47778=CARTESIAN_POINT('Ctrl Pts',(-12.1628543242716,31.5323367610234,26.1910788881732));
#47779=CARTESIAN_POINT('Ctrl Pts',(-12.2661130188982,31.6011830314681,26.1850485272849));
#47780=CARTESIAN_POINT('Ctrl Pts',(-12.3654937197075,31.6674437045248,26.1792446432306));
#47781=CARTESIAN_POINT('Ctrl Pts',(-12.4620108821194,31.7380968326876,26.1734407591764));
#47782=CARTESIAN_POINT('Ctrl Pts',(-12.5552605251456,31.812858859631,26.1676368751221));
#47783=CARTESIAN_POINT('Ctrl Pts',(-12.6484963941752,31.8876098434018,26.1618338483652));
#47784=CARTESIAN_POINT('Ctrl Pts',(-12.7384653851536,31.9664682636071,26.1560308216084));
#47785=CARTESIAN_POINT('Ctrl Pts',(-12.8247955502742,32.049109439652,26.1502277948515));
#47786=CARTESIAN_POINT('Ctrl Pts',(-12.9111333374235,32.1317579120274,26.1444242557496));
#47787=CARTESIAN_POINT('Ctrl Pts',(-12.9938313649679,32.2181895218882,26.1386207166476));
#47788=CARTESIAN_POINT('Ctrl Pts',(-13.0725540688902,32.3080422563223,26.1328171775457));
#47789=CARTESIAN_POINT('Ctrl Pts',(-13.1513023016507,32.3979241289314,26.1270117564249));
#47790=CARTESIAN_POINT('Ctrl Pts',(-13.2260723780103,32.4912290255449,26.1212063353041));
#47791=CARTESIAN_POINT('Ctrl Pts',(-13.2965690090939,32.5875618622892,26.1154009141833));
#47792=CARTESIAN_POINT('Ctrl Pts',(-13.3671437086616,32.6840013787204,26.1095890640968));
#47793=CARTESIAN_POINT('Ctrl Pts',(-13.4334352752984,32.7834751987622,26.1037772140103));
#47794=CARTESIAN_POINT('Ctrl Pts',(-13.4951916759194,32.8855591404383,26.0979653639237));
#47795=CARTESIAN_POINT('Ctrl Pts',(-13.5569886384688,32.9877101313838,26.0921496965835));
#47796=CARTESIAN_POINT('Ctrl Pts',(-13.6142443074278,33.0924743006253,26.0863340292433));
#47797=CARTESIAN_POINT('Ctrl Pts',(-13.6667533184719,33.1994042370718,26.0805183619031));
#47798=CARTESIAN_POINT('Ctrl Pts',(-13.7193375430087,33.3064873391147,26.0746943642469));
#47799=CARTESIAN_POINT('Ctrl Pts',(-13.7671613758866,33.4157420274988,26.0688703665907));
#47800=CARTESIAN_POINT('Ctrl Pts',(-13.8100680748157,33.5267022482641,26.0630463689346));
#47801=CARTESIAN_POINT('Ctrl Pts',(-13.8214514690128,33.5561406335206,26.0615012288334));
#47802=CARTESIAN_POINT('Ctrl Pts',(-13.8324890351497,33.5856989933228,26.0599560887323));
#47803=CARTESIAN_POINT('Ctrl Pts',(-13.843178444856,33.6153684818718,26.0584109486312));
#47804=CARTESIAN_POINT('Ctrl Pts',(-13.8896767283494,33.7444289564493,26.0516896829642));
#47805=CARTESIAN_POINT('Ctrl Pts',(-13.929706557768,33.8759349285887,26.0449684172972));
#47806=CARTESIAN_POINT('Ctrl Pts',(-13.9630405440442,34.0092756961385,26.0382471516302));
#47807=CARTESIAN_POINT('Ctrl Pts',(-13.9962417189321,34.1420851989211,26.0315526652574));
#47808=CARTESIAN_POINT('Ctrl Pts',(-14.0228002010074,34.2767147718557,26.0248581788846));
#47809=CARTESIAN_POINT('Ctrl Pts',(-14.0425382249071,34.412539618217,26.0181636925118));
#47810=CARTESIAN_POINT('Ctrl Pts',(-14.0621325522726,34.5473756340957,26.0115179432616));
#47811=CARTESIAN_POINT('Ctrl Pts',(-14.0750052824989,34.6833894343958,26.0048721940114));
#47812=CARTESIAN_POINT('Ctrl Pts',(-14.0810301740244,34.8199507881088,25.9982264447612));
#47813=CARTESIAN_POINT('Ctrl Pts',(-14.0836324814579,34.878935190466,25.9953559727201));
#47814=CARTESIAN_POINT('Ctrl Pts',(-14.0849578689422,34.9380215163847,25.9924855006789));
#47815=CARTESIAN_POINT('Ctrl Pts',(-14.0849990113761,34.997157983738,25.9896150286377));
#47816=CARTESIAN_POINT('Origin',(-10.,35.,32.7603849714045));
#47817=CARTESIAN_POINT('',(-7.51282733495085,38.2405550657615,28.0469627484298));
#47818=CARTESIAN_POINT('',(-7.51282733495086,38.2405550657615,27.9426390044296));
#47819=CARTESIAN_POINT('',(-7.51282733495086,38.2405550657615,32.7603849714045));
#47820=CARTESIAN_POINT('',(-14.0849997205636,35.0015109583762,27.1353849713726));
#47821=CARTESIAN_POINT('Ctrl Pts',(-7.51282733495086,38.2405550657615,27.9426390044296));
#47822=CARTESIAN_POINT('Ctrl Pts',(-7.41802037611531,38.1677893599836,27.9368359476833));
#47823=CARTESIAN_POINT('Ctrl Pts',(-7.32640226579339,38.0908542025866,27.9310328909369));
#47824=CARTESIAN_POINT('Ctrl Pts',(-7.2383497970762,38.0100686298972,27.9252298341906));
#47825=CARTESIAN_POINT('Ctrl Pts',(-7.15028244208156,37.9292693994822,27.9194257963712));
#47826=CARTESIAN_POINT('Ctrl Pts',(-7.06578222826958,37.8446187353752,27.9136217585517));
#47827=CARTESIAN_POINT('Ctrl Pts',(-6.98519006760836,37.7564734846453,27.9078177207322));
#47828=CARTESIAN_POINT('Ctrl Pts',(-6.90451482676891,37.6682373674703,27.9020076996944));
#47829=CARTESIAN_POINT('Ctrl Pts',(-6.8277559624221,37.5764997696668,27.8961976786565));
#47830=CARTESIAN_POINT('Ctrl Pts',(-6.75521511451344,37.4816518786724,27.8903876576187));
#47831=CARTESIAN_POINT('Ctrl Pts',(-6.6826367208746,37.3867548962567,27.8845746294271));
#47832=CARTESIAN_POINT('Ctrl Pts',(-6.61428092710793,37.288744748098,27.8787616012355));
#47833=CARTESIAN_POINT('Ctrl Pts',(-6.55040590798919,37.1880414987756,27.872948573044));
#47834=CARTESIAN_POINT('Ctrl Pts',(-6.48642760067838,37.0871754086947,27.8671261449777));
#47835=CARTESIAN_POINT('Ctrl Pts',(-6.42694474983516,36.983607869981,27.8613037169115));
#47836=CARTESIAN_POINT('Ctrl Pts',(-6.37216973770201,36.8777839566774,27.8554812888453));
#47837=CARTESIAN_POINT('Ctrl Pts',(-6.32164660039326,36.7801745560734,27.850110822985));
#47838=CARTESIAN_POINT('Ctrl Pts',(-6.27512835223445,36.6806459641039,27.8447403571246));
#47839=CARTESIAN_POINT('Ctrl Pts',(-6.2327445653037,36.5795605369061,27.8393698912643));
#47840=CARTESIAN_POINT('Ctrl Pts',(-6.18678478552992,36.4699463587314,27.8335463099825));
#47841=CARTESIAN_POINT('Ctrl Pts',(-6.14553895320145,36.3581478393045,27.8277227287006));
#47842=CARTESIAN_POINT('Ctrl Pts',(-6.10921899769923,36.2446076458609,27.8218991474188));
#47843=CARTESIAN_POINT('Ctrl Pts',(-6.07294486646626,36.1312107041455,27.8160829136503));
#47844=CARTESIAN_POINT('Ctrl Pts',(-6.04158437409596,36.0160768445666,27.8102666798818));
#47845=CARTESIAN_POINT('Ctrl Pts',(-6.01530181494215,35.8996695915705,27.8044504461132));
#47846=CARTESIAN_POINT('Ctrl Pts',(-5.98904556559313,35.7833788665002,27.7986400346078));
#47847=CARTESIAN_POINT('Ctrl Pts',(-5.96785722648496,35.6658176799201,27.7928296231025));
#47848=CARTESIAN_POINT('Ctrl Pts',(-5.95185140977864,35.5474650596055,27.7870192115971));
#47849=CARTESIAN_POINT('Ctrl Pts',(-5.93523969038897,35.4246321824225,27.7809888460595));
#47850=CARTESIAN_POINT('Ctrl Pts',(-5.92421075358353,35.3009471947128,27.774958480522));
#47851=CARTESIAN_POINT('Ctrl Pts',(-5.91883462399233,35.1769581127731,27.7689281149844));
#47852=CARTESIAN_POINT('Ctrl Pts',(-5.91366041635228,35.0576259344515,27.7631242438337));
#47853=CARTESIAN_POINT('Ctrl Pts',(-5.91372206606784,34.9380125375034,27.757320372683));
#47854=CARTESIAN_POINT('Ctrl Pts',(-5.91902913849428,34.8186113908173,27.7515165015323));
#47855=CARTESIAN_POINT('Ctrl Pts',(-5.92433542691345,34.6992278831154,27.7457134877804));
#47856=CARTESIAN_POINT('Ctrl Pts',(-5.93488557888585,34.5800569711454,27.7399104740284));
#47857=CARTESIAN_POINT('Ctrl Pts',(-5.95063705580308,34.4615905404203,27.7341074602764));
#47858=CARTESIAN_POINT('Ctrl Pts',(-5.9663899231729,34.3431136521391,27.7283039342668));
#47859=CARTESIAN_POINT('Ctrl Pts',(-5.98734497455411,34.2253417735434,27.7225004082571));
#47860=CARTESIAN_POINT('Ctrl Pts',(-6.01340806027706,34.1087594566358,27.7166968822474));
#47861=CARTESIAN_POINT('Ctrl Pts',(-6.03947959763761,33.9921393348611,27.7108914742926));
#47862=CARTESIAN_POINT('Ctrl Pts',(-6.0706623745295,33.876709940234,27.7050860663377));
#47863=CARTESIAN_POINT('Ctrl Pts',(-6.10681177311979,33.7629428347561,27.6992806583828));
#47864=CARTESIAN_POINT('Ctrl Pts',(-6.14300120363802,33.6490497433214,27.6934688215057));
#47865=CARTESIAN_POINT('Ctrl Pts',(-6.18416811069166,33.536823004872,27.6876569846286));
#47866=CARTESIAN_POINT('Ctrl Pts',(-6.23011885586395,33.4267164403429,27.6818451477515));
#47867=CARTESIAN_POINT('Ctrl Pts',(-6.27609978147261,33.3165375578534,27.6760294936616));
#47868=CARTESIAN_POINT('Ctrl Pts',(-6.32687062936867,33.2084819912689,27.6702138395717));
#47869=CARTESIAN_POINT('Ctrl Pts',(-6.38219146353194,33.1029796012012,27.6643981854818));
#47870=CARTESIAN_POINT('Ctrl Pts',(-6.43759153938857,32.9973260892611,27.6585742010352));
#47871=CARTESIAN_POINT('Ctrl Pts',(-6.49755440533462,32.8942334050838,27.6527502165887));
#47872=CARTESIAN_POINT('Ctrl Pts',(-6.56179637688084,32.794103165157,27.6469262321421));
#47873=CARTESIAN_POINT('Ctrl Pts',(-6.57884155236157,32.7675358374521,27.64538096766));
#47874=CARTESIAN_POINT('Ctrl Pts',(-6.59618775046187,32.7411768833744,27.643835703178));
#47875=CARTESIAN_POINT('Ctrl Pts',(-6.61382920367194,32.715033405475,27.6422904386959));
#47876=CARTESIAN_POINT('Ctrl Pts',(-6.68031409542711,32.6165071515693,27.6364668401181));
#47877=CARTESIAN_POINT('Ctrl Pts',(-6.75120994370549,32.5207261598631,27.6306432415404));
#47878=CARTESIAN_POINT('Ctrl Pts',(-6.82626268247139,32.4281103368678,27.6248196429626));
#47879=CARTESIAN_POINT('Ctrl Pts',(-6.9012207317816,32.3356113615987,27.6190033916635));
#47880=CARTESIAN_POINT('Ctrl Pts',(-6.9803249855821,32.2462699269102,27.6131871403643));
#47881=CARTESIAN_POINT('Ctrl Pts',(-7.06327782186871,32.1604775316135,27.6073708890651));
#47882=CARTESIAN_POINT('Ctrl Pts',(-7.14614762259942,32.0747710142632,27.6015604598171));
#47883=CARTESIAN_POINT('Ctrl Pts',(-7.23285805969597,31.9926067607567,27.5957500305691));
#47884=CARTESIAN_POINT('Ctrl Pts',(-7.32307131084594,31.9143432152645,27.5899396013212));
#47885=CARTESIAN_POINT('Ctrl Pts',(-7.41669921073822,31.8331173276134,27.5839092423548));
#47886=CARTESIAN_POINT('Ctrl Pts',(-7.51410005066375,31.7560936207688,27.5778788833884));
#47887=CARTESIAN_POINT('Ctrl Pts',(-7.61485387219103,31.6836310595777,27.571848524422));
#47888=CARTESIAN_POINT('Ctrl Pts',(-7.7118238918668,31.6138898241789,27.5660446351127));
#47889=CARTESIAN_POINT('Ctrl Pts',(-7.81189923141333,31.5483735852726,27.5602407458035));
#47890=CARTESIAN_POINT('Ctrl Pts',(-7.91467240806616,31.4873608448462,27.5544368564943));
#47891=CARTESIAN_POINT('Ctrl Pts',(-8.01743040437785,31.4263571164427,27.5486338244615));
#47892=CARTESIAN_POINT('Ctrl Pts',(-8.1228850942968,31.3698557720406,27.5428307924287));
#47893=CARTESIAN_POINT('Ctrl Pts',(-8.2306017580057,31.3180908673315,27.5370277603959));
#47894=CARTESIAN_POINT('Ctrl Pts',(-8.33832793221818,31.2663213922032,27.5312242160027));
#47895=CARTESIAN_POINT('Ctrl Pts',(-8.44831610923865,31.2192893651064,27.5254206716094));
#47896=CARTESIAN_POINT('Ctrl Pts',(-8.56010941160991,31.1771816557067,27.5196171272162));
#47897=CARTESIAN_POINT('Ctrl Pts',(-8.67193896737304,31.1350602912198,27.5138117007945));
#47898=CARTESIAN_POINT('Ctrl Pts',(-8.7855744307501,31.0978665641698,27.5080062743729));
#47899=CARTESIAN_POINT('Ctrl Pts',(-8.90054212403392,31.0657380134292,27.5022008479513));
#47900=CARTESIAN_POINT('Ctrl Pts',(-9.0156371330191,31.0335738833979,27.4963889925763));
#47901=CARTESIAN_POINT('Ctrl Pts',(-9.13206692326843,31.006486236081,27.4905771372013));
#47902=CARTESIAN_POINT('Ctrl Pts',(-9.24934578396128,30.9845618859279,27.4847652818263));
#47903=CARTESIAN_POINT('Ctrl Pts',(-9.36670167393422,30.9626231357635,27.4789496091988));
#47904=CARTESIAN_POINT('Ctrl Pts',(-9.484907341612,30.9458544937966,27.4731339365712));
#47905=CARTESIAN_POINT('Ctrl Pts',(-9.60347173726377,30.9342909183205,27.4673182639436));
#47906=CARTESIAN_POINT('Ctrl Pts',(-9.72220596261296,30.9227107793683,27.4614942610419));
#47907=CARTESIAN_POINT('Ctrl Pts',(-9.84129953521717,30.9163506096816,27.4556702581401));
#47908=CARTESIAN_POINT('Ctrl Pts',(-9.96026104661172,30.9151932951994,27.4498462552384));
#47909=CARTESIAN_POINT('Ctrl Pts',(-9.99182116247825,30.9148862632971,27.4483011655347));
#47910=CARTESIAN_POINT('Ctrl Pts',(-10.0233720118736,30.9149451379122,27.4467560758311));
#47911=CARTESIAN_POINT('Ctrl Pts',(-10.0549044960146,30.915368988964,27.4452109861274));
#47912=CARTESIAN_POINT('Ctrl Pts',(-10.1737535104193,30.9169665250009,27.4393873920324));
#47913=CARTESIAN_POINT('Ctrl Pts',(-10.2927243948804,30.9237581020526,27.4335637979374));
#47914=CARTESIAN_POINT('Ctrl Pts',(-10.4113266826636,30.9357614046258,27.4277402038423));
#47915=CARTESIAN_POINT('Ctrl Pts',(-10.529779336445,30.9477495632906,27.4219239570566));
#47916=CARTESIAN_POINT('Ctrl Pts',(-10.647863915818,30.9649363285096,27.4161077102708));
#47917=CARTESIAN_POINT('Ctrl Pts',(-10.7650898375638,30.9872873837693,27.4102914634851));
#47918=CARTESIAN_POINT('Ctrl Pts',(-10.8821984158978,31.0096160655724,27.4044810387755));
#47919=CARTESIAN_POINT('Ctrl Pts',(-10.9984496477042,31.0370986773648,27.3986706140659));
#47920=CARTESIAN_POINT('Ctrl Pts',(-11.1133585593071,31.0696491608996,27.3928601893562));
#47921=CARTESIAN_POINT('Ctrl Pts',(-11.2326169981372,31.1034317439505,27.386829828698));
#47922=CARTESIAN_POINT('Ctrl Pts',(-11.3504290441034,31.142673391791,27.3807994680398));
#47923=CARTESIAN_POINT('Ctrl Pts',(-11.4662642623488,31.1872196348388,27.3747691073816));
#47924=CARTESIAN_POINT('Ctrl Pts',(-11.5777491789926,31.2300929014343,27.3689652226434));
#47925=CARTESIAN_POINT('Ctrl Pts',(-11.6874026581099,31.2778793505669,27.3631613379053));
#47926=CARTESIAN_POINT('Ctrl Pts',(-11.7947684019703,31.3303908405269,27.3573574531672));
#47927=CARTESIAN_POINT('Ctrl Pts',(-11.9021182870467,31.3828945741174,27.3515544257095));
#47928=CARTESIAN_POINT('Ctrl Pts',(-12.0071807421609,31.4401217812231,27.3457513982518));
#47929=CARTESIAN_POINT('Ctrl Pts',(-12.1095217127996,31.5018371759984,27.3399483707941));
#47930=CARTESIAN_POINT('Ctrl Pts',(-12.2118717193363,31.5635580197547,27.334144830975));
#47931=CARTESIAN_POINT('Ctrl Pts',(-12.3114994139579,31.6297676281855,27.3283412911559));
#47932=CARTESIAN_POINT('Ctrl Pts',(-12.4079980611583,31.7001863177661,27.3225377513369));
#47933=CARTESIAN_POINT('Ctrl Pts',(-12.5045280019799,31.7706278434782,27.3167323294833));
#47934=CARTESIAN_POINT('Ctrl Pts',(-12.5979265476489,31.8452809243699,27.3109269076298));
#47935=CARTESIAN_POINT('Ctrl Pts',(-12.6878190122229,31.923824784325,27.3051214857763));
#47936=CARTESIAN_POINT('Ctrl Pts',(-12.7778110246595,32.0024556245785,27.2993096349375));
#47937=CARTESIAN_POINT('Ctrl Pts',(-12.8642888981799,32.0849855755752,27.2934977840986));
#47938=CARTESIAN_POINT('Ctrl Pts',(-12.9469137751714,32.1710559917692,27.2876859332597));
#47939=CARTESIAN_POINT('Ctrl Pts',(-13.0295929207846,32.2571829396402,27.2818702651549));
#47940=CARTESIAN_POINT('Ctrl Pts',(-13.1084137609984,32.3468546778158,27.27605459705));
#47941=CARTESIAN_POINT('Ctrl Pts',(-13.183077882607,32.4396796697956,27.2702389289451));
#47942=CARTESIAN_POINT('Ctrl Pts',(-13.2578489526581,32.5326376237402,27.2644149305119));
#47943=CARTESIAN_POINT('Ctrl Pts',(-13.3284511792542,32.6287575186502,27.2585909320788));
#47944=CARTESIAN_POINT('Ctrl Pts',(-13.3946295043692,32.7276189738369,27.2527669336456));
#47945=CARTESIAN_POINT('Ctrl Pts',(-13.4121869160277,32.7538473690533,27.2512218002834));
#47946=CARTESIAN_POINT('Ctrl Pts',(-13.4294331969676,32.7802686016505,27.2496766669212));
#47947=CARTESIAN_POINT('Ctrl Pts',(-13.4463641371064,32.8068745511333,27.248131533559));
#47948=CARTESIAN_POINT('Ctrl Pts',(-13.511628181384,32.9094330535468,27.242175476108));
#47949=CARTESIAN_POINT('Ctrl Pts',(-13.5724057738479,33.0150566328513,27.2362194186571));
#47950=CARTESIAN_POINT('Ctrl Pts',(-13.6284046854858,33.1233262301762,27.2302633612062));
#47951=CARTESIAN_POINT('Ctrl Pts',(-13.6843233504708,33.2314406767572,27.2243158388082));
#47952=CARTESIAN_POINT('Ctrl Pts',(-13.735476789618,33.3421932568942,27.2183683164102));
#47953=CARTESIAN_POINT('Ctrl Pts',(-13.7816163112617,33.4551365515363,27.2124207940122));
#47954=CARTESIAN_POINT('Ctrl Pts',(-13.8276986054601,33.5679397611495,27.2064806484032));
#47955=CARTESIAN_POINT('Ctrl Pts',(-13.8687792177871,33.6829279234472,27.2005405027941));
#47956=CARTESIAN_POINT('Ctrl Pts',(-13.9046557781041,33.7996299510075,27.194600357185));
#47957=CARTESIAN_POINT('Ctrl Pts',(-13.9404859561889,33.9161811028851,27.1886678911643));
#47958=CARTESIAN_POINT('Ctrl Pts',(-13.971125376415,34.0344413399889,27.1827354251435));
#47959=CARTESIAN_POINT('Ctrl Pts',(-13.9964203632244,34.1539212327418,27.1768029591227));
#47960=CARTESIAN_POINT('Ctrl Pts',(-14.021696079943,34.2733101039656,27.1708750125413));
#47961=CARTESIAN_POINT('Ctrl Pts',(-14.0416353884593,34.3939164074824,27.1649470659599));
#47962=CARTESIAN_POINT('Ctrl Pts',(-14.0561348460667,34.5152370573942,27.1590191193785));
#47963=CARTESIAN_POINT('Ctrl Pts',(-14.0706246909313,34.636477275043,27.153095102863));
#47964=CARTESIAN_POINT('Ctrl Pts',(-14.0796818242133,34.7584305156171,27.1471710863476));
#47965=CARTESIAN_POINT('Ctrl Pts',(-14.0832542386473,34.880585501012,27.1412470698321));
#47966=CARTESIAN_POINT('Ctrl Pts',(-14.0844325971131,34.9208782396713,27.1392930370229));
#47967=CARTESIAN_POINT('Ctrl Pts',(-14.0850146333955,34.9611928784735,27.1373390042137));
#47968=CARTESIAN_POINT('Ctrl Pts',(-14.0849997205639,35.0015109577178,27.1353849714045));
#47969=CARTESIAN_POINT('Ctrl Pts',(-14.0849997205636,35.0015109583762,27.1353849713726));
#47970=CARTESIAN_POINT('Ctrl Pts',(-14.0849517284655,35.1312615262673,27.1290965550734));
#47971=CARTESIAN_POINT('Ctrl Pts',(-14.0787177200379,35.260826007354,27.1228081387741));
#47972=CARTESIAN_POINT('Ctrl Pts',(-14.0663757192053,35.3896325323401,27.1165197224749));
#47973=CARTESIAN_POINT('Ctrl Pts',(-14.0539812321377,35.518986826657,27.1102045637293));
#47974=CARTESIAN_POINT('Ctrl Pts',(-14.0354267800673,35.6475764227977,27.1038894049837));
#47975=CARTESIAN_POINT('Ctrl Pts',(-14.0108419950697,35.7748364282771,27.0975742462381));
#47976=CARTESIAN_POINT('Ctrl Pts',(-13.9862032615903,35.902375691195,27.0912452296032));
#47977=CARTESIAN_POINT('Ctrl Pts',(-13.955507825809,36.0285792550034,27.0849162129684));
#47978=CARTESIAN_POINT('Ctrl Pts',(-13.918935263764,36.1528969591543,27.0785871963336));
#47979=CARTESIAN_POINT('Ctrl Pts',(-13.882247254912,36.2776070908842,27.0722382012035));
#47980=CARTESIAN_POINT('Ctrl Pts',(-13.8396450940903,36.4004191788262,27.0658892060733));
#47981=CARTESIAN_POINT('Ctrl Pts',(-13.7913574449856,36.5208003565073,27.0595402109431));
#47982=CARTESIAN_POINT('Ctrl Pts',(-13.7698384574765,36.5744472228773,27.0567108342923));
#47983=CARTESIAN_POINT('Ctrl Pts',(-13.7471909666541,36.6276116407118,27.0538814576414));
#47984=CARTESIAN_POINT('Ctrl Pts',(-13.723438111232,36.6802480863923,27.0510520809906));
#47985=CARTESIAN_POINT('Ctrl Pts',(-13.6745485456912,36.7885876066396,27.0452284866162));
#47986=CARTESIAN_POINT('Ctrl Pts',(-13.6208477443071,36.8949662781929,27.0394048922419));
#47987=CARTESIAN_POINT('Ctrl Pts',(-13.5625152040873,36.9989273174997,27.0335812978675));
#47988=CARTESIAN_POINT('Ctrl Pts',(-13.5042562589436,37.1027571946701,27.0277650508137));
#47989=CARTESIAN_POINT('Ctrl Pts',(-13.441377395838,37.2041751533971,27.0219488037599));
#47990=CARTESIAN_POINT('Ctrl Pts',(-13.3741058398894,37.3027450534577,27.0161325567061));
#47991=CARTESIAN_POINT('Ctrl Pts',(-13.3069016230506,37.4012162846349,27.01032213174));
#47992=CARTESIAN_POINT('Ctrl Pts',(-13.2353136897221,37.4968447933583,27.0045117067738));
#47993=CARTESIAN_POINT('Ctrl Pts',(-13.1596144705095,37.5892202296728,26.9987012818077));
#47994=CARTESIAN_POINT('Ctrl Pts',(-13.0810498924533,37.6850922512379,26.99267092125));
#47995=CARTESIAN_POINT('Ctrl Pts',(-12.9980568583433,37.7774596737138,26.9866405606923));
#47996=CARTESIAN_POINT('Ctrl Pts',(-12.9109886680953,37.8658977606015,26.9806102001345));
#47997=CARTESIAN_POINT('Ctrl Pts',(-12.8271904017444,37.9510144758964,26.9748063151707));
#47998=CARTESIAN_POINT('Ctrl Pts',(-12.7396178638162,38.0324913554615,26.9690024302068));
#47999=CARTESIAN_POINT('Ctrl Pts',(-12.6486256463042,38.1099850780574,26.963198545243));
#48000=CARTESIAN_POINT('Ctrl Pts',(-12.5576468692598,38.1874673540495,26.9573955175714));
#48001=CARTESIAN_POINT('Ctrl Pts',(-12.4632497279483,38.2609673784343,26.9515924898999));
#48002=CARTESIAN_POINT('Ctrl Pts',(-12.3658231667572,38.3301810376667,26.9457894622284));
#48003=CARTESIAN_POINT('Ctrl Pts',(-12.2683880037758,38.3994008077726,26.9399859222075));
#48004=CARTESIAN_POINT('Ctrl Pts',(-12.1679232220264,38.4643332237901,26.9341823821867));
#48005=CARTESIAN_POINT('Ctrl Pts',(-12.0648475745558,38.5247169381173,26.9283788421659));
#48006=CARTESIAN_POINT('Ctrl Pts',(-11.9617385008254,38.585120234196,26.9225734201231));
#48007=CARTESIAN_POINT('Ctrl Pts',(-11.8560172296798,38.6409716886629,26.9167679980803));
#48008=CARTESIAN_POINT('Ctrl Pts',(-11.7481274046206,38.6920557386386,26.9109625760375));
#48009=CARTESIAN_POINT('Ctrl Pts',(-11.6401181015986,38.7431963594561,26.9051507250288));
#48010=CARTESIAN_POINT('Ctrl Pts',(-11.5299358203959,38.7895588626861,26.8993388740202));
#48011=CARTESIAN_POINT('Ctrl Pts',(-11.4180446316806,38.8309756489127,26.8935270230115));
#48012=CARTESIAN_POINT('Ctrl Pts',(-11.3060799522349,38.8724196379056,26.8877113547481));
#48013=CARTESIAN_POINT('Ctrl Pts',(-11.192404517851,38.9089113161549,26.8818956864847));
#48014=CARTESIAN_POINT('Ctrl Pts',(-11.0774964194521,38.9403332937796,26.8760800182213));
#48015=CARTESIAN_POINT('Ctrl Pts',(-10.9624237277325,38.9718002799608,26.8702560196472));
#48016=CARTESIAN_POINT('Ctrl Pts',(-10.8461152446498,38.9981829813635,26.8644320210732));
#48017=CARTESIAN_POINT('Ctrl Pts',(-10.7290582092595,39.0194152718413,26.8586080224991));
#48018=CARTESIAN_POINT('Ctrl Pts',(-10.698002484593,39.0250482879597,26.8570628911401));
#48019=CARTESIAN_POINT('Ctrl Pts',(-10.6668940919761,39.0303190693622,26.8555177597811));
#48020=CARTESIAN_POINT('Ctrl Pts',(-10.6357421573143,39.0352269960206,26.8539726284221));
#48021=CARTESIAN_POINT('Ctrl Pts',(-10.5183157489126,39.0537272980548,26.8481482959058));
#48022=CARTESIAN_POINT('Ctrl Pts',(-10.399891739978,39.0671274618897,26.8423239633895));
#48023=CARTESIAN_POINT('Ctrl Pts',(-10.280950748406,39.0753271864931,26.8364996308732));
#48024=CARTESIAN_POINT('Ctrl Pts',(-10.1586484671851,39.0837586365015,26.8305107018764));
#48025=CARTESIAN_POINT('Ctrl Pts',(-10.0357999544713,39.08669119238,26.8245217728796));
#48026=CARTESIAN_POINT('Ctrl Pts',(-9.91293954859989,39.084072168535,26.8185328438828));
#48027=CARTESIAN_POINT('Ctrl Pts',(-9.79375530529611,39.0815315097039,26.812723112378));
#48028=CARTESIAN_POINT('Ctrl Pts',(-9.67456031682524,39.0737667410615,26.8069133808732));
#48029=CARTESIAN_POINT('Ctrl Pts',(-9.55584699425329,39.0607823270259,26.8011036493684));
#48030=CARTESIAN_POINT('Ctrl Pts',(-9.43721246835627,39.0478065314725,26.7952977741075));
#48031=CARTESIAN_POINT('Ctrl Pts',(-9.31905937694257,39.029618025078,26.7894918988466));
#48032=CARTESIAN_POINT('Ctrl Pts',(-9.2018775407792,39.0062732732662,26.7836860235857));
#48033=CARTESIAN_POINT('Ctrl Pts',(-9.08474582834405,38.9829385070122,26.7778826317482));
#48034=CARTESIAN_POINT('Ctrl Pts',(-8.96858494435268,38.9544519629652,26.7720792399107));
#48035=CARTESIAN_POINT('Ctrl Pts',(-8.85387638091336,38.9209215306828,26.7662758480732));
#48036=CARTESIAN_POINT('Ctrl Pts',(-8.73918981206799,38.8873975276347,26.760473568997));
#48037=CARTESIAN_POINT('Ctrl Pts',(-8.62595540081611,38.8488316768081,26.7546712899207));
#48038=CARTESIAN_POINT('Ctrl Pts',(-8.51464067433854,38.8053820667143,26.7488690108445));
#48039=CARTESIAN_POINT('Ctrl Pts',(-8.40328784783913,38.7619175849934,26.743064745805));
#48040=CARTESIAN_POINT('Ctrl Pts',(-8.29385639982131,38.7135661517273,26.7372604807654));
#48041=CARTESIAN_POINT('Ctrl Pts',(-8.18679482973066,38.6605343886526,26.7314562157259));
#48042=CARTESIAN_POINT('Ctrl Pts',(-8.07971025319162,38.6074912295886,26.7256507034086));
#48043=CARTESIAN_POINT('Ctrl Pts',(-7.97499692976636,38.549765928425,26.7198451910912));
#48044=CARTESIAN_POINT('Ctrl Pts',(-7.87307860825309,38.4876109865249,26.7140396787738));
#48045=CARTESIAN_POINT('Ctrl Pts',(-7.77108030047314,38.4254072649581,26.7082296102467));
#48046=CARTESIAN_POINT('Ctrl Pts',(-7.67188171481285,38.3587671863771,26.7024195417195));
#48047=CARTESIAN_POINT('Ctrl Pts',(-7.57587734912902,38.287986370643,26.6966094731923));
#48048=CARTESIAN_POINT('Ctrl Pts',(-7.55470410181315,38.2723760418201,26.6953280937783));
#48049=CARTESIAN_POINT('Ctrl Pts',(-7.5336860937674,38.2565644634426,26.6940467143642));
#48050=CARTESIAN_POINT('Ctrl Pts',(-7.51282733495086,38.2405550657615,26.6927653349501));
#48051=CARTESIAN_POINT('',(-14.0849999969886,34.9998431448262,27.2396150285597));
#48052=CARTESIAN_POINT('Ctrl Pts',(-14.0849999969886,34.9998431448262,27.2396150285597));
#48053=CARTESIAN_POINT('Ctrl Pts',(-14.0850045558039,35.1185689743034,27.2337980380796));
#48054=CARTESIAN_POINT('Ctrl Pts',(-14.0798288721455,35.2374885762744,27.2279810475995));
#48055=CARTESIAN_POINT('Ctrl Pts',(-14.0694482080588,35.3561127376648,27.2221640571194));
#48056=CARTESIAN_POINT('Ctrl Pts',(-14.0590806440589,35.474587198921,27.2163544075068));
#48057=CARTESIAN_POINT('Ctrl Pts',(-14.0435211990243,35.5927665569149,27.2105447578942));
#48058=CARTESIAN_POINT('Ctrl Pts',(-14.0227971293024,35.7101607258055,27.2047351082816));
#48059=CARTESIAN_POINT('Ctrl Pts',(-14.0020937762772,35.8274375422926,27.1989312662518));
#48060=CARTESIAN_POINT('Ctrl Pts',(-13.9762361395857,35.9439303302516,27.1931274242219));
#48061=CARTESIAN_POINT('Ctrl Pts',(-13.9453032926047,36.0591538742612,27.187323582192));
#48062=CARTESIAN_POINT('Ctrl Pts',(-13.9134326011801,36.1778708490754,27.1813437750787));
#48063=CARTESIAN_POINT('Ctrl Pts',(-13.8761740789372,36.2952399475765,27.1753639679655));
#48064=CARTESIAN_POINT('Ctrl Pts',(-13.8336711615995,36.4107410906047,27.1693841608522));
#48065=CARTESIAN_POINT('Ctrl Pts',(-13.7924649384881,36.5227184833897,27.1635867878363));
#48066=CARTESIAN_POINT('Ctrl Pts',(-13.7463298210225,36.6329398305309,27.1577894148203));
#48067=CARTESIAN_POINT('Ctrl Pts',(-13.6954469874095,36.7409470305687,27.1519920418044));
#48068=CARTESIAN_POINT('Ctrl Pts',(-13.6445714568429,36.8489387286871,27.1461955008664));
#48069=CARTESIAN_POINT('Ctrl Pts',(-13.5889497396612,36.9547165414042,27.1403989599284));
#48070=CARTESIAN_POINT('Ctrl Pts',(-13.5288104706594,37.0578439353275,27.1346024189904));
#48071=CARTESIAN_POINT('Ctrl Pts',(-13.4686655496186,37.1609810214215,27.128805333279));
#48072=CARTESIAN_POINT('Ctrl Pts',(-13.4040024389248,37.2614668398338,27.1230082475676));
#48073=CARTESIAN_POINT('Ctrl Pts',(-13.3350945484181,37.3588915517911,27.1172111618562));
#48074=CARTESIAN_POINT('Ctrl Pts',(-13.2661638155399,37.4563485592004,27.1114121544608));
#48075=CARTESIAN_POINT('Ctrl Pts',(-13.1929857408893,37.5507421081638,27.1056131470655));
#48076=CARTESIAN_POINT('Ctrl Pts',(-13.1158752615912,37.6416938418757,27.0998141396701));
#48077=CARTESIAN_POINT('Ctrl Pts',(-13.0386792540938,37.7327464560136,27.0940087002221));
#48078=CARTESIAN_POINT('Ctrl Pts',(-12.9575424012137,37.8203493229476,27.0882032607742));
#48079=CARTESIAN_POINT('Ctrl Pts',(-12.8728179773002,37.9041594083832,27.0823978213262));
#48080=CARTESIAN_POINT('Ctrl Pts',(-12.7880371252074,37.9880253130302,27.0765885153382));
#48081=CARTESIAN_POINT('Ctrl Pts',(-12.6996642465922,38.0680931317307,27.0707792093502));
#48082=CARTESIAN_POINT('Ctrl Pts',(-12.6080860325812,38.1440598350946,27.0649699033622));
#48083=CARTESIAN_POINT('Ctrl Pts',(-12.5163779071733,38.2201343036147,27.0591523563851));
#48084=CARTESIAN_POINT('Ctrl Pts',(-12.4214556969101,38.2920958001124,27.0533348094081));
#48085=CARTESIAN_POINT('Ctrl Pts',(-12.3237354569492,38.3596842896494,27.0475172624311));
#48086=CARTESIAN_POINT('Ctrl Pts',(-12.3029678636063,38.3740482562742,27.0462809121119));
#48087=CARTESIAN_POINT('Ctrl Pts',(-12.2820739852722,38.3882148807375,27.0450445617926));
#48088=CARTESIAN_POINT('Ctrl Pts',(-12.2610579524937,38.4021819374432,27.0438082114734));
#48089=CARTESIAN_POINT('Ctrl Pts',(-12.1620659091485,38.4679711136116,27.0379846173782));
#48090=CARTESIAN_POINT('Ctrl Pts',(-12.0600404855678,38.5295422904057,27.032161023283));
#48091=CARTESIAN_POINT('Ctrl Pts',(-11.955376494584,38.586603931915,27.0263374291879));
#48092=CARTESIAN_POINT('Ctrl Pts',(-11.8508445524174,38.6435935818808,27.020521182402));
#48093=CARTESIAN_POINT('Ctrl Pts',(-11.7436810193798,38.6960848189747,27.0147049356161));
#48094=CARTESIAN_POINT('Ctrl Pts',(-11.6343101666339,38.7438289596665,27.0088886888302));
#48095=CARTESIAN_POINT('Ctrl Pts',(-11.5250487943582,38.7915253083657,27.0030782641205));
#48096=CARTESIAN_POINT('Ctrl Pts',(-11.4135848700468,38.8344838514615,26.9972678394107));
#48097=CARTESIAN_POINT('Ctrl Pts',(-11.3003672509087,38.8725017769866,26.991457414701));
#48098=CARTESIAN_POINT('Ctrl Pts',(-11.1828641232769,38.9119587554081,26.9854270540428));
#48099=CARTESIAN_POINT('Ctrl Pts',(-11.0634723096386,38.9460934875123,26.9793966933847));
#48100=CARTESIAN_POINT('Ctrl Pts',(-10.9427168160288,38.9747339539618,26.9733663327265));
#48101=CARTESIAN_POINT('Ctrl Pts',(-10.8264964096308,39.0022988005015,26.9675624479883));
#48102=CARTESIAN_POINT('Ctrl Pts',(-10.7090133377308,39.0247745211941,26.96175856325));
#48103=CARTESIAN_POINT('Ctrl Pts',(-10.5907504314025,39.0420587486821,26.9559546785118));
#48104=CARTESIAN_POINT('Ctrl Pts',(-10.4725049934573,39.0593404231507,26.9501516510541));
#48105=CARTESIAN_POINT('Ctrl Pts',(-10.3534803540914,39.0714320703526,26.9443486235963));
#48106=CARTESIAN_POINT('Ctrl Pts',(-10.2341676060894,39.0782827920901,26.9385455961386));
#48107=CARTESIAN_POINT('Ctrl Pts',(-10.1148443237163,39.0851341186921,26.9327420563194));
#48108=CARTESIAN_POINT('Ctrl Pts',(-9.99523328981639,39.0867435763978,26.9269385165003));
#48109=CARTESIAN_POINT('Ctrl Pts',(-9.87582811889162,39.0831123354547,26.9211349766812));
#48110=CARTESIAN_POINT('Ctrl Pts',(-9.75638422597141,39.0794799169336,26.9153295548276));
#48111=CARTESIAN_POINT('Ctrl Pts',(-9.63714673673404,39.0706034322274,26.9095241329741));
#48112=CARTESIAN_POINT('Ctrl Pts',(-9.51860601690882,39.0565360633234,26.9037187111205));
#48113=CARTESIAN_POINT('Ctrl Pts',(-9.39993402384117,39.0424531160669,26.8979068602816));
#48114=CARTESIAN_POINT('Ctrl Pts',(-9.28196074611695,39.0231678583829,26.8920950094427));
#48115=CARTESIAN_POINT('Ctrl Pts',(-9.16516836200605,38.9987849574845,26.8862831586038));
#48116=CARTESIAN_POINT('Ctrl Pts',(-9.04829926780661,38.9743860417192,26.8804674904989));
#48117=CARTESIAN_POINT('Ctrl Pts',(-8.93261300664934,38.9448829154511,26.8746518223941));
#48118=CARTESIAN_POINT('Ctrl Pts',(-8.81857694846586,38.910430228671,26.8688361542892));
#48119=CARTESIAN_POINT('Ctrl Pts',(-8.70437754571248,38.8759281920677,26.863012155856));
#48120=CARTESIAN_POINT('Ctrl Pts',(-8.59183344779533,38.8364625788986,26.8571881574228));
#48121=CARTESIAN_POINT('Ctrl Pts',(-8.48139252895936,38.7922363255604,26.8513641589896));
#48122=CARTESIAN_POINT('Ctrl Pts',(-8.45209204920571,38.7805028987275,26.8498190256281));
#48123=CARTESIAN_POINT('Ctrl Pts',(-8.42293947092207,38.7684346380036,26.8482738922665));
#48124=CARTESIAN_POINT('Ctrl Pts',(-8.39394285403675,38.7560358682926,26.8467287589049));
#48125=CARTESIAN_POINT('Ctrl Pts',(-8.28465587827726,38.7093054496986,26.840905219114));
#48126=CARTESIAN_POINT('Ctrl Pts',(-8.1772338902608,38.6577259362034,26.8350816793232));
#48127=CARTESIAN_POINT('Ctrl Pts',(-8.07213713171789,38.6014677231789,26.8292581395323));
#48128=CARTESIAN_POINT('Ctrl Pts',(-7.96718840989531,38.5452887540954,26.823442802637));
#48129=CARTESIAN_POINT('Ctrl Pts',(-7.86455875644979,38.4844443913091,26.8176274657417));
#48130=CARTESIAN_POINT('Ctrl Pts',(-7.76468852857154,38.4191530567818,26.8118121288463));
#48131=CARTESIAN_POINT('Ctrl Pts',(-7.67859493062924,38.3628683558921,26.8067989904246));
#48132=CARTESIAN_POINT('Ctrl Pts',(-7.59455181840578,38.3032797833452,26.8017858520028));
#48133=CARTESIAN_POINT('Ctrl Pts',(-7.51282733495086,38.2405550657615,26.7967727135811));
#48134=CARTESIAN_POINT('Ctrl Pts',(-7.51282733495086,38.2405550657615,28.0469627484298));
#48135=CARTESIAN_POINT('Ctrl Pts',(-7.41670709116374,38.1667813948768,28.0410436570584));
#48136=CARTESIAN_POINT('Ctrl Pts',(-7.32400107801209,38.0888265544615,28.035124565687));
#48137=CARTESIAN_POINT('Ctrl Pts',(-7.23507125100175,38.0070573677539,28.0292054743156));
#48138=CARTESIAN_POINT('Ctrl Pts',(-7.14757772263507,37.9266088287515,28.0233819817235));
#48139=CARTESIAN_POINT('Ctrl Pts',(-7.06345707173295,37.8422087686331,28.0175584891315));
#48140=CARTESIAN_POINT('Ctrl Pts',(-6.98308656305463,37.7541710756557,28.0117349965394));
#48141=CARTESIAN_POINT('Ctrl Pts',(-6.90281747526042,37.6662444789101,28.0059188527097));
#48142=CARTESIAN_POINT('Ctrl Pts',(-6.82628939002253,37.5746896783972,28.0001027088799));
#48143=CARTESIAN_POINT('Ctrl Pts',(-6.75384498132295,37.4798593901102,27.9942865650502));
#48144=CARTESIAN_POINT('Ctrl Pts',(-6.68147310735251,37.3851240503417,27.9884762446156));
#48145=CARTESIAN_POINT('Ctrl Pts',(-6.6131770223021,37.2871200697274,27.982665924181));
#48146=CARTESIAN_POINT('Ctrl Pts',(-6.54926071521043,37.1862349801451,27.9768556037465));
#48147=CARTESIAN_POINT('Ctrl Pts',(-6.4829234357633,37.0815286433088,27.9708252044965));
#48148=CARTESIAN_POINT('Ctrl Pts',(-6.42130458400046,36.9737189565349,27.9647948052465));
#48149=CARTESIAN_POINT('Ctrl Pts',(-6.36469642355648,36.8632747803523,27.9587644059965));
#48150=CARTESIAN_POINT('Ctrl Pts',(-6.31021558851144,36.7569810782235,27.9529606281628));
#48151=CARTESIAN_POINT('Ctrl Pts',(-6.26037584188556,36.6482477169935,27.9471568503291));
#48152=CARTESIAN_POINT('Ctrl Pts',(-6.21539172638949,36.5375191755939,27.9413530724953));
#48153=CARTESIAN_POINT('Ctrl Pts',(-6.17041426163255,36.4268070050095,27.9355501527292));
#48154=CARTESIAN_POINT('Ctrl Pts',(-6.13029115401035,36.3141006191003,27.9297472329631));
#48155=CARTESIAN_POINT('Ctrl Pts',(-6.09518893192452,36.199864793481,27.9239443131969));
#48156=CARTESIAN_POINT('Ctrl Pts',(-6.06008361459922,36.085618894789,27.9181408817416));
#48157=CARTESIAN_POINT('Ctrl Pts',(-6.03000018301447,35.9698436786082,27.9123374502864));
#48158=CARTESIAN_POINT('Ctrl Pts',(-6.00505520043724,35.8530187855179,27.9065340188311));
#48159=CARTESIAN_POINT('Ctrl Pts',(-5.98010213067867,35.7361560177131,27.9007287058991));
#48160=CARTESIAN_POINT('Ctrl Pts',(-5.96029090822835,35.6182432953538,27.8949233929672));
#48161=CARTESIAN_POINT('Ctrl Pts',(-5.94568681023975,35.4997695062086,27.8891180800352));
#48162=CARTESIAN_POINT('Ctrl Pts',(-5.93106653992792,35.3811645212572,27.8833063384011));
#48163=CARTESIAN_POINT('Ctrl Pts',(-5.92166495405033,35.2619976348475,27.8774945967669));
#48164=CARTESIAN_POINT('Ctrl Pts',(-5.91749537731631,35.1427620599678,27.8716828551327));
#48165=CARTESIAN_POINT('Ctrl Pts',(-5.91332306213287,35.0234481748396,27.8658672965259));
#48166=CARTESIAN_POINT('Ctrl Pts',(-5.91438959577009,34.9040659187974,27.8600517379191));
#48167=CARTESIAN_POINT('Ctrl Pts',(-5.92065623087951,34.7851060416443,27.8542361793122));
#48168=CARTESIAN_POINT('Ctrl Pts',(-5.92693184288152,34.6659757556479,27.8484122899754));
#48169=CARTESIAN_POINT('Ctrl Pts',(-5.93842238513361,34.5472694612052,27.8425884006386));
#48170=CARTESIAN_POINT('Ctrl Pts',(-5.95503756801433,34.4294704882089,27.8367645113017));
#48171=CARTESIAN_POINT('Ctrl Pts',(-5.95944867244888,34.3981964675797,27.8352183481169));
#48172=CARTESIAN_POINT('Ctrl Pts',(-5.96422070095098,34.3669863273422,27.833672184932));
#48173=CARTESIAN_POINT('Ctrl Pts',(-5.96935137044259,34.3358489441046,27.8321260217471));
#48174=CARTESIAN_POINT('Ctrl Pts',(-5.98867604553686,34.2185699388332,27.8263023955636));
#48175=CARTESIAN_POINT('Ctrl Pts',(-6.0131547955719,34.1019459598726,27.8204787693801));
#48176=CARTESIAN_POINT('Ctrl Pts',(-6.04273187214429,33.9864646211121,27.8146551431966));
#48177=CARTESIAN_POINT('Ctrl Pts',(-6.07227163448797,33.8711289727844,27.8088388640583));
#48178=CARTESIAN_POINT('Ctrl Pts',(-6.10689682982483,33.7569334895309,27.80302258492));
#48179=CARTESIAN_POINT('Ctrl Pts',(-6.14650027428743,33.6443581358142,27.7972063057817));
#48180=CARTESIAN_POINT('Ctrl Pts',(-6.1860640773497,33.5318954653432,27.7913958484969));
#48181=CARTESIAN_POINT('Ctrl Pts',(-6.23059608170363,33.4210500812495,27.7855853912121));
#48182=CARTESIAN_POINT('Ctrl Pts',(-6.27993877937317,33.3122886755169,27.7797749339272));
#48183=CARTESIAN_POINT('Ctrl Pts',(-6.33114880464832,33.199411297514,27.7737445853961));
#48184=CARTESIAN_POINT('Ctrl Pts',(-6.38754071709162,33.0887791803389,27.7677142368649));
#48185=CARTESIAN_POINT('Ctrl Pts',(-6.44888258169824,32.980893741916,27.7616838883337));
#48186=CARTESIAN_POINT('Ctrl Pts',(-6.50792114793186,32.8770592458045,27.7558799706756));
#48187=CARTESIAN_POINT('Ctrl Pts',(-6.5715444214833,32.7757692666811,27.7500760530175));
#48188=CARTESIAN_POINT('Ctrl Pts',(-6.63949823731052,32.6774468998619,27.7442721353594));
#48189=CARTESIAN_POINT('Ctrl Pts',(-6.70744201668592,32.5791390547835,27.7384690749121));
#48190=CARTESIAN_POINT('Ctrl Pts',(-6.77971483427688,32.4837982861855,27.7326660144647));
#48191=CARTESIAN_POINT('Ctrl Pts',(-6.85601923051103,32.3918186564037,27.7268629540173));
#48192=CARTESIAN_POINT('Ctrl Pts',(-6.93233036422389,32.2998309050611,27.7210593811749));
#48193=CARTESIAN_POINT('Ctrl Pts',(-7.01267352362666,32.2112051968888,27.7152558083325));
#48194=CARTESIAN_POINT('Ctrl Pts',(-7.09671142810893,32.1263019524789,27.70945223549));
#48195=CARTESIAN_POINT('Ctrl Pts',(-7.18077658511862,32.0413711749217,27.7036467806156));
#48196=CARTESIAN_POINT('Ctrl Pts',(-7.2685385829815,31.9601655519409,27.6978413257411));
#48197=CARTESIAN_POINT('Ctrl Pts',(-7.35962429435116,31.883007678383,27.6920358708667));
#48198=CARTESIAN_POINT('Ctrl Pts',(-7.45081087175119,31.8057643621327,27.6862239871772));
#48199=CARTESIAN_POINT('Ctrl Pts',(-7.54532819768965,31.7325780065979,27.6804121034877));
#48200=CARTESIAN_POINT('Ctrl Pts',(-7.64277104928343,31.6637301257387,27.6746002197983));
#48201=CARTESIAN_POINT('Ctrl Pts',(-7.74027790067057,31.5948370260658,27.6687845189037));
#48202=CARTESIAN_POINT('Ctrl Pts',(-7.84071376164357,31.530288296142,27.6629688180091));
#48203=CARTESIAN_POINT('Ctrl Pts',(-7.94364692557595,31.4703205480799,27.6571531171144));
#48204=CARTESIAN_POINT('Ctrl Pts',(-8.04672752351718,31.4102669065589,27.6513290862311));
#48205=CARTESIAN_POINT('Ctrl Pts',(-8.15231220361358,31.3548075324376,27.6455050553477));
#48206=CARTESIAN_POINT('Ctrl Pts',(-8.25994721148222,31.3041318620422,27.6396810244644));
#48207=CARTESIAN_POINT('Ctrl Pts',(-8.28849729080766,31.2906901906167,27.6381362060358));
#48208=CARTESIAN_POINT('Ctrl Pts',(-8.3171915328134,31.2775848174412,27.6365913876072));
#48209=CARTESIAN_POINT('Ctrl Pts',(-8.3460212848029,31.2648186911912,27.6350465691787));
#48210=CARTESIAN_POINT('Ctrl Pts',(-8.45470265279246,31.2166934050185,27.6292229679152));
#48211=CARTESIAN_POINT('Ctrl Pts',(-8.56566144318004,31.1732378534696,27.6233993666517));
#48212=CARTESIAN_POINT('Ctrl Pts',(-8.67845927504702,31.1346727030831,27.6175757653883));
#48213=CARTESIAN_POINT('Ctrl Pts',(-8.79111479986565,31.0961562069361,27.6117595112475));
#48214=CARTESIAN_POINT('Ctrl Pts',(-8.90560436845581,31.0625179713262,27.6059432571067));
#48215=CARTESIAN_POINT('Ctrl Pts',(-9.02146780232413,31.033931450654,27.6001270029659));
#48216=CARTESIAN_POINT('Ctrl Pts',(-9.13721526030036,31.0053735442488,27.5943165707245));
#48217=CARTESIAN_POINT('Ctrl Pts',(-9.25433345359814,30.9818573905163,27.5885061384832));
#48218=CARTESIAN_POINT('Ctrl Pts',(-9.37234571834909,30.9635070788214,27.5826957062418));
#48219=CARTESIAN_POINT('Ctrl Pts',(-9.49482476356167,30.9444622053033,27.5766653483405));
#48220=CARTESIAN_POINT('Ctrl Pts',(-9.61826647477876,30.9309821007485,27.5706349904392));
#48221=CARTESIAN_POINT('Ctrl Pts',(-9.74212433676339,30.9231476428119,27.5646046325379));
#48222=CARTESIAN_POINT('Ctrl Pts',(-9.86133081644452,30.9156074016364,27.5588007398732));
#48223=CARTESIAN_POINT('Ctrl Pts',(-9.98092230995851,30.9132964462796,27.5529968472085));
#48224=CARTESIAN_POINT('Ctrl Pts',(-10.100405632154,30.9162341265651,27.5471929545439));
#48225=CARTESIAN_POINT('Ctrl Pts',(-10.2198713084547,30.9191713729992,27.5413899190271));
#48226=CARTESIAN_POINT('Ctrl Pts',(-10.3392284371046,30.9273557035237,27.5355868835104));
#48227=CARTESIAN_POINT('Ctrl Pts',(-10.4579843827478,30.9407543428416,27.5297838479936));
#48228=CARTESIAN_POINT('Ctrl Pts',(-10.576750816131,30.9541541654388,27.5239802999911));
#48229=CARTESIAN_POINT('Ctrl Pts',(-10.6949155551654,30.9727691666192,27.5181767519886));
#48230=CARTESIAN_POINT('Ctrl Pts',(-10.8119922730246,30.9965148247373,27.5123732039862));
#48231=CARTESIAN_POINT('Ctrl Pts',(-10.9291069600736,31.0202681838178,27.5065677738331));
#48232=CARTESIAN_POINT('Ctrl Pts',(-11.0451325242137,31.049155427883,27.50076234368));
#48233=CARTESIAN_POINT('Ctrl Pts',(-11.1595946251472,31.0830413194253,27.4949569135269));
#48234=CARTESIAN_POINT('Ctrl Pts',(-11.274183485032,31.1169647372757,27.4891450542568));
#48235=CARTESIAN_POINT('Ctrl Pts',(-11.38720503386,31.1558977362739,27.4833331949867));
#48236=CARTESIAN_POINT('Ctrl Pts',(-11.4982016966553,31.1996557161042,27.4775213357166));
#48237=CARTESIAN_POINT('Ctrl Pts',(-11.6092712644171,31.2434424371054,27.4717056590939));
#48238=CARTESIAN_POINT('Ctrl Pts',(-11.7183129253534,31.2920602844803,27.4658899824711));
#48239=CARTESIAN_POINT('Ctrl Pts',(-11.8248921418185,31.3452778941855,27.4600743058484));
#48240=CARTESIAN_POINT('Ctrl Pts',(-11.931624022648,31.3985717329421,27.4542502988344));
#48241=CARTESIAN_POINT('Ctrl Pts',(-12.0358860631754,31.4564782871829,27.4484262918204));
#48242=CARTESIAN_POINT('Ctrl Pts',(-12.1372710965806,31.5187218927926,27.4426022848063));
#48243=CARTESIAN_POINT('Ctrl Pts',(-12.1641676233916,31.5352345549763,27.441057228741));
#48244=CARTESIAN_POINT('Ctrl Pts',(-12.1908618429779,31.5520522309247,27.4395121726756));
#48245=CARTESIAN_POINT('Ctrl Pts',(-12.217346542732,31.5691692974683,27.4379671166102));
#48246=CARTESIAN_POINT('Ctrl Pts',(-12.3171719183238,31.6336864569078,27.4321435353173));
#48247=CARTESIAN_POINT('Ctrl Pts',(-12.4143400985931,31.7026681387707,27.4263199540244));
#48248=CARTESIAN_POINT('Ctrl Pts',(-12.5084262207643,31.7758686604014,27.4204963727315));
#48249=CARTESIAN_POINT('Ctrl Pts',(-12.6023936360806,31.8489768261829,27.4146801389518));
#48250=CARTESIAN_POINT('Ctrl Pts',(-12.6932864081474,31.9262929961999,27.4088639051721));
#48251=CARTESIAN_POINT('Ctrl Pts',(-12.7807072119933,32.0075273767052,27.4030476713923));
#48252=CARTESIAN_POINT('Ctrl Pts',(-12.8680405044135,32.0886804386212,27.3972372598756));
#48253=CARTESIAN_POINT('Ctrl Pts',(-12.951908445413,32.1737436317883,27.3914268483588));
#48254=CARTESIAN_POINT('Ctrl Pts',(-13.0319459604685,32.2623863141782,27.385616436842));
#48255=CARTESIAN_POINT('Ctrl Pts',(-13.1150133078971,32.3543845788666,27.3795860713087));
#48256=CARTESIAN_POINT('Ctrl Pts',(-13.1939541424458,32.450238416805,27.3735557057754));
#48257=CARTESIAN_POINT('Ctrl Pts',(-13.2684012350255,32.5495350712806,27.367525340242));
#48258=CARTESIAN_POINT('Ctrl Pts',(-13.3400521708365,32.6451022448201,27.3617214690796));
#48259=CARTESIAN_POINT('Ctrl Pts',(-13.4075405704582,32.7438579256658,27.3559175979173));
#48260=CARTESIAN_POINT('Ctrl Pts',(-13.4705799038275,32.8454002387569,27.3501137267549));
#48261=CARTESIAN_POINT('Ctrl Pts',(-13.533609924475,32.9469275511292,27.3443107129911));
#48262=CARTESIAN_POINT('Ctrl Pts',(-13.5921919706256,33.0512403302465,27.3385076992274));
#48263=CARTESIAN_POINT('Ctrl Pts',(-13.6460834093786,33.1579085875413,27.3327046854636));
#48264=CARTESIAN_POINT('Ctrl Pts',(-13.6999796053681,33.2645862609166,27.3269011594421));
#48265=CARTESIAN_POINT('Ctrl Pts',(-13.7491841865616,33.373619461399,27.3210976334205));
#48266=CARTESIAN_POINT('Ctrl Pts',(-13.7935012572056,33.4845551110054,27.315294107399));
#48267=CARTESIAN_POINT('Ctrl Pts',(-13.8378326988198,33.5955267344003,27.3094886994322));
#48268=CARTESIAN_POINT('Ctrl Pts',(-13.8772733264631,33.7084016548261,27.3036832914655));
#48269=CARTESIAN_POINT('Ctrl Pts',(-13.9116762321749,33.8227090187054,27.2978778834987));
#48270=CARTESIAN_POINT('Ctrl Pts',(-13.9461172357447,33.9371429668258,27.2920660466096));
#48271=CARTESIAN_POINT('Ctrl Pts',(-13.9755092638981,34.0530121335273,27.2862542097205));
#48272=CARTESIAN_POINT('Ctrl Pts',(-13.9997558844047,34.169832628219,27.2804423728314));
#48273=CARTESIAN_POINT('Ctrl Pts',(-14.0240184300848,34.2867298505785,27.2746267187295));
#48274=CARTESIAN_POINT('Ctrl Pts',(-14.0431287725431,34.4045792431493,27.2688110646276));
#48275=CARTESIAN_POINT('Ctrl Pts',(-14.0570422195955,34.5228905488052,27.2629954105257));
#48276=CARTESIAN_POINT('Ctrl Pts',(-14.0709755963022,34.6413713238538,27.2571714260672));
#48277=CARTESIAN_POINT('Ctrl Pts',(-14.0796971899385,34.7603149267955,27.2513474416087));
#48278=CARTESIAN_POINT('Ctrl Pts',(-14.0832143633154,34.8792297088905,27.2455234571501));
#48279=CARTESIAN_POINT('Ctrl Pts',(-14.0841475668188,34.9107810938712,27.2439781927807));
#48280=CARTESIAN_POINT('Ctrl Pts',(-14.0847146690769,34.9423304726006,27.2424329284112));
#48281=CARTESIAN_POINT('Ctrl Pts',(-14.0849164197748,34.9738687265078,27.2408876640418));
#48282=CARTESIAN_POINT('Ctrl Pts',(-14.0849718051389,34.9825267271777,27.2404634522263));
#48283=CARTESIAN_POINT('Ctrl Pts',(-14.0849996645293,34.9911849040951,27.2400392404109));
#48284=CARTESIAN_POINT('Ctrl Pts',(-14.0849999969885,34.9998431440964,27.2396150285955));
#48285=CARTESIAN_POINT('Origin',(-10.,35.,32.7603849714045));
#48286=CARTESIAN_POINT('',(-7.51282733495086,38.2405550657615,29.2969304734038));
#48287=CARTESIAN_POINT('',(-7.51282733495085,38.2405550657615,29.1925543226443));
#48288=CARTESIAN_POINT('',(-7.51282733495086,38.2405550657615,32.7603849714045));
#48289=CARTESIAN_POINT('',(-14.0823970704021,34.9955937245638,29.7396160303676));
#48290=CARTESIAN_POINT('Ctrl Pts',(-14.0849976427674,34.9956115396029,29.7396150285955));
#48291=CARTESIAN_POINT('Ctrl Pts',(-14.0851248516661,35.1140239221068,29.7338651219894));
#48292=CARTESIAN_POINT('Ctrl Pts',(-14.0800991461781,35.23251947308,29.7281152153833));
#48293=CARTESIAN_POINT('Ctrl Pts',(-14.069925823144,35.3506120278963,29.7223653087771));
#48294=CARTESIAN_POINT('Ctrl Pts',(-14.0597551855942,35.4686734094473,29.7166169199921));
#48295=CARTESIAN_POINT('Ctrl Pts',(-14.0444396668569,35.586331591759,29.710868531207));
#48296=CARTESIAN_POINT('Ctrl Pts',(-14.0240365959555,35.7031034592512,29.7051201424219));
#48297=CARTESIAN_POINT('Ctrl Pts',(-14.0036338790127,35.8198733009501,29.6993718533616));
#48298=CARTESIAN_POINT('Ctrl Pts',(-13.9781438571365,35.9357564482399,29.6936235643013));
#48299=CARTESIAN_POINT('Ctrl Pts',(-13.9476752271182,36.0502786778742,29.687875275241));
#48300=CARTESIAN_POINT('Ctrl Pts',(-13.9171996109861,36.1648271661664,29.6821256681627));
#48301=CARTESIAN_POINT('Ctrl Pts',(-13.8817432246565,36.2780137142396,29.6763760610845));
#48302=CARTESIAN_POINT('Ctrl Pts',(-13.8414647957863,36.389378718253,29.6706264540062));
#48303=CARTESIAN_POINT('Ctrl Pts',(-13.8011415409952,36.5008676605382,29.664870448182));
#48304=CARTESIAN_POINT('Ctrl Pts',(-13.7559856700422,36.6105306188601,29.6591144423578));
#48305=CARTESIAN_POINT('Ctrl Pts',(-13.7062043603838,36.7179273090186,29.6533584365337));
#48306=CARTESIAN_POINT('Ctrl Pts',(-13.656393756972,36.8253871966339,29.6475990435946));
#48307=CARTESIAN_POINT('Ctrl Pts',(-13.6019524871551,36.9305777917755,29.6418396506555));
#48308=CARTESIAN_POINT('Ctrl Pts',(-13.5431331597973,37.0330844576516,29.6360802577164));
#48309=CARTESIAN_POINT('Ctrl Pts',(-13.4842168562484,37.1357601276029,29.6303113691912));
#48310=CARTESIAN_POINT('Ctrl Pts',(-13.4209083020718,37.2357426795967,29.624542480666));
#48311=CARTESIAN_POINT('Ctrl Pts',(-13.3535030157968,37.3326471064098,29.6187735921407));
#48312=CARTESIAN_POINT('Ctrl Pts',(-13.303134059545,37.4050594512641,29.6144627597149));
#48313=CARTESIAN_POINT('Ctrl Pts',(-13.2504784154346,37.4757536320588,29.610151927289));
#48314=CARTESIAN_POINT('Ctrl Pts',(-13.1956731526218,37.5445821074613,29.6058410948631));
#48315=CARTESIAN_POINT('Ctrl Pts',(-13.1215708848067,37.6376451794332,29.6000124126795));
#48316=CARTESIAN_POINT('Ctrl Pts',(-13.0432813170809,37.7276176964846,29.5941837304958));
#48317=CARTESIAN_POINT('Ctrl Pts',(-12.9610914531482,37.8141006389418,29.5883550483122));
#48318=CARTESIAN_POINT('Ctrl Pts',(-12.8790055816135,37.9004741570961,29.5825337409873));
#48319=CARTESIAN_POINT('Ctrl Pts',(-12.7930295079769,37.9833665900373,29.5767124336624));
#48320=CARTESIAN_POINT('Ctrl Pts',(-12.7034913998388,38.0624106927383,29.5708911263375));
#48321=CARTESIAN_POINT('Ctrl Pts',(-12.6140433636273,38.1413752800824,29.565075675026));
#48322=CARTESIAN_POINT('Ctrl Pts',(-12.5210407253993,38.2164989707507,29.5592602237146));
#48323=CARTESIAN_POINT('Ctrl Pts',(-12.4248491102627,38.287450652475,29.5534447724031));
#48324=CARTESIAN_POINT('Ctrl Pts',(-12.3251341209551,38.3610012023275,29.5474163086486));
#48325=CARTESIAN_POINT('Ctrl Pts',(-12.2219923741619,38.4300679393296,29.5413878448941));
#48326=CARTESIAN_POINT('Ctrl Pts',(-12.115869891107,38.4943267740592,29.5353593811396));
#48327=CARTESIAN_POINT('Ctrl Pts',(-12.0136144202408,38.55624407201,29.5295505894295));
#48328=CARTESIAN_POINT('Ctrl Pts',(-11.9085920261414,38.6136975053864,29.5237417977195));
#48329=CARTESIAN_POINT('Ctrl Pts',(-11.8012314361141,38.666441096425,29.5179330060095));
#48330=CARTESIAN_POINT('Ctrl Pts',(-11.6938876777556,38.7191764184828,29.5121251249842));
#48331=CARTESIAN_POINT('Ctrl Pts',(-11.5842068181623,38.7672031871182,29.506317243959));
#48332=CARTESIAN_POINT('Ctrl Pts',(-11.4726412539763,38.8103218679118,29.5005093629338));
#48333=CARTESIAN_POINT('Ctrl Pts',(-11.3610669851957,38.8534439129213,29.4947010287647));
#48334=CARTESIAN_POINT('Ctrl Pts',(-11.247608099589,38.8916569618532,29.4888926945956));
#48335=CARTESIAN_POINT('Ctrl Pts',(-11.132735395391,38.9248102532515,29.4830843604265));
#48336=CARTESIAN_POINT('Ctrl Pts',(-11.0178267568282,38.9579739156295,29.4772742093001));
#48337=CARTESIAN_POINT('Ctrl Pts',(-10.9015038114156,38.986074559665,29.4714640581737));
#48338=CARTESIAN_POINT('Ctrl Pts',(-10.7842502614603,39.0090119141005,29.4656539070474));
#48339=CARTESIAN_POINT('Ctrl Pts',(-10.6668694190319,39.0319741697229,29.4598374483209));
#48340=CARTESIAN_POINT('Ctrl Pts',(-10.5485563555924,39.0497618685147,29.4540209895943));
#48341=CARTESIAN_POINT('Ctrl Pts',(-10.4298028153473,39.0623262473513,29.4482045308678));
#48342=CARTESIAN_POINT('Ctrl Pts',(-10.3109726770349,39.0748987304275,29.4423843204258));
#48343=CARTESIAN_POINT('Ctrl Pts',(-10.1917019019098,39.0822411583369,29.4365641099838));
#48344=CARTESIAN_POINT('Ctrl Pts',(-10.0724835403599,39.0843568816127,29.4307438995418));
#48345=CARTESIAN_POINT('Ctrl Pts',(-9.95309723424697,39.0864755853373,29.4249154900885));
#48346=CARTESIAN_POINT('Ctrl Pts',(-9.83376389507452,39.0833528986784,29.4190870806351));
#48347=CARTESIAN_POINT('Ctrl Pts',(-9.71497289432271,39.0750441162065,29.4132586711818));
#48348=CARTESIAN_POINT('Ctrl Pts',(-9.68442101642287,39.0729071790145,29.4117596615528));
#48349=CARTESIAN_POINT('Ctrl Pts',(-9.65390496521215,39.0704274626179,29.4102606519237));
#48350=CARTESIAN_POINT('Ctrl Pts',(-9.6234329543552,39.0676064534483,29.4087616422947));
#48351=CARTESIAN_POINT('Ctrl Pts',(-9.50487383801798,39.0566305990523,29.4029293636888));
#48352=CARTESIAN_POINT('Ctrl Pts',(-9.38661074311595,39.0404499089252,29.397097085083));
#48353=CARTESIAN_POINT('Ctrl Pts',(-9.26913529492874,39.0190871827918,29.3912648064771));
#48354=CARTESIAN_POINT('Ctrl Pts',(-9.15179756714227,38.9977495008973,29.3854393652467));
#48355=CARTESIAN_POINT('Ctrl Pts',(-9.0352460465635,38.9712419363312,29.3796139240163));
#48356=CARTESIAN_POINT('Ctrl Pts',(-8.9199682526141,38.9396391236557,29.3737884827859));
#48357=CARTESIAN_POINT('Ctrl Pts',(-8.8047986408493,38.9080659685682,29.3679685084276));
#48358=CARTESIAN_POINT('Ctrl Pts',(-8.69090076818878,38.8714071838209,29.3621485340693));
#48359=CARTESIAN_POINT('Ctrl Pts',(-8.5787523465093,38.8297885199378,29.356328559711));
#48360=CARTESIAN_POINT('Ctrl Pts',(-8.46668726322049,38.7882007832173,29.3505129102223));
#48361=CARTESIAN_POINT('Ctrl Pts',(-8.35636942347186,38.7416606445584,29.3446972607336));
#48362=CARTESIAN_POINT('Ctrl Pts',(-8.24826109381904,38.6903435889592,29.3388816112449));
#48363=CARTESIAN_POINT('Ctrl Pts',(-8.14019930221163,38.6390486241226,29.3330684652539));
#48364=CARTESIAN_POINT('Ctrl Pts',(-8.03434549466983,38.5829810088661,29.327255319263));
#48365=CARTESIAN_POINT('Ctrl Pts',(-7.93114120708155,38.5223640207912,29.321442173272));
#48366=CARTESIAN_POINT('Ctrl Pts',(-7.82794611936189,38.4617524362546,29.3156295454783));
#48367=CARTESIAN_POINT('Ctrl Pts',(-7.72740043409766,38.3965924885014,29.3098169176846));
#48368=CARTESIAN_POINT('Ctrl Pts',(-7.62991994784687,38.3271527687177,29.3040042898909));
#48369=CARTESIAN_POINT('Ctrl Pts',(-7.59037621104445,38.2989839925003,29.3016463510619));
#48370=CARTESIAN_POINT('Ctrl Pts',(-7.55133655523326,38.2701114467194,29.2992884122329));
#48371=CARTESIAN_POINT('Ctrl Pts',(-7.51282733495086,38.2405550657615,29.2969304734038));
#48372=CARTESIAN_POINT('',(-11.0579044229731,31.0543614925016,30.));
#48373=CARTESIAN_POINT('Ctrl Pts',(-11.057904422973,31.0543614925016,30.));
#48374=CARTESIAN_POINT('Ctrl Pts',(-12.3607928946041,31.403691892172,29.9343068491439));
#48375=CARTESIAN_POINT('Ctrl Pts',(-13.8213065450876,32.7806934417622,29.8475124055188));
#48376=CARTESIAN_POINT('Ctrl Pts',(-14.0838324696554,34.5614760231763,29.7607179618936));
#48377=CARTESIAN_POINT('Ctrl Pts',(-14.0807388749966,34.9955823652123,29.7396166691247));
#48378=CARTESIAN_POINT('',(-8.94137326277089,31.0545552302404,29.9999998972464));
#48379=CARTESIAN_POINT('Origin',(-10.,35.,30.));
#48380=CARTESIAN_POINT('',(-14.0849993157578,35.0023643727775,29.6353849714467));
#48381=CARTESIAN_POINT('Ctrl Pts',(-8.94137326277089,31.0545552302404,29.9999998972464));
#48382=CARTESIAN_POINT('Ctrl Pts',(-9.05557900702206,31.0239119792345,29.9942072258419));
#48383=CARTESIAN_POINT('Ctrl Pts',(-9.17130906545843,30.9981799216732,29.9884145544374));
#48384=CARTESIAN_POINT('Ctrl Pts',(-9.28810103205902,30.9775101169245,29.9826218830329));
#48385=CARTESIAN_POINT('Ctrl Pts',(-9.40474625781243,30.9568662823238,29.9768364897104));
#48386=CARTESIAN_POINT('Ctrl Pts',(-9.52245033541758,30.9412721240102,29.9710510963879));
#48387=CARTESIAN_POINT('Ctrl Pts',(-9.64073638462371,30.9308287508798,29.9652657030654));
#48388=CARTESIAN_POINT('Ctrl Pts',(-9.75890552637127,30.9203956994078,29.959486027709));
#48389=CARTESIAN_POINT('Ctrl Pts',(-9.87765508648077,30.9151033438613,29.9537063523527));
#48390=CARTESIAN_POINT('Ctrl Pts',(-9.99649934938507,30.9150014999458,29.9479266769964));
#48391=CARTESIAN_POINT('Ctrl Pts',(-10.115260739166,30.9148997270486,29.9421510319545));
#48392=CARTESIAN_POINT('Ctrl Pts',(-10.2341162885532,30.9199812664573,29.9363753869126));
#48393=CARTESIAN_POINT('Ctrl Pts',(-10.3525771683274,30.9302439458397,29.9305997418708));
#48394=CARTESIAN_POINT('Ctrl Pts',(-10.4709944600259,30.940502849035,29.9248262219967));
#48395=CARTESIAN_POINT('Ctrl Pts',(-10.5890169597165,30.955939066815,29.9190527021227));
#48396=CARTESIAN_POINT('Ctrl Pts',(-10.7061584327085,30.9764983822652,29.9132791822487));
#48397=CARTESIAN_POINT('Ctrl Pts',(-10.8232852272653,30.9970551215263,29.9075063858267));
#48398=CARTESIAN_POINT('Ctrl Pts',(-10.9395308077791,31.0227336104439,29.9017335894047));
#48399=CARTESIAN_POINT('Ctrl Pts',(-11.0544173397038,31.0534281871817,29.8959607929827));
#48400=CARTESIAN_POINT('Ctrl Pts',(-11.1693173531074,31.0841263658064,29.8901873191459));
#48401=CARTESIAN_POINT('Ctrl Pts',(-11.2828576018,31.1198416953922,29.8844138453092));
#48402=CARTESIAN_POINT('Ctrl Pts',(-11.3945743500606,31.1604183324022,29.8786403714724));
#48403=CARTESIAN_POINT('Ctrl Pts',(-11.5064001388795,31.2010345740303,29.8728612624662));
#48404=CARTESIAN_POINT('Ctrl Pts',(-11.6163984829982,31.2465214596229,29.86708215346));
#48405=CARTESIAN_POINT('Ctrl Pts',(-11.7241244467073,31.2966744820005,29.8613030444537));
#48406=CARTESIAN_POINT('Ctrl Pts',(-11.8319025585855,31.3468517825391,29.8555211378865));
#48407=CARTESIAN_POINT('Ctrl Pts',(-11.9374057320661,31.4016995289724,29.8497392313193));
#48408=CARTESIAN_POINT('Ctrl Pts',(-12.0402141148433,31.4609674534424,29.8439573247521));
#48409=CARTESIAN_POINT('Ctrl Pts',(-12.1431866646754,31.5203300184499,29.8381661854886));
#48410=CARTESIAN_POINT('Ctrl Pts',(-12.2434554767513,31.5841266426451,29.832375046225));
#48411=CARTESIAN_POINT('Ctrl Pts',(-12.34062969668,31.6520636769765,29.8265839069615));
#48412=CARTESIAN_POINT('Ctrl Pts',(-12.4324683408004,31.7162704709508,29.8211107436239));
#48413=CARTESIAN_POINT('Ctrl Pts',(-12.5215429394954,31.7841749336168,29.8156375802863));
#48414=CARTESIAN_POINT('Ctrl Pts',(-12.6075527664519,31.85549788199,29.8101644169487));
#48415=CARTESIAN_POINT('Ctrl Pts',(-12.6979865222769,31.9304893373405,29.804409740601));
#48416=CARTESIAN_POINT('Ctrl Pts',(-12.7853423440294,32.0095178940369,29.7986550642532));
#48417=CARTESIAN_POINT('Ctrl Pts',(-12.8692326967171,32.092298376365,29.7929003879054));
#48418=CARTESIAN_POINT('Ctrl Pts',(-12.9530188019921,32.1749759904749,29.7871528626793));
#48419=CARTESIAN_POINT('Ctrl Pts',(-13.0333477040205,32.2613959694969,29.7814053374532));
#48420=CARTESIAN_POINT('Ctrl Pts',(-13.1098641070867,32.351232317576,29.7756578122272));
#48421=CARTESIAN_POINT('Ctrl Pts',(-13.1876742137717,32.4425875766853,29.769813110528));
#48422=CARTESIAN_POINT('Ctrl Pts',(-13.2615413720246,32.5374755234182,29.7639684088288));
#48423=CARTESIAN_POINT('Ctrl Pts',(-13.3311299036824,32.6355130440637,29.7581237071296));
#48424=CARTESIAN_POINT('Ctrl Pts',(-13.3994485329896,32.7317615044294,29.7523856638158));
#48425=CARTESIAN_POINT('Ctrl Pts',(-13.4636431121346,32.8310452079152,29.746647620502));
#48426=CARTESIAN_POINT('Ctrl Pts',(-13.5234363744694,32.9329680420792,29.7409095771881));
#48427=CARTESIAN_POINT('Ctrl Pts',(-13.5832097718704,33.0348570147297,29.735173440207));
#48428=CARTESIAN_POINT('Ctrl Pts',(-13.6385845473066,33.1393830141318,29.7294373032259));
#48429=CARTESIAN_POINT('Ctrl Pts',(-13.689327483289,33.2461220906093,29.7237011662447));
#48430=CARTESIAN_POINT('Ctrl Pts',(-13.7400662411507,33.352852378302,29.7179655015712));
#48431=CARTESIAN_POINT('Ctrl Pts',(-13.7861737388538,33.4617950019341,29.7122298368976));
#48432=CARTESIAN_POINT('Ctrl Pts',(-13.8274636895596,33.5725033432253,29.7064941722241));
#48433=CARTESIAN_POINT('Ctrl Pts',(-13.8701221485458,33.6868809861062,29.7005684054926));
#48434=CARTESIAN_POINT('Ctrl Pts',(-13.9076379799982,33.8031429876553,29.6946426387612));
#48435=CARTESIAN_POINT('Ctrl Pts',(-13.939860989921,33.9207778819453,29.6887168720297));
#48436=CARTESIAN_POINT('Ctrl Pts',(-13.9710834695739,34.0347601915507,29.6829751014241));
#48437=CARTESIAN_POINT('Ctrl Pts',(-13.9973369048824,34.1500309688985,29.6772333308184));
#48438=CARTESIAN_POINT('Ctrl Pts',(-14.0185365826894,34.2661139505434,29.6714915602128));
#48439=CARTESIAN_POINT('Ctrl Pts',(-14.040755282028,34.3877767838648,29.6654737954184));
#48440=CARTESIAN_POINT('Ctrl Pts',(-14.0574222060512,34.5103313261811,29.6594560306241));
#48441=CARTESIAN_POINT('Ctrl Pts',(-14.0685010044489,34.6332240782187,29.6534382658297));
#48442=CARTESIAN_POINT('Ctrl Pts',(-14.0795798028465,34.7561168302564,29.6474205010354));
#48443=CARTESIAN_POINT('Ctrl Pts',(-14.0850705173113,34.8793472663617,29.6414027362411));
#48444=CARTESIAN_POINT('Ctrl Pts',(-14.0849993157578,35.0023643727775,29.6353849714467));
#48445=CARTESIAN_POINT('Ctrl Pts',(-14.0849993157573,35.0023643736406,29.6353849714045));
#48446=CARTESIAN_POINT('Ctrl Pts',(-14.0849113652874,35.1543190406916,29.6279516357298));
#48447=CARTESIAN_POINT('Ctrl Pts',(-14.0763451188053,35.3060182549354,29.6205183000551));
#48448=CARTESIAN_POINT('Ctrl Pts',(-14.0593832670936,35.4567630576578,29.6130849643803));
#48449=CARTESIAN_POINT('Ctrl Pts',(-14.0461086957647,35.5747379503874,29.6072675367608));
#48450=CARTESIAN_POINT('Ctrl Pts',(-14.0276650664714,35.6923278959856,29.6014501091414));
#48451=CARTESIAN_POINT('Ctrl Pts',(-14.0040820227916,35.8090439757872,29.5956326815219));
#48452=CARTESIAN_POINT('Ctrl Pts',(-13.9805290796663,35.9256110833537,29.5898226790592));
#48453=CARTESIAN_POINT('Ctrl Pts',(-13.9518498489588,36.0413061458505,29.5840126765965));
#48454=CARTESIAN_POINT('Ctrl Pts',(-13.9181257430916,36.1556451277631,29.5782026741339));
#48455=CARTESIAN_POINT('Ctrl Pts',(-13.8844358370561,36.2698681577824,29.5723985636319));
#48456=CARTESIAN_POINT('Ctrl Pts',(-13.8457113481323,36.3827374525738,29.5665944531299));
#48457=CARTESIAN_POINT('Ctrl Pts',(-13.8020846470484,36.4937795475501,29.5607903426279));
#48458=CARTESIAN_POINT('Ctrl Pts',(-13.756739739236,36.6091949568039,29.5547576413439));
#48459=CARTESIAN_POINT('Ctrl Pts',(-13.7060986387152,36.7226358434001,29.5487249400599));
#48460=CARTESIAN_POINT('Ctrl Pts',(-13.6503671389336,36.8335879447121,29.5426922387759));
#48461=CARTESIAN_POINT('Ctrl Pts',(-13.5968090770892,36.9402130943514,29.5368948030399));
#48462=CARTESIAN_POINT('Ctrl Pts',(-13.5385504059576,37.0445395351898,29.5310973673038));
#48463=CARTESIAN_POINT('Ctrl Pts',(-13.475822392104,37.1461322649241,29.5252999315678));
#48464=CARTESIAN_POINT('Ctrl Pts',(-13.4131040737471,37.2477092920733,29.5195033919069));
#48465=CARTESIAN_POINT('Ctrl Pts',(-13.3459180013724,37.346553100151,29.5137068522461));
#48466=CARTESIAN_POINT('Ctrl Pts',(-13.274540196362,37.4422554130167,29.5079103125853));
#48467=CARTESIAN_POINT('Ctrl Pts',(-13.2031564756587,37.5379656575567,29.5021132925153));
#48468=CARTESIAN_POINT('Ctrl Pts',(-13.1275805764068,37.6305335611139,29.4963162724454));
#48469=CARTESIAN_POINT('Ctrl Pts',(-13.0481300393714,37.7195823692401,29.4905192523754));
#48470=CARTESIAN_POINT('Ctrl Pts',(-12.9686540526691,37.80865970156,29.4847203753988));
#48471=CARTESIAN_POINT('Ctrl Pts',(-12.8853012324082,37.8942153914736,29.4789214984222));
#48472=CARTESIAN_POINT('Ctrl Pts',(-12.7984268784555,37.9759086017446,29.4731226214456));
#48473=CARTESIAN_POINT('Ctrl Pts',(-12.7114562804842,38.0576923160884,29.4673173201655));
#48474=CARTESIAN_POINT('Ctrl Pts',(-12.6209566598982,38.1356047289336,29.4615120188853));
#48475=CARTESIAN_POINT('Ctrl Pts',(-12.5273174902497,38.2093443728398,29.4557067176051));
#48476=CARTESIAN_POINT('Ctrl Pts',(-12.4336169181786,38.2831323703653,29.4498976095893));
#48477=CARTESIAN_POINT('Ctrl Pts',(-12.3367730289423,38.3527419116578,29.4440885015735));
#48478=CARTESIAN_POINT('Ctrl Pts',(-12.2372040492131,38.4179150138914,29.4382793935577));
#48479=CARTESIAN_POINT('Ctrl Pts',(-12.1374916958428,38.4831819616681,29.4324619207583));
#48480=CARTESIAN_POINT('Ctrl Pts',(-12.0350467707998,38.543999511847,29.4266444479589));
#48481=CARTESIAN_POINT('Ctrl Pts',(-11.9303119364292,38.6001556672009,29.4208269751595));
#48482=CARTESIAN_POINT('Ctrl Pts',(-11.9013775415724,38.6156695540793,29.4192198207103));
#48483=CARTESIAN_POINT('Ctrl Pts',(-11.8722684918198,38.6308279610645,29.4176126662611));
#48484=CARTESIAN_POINT('Ctrl Pts',(-11.8429943645596,38.6456270753057,29.4160055118119));
#48485=CARTESIAN_POINT('Ctrl Pts',(-11.7368983395956,38.6992623956694,29.4101808224181));
#48486=CARTESIAN_POINT('Ctrl Pts',(-11.6282883268288,38.7483487055701,29.4043561330244));
#48487=CARTESIAN_POINT('Ctrl Pts',(-11.5175910307645,38.792643202747,29.3985314436306));
#48488=CARTESIAN_POINT('Ctrl Pts',(-11.407033319077,38.8368818465291,29.3927140989116));
#48489=CARTESIAN_POINT('Ctrl Pts',(-11.2943939346871,38.8763405453162,29.3868967541926));
#48490=CARTESIAN_POINT('Ctrl Pts',(-11.1801237564454,38.9108225374559,29.3810794094736));
#48491=CARTESIAN_POINT('Ctrl Pts',(-11.0659679166969,38.9452700269888,29.3752678855772));
#48492=CARTESIAN_POINT('Ctrl Pts',(-10.9501849178431,38.9747505991847,29.3694563616807));
#48493=CARTESIAN_POINT('Ctrl Pts',(-10.8332446195773,38.9991159528008,29.3636448377843));
#48494=CARTESIAN_POINT('Ctrl Pts',(-10.7119091386374,39.0243970743912,29.3576148886784));
#48495=CARTESIAN_POINT('Ctrl Pts',(-10.589328073091,39.044170756343,29.3515849395726));
#48496=CARTESIAN_POINT('Ctrl Pts',(-10.466042848905,39.0583283582018,29.3455549904667));
#48497=CARTESIAN_POINT('Ctrl Pts',(-10.3473572312565,39.0719577589034,29.3397500106831));
#48498=CARTESIAN_POINT('Ctrl Pts',(-10.2280194980236,39.0803825800956,29.3339450308994));
#48499=CARTESIAN_POINT('Ctrl Pts',(-10.1085213539266,39.0835582664806,29.3281400511158));
#48500=CARTESIAN_POINT('Ctrl Pts',(-9.98904092901901,39.0867334819747,29.3223359320948));
#48501=CARTESIAN_POINT('Ctrl Pts',(-9.86940054845317,39.0846610997186,29.3165318130738));
#48502=CARTESIAN_POINT('Ctrl Pts',(-9.75009403409503,39.0773486493315,29.3107276940528));
#48503=CARTESIAN_POINT('Ctrl Pts',(-9.63077708468077,39.0700355593662,29.3049230673789));
#48504=CARTESIAN_POINT('Ctrl Pts',(-9.51179446694682,39.0574815149923,29.2991184407049));
#48505=CARTESIAN_POINT('Ctrl Pts',(-9.39363635173109,39.0397460472235,29.2933138140309));
#48506=CARTESIAN_POINT('Ctrl Pts',(-9.27544004699479,39.0220048472288,29.2875073112614));
#48507=CARTESIAN_POINT('Ctrl Pts',(-9.15806917818911,38.9990789538252,29.2817008084919));
#48508=CARTESIAN_POINT('Ctrl Pts',(-9.04200454416728,38.9710791614628,29.2758943057224));
#48509=CARTESIAN_POINT('Ctrl Pts',(-8.92581168937801,38.9430484367246,29.2700813883009));
#48510=CARTESIAN_POINT('Ctrl Pts',(-8.81092834683337,38.9099327200765,29.2642684708794));
#48511=CARTESIAN_POINT('Ctrl Pts',(-8.69782110222245,38.8718929631619,29.2584555534578));
#48512=CARTESIAN_POINT('Ctrl Pts',(-8.58463972000513,38.8338282725966,29.2526388258844));
#48513=CARTESIAN_POINT('Ctrl Pts',(-8.47323713413662,38.7908332606018,29.246822098311));
#48514=CARTESIAN_POINT('Ctrl Pts',(-8.36405932425061,38.7431167635312,29.2410053707375));
#48515=CARTESIAN_POINT('Ctrl Pts',(-8.25472550561882,38.6953320823593,29.2351803313984));
#48516=CARTESIAN_POINT('Ctrl Pts',(-8.14762317343606,38.6428126290242,29.2293552920593));
#48517=CARTESIAN_POINT('Ctrl Pts',(-8.04317324693783,38.5858128867106,29.2235302527202));
#48518=CARTESIAN_POINT('Ctrl Pts',(-8.01565368056036,38.5707950858879,29.2219955215613));
#48519=CARTESIAN_POINT('Ctrl Pts',(-7.98831807609793,38.5554665065085,29.2204607904023));
#48520=CARTESIAN_POINT('Ctrl Pts',(-7.96117377535177,38.5398322877909,29.2189260592434));
#48521=CARTESIAN_POINT('Ctrl Pts',(-7.85816140270912,38.4805005709941,29.2131017685561));
#48522=CARTESIAN_POINT('Ctrl Pts',(-7.75757564042123,38.4165731977983,29.2072774778688));
#48523=CARTESIAN_POINT('Ctrl Pts',(-7.65985336587902,38.3482739927927,29.2014531871815));
#48524=CARTESIAN_POINT('Ctrl Pts',(-7.61008379849843,38.3134894781927,29.1984868990024));
#48525=CARTESIAN_POINT('Ctrl Pts',(-7.56105664497159,38.2775717555271,29.1955206108233));
#48526=CARTESIAN_POINT('Ctrl Pts',(-7.51282733495086,38.2405550657615,29.1925543226443));
#48527=CARTESIAN_POINT('Origin',(-10.,35.,23.));
#48528=CARTESIAN_POINT('',(-13.1787500078856,36.1772652419347,17.9149433153638));
#48529=CARTESIAN_POINT('',(-13.1787500671536,36.1772650819042,17.5703580226472));
#48530=CARTESIAN_POINT('',(-13.1787500671536,36.1772650819043,23.));
#48531=CARTESIAN_POINT('',(-6.62123117139838,34.7273715616997,17.));
#48532=CARTESIAN_POINT('Ctrl Pts',(-13.1787500671536,36.1772650819042,17.5703580226472));
#48533=CARTESIAN_POINT('Ctrl Pts',(-13.1427559868796,36.2744532061821,17.5642606450182));
#48534=CARTESIAN_POINT('Ctrl Pts',(-13.1022540729216,36.3701148704846,17.5581632673893));
#48535=CARTESIAN_POINT('Ctrl Pts',(-13.0573974094917,36.4638053637467,17.5520658897603));
#48536=CARTESIAN_POINT('Ctrl Pts',(-13.0125843104849,36.5574048655711,17.5459744338544));
#48537=CARTESIAN_POINT('Ctrl Pts',(-12.9634250562128,36.6490366202576,17.5398829779485));
#48538=CARTESIAN_POINT('Ctrl Pts',(-12.9101211932366,36.7382749216321,17.5337915220426));
#48539=CARTESIAN_POINT('Ctrl Pts',(-12.8568511675345,36.8274565745633,17.5277039329908));
#48540=CARTESIAN_POINT('Ctrl Pts',(-12.7994419829177,36.9142474296897,17.521616343939));
#48541=CARTESIAN_POINT('Ctrl Pts',(-12.7381412063363,36.9982461801949,17.5155287548873));
#48542=CARTESIAN_POINT('Ctrl Pts',(-12.6768600667662,37.0822180226491,17.5094431159259));
#48543=CARTESIAN_POINT('Ctrl Pts',(-12.6116900644843,37.1633991936884,17.5033574769645));
#48544=CARTESIAN_POINT('Ctrl Pts',(-12.5429217250004,37.2414178912066,17.4972718380031));
#48545=CARTESIAN_POINT('Ctrl Pts',(-12.4741576889056,37.3194317064662,17.4911865798692));
#48546=CARTESIAN_POINT('Ctrl Pts',(-12.401796045861,37.3942831216331,17.4851013217353));
#48547=CARTESIAN_POINT('Ctrl Pts',(-12.3261665912132,37.4656346145412,17.4790160636014));
#48548=CARTESIAN_POINT('Ctrl Pts',(-12.2505223753453,37.5370000337045,17.4729296177578));
#48549=CARTESIAN_POINT('Ctrl Pts',(-12.1716093909688,37.604863880215,17.4668431719142));
#48550=CARTESIAN_POINT('Ctrl Pts',(-12.0897924734438,37.6689272152754,17.4607567260706));
#48551=CARTESIAN_POINT('Ctrl Pts',(-12.0078881301222,37.7330590054704,17.4546637765309));
#48552=CARTESIAN_POINT('Ctrl Pts',(-11.9230739945184,37.7933819118439,17.4485708269911));
#48553=CARTESIAN_POINT('Ctrl Pts',(-11.8357459700176,37.8496388887128,17.4424778774513));
#48554=CARTESIAN_POINT('Ctrl Pts',(-11.7483675492014,37.9059283310401,17.4363814117183));
#48555=CARTESIAN_POINT('Ctrl Pts',(-11.6584727190608,37.9581469561964,17.4302849459853));
#48556=CARTESIAN_POINT('Ctrl Pts',(-11.5664824782971,38.0060834498876,17.4241884802523));
#48557=CARTESIAN_POINT('Ctrl Pts',(-11.4743456381263,38.0540963371342,17.4180822989423));
#48558=CARTESIAN_POINT('Ctrl Pts',(-11.380107105204,38.0978132841681,17.4119761176324));
#48559=CARTESIAN_POINT('Ctrl Pts',(-11.2842084864572,38.1370708671962,17.4058699363224));
#48560=CARTESIAN_POINT('Ctrl Pts',(-11.2229005725148,38.1621682101333,17.4019662592606));
#48561=CARTESIAN_POINT('Ctrl Pts',(-11.1609145333314,38.1854439917115,17.3980625821987));
#48562=CARTESIAN_POINT('Ctrl Pts',(-11.0983685544785,38.2068663179236,17.3941589051368));
#48563=CARTESIAN_POINT('Ctrl Pts',(-11.0015155370981,38.2400389849919,17.3881140256857));
#48564=CARTESIAN_POINT('Ctrl Pts',(-10.902977197853,38.2688819196769,17.3820691462345));
#48565=CARTESIAN_POINT('Ctrl Pts',(-10.8031806010433,38.2932212170772,17.3760242667834));
#48566=CARTESIAN_POINT('Ctrl Pts',(-10.7035168525737,38.3175281142219,17.3699874342218));
#48567=CARTESIAN_POINT('Ctrl Pts',(-10.6025985948985,38.3373431845761,17.3639506016603));
#48568=CARTESIAN_POINT('Ctrl Pts',(-10.5008707652887,38.3525413552974,17.3579137690988));
#48569=CARTESIAN_POINT('Ctrl Pts',(-10.3992478574947,38.3677238506653,17.3518831629105));
#48570=CARTESIAN_POINT('Ctrl Pts',(-10.2968174665736,38.3782988468126,17.3458525567222));
#48571=CARTESIAN_POINT('Ctrl Pts',(-10.1940365532007,38.3841919092336,17.3398219505339));
#48572=CARTESIAN_POINT('Ctrl Pts',(-10.0913245511466,38.3900810205445,17.3337953876744));
#48573=CARTESIAN_POINT('Ctrl Pts',(-9.98826292812799,38.3912944108315,17.3277688248149));
#48574=CARTESIAN_POINT('Ctrl Pts',(-9.88531472849353,38.3878093734742,17.3217422619554));
#48575=CARTESIAN_POINT('Ctrl Pts',(-9.78240185029908,38.3843255318302,17.3157177668045));
#48576=CARTESIAN_POINT('Ctrl Pts',(-9.67960275408466,38.3761464790843,17.3096932716536));
#48577=CARTESIAN_POINT('Ctrl Pts',(-9.5773804931766,38.3633016241414,17.3036687765027));
#48578=CARTESIAN_POINT('Ctrl Pts',(-9.47516557914334,38.3504576923785,17.2976447143417));
#48579=CARTESIAN_POINT('Ctrl Pts',(-9.37352785126157,38.3329486791751,17.2916206521807));
#48580=CARTESIAN_POINT('Ctrl Pts',(-9.27292421516466,38.3108557603143,17.2855965900198));
#48581=CARTESIAN_POINT('Ctrl Pts',(-9.17230052182162,38.2887584368103,17.2795713268476));
#48582=CARTESIAN_POINT('Ctrl Pts',(-9.07271175622782,38.2620754860212,17.2735460636754));
#48583=CARTESIAN_POINT('Ctrl Pts',(-8.97460260719551,38.2309387566665,17.2675208005032));
#48584=CARTESIAN_POINT('Ctrl Pts',(-8.87637753594343,38.1997652372793,17.2614884180981));
#48585=CARTESIAN_POINT('Ctrl Pts',(-8.77963598915772,38.1641275636369,17.255456035693));
#48586=CARTESIAN_POINT('Ctrl Pts',(-8.68480545078267,38.1242068369762,17.2494236532879));
#48587=CARTESIAN_POINT('Ctrl Pts',(-8.58991797440138,38.0842621411742,17.2433876489291));
#48588=CARTESIAN_POINT('Ctrl Pts',(-8.49694418404904,38.0400294616795,17.2373516445702));
#48589=CARTESIAN_POINT('Ctrl Pts',(-8.40628759282379,37.9917362560414,17.2313156402113));
#48590=CARTESIAN_POINT('Ctrl Pts',(-8.31546419781163,37.9433541932174,17.2252685298934));
#48591=CARTESIAN_POINT('Ctrl Pts',(-8.22696689339884,37.8908969041228,17.2192214195756));
#48592=CARTESIAN_POINT('Ctrl Pts',(-8.14117103419852,37.8346357682068,17.2131743092577));
#48593=CARTESIAN_POINT('Ctrl Pts',(-8.06505357281228,37.7847212982015,17.2078093570279));
#48594=CARTESIAN_POINT('Ctrl Pts',(-7.99106216092855,37.731813522163,17.2024444047982));
#48595=CARTESIAN_POINT('Ctrl Pts',(-7.91943573511002,37.6761273142664,17.1970794525685));
#48596=CARTESIAN_POINT('Ctrl Pts',(-7.83581618354862,37.6111170100491,17.1908161929618));
#48597=CARTESIAN_POINT('Ctrl Pts',(-7.75512934647832,37.5420931533284,17.1845529333551));
#48598=CARTESIAN_POINT('Ctrl Pts',(-7.67777110567854,37.469343642525,17.1782896737485));
#48599=CARTESIAN_POINT('Ctrl Pts',(-7.60052564249751,37.3967001904493,17.1720355451083));
#48600=CARTESIAN_POINT('Ctrl Pts',(-7.52659940702115,37.3203421665363,17.1657814164681));
#48601=CARTESIAN_POINT('Ctrl Pts',(-7.45635611458709,37.2405983233729,17.1595272878279));
#48602=CARTESIAN_POINT('Ctrl Pts',(-7.38619919224281,37.1609525320328,17.1532808491697));
#48603=CARTESIAN_POINT('Ctrl Pts',(-7.31971646168714,37.077929507357,17.1470344105115));
#48604=CARTESIAN_POINT('Ctrl Pts',(-7.25723519115291,36.991895144291,17.1407879718533));
#48605=CARTESIAN_POINT('Ctrl Pts',(-7.1948270975312,36.9059615430854,17.1345488489089));
#48606=CARTESIAN_POINT('Ctrl Pts',(-7.13641136175374,36.817023952268,17.1283097259645));
#48607=CARTESIAN_POINT('Ctrl Pts',(-7.0822748183824,36.7254810422182,17.1220706030201));
#48608=CARTESIAN_POINT('Ctrl Pts',(-7.0281753355621,36.6340008002016,17.1158357512265));
#48609=CARTESIAN_POINT('Ctrl Pts',(-6.97834941786856,36.5399191321524,17.1096008994328));
#48610=CARTESIAN_POINT('Ctrl Pts',(-6.93304034137542,36.4436632276502,17.1033660476391));
#48611=CARTESIAN_POINT('Ctrl Pts',(-6.88775292182805,36.3474533317861,17.0971341759954));
#48612=CARTESIAN_POINT('Ctrl Pts',(-6.84697821549959,36.249071629913,17.0909023043518));
#48613=CARTESIAN_POINT('Ctrl Pts',(-6.8109130642717,36.1489689198873,17.0846704327082));
#48614=CARTESIAN_POINT('Ctrl Pts',(-6.77485770566963,36.048893390349,17.0784402531796));
#48615=CARTESIAN_POINT('Ctrl Pts',(-6.74350949055321,35.9470981596222,17.0722100736511));
#48616=CARTESIAN_POINT('Ctrl Pts',(-6.71701651636321,35.8440524324164,17.0659798941226));
#48617=CARTESIAN_POINT('Ctrl Pts',(-6.69051805353856,35.740985356896,17.0597484238677));
#48618=CARTESIAN_POINT('Ctrl Pts',(-6.66887694611004,35.6366676536819,17.0535169536129));
#48619=CARTESIAN_POINT('Ctrl Pts',(-6.65219090412263,35.5315819034361,17.047285483358));
#48620=CARTESIAN_POINT('Ctrl Pts',(-6.63550340623277,35.4264869841735,17.0410534693905));
#48621=CARTESIAN_POINT('Ctrl Pts',(-6.62377189134541,35.3206242807345,17.034821455423));
#48622=CARTESIAN_POINT('Ctrl Pts',(-6.61704244698939,35.2144836987476,17.0285894414554));
#48623=CARTESIAN_POINT('Ctrl Pts',(-6.61030846998724,35.1082716253162,17.0223532298881));
#48624=CARTESIAN_POINT('Ctrl Pts',(-6.60858331255194,35.0017816995389,17.0161170183208));
#48625=CARTESIAN_POINT('Ctrl Pts',(-6.61186097188341,34.8955060353267,17.0098808067535));
#48626=CARTESIAN_POINT('Ctrl Pts',(-6.61359203986214,34.8393774445761,17.0065872045023));
#48627=CARTESIAN_POINT('Ctrl Pts',(-6.61671768475108,34.7833086021908,17.0032936022512));
#48628=CARTESIAN_POINT('Ctrl Pts',(-6.62123117139838,34.7273715616998,17.));
#48629=CARTESIAN_POINT('',(-13.1787500671536,36.1772650819043,17.));
#48630=CARTESIAN_POINT('Origin',(-10.,35.,17.));
#48631=CARTESIAN_POINT('',(-13.1787500671536,36.1772650819043,16.));
#48632=CARTESIAN_POINT('',(-13.1787500671536,36.1772650819043,23.));
#48633=CARTESIAN_POINT('Origin',(-10.,35.,16.));
#48634=CARTESIAN_POINT('',(-10.7859693978642,31.6996294197336,16.9983166722812));
#48635=CARTESIAN_POINT('Origin',(-10.,35.,17.));
#48636=CARTESIAN_POINT('Ctrl Pts',(-10.7851701022683,31.7024383291583,16.996642740892));
#48637=CARTESIAN_POINT('Ctrl Pts',(-10.7411264267437,31.6919512539592,16.999386876595));
#48638=CARTESIAN_POINT('Ctrl Pts',(-10.6968789035782,31.6823480701864,17.0021729732053));
#48639=CARTESIAN_POINT('Ctrl Pts',(-10.4988382553133,31.6435031285275,17.0147342295983));
#48640=CARTESIAN_POINT('Ctrl Pts',(-10.3433284096488,31.6240511354772,17.0248328987275));
#48641=CARTESIAN_POINT('Ctrl Pts',(-10.021322125722,31.6062561466042,17.045626997098));
#48642=CARTESIAN_POINT('Ctrl Pts',(-9.85514091465291,31.6092808843973,17.0562905526885));
#48643=CARTESIAN_POINT('Ctrl Pts',(-9.59130494280269,31.6335234341404,17.0728388515459));
#48644=CARTESIAN_POINT('Ctrl Pts',(-9.49320747682181,31.6468879567694,17.0789100101203));
#48645=CARTESIAN_POINT('Ctrl Pts',(-9.35840574527622,31.6713053283894,17.0871363837311));
#48646=CARTESIAN_POINT('Ctrl Pts',(-9.32109954833055,31.678713237895,17.0894007906279));
#48647=CARTESIAN_POINT('Ctrl Pts',(-9.25714978418302,31.6925343532475,17.0932628810753));
#48648=CARTESIAN_POINT('Ctrl Pts',(-9.23044539200801,31.6986455480178,17.0948697313219));
#48649=CARTESIAN_POINT('Ctrl Pts',(-9.17591691225517,31.7118217782151,17.098139777934));
#48650=CARTESIAN_POINT('Ctrl Pts',(-9.14810257201344,31.7189178921617,17.0998018599688));
#48651=CARTESIAN_POINT('Ctrl Pts',(-9.07702610942875,31.7380159989879,17.1040358879454));
#48652=CARTESIAN_POINT('Ctrl Pts',(-9.03390552350392,31.7505258659306,17.1065918591574));
#48653=CARTESIAN_POINT('Ctrl Pts',(-8.81646979273867,31.818318018793,17.1194352130547));
#48654=CARTESIAN_POINT('Ctrl Pts',(-8.64657820423122,31.8867857793393,17.1293003925232));
#48655=CARTESIAN_POINT('Ctrl Pts',(-8.35934160216759,32.0305263578168,17.1464422259585));
#48656=CARTESIAN_POINT('Ctrl Pts',(-8.23956527355586,32.0999308126459,17.1537539082429));
#48657=CARTESIAN_POINT('Ctrl Pts',(-8.06417273695908,32.2164411131496,17.1651453164485));
#48658=CARTESIAN_POINT('Ctrl Pts',(-8.00527557065218,32.2583397943134,17.1690994156838));
#48659=CARTESIAN_POINT('Ctrl Pts',(-7.9096309651066,32.3310942205926,17.175815982098));
#48660=CARTESIAN_POINT('Ctrl Pts',(-7.8721176974738,32.3609059877608,17.1785303817331));
#48661=CARTESIAN_POINT('Ctrl Pts',(-7.81948420685802,32.4045856350584,17.1824749404527));
#48662=CARTESIAN_POINT('Ctrl Pts',(-7.80383698835832,32.4178123941095,17.1836653466823));
#48663=CARTESIAN_POINT('Ctrl Pts',(-7.77685357372822,32.4410444290983,17.1857511697483));
#48664=CARTESIAN_POINT('Ctrl Pts',(-7.76546280953573,32.4509850560138,17.186642134439));
#48665=CARTESIAN_POINT('Ctrl Pts',(-7.74059935982598,32.4729779299354,17.1886106717852));
#48666=CARTESIAN_POINT('Ctrl Pts',(-7.72715655682884,32.4850617410864,17.1896903936014));
#48667=CARTESIAN_POINT('Ctrl Pts',(-7.68771597842631,32.5210895826394,17.1929024025501));
#48668=CARTESIAN_POINT('Ctrl Pts',(-7.66199607375009,32.5453326733591,17.1950545426587));
#48669=CARTESIAN_POINT('Ctrl Pts',(-7.50555211679663,32.6974832505138,17.2084799205615));
#48670=CARTESIAN_POINT('Ctrl Pts',(-7.38498718494906,32.835386398258,17.2202835065605));
#48671=CARTESIAN_POINT('Ctrl Pts',(-7.18123271787017,33.1104549616444,17.2423263602993));
#48672=CARTESIAN_POINT('Ctrl Pts',(-7.09547533081672,33.2451286740339,17.2525469084595));
#48673=CARTESIAN_POINT('Ctrl Pts',(-6.97367055807644,33.469968232975,17.2684982720421));
#48674=CARTESIAN_POINT('Ctrl Pts',(-6.93144998863293,33.5565074950471,17.2743984365352));
#48675=CARTESIAN_POINT('Ctrl Pts',(-6.87798031957433,33.679090023124,17.2824270095669));
#48676=CARTESIAN_POINT('Ctrl Pts',(-6.86356451819029,33.7136941698809,17.284658445714));
#48677=CARTESIAN_POINT('Ctrl Pts',(-6.83970828396745,33.7737465691577,17.2884724309912));
#48678=CARTESIAN_POINT('Ctrl Pts',(-6.82999426406078,33.7990816411739,17.2900638451231));
#48679=CARTESIAN_POINT('Ctrl Pts',(-6.81069030079557,33.8512951102679,17.2933085782584));
#48680=CARTESIAN_POINT('Ctrl Pts',(-6.80113347061025,33.8781834908117,17.2949607148208));
#48681=CARTESIAN_POINT('Ctrl Pts',(-6.77744749324618,33.9475896671186,17.2991791018446));
#48682=CARTESIAN_POINT('Ctrl Pts',(-6.76381944918456,33.9902733672679,17.3017291516867));
#48683=CARTESIAN_POINT('Ctrl Pts',(-6.70058920045596,34.202763963745,17.3142250995888));
#48684=CARTESIAN_POINT('Ctrl Pts',(-6.66348371290786,34.3760085691405,17.3237717318427));
#48685=CARTESIAN_POINT('Ctrl Pts',(-6.61570910217244,34.7338105861568,17.3429884947556));
#48686=CARTESIAN_POINT('Ctrl Pts',(-6.60625019359733,34.9179185846505,17.3526186824546));
#48687=CARTESIAN_POINT('Ctrl Pts',(-6.61349238013712,35.1587867714413,17.3657576428875));
#48688=CARTESIAN_POINT('Ctrl Pts',(-6.61663722798599,35.2156451851466,17.3689000751842));
#48689=CARTESIAN_POINT('Ctrl Pts',(-6.62445738252534,35.3126465183482,17.3743701434751));
#48690=CARTESIAN_POINT('Ctrl Pts',(-6.62842133460257,35.3528353921515,17.3766686402334));
#48691=CARTESIAN_POINT('Ctrl Pts',(-6.63529971133893,35.4117723167526,17.380099017414));
#48692=CARTESIAN_POINT('Ctrl Pts',(-6.6376552271799,35.4305834016102,17.3812028673973));
#48693=CARTESIAN_POINT('Ctrl Pts',(-6.64194964881517,35.4626915286908,17.3831038201127));
#48694=CARTESIAN_POINT('Ctrl Pts',(-6.64381002726752,35.4759983936192,17.3838966491269));
#48695=CARTESIAN_POINT('Ctrl Pts',(-6.64833952165301,35.5070493591057,17.3857586777808));
#48696=CARTESIAN_POINT('Ctrl Pts',(-6.65107038291607,35.5247831959168,17.3868311454087));
#48697=CARTESIAN_POINT('Ctrl Pts',(-6.65943965434514,35.5764041635967,17.3899776426211));
#48698=CARTESIAN_POINT('Ctrl Pts',(-6.66545241734355,35.6102273395331,17.3920703653927));
#48699=CARTESIAN_POINT('Ctrl Pts',(-6.7083393281207,35.83187215234,17.4059632924908));
#48700=CARTESIAN_POINT('Ctrl Pts',(-6.76054939127837,36.0163615608002,17.4183557835258));
#48701=CARTESIAN_POINT('Ctrl Pts',(-6.88280270999425,36.3407449535208,17.4407017782544));
#48702=CARTESIAN_POINT('Ctrl Pts',(-6.94748646663371,36.4821215789602,17.4506519561146));
#48703=CARTESIAN_POINT('Ctrl Pts',(-7.06686039490361,36.7017830791203,17.4662438555088));
#48704=CARTESIAN_POINT('Ctrl Pts',(-7.11554988678168,36.7830658251065,17.4720479250566));
#48705=CARTESIAN_POINT('Ctrl Pts',(-7.18793324557844,36.8931607855543,17.4799555951851));
#48706=CARTESIAN_POINT('Ctrl Pts',(-7.20878951179149,36.9237778889776,17.4821601563955));
#48707=CARTESIAN_POINT('Ctrl Pts',(-7.24560880572158,36.9759691057734,17.4859290340767));
#48708=CARTESIAN_POINT('Ctrl Pts',(-7.26133352942859,36.9977063805835,17.4875021059801));
#48709=CARTESIAN_POINT('Ctrl Pts',(-7.29412165692374,37.0419166143423,17.4907094090485));
#48710=CARTESIAN_POINT('Ctrl Pts',(-7.31121094112717,37.0643678293169,17.4923424739859));
#48711=CARTESIAN_POINT('Ctrl Pts',(-7.35582814436308,37.1214900054473,17.4965104496895));
#48712=CARTESIAN_POINT('Ctrl Pts',(-7.38375895943528,37.1558403742924,17.4990293864204));
#48713=CARTESIAN_POINT('Ctrl Pts',(-7.51973144955706,37.3165285553142,17.5108904132821));
#48714=CARTESIAN_POINT('Ctrl Pts',(-7.63630078101025,37.435358478565,17.5198810883679));
#48715=CARTESIAN_POINT('Ctrl Pts',(-7.94683299614805,37.7085200222348,17.541911912794));
#48716=CARTESIAN_POINT('Ctrl Pts',(-8.14983486907573,37.8510416720303,17.5547004283059));
#48717=CARTESIAN_POINT('Ctrl Pts',(-8.40493313337227,37.9913358579405,17.5710015945399));
#48718=CARTESIAN_POINT('Ctrl Pts',(-8.4437668968697,38.0117215469657,17.5734903196969));
#48719=CARTESIAN_POINT('Ctrl Pts',(-8.50039306296983,38.0400597211273,17.577145143416));
#48720=CARTESIAN_POINT('Ctrl Pts',(-8.51787715361973,38.0486219677823,17.5782771145932));
#48721=CARTESIAN_POINT('Ctrl Pts',(-8.5487213565273,38.0633988398235,17.5802818418297));
#48722=CARTESIAN_POINT('Ctrl Pts',(-8.56204971772011,38.0696776903511,17.5811507330038));
#48723=CARTESIAN_POINT('Ctrl Pts',(-8.59184229922979,38.0834760480281,17.5830989460335));
#48724=CARTESIAN_POINT('Ctrl Pts',(-8.60832596063734,38.0909506603511,17.584180758451));
#48725=CARTESIAN_POINT('Ctrl Pts',(-8.65672487555514,38.1124318079675,17.5873668344585));
#48726=CARTESIAN_POINT('Ctrl Pts',(-8.68879634279656,38.1260781476977,17.5894903052495));
#48727=CARTESIAN_POINT('Ctrl Pts',(-8.88737486137295,38.2069795294698,17.6026882856611));
#48728=CARTESIAN_POINT('Ctrl Pts',(-9.05878728590457,38.2614048484046,17.6142793958227));
#48729=CARTESIAN_POINT('Ctrl Pts',(-9.39241175343074,38.338830877452,17.6363558036028));
#48730=CARTESIAN_POINT('Ctrl Pts',(-9.55359663419627,38.3641770308464,17.6468164142448));
#48731=CARTESIAN_POINT('Ctrl Pts',(-9.81317234771921,38.3860023173606,17.6630794146817));
#48732=CARTESIAN_POINT('Ctrl Pts',(-9.91066852454422,38.3899762481629,17.6690615626971));
#48733=CARTESIAN_POINT('Ctrl Pts',(-10.045797604665,38.3896490416361,17.6771748634721));
#48734=CARTESIAN_POINT('Ctrl Pts',(-10.0833841255746,38.3889327677104,17.679412796351));
#48735=CARTESIAN_POINT('Ctrl Pts',(-10.1480187572473,38.3866250229969,17.6832302743005));
#48736=CARTESIAN_POINT('Ctrl Pts',(-10.1750733932721,38.3853342477687,17.6848188640769));
#48737=CARTESIAN_POINT('Ctrl Pts',(-10.2304300624439,38.3820277825385,17.6880511882454));
#48738=CARTESIAN_POINT('Ctrl Pts',(-10.2587281194445,38.3799807346645,17.689693829833));
#48739=CARTESIAN_POINT('Ctrl Pts',(-10.3311383734469,38.3738279297547,17.6938740795105));
#48740=CARTESIAN_POINT('Ctrl Pts',(-10.3752025331188,38.369212198078,17.6963959332254));
#48741=CARTESIAN_POINT('Ctrl Pts',(-10.5814067108247,38.3435164725506,17.708111051368));
#48742=CARTESIAN_POINT('Ctrl Pts',(-10.7419810360386,38.3115869573673,17.7169691838201));
#48743=CARTESIAN_POINT('Ctrl Pts',(-11.085676112541,38.2169776767717,17.7359949379022));
#48744=CARTESIAN_POINT('Ctrl Pts',(-11.2669922509377,38.1499780525723,17.7460736057422));
#48745=CARTESIAN_POINT('Ctrl Pts',(-11.5191354814177,38.0314961386416,17.761251343863));
#48746=CARTESIAN_POINT('Ctrl Pts',(-11.5952419293796,37.9921467849032,17.7660006966031));
#48747=CARTESIAN_POINT('Ctrl Pts',(-11.6913588870011,37.9377415739088,17.7723209494345));
#48748=CARTESIAN_POINT('Ctrl Pts',(-11.7128117728121,37.9252856602422,17.7737530311017));
#48749=CARTESIAN_POINT('Ctrl Pts',(-11.7477043593022,37.9045110239774,17.7761207762636));
#48750=CARTESIAN_POINT('Ctrl Pts',(-11.7612263902153,37.8963315414164,17.7770479641744));
#48751=CARTESIAN_POINT('Ctrl Pts',(-11.7883066574618,37.8796909157193,17.7789252460971));
#48752=CARTESIAN_POINT('Ctrl Pts',(-11.8018632161967,37.8712278555233,17.7798754465478));
#48753=CARTESIAN_POINT('Ctrl Pts',(-11.8370991385832,37.8488830287239,17.7823714659029));
#48754=CARTESIAN_POINT('Ctrl Pts',(-11.858680703033,37.8348498572842,17.7839264790033));
#48755=CARTESIAN_POINT('Ctrl Pts',(-11.9531431078626,37.771884371514,17.7908420491013));
#48756=CARTESIAN_POINT('Ctrl Pts',(-12.0242622899506,37.7203806252843,17.7963383554722));
#48757=CARTESIAN_POINT('Ctrl Pts',(-12.2646849354758,37.5316176728037,17.8157459863821));
#48758=CARTESIAN_POINT('Ctrl Pts',(-12.422700858004,37.3808428703411,17.8299712066777));
#48759=CARTESIAN_POINT('Ctrl Pts',(-12.6570714645664,37.1095368911862,17.8527165106462));
#48760=CARTESIAN_POINT('Ctrl Pts',(-12.7422859494787,36.9975110474234,17.8614586231315));
#48761=CARTESIAN_POINT('Ctrl Pts',(-12.8435911066558,36.8455776319802,17.8724714955442));
#48762=CARTESIAN_POINT('Ctrl Pts',(-12.8662286105954,36.8102212479383,17.8749796047546));
#48763=CARTESIAN_POINT('Ctrl Pts',(-12.9027948517976,36.7507038531411,17.8791133768719));
#48764=CARTESIAN_POINT('Ctrl Pts',(-12.9170922270035,36.7267758804843,17.8807521934373));
#48765=CARTESIAN_POINT('Ctrl Pts',(-12.9446663129053,36.6793080578827,17.8839590674971));
#48766=CARTESIAN_POINT('Ctrl Pts',(-12.9579598466322,36.6557804368797,17.8855276397676));
#48767=CARTESIAN_POINT('Ctrl Pts',(-12.9867520941661,36.6033687299806,17.8889772226961));
#48768=CARTESIAN_POINT('Ctrl Pts',(-13.0021161604321,36.574413548406,17.8908534563623));
#48769=CARTESIAN_POINT('Ctrl Pts',(-13.0544872020102,36.4721598214295,17.8973813807106));
#48770=CARTESIAN_POINT('Ctrl Pts',(-13.0892503388676,36.3977411699346,17.9019575345575));
#48771=CARTESIAN_POINT('Ctrl Pts',(-13.1415553572831,36.2742596460579,17.9093185834347));
#48772=CARTESIAN_POINT('Ctrl Pts',(-13.1607162010614,36.2259585707977,17.9121421215577));
#48773=CARTESIAN_POINT('Ctrl Pts',(-13.1787500078856,36.1772652419345,17.9149433153638));
#48774=CARTESIAN_POINT('Origin',(-10.,35.,23.));
#48775=CARTESIAN_POINT('',(-13.1787500671498,36.1772650819144,19.1603162262584));
#48776=CARTESIAN_POINT('',(-13.1787500897853,36.1772650207959,18.8205585884996));
#48777=CARTESIAN_POINT('',(-13.1787500671536,36.1772650819043,23.));
#48778=CARTESIAN_POINT('',(-13.389748949659,35.0026684800589,17.6410178032058));
#48779=CARTESIAN_POINT('Ctrl Pts',(-13.1787500897853,36.1772650207959,18.8205585884996));
#48780=CARTESIAN_POINT('Ctrl Pts',(-13.1278282806594,36.3147597245981,18.8127838324376));
#48781=CARTESIAN_POINT('Ctrl Pts',(-13.0680280570975,36.4488359492941,18.8050415662166));
#48782=CARTESIAN_POINT('Ctrl Pts',(-12.9630886910638,36.6482401636516,18.7927316152069));
#48783=CARTESIAN_POINT('Ctrl Pts',(-12.924054066361,36.7165361208937,18.7883602818215));
#48784=CARTESIAN_POINT('Ctrl Pts',(-12.8696319512129,36.8045035021615,18.7824416265651));
#48785=CARTESIAN_POINT('Ctrl Pts',(-12.8563500412601,36.8254546802598,18.7810096908794));
#48786=CARTESIAN_POINT('Ctrl Pts',(-12.8350992651065,36.8581763082458,18.7787349125609));
#48787=CARTESIAN_POINT('Ctrl Pts',(-12.8272839994421,36.8700460438123,18.7779016731655));
#48788=CARTESIAN_POINT('Ctrl Pts',(-12.8107584435316,36.8948044803658,18.7761459289914));
#48789=CARTESIAN_POINT('Ctrl Pts',(-12.802033736237,36.9076828763056,18.7752224137424));
#48790=CARTESIAN_POINT('Ctrl Pts',(-12.7797674981871,36.9400674172989,18.7728750046548));
#48791=CARTESIAN_POINT('Ctrl Pts',(-12.7661092015947,36.9594919604339,18.7714437583405));
#48792=CARTESIAN_POINT('Ctrl Pts',(-12.7084912604756,37.0396320584636,18.7654468848372));
#48793=CARTESIAN_POINT('Ctrl Pts',(-12.6627304298567,37.0990209326818,18.7607810236025));
#48794=CARTESIAN_POINT('Ctrl Pts',(-12.5210168748795,37.2708403584923,18.746719921106));
#48795=CARTESIAN_POINT('Ctrl Pts',(-12.4196403145262,37.3785668372318,18.7371553329958));
#48796=CARTESIAN_POINT('Ctrl Pts',(-12.1614050163612,37.6193280921082,18.7144226847852));
#48797=CARTESIAN_POINT('Ctrl Pts',(-11.9988219908403,37.7454113249418,18.701368413872));
#48798=CARTESIAN_POINT('Ctrl Pts',(-11.7811821434201,37.8845451131068,18.6856402949913));
#48799=CARTESIAN_POINT('Ctrl Pts',(-11.7358926364506,37.91202465048,18.6824517258225));
#48800=CARTESIAN_POINT('Ctrl Pts',(-11.6636078735654,37.9535976613584,18.6774914018006));
#48801=CARTESIAN_POINT('Ctrl Pts',(-11.63703645124,37.9684073254537,18.675694594728));
#48802=CARTESIAN_POINT('Ctrl Pts',(-11.5869893954297,37.9954247737233,18.6723585764118));
#48803=CARTESIAN_POINT('Ctrl Pts',(-11.5635633846692,38.0077191552521,18.6708164266608));
#48804=CARTESIAN_POINT('Ctrl Pts',(-11.510525004539,38.0347674788116,18.6673670404646));
#48805=CARTESIAN_POINT('Ctrl Pts',(-11.4808355256115,38.0493648021045,18.6654652947617));
#48806=CARTESIAN_POINT('Ctrl Pts',(-11.3890990175868,38.0928127288703,18.6596738900431));
#48807=CARTESIAN_POINT('Ctrl Pts',(-11.3263865632731,38.1202221415413,18.655832464063));
#48808=CARTESIAN_POINT('Ctrl Pts',(-11.175488714436,38.1808018425857,18.6468274851246));
#48809=CARTESIAN_POINT('Ctrl Pts',(-11.0866653705874,38.2122319412057,18.6417150888241));
#48810=CARTESIAN_POINT('Ctrl Pts',(-10.7881266228143,38.3040665020567,18.6249528514246));
#48811=CARTESIAN_POINT('Ctrl Pts',(-10.5739159679095,38.3479264065704,18.6136248192712));
#48812=CARTESIAN_POINT('Ctrl Pts',(-10.2696063402654,38.3801536354768,18.5969865528056));
#48813=CARTESIAN_POINT('Ctrl Pts',(-10.1819048914782,38.3860056690546,18.5921241808017));
#48814=CARTESIAN_POINT('Ctrl Pts',(-10.0684420522953,38.3891560435511,18.5856374616524));
#48815=CARTESIAN_POINT('Ctrl Pts',(-10.0427951658551,38.3895768897431,18.5841582705194));
#48816=CARTESIAN_POINT('Ctrl Pts',(-10.0011954831906,38.3897873214299,18.5817344975548));
#48817=CARTESIAN_POINT('Ctrl Pts',(-9.98524414545605,38.38975541238,18.5807992627702));
#48818=CARTESIAN_POINT('Ctrl Pts',(-9.95354842323859,38.3894682852285,18.578928282167));
#48819=CARTESIAN_POINT('Ctrl Pts',(-9.93780446933173,38.3892159410399,18.5779927003318));
#48820=CARTESIAN_POINT('Ctrl Pts',(-9.89733806343113,38.3882852961738,18.5755729699747));
#48821=CARTESIAN_POINT('Ctrl Pts',(-9.87262060272855,38.3874461077077,18.574080549325));
#48822=CARTESIAN_POINT('Ctrl Pts',(-9.76257407699222,38.3825037790683,18.5673783106616));
#48823=CARTESIAN_POINT('Ctrl Pts',(-9.67741454847383,38.3754465238114,18.5620376944088));
#48824=CARTESIAN_POINT('Ctrl Pts',(-9.40233572272547,38.3421461775074,18.5444664096964));
#48825=CARTESIAN_POINT('Ctrl Pts',(-9.21434991361348,38.3030135644837,18.531980745581));
#48826=CARTESIAN_POINT('Ctrl Pts',(-8.87109217682399,38.2005792933359,18.5090907199521));
#48827=CARTESIAN_POINT('Ctrl Pts',(-8.71521672238509,38.1412553761799,18.4986556327387));
#48828=CARTESIAN_POINT('Ctrl Pts',(-8.52412634334786,38.0519125783087,18.4859060694986));
#48829=CARTESIAN_POINT('Ctrl Pts',(-8.48430723718972,38.0323339467858,18.4832506769565));
#48830=CARTESIAN_POINT('Ctrl Pts',(-8.41970730030144,37.9989802917374,18.4789431838222));
#48831=CARTESIAN_POINT('Ctrl Pts',(-8.39469551180887,37.9856666558795,18.4772754996969));
#48832=CARTESIAN_POINT('Ctrl Pts',(-8.34619143302035,37.9590624513042,18.4740406305722));
#48833=CARTESIAN_POINT('Ctrl Pts',(-8.32268521211471,37.9458018485712,18.4724725541925));
#48834=CARTESIAN_POINT('Ctrl Pts',(-8.26703045648805,37.9135230603468,18.4687575652132));
#48835=CARTESIAN_POINT('Ctrl Pts',(-8.23503261944236,37.8942512614012,18.4666198369451));
#48836=CARTESIAN_POINT('Ctrl Pts',(-8.12181685826711,37.8234871824903,18.4590422033253));
#48837=CARTESIAN_POINT('Ctrl Pts',(-8.04247637135539,37.769071185333,18.4537074721338));
#48838=CARTESIAN_POINT('Ctrl Pts',(-7.83823071677698,37.6158165567845,18.4397756986438));
#48839=CARTESIAN_POINT('Ctrl Pts',(-7.71779240633974,37.511428755291,18.4313562533397));
#48840=CARTESIAN_POINT('Ctrl Pts',(-7.4742206590898,37.2682728190713,18.4131084803104));
#48841=CARTESIAN_POINT('Ctrl Pts',(-7.354238683669,37.1271002551932,18.4033027723595));
#48842=CARTESIAN_POINT('Ctrl Pts',(-7.22612142652934,36.9486430538533,18.3908924263128));
#48843=CARTESIAN_POINT('Ctrl Pts',(-7.20629597877852,36.9201119076517,18.3889074823669));
#48844=CARTESIAN_POINT('Ctrl Pts',(-7.17683301593104,36.8762887997899,18.3858492750645));
#48845=CARTESIAN_POINT('Ctrl Pts',(-7.16687294609215,36.8612153407633,18.3847957162192));
#48846=CARTESIAN_POINT('Ctrl Pts',(-7.14890076295715,36.8335379027941,18.3828568142714));
#48847=CARTESIAN_POINT('Ctrl Pts',(-7.1408507715899,36.8209595722282,18.3819739153624));
#48848=CARTESIAN_POINT('Ctrl Pts',(-7.12235685123925,36.7916373485821,18.3799118583016));
#48849=CARTESIAN_POINT('Ctrl Pts',(-7.11197576631915,36.7748550545828,18.378728886131));
#48850=CARTESIAN_POINT('Ctrl Pts',(-7.07842754798129,36.7195465788642,18.3748236377314));
#48851=CARTESIAN_POINT('Ctrl Pts',(-7.05588111410464,36.6806515410949,18.3720669698688));
#48852=CARTESIAN_POINT('Ctrl Pts',(-7.00207898041549,36.5834305729399,18.3651722376466));
#48853=CARTESIAN_POINT('Ctrl Pts',(-6.97174536780424,36.5246166140466,18.3609977528751));
#48854=CARTESIAN_POINT('Ctrl Pts',(-6.8265729628989,36.2216930211849,18.3396049988428));
#48855=CARTESIAN_POINT('Ctrl Pts',(-6.73943060950019,35.9653441938233,18.3219512890962));
#48856=CARTESIAN_POINT('Ctrl Pts',(-6.66499312025702,35.6133717187204,18.2995522385174));
#48857=CARTESIAN_POINT('Ctrl Pts',(-6.64989085774551,35.5246586603036,18.2940447296492));
#48858=CARTESIAN_POINT('Ctrl Pts',(-6.63353339474193,35.3983774507571,18.2864006122948));
#48859=CARTESIAN_POINT('Ctrl Pts',(-6.62934539642089,35.3612335930106,18.2841757201296));
#48860=CARTESIAN_POINT('Ctrl Pts',(-6.62321559105519,35.2974013704534,18.2803910756214));
#48861=CARTESIAN_POINT('Ctrl Pts',(-6.62097392553736,35.2707459487775,18.2788222318819));
#48862=CARTESIAN_POINT('Ctrl Pts',(-6.61700987958879,35.2158335968354,18.275613110802));
#48863=CARTESIAN_POINT('Ctrl Pts',(-6.61532547781573,35.187575973454,18.2739741217276));
#48864=CARTESIAN_POINT('Ctrl Pts',(-6.61192136845952,35.1152198158909,18.2698072218175));
#48865=CARTESIAN_POINT('Ctrl Pts',(-6.61070845659356,35.0711020788213,18.2672949422737));
#48866=CARTESIAN_POINT('Ctrl Pts',(-6.60895982020982,34.8513442667541,18.2549044232832));
#48867=CARTESIAN_POINT('Ctrl Pts',(-6.62121350551241,34.6758656554659,18.2454216283818));
#48868=CARTESIAN_POINT('Ctrl Pts',(-6.68396046236489,34.2533018670943,18.2226743888106));
#48869=CARTESIAN_POINT('Ctrl Pts',(-6.74848100810393,34.0094093873721,18.209635051806));
#48870=CARTESIAN_POINT('Ctrl Pts',(-6.85151705257719,33.7435802144125,18.193508770649));
#48871=CARTESIAN_POINT('Ctrl Pts',(-6.86413372287889,33.7124138624643,18.1915858924437));
#48872=CARTESIAN_POINT('Ctrl Pts',(-6.88415465444445,33.6649975807396,18.1886034287414));
#48873=CARTESIAN_POINT('Ctrl Pts',(-6.89122754008479,33.6486090726427,18.1875620351187));
#48874=CARTESIAN_POINT('Ctrl Pts',(-6.90448492406748,33.6185454335661,18.1856308147937));
#48875=CARTESIAN_POINT('Ctrl Pts',(-6.91063127883601,33.6048544235058,18.1847431853012));
#48876=CARTESIAN_POINT('Ctrl Pts',(-6.92525000528413,33.5728615126812,18.1826501167789));
#48877=CARTESIAN_POINT('Ctrl Pts',(-6.93379503460657,33.5545938776892,18.1814405192206));
#48878=CARTESIAN_POINT('Ctrl Pts',(-6.96294610069723,33.4936963885261,18.177362180186));
#48879=CARTESIAN_POINT('Ctrl Pts',(-6.98428140872673,33.4514239242431,18.1744551609298));
#48880=CARTESIAN_POINT('Ctrl Pts',(-7.039899528721,33.346736612388,18.1670885310381));
#48881=CARTESIAN_POINT('Ctrl Pts',(-7.07527638456773,33.2849299224575,18.1625866505059));
#48882=CARTESIAN_POINT('Ctrl Pts',(-7.19900649314821,33.0837365051866,18.1475178717461));
#48883=CARTESIAN_POINT('Ctrl Pts',(-7.29558860097697,32.9496852513521,18.13680640595));
#48884=CARTESIAN_POINT('Ctrl Pts',(-7.50986707701628,32.6939007421099,18.1154839016283));
#48885=CARTESIAN_POINT('Ctrl Pts',(-7.62769486318381,32.572854102371,18.1049119870985));
#48886=CARTESIAN_POINT('Ctrl Pts',(-7.78735088589727,32.4316222197916,18.0920291876821));
#48887=CARTESIAN_POINT('Ctrl Pts',(-7.82121822514116,32.4028302361729,18.0893690830604));
#48888=CARTESIAN_POINT('Ctrl Pts',(-7.87763859666961,32.3567456220642,18.0850529184204));
#48889=CARTESIAN_POINT('Ctrl Pts',(-7.89985932065496,32.3390564017648,18.0833812792042));
#48890=CARTESIAN_POINT('Ctrl Pts',(-7.94368724137733,32.3050574113178,18.0801377833348));
#48891=CARTESIAN_POINT('Ctrl Pts',(-7.96527262173455,32.2887231281411,18.0785650460092));
#48892=CARTESIAN_POINT('Ctrl Pts',(-8.01721856005453,32.2503839211067,18.0748371619889));
#48893=CARTESIAN_POINT('Ctrl Pts',(-8.0477534391205,32.2286204981029,18.0726912674813));
#48894=CARTESIAN_POINT('Ctrl Pts',(-8.15838632296632,32.1525040892002,18.0650698788626));
#48895=CARTESIAN_POINT('Ctrl Pts',(-8.24044592110707,32.10107854891,18.0597008640835));
#48896=CARTESIAN_POINT('Ctrl Pts',(-8.4643861482978,31.9737561311255,18.0456486880187));
#48897=CARTESIAN_POINT('Ctrl Pts',(-8.60965559581636,31.9043243903016,18.0371469933706));
#48898=CARTESIAN_POINT('Ctrl Pts',(-8.92931242851481,31.7786019036434,18.0189325886959));
#48899=CARTESIAN_POINT('Ctrl Pts',(-9.10442734983922,31.7255972688611,18.0092408203109));
#48900=CARTESIAN_POINT('Ctrl Pts',(-9.31701251105216,31.6795860704288,17.9969547677973));
#48901=CARTESIAN_POINT('Ctrl Pts',(-9.35119808591971,31.6727373934834,17.9949630454292));
#48902=CARTESIAN_POINT('Ctrl Pts',(-9.40328345824383,31.6631358883837,17.9918959692929));
#48903=CARTESIAN_POINT('Ctrl Pts',(-9.42111068902769,31.6599970263153,17.990840455264));
#48904=CARTESIAN_POINT('Ctrl Pts',(-9.45349244477459,31.6545625634264,17.9889114062777));
#48905=CARTESIAN_POINT('Ctrl Pts',(-9.4680380059237,31.6522188593565,17.988040498488));
#48906=CARTESIAN_POINT('Ctrl Pts',(-9.50183579229274,31.6469988988546,17.9860066638246));
#48907=CARTESIAN_POINT('Ctrl Pts',(-9.52109777951664,31.6441936013375,17.9848400197797));
#48908=CARTESIAN_POINT('Ctrl Pts',(-9.5838179358729,31.6356100793622,17.9810191482581));
#48909=CARTESIAN_POINT('Ctrl Pts',(-9.62736262386855,31.6305092303872,17.9783320502771));
#48910=CARTESIAN_POINT('Ctrl Pts',(-9.9168360425269,31.6022797268836,17.9602941827535));
#48911=CARTESIAN_POINT('Ctrl Pts',(-10.1645559663494,31.6052485178992,17.9440864350204));
#48912=CARTESIAN_POINT('Ctrl Pts',(-10.5750465582232,31.6552347056375,17.9176488491895));
#48913=CARTESIAN_POINT('Ctrl Pts',(-10.7386528338555,31.6875178142305,17.9072123375417));
#48914=CARTESIAN_POINT('Ctrl Pts',(-10.9419323896949,31.7434483166295,17.8944687327603));
#48915=CARTESIAN_POINT('Ctrl Pts',(-10.9843899300566,31.7560298647002,17.8918186452865));
#48916=CARTESIAN_POINT('Ctrl Pts',(-11.0534808670315,31.7779852198053,17.88752345164));
#48917=CARTESIAN_POINT('Ctrl Pts',(-11.0802642196022,31.7868659428537,17.8858626945999));
#48918=CARTESIAN_POINT('Ctrl Pts',(-11.1322897339523,31.8048404319631,17.8826441643419));
#48919=CARTESIAN_POINT('Ctrl Pts',(-11.157540908227,31.8139014745961,17.8810854650393));
#48920=CARTESIAN_POINT('Ctrl Pts',(-11.2173913326308,31.8361834610762,17.8773979035282));
#48921=CARTESIAN_POINT('Ctrl Pts',(-11.2518870682638,31.8496737199851,17.8752780658735));
#48922=CARTESIAN_POINT('Ctrl Pts',(-11.3737357018973,31.899642688006,17.867803085788));
#48923=CARTESIAN_POINT('Ctrl Pts',(-11.4597771528815,31.9392128422422,17.8625500290831));
#48924=CARTESIAN_POINT('Ctrl Pts',(-11.682179435475,32.0530098960424,17.8489148092356));
#48925=CARTESIAN_POINT('Ctrl Pts',(-11.8152935379764,32.1330868631926,17.8407009522263));
#48926=CARTESIAN_POINT('Ctrl Pts',(-12.0994948645564,32.3318087180425,17.8223251054345));
#48927=CARTESIAN_POINT('Ctrl Pts',(-12.2469229880581,32.4547211164256,17.8121931739081));
#48928=CARTESIAN_POINT('Ctrl Pts',(-12.4075838113332,32.6135539896643,17.7994264046186));
#48929=CARTESIAN_POINT('Ctrl Pts',(-12.4316358390742,32.6380661896071,17.7974638258578));
#48930=CARTESIAN_POINT('Ctrl Pts',(-12.4676794551313,32.6759335135489,17.7944355565083));
#48931=CARTESIAN_POINT('Ctrl Pts',(-12.4799449135196,32.689026153061,17.7933891652836));
#48932=CARTESIAN_POINT('Ctrl Pts',(-12.5012142106865,32.7120941680484,17.7915453179189));
#48933=CARTESIAN_POINT('Ctrl Pts',(-12.5102635598188,32.7220266762317,17.7907512581966));
#48934=CARTESIAN_POINT('Ctrl Pts',(-12.5319400045785,32.7461046157187,17.7888261350229));
#48935=CARTESIAN_POINT('Ctrl Pts',(-12.54450763853,32.7603023796487,17.7876909037504));
#48936=CARTESIAN_POINT('Ctrl Pts',(-12.5834775496722,32.8050783819994,17.7841125453147));
#48937=CARTESIAN_POINT('Ctrl Pts',(-12.6094518021758,32.836022610098,17.7816422801798));
#48938=CARTESIAN_POINT('Ctrl Pts',(-12.6707076162852,32.9117060530137,17.775621798458));
#48939=CARTESIAN_POINT('Ctrl Pts',(-12.7054258833151,32.9568844992691,17.7720453366169));
#48940=CARTESIAN_POINT('Ctrl Pts',(-12.8475522043249,33.1518096133732,17.7567547109341));
#48941=CARTESIAN_POINT('Ctrl Pts',(-12.9437936577634,33.3093078219513,17.7447596745295));
#48942=CARTESIAN_POINT('Ctrl Pts',(-13.1062734859634,33.631547451641,17.7216514940857));
#48943=CARTESIAN_POINT('Ctrl Pts',(-13.1733516966057,33.7952380719363,17.7105578478115));
#48944=CARTESIAN_POINT('Ctrl Pts',(-13.2410702762761,34.0060809186809,17.6971678942629));
#48945=CARTESIAN_POINT('Ctrl Pts',(-13.2539221383331,34.0489991164086,17.6944858759613));
#48946=CARTESIAN_POINT('Ctrl Pts',(-13.2735617939049,34.1196521141618,17.690139719863));
#48947=CARTESIAN_POINT('Ctrl Pts',(-13.2808563328518,34.1472391801397,17.6884597196753));
#48948=CARTESIAN_POINT('Ctrl Pts',(-13.2944060712666,34.201232275468,17.6852036605684));
#48949=CARTESIAN_POINT('Ctrl Pts',(-13.3006942258176,34.2276277256105,17.6836266700366));
#48950=CARTESIAN_POINT('Ctrl Pts',(-13.3125727059751,34.2802862109926,17.6805087444614));
#48951=CARTESIAN_POINT('Ctrl Pts',(-13.3181692525206,34.3065457906286,17.6789677179711));
#48952=CARTESIAN_POINT('Ctrl Pts',(-13.3306122343721,34.3685331798546,17.6753607697588));
#48953=CARTESIAN_POINT('Ctrl Pts',(-13.3371967839182,34.4043105150398,17.6733028638893));
#48954=CARTESIAN_POINT('Ctrl Pts',(-13.374326420083,34.6260491159392,17.6606823226094));
#48955=CARTESIAN_POINT('Ctrl Pts',(-13.3898959837627,34.8141824997077,17.6505782097631));
#48956=CARTESIAN_POINT('Ctrl Pts',(-13.3897489686288,35.0026442731042,17.6405623182023));
#48957=CARTESIAN_POINT('Ctrl Pts',(-13.389748949659,35.0026684800589,17.6410178032058));
#48958=CARTESIAN_POINT('Ctrl Pts',(-13.3896451106924,35.1345742916728,17.633279295912));
#48959=CARTESIAN_POINT('Ctrl Pts',(-13.3818383067087,35.2661542793446,17.6255407886183));
#48960=CARTESIAN_POINT('Ctrl Pts',(-13.3664640668758,35.3966418396162,17.6178022813246));
#48961=CARTESIAN_POINT('Ctrl Pts',(-13.3507859989956,35.5297081147419,17.6099108444822));
#48962=CARTESIAN_POINT('Ctrl Pts',(-13.3272384397749,35.6616386106036,17.6020194076398));
#48963=CARTESIAN_POINT('Ctrl Pts',(-13.2960136305224,35.7916433603022,17.5941279707973));
#48964=CARTESIAN_POINT('Ctrl Pts',(-13.2922024269181,35.807511337801,17.5931647664334));
#48965=CARTESIAN_POINT('Ctrl Pts',(-13.2882769070792,35.8233506505285,17.5922015620694));
#48966=CARTESIAN_POINT('Ctrl Pts',(-13.2842374693377,35.8391598819644,17.5912383577054));
#48967=CARTESIAN_POINT('Ctrl Pts',(-13.2586267193139,35.9393932065711,17.5851314716073));
#48968=CARTESIAN_POINT('Ctrl Pts',(-13.228380821193,36.0386188205438,17.5790245855091));
#48969=CARTESIAN_POINT('Ctrl Pts',(-13.1935954601691,36.1363771817876,17.572917699411));
#48970=CARTESIAN_POINT('Ctrl Pts',(-13.18873541208,36.1500355231923,17.5720644738231));
#48971=CARTESIAN_POINT('Ctrl Pts',(-13.1837868341332,36.1636652362783,17.5712112482351));
#48972=CARTESIAN_POINT('Ctrl Pts',(-13.1787500671536,36.1772650819042,17.5703580226472));
#48973=CARTESIAN_POINT('Ctrl Pts',(-13.1787500078856,36.1772652419345,17.9149433153638));
#48974=CARTESIAN_POINT('Ctrl Pts',(-13.2574737368644,35.9647022228304,17.9271714835018));
#48975=CARTESIAN_POINT('Ctrl Pts',(-13.3147215403028,35.744662343441,17.938932006304));
#48976=CARTESIAN_POINT('Ctrl Pts',(-13.3598257005944,35.4543632313368,17.954834547551));
#48977=CARTESIAN_POINT('Ctrl Pts',(-13.3681327804114,35.3880146410483,17.9584979595338));
#48978=CARTESIAN_POINT('Ctrl Pts',(-13.3787671680747,35.276384512114,17.964771474124));
#48979=CARTESIAN_POINT('Ctrl Pts',(-13.3821578636708,35.2312222999742,17.9673395823382));
#48980=CARTESIAN_POINT('Ctrl Pts',(-13.3857286073074,35.1662482708981,17.9710943312934));
#48981=CARTESIAN_POINT('Ctrl Pts',(-13.3866414468256,35.1464798948084,17.9722446909789));
#48982=CARTESIAN_POINT('Ctrl Pts',(-13.387939505466,35.1117771359175,17.9742798447986));
#48983=CARTESIAN_POINT('Ctrl Pts',(-13.3883991762541,35.0968464327591,17.9751606377858));
#48984=CARTESIAN_POINT('Ctrl Pts',(-13.3891957309927,35.0638926544424,17.9771164546381));
#48985=CARTESIAN_POINT('Ctrl Pts',(-13.3894875568287,35.0458698624516,17.9781937406211));
#48986=CARTESIAN_POINT('Ctrl Pts',(-13.3899283128212,34.9922176524452,17.981421718358));
#48987=CARTESIAN_POINT('Ctrl Pts',(-13.3896592369081,34.956588344402,17.9835928974183));
#48988=CARTESIAN_POINT('Ctrl Pts',(-13.3847778707467,34.7472700987069,17.9964849456708));
#48989=CARTESIAN_POINT('Ctrl Pts',(-13.3673782870388,34.574150112671,18.0076869690477));
#48990=CARTESIAN_POINT('Ctrl Pts',(-13.307490239155,34.2393407127586,18.0296129566669));
#48991=CARTESIAN_POINT('Ctrl Pts',(-13.2661670724509,34.0779071717534,18.0403067371467));
#48992=CARTESIAN_POINT('Ctrl Pts',(-13.1817362310069,33.8266783060786,18.056862752586));
#48993=CARTESIAN_POINT('Ctrl Pts',(-13.1462564350678,33.7346136586263,18.0629141153332));
#48994=CARTESIAN_POINT('Ctrl Pts',(-13.0917428664217,33.6096942284475,18.0710987307272));
#48995=CARTESIAN_POINT('Ctrl Pts',(-13.0761012990294,33.5754210936235,18.0733417216152));
#48996=CARTESIAN_POINT('Ctrl Pts',(-13.0482554303218,33.5170046742794,18.0771617579532));
#48997=CARTESIAN_POINT('Ctrl Pts',(-13.0363277520216,33.4927342138675,18.0787479850568));
#48998=CARTESIAN_POINT('Ctrl Pts',(-13.011355193237,33.4434197286816,18.0819701373425));
#48999=CARTESIAN_POINT('Ctrl Pts',(-12.9982852481794,33.4183907304188,18.083605041529));
#49000=CARTESIAN_POINT('Ctrl Pts',(-12.9641061669834,33.354884344402,18.0877539442405));
#49001=CARTESIAN_POINT('Ctrl Pts',(-12.9425594343131,33.3166476561134,18.0902525271073));
#49002=CARTESIAN_POINT('Ctrl Pts',(-12.841974288071,33.1459859216965,18.1014228192928));
#49003=CARTESIAN_POINT('Ctrl Pts',(-12.7546946967595,33.01862417274,18.1097990609624));
#49004=CARTESIAN_POINT('Ctrl Pts',(-12.6379658746111,32.8709872291919,18.1198580992063));
#49005=CARTESIAN_POINT('Ctrl Pts',(-12.6164948149473,32.8446544932345,18.1216674037375));
#49006=CARTESIAN_POINT('Ctrl Pts',(-12.4712502278462,32.6718917774241,18.1336629451838));
#49007=CARTESIAN_POINT('Ctrl Pts',(-12.3356489064617,32.5358773968653,18.1436957400029));
#49008=CARTESIAN_POINT('Ctrl Pts',(-12.1380004880188,32.368674836656,18.1579332351119));
#49009=CARTESIAN_POINT('Ctrl Pts',(-12.0854361190351,32.326823384687,18.1616891628925));
#49010=CARTESIAN_POINT('Ctrl Pts',(-12.0128206541591,32.2724530486525,18.166889304276));
#49011=CARTESIAN_POINT('Ctrl Pts',(-11.9938285773464,32.2585392770875,18.1682503985757));
#49012=CARTESIAN_POINT('Ctrl Pts',(-11.9633395140369,32.2366871049758,18.1704397425555));
#49013=CARTESIAN_POINT('Ctrl Pts',(-11.9519353703066,32.2286197485778,18.171259589436));
#49014=CARTESIAN_POINT('Ctrl Pts',(-11.9275130570899,32.2115687829466,18.1730180660892));
#49015=CARTESIAN_POINT('Ctrl Pts',(-11.9144812785049,32.2026053819707,18.1739580397653));
#49016=CARTESIAN_POINT('Ctrl Pts',(-11.8806712345647,32.179697364679,18.1763999673659));
#49017=CARTESIAN_POINT('Ctrl Pts',(-11.8598007858599,32.1658912858409,18.1779104491723));
#49018=CARTESIAN_POINT('Ctrl Pts',(-11.7642843321946,32.1042152447318,18.1848305649245));
#49019=CARTESIAN_POINT('Ctrl Pts',(-11.6879353312886,32.05905791051,18.1903810266286));
#49020=CARTESIAN_POINT('Ctrl Pts',(-11.4264553756632,31.9179408479928,18.2092448853357));
#49021=CARTESIAN_POINT('Ctrl Pts',(-11.234257509621,31.8360663435837,18.2228446642719));
#49022=CARTESIAN_POINT('Ctrl Pts',(-10.8952326188486,31.7272729549394,18.2454917925623));
#49023=CARTESIAN_POINT('Ctrl Pts',(-10.7519069833692,31.6914007941183,18.2546930563343));
#49024=CARTESIAN_POINT('Ctrl Pts',(-10.5638749337427,31.657195287625,18.2662352166154));
#49025=CARTESIAN_POINT('Ctrl Pts',(-10.5209189285271,31.6502325424156,18.2688378313032));
#49026=CARTESIAN_POINT('Ctrl Pts',(-10.4499424724363,31.6401263653891,18.2730837208633));
#49027=CARTESIAN_POINT('Ctrl Pts',(-10.4219966768903,31.6365021264532,18.2747416764053));
#49028=CARTESIAN_POINT('Ctrl Pts',(-10.3670715493681,31.6300743234197,18.2779742172728));
#49029=CARTESIAN_POINT('Ctrl Pts',(-10.3400973946498,31.6272452782984,18.2795494756072));
#49030=CARTESIAN_POINT('Ctrl Pts',(-10.2752487927842,31.6212298738484,18.2833085758431));
#49031=CARTESIAN_POINT('Ctrl Pts',(-10.2373486060489,31.6183561294805,18.285482672281));
#49032=CARTESIAN_POINT('Ctrl Pts',(-10.0985023867817,31.6101741286913,18.293371603538));
#49033=CARTESIAN_POINT('Ctrl Pts',(-9.99737718196369,31.6087439217334,18.2989690461317));
#49034=CARTESIAN_POINT('Ctrl Pts',(-9.63158270987046,31.6199361273164,18.3188933922899));
#49035=CARTESIAN_POINT('Ctrl Pts',(-9.36871450613035,31.6590375405653,18.3325299046251));
#49036=CARTESIAN_POINT('Ctrl Pts',(-9.02690851700285,31.7516972245671,18.3517722572991));
#49037=CARTESIAN_POINT('Ctrl Pts',(-8.94169128184659,31.7784540800753,18.3567099340684));
#49038=CARTESIAN_POINT('Ctrl Pts',(-8.83334038820817,31.8172376219756,18.3632854085892));
#49039=CARTESIAN_POINT('Ctrl Pts',(-8.80914498459322,31.8262112150819,18.3647733239792));
#49040=CARTESIAN_POINT('Ctrl Pts',(-8.77012868800927,31.8411905313918,18.3672080561683));
#49041=CARTESIAN_POINT('Ctrl Pts',(-8.75524326046369,31.8470265875581,18.3681453780294));
#49042=CARTESIAN_POINT('Ctrl Pts',(-8.7257924319867,31.8588142841921,18.3700176763244));
#49043=CARTESIAN_POINT('Ctrl Pts',(-8.71122613660854,31.8647624444458,18.3709524520316));
#49044=CARTESIAN_POINT('Ctrl Pts',(-8.67396546723535,31.8802814045573,18.3733651266888));
#49045=CARTESIAN_POINT('Ctrl Pts',(-8.65133336133557,31.8899984055399,18.3748511897266));
#49046=CARTESIAN_POINT('Ctrl Pts',(-8.55186335758576,31.9339953614789,18.3814676058993));
#49047=CARTESIAN_POINT('Ctrl Pts',(-8.47621634746672,31.9708804295639,18.3867246618528));
#49048=CARTESIAN_POINT('Ctrl Pts',(-8.23843695988298,32.0979819872935,18.4038126259038));
#49049=CARTESIAN_POINT('Ctrl Pts',(-8.08230345588369,32.1987051232657,18.4158861790797));
#49050=CARTESIAN_POINT('Ctrl Pts',(-7.79745859456951,32.4174858910498,18.438868168231));
#49051=CARTESIAN_POINT('Ctrl Pts',(-7.66804239486149,32.5337162001579,18.4497687312902));
#49052=CARTESIAN_POINT('Ctrl Pts',(-7.51732984544045,32.6915939150976,18.4629626473845));
#49053=CARTESIAN_POINT('Ctrl Pts',(-7.48720530877304,32.7244225189734,18.4656293339936));
#49054=CARTESIAN_POINT('Ctrl Pts',(-7.43896051606056,32.779124608657,18.4699511327769));
#49055=CARTESIAN_POINT('Ctrl Pts',(-7.42045319735698,32.8006480253532,18.4716219949042));
#49056=CARTESIAN_POINT('Ctrl Pts',(-7.38487822813602,32.8430874516784,18.4748604004166));
#49057=CARTESIAN_POINT('Ctrl Pts',(-7.3677858166782,32.8639798274188,18.4764288706277));
#49058=CARTESIAN_POINT('Ctrl Pts',(-7.32768172759338,32.9142123136093,18.4801406798094));
#49059=CARTESIAN_POINT('Ctrl Pts',(-7.30490076097197,32.9437326367169,18.4822749089106));
#49060=CARTESIAN_POINT('Ctrl Pts',(-7.22549258662012,33.0502197240417,18.4898150291918));
#49061=CARTESIAN_POINT('Ctrl Pts',(-7.17163557473333,33.1292003437612,18.4951173132169));
#49062=CARTESIAN_POINT('Ctrl Pts',(-7.03809095549763,33.3440198283868,18.5089225950051));
#49063=CARTESIAN_POINT('Ctrl Pts',(-6.96440467901353,33.4833128932906,18.5172526612765));
#49064=CARTESIAN_POINT('Ctrl Pts',(-6.82458713481651,33.7989812725241,18.5355573459174));
#49065=CARTESIAN_POINT('Ctrl Pts',(-6.76292868593539,33.9767467743751,18.5455065568653));
#49066=CARTESIAN_POINT('Ctrl Pts',(-6.70772591617784,34.1922042228426,18.5580733603935));
#49067=CARTESIAN_POINT('Ctrl Pts',(-6.69965101103648,34.2258559447375,18.5600507823694));
#49068=CARTESIAN_POINT('Ctrl Pts',(-6.68815172819012,34.2772332962,18.5631000415621));
#49069=CARTESIAN_POINT('Ctrl Pts',(-6.68435118572477,34.2948733502009,18.5641523731711));
#49070=CARTESIAN_POINT('Ctrl Pts',(-6.67766161796203,34.3271731455828,18.5660904572285));
#49071=CARTESIAN_POINT('Ctrl Pts',(-6.67472841789347,34.3418228357329,18.5669737907543));
#49072=CARTESIAN_POINT('Ctrl Pts',(-6.66813730901591,34.3759108369394,18.5690390367213));
#49073=CARTESIAN_POINT('Ctrl Pts',(-6.66455259353223,34.3953622306618,18.5702247986471));
#49074=CARTESIAN_POINT('Ctrl Pts',(-6.65333058821598,34.4593941833802,18.5741496315848));
#49075=CARTESIAN_POINT('Ctrl Pts',(-6.64641561736558,34.504094595666,18.5769235469875));
#49076=CARTESIAN_POINT('Ctrl Pts',(-6.63151573486521,34.6150669633137,18.5838724460606));
#49077=CARTESIAN_POINT('Ctrl Pts',(-6.62459014109601,34.6814610339877,18.5880845230382));
#49078=CARTESIAN_POINT('Ctrl Pts',(-6.59899064905051,35.0248741805579,18.6100205052718));
#49079=CARTESIAN_POINT('Ctrl Pts',(-6.61244268644938,35.3032706506471,18.6281900922993));
#49080=CARTESIAN_POINT('Ctrl Pts',(-6.67380871640482,35.6585780828493,18.6505648944949));
#49081=CARTESIAN_POINT('Ctrl Pts',(-6.69090473181836,35.7397052143762,18.6556269678899));
#49082=CARTESIAN_POINT('Ctrl Pts',(-6.71891389856819,35.8520329631934,18.6625699168365));
#49083=CARTESIAN_POINT('Ctrl Pts',(-6.72733305303587,35.8838197462793,18.6645272979804));
#49084=CARTESIAN_POINT('Ctrl Pts',(-6.74351583598507,35.9415131472858,18.6680675330598));
#49085=CARTESIAN_POINT('Ctrl Pts',(-6.75112944201349,35.9674586697056,18.6696549991719));
#49086=CARTESIAN_POINT('Ctrl Pts',(-6.76720466728399,36.0199084677491,18.6728556531484));
#49087=CARTESIAN_POINT('Ctrl Pts',(-6.77568377932629,36.0464052380243,18.6744681374077));
#49088=CARTESIAN_POINT('Ctrl Pts',(-6.79770348406088,36.1124053628343,18.678475183605));
#49089=CARTESIAN_POINT('Ctrl Pts',(-6.81164982337988,36.151769088874,18.6808564782364));
#49090=CARTESIAN_POINT('Ctrl Pts',(-6.87478416354492,36.3200232092906,18.6910104763902));
#49091=CARTESIAN_POINT('Ctrl Pts',(-6.93108945298465,36.4461081662682,18.6985502284358));
#49092=CARTESIAN_POINT('Ctrl Pts',(-7.05801722143222,36.6892999880298,18.7132834687168));
#49093=CARTESIAN_POINT('Ctrl Pts',(-7.12834390326038,36.8062638320009,18.7204672411293));
#49094=CARTESIAN_POINT('Ctrl Pts',(-7.30011764709784,37.0564458450041,18.7365948897122));
#49095=CARTESIAN_POINT('Ctrl Pts',(-7.40476058402889,37.1870195002611,18.7455477509877));
#49096=CARTESIAN_POINT('Ctrl Pts',(-7.53809854519715,37.330293189993,18.7566882544843));
#49097=CARTESIAN_POINT('Ctrl Pts',(-7.55787202794012,37.3510074389266,18.7583343782505));
#49098=CARTESIAN_POINT('Ctrl Pts',(-7.58951273439657,37.3833236256132,18.7609638906814));
#49099=CARTESIAN_POINT('Ctrl Pts',(-7.60120722331595,37.395093641453,18.7619348118881));
#49100=CARTESIAN_POINT('Ctrl Pts',(-7.62386809544514,37.4175684226488,18.763815512673));
#49101=CARTESIAN_POINT('Ctrl Pts',(-7.63482139908449,37.4282854151188,18.7647243494528));
#49102=CARTESIAN_POINT('Ctrl Pts',(-7.66207750307962,37.4545941306971,18.7669846204552));
#49103=CARTESIAN_POINT('Ctrl Pts',(-7.67846386531112,37.4700979460759,18.76834235092));
#49104=CARTESIAN_POINT('Ctrl Pts',(-7.7423009904672,37.5293005692098,18.7736230666405));
#49105=CARTESIAN_POINT('Ctrl Pts',(-7.79083819078676,37.5718027125818,18.7776197936291));
#49106=CARTESIAN_POINT('Ctrl Pts',(-7.92840390429801,37.6854950034228,18.7888300672702));
#49107=CARTESIAN_POINT('Ctrl Pts',(-8.01985465427923,37.7536186715916,18.7961510145572));
#49108=CARTESIAN_POINT('Ctrl Pts',(-8.32923100282967,37.9606866546992,18.8201381309361));
#49109=CARTESIAN_POINT('Ctrl Pts',(-8.55966214074549,38.0793834557709,18.8367393744504));
#49110=CARTESIAN_POINT('Ctrl Pts',(-8.84841550554478,38.1885401013835,18.8554885685725));
#49111=CARTESIAN_POINT('Ctrl Pts',(-8.8958546019063,38.2052766139491,18.8585103434692));
#49112=CARTESIAN_POINT('Ctrl Pts',(-8.97174754735594,38.2301666066708,18.8632544358456));
#49113=CARTESIAN_POINT('Ctrl Pts',(-8.9999645191197,38.2390135123422,18.8649988508767));
#49114=CARTESIAN_POINT('Ctrl Pts',(-9.05375818275718,38.2551095137381,18.8682887301039));
#49115=CARTESIAN_POINT('Ctrl Pts',(-9.07931128525613,38.2624291368385,18.8698363540595));
#49116=CARTESIAN_POINT('Ctrl Pts',(-9.13816202739051,38.2785402534777,18.8733672540571));
#49117=CARTESIAN_POINT('Ctrl Pts',(-9.17151311934725,38.2871264802635,18.8753438874345));
#49118=CARTESIAN_POINT('Ctrl Pts',(-9.27921664916526,38.3131113315731,18.8816540075309));
#49119=CARTESIAN_POINT('Ctrl Pts',(-9.35403032508145,38.3285071268317,18.8859251773574));
#49120=CARTESIAN_POINT('Ctrl Pts',(-9.53807991223995,38.3599422924838,18.8962168845084));
#49121=CARTESIAN_POINT('Ctrl Pts',(-9.64770240680229,38.373198923697,18.9021621190918));
#49122=CARTESIAN_POINT('Ctrl Pts',(-9.97124758164976,38.3963775051253,18.9194654657229));
#49123=CARTESIAN_POINT('Ctrl Pts',(-10.1856666571974,38.3914189824154,18.9306019144693));
#49124=CARTESIAN_POINT('Ctrl Pts',(-10.4657257158652,38.3582930408322,18.9461040473908));
#49125=CARTESIAN_POINT('Ctrl Pts',(-10.5330205381347,38.348271267213,18.9499057276965));
#49126=CARTESIAN_POINT('Ctrl Pts',(-10.6232488906448,38.3320452606206,18.9551602437128));
#49127=CARTESIAN_POINT('Ctrl Pts',(-10.646488931375,38.3276142794452,18.9565278473308));
#49128=CARTESIAN_POINT('Ctrl Pts',(-10.6834014258582,38.3201752180674,18.9587253813454));
#49129=CARTESIAN_POINT('Ctrl Pts',(-10.6971053412979,38.3173249939127,18.959546812163));
#49130=CARTESIAN_POINT('Ctrl Pts',(-10.7262329422082,38.3110784041568,18.9613054144346));
#49131=CARTESIAN_POINT('Ctrl Pts',(-10.7416512321639,38.3076589772876,18.9622438986756));
#49132=CARTESIAN_POINT('Ctrl Pts',(-10.7813302888713,38.2985676883638,18.9646776954431));
#49133=CARTESIAN_POINT('Ctrl Pts',(-10.8055530423254,38.2927359492437,18.9661814368163));
#49134=CARTESIAN_POINT('Ctrl Pts',(-10.9144544496812,38.265243895829,18.9730165798034));
#49135=CARTESIAN_POINT('Ctrl Pts',(-10.9983348363186,38.240581704884,18.978484793347));
#49136=CARTESIAN_POINT('Ctrl Pts',(-11.272293649203,38.1483873099071,18.9968276151663));
#49137=CARTESIAN_POINT('Ctrl Pts',(-11.4573045305303,38.0671387423422,19.0099758697996));
#49138=CARTESIAN_POINT('Ctrl Pts',(-11.7699493716988,37.8951271926131,19.0327164826388));
#49139=CARTESIAN_POINT('Ctrl Pts',(-11.9006164884307,37.8110762423608,19.0424098985284));
#49140=CARTESIAN_POINT('Ctrl Pts',(-12.0602197371496,37.6921775530949,19.0544328831739));
#49141=CARTESIAN_POINT('Ctrl Pts',(-12.0948515084282,37.6653185119369,19.057054615581));
#49142=CARTESIAN_POINT('Ctrl Pts',(-12.1509258423316,37.620061128751,19.0613229001861));
#49143=CARTESIAN_POINT('Ctrl Pts',(-12.1726757357922,37.6020535191987,19.0629844555667));
#49144=CARTESIAN_POINT('Ctrl Pts',(-12.2148345538133,37.566251334666,19.0662179693834));
#49145=CARTESIAN_POINT('Ctrl Pts',(-12.2352602458271,37.5484798820384,19.0677906801247));
#49146=CARTESIAN_POINT('Ctrl Pts',(-12.2836641032722,37.5053362305936,19.0715337851037));
#49147=CARTESIAN_POINT('Ctrl Pts',(-12.31143575106,37.4797371423685,19.0736946403023));
#49148=CARTESIAN_POINT('Ctrl Pts',(-12.4106089966362,37.3852081056333,19.0814674795521));
#49149=CARTESIAN_POINT('Ctrl Pts',(-12.4794055762551,37.3136127210192,19.0869667195723));
#49150=CARTESIAN_POINT('Ctrl Pts',(-12.6561208494848,37.1127574764076,19.1015431875277));
#49151=CARTESIAN_POINT('Ctrl Pts',(-12.7577173892411,36.9783123975225,19.1104189085226));
#49152=CARTESIAN_POINT('Ctrl Pts',(-12.9417520109245,36.6928833302103,19.1284390167693));
#49153=CARTESIAN_POINT('Ctrl Pts',(-13.0235344597169,36.5420720942912,19.1375634827756));
#49154=CARTESIAN_POINT('Ctrl Pts',(-13.1080563742962,36.3533839020144,19.1492398646752));
#49155=CARTESIAN_POINT('Ctrl Pts',(-13.1220429590985,36.3207989877073,19.1512655420536));
#49156=CARTESIAN_POINT('Ctrl Pts',(-13.1423541552481,36.2713533634722,19.1543618390188));
#49157=CARTESIAN_POINT('Ctrl Pts',(-13.1490601993261,36.2546508842353,19.155411566517));
#49158=CARTESIAN_POINT('Ctrl Pts',(-13.1610912394212,36.2239814758689,19.1573474253524));
#49159=CARTESIAN_POINT('Ctrl Pts',(-13.1664573193219,36.2100316091788,19.158231182366));
#49160=CARTESIAN_POINT('Ctrl Pts',(-13.174089201427,36.1897930383037,19.1595179084281));
#49161=CARTESIAN_POINT('Ctrl Pts',(-13.1764289149267,36.1835324577998,19.1599165583278));
#49162=CARTESIAN_POINT('Ctrl Pts',(-13.1787500671498,36.1772650819144,19.1603162262584));
#49163=CARTESIAN_POINT('Origin',(-10.,35.,23.));
#49164=CARTESIAN_POINT('',(-13.1787500668679,36.1772650826756,20.4156323441327));
#49165=CARTESIAN_POINT('',(-13.1787500740781,36.1772650632072,20.0676095644498));
#49166=CARTESIAN_POINT('',(-13.1787500671536,36.1772650819043,23.));
#49167=CARTESIAN_POINT('Ctrl Pts',(-13.1787500740781,36.1772650632072,20.0676095644498));
#49168=CARTESIAN_POINT('Ctrl Pts',(-13.1746481889117,36.1883406214516,20.0668917208588));
#49169=CARTESIAN_POINT('Ctrl Pts',(-13.1704879689934,36.1993959560735,20.066175595704));
#49170=CARTESIAN_POINT('Ctrl Pts',(-13.1502072770507,36.2524466119533,20.0627410937961));
#49171=CARTESIAN_POINT('Ctrl Pts',(-13.1333097411937,36.2941401629776,20.0600477707336));
#49172=CARTESIAN_POINT('Ctrl Pts',(-13.104369160782,36.3616562938897,20.0556942975385));
#49173=CARTESIAN_POINT('Ctrl Pts',(-13.092822079692,36.3876841882828,20.0540179476221));
#49174=CARTESIAN_POINT('Ctrl Pts',(-13.0697111426167,36.4380558681641,20.050776518079));
#49175=CARTESIAN_POINT('Ctrl Pts',(-13.0581822547919,36.4624132579488,20.049210410293));
#49176=CARTESIAN_POINT('Ctrl Pts',(-13.030131040444,36.5198950407201,20.045516217134));
#49177=CARTESIAN_POINT('Ctrl Pts',(-13.0133540221758,36.5528917369351,20.0433970020786));
#49178=CARTESIAN_POINT('Ctrl Pts',(-12.9550659329678,36.6630283007685,20.0363216581615));
#49179=CARTESIAN_POINT('Ctrl Pts',(-12.9111049838055,36.73883503347,20.0314497067886));
#49180=CARTESIAN_POINT('Ctrl Pts',(-12.7185874906963,37.0430060999382,20.0117420460759));
#49181=CARTESIAN_POINT('Ctrl Pts',(-12.5457249798516,37.2547431657124,19.9977238366642));
#49182=CARTESIAN_POINT('Ctrl Pts',(-12.301572191913,37.4894923488405,19.9793837759671));
#49183=CARTESIAN_POINT('Ctrl Pts',(-12.2524099465646,37.534059048756,19.9757471210263));
#49184=CARTESIAN_POINT('Ctrl Pts',(-12.1677320496253,37.6064096683398,19.9695147238718));
#49185=CARTESIAN_POINT('Ctrl Pts',(-12.1329116527835,37.6349802803739,19.9669602621342));
#49186=CARTESIAN_POINT('Ctrl Pts',(-12.0820209617161,37.6750670572722,19.963221950236));
#49187=CARTESIAN_POINT('Ctrl Pts',(-12.0664016676778,37.6871507499599,19.9620739438972));
#49188=CARTESIAN_POINT('Ctrl Pts',(-12.038782313622,37.7081349551153,19.960041072472));
#49189=CARTESIAN_POINT('Ctrl Pts',(-12.0268276111752,37.7170936825634,19.959160167627));
#49190=CARTESIAN_POINT('Ctrl Pts',(-12.0002814568725,37.7367144008505,19.9572015004046));
#49191=CARTESIAN_POINT('Ctrl Pts',(-11.9856639066511,37.7473387916401,19.9561214381139));
#49192=CARTESIAN_POINT('Ctrl Pts',(-11.94181470817,37.778676705131,19.9528786920042));
#49193=CARTESIAN_POINT('Ctrl Pts',(-11.912339749599,37.7990435964089,19.9506952775332));
#49194=CARTESIAN_POINT('Ctrl Pts',(-11.7563138613436,37.9032410959823,19.9391411644117));
#49195=CARTESIAN_POINT('Ctrl Pts',(-11.624568263956,37.9789625652757,19.9294056030737));
#49196=CARTESIAN_POINT('Ctrl Pts',(-11.3683758866146,38.1041488289136,19.9110351726018));
#49197=CARTESIAN_POINT('Ctrl Pts',(-11.2451910205221,38.1555814743432,19.9024248664836));
#49198=CARTESIAN_POINT('Ctrl Pts',(-11.0288920205865,38.2312472263064,19.8878753173445));
#49199=CARTESIAN_POINT('Ctrl Pts',(-10.937186569662,38.2590276260626,19.8818722575603));
#49200=CARTESIAN_POINT('Ctrl Pts',(-10.7773697535569,38.3001355649519,19.8717198153037));
#49201=CARTESIAN_POINT('Ctrl Pts',(-10.7098018875377,38.3153251427303,19.8675197638821));
#49202=CARTESIAN_POINT('Ctrl Pts',(-10.6091932039276,38.3347252168402,19.8613993562556));
#49203=CARTESIAN_POINT('Ctrl Pts',(-10.5764825577093,38.3405353777558,19.8594299840065));
#49204=CARTESIAN_POINT('Ctrl Pts',(-10.5178134127196,38.3500689034386,19.8559332230054));
#49205=CARTESIAN_POINT('Ctrl Pts',(-10.4918875079849,38.3539736321139,19.8544003109999));
#49206=CARTESIAN_POINT('Ctrl Pts',(-10.4359887075654,38.361730498224,19.8511206308588));
#49207=CARTESIAN_POINT('Ctrl Pts',(-10.4060041946999,38.3654834385051,19.849377057284));
#49208=CARTESIAN_POINT('Ctrl Pts',(-10.324246597414,38.374607848468,19.8446629714049));
#49209=CARTESIAN_POINT('Ctrl Pts',(-10.2723925404282,38.3791887626699,19.8417167821468));
#49210=CARTESIAN_POINT('Ctrl Pts',(-9.98601941611297,38.3978524774416,19.8256514175369));
#49211=CARTESIAN_POINT('Ctrl Pts',(-9.75063268142627,38.3887201089399,19.8132607551762));
#49212=CARTESIAN_POINT('Ctrl Pts',(-9.33497104200979,38.3290174259411,19.7909831091838));
#49213=CARTESIAN_POINT('Ctrl Pts',(-9.15435588456849,38.2877790080985,19.7811409946492));
#49214=CARTESIAN_POINT('Ctrl Pts',(-8.95044428321495,38.2233018574705,19.768972268358));
#49215=CARTESIAN_POINT('Ctrl Pts',(-8.92297318446377,38.2142269969063,19.7673097128734));
#49216=CARTESIAN_POINT('Ctrl Pts',(-8.87987539986128,38.1993754645878,19.7646598753113));
#49217=CARTESIAN_POINT('Ctrl Pts',(-8.86416878390821,38.1938331055786,19.7636853845228));
#49218=CARTESIAN_POINT('Ctrl Pts',(-8.83428349181316,38.1830392218888,19.7618132767603));
#49219=CARTESIAN_POINT('Ctrl Pts',(-8.82009811659088,38.1778082348519,19.7609168055625));
#49220=CARTESIAN_POINT('Ctrl Pts',(-8.78845175370926,38.1658972532263,19.7588998727725));
#49221=CARTESIAN_POINT('Ctrl Pts',(-8.77101008686548,38.1591673475547,19.7577766439844));
#49222=CARTESIAN_POINT('Ctrl Pts',(-8.70998068782779,38.1350371429179,19.7538077436741));
#49223=CARTESIAN_POINT('Ctrl Pts',(-8.66670126424905,38.116876920112,19.7509235806817));
#49224=CARTESIAN_POINT('Ctrl Pts',(-8.43337429521405,38.0132232174265,19.7350453057583));
#49225=CARTESIAN_POINT('Ctrl Pts',(-8.25114908510957,37.9112445165442,19.7214711749323));
#49226=CARTESIAN_POINT('Ctrl Pts',(-8.04009636564505,37.7661278883454,19.7050222434688));
#49227=CARTESIAN_POINT('Ctrl Pts',(-8.00132003569355,37.7382410991211,19.7019654143914));
#49228=CARTESIAN_POINT('Ctrl Pts',(-7.88169184199549,37.6483125797003,19.6924382532026));
#49229=CARTESIAN_POINT('Ctrl Pts',(-7.80303617469414,37.5834360116449,19.6860335012907));
#49230=CARTESIAN_POINT('Ctrl Pts',(-7.67377195495666,37.4666365112751,19.6752958110445));
#49231=CARTESIAN_POINT('Ctrl Pts',(-7.62168775418397,37.4164570426838,19.6709037698695));
#49232=CARTESIAN_POINT('Ctrl Pts',(-7.54769891797832,37.3404623048075,19.6645637840062));
#49233=CARTESIAN_POINT('Ctrl Pts',(-7.52451447077213,37.3159265781363,19.6625615742977));
#49234=CARTESIAN_POINT('Ctrl Pts',(-7.4837856083522,37.2715133096524,19.6590147723866));
#49235=CARTESIAN_POINT('Ctrl Pts',(-7.46610086686064,37.2517688209343,19.6574643827435));
#49236=CARTESIAN_POINT('Ctrl Pts',(-7.42892518230136,37.2092706455652,19.6541819018539));
#49237=CARTESIAN_POINT('Ctrl Pts',(-7.40950055397257,37.1864618008938,19.6524525883054));
#49238=CARTESIAN_POINT('Ctrl Pts',(-7.35793194002284,37.1242566623269,19.6478203001039));
#49239=CARTESIAN_POINT('Ctrl Pts',(-7.32636712091726,37.0843890246193,19.6449402007254));
#49240=CARTESIAN_POINT('Ctrl Pts',(-7.14580335498472,36.8454757933509,19.6281597817043));
#49241=CARTESIAN_POINT('Ctrl Pts',(-7.01817291413066,36.6312380959689,19.6150946905916));
#49242=CARTESIAN_POINT('Ctrl Pts',(-6.86567257296838,36.2963901077095,19.5955562926053));
#49243=CARTESIAN_POINT('Ctrl Pts',(-6.82199734694118,36.1852981352074,19.5891901021845));
#49244=CARTESIAN_POINT('Ctrl Pts',(-6.76329638196891,36.0092334878109,19.5789694892443));
#49245=CARTESIAN_POINT('Ctrl Pts',(-6.74417400275514,35.9457264251997,19.5752567306465));
#49246=CARTESIAN_POINT('Ctrl Pts',(-6.72100311517982,35.8597111540797,19.5701438171519));
#49247=CARTESIAN_POINT('Ctrl Pts',(-6.71530068859649,35.8376599621526,19.5688256990064));
#49248=CARTESIAN_POINT('Ctrl Pts',(-6.70612460584923,35.8006409937981,19.5665980593921));
#49249=CARTESIAN_POINT('Ctrl Pts',(-6.70252960948114,35.7857035889831,19.5656951610231));
#49250=CARTESIAN_POINT('Ctrl Pts',(-6.69528111933497,35.7546594863426,19.5638094620014));
#49251=CARTESIAN_POINT('Ctrl Pts',(-6.69164361627216,35.738549817976,19.5628258901429));
#49252=CARTESIAN_POINT('Ctrl Pts',(-6.6820983079581,35.6947897978722,19.5601417160081));
#49253=CARTESIAN_POINT('Ctrl Pts',(-6.67641863314986,35.6670916621244,19.5584293590153));
#49254=CARTESIAN_POINT('Ctrl Pts',(-6.6440048582426,35.4983162076584,19.5479272858178));
#49255=CARTESIAN_POINT('Ctrl Pts',(-6.62591283485192,35.3557396668313,19.5387733092486));
#49256=CARTESIAN_POINT('Ctrl Pts',(-6.60455275586004,35.0156156354847,19.5168567475431));
#49257=CARTESIAN_POINT('Ctrl Pts',(-6.60939366282214,34.8180503603989,19.5040823821948));
#49258=CARTESIAN_POINT('Ctrl Pts',(-6.64341459676024,34.5148515074624,19.4849484694782));
#49259=CARTESIAN_POINT('Ctrl Pts',(-6.66054759682791,34.4083108671089,19.4783101271036));
#49260=CARTESIAN_POINT('Ctrl Pts',(-6.69071701979547,34.2647735857211,19.4694918551654));
#49261=CARTESIAN_POINT('Ctrl Pts',(-6.69935316299162,34.2269266732445,19.4671784081731));
#49262=CARTESIAN_POINT('Ctrl Pts',(-6.71515758638176,34.1627673951826,19.4632750764709));
#49263=CARTESIAN_POINT('Ctrl Pts',(-6.72199659912525,34.1363786214932,19.4616749996981));
#49264=CARTESIAN_POINT('Ctrl Pts',(-6.73563134885518,34.0862652333679,19.4586457208562));
#49265=CARTESIAN_POINT('Ctrl Pts',(-6.74236926027316,34.0625268404369,19.4572147959216));
#49266=CARTESIAN_POINT('Ctrl Pts',(-6.75880169764879,34.0069511230665,19.453873141394));
#49267=CARTESIAN_POINT('Ctrl Pts',(-6.76870714444392,33.975178503657,19.4519692488166));
#49268=CARTESIAN_POINT('Ctrl Pts',(-6.80619309705904,33.86089010105,19.4451393586131));
#49269=CARTESIAN_POINT('Ctrl Pts',(-6.8364807470101,33.7792946699934,19.44029949432));
#49270=CARTESIAN_POINT('Ctrl Pts',(-6.97200284650646,33.4532495636193,19.4209636923964));
#49271=CARTESIAN_POINT('Ctrl Pts',(-7.10269551438376,33.2204429127832,19.4072427031282));
#49272=CARTESIAN_POINT('Ctrl Pts',(-7.300758236245,32.9483002251139,19.3890639541454));
#49273=CARTESIAN_POINT('Ctrl Pts',(-7.34402222694572,32.8925942210297,19.3852088298101));
#49274=CARTESIAN_POINT('Ctrl Pts',(-7.41897360533566,32.8020649558604,19.3786433969239));
#49275=CARTESIAN_POINT('Ctrl Pts',(-7.44970645616594,32.7664785435094,19.3759803259579));
#49276=CARTESIAN_POINT('Ctrl Pts',(-7.49460319739658,32.7166264020737,19.3721114058172));
#49277=CARTESIAN_POINT('Ctrl Pts',(-7.50817047492936,32.7018281827625,19.3709449417286));
#49278=CARTESIAN_POINT('Ctrl Pts',(-7.53208044883887,32.676209523852,19.3688920674883));
#49279=CARTESIAN_POINT('Ctrl Pts',(-7.54236462911873,32.6653356854624,19.3680099072379));
#49280=CARTESIAN_POINT('Ctrl Pts',(-7.56506307204315,32.6416519782033,19.366064224167));
#49281=CARTESIAN_POINT('Ctrl Pts',(-7.57750645713788,32.6288719480635,19.3649986225416));
#49282=CARTESIAN_POINT('Ctrl Pts',(-7.61368819539718,32.5922934352367,19.3619047098435));
#49283=CARTESIAN_POINT('Ctrl Pts',(-7.63767978540804,32.5687497144543,19.3598587429436));
#49284=CARTESIAN_POINT('Ctrl Pts',(-7.80847053961603,32.4060620111369,19.3453577430601));
#49285=CARTESIAN_POINT('Ctrl Pts',(-7.96710660652606,32.2799541602845,19.33223913149));
#49286=CARTESIAN_POINT('Ctrl Pts',(-8.26023889405901,32.0869683071562,19.3096377418253));
#49287=CARTESIAN_POINT('Ctrl Pts',(-8.38971074011162,32.0134472314179,19.3001297483767));
#49288=CARTESIAN_POINT('Ctrl Pts',(-8.60679005159429,31.9084127982974,19.2851090027198));
#49289=CARTESIAN_POINT('Ctrl Pts',(-8.69159424775899,31.8715783239885,19.2794505214719));
#49290=CARTESIAN_POINT('Ctrl Pts',(-8.81218468804827,31.8249632312105,19.2716938098448));
#49291=CARTESIAN_POINT('Ctrl Pts',(-8.84678053863947,31.8122345234694,19.2695006731047));
#49292=CARTESIAN_POINT('Ctrl Pts',(-8.90699300037439,31.7911893824084,19.2657375593471));
#49293=CARTESIAN_POINT('Ctrl Pts',(-8.93251327023129,31.7826094385677,19.2641591333279));
#49294=CARTESIAN_POINT('Ctrl Pts',(-8.98527935284905,31.7655663806991,19.2609284559228));
#49295=CARTESIAN_POINT('Ctrl Pts',(-9.01253526895736,31.7571413372478,19.2592775386029));
#49296=CARTESIAN_POINT('Ctrl Pts',(-9.08328316424185,31.7362472454735,19.2550363550548));
#49297=CARTESIAN_POINT('Ctrl Pts',(-9.12692493479394,31.7243028221104,19.2524628938555));
#49298=CARTESIAN_POINT('Ctrl Pts',(-9.36522482443571,31.6641830225298,19.2386207620168));
#49299=CARTESIAN_POINT('Ctrl Pts',(-9.5636312785151,31.6324774247616,19.2278820128614));
#49300=CARTESIAN_POINT('Ctrl Pts',(-9.9266933244055,31.6071060370756,19.2085661712198));
#49301=CARTESIAN_POINT('Ctrl Pts',(-10.0902933164566,31.6075164136381,19.1999726962771));
#49302=CARTESIAN_POINT('Ctrl Pts',(-10.3320395342068,31.6256255621093,19.1867233754342));
#49303=CARTESIAN_POINT('Ctrl Pts',(-10.4106269333618,31.6342850999612,19.182327065726));
#49304=CARTESIAN_POINT('Ctrl Pts',(-10.5127328363551,31.6491652684983,19.1764173597361));
#49305=CARTESIAN_POINT('Ctrl Pts',(-10.5365932898354,31.6529033582388,19.1750221288207));
#49306=CARTESIAN_POINT('Ctrl Pts',(-10.5758293217941,31.659480570528,19.172701363434));
#49307=CARTESIAN_POINT('Ctrl Pts',(-10.5912293195967,31.6621717623279,19.1717837275779));
#49308=CARTESIAN_POINT('Ctrl Pts',(-10.6205078232576,31.6674972400463,19.1700253444571));
#49309=CARTESIAN_POINT('Ctrl Pts',(-10.6343894912911,31.6701119296227,19.1691857716318));
#49310=CARTESIAN_POINT('Ctrl Pts',(-10.6721683023672,31.6774725836025,19.1668856000318));
#49311=CARTESIAN_POINT('Ctrl Pts',(-10.6960308013067,31.6823894580117,19.1654160213758));
#49312=CARTESIAN_POINT('Ctrl Pts',(-10.7923723209155,31.7033257759096,19.1594207118596));
#49313=CARTESIAN_POINT('Ctrl Pts',(-10.8643649064742,31.7214657887102,19.1547981933379));
#49314=CARTESIAN_POINT('Ctrl Pts',(-11.1356775609669,31.7993857317645,19.1369723423511));
#49315=CARTESIAN_POINT('Ctrl Pts',(-11.3299418694936,31.8751078431174,19.1233948854259));
#49316=CARTESIAN_POINT('Ctrl Pts',(-11.6138236153652,32.0170599741632,19.1031332904401));
#49317=CARTESIAN_POINT('Ctrl Pts',(-11.7091919274473,32.0706615010458,19.096240130547));
#49318=CARTESIAN_POINT('Ctrl Pts',(-11.8660783264693,32.1691142894761,19.0848010239855));
#49319=CARTESIAN_POINT('Ctrl Pts',(-11.9289786386675,32.2115945419809,19.0801848533728));
#49320=CARTESIAN_POINT('Ctrl Pts',(-12.0182121526282,32.2763250965903,19.0735902758953));
#49321=CARTESIAN_POINT('Ctrl Pts',(-12.045712752512,32.2969193987151,19.0715511663265));
#49322=CARTESIAN_POINT('Ctrl Pts',(-12.0939168991972,32.3341750082714,19.0679635834466));
#49323=CARTESIAN_POINT('Ctrl Pts',(-12.1147461978105,32.3506681133217,19.0664088054572));
#49324=CARTESIAN_POINT('Ctrl Pts',(-12.1583737002382,32.3860557375712,19.0631415289015));
#49325=CARTESIAN_POINT('Ctrl Pts',(-12.1811226673032,32.4050075862408,19.0614314792296));
#49326=CARTESIAN_POINT('Ctrl Pts',(-12.2419873958665,32.457079051722,19.0568364870027));
#49327=CARTESIAN_POINT('Ctrl Pts',(-12.2796169646292,32.4907568277201,19.0539742479324));
#49328=CARTESIAN_POINT('Ctrl Pts',(-12.5039500931819,32.7007442959409,19.0367435136889));
#49329=CARTESIAN_POINT('Ctrl Pts',(-12.6708715753343,32.8969548691086,19.0232783395124));
#49330=CARTESIAN_POINT('Ctrl Pts',(-12.9075582767635,33.2493877737716,19.000718507335));
#49331=CARTESIAN_POINT('Ctrl Pts',(-12.9905972085184,33.3953647767369,18.991734581058));
#49332=CARTESIAN_POINT('Ctrl Pts',(-13.0747329638813,33.5726813072942,18.9805621173631));
#49333=CARTESIAN_POINT('Ctrl Pts',(-13.086654245125,33.5986481859257,18.9789195747798));
#49334=CARTESIAN_POINT('Ctrl Pts',(-13.1049713986649,33.6399145169202,18.9762944763266));
#49335=CARTESIAN_POINT('Ctrl Pts',(-13.1115859536996,33.6551160885171,18.9753243173024));
#49336=CARTESIAN_POINT('Ctrl Pts',(-13.1240326132902,33.6843043947198,18.9734544326089));
#49337=CARTESIAN_POINT('Ctrl Pts',(-13.1298828549991,33.6982826822769,18.9725557686771));
#49338=CARTESIAN_POINT('Ctrl Pts',(-13.1441674203176,33.7330665727496,18.9703123790643));
#49339=CARTESIAN_POINT('Ctrl Pts',(-13.1524890655588,33.7539174552925,18.9689613431577));
#49340=CARTESIAN_POINT('Ctrl Pts',(-13.1819053277365,33.8298045141081,18.964025611232));
#49341=CARTESIAN_POINT('Ctrl Pts',(-13.2017696931057,33.8853031942499,18.9603808025434));
#49342=CARTESIAN_POINT('Ctrl Pts',(-13.282114859431,34.1296808341905,18.9442618499703));
#49343=CARTESIAN_POINT('Ctrl Pts',(-13.3273998389391,34.323139501773,18.9313474947223));
#49344=CARTESIAN_POINT('Ctrl Pts',(-13.3782228220261,34.6780122634763,18.908343335226));
#49345=CARTESIAN_POINT('Ctrl Pts',(-13.3896658156566,34.8380079264556,18.8982113280507));
#49346=CARTESIAN_POINT('Ctrl Pts',(-13.3897786081615,35.0538627721316,18.8849937840186));
#49347=CARTESIAN_POINT('Ctrl Pts',(-13.3884380466477,35.1094913576134,18.8816262725728));
#49348=CARTESIAN_POINT('Ctrl Pts',(-13.3840803196029,35.1988752088003,18.8762763153671));
#49349=CARTESIAN_POINT('Ctrl Pts',(-13.3819255185102,35.2326604180868,18.8742681345242));
#49350=CARTESIAN_POINT('Ctrl Pts',(-13.3771810294872,35.2928419726195,18.8707147101195));
#49351=CARTESIAN_POINT('Ctrl Pts',(-13.3747870021675,35.3192504911896,18.8691635881286));
#49352=CARTESIAN_POINT('Ctrl Pts',(-13.3690346183339,35.3753728951024,18.8658835758968));
#49353=CARTESIAN_POINT('Ctrl Pts',(-13.3655924526277,35.4050760364955,18.8641574090822));
#49354=CARTESIAN_POINT('Ctrl Pts',(-13.3551001603312,35.4862126207624,18.8594666442448));
#49355=CARTESIAN_POINT('Ctrl Pts',(-13.3472607242299,35.5375368298244,18.8565264589389));
#49356=CARTESIAN_POINT('Ctrl Pts',(-13.3091780690012,35.7534996137863,18.8442430039122));
#49357=CARTESIAN_POINT('Ctrl Pts',(-13.2679409780853,35.9159642102598,18.8352348808651));
#49358=CARTESIAN_POINT('Ctrl Pts',(-13.2033727732961,36.1091086076841,18.8244023662525));
#49359=CARTESIAN_POINT('Ctrl Pts',(-13.1913324612675,36.1432911799257,18.8224796684973));
#49360=CARTESIAN_POINT('Ctrl Pts',(-13.1787500897853,36.1772650207959,18.8205585884996));
#49361=CARTESIAN_POINT('',(-13.3897486112447,35.0022154189341,19.236243357794));
#49362=CARTESIAN_POINT('Ctrl Pts',(-13.1787500671498,36.1772650819144,19.1603162262584));
#49363=CARTESIAN_POINT('Ctrl Pts',(-13.1833209132271,36.1649232758945,19.1611032580501));
#49364=CARTESIAN_POINT('Ctrl Pts',(-13.1878197822913,36.1525551186986,19.1618942373848));
#49365=CARTESIAN_POINT('Ctrl Pts',(-13.2075901839104,36.0972015494627,19.1654433738761));
#49366=CARTESIAN_POINT('Ctrl Pts',(-13.2220643860508,36.0539386562107,19.1682417168197));
#49367=CARTESIAN_POINT('Ctrl Pts',(-13.2557961376661,35.9459174962265,19.1752668961463));
#49368=CARTESIAN_POINT('Ctrl Pts',(-13.2739988194855,35.8808514098209,19.17953178583));
#49369=CARTESIAN_POINT('Ctrl Pts',(-13.3561519696634,35.5493074944838,19.2012975900872));
#49370=CARTESIAN_POINT('Ctrl Pts',(-13.3895698315011,35.2762817947677,19.2192236441355));
#49371=CARTESIAN_POINT('Ctrl Pts',(-13.3897492734148,35.0022194331732,19.2362442617547));
#49372=CARTESIAN_POINT('Ctrl Pts',(-13.3897492759939,35.0022154907005,19.2362445066015));
#49373=CARTESIAN_POINT('Ctrl Pts',(-13.3897859513971,34.9461013207655,19.2397294702646));
#49374=CARTESIAN_POINT('Ctrl Pts',(-13.3884292511353,34.8899920833807,19.2431782295167));
#49375=CARTESIAN_POINT('Ctrl Pts',(-13.3835973433518,34.7914781253556,19.2491688806532));
#49376=CARTESIAN_POINT('Ctrl Pts',(-13.3807160429095,34.7490585006874,19.2517273939982));
#49377=CARTESIAN_POINT('Ctrl Pts',(-13.3747937564741,34.6808690193758,19.2558074152118));
#49378=CARTESIAN_POINT('Ctrl Pts',(-13.3722536726454,34.6550613026596,19.2573440137728));
#49379=CARTESIAN_POINT('Ctrl Pts',(-13.3666222901008,34.603877871851,19.2603770776508));
#49380=CARTESIAN_POINT('Ctrl Pts',(-13.3635396053426,34.5785029524776,19.2618737031685));
#49381=CARTESIAN_POINT('Ctrl Pts',(-13.3563330893324,34.5243104450402,19.2650557919355));
#49382=CARTESIAN_POINT('Ctrl Pts',(-13.3521244500627,34.4955060881943,19.2667384995122));
#49383=CARTESIAN_POINT('Ctrl Pts',(-13.3399839648154,34.4192913716709,19.2711700603055));
#49384=CARTESIAN_POINT('Ctrl Pts',(-13.331413715781,34.3719885568378,19.2738990212357));
#49385=CARTESIAN_POINT('Ctrl Pts',(-13.276703108367,34.1027912260741,19.2893334004269));
#49386=CARTESIAN_POINT('Ctrl Pts',(-13.2094077981967,33.8857823812972,19.301350816821));
#49387=CARTESIAN_POINT('Ctrl Pts',(-13.0664686385234,33.5485648649071,19.3207686233031));
#49388=CARTESIAN_POINT('Ctrl Pts',(-13.0041014865471,33.4235280404811,19.3281642250464));
#49389=CARTESIAN_POINT('Ctrl Pts',(-12.8978338807741,33.239817879346,19.3398060197016));
#49390=CARTESIAN_POINT('Ctrl Pts',(-12.8594500708009,33.1781256557972,19.3438595595536));
#49391=CARTESIAN_POINT('Ctrl Pts',(-12.8060708022103,33.0981788411377,19.3493707187719));
#49392=CARTESIAN_POINT('Ctrl Pts',(-12.7928220670751,33.078775936306,19.3507291241371));
#49393=CARTESIAN_POINT('Ctrl Pts',(-12.7704993626501,33.0468029720778,19.3530051875142));
#49394=CARTESIAN_POINT('Ctrl Pts',(-12.7615386494156,33.0341542211689,19.3539155624273));
#49395=CARTESIAN_POINT('Ctrl Pts',(-12.7441683572752,33.0099878257811,19.3556749693573));
#49396=CARTESIAN_POINT('Ctrl Pts',(-12.7357723256925,32.9984610440331,19.356522997312));
#49397=CARTESIAN_POINT('Ctrl Pts',(-12.7124179384345,32.9668196491567,19.3588745475498));
#49398=CARTESIAN_POINT('Ctrl Pts',(-12.6973091128324,32.9468178647107,19.3603877159618));
#49399=CARTESIAN_POINT('Ctrl Pts',(-12.6321300198654,32.8624918262777,19.3668749505465));
#49400=CARTESIAN_POINT('Ctrl Pts',(-12.5799731120531,32.79982128501,19.3719662232217));
#49401=CARTESIAN_POINT('Ctrl Pts',(-12.3913289807048,32.5890904959606,19.3898815374649));
#49402=CARTESIAN_POINT('Ctrl Pts',(-12.2439493319577,32.4513470055959,19.4030089220356));
#49403=CARTESIAN_POINT('Ctrl Pts',(-11.9575449564879,32.2278806502156,19.4261891081191));
#49404=CARTESIAN_POINT('Ctrl Pts',(-11.8228877864242,32.1375325555115,19.4363173200672));
#49405=CARTESIAN_POINT('Ctrl Pts',(-11.6445808430822,32.0356040037148,19.4487200711556));
#49406=CARTESIAN_POINT('Ctrl Pts',(-11.6064794796322,32.0147841424693,19.4513166603101));
#49407=CARTESIAN_POINT('Ctrl Pts',(-11.5430275658565,31.9816786837632,19.4555550498077));
#49408=CARTESIAN_POINT('Ctrl Pts',(-11.517906023229,31.9689673355246,19.4572114402722));
#49409=CARTESIAN_POINT('Ctrl Pts',(-11.4685520455162,31.9447620293955,19.4604245764479));
#49410=CARTESIAN_POINT('Ctrl Pts',(-11.4443358755747,31.9332398029091,19.4619822017545));
#49411=CARTESIAN_POINT('Ctrl Pts',(-11.3856318006525,31.9061575852501,19.4657141376613));
#49412=CARTESIAN_POINT('Ctrl Pts',(-11.3510147644108,31.8908850707872,19.4678786573922));
#49413=CARTESIAN_POINT('Ctrl Pts',(-11.2307700840454,31.8402225544561,19.4752807359053));
#49414=CARTESIAN_POINT('Ctrl Pts',(-11.1439488643843,31.8077638749011,19.4804228455331));
#49415=CARTESIAN_POINT('Ctrl Pts',(-10.8030076912662,31.6960006957601,19.5000159423903));
#49416=CARTESIAN_POINT('Ctrl Pts',(-10.5412490019225,31.6431751690629,19.5137249585293));
#49417=CARTESIAN_POINT('Ctrl Pts',(-10.2103794336094,31.6161438562228,19.5317064137122));
#49418=CARTESIAN_POINT('Ctrl Pts',(-10.1446042300187,31.6126956646164,19.5353173718313));
#49419=CARTESIAN_POINT('Ctrl Pts',(-10.0339828742907,31.6101242586555,19.5415104164065));
#49420=CARTESIAN_POINT('Ctrl Pts',(-9.98917784940192,31.6099712593154,19.5440518981458));
#49421=CARTESIAN_POINT('Ctrl Pts',(-9.92467973627502,31.6110296060087,19.5477745778743));
#49422=CARTESIAN_POINT('Ctrl Pts',(-9.90497795183971,31.6115247908046,19.5489203448823));
#49423=CARTESIAN_POINT('Ctrl Pts',(-9.87035382763641,31.6126972320095,19.5509508208465));
#49424=CARTESIAN_POINT('Ctrl Pts',(-9.85542991136827,31.6133013642996,19.551831604835));
#49425=CARTESIAN_POINT('Ctrl Pts',(-9.82242917742865,31.6148557921981,19.5537919824455));
#49426=CARTESIAN_POINT('Ctrl Pts',(-9.80435589183241,31.6158522409432,19.5548739041302));
#49427=CARTESIAN_POINT('Ctrl Pts',(-9.75038309739215,31.6192617592164,19.5581279409394));
#49428=CARTESIAN_POINT('Ctrl Pts',(-9.71451419376199,31.6221016470966,19.5603209918448));
#49429=CARTESIAN_POINT('Ctrl Pts',(-9.52853492721746,31.6398096201221,19.5718274999163));
#49430=CARTESIAN_POINT('Ctrl Pts',(-9.37950415595507,31.6641138383263,19.5815003205184));
#49431=CARTESIAN_POINT('Ctrl Pts',(-9.10403298677183,31.7281395686387,19.5997200329444));
#49432=CARTESIAN_POINT('Ctrl Pts',(-8.97731579142982,31.7655066802657,19.6082423553762));
#49433=CARTESIAN_POINT('Ctrl Pts',(-8.71672277903737,31.859202815516,19.6258343873426));
#49434=CARTESIAN_POINT('Ctrl Pts',(-8.58362070499405,31.9169356582054,19.6348561736552));
#49435=CARTESIAN_POINT('Ctrl Pts',(-8.41696361149814,32.0023025669185,19.6461522068079));
#49436=CARTESIAN_POINT('Ctrl Pts',(-8.37968091993087,32.0222893980235,19.6486800011991));
#49437=CARTESIAN_POINT('Ctrl Pts',(-8.31841797384137,32.0566232111149,19.652836635119));
#49438=CARTESIAN_POINT('Ctrl Pts',(-8.29422433373469,32.0705777910784,19.6544789544498));
#49439=CARTESIAN_POINT('Ctrl Pts',(-8.24701869200418,32.0985885309955,19.6576859501265));
#49440=CARTESIAN_POINT('Ctrl Pts',(-8.22399652542444,32.1126233881965,19.6592512283196));
#49441=CARTESIAN_POINT('Ctrl Pts',(-8.17354492233872,32.1442116320417,19.6626854777171));
#49442=CARTESIAN_POINT('Ctrl Pts',(-8.14619586299924,32.1618887127506,19.6645498156955));
#49443=CARTESIAN_POINT('Ctrl Pts',(-8.05189841026667,32.2247826603346,19.6709919374897));
#49444=CARTESIAN_POINT('Ctrl Pts',(-7.98631255448871,32.2719979245523,19.675496838413));
#49445=CARTESIAN_POINT('Ctrl Pts',(-7.70095134512102,32.4933340632817,19.6953339550285));
#49446=CARTESIAN_POINT('Ctrl Pts',(-7.5016156007714,32.6919565368106,19.7097473743365));
#49447=CARTESIAN_POINT('Ctrl Pts',(-7.28779451961526,32.9655892205927,19.7285441706244));
#49448=CARTESIAN_POINT('Ctrl Pts',(-7.24815234748168,33.019540612387,19.7322119169322));
#49449=CARTESIAN_POINT('Ctrl Pts',(-7.1843913628039,33.1119302622325,19.738491877043));
#49450=CARTESIAN_POINT('Ctrl Pts',(-7.15939938875763,33.1497440470904,19.7410619858739));
#49451=CARTESIAN_POINT('Ctrl Pts',(-7.12459263146445,33.2047759458082,19.7448191366729));
#49452=CARTESIAN_POINT('Ctrl Pts',(-7.11415798676445,33.2215982530906,19.7459698343339));
#49453=CARTESIAN_POINT('Ctrl Pts',(-7.09610629491205,33.2512776917493,19.7480055885666));
#49454=CARTESIAN_POINT('Ctrl Pts',(-7.0884259896767,33.2640952986017,19.7488866424555));
#49455=CARTESIAN_POINT('Ctrl Pts',(-7.07166314076046,33.2924949309947,19.7508432691994));
#49456=CARTESIAN_POINT('Ctrl Pts',(-7.06262015615893,33.308098719567,19.7519211083327));
#49457=CARTESIAN_POINT('Ctrl Pts',(-7.03607660937178,33.3547542230724,19.7551504412399));
#49458=CARTESIAN_POINT('Ctrl Pts',(-7.01894136126975,33.3860096940951,19.7573224239395));
#49459=CARTESIAN_POINT('Ctrl Pts',(-6.93478191111249,33.5454340418753,19.7684223412914));
#49460=CARTESIAN_POINT('Ctrl Pts',(-6.87552155421854,33.6775205607052,19.7776814933723));
#49461=CARTESIAN_POINT('Ctrl Pts',(-6.78145685926589,33.929129914246,19.7949788906622));
#49462=CARTESIAN_POINT('Ctrl Pts',(-6.74443751229219,34.047583495572,19.802991267768));
#49463=CARTESIAN_POINT('Ctrl Pts',(-6.68810899949707,34.2700014601163,19.8176172217993));
#49464=CARTESIAN_POINT('Ctrl Pts',(-6.66700664612224,34.3733596589572,19.8242535637967));
#49465=CARTESIAN_POINT('Ctrl Pts',(-6.63934684936884,34.5506737391051,19.8353252439669));
#49466=CARTESIAN_POINT('Ctrl Pts',(-6.6303363811157,34.6241648655108,19.8398248364971));
#49467=CARTESIAN_POINT('Ctrl Pts',(-6.62070470724929,34.7318069576637,19.8462872715072));
#49468=CARTESIAN_POINT('Ctrl Pts',(-6.61818142459289,34.7657620153388,19.848307423722));
#49469=CARTESIAN_POINT('Ctrl Pts',(-6.61460250033738,34.826238860104,19.8518740462407));
#49470=CARTESIAN_POINT('Ctrl Pts',(-6.61334599840029,34.8527454675655,19.8534265593735));
#49471=CARTESIAN_POINT('Ctrl Pts',(-6.61134000417948,34.9090297737922,19.8567014727689));
#49472=CARTESIAN_POINT('Ctrl Pts',(-6.6106714828239,34.9388082220139,19.8584212579233));
#49473=CARTESIAN_POINT('Ctrl Pts',(-6.60991976005278,35.0199362365609,19.8630739525241));
#49474=CARTESIAN_POINT('Ctrl Pts',(-6.6106106493336,35.0712860793639,19.8659831357775));
#49475=CARTESIAN_POINT('Ctrl Pts',(-6.6214922543671,35.3719473195746,19.8828425627138));
#49476=CARTESIAN_POINT('Ctrl Pts',(-6.65801709166713,35.6195326687046,19.8959510611556));
#49477=CARTESIAN_POINT('Ctrl Pts',(-6.75155910422572,35.9757811740877,19.9155113669309));
#49478=CARTESIAN_POINT('Ctrl Pts',(-6.78774636918095,36.0890089950618,19.9218522234144));
#49479=CARTESIAN_POINT('Ctrl Pts',(-6.85321779018722,36.261959684961,19.9320373567151));
#49480=CARTESIAN_POINT('Ctrl Pts',(-6.87844063718257,36.3231199969566,19.9357411443414));
#49481=CARTESIAN_POINT('Ctrl Pts',(-6.91472265543276,36.4042744205853,19.9408435492707));
#49482=CARTESIAN_POINT('Ctrl Pts',(-6.92421942558523,36.4249549953694,19.9421605608939));
#49483=CARTESIAN_POINT('Ctrl Pts',(-6.94047376995444,36.4594314825958,19.9443868850372));
#49484=CARTESIAN_POINT('Ctrl Pts',(-6.94711839880611,36.4732803286641,19.9452895925584));
#49485=CARTESIAN_POINT('Ctrl Pts',(-6.96110536812461,36.5019312482451,19.9471755395472));
#49486=CARTESIAN_POINT('Ctrl Pts',(-6.96846211926132,36.51672545655,19.9481595579424));
#49487=CARTESIAN_POINT('Ctrl Pts',(-6.98871563213885,36.556718608566,19.9508461969604));
#49488=CARTESIAN_POINT('Ctrl Pts',(-7.00182009215659,36.5818101961619,19.9525606067622));
#49489=CARTESIAN_POINT('Ctrl Pts',(-7.08629060749199,36.7387275934138,19.9634510523104));
#49490=CARTESIAN_POINT('Ctrl Pts',(-7.16601568452584,36.8658512162986,19.9730242246334));
#49491=CARTESIAN_POINT('Ctrl Pts',(-7.40146450523306,37.1912073720351,19.9988694706518));
#49492=CARTESIAN_POINT('Ctrl Pts',(-7.57132958598149,37.3781022593344,20.0151344717468));
#49493=CARTESIAN_POINT('Ctrl Pts',(-7.80858444641188,37.5869350989711,20.0345205536798));
#49494=CARTESIAN_POINT('Ctrl Pts',(-7.85802584857969,37.6280188176932,20.0384103482283));
#49495=CARTESIAN_POINT('Ctrl Pts',(-7.93404264179854,37.6876141419592,20.0441730478829));
#49496=CARTESIAN_POINT('Ctrl Pts',(-7.95976165249794,37.7071899039101,20.0460869995352));
#49497=CARTESIAN_POINT('Ctrl Pts',(-8.00493617232509,37.7405645362262,20.0493884189096));
#49498=CARTESIAN_POINT('Ctrl Pts',(-8.02426428940801,37.7545311939911,20.0507822448012));
#49499=CARTESIAN_POINT('Ctrl Pts',(-8.06825554290844,37.7856183633018,20.0539135108066));
#49500=CARTESIAN_POINT('Ctrl Pts',(-8.09300215911319,37.802617639262,20.0556463197875));
#49501=CARTESIAN_POINT('Ctrl Pts',(-8.16050267116758,37.8476779289139,20.0602985979658));
#49502=CARTESIAN_POINT('Ctrl Pts',(-8.20367186002381,37.8751044513944,20.0631948420224));
#49503=CARTESIAN_POINT('Ctrl Pts',(-8.45781675896607,38.0286097414877,20.0798277144288));
#49504=CARTESIAN_POINT('Ctrl Pts',(-8.68138044176266,38.1324207425783,20.0927522951134));
#49505=CARTESIAN_POINT('Ctrl Pts',(-9.08118647019215,38.2676064883701,20.1151586074467));
#49506=CARTESIAN_POINT('Ctrl Pts',(-9.2522846978392,38.3109482404968,20.1245686240925));
#49507=CARTESIAN_POINT('Ctrl Pts',(-9.45422299637824,38.34564721471,20.136230884418));
#49508=CARTESIAN_POINT('Ctrl Pts',(-9.48255203168395,38.3501455651758,20.1378796420496));
#49509=CARTESIAN_POINT('Ctrl Pts',(-9.52736315677967,38.3566791835309,20.1405124568663));
#49510=CARTESIAN_POINT('Ctrl Pts',(-9.5438095815106,38.3589538555199,20.1414839965556));
#49511=CARTESIAN_POINT('Ctrl Pts',(-9.57528735065574,38.3630720417082,20.1433546400792));
#49512=CARTESIAN_POINT('Ctrl Pts',(-9.59031537983691,38.3649357899928,20.1442526561776));
#49513=CARTESIAN_POINT('Ctrl Pts',(-9.62759228764077,38.3693053961751,20.1464916925396));
#49514=CARTESIAN_POINT('Ctrl Pts',(-9.64985427099698,38.371691603106,20.1478389683194));
#49515=CARTESIAN_POINT('Ctrl Pts',(-9.73037933845661,38.3795168139083,20.1527448387466));
#49516=CARTESIAN_POINT('Ctrl Pts',(-9.7887544343873,38.3836671926511,20.1563626406687));
#49517=CARTESIAN_POINT('Ctrl Pts',(-10.0705888312135,38.396384062205,20.1740357449717));
#49518=CARTESIAN_POINT('Ctrl Pts',(-10.2944178722726,38.3843352061911,20.1886533522992));
#49519=CARTESIAN_POINT('Ctrl Pts',(-10.6811970049692,38.3248316346608,20.2136570634508));
#49520=CARTESIAN_POINT('Ctrl Pts',(-10.8448614882688,38.2870589952907,20.2241632800895));
#49521=CARTESIAN_POINT('Ctrl Pts',(-11.0468413028531,38.2243512316133,20.2369384049874));
#49522=CARTESIAN_POINT('Ctrl Pts',(-11.08835357324,38.2105769490652,20.2395546682865));
#49523=CARTESIAN_POINT('Ctrl Pts',(-11.1561937118057,38.1865996582169,20.2438164488122));
#49524=CARTESIAN_POINT('Ctrl Pts',(-11.1826803699991,38.1768645698736,20.2454768790858));
#49525=CARTESIAN_POINT('Ctrl Pts',(-11.2340602819566,38.1572483865664,20.248692009257));
#49526=CARTESIAN_POINT('Ctrl Pts',(-11.2589640144119,38.1474008045813,20.2502476657056));
#49527=CARTESIAN_POINT('Ctrl Pts',(-11.3185585680652,38.1230150434055,20.2539651822138));
#49528=CARTESIAN_POINT('Ctrl Pts',(-11.3531296118309,38.1081924123281,20.2561174499319));
#49529=CARTESIAN_POINT('Ctrl Pts',(-11.4706736034283,38.0554614535248,20.2634275851432));
#49530=CARTESIAN_POINT('Ctrl Pts',(-11.552362497242,38.0147799449385,20.2684932738229));
#49531=CARTESIAN_POINT('Ctrl Pts',(-11.8670839962399,37.841858091817,20.2881167815834));
#49532=CARTESIAN_POINT('Ctrl Pts',(-12.0857190100495,37.6855031020326,20.301911856918));
#49533=CARTESIAN_POINT('Ctrl Pts',(-12.3324347132558,37.4605910924204,20.3199932492261));
#49534=CARTESIAN_POINT('Ctrl Pts',(-12.3798933573563,37.4147188148722,20.3236114857764));
#49535=CARTESIAN_POINT('Ctrl Pts',(-12.4573189112764,37.3353805151204,20.3298156795104));
#49536=CARTESIAN_POINT('Ctrl Pts',(-12.4880151238788,37.3026503703234,20.3323608406852));
#49537=CARTESIAN_POINT('Ctrl Pts',(-12.5312525755986,37.2546738822414,20.336087948429));
#49538=CARTESIAN_POINT('Ctrl Pts',(-12.5443256166716,37.2399109429867,20.3372343468971));
#49539=CARTESIAN_POINT('Ctrl Pts',(-12.567073806651,37.2137660818011,20.3392654935164));
#49540=CARTESIAN_POINT('Ctrl Pts',(-12.5768036806673,37.202432966661,20.340146306676));
#49541=CARTESIAN_POINT('Ctrl Pts',(-12.5981528983106,37.1772307886925,20.3421061837542));
#49542=CARTESIAN_POINT('Ctrl Pts',(-12.6097361740289,37.163332951671,20.343187567674));
#49543=CARTESIAN_POINT('Ctrl Pts',(-12.6432925477366,37.1224096570335,20.3463718478109));
#49544=CARTESIAN_POINT('Ctrl Pts',(-12.6649603964635,37.0951382120961,20.3484939274892));
#49545=CARTESIAN_POINT('Ctrl Pts',(-12.7979282938112,36.9223826739345,20.3619118902352));
#49546=CARTESIAN_POINT('Ctrl Pts',(-12.8976955683043,36.7684198104552,20.3737452838208));
#49547=CARTESIAN_POINT('Ctrl Pts',(-13.0591714039707,36.4685568064207,20.3956963255708));
#49548=CARTESIAN_POINT('Ctrl Pts',(-13.124069307029,36.3249093741373,20.4057970344023));
#49549=CARTESIAN_POINT('Ctrl Pts',(-13.1787500668679,36.1772650826756,20.4156323441327));
#49550=CARTESIAN_POINT('Origin',(-10.,35.,23.));
#49551=CARTESIAN_POINT('',(-13.1787500358286,36.1772651664852,21.6644776847947));
#49552=CARTESIAN_POINT('',(-13.1787500764527,36.1772650567955,21.3230161660245));
#49553=CARTESIAN_POINT('',(-13.1787500671536,36.1772650819043,23.));
#49554=CARTESIAN_POINT('',(-13.3897498409689,34.9989616594858,20.1438254858951));
#49555=CARTESIAN_POINT('Ctrl Pts',(-13.1787500764527,36.1772650567955,21.3230161660245));
#49556=CARTESIAN_POINT('Ctrl Pts',(-13.1402670886756,36.2811735178786,21.3160961033474));
#49557=CARTESIAN_POINT('Ctrl Pts',(-13.0967087805464,36.3831420775156,21.3090033589191));
#49558=CARTESIAN_POINT('Ctrl Pts',(-12.9319072502346,36.7219284421956,21.2847566554013));
#49559=CARTESIAN_POINT('Ctrl Pts',(-12.787829044545,36.946578925495,21.2675899894107));
#49560=CARTESIAN_POINT('Ctrl Pts',(-12.5843279146492,37.1942261447432,21.2480503943131));
#49561=CARTESIAN_POINT('Ctrl Pts',(-12.5486913805438,37.2355205002278,21.24476435188));
#49562=CARTESIAN_POINT('Ctrl Pts',(-12.4914291974183,37.2987237562876,21.2396882918648));
#49563=CARTESIAN_POINT('Ctrl Pts',(-12.4704765363389,37.321227289646,21.2378712414739));
#49564=CARTESIAN_POINT('Ctrl Pts',(-12.4309565104849,37.3625311455461,21.2345167826778));
#49565=CARTESIAN_POINT('Ctrl Pts',(-12.4124700611279,37.3814053061226,21.2329761367735));
#49566=CARTESIAN_POINT('Ctrl Pts',(-12.3706686878054,37.4230969994869,21.2295541942591));
#49567=CARTESIAN_POINT('Ctrl Pts',(-12.3472410722571,37.4457981419276,21.2276780039746));
#49568=CARTESIAN_POINT('Ctrl Pts',(-12.2755071035913,37.5133274749273,21.2220534768247));
#49569=CARTESIAN_POINT('Ctrl Pts',(-12.226216491852,37.5570898480338,21.2183492704528));
#49570=CARTESIAN_POINT('Ctrl Pts',(-12.1071696258625,37.6567316170979,21.209738350357));
#49571=CARTESIAN_POINT('Ctrl Pts',(-12.0364173039599,37.7113451824053,21.204876513967));
#49572=CARTESIAN_POINT('Ctrl Pts',(-11.8490708954995,37.8444821088063,21.192514726961));
#49573=CARTESIAN_POINT('Ctrl Pts',(-11.7296049591917,37.9186656463085,21.185113627102));
#49574=CARTESIAN_POINT('Ctrl Pts',(-11.4575838212683,38.0649976550872,21.1687011831968));
#49575=CARTESIAN_POINT('Ctrl Pts',(-11.3035639542655,38.1336033100024,21.1596847172857));
#49576=CARTESIAN_POINT('Ctrl Pts',(-11.1180931056047,38.2001713284898,21.1484690616378));
#49577=CARTESIAN_POINT('Ctrl Pts',(-11.0909596614066,38.209522647731,21.146819427164));
#49578=CARTESIAN_POINT('Ctrl Pts',(-11.0479440506684,38.223739149603,21.1441855309555));
#49579=CARTESIAN_POINT('Ctrl Pts',(-11.0321386624572,38.2288342469343,21.1432138040647));
#49580=CARTESIAN_POINT('Ctrl Pts',(-11.0016831651396,38.2384055569475,21.1413326825629));
#49581=CARTESIAN_POINT('Ctrl Pts',(-10.9870391587164,38.2428989159647,21.1404242461049));
#49582=CARTESIAN_POINT('Ctrl Pts',(-10.9507887981037,38.2537536827921,21.1381665144));
#49583=CARTESIAN_POINT('Ctrl Pts',(-10.9291487169067,38.2599992283481,21.1368109541544));
#49584=CARTESIAN_POINT('Ctrl Pts',(-10.8455691681973,38.2832213618119,21.1315498158576));
#49585=CARTESIAN_POINT('Ctrl Pts',(-10.7832174746857,38.2986510930381,21.1275711614449));
#49586=CARTESIAN_POINT('Ctrl Pts',(-10.6099031652785,38.3363492778771,21.1164316171922));
#49587=CARTESIAN_POINT('Ctrl Pts',(-10.4982069549816,38.3548466145101,21.1091647365135));
#49588=CARTESIAN_POINT('Ctrl Pts',(-10.1276278474889,38.3972995616737,21.0851322998734));
#49589=CARTESIAN_POINT('Ctrl Pts',(-9.86686539711964,38.3970943769782,21.0684275607769));
#49590=CARTESIAN_POINT('Ctrl Pts',(-9.55889844332096,38.3613009783166,21.0495996918934));
#49591=CARTESIAN_POINT('Ctrl Pts',(-9.50926812009674,38.3544146245683,21.0465902282935));
#49592=CARTESIAN_POINT('Ctrl Pts',(-9.43065626371985,38.3417248028084,21.04186079421));
#49593=CARTESIAN_POINT('Ctrl Pts',(-9.40156798094662,38.3366384504322,21.0401189581931));
#49594=CARTESIAN_POINT('Ctrl Pts',(-9.34642145606504,38.3262511971017,21.0368312576107));
#49595=CARTESIAN_POINT('Ctrl Pts',(-9.3203520254786,38.321022527673,21.0352832722747));
#49596=CARTESIAN_POINT('Ctrl Pts',(-9.26059185481515,38.3083034365583,21.0317478201388));
#49597=CARTESIAN_POINT('Ctrl Pts',(-9.22694830050268,38.3006040701895,21.029767060457));
#49598=CARTESIAN_POINT('Ctrl Pts',(-9.11881703001145,38.2741139890942,21.0234270828467));
#49599=CARTESIAN_POINT('Ctrl Pts',(-9.04484631925979,38.2533042412468,21.0191310555369));
#49600=CARTESIAN_POINT('Ctrl Pts',(-8.86555302330443,38.1962213568535,21.0087623787634));
#49601=CARTESIAN_POINT('Ctrl Pts',(-8.76118760718904,38.1572372406447,21.0027666627582));
#49602=CARTESIAN_POINT('Ctrl Pts',(-8.45703801181351,38.0262179875849,20.9851062495034));
#49603=CARTESIAN_POINT('Ctrl Pts',(-8.26410524917939,37.9198257217929,20.9736757605094));
#49604=CARTESIAN_POINT('Ctrl Pts',(-8.03153522371403,37.7603301151047,20.9581149131681));
#49605=CARTESIAN_POINT('Ctrl Pts',(-7.98120728540772,37.7237384119442,20.9546267478011));
#49606=CARTESIAN_POINT('Ctrl Pts',(-7.91376695178496,37.671808662366,20.9497424166574));
#49607=CARTESIAN_POINT('Ctrl Pts',(-7.89575868129411,37.6576490119732,20.9484169032379));
#49608=CARTESIAN_POINT('Ctrl Pts',(-7.86601462959727,37.6337698546867,20.9461893013062));
#49609=CARTESIAN_POINT('Ctrl Pts',(-7.85419800871779,37.62415148478,20.945294066193));
#49610=CARTESIAN_POINT('Ctrl Pts',(-7.82978275251786,37.6040030252424,20.9434220423155));
#49611=CARTESIAN_POINT('Ctrl Pts',(-7.81719520779816,37.5934605975639,20.942444450851));
#49612=CARTESIAN_POINT('Ctrl Pts',(-7.7834828158011,37.5648062171452,20.9397936532997));
#49613=CARTESIAN_POINT('Ctrl Pts',(-7.76250402743272,37.5465252842937,20.9381091598229));
#49614=CARTESIAN_POINT('Ctrl Pts',(-7.63905645419594,37.4362498518559,20.9279992134172));
#49615=CARTESIAN_POINT('Ctrl Pts',(-7.54205407463878,37.3383461351494,20.9192368892726));
#49616=CARTESIAN_POINT('Ctrl Pts',(-7.26378710599566,37.0209953981113,20.8921162783271));
#49617=CARTESIAN_POINT('Ctrl Pts',(-7.10390926385604,36.784374998941,20.8736973182101));
#49618=CARTESIAN_POINT('Ctrl Pts',(-6.95198716001513,36.4841580751381,20.8532253379525));
#49619=CARTESIAN_POINT('Ctrl Pts',(-6.92958422965808,36.4372386403844,20.8500975192902));
#49620=CARTESIAN_POINT('Ctrl Pts',(-6.89588501118752,36.3622728857203,20.8452100005472));
#49621=CARTESIAN_POINT('Ctrl Pts',(-6.88387005089418,36.3345604173895,20.8434264313684));
#49622=CARTESIAN_POINT('Ctrl Pts',(-6.86304357668276,36.2847089074802,20.8402582346486));
#49623=CARTESIAN_POINT('Ctrl Pts',(-6.85409218511805,36.2626308414514,20.8388690243188));
#49624=CARTESIAN_POINT('Ctrl Pts',(-6.83363778395511,36.210613047384,20.8356275429106));
#49625=CARTESIAN_POINT('Ctrl Pts',(-6.82232535535287,36.1806005198627,20.8337816455484));
#49626=CARTESIAN_POINT('Ctrl Pts',(-6.79007856078249,36.0912246149537,20.8283528880154));
#49627=CARTESIAN_POINT('Ctrl Pts',(-6.77036920022641,36.0314322051005,20.8248095574175));
#49628=CARTESIAN_POINT('Ctrl Pts',(-6.70800966867564,35.8228871798355,20.812712914069));
#49629=CARTESIAN_POINT('Ctrl Pts',(-6.67388256622869,35.6717826933221,20.8044111253319));
#49630=CARTESIAN_POINT('Ctrl Pts',(-6.62072192194677,35.3285780473721,20.7859521737936));
#49631=CARTESIAN_POINT('Ctrl Pts',(-6.60751700831568,35.136136613001,20.7758747215507));
#49632=CARTESIAN_POINT('Ctrl Pts',(-6.61181674793735,34.8776111047162,20.7616435944293));
#49633=CARTESIAN_POINT('Ctrl Pts',(-6.61484342204103,34.8116423361436,20.7579495644333));
#49634=CARTESIAN_POINT('Ctrl Pts',(-6.62154953261965,34.7224653425152,20.7528218626585));
#49635=CARTESIAN_POINT('Ctrl Pts',(-6.62354664442012,34.6991416963975,20.7514682646804));
#49636=CARTESIAN_POINT('Ctrl Pts',(-6.62711932350132,34.6619531609368,20.7492874503246));
#49637=CARTESIAN_POINT('Ctrl Pts',(-6.62853925496047,34.6480736543568,20.7484684994737));
#49638=CARTESIAN_POINT('Ctrl Pts',(-6.63175583893251,34.6184403848103,20.7467085169525));
#49639=CARTESIAN_POINT('Ctrl Pts',(-6.63357741781179,34.6026897382002,20.745766101977));
#49640=CARTESIAN_POINT('Ctrl Pts',(-6.63858116388066,34.5619315464553,20.7433104000562));
#49641=CARTESIAN_POINT('Ctrl Pts',(-6.6419318659679,34.5369461297512,20.7417884103346));
#49642=CARTESIAN_POINT('Ctrl Pts',(-6.65865396292542,34.422000639533,20.7347169890567));
#49643=CARTESIAN_POINT('Ctrl Pts',(-6.67536293949245,34.3325703367701,20.7290193888631));
#49644=CARTESIAN_POINT('Ctrl Pts',(-6.74505854337428,34.0279711327977,20.7091653277677));
#49645=CARTESIAN_POINT('Ctrl Pts',(-6.81552330891013,33.8173758536015,20.6946985810215));
#49646=CARTESIAN_POINT('Ctrl Pts',(-6.960771753636,33.4928681796736,20.6721745097831));
#49647=CARTESIAN_POINT('Ctrl Pts',(-7.02271238128343,33.3739249693935,20.6638530143631));
#49648=CARTESIAN_POINT('Ctrl Pts',(-7.11335725474402,33.2225008438249,20.6532047237716));
#49649=CARTESIAN_POINT('Ctrl Pts',(-7.13585969464756,33.1864647381241,20.6506656764381));
#49650=CARTESIAN_POINT('Ctrl Pts',(-7.17428923733135,33.1274226957785,20.6464956784856));
#49651=CARTESIAN_POINT('Ctrl Pts',(-7.18983388803537,33.1041747001132,20.6448510683413));
#49652=CARTESIAN_POINT('Ctrl Pts',(-7.22108972324115,33.0586589123826,20.6416249091609));
#49653=CARTESIAN_POINT('Ctrl Pts',(-7.23678524282947,33.0363829767677,20.6400429445881));
#49654=CARTESIAN_POINT('Ctrl Pts',(-7.27545215822539,32.9828866450222,20.6362348821541));
#49655=CARTESIAN_POINT('Ctrl Pts',(-7.2986939950278,32.951865905135,20.6340192190981));
#49656=CARTESIAN_POINT('Ctrl Pts',(-7.38829184746641,32.8364592967501,20.6257390718982));
#49657=CARTESIAN_POINT('Ctrl Pts',(-7.4581140913868,32.7548392455734,20.6198087820014));
#49658=CARTESIAN_POINT('Ctrl Pts',(-7.66562670514252,32.5343786086058,20.6033703056137));
#49659=CARTESIAN_POINT('Ctrl Pts',(-7.81160649093395,32.4039409593276,20.593145506339));
#49660=CARTESIAN_POINT('Ctrl Pts',(-8.08489373022266,32.1992685009152,20.5749368864106));
#49661=CARTESIAN_POINT('Ctrl Pts',(-8.20729830180845,32.1193853493378,20.5670502833848));
#49662=CARTESIAN_POINT('Ctrl Pts',(-8.35909633188967,32.0337497459747,20.5571253165051));
#49663=CARTESIAN_POINT('Ctrl Pts',(-8.38390857876547,32.0201587584433,20.555498513415));
#49664=CARTESIAN_POINT('Ctrl Pts',(-8.42347326230401,31.9991265631009,20.552892784773));
#49665=CARTESIAN_POINT('Ctrl Pts',(-8.43811552169387,31.9914796343646,20.5519259460265));
#49666=CARTESIAN_POINT('Ctrl Pts',(-8.46648192394435,31.9769281536673,20.5500469685834));
#49667=CARTESIAN_POINT('Ctrl Pts',(-8.48019804154927,31.9700093976188,20.5491356886571));
#49668=CARTESIAN_POINT('Ctrl Pts',(-8.51435711778015,31.953068980097,20.5468602281064));
#49669=CARTESIAN_POINT('Ctrl Pts',(-8.53485474279792,31.9431596824384,20.545489565854));
#49670=CARTESIAN_POINT('Ctrl Pts',(-8.61536854905398,31.9052322009635,20.5400897409359));
#49671=CARTESIAN_POINT('Ctrl Pts',(-8.67609763291702,31.8787705415132,20.5359827085348));
#49672=CARTESIAN_POINT('Ctrl Pts',(-8.84804562636995,31.8097681132631,20.5243341378571));
#49673=CARTESIAN_POINT('Ctrl Pts',(-8.96078709549218,31.7712831686984,20.5166762908007));
#49674=CARTESIAN_POINT('Ctrl Pts',(-9.31488547436865,31.6708811573794,20.4929544557103));
#49675=CARTESIAN_POINT('Ctrl Pts',(-9.5612518294219,31.6295473465749,20.476977211535));
#49676=CARTESIAN_POINT('Ctrl Pts',(-9.86126606251305,31.6127002547486,20.4587111187294));
#49677=CARTESIAN_POINT('Ctrl Pts',(-9.91264263792916,31.6109860145143,20.4556212561396));
#49678=CARTESIAN_POINT('Ctrl Pts',(-9.9938332417984,31.6101246719796,20.4507964703319));
#49679=CARTESIAN_POINT('Ctrl Pts',(-10.0236295128718,31.6102014072492,20.4490381392533));
#49680=CARTESIAN_POINT('Ctrl Pts',(-10.0799514296053,31.6110891371298,20.445736744064));
#49681=CARTESIAN_POINT('Ctrl Pts',(-10.1064759378639,31.6118187768088,20.444191305581));
#49682=CARTESIAN_POINT('Ctrl Pts',(-10.1669916357057,31.6141948122974,20.4406854894196));
#49683=CARTESIAN_POINT('Ctrl Pts',(-10.2009723617675,31.6160417843793,20.4387314095428));
#49684=CARTESIAN_POINT('Ctrl Pts',(-10.3086552074759,31.623522533375,20.4325805174505));
#49685=CARTESIAN_POINT('Ctrl Pts',(-10.3822059413008,31.6310553852561,20.4284415074141));
#49686=CARTESIAN_POINT('Ctrl Pts',(-10.5597107176296,31.6551236244737,20.418554101261));
#49687=CARTESIAN_POINT('Ctrl Pts',(-10.6632556300735,31.6741064314767,20.4128728242203));
#49688=CARTESIAN_POINT('Ctrl Pts',(-10.8868065408144,31.7259473379431,20.4006108908022));
#49689=CARTESIAN_POINT('Ctrl Pts',(-11.0062228896755,31.7606540440783,20.3940639114528));
#49690=CARTESIAN_POINT('Ctrl Pts',(-11.2600069298808,31.8498044078353,20.3797477177074));
#49691=CARTESIAN_POINT('Ctrl Pts',(-11.3933258856956,31.9064607772689,20.3719694648174));
#49692=CARTESIAN_POINT('Ctrl Pts',(-11.5544680356929,31.9874751125343,20.3617858243671));
#49693=CARTESIAN_POINT('Ctrl Pts',(-11.586076725617,32.0039964150502,20.3597487195188));
#49694=CARTESIAN_POINT('Ctrl Pts',(-11.6332707830033,32.0296200537614,20.356638431783));
#49695=CARTESIAN_POINT('Ctrl Pts',(-11.6490546933376,32.0383536567832,20.3555864238806));
#49696=CARTESIAN_POINT('Ctrl Pts',(-11.6777844646556,32.0545513678361,20.3536485543875));
#49697=CARTESIAN_POINT('Ctrl Pts',(-11.6907517447967,32.0619756867108,20.3527651052668));
#49698=CARTESIAN_POINT('Ctrl Pts',(-11.72077859221,32.0794319470043,20.350699069882));
#49699=CARTESIAN_POINT('Ctrl Pts',(-11.7377998013694,32.0895277832822,20.3495126251859));
#49700=CARTESIAN_POINT('Ctrl Pts',(-11.7934809581228,32.1232166708795,20.3455834126762));
#49701=CARTESIAN_POINT('Ctrl Pts',(-11.8317550446842,32.1474346097968,20.3428057028407));
#49702=CARTESIAN_POINT('Ctrl Pts',(-11.9253085770032,32.2092898366946,20.3358450494066));
#49703=CARTESIAN_POINT('Ctrl Pts',(-11.9799805734388,32.2478095344636,20.3316248689289));
#49704=CARTESIAN_POINT('Ctrl Pts',(-12.2569543912757,32.4554800244865,20.3095721389797));
#49705=CARTESIAN_POINT('Ctrl Pts',(-12.4589041246991,32.650052979678,20.2912917732139));
#49706=CARTESIAN_POINT('Ctrl Pts',(-12.6859950186215,32.9305834338275,20.2689104909987));
#49707=CARTESIAN_POINT('Ctrl Pts',(-12.7349997054509,32.9957963060646,20.263932575384));
#49708=CARTESIAN_POINT('Ctrl Pts',(-12.8002843966378,33.0895340107787,20.2570834576977));
#49709=CARTESIAN_POINT('Ctrl Pts',(-12.8185726964726,33.116619776858,20.25513845529));
#49710=CARTESIAN_POINT('Ctrl Pts',(-12.851245136309,33.1665511471194,20.2516135245821));
#49711=CARTESIAN_POINT('Ctrl Pts',(-12.8657533698945,33.1893119514426,20.2500291264053));
#49712=CARTESIAN_POINT('Ctrl Pts',(-12.8946967509512,33.2359383426637,20.2468276930368));
#49713=CARTESIAN_POINT('Ctrl Pts',(-12.9091123117754,33.2598136777781,20.2452114493914));
#49714=CARTESIAN_POINT('Ctrl Pts',(-12.9445447384575,33.3201685938597,20.2411814734842));
#49715=CARTESIAN_POINT('Ctrl Pts',(-12.9651800502123,33.3568673941831,20.2387813403999));
#49716=CARTESIAN_POINT('Ctrl Pts',(-13.0525325701925,33.5192266685033,20.2283675269239));
#49717=CARTESIAN_POINT('Ctrl Pts',(-13.111987825755,33.6486368332558,20.2206030369261));
#49718=CARTESIAN_POINT('Ctrl Pts',(-13.2363893698021,33.9715509248681,20.2020406417496));
#49719=CARTESIAN_POINT('Ctrl Pts',(-13.2923435131101,34.1678987840244,20.1914318998722));
#49720=CARTESIAN_POINT('Ctrl Pts',(-13.3487488038878,34.465161910175,20.1750617541494));
#49721=CARTESIAN_POINT('Ctrl Pts',(-13.3629151548252,34.5630003003109,20.1696205142505));
#49722=CARTESIAN_POINT('Ctrl Pts',(-13.3754286230421,34.6876131109885,20.1624711018325));
#49723=CARTESIAN_POINT('Ctrl Pts',(-13.377762174746,34.7139465840842,20.1609479117543));
#49724=CARTESIAN_POINT('Ctrl Pts',(-13.3810224023721,34.7563764520376,20.158469985341));
#49725=CARTESIAN_POINT('Ctrl Pts',(-13.3821427003247,34.7724573671774,20.1575253854599));
#49726=CARTESIAN_POINT('Ctrl Pts',(-13.3840196626613,34.802487637254,20.1557501933554));
#49727=CARTESIAN_POINT('Ctrl Pts',(-13.3848048711002,34.816434825108,20.1549211865484));
#49728=CARTESIAN_POINT('Ctrl Pts',(-13.3862870526388,34.846019257766,20.1531536454526));
#49729=CARTESIAN_POINT('Ctrl Pts',(-13.3869619660537,34.8616573387686,20.1522139712181));
#49730=CARTESIAN_POINT('Ctrl Pts',(-13.3889969374834,34.9178389117,20.1488201544703));
#49731=CARTESIAN_POINT('Ctrl Pts',(-13.3897374160989,34.9583996272579,20.1463364607818));
#49732=CARTESIAN_POINT('Ctrl Pts',(-13.3897498409689,34.9989616594858,20.1438254858951));
#49733=CARTESIAN_POINT('Ctrl Pts',(-13.3897498397739,34.9989577654279,20.1438257269549));
#49734=CARTESIAN_POINT('Ctrl Pts',(-13.389815647109,35.212988665529,20.1305762467729));
#49735=CARTESIAN_POINT('Ctrl Pts',(-13.3696105698165,35.426542922744,20.1166329548135));
#49736=CARTESIAN_POINT('Ctrl Pts',(-13.2942105014199,35.8207824637724,20.0908445206738));
#49737=CARTESIAN_POINT('Ctrl Pts',(-13.2438204622287,36.0015675863871,20.0789970994992));
#49738=CARTESIAN_POINT('Ctrl Pts',(-13.1787500740781,36.1772650632072,20.0676095644498));
#49739=CARTESIAN_POINT('Ctrl Pts',(-13.1787500668679,36.1772650826756,20.4156323441327));
#49740=CARTESIAN_POINT('Ctrl Pts',(-13.1797425060653,36.1745853835903,20.4158108520197));
#49741=CARTESIAN_POINT('Ctrl Pts',(-13.1807315795116,36.1719043681469,20.4159892768759));
#49742=CARTESIAN_POINT('Ctrl Pts',(-13.2150217790527,36.0785929896502,20.4221933131743));
#49743=CARTESIAN_POINT('Ctrl Pts',(-13.2444410083631,35.9865764817198,20.4281141169251));
#49744=CARTESIAN_POINT('Ctrl Pts',(-13.2797552998974,35.8573274305439,20.4361577408318));
#49745=CARTESIAN_POINT('Ctrl Pts',(-13.2890192969764,35.8210708756514,20.4383851970052));
#49746=CARTESIAN_POINT('Ctrl Pts',(-13.3039345590445,35.7583872572105,20.442188056826));
#49747=CARTESIAN_POINT('Ctrl Pts',(-13.3098735122455,35.7320329215109,20.4437724006817));
#49748=CARTESIAN_POINT('Ctrl Pts',(-13.3213964926778,35.6778891089177,20.4469987021115));
#49749=CARTESIAN_POINT('Ctrl Pts',(-13.3269482994619,35.650094907814,20.4486395360157));
#49750=CARTESIAN_POINT('Ctrl Pts',(-13.3402905138677,35.5786454319229,20.4528201443975));
#49751=CARTESIAN_POINT('Ctrl Pts',(-13.3475742214937,35.5349003089246,20.4553440538966));
#49752=CARTESIAN_POINT('Ctrl Pts',(-13.3779360928064,35.3275096800624,20.4671587069783));
#49753=CARTESIAN_POINT('Ctrl Pts',(-13.3898865541809,35.1624564179043,20.4761051573321));
#49754=CARTESIAN_POINT('Ctrl Pts',(-13.3895661465026,34.7779583694554,20.496610089433));
#49755=CARTESIAN_POINT('Ctrl Pts',(-13.3681189643523,34.5592939174178,20.5080099220275));
#49756=CARTESIAN_POINT('Ctrl Pts',(-13.3135660143134,34.2826222305813,20.5235640353451));
#49757=CARTESIAN_POINT('Ctrl Pts',(-13.2997048073285,34.2213487326185,20.5270844963043));
#49758=CARTESIAN_POINT('Ctrl Pts',(-13.2784570013726,34.1382266811757,20.5320070886447));
#49759=CARTESIAN_POINT('Ctrl Pts',(-13.2725372796528,34.1160128654812,20.5333371291529));
#49760=CARTESIAN_POINT('Ctrl Pts',(-13.2623153214775,34.0791653746228,20.5355701438627));
#49761=CARTESIAN_POINT('Ctrl Pts',(-13.2581393070868,34.0644969739984,20.5364661906848));
#49762=CARTESIAN_POINT('Ctrl Pts',(-13.2492696500637,34.0341218917911,20.5383373894828));
#49763=CARTESIAN_POINT('Ctrl Pts',(-13.2445608562356,34.0184203525582,20.5393133146451));
#49764=CARTESIAN_POINT('Ctrl Pts',(-13.2315887840289,33.976278173755,20.5419548364519));
#49765=CARTESIAN_POINT('Ctrl Pts',(-13.2231151333839,33.9499042061093,20.5436315920241));
#49766=CARTESIAN_POINT('Ctrl Pts',(-13.1716750416938,33.7962896327822,20.553524437595));
#49767=CARTESIAN_POINT('Ctrl Pts',(-13.1215037817248,33.6715991700884,20.562061248656));
#49768=CARTESIAN_POINT('Ctrl Pts',(-12.9399346243912,33.2878556099403,20.589325940471));
#49769=CARTESIAN_POINT('Ctrl Pts',(-12.7825810086151,33.0424625581116,20.6081405644321));
#49770=CARTESIAN_POINT('Ctrl Pts',(-12.5628257386086,32.7807730967697,20.6289128143236));
#49771=CARTESIAN_POINT('Ctrl Pts',(-12.5289001868035,32.7421895358724,20.6320009565101));
#49772=CARTESIAN_POINT('Ctrl Pts',(-12.4739358009627,32.6824724206787,20.6368237023879));
#49773=CARTESIAN_POINT('Ctrl Pts',(-12.4534737785582,32.6608208852368,20.6385816805327));
#49774=CARTESIAN_POINT('Ctrl Pts',(-12.4142506512456,32.6203985808672,20.6418827742585));
#49775=CARTESIAN_POINT('Ctrl Pts',(-12.3955494715002,32.6015730343549,20.6434282588747));
#49776=CARTESIAN_POINT('Ctrl Pts',(-12.3523583605508,32.5591038974443,20.6469346693323));
#49777=CARTESIAN_POINT('Ctrl Pts',(-12.3277292768483,32.5356055158479,20.6488892890816));
#49778=CARTESIAN_POINT('Ctrl Pts',(-12.2484675891758,32.4622312552077,20.6550439668156));
#49779=CARTESIAN_POINT('Ctrl Pts',(-12.1925527628919,32.4137691199468,20.6591861171708));
#49780=CARTESIAN_POINT('Ctrl Pts',(-12.0532841989469,32.300829128104,20.6690830366963));
#49781=CARTESIAN_POINT('Ctrl Pts',(-11.9684232613417,32.2383317956253,20.6747705005376));
#49782=CARTESIAN_POINT('Ctrl Pts',(-11.7775198450321,32.1110148445428,20.6870309010475));
#49783=CARTESIAN_POINT('Ctrl Pts',(-11.670549371612,32.0478690963406,20.6935705798324));
#49784=CARTESIAN_POINT('Ctrl Pts',(-11.4319116761727,31.9241313661927,20.7078775084907));
#49785=CARTESIAN_POINT('Ctrl Pts',(-11.2993455873243,31.8658283131306,20.7156539419354));
#49786=CARTESIAN_POINT('Ctrl Pts',(-11.1299936393782,31.8039414663263,20.7258346380206));
#49787=CARTESIAN_POINT('Ctrl Pts',(-11.0963225879659,31.792235615245,20.7278707354697));
#49788=CARTESIAN_POINT('Ctrl Pts',(-11.045347826199,31.7754103720041,20.7309797901621));
#49789=CARTESIAN_POINT('Ctrl Pts',(-11.0281765984122,31.7698942436056,20.7320315974449));
#49790=CARTESIAN_POINT('Ctrl Pts',(-10.996699326441,31.7600588248876,20.7339692903609));
#49791=CARTESIAN_POINT('Ctrl Pts',(-10.9824075808536,31.7556967336545,20.7348527668899));
#49792=CARTESIAN_POINT('Ctrl Pts',(-10.9491168725208,31.7457759651913,20.7369191236008));
#49793=CARTESIAN_POINT('Ctrl Pts',(-10.9300976093357,31.7402890769505,20.7381058664843));
#49794=CARTESIAN_POINT('Ctrl Pts',(-10.8673803913281,31.7227892767996,20.7420371358552));
#49795=CARTESIAN_POINT('Ctrl Pts',(-10.8234912005484,31.7114865533703,20.7448166523558));
#49796=CARTESIAN_POINT('Ctrl Pts',(-10.7142567059567,31.6856793011802,20.7517829456565));
#49797=CARTESIAN_POINT('Ctrl Pts',(-10.6486841291773,31.6722241161883,20.756007030276));
#49798=CARTESIAN_POINT('Ctrl Pts',(-10.306785163656,31.6125570765483,20.7781167424471));
#49799=CARTESIAN_POINT('Ctrl Pts',(-10.0258548807651,31.5987863553112,20.7964512385192));
#49800=CARTESIAN_POINT('Ctrl Pts',(-9.66575819337621,31.6257990533152,20.8188361769607));
#49801=CARTESIAN_POINT('Ctrl Pts',(-9.58532443139292,31.6347369463962,20.8237735179649));
#49802=CARTESIAN_POINT('Ctrl Pts',(-9.47305112889551,31.6513000427277,20.8305772292584));
#49803=CARTESIAN_POINT('Ctrl Pts',(-9.44088943014509,31.6565194783803,20.8325161164076));
#49804=CARTESIAN_POINT('Ctrl Pts',(-9.38225464696641,31.6669049079264,20.8360334522105));
#49805=CARTESIAN_POINT('Ctrl Pts',(-9.35575869732726,31.6719246672362,20.8376163014039));
#49806=CARTESIAN_POINT('Ctrl Pts',(-9.30195502547475,31.6827846158784,20.8408180503895));
#49807=CARTESIAN_POINT('Ctrl Pts',(-9.27465389840548,31.6886471356912,20.8424361151924));
#49808=CARTESIAN_POINT('Ctrl Pts',(-9.20621603358119,31.7042302060499,20.8464774005731));
#49809=CARTESIAN_POINT('Ctrl Pts',(-9.16518226108181,31.7143842150928,20.848886855502));
#49810=CARTESIAN_POINT('Ctrl Pts',(-8.98474201328525,31.762633844568,20.8594352965703));
#49811=CARTESIAN_POINT('Ctrl Pts',(-8.84765884685266,31.808855319541,20.8673163995646));
#49812=CARTESIAN_POINT('Ctrl Pts',(-8.59151044541241,31.9138908563147,20.8821575270251));
#49813=CARTESIAN_POINT('Ctrl Pts',(-8.47213069762243,31.9712166995524,20.8891280360757));
#49814=CARTESIAN_POINT('Ctrl Pts',(-8.22435600619584,32.108583239846,20.904191122184));
#49815=CARTESIAN_POINT('Ctrl Pts',(-8.09735488610336,32.1905275547102,20.9122867878498));
#49816=CARTESIAN_POINT('Ctrl Pts',(-7.94737604290737,32.3021424236888,20.922839006702));
#49817=CARTESIAN_POINT('Ctrl Pts',(-7.91884622173413,32.324089062384,20.9248943191478));
#49818=CARTESIAN_POINT('Ctrl Pts',(-7.87650097398503,32.3577500714075,20.9280268777391));
#49819=CARTESIAN_POINT('Ctrl Pts',(-7.8624202848406,32.3691283330538,20.9290824939516));
#49820=CARTESIAN_POINT('Ctrl Pts',(-7.8368896505127,32.3900992772204,20.9310235583407));
#49821=CARTESIAN_POINT('Ctrl Pts',(-7.82541100869835,32.3996556266936,20.9319065336308));
#49822=CARTESIAN_POINT('Ctrl Pts',(-7.79893616242646,32.4219947026402,20.9339668693319));
#49823=CARTESIAN_POINT('Ctrl Pts',(-7.78398791222559,32.4348326144344,20.935148012226));
#49824=CARTESIAN_POINT('Ctrl Pts',(-7.73543558904368,32.4772716093215,20.9390407552629));
#49825=CARTESIAN_POINT('Ctrl Pts',(-7.70230735446399,32.5074072528284,20.9417864512292));
#49826=CARTESIAN_POINT('Ctrl Pts',(-7.62199190422747,32.5834293511702,20.9486474289154));
#49827=CARTESIAN_POINT('Ctrl Pts',(-7.57552621564693,32.6300501686825,20.9527987036615));
#49828=CARTESIAN_POINT('Ctrl Pts',(-7.34854216910096,32.8714569250744,20.9738968739488));
#49829=CARTESIAN_POINT('Ctrl Pts',(-7.18997344677847,33.0856589319398,20.9912726918922));
#49830=CARTESIAN_POINT('Ctrl Pts',(-7.01179353570882,33.3969735796828,21.0136402124513));
#49831=CARTESIAN_POINT('Ctrl Pts',(-6.96889511597271,33.4796456953558,21.0193472387506));
#49832=CARTESIAN_POINT('Ctrl Pts',(-6.91339543848853,33.5983174965646,21.0272161549342));
#49833=CARTESIAN_POINT('Ctrl Pts',(-6.89791568122033,33.6329174810132,21.0294733407504));
#49834=CARTESIAN_POINT('Ctrl Pts',(-6.87247524486415,33.6924397935413,21.0332949632924));
#49835=CARTESIAN_POINT('Ctrl Pts',(-6.86222452049364,33.71723350163,21.0348689683744));
#49836=CARTESIAN_POINT('Ctrl Pts',(-6.84182957145973,33.7682711069477,21.0380735674958));
#49837=CARTESIAN_POINT('Ctrl Pts',(-6.83171555580551,33.7945248771616,21.039703064246));
#49838=CARTESIAN_POINT('Ctrl Pts',(-6.80686219933836,33.8615131432614,21.0438147284361));
#49839=CARTESIAN_POINT('Ctrl Pts',(-6.79257443114171,33.9024104607707,21.0462820811328));
#49840=CARTESIAN_POINT('Ctrl Pts',(-6.72912246092845,34.0958680872891,21.0577690469058));
#49841=CARTESIAN_POINT('Ctrl Pts',(-6.69003258528172,34.2515230287149,21.0664650471424));
#49842=CARTESIAN_POINT('Ctrl Pts',(-6.62808213176658,34.6016333246794,21.0854512244782));
#49843=CARTESIAN_POINT('Ctrl Pts',(-6.61073871748351,34.7964625318229,21.095635732872));
#49844=CARTESIAN_POINT('Ctrl Pts',(-6.61004403236768,35.0798746583062,21.1110424746374));
#49845=CARTESIAN_POINT('Ctrl Pts',(-6.61326910226161,35.1680262790533,21.1159213023215));
#49846=CARTESIAN_POINT('Ctrl Pts',(-6.62186746255237,35.2815785732353,21.1224286776713));
#49847=CARTESIAN_POINT('Ctrl Pts',(-6.62409999441359,35.3071888683805,21.1239110626468));
#49848=CARTESIAN_POINT('Ctrl Pts',(-6.62819059256733,35.3486562737177,21.1263387175266));
#49849=CARTESIAN_POINT('Ctrl Pts',(-6.62986982515734,35.3645304639123,21.1272745824342));
#49850=CARTESIAN_POINT('Ctrl Pts',(-6.63342828175083,35.3960403082881,21.1291462701152));
#49851=CARTESIAN_POINT('Ctrl Pts',(-6.63530446779698,35.4116758548307,21.1300819190504));
#49852=CARTESIAN_POINT('Ctrl Pts',(-6.6404032897058,35.4518021558286,21.132499866595));
#49853=CARTESIAN_POINT('Ctrl Pts',(-6.64378476590792,35.4762714232378,21.1339903971671));
#49854=CARTESIAN_POINT('Ctrl Pts',(-6.65998278926792,35.5847293276504,21.1406619454116));
#49855=CARTESIAN_POINT('Ctrl Pts',(-6.67568611000042,35.6682501579278,21.1459721910308));
#49856=CARTESIAN_POINT('Ctrl Pts',(-6.73647559923416,35.9357816445134,21.1633658340175));
#49857=CARTESIAN_POINT('Ctrl Pts',(-6.79384818005745,36.1166333244834,21.1756994660848));
#49858=CARTESIAN_POINT('Ctrl Pts',(-6.93043900063315,36.4480233758005,21.1986138881485));
#49859=CARTESIAN_POINT('Ctrl Pts',(-7.00645753782626,36.5992789627376,21.2092111198128));
#49860=CARTESIAN_POINT('Ctrl Pts',(-7.11632520716456,36.7823580349376,21.2221167445271));
#49861=CARTESIAN_POINT('Ctrl Pts',(-7.13994346702926,36.8200157650581,21.2247770012469));
#49862=CARTESIAN_POINT('Ctrl Pts',(-7.17983596922893,36.8809264604542,21.2290911223918));
#49863=CARTESIAN_POINT('Ctrl Pts',(-7.19567308560185,36.9044579649717,21.2307606300248));
#49864=CARTESIAN_POINT('Ctrl Pts',(-7.22716059674186,36.9499989318475,21.233998247697));
#49865=CARTESIAN_POINT('Ctrl Pts',(-7.24278229734094,36.9720255557289,21.2355672601181));
#49866=CARTESIAN_POINT('Ctrl Pts',(-7.28063547956017,37.0240693456179,21.2392832881431));
#49867=CARTESIAN_POINT('Ctrl Pts',(-7.30310341070712,37.0539106733541,21.2414211354459));
#49868=CARTESIAN_POINT('Ctrl Pts',(-7.3850914081183,37.159139396174,21.2489926650137));
#49869=CARTESIAN_POINT('Ctrl Pts',(-7.44731851084905,37.2323640575236,21.2543215322003));
#49870=CARTESIAN_POINT('Ctrl Pts',(-7.62047122176675,37.4193948861021,21.2682290237367));
#49871=CARTESIAN_POINT('Ctrl Pts',(-7.73642765146448,37.5282152295015,21.2766310950034));
#49872=CARTESIAN_POINT('Ctrl Pts',(-8.00343276518211,37.7456393773768,21.2948886017388));
#49873=CARTESIAN_POINT('Ctrl Pts',(-8.15663440121449,37.8507551754478,21.3047209487584));
#49874=CARTESIAN_POINT('Ctrl Pts',(-8.34779037152248,37.9600361858194,21.3171602556404));
#49875=CARTESIAN_POINT('Ctrl Pts',(-8.37819848513812,37.9768054234377,21.3191442489981));
#49876=CARTESIAN_POINT('Ctrl Pts',(-8.42481328278357,38.0015859805632,21.3222016483387));
#49877=CARTESIAN_POINT('Ctrl Pts',(-8.44083616375052,38.0099401476889,21.3232553930993));
#49878=CARTESIAN_POINT('Ctrl Pts',(-8.47022682634529,38.0249664955053,21.3251947955204));
#49879=CARTESIAN_POINT('Ctrl Pts',(-8.48357300990874,38.0316789769413,21.3260780115949));
#49880=CARTESIAN_POINT('Ctrl Pts',(-8.51466427973469,38.0470597091706,21.3281412813292));
#49881=CARTESIAN_POINT('Ctrl Pts',(-8.53244115773614,38.0556613156932,21.3293251566281));
#49882=CARTESIAN_POINT('Ctrl Pts',(-8.59100797757151,38.0833707946534,21.3332366609151));
#49883=CARTESIAN_POINT('Ctrl Pts',(-8.63210215704156,38.1018202806324,21.335998819727));
#49884=CARTESIAN_POINT('Ctrl Pts',(-8.73461192320585,38.1454094918872,21.3429109901449));
#49885=CARTESIAN_POINT('Ctrl Pts',(-8.7964205866403,38.1695746663377,21.3470976310758));
#49886=CARTESIAN_POINT('Ctrl Pts',(-9.11543363832712,38.2836215597325,21.368674145764));
#49887=CARTESIAN_POINT('Ctrl Pts',(-9.38213575284987,38.3440847577589,21.3865026970966));
#49888=CARTESIAN_POINT('Ctrl Pts',(-9.74023510837264,38.3809143995264,21.4088888187047));
#49889=CARTESIAN_POINT('Ctrl Pts',(-9.827587495936,38.3864931647787,21.4142409768036));
#49890=CARTESIAN_POINT('Ctrl Pts',(-9.95205552033723,38.3896129003117,21.4217121324108));
#49891=CARTESIAN_POINT('Ctrl Pts',(-9.98906068059602,38.3899343328772,21.4239140865079));
#49892=CARTESIAN_POINT('Ctrl Pts',(-10.0530088835909,38.3894426011005,21.4276873534833));
#49893=CARTESIAN_POINT('Ctrl Pts',(-10.0799500732001,38.3889141529525,21.4292672418271));
#49894=CARTESIAN_POINT('Ctrl Pts',(-10.1353445886381,38.387166631661,21.4324965665023));
#49895=CARTESIAN_POINT('Ctrl Pts',(-10.1637946459336,38.3859101190277,21.4341447244349));
#49896=CARTESIAN_POINT('Ctrl Pts',(-10.2371523686184,38.3817434400452,21.4383695440258));
#49897=CARTESIAN_POINT('Ctrl Pts',(-10.2820247112337,38.3782972440925,21.4409296549925));
#49898=CARTESIAN_POINT('Ctrl Pts',(-10.5256891312304,38.354694821158,21.4547205458477));
#49899=CARTESIAN_POINT('Ctrl Pts',(-10.7224763350515,38.3178857516672,21.4654249146074));
#49900=CARTESIAN_POINT('Ctrl Pts',(-11.1225155014591,38.2057539380884,21.4874766703825));
#49901=CARTESIAN_POINT('Ctrl Pts',(-11.3240902377039,38.1278850788692,21.4987635220807));
#49902=CARTESIAN_POINT('Ctrl Pts',(-11.5530583861937,38.0133123274318,21.5131507330899));
#49903=CARTESIAN_POINT('Ctrl Pts',(-11.5889067402504,37.9945645101524,21.5154526623596));
#49904=CARTESIAN_POINT('Ctrl Pts',(-11.6410367674659,37.9661022029266,21.518885668097));
#49905=CARTESIAN_POINT('Ctrl Pts',(-11.6575873778843,37.9568848470562,21.519988513745));
#49906=CARTESIAN_POINT('Ctrl Pts',(-11.6870198376183,37.9401685810241,21.5219744707776));
#49907=CARTESIAN_POINT('Ctrl Pts',(-11.6999307728334,37.9327227224269,21.5228543382273));
#49908=CARTESIAN_POINT('Ctrl Pts',(-11.7289774575403,37.9157149688938,21.5248537058461));
#49909=CARTESIAN_POINT('Ctrl Pts',(-11.7450831514072,37.9061041941658,21.5259761376055));
#49910=CARTESIAN_POINT('Ctrl Pts',(-11.7947931052927,37.8758784714215,21.5294816164314));
#49911=CARTESIAN_POINT('Ctrl Pts',(-11.8281169645073,37.8548112635178,21.5318904087556));
#49912=CARTESIAN_POINT('Ctrl Pts',(-11.9071561586478,37.8028916520861,21.5377324749079));
#49913=CARTESIAN_POINT('Ctrl Pts',(-11.9525002551562,37.7714956984792,21.5411901997962));
#49914=CARTESIAN_POINT('Ctrl Pts',(-12.136514583697,37.6373278664343,21.5556071252993));
#49915=CARTESIAN_POINT('Ctrl Pts',(-12.268001015821,37.5251461274097,21.5668228749371));
#49916=CARTESIAN_POINT('Ctrl Pts',(-12.5240270088587,37.2705124309373,21.5899908266797));
#49917=CARTESIAN_POINT('Ctrl Pts',(-12.6463770424732,37.1266512374872,21.6018687630537));
#49918=CARTESIAN_POINT('Ctrl Pts',(-12.7825202299871,36.9365018174192,21.6160149011046));
#49919=CARTESIAN_POINT('Ctrl Pts',(-12.808157399601,36.8991341279968,21.6187285328247));
#49920=CARTESIAN_POINT('Ctrl Pts',(-12.8487096072503,36.8374093653372,21.6231061785001));
#49921=CARTESIAN_POINT('Ctrl Pts',(-12.86407905636,36.8133589924949,21.6247867373711));
#49922=CARTESIAN_POINT('Ctrl Pts',(-12.8933487524465,36.7662566186755,21.628030633002));
#49923=CARTESIAN_POINT('Ctrl Pts',(-12.9072817377776,36.7432275826075,21.6295950738596));
#49924=CARTESIAN_POINT('Ctrl Pts',(-12.9396201242865,36.6883109745446,21.6332764619072));
#49925=CARTESIAN_POINT('Ctrl Pts',(-12.9577834163658,36.6562843457432,21.6353847132555));
#49926=CARTESIAN_POINT('Ctrl Pts',(-13.0195448673777,36.5431254308602,21.6427062204683));
#49927=CARTESIAN_POINT('Ctrl Pts',(-13.0603570280963,36.4605150202644,21.6478240567444));
#49928=CARTESIAN_POINT('Ctrl Pts',(-13.1268588912888,36.3108378906477,21.6567778185595));
#49929=CARTESIAN_POINT('Ctrl Pts',(-13.1538692920563,36.2444460084989,21.6606432273797));
#49930=CARTESIAN_POINT('Ctrl Pts',(-13.1787500358286,36.1772651664852,21.6644776847947));
#49931=CARTESIAN_POINT('Origin',(-10.,35.,23.));
#49932=CARTESIAN_POINT('',(-13.1787500671534,36.1772650819049,22.9104832616759));
#49933=CARTESIAN_POINT('',(-13.1787500907405,36.1772650182168,22.5700365663484));
#49934=CARTESIAN_POINT('',(-13.1787500671536,36.1772650819043,23.));
#49935=CARTESIAN_POINT('Ctrl Pts',(-13.1787500907405,36.1772650182168,22.5700365663484));
#49936=CARTESIAN_POINT('Ctrl Pts',(-13.1240748334016,36.3248944614926,22.5616683248361));
#49937=CARTESIAN_POINT('Ctrl Pts',(-13.0591692600091,36.4685690213728,22.5533981955439));
#49938=CARTESIAN_POINT('Ctrl Pts',(-12.953278579165,36.6651978966316,22.5413012604624));
#49939=CARTESIAN_POINT('Ctrl Pts',(-12.9203862141367,36.722231662174,22.5376917011256));
#49940=CARTESIAN_POINT('Ctrl Pts',(-12.862359117909,36.8164006997973,22.5315008009975));
#49941=CARTESIAN_POINT('Ctrl Pts',(-12.8381097881809,36.854061395087,22.5289600288544));
#49942=CARTESIAN_POINT('Ctrl Pts',(-12.8021282474947,36.9075824146467,22.5252382085787));
#49943=CARTESIAN_POINT('Ctrl Pts',(-12.7909917220288,36.9238395336274,22.5240925693446));
#49944=CARTESIAN_POINT('Ctrl Pts',(-12.7711659513161,36.9522467660789,22.522062233656));
#49945=CARTESIAN_POINT('Ctrl Pts',(-12.7625371644089,36.9644379776868,22.5211814602275));
#49946=CARTESIAN_POINT('Ctrl Pts',(-12.7432722266394,36.9912785471148,22.5192209971691));
#49947=CARTESIAN_POINT('Ctrl Pts',(-12.7325992555222,37.0058998075448,22.5181389779323));
#49948=CARTESIAN_POINT('Ctrl Pts',(-12.7003592927021,37.049331579848,22.5148843473055));
#49949=CARTESIAN_POINT('Ctrl Pts',(-12.6784506995931,37.0778839863913,22.512690789305));
#49950=CARTESIAN_POINT('Ctrl Pts',(-12.5622988252026,37.2243694035762,22.501176388498));
#49951=CARTESIAN_POINT('Ctrl Pts',(-12.4607148884698,37.3362511881488,22.4914956445948));
#49952=CARTESIAN_POINT('Ctrl Pts',(-12.2567899647403,37.5327443441236,22.4732517459289));
#49953=CARTESIAN_POINT('Ctrl Pts',(-12.1562644065705,37.6188587491143,22.4647131265315));
#49954=CARTESIAN_POINT('Ctrl Pts',(-11.9358421855869,37.7863642726116,22.447127787365));
#49955=CARTESIAN_POINT('Ctrl Pts',(-11.815233037322,37.8663999118682,22.438127609866));
#49956=CARTESIAN_POINT('Ctrl Pts',(-11.6532220051078,37.9595690612221,22.4268534458134));
#49957=CARTESIAN_POINT('Ctrl Pts',(-11.6161847975068,37.9799562025201,22.4243271679779));
#49958=CARTESIAN_POINT('Ctrl Pts',(-11.5540650684416,38.0126510786662,22.4201723334279));
#49959=CARTESIAN_POINT('Ctrl Pts',(-11.5291952260054,38.0253506886248,22.4185303210996));
#49960=CARTESIAN_POINT('Ctrl Pts',(-11.4800059931705,38.0497072693643,22.415323439542));
#49961=CARTESIAN_POINT('Ctrl Pts',(-11.4556988504484,38.0613841782599,22.4137579747704));
#49962=CARTESIAN_POINT('Ctrl Pts',(-11.4017242153313,38.0865248280804,22.4103227341902));
#49963=CARTESIAN_POINT('Ctrl Pts',(-11.3719965608593,38.0998535177034,22.408457601695));
#49964=CARTESIAN_POINT('Ctrl Pts',(-11.2678131543279,38.1447727838095,22.4020095182351));
#49965=CARTESIAN_POINT('Ctrl Pts',(-11.1924201109888,38.1741269200825,22.3974996356972));
#49966=CARTESIAN_POINT('Ctrl Pts',(-10.8514430469606,38.2930193095256,22.3776650327892));
#49967=CARTESIAN_POINT('Ctrl Pts',(-10.576441979743,38.3521092583466,22.3632575660505));
#49968=CARTESIAN_POINT('Ctrl Pts',(-10.2306418796184,38.3825565690339,22.3444676418831));
#49969=CARTESIAN_POINT('Ctrl Pts',(-10.1638143312928,38.386450735793,22.3408003520829));
#49970=CARTESIAN_POINT('Ctrl Pts',(-10.051617552822,38.3896599509054,22.3345210897479));
#49971=CARTESIAN_POINT('Ctrl Pts',(-10.0062969927845,38.3900470341661,22.3319512098715));
#49972=CARTESIAN_POINT('Ctrl Pts',(-9.94119071108923,38.3892976234969,22.3281943332827));
#49973=CARTESIAN_POINT('Ctrl Pts',(-9.92139969834953,38.388896408077,22.3270436734235));
#49974=CARTESIAN_POINT('Ctrl Pts',(-9.88667697117286,38.3878881699818,22.3250079580833));
#49975=CARTESIAN_POINT('Ctrl Pts',(-9.87174398862509,38.3873557157185,22.3241269046615));
#49976=CARTESIAN_POINT('Ctrl Pts',(-9.83879511612483,38.3859626885178,22.3221702433607));
#49977=CARTESIAN_POINT('Ctrl Pts',(-9.82078249799305,38.385057074477,22.3210923686942));
#49978=CARTESIAN_POINT('Ctrl Pts',(-9.76719231671656,38.3819338132044,22.3178628266232));
#49979=CARTESIAN_POINT('Ctrl Pts',(-9.73164263613224,38.3792987205387,22.315690666583));
#49980=CARTESIAN_POINT('Ctrl Pts',(-9.52762696058861,38.3609368272521,22.3030781511606));
#49981=CARTESIAN_POINT('Ctrl Pts',(-9.36049586365792,38.3331754301121,22.2921819110593));
#49982=CARTESIAN_POINT('Ctrl Pts',(-9.03469859496188,38.2536468917318,22.2705642625866));
#49983=CARTESIAN_POINT('Ctrl Pts',(-8.87635205915459,38.2024128624622,22.2598737825077));
#49984=CARTESIAN_POINT('Ctrl Pts',(-8.65816652165064,38.1136307064377,22.245136206382));
#49985=CARTESIAN_POINT('Ctrl Pts',(-8.59475315223077,38.0855300236096,22.2408496240776));
#49986=CARTESIAN_POINT('Ctrl Pts',(-8.48292021989554,38.0318093784302,22.2332891459944));
#49987=CARTESIAN_POINT('Ctrl Pts',(-8.4341762795063,38.0069246355187,22.2299933809457));
#49988=CARTESIAN_POINT('Ctrl Pts',(-8.35926028906029,37.966362523062,22.2249251786272));
#49989=CARTESIAN_POINT('Ctrl Pts',(-8.33266280069066,37.9514945657911,22.2231251927658));
#49990=CARTESIAN_POINT('Ctrl Pts',(-8.28336520002296,37.9230581828056,22.2197867477784));
#49991=CARTESIAN_POINT('Ctrl Pts',(-8.26061657955208,37.9095789303039,22.2182452969182));
#49992=CARTESIAN_POINT('Ctrl Pts',(-8.20984725963833,37.8786883038778,22.2148019413831));
#49993=CARTESIAN_POINT('Ctrl Pts',(-8.18191811509319,37.8611311668697,22.2129054537828));
#49994=CARTESIAN_POINT('Ctrl Pts',(-8.09727621906227,37.8061826628612,22.2071471304879));
#49995=CARTESIAN_POINT('Ctrl Pts',(-8.04142568974309,37.767491002517,22.2033327186608));
#49996=CARTESIAN_POINT('Ctrl Pts',(-7.78494965597834,37.5781558283928,22.1856728776683));
#49997=CARTESIAN_POINT('Ctrl Pts',(-7.60029304008272,37.4072280026226,22.1726005173881));
#49998=CARTESIAN_POINT('Ctrl Pts',(-7.37136608705129,37.1425465210397,22.1539345267788));
#49999=CARTESIAN_POINT('Ctrl Pts',(-7.30987100487107,37.0648064418633,22.1486010838034));
#50000=CARTESIAN_POINT('Ctrl Pts',(-7.22811837760224,36.9515951551464,22.1408731518037));
#50001=CARTESIAN_POINT('Ctrl Pts',(-7.20495776541068,36.9182778810178,22.1386032305441));
#50002=CARTESIAN_POINT('Ctrl Pts',(-7.16496794475606,36.8584890737967,22.1345224653878));
#50003=CARTESIAN_POINT('Ctrl Pts',(-7.14789738789962,36.8321841976466,22.1327246341959));
#50004=CARTESIAN_POINT('Ctrl Pts',(-7.1220499668426,36.7911179193518,22.1299080658624));
#50005=CARTESIAN_POINT('Ctrl Pts',(-7.11301579520889,36.7765196221734,22.1289049352438));
#50006=CARTESIAN_POINT('Ctrl Pts',(-7.09624203462262,36.748949086996,22.1270056462231));
#50007=CARTESIAN_POINT('Ctrl Pts',(-7.08847770369093,36.7359928326479,22.1261110472179));
#50008=CARTESIAN_POINT('Ctrl Pts',(-7.07001483287942,36.7047117752317,22.1239467244453));
#50009=CARTESIAN_POINT('Ctrl Pts',(-7.05940139866072,36.6863377868322,22.1226718851205));
#50010=CARTESIAN_POINT('Ctrl Pts',(-7.02428562987325,36.6242057010499,22.118352224853));
#50011=CARTESIAN_POINT('Ctrl Pts',(-7.00058306537671,36.5800055927959,22.1152648488027));
#50012=CARTESIAN_POINT('Ctrl Pts',(-6.88474934629017,36.3519949274575,22.099325458337));
#50013=CARTESIAN_POINT('Ctrl Pts',(-6.80850146248942,36.1606070220361,22.0859336384872));
#50014=CARTESIAN_POINT('Ctrl Pts',(-6.70408338379959,35.8083990017249,22.062346420005));
#50015=CARTESIAN_POINT('Ctrl Pts',(-6.66925905913548,35.6501926389613,22.0521019447303));
#50016=CARTESIAN_POINT('Ctrl Pts',(-6.63669862728671,35.4273510782366,22.0382965542551));
#50017=CARTESIAN_POINT('Ctrl Pts',(-6.62929335743372,35.3643660270074,22.0344606193522));
#50018=CARTESIAN_POINT('Ctrl Pts',(-6.620801378988,35.2691762886354,22.0287603734784));
#50019=CARTESIAN_POINT('Ctrl Pts',(-6.61839976213907,35.2371057417626,22.0268563351426));
#50020=CARTESIAN_POINT('Ctrl Pts',(-6.61501361606447,35.1812184367081,22.0235657910832));
#50021=CARTESIAN_POINT('Ctrl Pts',(-6.61382326067023,35.1574168803638,22.0221730578377));
#50022=CARTESIAN_POINT('Ctrl Pts',(-6.61169611075612,35.103489693268,22.0190363317463));
#50023=CARTESIAN_POINT('Ctrl Pts',(-6.61090989077505,35.0733599246977,22.0172970754516));
#50024=CARTESIAN_POINT('Ctrl Pts',(-6.60986657974326,34.9915451606357,22.0126077806275));
#50025=CARTESIAN_POINT('Ctrl Pts',(-6.61038950006398,34.9398572932841,22.009681622323));
#50026=CARTESIAN_POINT('Ctrl Pts',(-6.62000305866061,34.6485360722685,21.9933597521017));
#50027=CARTESIAN_POINT('Ctrl Pts',(-6.65331888001949,34.410387545852,21.9807292090286));
#50028=CARTESIAN_POINT('Ctrl Pts',(-6.75543340137381,34.0019990613022,21.9583899477608));
#50029=CARTESIAN_POINT('Ctrl Pts',(-6.81338542707709,33.8300893896225,21.9487366449005));
#50030=CARTESIAN_POINT('Ctrl Pts',(-6.89610746265219,33.6372522247897,21.9367942635273));
#50031=CARTESIAN_POINT('Ctrl Pts',(-6.90776787490348,33.6109964899008,21.9351430178509));
#50032=CARTESIAN_POINT('Ctrl Pts',(-6.92669539641054,33.5697972673561,21.9325071339685));
#50033=CARTESIAN_POINT('Ctrl Pts',(-6.93374134454911,33.5547530053815,21.9315350624761));
#50034=CARTESIAN_POINT('Ctrl Pts',(-6.94741911519368,33.5260989854699,21.9296641597028));
#50035=CARTESIAN_POINT('Ctrl Pts',(-6.95403197758398,33.5124809137856,21.928766426658));
#50036=CARTESIAN_POINT('Ctrl Pts',(-6.97063926822555,33.478856094825,21.9265292187996));
#50037=CARTESIAN_POINT('Ctrl Pts',(-6.98074081353265,33.4589032705041,21.9251835109177));
#50038=CARTESIAN_POINT('Ctrl Pts',(-7.01790422861383,33.3872651962381,21.9202899813154));
#50039=CARTESIAN_POINT('Ctrl Pts',(-7.0461006201939,33.3361831949844,21.9166833221699));
#50040=CARTESIAN_POINT('Ctrl Pts',(-7.1761218337607,33.1143614177892,21.9005780598949));
#50041=CARTESIAN_POINT('Ctrl Pts',(-7.29153158692936,32.952045916123,21.8876329515913));
#50042=CARTESIAN_POINT('Ctrl Pts',(-7.44846752083327,32.7679726580888,21.8721105511825));
#50043=CARTESIAN_POINT('Ctrl Pts',(-7.47706437847027,32.735698778186,21.8693527459737));
#50044=CARTESIAN_POINT('Ctrl Pts',(-7.57490202988622,32.6294363836983,21.8601597966048));
#50045=CARTESIAN_POINT('Ctrl Pts',(-7.6468462254978,32.5580045040303,21.8537928138538));
#50046=CARTESIAN_POINT('Ctrl Pts',(-7.77521704371321,32.4414979959072,21.8431098197026));
#50047=CARTESIAN_POINT('Ctrl Pts',(-7.83007809760845,32.3948067609101,21.8387355263668));
#50048=CARTESIAN_POINT('Ctrl Pts',(-7.9127393274734,32.3288796334042,21.8324157722934));
#50049=CARTESIAN_POINT('Ctrl Pts',(-7.93940298999155,32.3082568448392,21.8304165424675));
#50050=CARTESIAN_POINT('Ctrl Pts',(-7.98757233747021,32.2721359549518,21.8268730029141));
#50051=CARTESIAN_POINT('Ctrl Pts',(-8.00896026393256,32.2564861630127,21.8253229367178));
#50052=CARTESIAN_POINT('Ctrl Pts',(-8.05493692332513,32.2236653744321,21.8220390784082));
#50053=CARTESIAN_POINT('Ctrl Pts',(-8.07957453643129,32.2065665485705,21.8203080919864));
#50054=CARTESIAN_POINT('Ctrl Pts',(-8.1467024904504,32.1612868003273,21.8156662648115));
#50055=CARTESIAN_POINT('Ctrl Pts',(-8.18960781887453,32.1337332958274,21.8127784657201));
#50056=CARTESIAN_POINT('Ctrl Pts',(-8.44415620060174,31.9782611691288,21.7960670437488));
#50057=CARTESIAN_POINT('Ctrl Pts',(-8.66866182100946,31.8728439018321,21.7830677304709));
#50058=CARTESIAN_POINT('Ctrl Pts',(-9.01623991895204,31.7539202875529,21.7635622020818));
#50059=CARTESIAN_POINT('Ctrl Pts',(-9.13180493708184,31.7211203909402,21.7571573977968));
#50060=CARTESIAN_POINT('Ctrl Pts',(-9.31376983133033,31.6797704506472,21.7468827496576));
#50061=CARTESIAN_POINT('Ctrl Pts',(-9.37909728951348,31.6669361288875,21.7431563619037));
#50062=CARTESIAN_POINT('Ctrl Pts',(-9.4672545123361,31.6522981821704,21.7380274703794));
#50063=CARTESIAN_POINT('Ctrl Pts',(-9.48978981083185,31.6487896637498,21.7367076573531));
#50064=CARTESIAN_POINT('Ctrl Pts',(-9.52756791276552,31.6432978667114,21.7344779852149));
#50065=CARTESIAN_POINT('Ctrl Pts',(-9.5427923625267,31.6411903212946,21.7335747765295));
#50066=CARTESIAN_POINT('Ctrl Pts',(-9.57439489128271,31.6370343778509,21.7316893902204));
#50067=CARTESIAN_POINT('Ctrl Pts',(-9.59077432647982,31.6350019602782,21.7307064528448));
#50068=CARTESIAN_POINT('Ctrl Pts',(-9.63520371504883,31.6298181861203,21.7280258497445));
#50069=CARTESIAN_POINT('Ctrl Pts',(-9.6632786462595,31.6268975104417,21.7263164799453));
#50070=CARTESIAN_POINT('Ctrl Pts',(-9.83078740627791,31.61158334856,21.7160381847619));
#50071=CARTESIAN_POINT('Ctrl Pts',(-9.97083258109448,31.6074872991042,21.7071230645722));
#50072=CARTESIAN_POINT('Ctrl Pts',(-10.3106000012477,31.618590645801,21.6852706723473));
#50073=CARTESIAN_POINT('Ctrl Pts',(-10.5095317489432,31.642800216435,21.6723092961866));
#50074=CARTESIAN_POINT('Ctrl Pts',(-10.8113716252329,31.7069969791034,21.6529507523898));
#50075=CARTESIAN_POINT('Ctrl Pts',(-10.9164288150099,31.7346738502891,21.6462658129306));
#50076=CARTESIAN_POINT('Ctrl Pts',(-11.0570826479788,31.7790537778506,21.6373977359519));
#50077=CARTESIAN_POINT('Ctrl Pts',(-11.0939768985247,31.7913970290446,21.6350790906563));
#50078=CARTESIAN_POINT('Ctrl Pts',(-11.1563641943484,31.8134704131955,21.6311696554965));
#50079=CARTESIAN_POINT('Ctrl Pts',(-11.1819664934257,31.8228779956116,21.6295685967896));
#50080=CARTESIAN_POINT('Ctrl Pts',(-11.2304957023538,31.8413779088336,21.6265391418273));
#50081=CARTESIAN_POINT('Ctrl Pts',(-11.2534422592592,31.8504134020597,21.6251090013564));
#50082=CARTESIAN_POINT('Ctrl Pts',(-11.3070591832291,31.8722045179716,21.6217716846679));
#50083=CARTESIAN_POINT('Ctrl Pts',(-11.3376449986924,31.8851622428578,21.6198712984982));
#50084=CARTESIAN_POINT('Ctrl Pts',(-11.4468686778143,31.9333406120716,21.6130920692451));
#50085=CARTESIAN_POINT('Ctrl Pts',(-11.5243504206456,31.9711080911887,21.6082974731666));
#50086=CARTESIAN_POINT('Ctrl Pts',(-11.8417918393518,32.1411114185032,21.5885705416975));
#50087=CARTESIAN_POINT('Ctrl Pts',(-12.0666879679872,32.299216324603,21.5744752797977));
#50088=CARTESIAN_POINT('Ctrl Pts',(-12.3194610678473,32.527163003976,21.5560460291012));
#50089=CARTESIAN_POINT('Ctrl Pts',(-12.3674970106603,32.5731132133238,21.5524031605411));
#50090=CARTESIAN_POINT('Ctrl Pts',(-12.445805707116,32.6525602928082,21.5461612535621));
#50091=CARTESIAN_POINT('Ctrl Pts',(-12.4768170330812,32.6853044006922,21.5436036597938));
#50092=CARTESIAN_POINT('Ctrl Pts',(-12.5204614908523,32.7332690282505,21.5398615764893));
#50093=CARTESIAN_POINT('Ctrl Pts',(-12.5336302373429,32.7479979563091,21.5387130307118));
#50094=CARTESIAN_POINT('Ctrl Pts',(-12.5565294316919,32.7740652431572,21.5366795845223));
#50095=CARTESIAN_POINT('Ctrl Pts',(-12.5663148466432,32.7853541202747,21.5357986529009));
#50096=CARTESIAN_POINT('Ctrl Pts',(-12.5877666462179,32.8104349434227,21.533840407924));
#50097=CARTESIAN_POINT('Ctrl Pts',(-12.5993974742058,32.8242555087767,21.5327608015043));
#50098=CARTESIAN_POINT('Ctrl Pts',(-12.6330425918723,32.8648898460294,21.5295867470802));
#50099=CARTESIAN_POINT('Ctrl Pts',(-12.6547557452605,32.8919486740716,21.5274732911627));
#50100=CARTESIAN_POINT('Ctrl Pts',(-12.7903104244531,33.0662924111964,21.5138823619218));
#50101=CARTESIAN_POINT('Ctrl Pts',(-12.8922641625607,33.2224017677656,21.5018489434669));
#50102=CARTESIAN_POINT('Ctrl Pts',(-13.0562996617983,33.5253717271096,21.4796451306051));
#50103=CARTESIAN_POINT('Ctrl Pts',(-13.1218667113147,33.6697925283375,21.4694888105455));
#50104=CARTESIAN_POINT('Ctrl Pts',(-13.2105289880325,33.9081640681836,21.4536217906998));
#50105=CARTESIAN_POINT('Ctrl Pts',(-13.240134312842,33.9994329603985,21.4477424264719));
#50106=CARTESIAN_POINT('Ctrl Pts',(-13.2758327438995,34.1278082103715,21.4397439961777));
#50107=CARTESIAN_POINT('Ctrl Pts',(-13.2852397255235,34.1639385208381,21.4375218599814));
#50108=CARTESIAN_POINT('Ctrl Pts',(-13.3004184563616,34.2264548939642,21.4337251817474));
#50109=CARTESIAN_POINT('Ctrl Pts',(-13.3064751189927,34.2527675271827,21.4321417758316));
#50110=CARTESIAN_POINT('Ctrl Pts',(-13.3182496956387,34.3068702776582,21.4289148941704));
#50111=CARTESIAN_POINT('Ctrl Pts',(-13.3239344023853,34.3346654868932,21.4272725738821));
#50112=CARTESIAN_POINT('Ctrl Pts',(-13.3376335907142,34.4062112064827,21.4230829777617));
#50113=CARTESIAN_POINT('Ctrl Pts',(-13.3451372988414,34.4500547052136,21.4205517055033));
#50114=CARTESIAN_POINT('Ctrl Pts',(-13.3771969725709,34.6624345785642,21.4084462577946));
#50115=CARTESIAN_POINT('Ctrl Pts',(-13.3898921005314,34.8325187363542,21.3992403245363));
#50116=CARTESIAN_POINT('Ctrl Pts',(-13.389547595615,35.2420129420187,21.3774222643481));
#50117=CARTESIAN_POINT('Ctrl Pts',(-13.3640366786116,35.4804553378116,21.3650138727178));
#50118=CARTESIAN_POINT('Ctrl Pts',(-13.3041286241496,35.7584090300179,21.3491057155548));
#50119=CARTESIAN_POINT('Ctrl Pts',(-13.2937170393995,35.8024200146644,21.3465411345039));
#50120=CARTESIAN_POINT('Ctrl Pts',(-13.2775434416502,35.8651572202666,21.3428027266053));
#50121=CARTESIAN_POINT('Ctrl Pts',(-13.272494286683,35.8840639862052,21.3416652449651));
#50122=CARTESIAN_POINT('Ctrl Pts',(-13.2632990017694,35.9173375929995,21.3396425222441));
#50123=CARTESIAN_POINT('Ctrl Pts',(-13.2592210829668,35.9317223597353,21.338761064133));
#50124=CARTESIAN_POINT('Ctrl Pts',(-13.2500375059252,35.9633190315991,21.3368090748593));
#50125=CARTESIAN_POINT('Ctrl Pts',(-13.2448902763815,35.9805174190649,21.3357363553798));
#50126=CARTESIAN_POINT('Ctrl Pts',(-13.2292397832685,36.0313370858835,21.332537864918));
#50127=CARTESIAN_POINT('Ctrl Pts',(-13.2183491101846,36.0648354603712,21.3303921567018));
#50128=CARTESIAN_POINT('Ctrl Pts',(-13.1978681340611,36.1246459099784,21.3265010764352));
#50129=CARTESIAN_POINT('Ctrl Pts',(-13.1884710276968,36.1510173784738,21.3247642005658));
#50130=CARTESIAN_POINT('Ctrl Pts',(-13.1787500764527,36.1772650567955,21.3230161660245));
#50131=CARTESIAN_POINT('',(-13.3897506916886,35.0009530681513,21.7311315226218));
#50132=CARTESIAN_POINT('Ctrl Pts',(-13.1787500358286,36.1772651664852,21.6644776847947));
#50133=CARTESIAN_POINT('Ctrl Pts',(-13.2052005884591,36.1058456617591,21.6685540708782));
#50134=CARTESIAN_POINT('Ctrl Pts',(-13.229244265339,36.0335344957176,21.6725954405618));
#50135=CARTESIAN_POINT('Ctrl Pts',(-13.2853773975532,35.8435413485962,21.6830989269644));
#50136=CARTESIAN_POINT('Ctrl Pts',(-13.3135856461982,35.7248549705581,21.689546781913));
#50137=CARTESIAN_POINT('Ctrl Pts',(-13.3523689842039,35.5110130260137,21.7013224548051));
#50138=CARTESIAN_POINT('Ctrl Pts',(-13.3654247099463,35.4164440716398,21.7065851171462));
#50139=CARTESIAN_POINT('Ctrl Pts',(-13.3769574710367,35.2953803598093,21.713529728992));
#50140=CARTESIAN_POINT('Ctrl Pts',(-13.3791392803472,35.2692748645804,21.7150394842961));
#50141=CARTESIAN_POINT('Ctrl Pts',(-13.3821708195026,35.2271206727215,21.7175008534419));
#50142=CARTESIAN_POINT('Ctrl Pts',(-13.3832094035605,35.2110861454004,21.7184425739285));
#50143=CARTESIAN_POINT('Ctrl Pts',(-13.3849363276215,35.1811231303917,21.7202135320163));
#50144=CARTESIAN_POINT('Ctrl Pts',(-13.3856527877675,35.1671966216966,21.7210412028214));
#50145=CARTESIAN_POINT('Ctrl Pts',(-13.3869928539982,35.1375890736215,21.7228099230972));
#50146=CARTESIAN_POINT('Ctrl Pts',(-13.3875935323677,35.1219072807308,21.7237521568866));
#50147=CARTESIAN_POINT('Ctrl Pts',(-13.3891851612891,35.071140361859,21.7268187924234));
#50148=CARTESIAN_POINT('Ctrl Pts',(-13.3897400387479,35.0360451300958,21.7289639786243));
#50149=CARTESIAN_POINT('Ctrl Pts',(-13.3897498670814,35.0009492742509,21.7311303263703));
#50150=CARTESIAN_POINT('Ctrl Pts',(-13.3897498660416,35.0009529799439,21.7311300976305));
#50151=CARTESIAN_POINT('Ctrl Pts',(-13.3897871967006,34.8681678178271,21.7393264681746));
#50152=CARTESIAN_POINT('Ctrl Pts',(-13.3820221592067,34.7355012784614,21.7478135385921));
#50153=CARTESIAN_POINT('Ctrl Pts',(-13.3370444115537,34.3534811525516,21.7725674067684));
#50154=CARTESIAN_POINT('Ctrl Pts',(-13.2797947392605,34.107345296519,21.7888426133663));
#50155=CARTESIAN_POINT('Ctrl Pts',(-13.1743644891748,33.8092252777544,21.8082373372983));
#50156=CARTESIAN_POINT('Ctrl Pts',(-13.1512200789771,33.7492613384332,21.812126653608));
#50157=CARTESIAN_POINT('Ctrl Pts',(-13.1138941227878,33.6601817731483,21.8178887982532));
#50158=CARTESIAN_POINT('Ctrl Pts',(-13.1009786533478,33.6305544958312,21.8198026613793));
#50159=CARTESIAN_POINT('Ctrl Pts',(-13.077800747378,33.5793958307059,21.8231039824557));
#50160=CARTESIAN_POINT('Ctrl Pts',(-13.0677312919129,33.5577800410288,21.8244977974237));
#50161=CARTESIAN_POINT('Ctrl Pts',(-13.0444706661095,33.5091932600773,21.8276291075011));
#50162=CARTESIAN_POINT('Ctrl Pts',(-13.0311474861603,33.4822874536548,21.8293619705711));
#50163=CARTESIAN_POINT('Ctrl Pts',(-12.9941673416453,33.4100369769172,21.8340145630055));
#50164=CARTESIAN_POINT('Ctrl Pts',(-12.9698383377374,33.3650440019246,21.8369110616529));
#50165=CARTESIAN_POINT('Ctrl Pts',(-12.8227627523316,33.1071730957554,21.853541525632));
#50166=CARTESIAN_POINT('Ctrl Pts',(-12.6781801189912,32.9075981196782,21.8664638158916));
#50167=CARTESIAN_POINT('Ctrl Pts',(-12.4321209232357,32.6357196241759,21.8859314784994));
#50168=CARTESIAN_POINT('Ctrl Pts',(-12.3462237179379,32.5504561934043,21.8923819588513));
#50169=CARTESIAN_POINT('Ctrl Pts',(-12.2060547807196,32.4254712953345,21.9027204457817));
#50170=CARTESIAN_POINT('Ctrl Pts',(-12.1548471869276,32.3824614284095,21.9064628609247));
#50171=CARTESIAN_POINT('Ctrl Pts',(-12.0844870797371,32.3268295159777,21.9116105286617));
#50172=CARTESIAN_POINT('Ctrl Pts',(-12.0664269862487,32.312844204056,21.9129323165402));
#50173=CARTESIAN_POINT('Ctrl Pts',(-12.0359757077302,32.2897519657831,21.915164349922));
#50174=CARTESIAN_POINT('Ctrl Pts',(-12.0236610282268,32.2805446271314,21.9160679129245));
#50175=CARTESIAN_POINT('Ctrl Pts',(-11.9980080842283,32.2616353824461,21.9179529107245));
#50176=CARTESIAN_POINT('Ctrl Pts',(-11.9846610627102,32.2519465936043,21.9189350918329));
#50177=CARTESIAN_POINT('Ctrl Pts',(-11.94832746727,32.2259742839834,21.9216114751428));
#50178=CARTESIAN_POINT('Ctrl Pts',(-11.9252082416032,32.2098796250075,21.92331732207));
#50179=CARTESIAN_POINT('Ctrl Pts',(-11.788424375324,32.1171657477977,21.9334139011426));
#50180=CARTESIAN_POINT('Ctrl Pts',(-11.6704058533844,32.0472161404183,21.9421366455033));
#50181=CARTESIAN_POINT('Ctrl Pts',(-11.3685700309193,31.8922147832037,21.9639392891909));
#50182=CARTESIAN_POINT('Ctrl Pts',(-11.1807258807694,31.8161013081737,21.9770543761855));
#50183=CARTESIAN_POINT('Ctrl Pts',(-10.8827796239532,31.7253975200335,21.9965967614637));
#50184=CARTESIAN_POINT('Ctrl Pts',(-10.7768680187487,31.6986667489452,22.0033193268099));
#50185=CARTESIAN_POINT('Ctrl Pts',(-10.6316422157301,31.6693916961895,22.0122275768809));
#50186=CARTESIAN_POINT('Ctrl Pts',(-10.5933116178055,31.6623503664467,22.0145503874427));
#50187=CARTESIAN_POINT('Ctrl Pts',(-10.5279481342339,31.651504755951,22.0184647135941));
#50188=CARTESIAN_POINT('Ctrl Pts',(-10.5009758692781,31.6473632950838,22.0200665596888));
#50189=CARTESIAN_POINT('Ctrl Pts',(-10.4495495423893,31.6401015162877,22.0230961623548));
#50190=CARTESIAN_POINT('Ctrl Pts',(-10.4251058324832,31.6369213970013,22.0245256801874));
#50191=CARTESIAN_POINT('Ctrl Pts',(-10.3614124523037,31.6293404448622,22.0282245237038));
#50192=CARTESIAN_POINT('Ctrl Pts',(-10.3221161121198,31.6253583610429,22.0304808456655));
#50193=CARTESIAN_POINT('Ctrl Pts',(-10.17830453932,31.6133202809862,22.0386533215906));
#50194=CARTESIAN_POINT('Ctrl Pts',(-10.0734964515061,31.6094258547114,22.0444436988178));
#50195=CARTESIAN_POINT('Ctrl Pts',(-9.71660611565063,31.6127246681469,22.0638272162417));
#50196=CARTESIAN_POINT('Ctrl Pts',(-9.46560577388935,31.6431621920133,22.0768390208613));
#50197=CARTESIAN_POINT('Ctrl Pts',(-9.15738022643535,31.7160118582454,22.0940076768971));
#50198=CARTESIAN_POINT('Ctrl Pts',(-9.0948937655809,31.732681822105,22.0975560429474));
#50199=CARTESIAN_POINT('Ctrl Pts',(-8.99053895859396,31.7637445592702,22.1036530666487));
#50200=CARTESIAN_POINT('Ctrl Pts',(-8.94840541126325,31.7771892220145,22.1061627413326));
#50201=CARTESIAN_POINT('Ctrl Pts',(-8.88798770104519,31.7977791696906,22.1098470753705));
#50202=CARTESIAN_POINT('Ctrl Pts',(-8.86948207477235,31.8042655335771,22.110987304417));
#50203=CARTESIAN_POINT('Ctrl Pts',(-8.83711662853796,31.8159261676621,22.1130038592239));
#50204=CARTESIAN_POINT('Ctrl Pts',(-8.82323278726384,31.8210311703321,22.1138762480749));
#50205=CARTESIAN_POINT('Ctrl Pts',(-8.79242670489897,31.8325878457828,22.1158286510366));
#50206=CARTESIAN_POINT('Ctrl Pts',(-8.77552267719398,31.8390842669947,22.116911108101));
#50207=CARTESIAN_POINT('Ctrl Pts',(-8.72514961835843,31.8589079368591,22.1201683968653));
#50208=CARTESIAN_POINT('Ctrl Pts',(-8.69184114462838,31.8726332114071,22.1223642235575));
#50209=CARTESIAN_POINT('Ctrl Pts',(-8.51964182168825,31.9468228370251,22.1339131329145));
#50210=CARTESIAN_POINT('Ctrl Pts',(-8.38470903366246,32.0160128949617,22.1436284602083));
#50211=CARTESIAN_POINT('Ctrl Pts',(-8.14053051457069,32.1626481525991,22.1619784413374));
#50212=CARTESIAN_POINT('Ctrl Pts',(-8.03034162285736,32.238000588316,22.1705886982985));
#50213=CARTESIAN_POINT('Ctrl Pts',(-7.84914557794703,32.3782824252039,22.1851383292965));
#50214=CARTESIAN_POINT('Ctrl Pts',(-7.77592928735999,32.4400996975595,22.191141514427));
#50215=CARTESIAN_POINT('Ctrl Pts',(-7.65446323979724,32.5518055802909,22.2012941381525));
#50216=CARTESIAN_POINT('Ctrl Pts',(-7.60494707278587,32.6002247757725,22.2054942486877));
#50217=CARTESIAN_POINT('Ctrl Pts',(-7.53391680625709,32.6740717301949,22.211614716734));
#50218=CARTESIAN_POINT('Ctrl Pts',(-7.51124033835845,32.6983518732947,22.213584092283));
#50219=CARTESIAN_POINT('Ctrl Pts',(-7.47131293553962,32.7423830903402,22.2170808483868));
#50220=CARTESIAN_POINT('Ctrl Pts',(-7.45392758289421,32.7620081133185,22.2186137523732));
#50221=CARTESIAN_POINT('Ctrl Pts',(-7.4169986531111,32.8046817735381,22.2218934033547));
#50222=CARTESIAN_POINT('Ctrl Pts',(-7.39753196867647,32.8277941385416,22.2236369559785));
#50223=CARTESIAN_POINT('Ctrl Pts',(-7.34538328570631,32.8914165980645,22.2283509535885));
#50224=CARTESIAN_POINT('Ctrl Pts',(-7.31332041030026,32.9324248386212,22.2312970767807));
#50225=CARTESIAN_POINT('Ctrl Pts',(-7.14180156178449,33.1625273605921,22.2473632307134));
#50226=CARTESIAN_POINT('Ctrl Pts',(-7.02135205553594,33.3649857624503,22.2597546337074));
#50227=CARTESIAN_POINT('Ctrl Pts',(-6.84536550365538,33.7458966409345,22.2820149374201));
#50228=CARTESIAN_POINT('Ctrl Pts',(-6.78175997293218,33.9195327300596,22.2918389028713));
#50229=CARTESIAN_POINT('Ctrl Pts',(-6.72486051399581,34.1255207552602,22.3039957312443));
#50230=CARTESIAN_POINT('Ctrl Pts',(-6.71747123191749,34.1536801024915,22.3056684144008));
#50231=CARTESIAN_POINT('Ctrl Pts',(-6.70641680112374,34.1981312548462,22.3083307426546));
#50232=CARTESIAN_POINT('Ctrl Pts',(-6.70250762009858,34.2143615645847,22.3093073938329));
#50233=CARTESIAN_POINT('Ctrl Pts',(-6.69529062534935,34.2453284753201,22.3111806270871));
#50234=CARTESIAN_POINT('Ctrl Pts',(-6.69196116566526,34.2600593280704,22.3120760213429));
#50235=CARTESIAN_POINT('Ctrl Pts',(-6.68399119241162,34.2964508742514,22.3142979522997));
#50236=CARTESIAN_POINT('Ctrl Pts',(-6.67946440979049,34.3181355550316,22.3156305343772));
#50237=CARTESIAN_POINT('Ctrl Pts',(-6.6640779178295,34.3956311686845,22.3204196891367));
#50238=CARTESIAN_POINT('Ctrl Pts',(-6.65441075713335,34.4516664648283,22.3239319989747));
#50239=CARTESIAN_POINT('Ctrl Pts',(-6.61344575588223,34.7308663815522,22.3415921554194));
#50240=CARTESIAN_POINT('Ctrl Pts',(-6.60304682726792,34.9565187894291,22.3563253559259));
#50241=CARTESIAN_POINT('Ctrl Pts',(-6.62411897839837,35.3494355253839,22.3814689111761));
#50242=CARTESIAN_POINT('Ctrl Pts',(-6.64560491559087,35.516453853132,22.392003007808));
#50243=CARTESIAN_POINT('Ctrl Pts',(-6.68819631154312,35.7240689634728,22.4048054868156));
#50244=CARTESIAN_POINT('Ctrl Pts',(-6.69781864164055,35.7667581624873,22.4074231291862));
#50245=CARTESIAN_POINT('Ctrl Pts',(-6.71500267386269,35.83665650359,22.4116865502195));
#50246=CARTESIAN_POINT('Ctrl Pts',(-6.72208235676282,35.8639777392101,22.4133472646366));
#50247=CARTESIAN_POINT('Ctrl Pts',(-6.73654233511079,35.9170420311705,22.4165625403042));
#50248=CARTESIAN_POINT('Ctrl Pts',(-6.74388808026892,35.9427922591487,22.4181180634545));
#50249=CARTESIAN_POINT('Ctrl Pts',(-6.76227949196456,36.0044821682919,22.4218345917871));
#50250=CARTESIAN_POINT('Ctrl Pts',(-6.77361959960515,36.0403308060633,22.4239860182427));
#50251=CARTESIAN_POINT('Ctrl Pts',(-6.81447741735757,36.1623913525112,22.4312898845888));
#50252=CARTESIAN_POINT('Ctrl Pts',(-6.84687438983762,36.2476011219593,22.4363503663778));
#50253=CARTESIAN_POINT('Ctrl Pts',(-6.9879272825928,36.5778597812969,22.4559759662225));
#50254=CARTESIAN_POINT('Ctrl Pts',(-7.12203266361379,36.8109440050839,22.4697769151542));
#50255=CARTESIAN_POINT('Ctrl Pts',(-7.32162444066562,37.0787173494879,22.4878651231777));
#50256=CARTESIAN_POINT('Ctrl Pts',(-7.36260474475307,37.1304710405901,22.4914838524526));
#50257=CARTESIAN_POINT('Ctrl Pts',(-7.43394002675994,37.2153453461314,22.497688800945));
#50258=CARTESIAN_POINT('Ctrl Pts',(-7.4634905847049,37.2491194671204,22.5002342112493));
#50259=CARTESIAN_POINT('Ctrl Pts',(-7.50697878240321,37.2968759556688,22.5039616193136));
#50260=CARTESIAN_POINT('Ctrl Pts',(-7.52038286599269,37.3113400388686,22.505108061081));
#50261=CARTESIAN_POINT('Ctrl Pts',(-7.54416065250997,37.3365532938056,22.5071392542106));
#50262=CARTESIAN_POINT('Ctrl Pts',(-7.55448038674853,37.3473521261819,22.5080200699032));
#50263=CARTESIAN_POINT('Ctrl Pts',(-7.57745693619613,37.3710793899617,22.5099799145479));
#50264=CARTESIAN_POINT('Ctrl Pts',(-7.59014593088893,37.3839747697212,22.5110612629601));
#50265=CARTESIAN_POINT('Ctrl Pts',(-7.62756282720698,37.4213962736053,22.5142453382233));
#50266=CARTESIAN_POINT('Ctrl Pts',(-7.65256553169329,37.4456429148682,22.516367245006));
#50267=CARTESIAN_POINT('Ctrl Pts',(-7.81040413290899,37.5940581561363,22.5297023582383));
#50268=CARTESIAN_POINT('Ctrl Pts',(-7.95266982387728,37.7077476531749,22.5414453349241));
#50269=CARTESIAN_POINT('Ctrl Pts',(-8.29801832697801,37.9408890909804,22.568302210783));
#50270=CARTESIAN_POINT('Ctrl Pts',(-8.50584439936249,38.0517374492212,22.5832951254527));
#50271=CARTESIAN_POINT('Ctrl Pts',(-8.76843260760859,38.1584807113425,22.6004868945263));
#50272=CARTESIAN_POINT('Ctrl Pts',(-8.81376362727027,38.1757837267063,22.603398381087));
#50273=CARTESIAN_POINT('Ctrl Pts',(-8.88695075780059,38.2019336577603,22.6080114324668));
#50274=CARTESIAN_POINT('Ctrl Pts',(-8.91457565630795,38.2114034063355,22.6097330393229));
#50275=CARTESIAN_POINT('Ctrl Pts',(-8.96765906593314,38.2288370308799,22.6130048958773));
#50276=CARTESIAN_POINT('Ctrl Pts',(-8.99309583709367,38.236859657542,22.6145569457201));
#50277=CARTESIAN_POINT('Ctrl Pts',(-9.05171559621727,38.2545901280128,22.6180988632354));
#50278=CARTESIAN_POINT('Ctrl Pts',(-9.08495799973722,38.2640922895552,22.6200820313661));
#50279=CARTESIAN_POINT('Ctrl Pts',(-9.19200487203,38.292927125482,22.626392044211));
#50280=CARTESIAN_POINT('Ctrl Pts',(-9.26632101758552,38.3102781610593,22.6306569510443));
#50281=CARTESIAN_POINT('Ctrl Pts',(-9.57740228938219,38.3719157862724,22.6481279932382));
#50282=CARTESIAN_POINT('Ctrl Pts',(-9.81795078746105,38.3934150874859,22.660674800165));
#50283=CARTESIAN_POINT('Ctrl Pts',(-10.200571702129,38.3867823715123,22.681103085593));
#50284=CARTESIAN_POINT('Ctrl Pts',(-10.3420831469256,38.3754251200986,22.6887776084487));
#50285=CARTESIAN_POINT('Ctrl Pts',(-10.5101320608057,38.351261317329,22.6984497930879));
#50286=CARTESIAN_POINT('Ctrl Pts',(-10.5377616887143,38.3469388096134,22.7000584480233));
#50287=CARTESIAN_POINT('Ctrl Pts',(-10.5815525963573,38.339531736401,22.7026417857048));
#50288=CARTESIAN_POINT('Ctrl Pts',(-10.5977509274284,38.3366704129808,22.7036047330348));
#50289=CARTESIAN_POINT('Ctrl Pts',(-10.6288961664269,38.3309347541883,22.705471533659));
#50290=CARTESIAN_POINT('Ctrl Pts',(-10.64384558234,38.3280774567546,22.7063744717012));
#50291=CARTESIAN_POINT('Ctrl Pts',(-10.6811594660227,38.3206848068373,22.7086446819186));
#50292=CARTESIAN_POINT('Ctrl Pts',(-10.7034981331256,38.3160241433137,22.7100185920139));
#50293=CARTESIAN_POINT('Ctrl Pts',(-10.7859265184943,38.2979561943271,22.7151388463239));
#50294=CARTESIAN_POINT('Ctrl Pts',(-10.8456917047292,38.2831387625296,22.7189510136887));
#50295=CARTESIAN_POINT('Ctrl Pts',(-11.1174819575795,38.2078412579838,22.7366488834324));
#50296=CARTESIAN_POINT('Ctrl Pts',(-11.3236941565528,38.1283933409034,22.7510560544434));
#50297=CARTESIAN_POINT('Ctrl Pts',(-11.6203304299284,37.9794889124857,22.7722596522514));
#50298=CARTESIAN_POINT('Ctrl Pts',(-11.7174102892579,37.9246076939456,22.7792921829856));
#50299=CARTESIAN_POINT('Ctrl Pts',(-11.8765850910188,37.8239585697418,22.7909295381597));
#50300=CARTESIAN_POINT('Ctrl Pts',(-11.9401410101294,37.7806775938133,22.7956079225141));
#50301=CARTESIAN_POINT('Ctrl Pts',(-12.030028303397,37.7148815250112,22.8022729919868));
#50302=CARTESIAN_POINT('Ctrl Pts',(-12.0575699910443,37.6940680154032,22.804322216628));
#50303=CARTESIAN_POINT('Ctrl Pts',(-12.1057546284907,37.6564844128666,22.8079212169355));
#50304=CARTESIAN_POINT('Ctrl Pts',(-12.1265268242327,37.6398855499504,22.809477434317));
#50305=CARTESIAN_POINT('Ctrl Pts',(-12.1699476299181,37.6043432897772,22.812741481674));
#50306=CARTESIAN_POINT('Ctrl Pts',(-12.1925484534373,37.5853448602842,22.8144469456281));
#50307=CARTESIAN_POINT('Ctrl Pts',(-12.2528068087566,37.533332627246,22.8190140901353));
#50308=CARTESIAN_POINT('Ctrl Pts',(-12.2899864433215,37.499775023734,22.8218535611006));
#50309=CARTESIAN_POINT('Ctrl Pts',(-12.5155550441293,37.2869235113488,22.8392506164396));
#50310=CARTESIAN_POINT('Ctrl Pts',(-12.6835313330988,37.0872725588065,22.8528762465068));
#50311=CARTESIAN_POINT('Ctrl Pts',(-12.8894240682693,36.7760681177932,22.8727119541689));
#50312=CARTESIAN_POINT('Ctrl Pts',(-12.9470511194547,36.6787126695618,22.8787610932485));
#50313=CARTESIAN_POINT('Ctrl Pts',(-13.0295991552326,36.5218590229713,22.8885358050778));
#50314=CARTESIAN_POINT('Ctrl Pts',(-13.0578738109652,36.4642174124952,22.8921340885628));
#50315=CARTESIAN_POINT('Ctrl Pts',(-13.0938327008631,36.3853199706915,22.8971127072279));
#50316=CARTESIAN_POINT('Ctrl Pts',(-13.1029674863365,36.3647362097376,22.898416407167));
#50317=CARTESIAN_POINT('Ctrl Pts',(-13.1179696486694,36.3300018609973,22.9006268686073));
#50318=CARTESIAN_POINT('Ctrl Pts',(-13.1239475977154,36.3158993428972,22.9015272402178));
#50319=CARTESIAN_POINT('Ctrl Pts',(-13.13620761629,36.2864224305801,22.9034160612439));
#50320=CARTESIAN_POINT('Ctrl Pts',(-13.1424725488627,36.2710417524475,22.904405382709));
#50321=CARTESIAN_POINT('Ctrl Pts',(-13.1589894394447,36.2296234539651,22.9070783602887));
#50322=CARTESIAN_POINT('Ctrl Pts',(-13.1690321917515,36.2035044544652,22.908773312553));
#50323=CARTESIAN_POINT('Ctrl Pts',(-13.1787500671531,36.1772650819055,22.9104832616759));
#50324=CARTESIAN_POINT('Origin',(-10.,35.,23.));
#50325=CARTESIAN_POINT('',(-13.178750056895,36.1772651096035,24.1659535227378));
#50326=CARTESIAN_POINT('',(-13.1787500981843,36.1772649981177,23.8178418924018));
#50327=CARTESIAN_POINT('',(-13.1787500671536,36.1772650819043,23.));
#50328=CARTESIAN_POINT('',(-13.3897493118688,34.997840096011,22.6386987365911));
#50329=CARTESIAN_POINT('Ctrl Pts',(-13.1787500981843,36.1772649981177,23.8178418924018));
#50330=CARTESIAN_POINT('Ctrl Pts',(-13.1694440470449,36.2023924002069,23.8161924048054));
#50331=CARTESIAN_POINT('Ctrl Pts',(-13.1598380975955,36.227414744048,23.8145512589474));
#50332=CARTESIAN_POINT('Ctrl Pts',(-13.1303459993096,36.3015952007151,23.8096904199983));
#50333=CARTESIAN_POINT('Ctrl Pts',(-13.1096041701896,36.3503993931377,23.8064984235902));
#50334=CARTESIAN_POINT('Ctrl Pts',(-13.0751712850199,36.426412371984,23.8015343405411));
#50335=CARTESIAN_POINT('Ctrl Pts',(-13.0622446906755,36.4539560626101,23.7997371210261));
#50336=CARTESIAN_POINT('Ctrl Pts',(-13.037392130686,36.5051091176036,23.7964012308428));
#50337=CARTESIAN_POINT('Ctrl Pts',(-13.0255573687388,36.5287599806311,23.7948596086142));
#50338=CARTESIAN_POINT('Ctrl Pts',(-12.9983125749134,36.5816507236623,23.7914125762159));
#50339=CARTESIAN_POINT('Ctrl Pts',(-12.9827491305477,36.6108088163751,23.7895126359239));
#50340=CARTESIAN_POINT('Ctrl Pts',(-12.9337347569534,36.6994901666946,23.78373133017));
#50341=CARTESIAN_POINT('Ctrl Pts',(-12.8989090301473,36.7582359773237,23.779897966608));
#50342=CARTESIAN_POINT('Ctrl Pts',(-12.7279490069987,37.027714544724,23.7622230032025));
#50343=CARTESIAN_POINT('Ctrl Pts',(-12.5704739595874,37.2239604773315,23.749152693907));
#50344=CARTESIAN_POINT('Ctrl Pts',(-12.2903365481919,37.5031344233068,23.7280551178306));
#50345=CARTESIAN_POINT('Ctrl Pts',(-12.181471230538,37.5985569296795,23.7202397615594));
#50346=CARTESIAN_POINT('Ctrl Pts',(-12.0444421099716,37.7039714192192,23.7103945622788));
#50347=CARTESIAN_POINT('Ctrl Pts',(-12.0218109287665,37.7209346619372,23.7087681940128));
#50348=CARTESIAN_POINT('Ctrl Pts',(-11.9856313184478,37.7473525712948,23.7061630018856));
#50349=CARTESIAN_POINT('Ctrl Pts',(-11.972220989971,37.7569951442803,23.7051962563634));
#50350=CARTESIAN_POINT('Ctrl Pts',(-11.9462020140114,37.7754168740919,23.7033173185527));
#50351=CARTESIAN_POINT('Ctrl Pts',(-11.9336033012458,37.7842089259797,23.70240598313));
#50352=CARTESIAN_POINT('Ctrl Pts',(-11.9021830721159,37.8058195219928,23.7001301771527));
#50353=CARTESIAN_POINT('Ctrl Pts',(-11.883291479793,37.8185345075371,23.6987592207321));
#50354=CARTESIAN_POINT('Ctrl Pts',(-11.8089231531161,37.8675066344641,23.6933566481783));
#50355=CARTESIAN_POINT('Ctrl Pts',(-11.7525190574556,37.9023220098992,23.6892470656246));
#50356=CARTESIAN_POINT('Ctrl Pts',(-11.5919348887097,37.9950542825703,23.6775882311117));
#50357=CARTESIAN_POINT('Ctrl Pts',(-11.4856684540666,38.0491627629834,23.6699224584744));
#50358=CARTESIAN_POINT('Ctrl Pts',(-11.1494210048519,38.1986153519764,23.6462064435097));
#50359=CARTESIAN_POINT('Ctrl Pts',(-10.9115914089616,38.2743467580589,23.6302433837918));
#50360=CARTESIAN_POINT('Ctrl Pts',(-10.6177625164372,38.3333702471048,23.6120248941159));
#50361=CARTESIAN_POINT('Ctrl Pts',(-10.5677172143813,38.3422575175997,23.6089692491099));
#50362=CARTESIAN_POINT('Ctrl Pts',(-10.4878872640331,38.3545891320663,23.6041679680593));
#50363=CARTESIAN_POINT('Ctrl Pts',(-10.4582256612732,38.3587693515591,23.6023998525243));
#50364=CARTESIAN_POINT('Ctrl Pts',(-10.4022183564581,38.365906717322,23.599090050561));
#50365=CARTESIAN_POINT('Ctrl Pts',(-10.3758859713122,38.3689490099072,23.5975458420579));
#50366=CARTESIAN_POINT('Ctrl Pts',(-10.3159376064496,38.3751634613507,23.5940561779519));
#50367=CARTESIAN_POINT('Ctrl Pts',(-10.2823042112321,38.3781428938766,23.5921167952211));
#50368=CARTESIAN_POINT('Ctrl Pts',(-10.1764762535761,38.3859261165218,23.5860680207337));
#50369=CARTESIAN_POINT('Ctrl Pts',(-10.104166980661,38.3889216267094,23.582013627439));
#50370=CARTESIAN_POINT('Ctrl Pts',(-9.92981838308282,38.3905579954587,23.57238083607));
#50371=CARTESIAN_POINT('Ctrl Pts',(-9.8278278545131,38.3869112206398,23.5668646894312));
#50372=CARTESIAN_POINT('Ctrl Pts',(-9.6783393914639,38.3747949007638,23.5588416264451));
#50373=CARTESIAN_POINT('Ctrl Pts',(-9.63061350507016,38.3699050256527,23.5562891447993));
#50374=CARTESIAN_POINT('Ctrl Pts',(-9.37552963722338,38.3382855064769,23.5426418228869));
#50375=CARTESIAN_POINT('Ctrl Pts',(-9.1708961320108,38.2934304167805,23.5317000523753));
#50376=CARTESIAN_POINT('Ctrl Pts',(-8.92768901535505,38.2160051841248,23.5174466710071));
#50377=CARTESIAN_POINT('Ctrl Pts',(-8.88395227236528,38.2010900073663,23.5148310170969));
#50378=CARTESIAN_POINT('Ctrl Pts',(-8.82307951324614,38.1789319507984,23.5110989805216));
#50379=CARTESIAN_POINT('Ctrl Pts',(-8.80567568239572,38.1724343288568,23.5100213329413));
#50380=CARTESIAN_POINT('Ctrl Pts',(-8.77423159431035,38.1603994445343,23.5080534799556));
#50381=CARTESIAN_POINT('Ctrl Pts',(-8.76017301405214,38.1549107551086,23.507166026257));
#50382=CARTESIAN_POINT('Ctrl Pts',(-8.73061806457926,38.1431439832503,23.5052834440944));
#50383=CARTESIAN_POINT('Ctrl Pts',(-8.71513092735981,38.1368449176771,23.5042871921066));
#50384=CARTESIAN_POINT('Ctrl Pts',(-8.67269888365236,38.1192196323019,23.5015320029517));
#50385=CARTESIAN_POINT('Ctrl Pts',(-8.64585349441067,38.1076593257293,23.4997602926481));
#50386=CARTESIAN_POINT('Ctrl Pts',(-8.58537585143135,38.080683720785,23.4957092544685));
#50387=CARTESIAN_POINT('Ctrl Pts',(-8.55183997815384,38.0650621545962,23.4934204316772));
#50388=CARTESIAN_POINT('Ctrl Pts',(-8.44181771393183,38.0116032794516,23.4857853553859));
#50389=CARTESIAN_POINT('Ctrl Pts',(-8.36650693795593,37.9714281500254,23.480355326714));
#50390=CARTESIAN_POINT('Ctrl Pts',(-8.05246275588005,37.7883496970749,23.4570436344576));
#50391=CARTESIAN_POINT('Ctrl Pts',(-7.83024639287046,37.6191618495753,23.4389595248882));
#50392=CARTESIAN_POINT('Ctrl Pts',(-7.58602075993207,37.3805668005,23.418022523368));
#50393=CARTESIAN_POINT('Ctrl Pts',(-7.54208347470578,37.3351747711789,23.4141997906668));
#50394=CARTESIAN_POINT('Ctrl Pts',(-7.47748959503964,37.2645977908168,23.4084903912907));
#50395=CARTESIAN_POINT('Ctrl Pts',(-7.45588682222745,37.240301351695,23.4065647516059));
#50396=CARTESIAN_POINT('Ctrl Pts',(-7.41737208023839,37.1957084724819,23.4031006310243));
#50397=CARTESIAN_POINT('Ctrl Pts',(-7.40034169456701,37.1755181960916,23.4015573999201));
#50398=CARTESIAN_POINT('Ctrl Pts',(-7.36394537603487,37.1313309896768,23.3982330277994));
#50399=CARTESIAN_POINT('Ctrl Pts',(-7.34466728025906,37.1072645789736,23.3964554564036));
#50400=CARTESIAN_POINT('Ctrl Pts',(-7.29097505295884,37.0383292244939,23.3914535547448));
#50401=CARTESIAN_POINT('Ctrl Pts',(-7.25735066109879,36.9928565692545,23.3882595940673));
#50402=CARTESIAN_POINT('Ctrl Pts',(-7.18326972081692,36.8872428654232,23.3810586019873));
#50403=CARTESIAN_POINT('Ctrl Pts',(-7.14357238987514,36.8266026573691,23.3770777801798));
#50404=CARTESIAN_POINT('Ctrl Pts',(-7.0045879838954,36.5986691191853,23.3625813834011));
#50405=CARTESIAN_POINT('Ctrl Pts',(-6.91781022090188,36.4241992602515,23.3524011966253));
#50406=CARTESIAN_POINT('Ctrl Pts',(-6.79247288801839,36.1062782847982,23.3341807746097));
#50407=CARTESIAN_POINT('Ctrl Pts',(-6.74746016543556,35.9659489878006,23.3262327773586));
#50408=CARTESIAN_POINT('Ctrl Pts',(-6.70484339488062,35.7957063970745,23.3162390737919));
#50409=CARTESIAN_POINT('Ctrl Pts',(-6.69831630727073,35.7681734210844,23.3146119696541));
#50410=CARTESIAN_POINT('Ctrl Pts',(-6.68852571355139,35.7244418729553,23.3120058696344));
#50411=CARTESIAN_POINT('Ctrl Pts',(-6.68503452159498,35.708295015611,23.3110389664242));
#50412=CARTESIAN_POINT('Ctrl Pts',(-6.6785249078087,35.6770851279166,23.3091599630209));
#50413=CARTESIAN_POINT('Ctrl Pts',(-6.67549063766089,35.6620260749826,23.3082487229304));
#50414=CARTESIAN_POINT('Ctrl Pts',(-6.66821432190783,35.624601838705,23.3059735057705));
#50415=CARTESIAN_POINT('Ctrl Pts',(-6.664095055223,35.6022137488682,23.304603050029));
#50416=CARTESIAN_POINT('Ctrl Pts',(-6.64887776011335,35.5145561510175,23.2992051424694));
#50417=CARTESIAN_POINT('Ctrl Pts',(-6.6394680226325,35.4490121989421,23.2950998881306));
#50418=CARTESIAN_POINT('Ctrl Pts',(-6.61853351234081,35.2650338455354,23.283458469059));
#50419=CARTESIAN_POINT('Ctrl Pts',(-6.61131597000853,35.146207252024,23.2758061427764));
#50420=CARTESIAN_POINT('Ctrl Pts',(-6.60835629606417,34.7780968254941,23.2520801987147));
#50421=CARTESIAN_POINT('Ctrl Pts',(-6.63383047159029,34.5294389852347,23.2360930170618));
#50422=CARTESIAN_POINT('Ctrl Pts',(-6.6971695240008,34.2355682775101,23.2178191134987));
#50423=CARTESIAN_POINT('Ctrl Pts',(-6.70913613335116,34.1855919602214,23.2147302498774));
#50424=CARTESIAN_POINT('Ctrl Pts',(-6.72982897005069,34.1070979865729,23.209906648742));
#50425=CARTESIAN_POINT('Ctrl Pts',(-6.73780273619619,34.078391803655,23.2081485227569));
#50426=CARTESIAN_POINT('Ctrl Pts',(-6.75359194803223,34.024323896758,23.2048473030709));
#50427=CARTESIAN_POINT('Ctrl Pts',(-6.76132874644872,33.9989417256242,23.2033018380946));
#50428=CARTESIAN_POINT('Ctrl Pts',(-6.77966767816542,33.9412162177968,23.1997956777938));
#50429=CARTESIAN_POINT('Ctrl Pts',(-6.79046058297763,33.9089362021686,23.1978412850797));
#50430=CARTESIAN_POINT('Ctrl Pts',(-6.82623977061605,33.8070544435604,23.1916881984726));
#50431=CARTESIAN_POINT('Ctrl Pts',(-6.8530189159206,33.7381029237299,23.1875473679018));
#50432=CARTESIAN_POINT('Ctrl Pts',(-6.92333828605412,33.5732409311739,23.1776544468405));
#50433=CARTESIAN_POINT('Ctrl Pts',(-6.96913370522978,33.4783757844422,23.1719695833861));
#50434=CARTESIAN_POINT('Ctrl Pts',(-7.07840889812364,33.2765929052141,23.1597085400523));
#50435=CARTESIAN_POINT('Ctrl Pts',(-7.14350115414826,33.1707266542365,23.1531657939876));
#50436=CARTESIAN_POINT('Ctrl Pts',(-7.2967056248336,32.9497448973863,23.1388544187194));
#50437=CARTESIAN_POINT('Ctrl Pts',(-7.38667947823775,32.8362314058612,23.1310766571475));
#50438=CARTESIAN_POINT('Ctrl Pts',(-7.50750469824291,32.7023614232893,23.1208944326394));
#50439=CARTESIAN_POINT('Ctrl Pts',(-7.53180444153565,32.6762774836675,23.1188582708401));
#50440=CARTESIAN_POINT('Ctrl Pts',(-7.56901054606389,32.6375816141312,23.11574913724));
#50441=CARTESIAN_POINT('Ctrl Pts',(-7.58161436727421,32.6246808099203,23.1146973169989));
#50442=CARTESIAN_POINT('Ctrl Pts',(-7.60484796358133,32.6012763628509,23.112759612337));
#50443=CARTESIAN_POINT('Ctrl Pts',(-7.61544509433741,32.5907415580135,23.1118761372337));
#50444=CARTESIAN_POINT('Ctrl Pts',(-7.64024170948591,32.5664146398687,23.1098098000257));
#50445=CARTESIAN_POINT('Ctrl Pts',(-7.65449268376823,32.5526765063624,23.108623075485));
#50446=CARTESIAN_POINT('Ctrl Pts',(-7.70176270925975,32.5078996688428,23.1046919343801));
#50447=CARTESIAN_POINT('Ctrl Pts',(-7.73528264588995,32.477399439137,23.1019125308104));
#50448=CARTESIAN_POINT('Ctrl Pts',(-7.81979433282978,32.40354335991,23.0949465905495));
#50449=CARTESIAN_POINT('Ctrl Pts',(-7.87147726008746,32.3610089282996,23.0907227504941));
#50450=CARTESIAN_POINT('Ctrl Pts',(-8.1458269260407,32.1485267275507,23.0686166221264));
#50451=CARTESIAN_POINT('Ctrl Pts',(-8.38771595592868,32.0050987041101,23.0502855313726));
#50452=CARTESIAN_POINT('Ctrl Pts',(-8.71868527498482,31.8607025106908,23.0279008285589));
#50453=CARTESIAN_POINT('Ctrl Pts',(-8.79401063808962,31.83100213861,23.0229609415297));
#50454=CARTESIAN_POINT('Ctrl Pts',(-8.90105552995791,31.7931654272864,23.0161543785634));
#50455=CARTESIAN_POINT('Ctrl Pts',(-8.93193473242825,31.7827490585224,23.014215105562));
#50456=CARTESIAN_POINT('Ctrl Pts',(-8.98863444207013,31.7645290906823,23.0106972902869));
#50457=CARTESIAN_POINT('Ctrl Pts',(-9.01440678523066,31.7565853835132,23.0091143431091));
#50458=CARTESIAN_POINT('Ctrl Pts',(-9.0670490480128,31.7410450918367,23.0059126139253));
#50459=CARTESIAN_POINT('Ctrl Pts',(-9.0939235462556,31.7334712460837,23.0042946641622));
#50460=CARTESIAN_POINT('Ctrl Pts',(-9.16169917519376,31.7152713441513,23.0002540950105));
#50461=CARTESIAN_POINT('Ctrl Pts',(-9.2027117367464,31.7050762886332,22.9978452306953));
#50462=CARTESIAN_POINT('Ctrl Pts',(-9.38463472994689,31.6634490439883,22.9873054408207));
#50463=CARTESIAN_POINT('Ctrl Pts',(-9.52728472119763,31.6402689021603,22.9794318342961));
#50464=CARTESIAN_POINT('Ctrl Pts',(-9.80279090209768,31.61340138008,22.964591953365));
#50465=CARTESIAN_POINT('Ctrl Pts',(-9.93523275854053,31.6082825495473,22.9576156553733));
#50466=CARTESIAN_POINT('Ctrl Pts',(-10.2186429965412,31.6139383961391,22.9425441038466));
#50467=CARTESIAN_POINT('Ctrl Pts',(-10.3692683777537,31.6270413314131,22.9344458532902));
#50468=CARTESIAN_POINT('Ctrl Pts',(-10.5540757490596,31.6556464104576,22.9238905821411));
#50469=CARTESIAN_POINT('Ctrl Pts',(-10.5895579876908,31.6617187011541,22.9218350723981));
#50470=CARTESIAN_POINT('Ctrl Pts',(-10.6427291402081,31.6716923104537,22.918702272269));
#50471=CARTESIAN_POINT('Ctrl Pts',(-10.6604955359162,31.6751724196638,22.9176466167639));
#50472=CARTESIAN_POINT('Ctrl Pts',(-10.6927275976253,31.6817546202959,22.9157138968354));
#50473=CARTESIAN_POINT('Ctrl Pts',(-10.7072020536281,31.6848093335655,22.9148394107943));
#50474=CARTESIAN_POINT('Ctrl Pts',(-10.7408229476522,31.6921349433345,22.9127930259245));
#50475=CARTESIAN_POINT('Ctrl Pts',(-10.7599527147625,31.6964773795904,22.9116173217179));
#50476=CARTESIAN_POINT('Ctrl Pts',(-10.8221236798561,31.711158693517,22.907761716833));
#50477=CARTESIAN_POINT('Ctrl Pts',(-10.8649986353705,31.7221742801175,22.9050485713767));
#50478=CARTESIAN_POINT('Ctrl Pts',(-10.9700246437505,31.7513619429165,22.8982884150339));
#50479=CARTESIAN_POINT('Ctrl Pts',(-11.0318934371808,31.770481130059,22.894206648712));
#50480=CARTESIAN_POINT('Ctrl Pts',(-11.3326357937338,31.8729430700979,22.8739873588518));
#50481=CARTESIAN_POINT('Ctrl Pts',(-11.5622427693034,31.9810894878182,22.8574401783296));
#50482=CARTESIAN_POINT('Ctrl Pts',(-11.8661939716176,32.168298586302,22.8350714814403));
#50483=CARTESIAN_POINT('Ctrl Pts',(-11.9521627892503,32.2268651951213,22.8286739422701));
#50484=CARTESIAN_POINT('Ctrl Pts',(-12.066813975298,32.3129501226264,22.820049079161));
#50485=CARTESIAN_POINT('Ctrl Pts',(-12.0979036647445,32.3371523772841,22.8176999712436));
#50486=CARTESIAN_POINT('Ctrl Pts',(-12.1477355377951,32.3773593728496,22.8139162615041));
#50487=CARTESIAN_POINT('Ctrl Pts',(-12.1667368720697,32.3930356399658,22.8124689844635));
#50488=CARTESIAN_POINT('Ctrl Pts',(-12.2064373081224,32.426522778753,22.8094347744225));
#50489=CARTESIAN_POINT('Ctrl Pts',(-12.2270955442067,32.4443795071023,22.8078498350675));
#50490=CARTESIAN_POINT('Ctrl Pts',(-12.2767796559105,32.4883858712774,22.8040215391787));
#50491=CARTESIAN_POINT('Ctrl Pts',(-12.3055739584146,32.5147917524815,22.801788898798));
#50492=CARTESIAN_POINT('Ctrl Pts',(-12.4136911549082,32.6174376465673,22.7933426946227));
#50493=CARTESIAN_POINT('Ctrl Pts',(-12.4897454112563,32.6970281644076,22.7872708146075));
#50494=CARTESIAN_POINT('Ctrl Pts',(-12.6964471328915,32.9355740600739,22.7701517313383));
#50495=CARTESIAN_POINT('Ctrl Pts',(-12.8166747149855,33.1028903693201,22.7594226545617));
#50496=CARTESIAN_POINT('Ctrl Pts',(-12.9884260337641,33.3945798929774,22.7413164429681));
#50497=CARTESIAN_POINT('Ctrl Pts',(-13.0490531827442,33.5129453193569,22.7341029229709));
#50498=CARTESIAN_POINT('Ctrl Pts',(-13.113870881966,33.660223889843,22.7249368637606));
#50499=CARTESIAN_POINT('Ctrl Pts',(-13.1248506179628,33.6860363771903,22.7233234641984));
#50500=CARTESIAN_POINT('Ctrl Pts',(-13.1417656050304,33.7272136376652,22.7207342724987));
#50501=CARTESIAN_POINT('Ctrl Pts',(-13.1479116117321,33.7424910731574,22.719770307238));
#50502=CARTESIAN_POINT('Ctrl Pts',(-13.1595858714477,33.7721323139816,22.7178924862814));
#50503=CARTESIAN_POINT('Ctrl Pts',(-13.1651280048847,33.7864899620716,22.7169794300388));
#50504=CARTESIAN_POINT('Ctrl Pts',(-13.1786788532794,33.822319652334,22.7146930548227));
#50505=CARTESIAN_POINT('Ctrl Pts',(-13.1865678774194,33.8438359315183,22.7133131208587));
#50506=CARTESIAN_POINT('Ctrl Pts',(-13.216830825245,33.9290374133678,22.707826128039));
#50507=CARTESIAN_POINT('Ctrl Pts',(-13.2375172912439,33.9933014483144,22.7036381059386));
#50508=CARTESIAN_POINT('Ctrl Pts',(-13.2904172436133,34.1761903180638,22.6916605835383));
#50509=CARTESIAN_POINT('Ctrl Pts',(-13.3181174214828,34.2960097984519,22.6837479201958));
#50510=CARTESIAN_POINT('Ctrl Pts',(-13.3727273443506,34.6088327219239,22.6632787510039));
#50511=CARTESIAN_POINT('Ctrl Pts',(-13.3896252539285,34.8031437948669,22.6507666687411));
#50512=CARTESIAN_POINT('Ctrl Pts',(-13.3897493118688,34.997840096011,22.6386987365911));
#50513=CARTESIAN_POINT('Ctrl Pts',(-13.3897493143602,34.9978440095506,22.6386984940168));
#50514=CARTESIAN_POINT('Ctrl Pts',(-13.3897813532124,35.0482169959177,22.6355762082653));
#50515=CARTESIAN_POINT('Ctrl Pts',(-13.388690550124,35.0985867233104,22.6324834989972));
#50516=CARTESIAN_POINT('Ctrl Pts',(-13.3847480802509,35.1882419257925,22.6270318747773));
#50517=CARTESIAN_POINT('Ctrl Pts',(-13.3823338315342,35.2275360092128,22.6246607571154));
#50518=CARTESIAN_POINT('Ctrl Pts',(-13.3771512899539,35.2931818710239,22.620729142537));
#50519=CARTESIAN_POINT('Ctrl Pts',(-13.3747575965931,35.3195585528621,22.6191574267673));
#50520=CARTESIAN_POINT('Ctrl Pts',(-13.3694901232354,35.3709085110181,22.6161126305208));
#50521=CARTESIAN_POINT('Ctrl Pts',(-13.3666472033063,35.3958831560609,22.6146387018143));
#50522=CARTESIAN_POINT('Ctrl Pts',(-13.360026985118,35.4487966316066,22.6115298301513));
#50523=CARTESIAN_POINT('Ctrl Pts',(-13.3561783869392,35.47672472364,22.6098972152488));
#50524=CARTESIAN_POINT('Ctrl Pts',(-13.345491508273,35.547715740626,22.6057665190862));
#50525=CARTESIAN_POINT('Ctrl Pts',(-13.3381698751238,35.5907013570226,22.6032835401932));
#50526=CARTESIAN_POINT('Ctrl Pts',(-13.3010067506192,35.7860401113829,22.5920677815193));
#50527=CARTESIAN_POINT('Ctrl Pts',(-13.2615494772013,35.9363795930766,22.5836353822097));
#50528=CARTESIAN_POINT('Ctrl Pts',(-13.2013205570211,36.1149222559032,22.5735644268251));
#50529=CARTESIAN_POINT('Ctrl Pts',(-13.190262087422,36.1461813115495,22.5717985181564));
#50530=CARTESIAN_POINT('Ctrl Pts',(-13.1787500907405,36.1772650182168,22.5700365663484));
#50531=CARTESIAN_POINT('Ctrl Pts',(-13.1787500671531,36.1772650819055,22.9104832616759));
#50532=CARTESIAN_POINT('Ctrl Pts',(-13.1790010362648,36.1765874366642,22.9105274219881));
#50533=CARTESIAN_POINT('Ctrl Pts',(-13.1792517886975,36.1759097111395,22.9105715923064));
#50534=CARTESIAN_POINT('Ctrl Pts',(-13.237959351312,36.017080776246,22.9209242746198));
#50535=CARTESIAN_POINT('Ctrl Pts',(-13.2845300025084,35.8548021059035,22.9317479373225));
#50536=CARTESIAN_POINT('Ctrl Pts',(-13.3479888675779,35.5494604665671,22.9518446707695));
#50537=CARTESIAN_POINT('Ctrl Pts',(-13.3682219563147,35.4074566325111,22.9610883679741));
#50538=CARTESIAN_POINT('Ctrl Pts',(-13.3862516561372,35.177179987411,22.9756973013826));
#50539=CARTESIAN_POINT('Ctrl Pts',(-13.3897019621106,35.0895291320123,22.981172033509));
#50540=CARTESIAN_POINT('Ctrl Pts',(-13.3897847495307,34.9368201348819,22.9905428193598));
#50541=CARTESIAN_POINT('Ctrl Pts',(-13.3879493868519,34.8718120078073,22.9944794268219));
#50542=CARTESIAN_POINT('Ctrl Pts',(-13.3823960459844,34.7744882129693,23.0002963219772));
#50543=CARTESIAN_POINT('Ctrl Pts',(-13.3800816063056,34.7421104449772,23.002218818337));
#50544=CARTESIAN_POINT('Ctrl Pts',(-13.3750412188899,34.6834572553323,23.0056796193798));
#50545=CARTESIAN_POINT('Ctrl Pts',(-13.3724725428528,34.6571712605943,23.0072226311836));
#50546=CARTESIAN_POINT('Ctrl Pts',(-13.3662351554364,34.6002260632992,23.0105491027415));
#50547=CARTESIAN_POINT('Ctrl Pts',(-13.3624541975311,34.5695813871893,23.0123289563566));
#50548=CARTESIAN_POINT('Ctrl Pts',(-13.3505367053427,34.4827673434493,23.0173448377495));
#50549=CARTESIAN_POINT('Ctrl Pts',(-13.3414073772441,34.4267434342593,23.020550214379));
#50550=CARTESIAN_POINT('Ctrl Pts',(-13.3173627889314,34.2994206011118,23.0277818538587));
#50551=CARTESIAN_POINT('Ctrl Pts',(-13.301547801169,34.2283197839812,23.0317815621783));
#50552=CARTESIAN_POINT('Ctrl Pts',(-13.2346136479775,33.9673721187257,23.0464065155067));
#50553=CARTESIAN_POINT('Ctrl Pts',(-13.1693041380711,33.7815755641973,23.0566891604838));
#50554=CARTESIAN_POINT('Ctrl Pts',(-13.0286977226376,33.470860464845,23.074882961935));
#50555=CARTESIAN_POINT('Ctrl Pts',(-12.960786560075,33.3431922308508,23.0826902191492));
#50556=CARTESIAN_POINT('Ctrl Pts',(-12.8700995584479,33.1961891904062,23.0925263426979));
#50557=CARTESIAN_POINT('Ctrl Pts',(-12.8549505523261,33.1723068788148,23.0941526470204));
#50558=CARTESIAN_POINT('Ctrl Pts',(-12.8304839003608,33.1347818451024,23.0967577600203));
#50559=CARTESIAN_POINT('Ctrl Pts',(-12.8213619693701,33.1210123767248,23.0977244916006));
#50560=CARTESIAN_POINT('Ctrl Pts',(-12.8035615170438,33.0945646355133,23.0996034230145));
#50561=CARTESIAN_POINT('Ctrl Pts',(-12.7948968514952,33.0818778288787,23.1005147662609));
#50562=CARTESIAN_POINT('Ctrl Pts',(-12.7731755057489,33.050533079188,23.1027906218577));
#50563=CARTESIAN_POINT('Ctrl Pts',(-12.7600165841288,33.0319471413214,23.1041616206865));
#50564=CARTESIAN_POINT('Ctrl Pts',(-12.707829826336,32.9597902875326,23.1095645912291));
#50565=CARTESIAN_POINT('Ctrl Pts',(-12.6674235593339,32.9072390443733,23.113674543376));
#50566=CARTESIAN_POINT('Ctrl Pts',(-12.550116570713,32.7635929584303,23.1253348666963));
#50567=CARTESIAN_POINT('Ctrl Pts',(-12.4699139823224,32.6753208039544,23.1330017892973));
#50568=CARTESIAN_POINT('Ctrl Pts',(-12.2084708573829,32.4164075385744,23.1567169592011));
#50569=CARTESIAN_POINT('Ctrl Pts',(-12.0129460402042,32.2613181029668,23.1726779604988));
#50570=CARTESIAN_POINT('Ctrl Pts',(-11.7591365899137,32.1019961142846,23.1908948273533));
#50571=CARTESIAN_POINT('Ctrl Pts',(-11.7154874732903,32.075946099827,23.1939506750723));
#50572=CARTESIAN_POINT('Ctrl Pts',(-11.6452074716319,32.0361183147008,23.1987521980932));
#50573=CARTESIAN_POINT('Ctrl Pts',(-11.6189525312298,32.0216959428165,23.2005203567485));
#50574=CARTESIAN_POINT('Ctrl Pts',(-11.5691104855404,31.9951705683002,23.2038301954978));
#50575=CARTESIAN_POINT('Ctrl Pts',(-11.5455660218386,31.9829926482725,23.2053743983222));
#50576=CARTESIAN_POINT('Ctrl Pts',(-11.4917133231471,31.9559342575447,23.2088639909069));
#50577=CARTESIAN_POINT('Ctrl Pts',(-11.4613205080669,31.9412277998095,23.2108033087802));
#50578=CARTESIAN_POINT('Ctrl Pts',(-11.3651288806111,31.8964437026354,23.2168516383603));
#50579=CARTESIAN_POINT('Ctrl Pts',(-11.29858204463,31.8680159256617,23.2209056636385));
#50580=CARTESIAN_POINT('Ctrl Pts',(-11.136151867512,31.804696400042,23.2305373551007));
#50581=CARTESIAN_POINT('Ctrl Pts',(-11.0395035859398,31.7719602944652,23.2360527903826));
#50582=CARTESIAN_POINT('Ctrl Pts',(-10.8954845330859,31.7303197202495,23.2440726517501));
#50583=CARTESIAN_POINT('Ctrl Pts',(-10.8491696145934,31.717986480605,23.2466226662982));
#50584=CARTESIAN_POINT('Ctrl Pts',(-10.5996093179044,31.657167400373,23.2602609581185));
#50585=CARTESIAN_POINT('Ctrl Pts',(-10.3924902656419,31.62657498258,23.2711961614971));
#50586=CARTESIAN_POINT('Ctrl Pts',(-10.1376220864304,31.6127278166058,23.285448443925));
#50587=CARTESIAN_POINT('Ctrl Pts',(-10.0913035027647,31.6111630426429,23.2880714943449));
#50588=CARTESIAN_POINT('Ctrl Pts',(-10.0263719791877,31.610301559026,23.2918124098229));
#50589=CARTESIAN_POINT('Ctrl Pts',(-10.0077729005632,31.610207889779,23.2928912982889));
#50590=CARTESIAN_POINT('Ctrl Pts',(-9.97407740020386,31.610315500748,23.2948606776596));
#50591=CARTESIAN_POINT('Ctrl Pts',(-9.9589810600504,31.6104645706882,23.2957484012477));
#50592=CARTESIAN_POINT('Ctrl Pts',(-9.92718124961997,31.6109910558264,23.2976305159197));
#50593=CARTESIAN_POINT('Ctrl Pts',(-9.91047896593155,31.6113911183827,23.2986260179514));
#50594=CARTESIAN_POINT('Ctrl Pts',(-9.86462320596399,31.612828734458,23.3013769920706));
#50595=CARTESIAN_POINT('Ctrl Pts',(-9.83547975630948,31.614119165717,23.3031451758726));
#50596=CARTESIAN_POINT('Ctrl Pts',(-9.6251088743864,31.6261564363506,23.3160347380531));
#50597=CARTESIAN_POINT('Ctrl Pts',(-9.44500128685725,31.6510704660152,23.3277302093005));
#50598=CARTESIAN_POINT('Ctrl Pts',(-9.03504994591969,31.7417662843148,23.3547950441538));
#50599=CARTESIAN_POINT('Ctrl Pts',(-8.80837231914258,31.8176625754771,23.3700577075697));
#50600=CARTESIAN_POINT('Ctrl Pts',(-8.54439843685343,31.938250187376,23.3877128278553));
#50601=CARTESIAN_POINT('Ctrl Pts',(-8.49778369292848,31.9608497182314,23.3908289163907));
#50602=CARTESIAN_POINT('Ctrl Pts',(-8.42487103274369,31.9982865615605,23.3957024282971));
#50603=CARTESIAN_POINT('Ctrl Pts',(-8.39822333882072,32.0124213071822,23.3974834926456));
#50604=CARTESIAN_POINT('Ctrl Pts',(-8.35086869849873,32.0383553973183,23.4006494198237));
#50605=CARTESIAN_POINT('Ctrl Pts',(-8.33009108193094,32.0500208390009,23.4020388292089));
#50606=CARTESIAN_POINT('Ctrl Pts',(-8.28159297876372,32.0779263524652,23.4052835299536));
#50607=CARTESIAN_POINT('Ctrl Pts',(-8.25397667995462,32.0943434890479,23.4071324037281));
#50608=CARTESIAN_POINT('Ctrl Pts',(-8.17271133678789,32.1442305518428,23.4125802022864));
#50609=CARTESIAN_POINT('Ctrl Pts',(-8.11975940755048,32.1788124816991,23.4161391612297));
#50610=CARTESIAN_POINT('Ctrl Pts',(-7.93675195973932,32.3057741395555,23.4285150176036));
#50611=CARTESIAN_POINT('Ctrl Pts',(-7.81227382540192,32.40583241055,23.4370614599859));
#50612=CARTESIAN_POINT('Ctrl Pts',(-7.54770180353582,32.6511383752549,23.4562265243886));
#50613=CARTESIAN_POINT('Ctrl Pts',(-7.41259936293109,32.8008496255516,23.4667596128032));
#50614=CARTESIAN_POINT('Ctrl Pts',(-7.25827255709008,33.0059075604897,23.4809902501718));
#50615=CARTESIAN_POINT('Ctrl Pts',(-7.22605193391819,33.0509783340861,23.4841086724474));
#50616=CARTESIAN_POINT('Ctrl Pts',(-7.18264621140156,33.1149527645479,23.4885522307905));
#50617=CARTESIAN_POINT('Ctrl Pts',(-7.17051698050485,33.1332083035395,23.4898221336829));
#50618=CARTESIAN_POINT('Ctrl Pts',(-7.15027025870247,33.1643320273062,23.4919926734218));
#50619=CARTESIAN_POINT('Ctrl Pts',(-7.14206061492794,33.1771398928868,23.4928874607243));
#50620=CARTESIAN_POINT('Ctrl Pts',(-7.12494242745946,33.2042458972411,23.4947852347788));
#50621=CARTESIAN_POINT('Ctrl Pts',(-7.11605392912648,33.2185556767856,23.4957893461617));
#50622=CARTESIAN_POINT('Ctrl Pts',(-7.09172521015697,33.2583822717003,23.4985888414825));
#50623=CARTESIAN_POINT('Ctrl Pts',(-7.07651489579452,33.284036923941,23.5003976516913));
#50624=CARTESIAN_POINT('Ctrl Pts',(-7.04270596196799,33.3428156470571,23.5045485258767));
#50625=CARTESIAN_POINT('Ctrl Pts',(-7.02432182693637,33.3760581310844,23.506900737016));
#50626=CARTESIAN_POINT('Ctrl Pts',(-6.96473670443895,33.4882111376033,23.5148353098581));
#50627=CARTESIAN_POINT('Ctrl Pts',(-6.92608723196081,33.5684318075203,23.5205078409061));
#50628=CARTESIAN_POINT('Ctrl Pts',(-6.77279864837253,33.9215102555887,23.5452157101113));
#50629=CARTESIAN_POINT('Ctrl Pts',(-6.69098154746527,34.2072672839233,23.5644121033627));
#50630=CARTESIAN_POINT('Ctrl Pts',(-6.63992642826559,34.549638822686,23.585434055818));
#50631=CARTESIAN_POINT('Ctrl Pts',(-6.63363163752506,34.599395396823,23.58844645004));
#50632=CARTESIAN_POINT('Ctrl Pts',(-6.62538676749286,34.6786543079254,23.593179361793));
#50633=CARTESIAN_POINT('Ctrl Pts',(-6.62271470197707,34.7080725753672,23.5949218003576));
#50634=CARTESIAN_POINT('Ctrl Pts',(-6.61836888853687,34.7640278650643,23.5982099887422));
#50635=CARTESIAN_POINT('Ctrl Pts',(-6.61662218436591,34.7905568372708,23.5997578687227));
#50636=CARTESIAN_POINT('Ctrl Pts',(-6.6133266858152,34.8515458972155,23.6032921769436));
#50637=CARTESIAN_POINT('Ctrl Pts',(-6.61199140036092,34.8860148651668,23.6052719137775));
#50638=CARTESIAN_POINT('Ctrl Pts',(-6.60938345397695,34.9971816450453,23.611604554602));
#50639=CARTESIAN_POINT('Ctrl Pts',(-6.61018768586979,35.0739065300959,23.6158944818222));
#50640=CARTESIAN_POINT('Ctrl Pts',(-6.61852832529547,35.2615268822037,23.626244239358));
#50641=CARTESIAN_POINT('Ctrl Pts',(-6.62891537096276,35.3722064551309,23.6322275374187));
#50642=CARTESIAN_POINT('Ctrl Pts',(-6.67578277287569,35.6983356425664,23.6497991201291));
#50643=CARTESIAN_POINT('Ctrl Pts',(-6.72765817888526,35.9109655475504,23.6611563387769));
#50644=CARTESIAN_POINT('Ctrl Pts',(-6.82059014850658,36.1772039111982,23.6767013508439));
#50645=CARTESIAN_POINT('Ctrl Pts',(-6.84325253315092,36.2366893158103,23.6802668779848));
#50646=CARTESIAN_POINT('Ctrl Pts',(-6.87640281495692,36.3168444539819,23.6852428101942));
#50647=CARTESIAN_POINT('Ctrl Pts',(-6.88544906112173,36.3380998006529,23.6865790925589));
#50648=CARTESIAN_POINT('Ctrl Pts',(-6.90083553885204,36.373250866194,23.6888195826673));
#50649=CARTESIAN_POINT('Ctrl Pts',(-6.90705391012291,36.3871996162766,23.6897167607591));
#50650=CARTESIAN_POINT('Ctrl Pts',(-6.92012699800989,36.4159996070253,23.6915868804811));
#50651=CARTESIAN_POINT('Ctrl Pts',(-6.92699525970748,36.4308439597377,23.6925605551736));
#50652=CARTESIAN_POINT('Ctrl Pts',(-6.9457129090319,36.4705419181782,23.6951895581798));
#50653=CARTESIAN_POINT('Ctrl Pts',(-6.95775788990161,36.4953013092134,23.6968558729484));
#50654=CARTESIAN_POINT('Ctrl Pts',(-7.02841392737375,36.6361520751646,23.7064769317425));
#50655=CARTESIAN_POINT('Ctrl Pts',(-7.0933612405727,36.74893177814,23.7147327644));
#50656=CARTESIAN_POINT('Ctrl Pts',(-7.32786337109546,37.1068508177878,23.7421945215145));
#50657=CARTESIAN_POINT('Ctrl Pts',(-7.52327651724279,37.3334601426814,23.7615235411329));
#50658=CARTESIAN_POINT('Ctrl Pts',(-7.7829469991365,37.5646739473172,23.7826314286395));
#50659=CARTESIAN_POINT('Ctrl Pts',(-7.82079914019173,37.5969136430714,23.7856170967689));
#50660=CARTESIAN_POINT('Ctrl Pts',(-7.8821818061923,37.6469073226659,23.7903182818475));
#50661=CARTESIAN_POINT('Ctrl Pts',(-7.90525717897291,37.6652063470725,23.7920552158234));
#50662=CARTESIAN_POINT('Ctrl Pts',(-7.94962858653411,37.6994610539502,23.795338973765));
#50663=CARTESIAN_POINT('Ctrl Pts',(-7.9708796360039,37.7154711419472,23.7968878418707));
#50664=CARTESIAN_POINT('Ctrl Pts',(-8.02024647532204,37.7517599030373,23.800432742459));
#50665=CARTESIAN_POINT('Ctrl Pts',(-8.0484894770182,37.7718609971389,23.8024219380572));
#50666=CARTESIAN_POINT('Ctrl Pts',(-8.14106819544522,37.8356345368181,23.8088227462943));
#50667=CARTESIAN_POINT('Ctrl Pts',(-8.20660133201395,37.877528998706,23.8131693798985));
#50668=CARTESIAN_POINT('Ctrl Pts',(-8.37107695936773,37.9748723647408,23.8236957393256));
#50669=CARTESIAN_POINT('Ctrl Pts',(-8.47147183575167,38.027682251715,23.8297951377052));
#50670=CARTESIAN_POINT('Ctrl Pts',(-8.78507571381331,38.1730621215018,23.8482176561924));
#50671=CARTESIAN_POINT('Ctrl Pts',(-9.00528612859248,38.248828864041,23.8602789028901));
#50672=CARTESIAN_POINT('Ctrl Pts',(-9.28041509113971,38.3128728074358,23.8760028044217));
#50673=CARTESIAN_POINT('Ctrl Pts',(-9.32958717842764,38.3231723987147,23.8788392182005));
#50674=CARTESIAN_POINT('Ctrl Pts',(-9.39983482402353,38.3362639888771,23.8829513012432));
#50675=CARTESIAN_POINT('Ctrl Pts',(-9.42073788771664,38.3399567358594,23.8841824021774));
#50676=CARTESIAN_POINT('Ctrl Pts',(-9.45657338143525,38.3459409386346,23.8863078733471));
#50677=CARTESIAN_POINT('Ctrl Pts',(-9.47148878515081,38.348329306437,23.8871969790942));
#50678=CARTESIAN_POINT('Ctrl Pts',(-9.50338598360247,38.3532184808963,23.8891085218536));
#50679=CARTESIAN_POINT('Ctrl Pts',(-9.52037084487927,38.3556900195747,23.8901323806456));
#50680=CARTESIAN_POINT('Ctrl Pts',(-9.56841966752616,38.3623095705297,23.8930442927407));
#50681=CARTESIAN_POINT('Ctrl Pts',(-9.59952264710387,38.3661558148426,23.8949474910764));
#50682=CARTESIAN_POINT('Ctrl Pts',(-9.81157920205511,38.3893985893415,23.908027323243));
#50683=CARTESIAN_POINT('Ctrl Pts',(-9.99377378532583,38.3946245500903,23.9197636325374));
#50684=CARTESIAN_POINT('Ctrl Pts',(-10.4086339630798,38.3731180695714,23.9465417353679));
#50685=CARTESIAN_POINT('Ctrl Pts',(-10.6399393699847,38.3369769890681,23.9614767965651));
#50686=CARTESIAN_POINT('Ctrl Pts',(-10.9161280140314,38.264020993372,23.9788596037172));
#50687=CARTESIAN_POINT('Ctrl Pts',(-10.966226371067,38.2495431424341,23.9819970189684));
#50688=CARTESIAN_POINT('Ctrl Pts',(-11.0448189971437,38.2248523292749,23.986895993547));
#50689=CARTESIAN_POINT('Ctrl Pts',(-11.0735431648861,38.2154042427478,23.988681609264));
#50690=CARTESIAN_POINT('Ctrl Pts',(-11.1269277328669,38.1970495984058,23.9919921397577));
#50691=CARTESIAN_POINT('Ctrl Pts',(-11.1516184652904,38.1882388895907,23.9935200190865));
#50692=CARTESIAN_POINT('Ctrl Pts',(-11.2073334278124,38.1676257148147,23.9969614169578));
#50693=CARTESIAN_POINT('Ctrl Pts',(-11.2382917465465,38.1556521254748,23.9988691756973));
#50694=CARTESIAN_POINT('Ctrl Pts',(-11.3331159425852,38.1173670753526,24.0047027745979));
#50695=CARTESIAN_POINT('Ctrl Pts',(-11.3963592499947,38.0895561717351,24.0085792840567));
#50696=CARTESIAN_POINT('Ctrl Pts',(-11.5448704951598,38.0187564736,24.0176868664591));
#50697=CARTESIAN_POINT('Ctrl Pts',(-11.6292594306088,37.9740596565543,24.0228650414919));
#50698=CARTESIAN_POINT('Ctrl Pts',(-11.8271671203197,37.8582819067838,24.0351629231767));
#50699=CARTESIAN_POINT('Ctrl Pts',(-11.9385790619074,37.7839229222697,24.042212872294));
#50700=CARTESIAN_POINT('Ctrl Pts',(-12.1661883104333,37.6117068324503,24.0573869994672));
#50701=CARTESIAN_POINT('Ctrl Pts',(-12.2807913119895,37.5122433523538,24.0655129903433));
#50702=CARTESIAN_POINT('Ctrl Pts',(-12.4139150553755,37.380066759976,24.0761010639822));
#50703=CARTESIAN_POINT('Ctrl Pts',(-12.4390797937873,37.3542712713051,24.0781587346993));
#50704=CARTESIAN_POINT('Ctrl Pts',(-12.4762666280471,37.314916129411,24.081294177059));
#50705=CARTESIAN_POINT('Ctrl Pts',(-12.4885997937082,37.3016524789963,24.0823502595232));
#50706=CARTESIAN_POINT('Ctrl Pts',(-12.5108121476394,37.27737705764,24.0842833595824));
#50707=CARTESIAN_POINT('Ctrl Pts',(-12.5207263914183,37.2663985391161,24.0851577916669));
#50708=CARTESIAN_POINT('Ctrl Pts',(-12.5436136882859,37.2407183868211,24.0872035185065));
#50709=CARTESIAN_POINT('Ctrl Pts',(-12.5565313253448,37.2259687837473,24.0883786099033));
#50710=CARTESIAN_POINT('Ctrl Pts',(-12.5981561094729,37.1776005579619,24.0922300490401));
#50711=CARTESIAN_POINT('Ctrl Pts',(-12.6263326172292,37.1435335195029,24.0949395467786));
#50712=CARTESIAN_POINT('Ctrl Pts',(-12.6940406788553,37.0583309904781,24.1016884379336));
#50713=CARTESIAN_POINT('Ctrl Pts',(-12.7327908405863,37.0065978751163,24.1057624498016));
#50714=CARTESIAN_POINT('Ctrl Pts',(-12.9150806390208,36.7481519840138,24.1258881737976));
#50715=CARTESIAN_POINT('Ctrl Pts',(-13.0367913981084,36.5269734099696,24.1423473991613));
#50716=CARTESIAN_POINT('Ctrl Pts',(-13.1489048712689,36.2556117805636,24.1607545473902));
#50717=CARTESIAN_POINT('Ctrl Pts',(-13.1641921164709,36.2165732090061,24.1633644668778));
#50718=CARTESIAN_POINT('Ctrl Pts',(-13.178750056895,36.1772651096035,24.1659535227378));
#50719=CARTESIAN_POINT('Origin',(-10.,35.,23.));
#50720=CARTESIAN_POINT('',(-13.1787500473324,36.1772651354237,25.4139790685233));
#50721=CARTESIAN_POINT('',(-13.1787500684596,36.1772650783778,25.0733222522952));
#50722=CARTESIAN_POINT('',(-13.1787500671536,36.1772650819043,23.));
#50723=CARTESIAN_POINT('Ctrl Pts',(-13.1787500684596,36.1772650783778,25.0733222522952));
#50724=CARTESIAN_POINT('Ctrl Pts',(-13.1307659665353,36.3068276298187,25.064834390241));
#50725=CARTESIAN_POINT('Ctrl Pts',(-13.0749065290861,36.4333323936619,25.0560136504007));
#50726=CARTESIAN_POINT('Ctrl Pts',(-12.8969145979482,36.7778027413596,25.0310689985252));
#50727=CARTESIAN_POINT('Ctrl Pts',(-12.7581866467696,36.9862364570538,25.0149288008823));
#50728=CARTESIAN_POINT('Ctrl Pts',(-12.5543852563375,37.2293701933785,24.9954297643669));
#50729=CARTESIAN_POINT('Ctrl Pts',(-12.5094137971869,37.2798725539082,24.9913315841711));
#50730=CARTESIAN_POINT('Ctrl Pts',(-12.4403347371283,37.3529249384142,24.985328245993));
#50731=CARTESIAN_POINT('Ctrl Pts',(-12.4173620284244,37.376520636002,24.9833767580414));
#50732=CARTESIAN_POINT('Ctrl Pts',(-12.3753325337511,37.418449776571,24.9798850971513));
#50733=CARTESIAN_POINT('Ctrl Pts',(-12.3563983875437,37.4369018580045,24.9783398202262));
#50734=CARTESIAN_POINT('Ctrl Pts',(-12.3151515604359,37.4761682535823,24.9750314798694));
#50735=CARTESIAN_POINT('Ctrl Pts',(-12.2927696955729,37.4969067220169,24.973271698899));
#50736=CARTESIAN_POINT('Ctrl Pts',(-12.2304337736215,37.553120575905,24.9684641070128));
#50737=CARTESIAN_POINT('Ctrl Pts',(-12.189915463833,37.5879586914813,24.9654423232322));
#50738=CARTESIAN_POINT('Ctrl Pts',(-11.9992991484955,37.7441689558281,24.9516606629629));
#50739=CARTESIAN_POINT('Ctrl Pts',(-11.8398284350779,37.853541832687,24.9413606289992));
#50740=CARTESIAN_POINT('Ctrl Pts',(-11.5357026069175,38.0259769091778,24.9228168968916));
#50741=CARTESIAN_POINT('Ctrl Pts',(-11.3943239200313,38.0936668160623,24.9145663846892));
#50742=CARTESIAN_POINT('Ctrl Pts',(-11.1769089501328,38.1798219152437,24.9017726056846));
#50743=CARTESIAN_POINT('Ctrl Pts',(-11.104086921635,38.2058341240274,24.8974689607672));
#50744=CARTESIAN_POINT('Ctrl Pts',(-11.0075998701456,38.2366220979135,24.8916668246521));
#50745=CARTESIAN_POINT('Ctrl Pts',(-10.9846786870032,38.2436688974761,24.8902812101687));
#50746=CARTESIAN_POINT('Ctrl Pts',(-10.9467279707565,38.2548970059149,24.8879721549258));
#50747=CARTESIAN_POINT('Ctrl Pts',(-10.9317404144614,38.2592189489255,24.8870564508939));
#50748=CARTESIAN_POINT('Ctrl Pts',(-10.9030914715806,38.2672666496007,24.8852979081742));
#50749=CARTESIAN_POINT('Ctrl Pts',(-10.8894356113586,38.2710105231959,24.8844562004594));
#50750=CARTESIAN_POINT('Ctrl Pts',(-10.852049907661,38.2810087227404,24.8821431294106));
#50751=CARTESIAN_POINT('Ctrl Pts',(-10.8282754354986,38.287090964748,24.8806626214447));
#50752=CARTESIAN_POINT('Ctrl Pts',(-10.7306792828961,38.3109330769719,24.8745517855972));
#50753=CARTESIAN_POINT('Ctrl Pts',(-10.656341284176,38.3264672717401,24.8698200864907));
#50754=CARTESIAN_POINT('Ctrl Pts',(-10.3781507279653,38.3749123085134,24.8519748735418));
#50755=CARTESIAN_POINT('Ctrl Pts',(-10.1719425600578,38.3916763004284,24.8385046514535));
#50756=CARTESIAN_POINT('Ctrl Pts',(-9.80218809235398,38.3879116881612,24.8149018098583));
#50757=CARTESIAN_POINT('Ctrl Pts',(-9.63920413326415,38.374450116284,24.8046838239203));
#50758=CARTESIAN_POINT('Ctrl Pts',(-9.43483469850828,38.3425865386903,24.7921923868279));
#50759=CARTESIAN_POINT('Ctrl Pts',(-9.39199372105874,38.3350600017291,24.7895909629063));
#50760=CARTESIAN_POINT('Ctrl Pts',(-9.32166326175944,38.3213036289955,24.7853468304464));
#50761=CARTESIAN_POINT('Ctrl Pts',(-9.29408649567778,38.315551948378,24.7836894525287));
#50762=CARTESIAN_POINT('Ctrl Pts',(-9.24041235176783,38.3036571040734,24.7804758483898));
#50763=CARTESIAN_POINT('Ctrl Pts',(-9.21430990540812,38.2975467839535,24.7789187235205));
#50764=CARTESIAN_POINT('Ctrl Pts',(-9.15160397585775,38.2820811034703,24.7751904030704));
#50765=CARTESIAN_POINT('Ctrl Pts',(-9.11507863307438,38.2724221181932,24.7730289487159));
#50766=CARTESIAN_POINT('Ctrl Pts',(-8.98990788496932,38.2370721218985,24.7656499730415));
#50767=CARTESIAN_POINT('Ctrl Pts',(-8.90215147728608,38.2083722635716,24.7605270737406));
#50768=CARTESIAN_POINT('Ctrl Pts',(-8.56589816880191,38.082988402781,24.7409263409843));
#50769=CARTESIAN_POINT('Ctrl Pts',(-8.32800097456888,37.9607221207794,24.7271956836636));
#50770=CARTESIAN_POINT('Ctrl Pts',(-8.05223278435334,37.7750584524099,24.7091890787451));
#50771=CARTESIAN_POINT('Ctrl Pts',(-7.99866315804326,37.7366761811603,24.7055762790202));
#50772=CARTESIAN_POINT('Ctrl Pts',(-7.91059169059765,37.6696042425872,24.699380413987));
#50773=CARTESIAN_POINT('Ctrl Pts',(-7.87547837994948,37.6417458971431,24.6968380021484));
#50774=CARTESIAN_POINT('Ctrl Pts',(-7.82573407681131,37.6006463193765,24.6931142062832));
#50775=CARTESIAN_POINT('Ctrl Pts',(-7.81064886358121,37.5879596488668,24.6919682831208));
#50776=CARTESIAN_POINT('Ctrl Pts',(-7.78432814066581,37.5654290845402,24.6899376440576));
#50777=CARTESIAN_POINT('Ctrl Pts',(-7.77304572412354,37.5556413709203,24.6890568556549));
#50778=CARTESIAN_POINT('Ctrl Pts',(-7.74823554114634,37.5338290085789,24.6870966113779));
#50779=CARTESIAN_POINT('Ctrl Pts',(-7.73473931850067,37.5217705358107,24.6860148294879));
#50780=CARTESIAN_POINT('Ctrl Pts',(-7.69471106539412,37.4854258687375,24.6827616386347));
#50781=CARTESIAN_POINT('Ctrl Pts',(-7.66846914396718,37.4608255659265,24.6805693092405));
#50782=CARTESIAN_POINT('Ctrl Pts',(-7.53435401944144,37.3310292268565,24.6690741202448));
#50783=CARTESIAN_POINT('Ctrl Pts',(-7.43319833019352,37.2191506102405,24.6594126680355));
#50784=CARTESIAN_POINT('Ctrl Pts',(-7.25824653656227,36.9976283101894,24.6412277388753));
#50785=CARTESIAN_POINT('Ctrl Pts',(-7.18274818527904,36.8896628136849,24.6327288820794));
#50786=CARTESIAN_POINT('Ctrl Pts',(-7.0374692814943,36.6537710593604,24.615127176128));
#50787=CARTESIAN_POINT('Ctrl Pts',(-6.96925844379516,36.5251758384331,24.6060742301639));
#50788=CARTESIAN_POINT('Ctrl Pts',(-6.89212047061677,36.3539874192748,24.5947466750237));
#50789=CARTESIAN_POINT('Ctrl Pts',(-6.87545333140142,36.3150686141046,24.5922167013959));
#50790=CARTESIAN_POINT('Ctrl Pts',(-6.8490047142653,36.2499656544263,24.5880574786862));
#50791=CARTESIAN_POINT('Ctrl Pts',(-6.838810531346,36.2239553263872,24.5864147150729));
#50792=CARTESIAN_POINT('Ctrl Pts',(-6.81941333302961,36.1726040106012,24.5832075458548));
#50793=CARTESIAN_POINT('Ctrl Pts',(-6.81018880495963,36.1472734256455,24.5816425293851));
#50794=CARTESIAN_POINT('Ctrl Pts',(-6.7904975800991,36.0911270500908,24.5782096847999));
#50795=CARTESIAN_POINT('Ctrl Pts',(-6.78017044304921,36.0602649436259,24.5763464755342));
#50796=CARTESIAN_POINT('Ctrl Pts',(-6.74579996919094,35.9524137721716,24.5699128281044));
#50797=CARTESIAN_POINT('Ctrl Pts',(-6.72406007349754,35.8747164062729,24.5654150091625));
#50798=CARTESIAN_POINT('Ctrl Pts',(-6.63921363116226,35.5236489979135,24.5455744501793));
#50799=CARTESIAN_POINT('Ctrl Pts',(-6.60741895386023,35.243880156947,24.5311526757082));
#50800=CARTESIAN_POINT('Ctrl Pts',(-6.61117049327251,34.8964530030295,24.512346249462));
#50801=CARTESIAN_POINT('Ctrl Pts',(-6.61387656327999,34.8295459633342,24.5086778690344));
#50802=CARTESIAN_POINT('Ctrl Pts',(-6.62173408140458,34.7175478064566,24.5023969392579));
#50803=CARTESIAN_POINT('Ctrl Pts',(-6.6258130805747,34.6723995079999,24.4998265116199));
#50804=CARTESIAN_POINT('Ctrl Pts',(-6.6329722735689,34.6076719882143,24.4960689756137));
#50805=CARTESIAN_POINT('Ctrl Pts',(-6.6353209161597,34.5880150474372,24.4949182216722));
#50806=CARTESIAN_POINT('Ctrl Pts',(-6.6397442826629,34.553558649893,24.4928824052194));
#50807=CARTESIAN_POINT('Ctrl Pts',(-6.64174489819024,34.5387505834577,24.4920013462472));
#50808=CARTESIAN_POINT('Ctrl Pts',(-6.64637609662239,34.5061001997566,24.4900447548531));
#50809=CARTESIAN_POINT('Ctrl Pts',(-6.6490511581528,34.4882655716222,24.4889669568071));
#50810=CARTESIAN_POINT('Ctrl Pts',(-6.65743603863847,34.4352509858389,24.4857378774868));
#50811=CARTESIAN_POINT('Ctrl Pts',(-6.66355835072107,34.4001398588864,24.4835661119076));
#50812=CARTESIAN_POINT('Ctrl Pts',(-6.69730641142036,34.2231370476805,24.4724713568811));
#50813=CARTESIAN_POINT('Ctrl Pts',(-6.73343327716103,34.0830287871982,24.4632175107088));
#50814=CARTESIAN_POINT('Ctrl Pts',(-6.81690276305331,33.8279801492812,24.445936833305));
#50815=CARTESIAN_POINT('Ctrl Pts',(-6.86183874362242,33.7124891902504,24.4379359133095));
#50816=CARTESIAN_POINT('Ctrl Pts',(-6.95660901619957,33.5035630070515,24.4233106537873));
#50817=CARTESIAN_POINT('Ctrl Pts',(-7.00469479561024,33.4094962923371,24.4166641890884));
#50818=CARTESIAN_POINT('Ctrl Pts',(-7.09386509502281,33.2534964684357,24.4055779659803));
#50819=CARTESIAN_POINT('Ctrl Pts',(-7.13273453349769,33.1903910131828,24.4010737232964));
#50820=CARTESIAN_POINT('Ctrl Pts',(-7.19244624234888,33.1002087130594,24.3946060018994));
#50821=CARTESIAN_POINT('Ctrl Pts',(-7.21167640617214,33.0720952567253,24.3925850801741));
#50822=CARTESIAN_POINT('Ctrl Pts',(-7.24663772007443,33.0226013572735,24.3890176030153));
#50823=CARTESIAN_POINT('Ctrl Pts',(-7.26220218565181,33.0011072004863,24.3874649942433));
#50824=CARTESIAN_POINT('Ctrl Pts',(-7.29576401053198,32.9558866379838,24.3841903847806));
#50825=CARTESIAN_POINT('Ctrl Pts',(-7.31382492081051,32.9322100568245,24.382470992412));
#50826=CARTESIAN_POINT('Ctrl Pts',(-7.36385105411483,32.8683910711449,24.3778206556649));
#50827=CARTESIAN_POINT('Ctrl Pts',(-7.39642012803601,32.8287307562785,24.3749133950319));
#50828=CARTESIAN_POINT('Ctrl Pts',(-7.59276946009868,32.600404329679,24.3580376394101));
#50829=CARTESIAN_POINT('Ctrl Pts',(-7.77609952918974,32.4295727911918,24.3449135142832));
#50830=CARTESIAN_POINT('Ctrl Pts',(-8.11316344057911,32.1787861934753,24.3226016356645));
#50831=CARTESIAN_POINT('Ctrl Pts',(-8.2572263576797,32.0875908660576,24.313500107718));
#50832=CARTESIAN_POINT('Ctrl Pts',(-8.43415976623623,31.9934304034561,24.3021134264023));
#50833=CARTESIAN_POINT('Ctrl Pts',(-8.4609962638033,31.9796053662315,24.3003807724348));
#50834=CARTESIAN_POINT('Ctrl Pts',(-8.50315869420564,31.9585928353277,24.2976444958469));
#50835=CARTESIAN_POINT('Ctrl Pts',(-8.51836052225759,31.9511582744559,24.2966550937034));
#50836=CARTESIAN_POINT('Ctrl Pts',(-8.54730742930555,31.9372692031222,24.2947645765025));
#50837=CARTESIAN_POINT('Ctrl Pts',(-8.56104115305781,31.930792766629,24.2938647649355));
#50838=CARTESIAN_POINT('Ctrl Pts',(-8.59454285991083,31.9152685814993,24.2916634499116));
#50839=CARTESIAN_POINT('Ctrl Pts',(-8.61435507503563,31.9063184093079,24.2903563731094));
#50840=CARTESIAN_POINT('Ctrl Pts',(-8.68394411310862,31.8756840957899,24.285750508426));
#50841=CARTESIAN_POINT('Ctrl Pts',(-8.73415241136013,31.8550068100978,24.2824011031133));
#50842=CARTESIAN_POINT('Ctrl Pts',(-8.97360946777982,31.7630540204179,24.26637388975));
#50843=CARTESIAN_POINT('Ctrl Pts',(-9.16848723102129,31.7076028752931,24.2532037402413));
#50844=CARTESIAN_POINT('Ctrl Pts',(-9.55640992597417,31.6338819656676,24.2278574991085));
#50845=CARTESIAN_POINT('Ctrl Pts',(-9.74842605747257,31.6141098051895,24.2157107681617));
#50846=CARTESIAN_POINT('Ctrl Pts',(-9.9858867655,31.6099835110576,24.201351341659));
#50847=CARTESIAN_POINT('Ctrl Pts',(-10.0306799890562,31.6100929209268,24.198669995993));
#50848=CARTESIAN_POINT('Ctrl Pts',(-10.1038852804712,31.6117229550522,24.1943307772204));
#50849=CARTESIAN_POINT('Ctrl Pts',(-10.1323025345119,31.6127135347298,24.192656906725));
#50850=CARTESIAN_POINT('Ctrl Pts',(-10.1876405912292,31.6153400094382,24.1894168859055));
#50851=CARTESIAN_POINT('Ctrl Pts',(-10.214560890434,31.6169398573052,24.1878497526763));
#50852=CARTESIAN_POINT('Ctrl Pts',(-10.2784989357181,31.6215059126574,24.1841477910255));
#50853=CARTESIAN_POINT('Ctrl Pts',(-10.3154930659426,31.6247595293507,24.1820219388386));
#50854=CARTESIAN_POINT('Ctrl Pts',(-10.4405514020079,31.6378325089201,24.1748833829223));
#50855=CARTESIAN_POINT('Ctrl Pts',(-10.5282846130177,31.6504966188538,24.1699571137163));
#50856=CARTESIAN_POINT('Ctrl Pts',(-10.8821332536775,31.7158253221721,24.1502669074199));
#50857=CARTESIAN_POINT('Ctrl Pts',(-11.1419485056802,31.7968911083043,24.1363061019223));
#50858=CARTESIAN_POINT('Ctrl Pts',(-11.4497556915204,31.9351993029143,24.1180325298672));
#50859=CARTESIAN_POINT('Ctrl Pts',(-11.5093786412316,31.9641195480346,24.114400552371));
#50860=CARTESIAN_POINT('Ctrl Pts',(-11.6080048980004,32.015582137231,24.1081753158729));
#50861=CARTESIAN_POINT('Ctrl Pts',(-11.6474766874405,32.0371888525677,24.1056232141005));
#50862=CARTESIAN_POINT('Ctrl Pts',(-11.7036287547125,32.069395314039,24.1018877452565));
#50863=CARTESIAN_POINT('Ctrl Pts',(-11.7206662167474,32.0793660809494,24.1007401468952));
#50864=CARTESIAN_POINT('Ctrl Pts',(-11.7504422374339,32.0971427500939,24.0987077157912));
#50865=CARTESIAN_POINT('Ctrl Pts',(-11.7632177909871,32.1048849333368,24.0978268369253));
#50866=CARTESIAN_POINT('Ctrl Pts',(-11.7913388541426,32.1221819170472,24.0958678741783));
#50867=CARTESIAN_POINT('Ctrl Pts',(-11.8066591878827,32.1317750514576,24.094787485375));
#50868=CARTESIAN_POINT('Ctrl Pts',(-11.8512086648229,32.1601691334563,24.0916089328252));
#50869=CARTESIAN_POINT('Ctrl Pts',(-11.8802254548769,32.1792970896094,24.0894916840431));
#50870=CARTESIAN_POINT('Ctrl Pts',(-12.0617399108782,32.3029972225237,24.0759728494951));
#50871=CARTESIAN_POINT('Ctrl Pts',(-12.2057505547567,32.4194477007096,24.0640230841181));
#50872=CARTESIAN_POINT('Ctrl Pts',(-12.4547290570156,32.6569143889609,24.0418481997046));
#50873=CARTESIAN_POINT('Ctrl Pts',(-12.5620477518626,32.7747665669644,24.0316393548772));
#50874=CARTESIAN_POINT('Ctrl Pts',(-12.7202811607275,32.9752222657937,24.0157044531034));
#50875=CARTESIAN_POINT('Ctrl Pts',(-12.7766340598312,33.0532179199692,24.0098078003098));
#50876=CARTESIAN_POINT('Ctrl Pts',(-12.8501732572456,33.1647033509829,24.001790508696));
#50877=CARTESIAN_POINT('Ctrl Pts',(-12.8702321752451,33.1962348229104,23.9995661478259));
#50878=CARTESIAN_POINT('Ctrl Pts',(-12.903882554509,33.2511145105134,23.9957668848981));
#50879=CARTESIAN_POINT('Ctrl Pts',(-12.9177235470911,33.2743048614257,23.994183087062));
#50880=CARTESIAN_POINT('Ctrl Pts',(-12.9455273948703,33.3221807098169,23.9909564505232));
#50881=CARTESIAN_POINT('Ctrl Pts',(-12.9594605809514,33.3468810250783,23.9893147539574));
#50882=CARTESIAN_POINT('Ctrl Pts',(-12.9944190202137,33.4107130952642,23.9851289293572));
#50883=CARTESIAN_POINT('Ctrl Pts',(-13.01498835829,33.4500891668177,23.9826007466813));
#50884=CARTESIAN_POINT('Ctrl Pts',(-13.109637786221,33.6402966663951,23.9706260368517));
#50885=CARTESIAN_POINT('Ctrl Pts',(-13.1732114456117,33.7960989146199,23.9615368528855));
#50886=CARTESIAN_POINT('Ctrl Pts',(-13.2835713952204,34.1370027642995,23.9424376319687));
#50887=CARTESIAN_POINT('Ctrl Pts',(-13.3268235370846,34.3226200225679,23.9324995132982));
#50888=CARTESIAN_POINT('Ctrl Pts',(-13.3665599552516,34.5951205098924,23.9174973927582));
#50889=CARTESIAN_POINT('Ctrl Pts',(-13.3756656442352,34.6797929363055,23.9127763696353));
#50890=CARTESIAN_POINT('Ctrl Pts',(-13.3832899180907,34.7893691713031,23.9064907039485));
#50891=CARTESIAN_POINT('Ctrl Pts',(-13.3847357966339,34.8140442882095,23.9050637577592));
#50892=CARTESIAN_POINT('Ctrl Pts',(-13.3866610208941,34.8544655043237,23.9027042457129));
#50893=CARTESIAN_POINT('Ctrl Pts',(-13.3873006974258,34.8702035171999,23.901780119111));
#50894=CARTESIAN_POINT('Ctrl Pts',(-13.3883026537344,34.8999651424344,23.900021288718));
#50895=CARTESIAN_POINT('Ctrl Pts',(-13.3886876087989,34.9139876731016,23.8991878951735));
#50896=CARTESIAN_POINT('Ctrl Pts',(-13.3894915959102,34.9518369977503,23.896926466669));
#50897=CARTESIAN_POINT('Ctrl Pts',(-13.389746412554,34.97566603434,23.8954899494278));
#50898=CARTESIAN_POINT('Ctrl Pts',(-13.3897612597053,35.0753306280261,23.8894337867824));
#50899=CARTESIAN_POINT('Ctrl Pts',(-13.387227647782,35.151139962788,23.8847114418519));
#50900=CARTESIAN_POINT('Ctrl Pts',(-13.3720525334123,35.3774441921629,23.8703858501299));
#50901=CARTESIAN_POINT('Ctrl Pts',(-13.3518967387176,35.5272458346233,23.8606069283636));
#50902=CARTESIAN_POINT('Ctrl Pts',(-13.2871051319953,35.8460051064849,23.8396685724383));
#50903=CARTESIAN_POINT('Ctrl Pts',(-13.2392693847419,36.0138560049049,23.8285688711194));
#50904=CARTESIAN_POINT('Ctrl Pts',(-13.1787500981843,36.1772649981177,23.8178418924018));
#50905=CARTESIAN_POINT('',(-13.3897487153608,34.997048862956,24.2344129021999));
#50906=CARTESIAN_POINT('Ctrl Pts',(-13.178750056895,36.1772651096035,24.1659535227378));
#50907=CARTESIAN_POINT('Ctrl Pts',(-13.2007132313444,36.1179620338044,24.1698595619065));
#50908=CARTESIAN_POINT('Ctrl Pts',(-13.2210164453761,36.0580454759536,24.1737179086272));
#50909=CARTESIAN_POINT('Ctrl Pts',(-13.2512687078543,35.9598019389304,24.1799026900532));
#50910=CARTESIAN_POINT('Ctrl Pts',(-13.2622417301508,35.9218172623397,24.182260312743));
#50911=CARTESIAN_POINT('Ctrl Pts',(-13.2789753117563,35.8598452481243,24.1860538843696));
#50912=CARTESIAN_POINT('Ctrl Pts',(-13.2851427481617,35.8359725581357,24.1875026395995));
#50913=CARTESIAN_POINT('Ctrl Pts',(-13.2975842852012,35.7855489298977,24.1905369669661));
#50914=CARTESIAN_POINT('Ctrl Pts',(-13.303799450826,35.7589851722001,24.1921205795992));
#50915=CARTESIAN_POINT('Ctrl Pts',(-13.3155724314958,35.7057797025507,24.1952639922042));
#50916=CARTESIAN_POINT('Ctrl Pts',(-13.3211314305274,35.6791403530215,24.1968237246703));
#50917=CARTESIAN_POINT('Ctrl Pts',(-13.3336011557114,35.6155649456605,24.2005142969583));
#50918=CARTESIAN_POINT('Ctrl Pts',(-13.3402197721034,35.5785748800576,24.2026361865005));
#50919=CARTESIAN_POINT('Ctrl Pts',(-13.3753506445415,35.3614747083645,24.2149560550524));
#50920=CARTESIAN_POINT('Ctrl Pts',(-13.3899074801705,35.1794100348603,24.2247295043398));
#50921=CARTESIAN_POINT('Ctrl Pts',(-13.3897487153608,34.997048862956,24.2344129021999));
#50922=CARTESIAN_POINT('Ctrl Pts',(-13.3897487163589,34.9970500096102,24.2344128413124));
#50923=CARTESIAN_POINT('Ctrl Pts',(-13.3895571294199,34.776902993936,24.2461026719699));
#50924=CARTESIAN_POINT('Ctrl Pts',(-13.3679200225697,34.557313328916,24.2576093550979));
#50925=CARTESIAN_POINT('Ctrl Pts',(-13.3196008701561,34.3133621496472,24.2715832846215));
#50926=CARTESIAN_POINT('Ctrl Pts',(-13.3136953173194,34.2854059074429,24.2732031673232));
#50927=CARTESIAN_POINT('Ctrl Pts',(-13.3021887967361,34.2341485902329,24.2762127610933));
#50928=CARTESIAN_POINT('Ctrl Pts',(-13.2966927381551,34.2108256519966,24.2775973559733));
#50929=CARTESIAN_POINT('Ctrl Pts',(-13.287212423525,34.1724235763176,24.2799051712831));
#50930=CARTESIAN_POINT('Ctrl Pts',(-13.2833704138438,34.1573096848357,24.2808206721075));
#50931=CARTESIAN_POINT('Ctrl Pts',(-13.2753374520107,34.1265983334656,24.2826966460185));
#50932=CARTESIAN_POINT('Ctrl Pts',(-13.2711390869676,34.1110034051284,24.2836574706757));
#50933=CARTESIAN_POINT('Ctrl Pts',(-13.2597374138959,34.0698261488127,24.2862151579761));
#50934=CARTESIAN_POINT('Ctrl Pts',(-13.2523445416499,34.0442980129955,24.2878220441492));
#50935=CARTESIAN_POINT('Ctrl Pts',(-13.2156248932012,33.9228652515296,24.2955587624173));
#50936=CARTESIAN_POINT('Ctrl Pts',(-13.1823537217997,33.8282132618164,24.3018665739979));
#50937=CARTESIAN_POINT('Ctrl Pts',(-13.0668205335138,33.5409423662535,24.3216069462704));
#50938=CARTESIAN_POINT('Ctrl Pts',(-12.9708678509696,33.3543424825361,24.3352544126521));
#50939=CARTESIAN_POINT('Ctrl Pts',(-12.7852138530299,33.0631262000625,24.3571349096755));
#50940=CARTESIAN_POINT('Ctrl Pts',(-12.7052748078133,32.9529553537417,24.3655785682729));
#50941=CARTESIAN_POINT('Ctrl Pts',(-12.5925136060476,32.8157361353924,24.3762859235845));
#50942=CARTESIAN_POINT('Ctrl Pts',(-12.5655134067423,32.7840856021571,24.3787706258087));
#50943=CARTESIAN_POINT('Ctrl Pts',(-12.5195152074529,32.7321330698409,24.3828761294415));
#50944=CARTESIAN_POINT('Ctrl Pts',(-12.5008383397385,32.7115540293398,24.3845097291301));
#50945=CARTESIAN_POINT('Ctrl Pts',(-12.4634754324667,32.6713895982252,24.3877137161917));
#50946=CARTESIAN_POINT('Ctrl Pts',(-12.4448037123579,32.6517937740114,24.389284523467));
#50947=CARTESIAN_POINT('Ctrl Pts',(-12.4028608287367,32.6088176824744,24.3927479275085));
#50948=CARTESIAN_POINT('Ctrl Pts',(-12.3794789060723,32.5855490725045,24.3946355931771));
#50949=CARTESIAN_POINT('Ctrl Pts',(-12.2956055900131,32.5044842252876,24.4012616117989));
#50950=CARTESIAN_POINT('Ctrl Pts',(-12.2333161656908,32.4485877611927,24.405921185441));
#50951=CARTESIAN_POINT('Ctrl Pts',(-11.9563650478823,32.2179836515277,24.4256870232476));
#50952=CARTESIAN_POINT('Ctrl Pts',(-11.7228465203349,32.0676341469896,24.4399207379714));
#50953=CARTESIAN_POINT('Ctrl Pts',(-11.4136172364634,31.9183548791206,24.4585100745465));
#50954=CARTESIAN_POINT('Ctrl Pts',(-11.3527353409404,31.8911486768247,24.4621639210147));
#50955=CARTESIAN_POINT('Ctrl Pts',(-11.2493040403035,31.8485420462282,24.4684226242142));
#50956=CARTESIAN_POINT('Ctrl Pts',(-11.2071758782604,31.8321657535569,24.4709857455939));
#50957=CARTESIAN_POINT('Ctrl Pts',(-11.1461645194306,31.8098427955497,24.4747344849037));
#50958=CARTESIAN_POINT('Ctrl Pts',(-11.1275353565801,31.803210974512,24.475883982469));
#50959=CARTESIAN_POINT('Ctrl Pts',(-11.0947301526005,31.7918550208442,24.477918449241));
#50960=CARTESIAN_POINT('Ctrl Pts',(-11.0805792422273,31.7870610333325,24.4787994346731));
#50961=CARTESIAN_POINT('Ctrl Pts',(-11.0492623178913,31.7766819139516,24.4807569623977));
#50962=CARTESIAN_POINT('Ctrl Pts',(-11.0320833147195,31.7711403104398,24.4818357858848));
#50963=CARTESIAN_POINT('Ctrl Pts',(-10.9807753348092,31.7550406697284,24.4850710629145));
#50964=CARTESIAN_POINT('Ctrl Pts',(-10.9465238432179,31.7448849930582,24.4872481124605));
#50965=CARTESIAN_POINT('Ctrl Pts',(-10.6997374703552,31.6759362797509,24.5030263860203));
#50966=CARTESIAN_POINT('Ctrl Pts',(-10.4820847485064,31.637468725765,24.517392662528));
#50967=CARTESIAN_POINT('Ctrl Pts',(-10.1276831287408,31.6099675451656,24.5402396129539));
#50968=CARTESIAN_POINT('Ctrl Pts',(-9.99260102881325,31.6075711343711,24.5488308960645));
#50969=CARTESIAN_POINT('Ctrl Pts',(-9.79807649492301,31.6157428671968,24.5609265277053));
#50970=CARTESIAN_POINT('Ctrl Pts',(-9.73850081803834,31.6198242265351,24.5645946045661));
#50971=CARTESIAN_POINT('Ctrl Pts',(-9.63041023668735,31.6301043339381,24.571181857579));
#50972=CARTESIAN_POINT('Ctrl Pts',(-9.58186320276847,31.6357830948378,24.5741154059996));
#50973=CARTESIAN_POINT('Ctrl Pts',(-9.50445784953081,31.6465390938552,24.5787546789085));
#50974=CARTESIAN_POINT('Ctrl Pts',(-9.47551449149635,31.6509438488195,24.5804808506917));
#50975=CARTESIAN_POINT('Ctrl Pts',(-9.42033877975739,31.6600736315029,24.583756181418));
#50976=CARTESIAN_POINT('Ctrl Pts',(-9.39409811921259,31.6647341563619,24.5853072139116));
#50977=CARTESIAN_POINT('Ctrl Pts',(-9.33409786985865,31.6761221169906,24.5888396646425));
#50978=CARTESIAN_POINT('Ctrl Pts',(-9.30038004095852,31.6830553419444,24.5908145091278));
#50979=CARTESIAN_POINT('Ctrl Pts',(-9.19006831700129,31.70749516327,24.5972466329625));
#50980=CARTESIAN_POINT('Ctrl Pts',(-9.11397440444536,31.72715149279,24.6016370341393));
#50981=CARTESIAN_POINT('Ctrl Pts',(-8.80896738192478,31.8173589582658,24.6191471244879));
#50982=CARTESIAN_POINT('Ctrl Pts',(-8.58715702218629,31.9094272066104,24.6316240759671));
#50983=CARTESIAN_POINT('Ctrl Pts',(-8.29249733212567,32.0701395710731,24.649543263346));
#50984=CARTESIAN_POINT('Ctrl Pts',(-8.21009829635418,32.119740058332,24.6547255568649));
#50985=CARTESIAN_POINT('Ctrl Pts',(-8.09669859159546,32.1947485535841,24.6622559083283));
#50986=CARTESIAN_POINT('Ctrl Pts',(-8.06386495577287,32.2173083578861,24.6644860738599));
#50987=CARTESIAN_POINT('Ctrl Pts',(-8.00626338212422,32.2583990774589,24.6685022946936));
#50988=CARTESIAN_POINT('Ctrl Pts',(-7.98133681224192,32.2767005099841,24.6702759227249));
#50989=CARTESIAN_POINT('Ctrl Pts',(-7.94303937728579,32.3056337137126,24.6730626860955));
#50990=CARTESIAN_POINT('Ctrl Pts',(-7.92949201014461,32.3160303048044,24.6740607360829));
#50991=CARTESIAN_POINT('Ctrl Pts',(-7.9040892151567,32.3358318302873,24.6759566466741));
#50992=CARTESIAN_POINT('Ctrl Pts',(-7.89221736981219,32.3452144334309,24.6768530415));
#50993=CARTESIAN_POINT('Ctrl Pts',(-7.86370539158185,32.3680599266628,24.6790304474461));
#50994=CARTESIAN_POINT('Ctrl Pts',(-7.84712937311779,32.3816014024637,24.6803167366112));
#50995=CARTESIAN_POINT('Ctrl Pts',(-7.79069412837696,32.4286033057907,24.6847633795506));
#50996=CARTESIAN_POINT('Ctrl Pts',(-7.75147953748288,32.4628227273603,24.6879699769514));
#50997=CARTESIAN_POINT('Ctrl Pts',(-7.56239648637438,32.6356474182684,24.7039532512296));
#50998=CARTESIAN_POINT('Ctrl Pts',(-7.42447636238676,32.7866886688679,24.7172487192416));
#50999=CARTESIAN_POINT('Ctrl Pts',(-7.18378494213049,33.1034594890089,24.7427898806746));
#51000=CARTESIAN_POINT('Ctrl Pts',(-7.08000827381709,33.2674871264373,24.7550068616978));
#51001=CARTESIAN_POINT('Ctrl Pts',(-6.9701702869206,33.4792942672342,24.7694330112034));
#51002=CARTESIAN_POINT('Ctrl Pts',(-6.95032697822871,33.5194903699591,24.7721164481372));
#51003=CARTESIAN_POINT('Ctrl Pts',(-6.91920508131765,33.5858159424972,24.7764581553831));
#51004=CARTESIAN_POINT('Ctrl Pts',(-6.9074484187723,33.6117137648897,24.778132458361));
#51005=CARTESIAN_POINT('Ctrl Pts',(-6.88518322858662,33.662446810321,24.7813727219609));
#51006=CARTESIAN_POINT('Ctrl Pts',(-6.87464240460729,33.687265442976,24.782939673417));
#51007=CARTESIAN_POINT('Ctrl Pts',(-6.85029934367223,33.746537530876,24.7866402655671));
#51008=CARTESIAN_POINT('Ctrl Pts',(-6.8367644525545,33.7810974562904,24.788764948696));
#51009=CARTESIAN_POINT('Ctrl Pts',(-6.79290373373962,33.8987457486543,24.7958933691082));
#51010=CARTESIAN_POINT('Ctrl Pts',(-6.76526173564407,33.9827991857603,24.8008110292986));
#51011=CARTESIAN_POINT('Ctrl Pts',(-6.66630371271383,34.3287819850475,24.8205042823905));
#51012=CARTESIAN_POINT('Ctrl Pts',(-6.62328163017125,34.5977212700414,24.8344744210542));
#51013=CARTESIAN_POINT('Ctrl Pts',(-6.61022302245382,34.9351243512093,24.852758806131));
#51014=CARTESIAN_POINT('Ctrl Pts',(-6.6096026836829,35.0014027238726,24.8563915467869));
#51015=CARTESIAN_POINT('Ctrl Pts',(-6.61182336643764,35.1126475112598,24.8626179514774));
#51016=CARTESIAN_POINT('Ctrl Pts',(-6.61361745513232,35.1576173247334,24.8651704381664));
#51017=CARTESIAN_POINT('Ctrl Pts',(-6.61748568384727,35.2222424504657,24.868906370373));
#51018=CARTESIAN_POINT('Ctrl Pts',(-6.61883735722829,35.2419379015168,24.87005403492));
#51019=CARTESIAN_POINT('Ctrl Pts',(-6.62151395632357,35.2765145475507,24.8720865365758));
#51020=CARTESIAN_POINT('Ctrl Pts',(-6.62276533855362,35.2914005346689,24.8729674187618));
#51021=CARTESIAN_POINT('Ctrl Pts',(-6.62574829502362,35.3242795212311,24.8749263300077));
#51022=CARTESIAN_POINT('Ctrl Pts',(-6.62752538518625,35.3422670251966,24.8760066631514));
#51023=CARTESIAN_POINT('Ctrl Pts',(-6.63325599820558,35.3958851487253,24.8792510750172));
#51024=CARTESIAN_POINT('Ctrl Pts',(-6.63763087478682,35.4314671134746,24.8814359148847));
#51025=CARTESIAN_POINT('Ctrl Pts',(-6.66306125046046,35.6143064176287,24.8928042609559));
#51026=CARTESIAN_POINT('Ctrl Pts',(-6.69322803313417,35.7601215597907,24.9023376545813));
#51027=CARTESIAN_POINT('Ctrl Pts',(-6.76689822811388,36.0265275527062,24.9201419967892));
#51028=CARTESIAN_POINT('Ctrl Pts',(-6.807853772502,36.1475671557489,24.9283876597907));
#51029=CARTESIAN_POINT('Ctrl Pts',(-6.91181702503027,36.4057863683384,24.9460993640372));
#51030=CARTESIAN_POINT('Ctrl Pts',(-6.97735543101067,36.5416675614485,24.9554947061437));
#51031=CARTESIAN_POINT('Ctrl Pts',(-7.07280155197289,36.7098941663039,24.9671672477218));
#51032=CARTESIAN_POINT('Ctrl Pts',(-7.09457623989875,36.7466372943779,24.9697202037764));
#51033=CARTESIAN_POINT('Ctrl Pts',(-7.13177294527595,36.8067825466747,24.9739067234383));
#51034=CARTESIAN_POINT('Ctrl Pts',(-7.14680069096711,36.8304216404095,24.9755541697578));
#51035=CARTESIAN_POINT('Ctrl Pts',(-7.17683475990685,36.8763973432739,24.9787632310184));
#51036=CARTESIAN_POINT('Ctrl Pts',(-7.19181742038286,36.8987468560434,24.9803255511098));
#51037=CARTESIAN_POINT('Ctrl Pts',(-7.22538586335744,36.9475540279545,24.9837438659799));
#51038=CARTESIAN_POINT('Ctrl Pts',(-7.24408739419775,36.9739291046112,24.9855953902285));
#51039=CARTESIAN_POINT('Ctrl Pts',(-7.31045474192111,37.0647458723186,24.991990265523));
#51040=CARTESIAN_POINT('Ctrl Pts',(-7.36002806416642,37.1277637859511,24.9964618445592));
#51041=CARTESIAN_POINT('Ctrl Pts',(-7.59357434012739,37.4039059122624,25.016337395564));
#51042=CARTESIAN_POINT('Ctrl Pts',(-7.80140770260872,37.5953478339783,25.0308081024945));
#51043=CARTESIAN_POINT('Ctrl Pts',(-8.08505388986765,37.7978345718395,25.049670948102));
#51044=CARTESIAN_POINT('Ctrl Pts',(-8.14074216325374,37.8351466084457,25.0533430396186));
#51045=CARTESIAN_POINT('Ctrl Pts',(-8.23591532942056,37.8949038341931,25.059629642526));
#51046=CARTESIAN_POINT('Ctrl Pts',(-8.27481240491492,37.9182512376974,25.0622019332675));
#51047=CARTESIAN_POINT('Ctrl Pts',(-8.33134417493411,37.9506583912907,25.0659617118118));
#51048=CARTESIAN_POINT('Ctrl Pts',(-8.34860961260138,37.9603558826564,25.0671127853782));
#51049=CARTESIAN_POINT('Ctrl Pts',(-8.3790514016389,37.9771049728383,25.0691489450983));
#51050=CARTESIAN_POINT('Ctrl Pts',(-8.39219096032385,37.9842215832456,25.0700300226802));
#51051=CARTESIAN_POINT('Ctrl Pts',(-8.42128802356145,37.9997330950391,25.071986375748));
#51052=CARTESIAN_POINT('Ctrl Pts',(-8.43726551186566,38.00808760403,25.0730639129007));
#51053=CARTESIAN_POINT('Ctrl Pts',(-8.48403694018498,38.0320708398913,25.0762260874992));
#51054=CARTESIAN_POINT('Ctrl Pts',(-8.51500312988847,38.0473565060075,25.0783295298762));
#51055=CARTESIAN_POINT('Ctrl Pts',(-8.71707494132392,38.1432927835117,25.0920936307588));
#51056=CARTESIAN_POINT('Ctrl Pts',(-8.89443232965063,38.2099682747959,25.104329315168));
#51057=CARTESIAN_POINT('Ctrl Pts',(-9.22701757636996,38.3041496762514,25.1266041489797));
#51058=CARTESIAN_POINT('Ctrl Pts',(-9.38041031092342,38.3363187591695,25.1366350503712));
#51059=CARTESIAN_POINT('Ctrl Pts',(-9.62983306750515,38.3708237769615,25.152339574112));
#51060=CARTESIAN_POINT('Ctrl Pts',(-9.72469282572834,38.3798942411668,25.1581772941412));
#51061=CARTESIAN_POINT('Ctrl Pts',(-9.85700697659508,38.3869374285528,25.1661302544727));
#51062=CARTESIAN_POINT('Ctrl Pts',(-9.89422909683124,38.3883041232661,25.1683470025551));
#51063=CARTESIAN_POINT('Ctrl Pts',(-9.95844636072211,38.3896027087542,25.1721374235817));
#51064=CARTESIAN_POINT('Ctrl Pts',(-9.98543149969333,38.3898261090519,25.1737198832375));
#51065=CARTESIAN_POINT('Ctrl Pts',(-10.0408137242746,38.3896232365558,25.176947376927));
#51066=CARTESIAN_POINT('Ctrl Pts',(-10.0692085970337,38.3891623872687,25.178591223061));
#51067=CARTESIAN_POINT('Ctrl Pts',(-10.1421888457753,38.3870603269161,25.182790040654));
#51068=CARTESIAN_POINT('Ctrl Pts',(-10.1867543786129,38.3848956244716,25.1853288658937));
#51069=CARTESIAN_POINT('Ctrl Pts',(-10.4075522289393,38.3697965083944,25.197800676584));
#51070=CARTESIAN_POINT('Ctrl Pts',(-10.5826343583623,38.3439757491143,25.207333802329));
#51071=CARTESIAN_POINT('Ctrl Pts',(-10.9104044182862,38.2690986122176,25.2252288143845));
#51072=CARTESIAN_POINT('Ctrl Pts',(-11.0631822115104,38.2226514571052,25.2335967952355));
#51073=CARTESIAN_POINT('Ctrl Pts',(-11.2778418210958,38.1404583070954,25.2460122291844));
#51074=CARTESIAN_POINT('Ctrl Pts',(-11.3427634081787,38.1132528833275,25.249859945877));
#51075=CARTESIAN_POINT('Ctrl Pts',(-11.4495046871387,38.0645628796317,25.2564141280826));
#51076=CARTESIAN_POINT('Ctrl Pts',(-11.4918100652356,38.0441931213978,25.2590735633989));
#51077=CARTESIAN_POINT('Ctrl Pts',(-11.5515707743348,38.0138738889166,25.2629381110689));
#51078=CARTESIAN_POINT('Ctrl Pts',(-11.5693835782578,38.0046368878415,25.2641039588151));
#51079=CARTESIAN_POINT('Ctrl Pts',(-11.6003370923788,37.9882353045052,25.2661561336867));
#51080=CARTESIAN_POINT('Ctrl Pts',(-11.6135140243236,37.9811409774366,25.2670382201213));
#51081=CARTESIAN_POINT('Ctrl Pts',(-11.6422987305008,37.9653968250983,25.2689842001476));
#51082=CARTESIAN_POINT('Ctrl Pts',(-11.6578852319457,37.9567110066799,25.2700501788637));
#51083=CARTESIAN_POINT('Ctrl Pts',(-11.7026614991945,37.9312933781259,25.2731464020084));
#51084=CARTESIAN_POINT('Ctrl Pts',(-11.7316708777227,37.9142499612563,25.2751943427611));
#51085=CARTESIAN_POINT('Ctrl Pts',(-11.975306720037,37.766188390602,25.2927220602243));
#51086=CARTESIAN_POINT('Ctrl Pts',(-12.1749849035422,37.6121003403513,25.3092035926164));
#51087=CARTESIAN_POINT('Ctrl Pts',(-12.4401587470516,37.3558016131274,25.3328070381349));
#51088=CARTESIAN_POINT('Ctrl Pts',(-12.520250813079,37.2699153350808,25.3402293868745));
#51089=CARTESIAN_POINT('Ctrl Pts',(-12.6469040594358,37.1191118326437,25.3524164956147));
#51090=CARTESIAN_POINT('Ctrl Pts',(-12.6959178312605,37.0563960387051,25.3572645763915));
#51091=CARTESIAN_POINT('Ctrl Pts',(-12.7632229329192,36.9637275434503,25.3641209390319));
#51092=CARTESIAN_POINT('Ctrl Pts',(-12.7833257353138,36.9351291508179,25.3661969174104));
#51093=CARTESIAN_POINT('Ctrl Pts',(-12.8179653236338,36.884193805346,25.3698259824461));
#51094=CARTESIAN_POINT('Ctrl Pts',(-12.8326875270972,36.8619871898949,25.3713858794255));
#51095=CARTESIAN_POINT('Ctrl Pts',(-12.8630497633172,36.8149958189048,25.3746413425437));
#51096=CARTESIAN_POINT('Ctrl Pts',(-12.8786333281256,36.7901770890239,25.3763347577147));
#51097=CARTESIAN_POINT('Ctrl Pts',(-12.9194152057811,36.7233171511918,25.3808300696828));
#51098=CARTESIAN_POINT('Ctrl Pts',(-12.9440273257785,36.6809255167799,25.3836109977847));
#51099=CARTESIAN_POINT('Ctrl Pts',(-13.0495231215506,36.4897908377745,25.3958677956707));
#51100=CARTESIAN_POINT('Ctrl Pts',(-13.1200460176431,36.3357727065211,25.4049838019441));
#51101=CARTESIAN_POINT('Ctrl Pts',(-13.1787500473324,36.1772651354238,25.4139790685232));
#51102=CARTESIAN_POINT('Origin',(-10.,35.,23.));
#51103=CARTESIAN_POINT('',(-13.178750052031,36.1772651227369,26.6607620761902));
#51104=CARTESIAN_POINT('',(-13.1787501361565,36.1772648955886,26.3195304627418));
#51105=CARTESIAN_POINT('',(-13.1787500671536,36.1772650819043,23.));
#51106=CARTESIAN_POINT('',(-13.3897489515612,35.0026660626174,25.139683636804));
#51107=CARTESIAN_POINT('Ctrl Pts',(-13.1787501361565,36.1772648955886,26.3195304627418));
#51108=CARTESIAN_POINT('Ctrl Pts',(-13.1275293037145,36.3155670132421,26.3116510922332));
#51109=CARTESIAN_POINT('Ctrl Pts',(-13.0673160770592,36.4504360067458,26.3039018533949));
#51110=CARTESIAN_POINT('Ctrl Pts',(-12.9360697556378,36.6993528101704,26.2888533953585));
#51111=CARTESIAN_POINT('Ctrl Pts',(-12.8667215596882,36.8138925045017,26.2815932999696));
#51112=CARTESIAN_POINT('Ctrl Pts',(-12.7748582381106,36.9471402705108,26.2723743592933));
#51113=CARTESIAN_POINT('Ctrl Pts',(-12.7586346998618,36.9700578567182,26.2707593878122));
#51114=CARTESIAN_POINT('Ctrl Pts',(-12.732444421697,37.0060966882031,26.2681682566491));
#51115=CARTESIAN_POINT('Ctrl Pts',(-12.7226631404088,37.0193518364037,26.2672039542068));
#51116=CARTESIAN_POINT('Ctrl Pts',(-12.7035594609724,37.0448491562393,26.2653260017636));
#51117=CARTESIAN_POINT('Ctrl Pts',(-12.6942496972644,37.0570999892027,26.2644131582124));
#51118=CARTESIAN_POINT('Ctrl Pts',(-12.6708782214884,37.0874240017261,26.262128083507));
#51119=CARTESIAN_POINT('Ctrl Pts',(-12.6567162805108,37.1054187182352,26.2607492532518));
#51120=CARTESIAN_POINT('Ctrl Pts',(-12.6001877712615,37.1757675558729,26.2552727190622));
#51121=CARTESIAN_POINT('Ctrl Pts',(-12.5564494902722,37.2269947640009,26.2510944263239));
#51122=CARTESIAN_POINT('Ctrl Pts',(-12.4289837806037,37.3675792125859,26.2391567536474));
#51123=CARTESIAN_POINT('Ctrl Pts',(-12.341900084493,37.4537511963823,26.2312750484712));
#51124=CARTESIAN_POINT('Ctrl Pts',(-12.0685105409671,37.6964405626681,26.2077111659704));
#51125=CARTESIAN_POINT('Ctrl Pts',(-11.8698015821148,37.8378520034734,26.1921269069638));
#51126=CARTESIAN_POINT('Ctrl Pts',(-11.6128238807767,37.9819196123726,26.1742101421693));
#51127=CARTESIAN_POINT('Ctrl Pts',(-11.5674350984947,38.0060261291993,26.1711195098881));
#51128=CARTESIAN_POINT('Ctrl Pts',(-11.4946394343588,38.0425914087537,26.1662764067341));
#51129=CARTESIAN_POINT('Ctrl Pts',(-11.4675859575751,38.0557324921846,26.1645007869129));
#51130=CARTESIAN_POINT('Ctrl Pts',(-11.4187814457073,38.0786413446195,26.161339755989));
#51131=CARTESIAN_POINT('Ctrl Pts',(-11.3970957423347,38.0885428358814,26.1599498773572));
#51132=CARTESIAN_POINT('Ctrl Pts',(-11.3458353109171,38.1112974963614,26.1566979982741));
#51133=CARTESIAN_POINT('Ctrl Pts',(-11.31617778294,38.1239591772765,26.1548425128361));
#51134=CARTESIAN_POINT('Ctrl Pts',(-11.2272517195581,38.160433124529,26.149352274682));
#51135=CARTESIAN_POINT('Ctrl Pts',(-11.1674845477299,38.1829962091945,26.1457584688189));
#51136=CARTESIAN_POINT('Ctrl Pts',(-10.9515859052322,38.2576013036794,26.133071779718));
#51137=CARTESIAN_POINT('Ctrl Pts',(-10.7923438257267,38.2999514203855,26.1242691563581));
#51138=CARTESIAN_POINT('Ctrl Pts',(-10.4225482046364,38.3699727235213,26.1042887597988));
#51139=CARTESIAN_POINT('Ctrl Pts',(-10.2112343148089,38.389782548502,26.0932033489857));
#51140=CARTESIAN_POINT('Ctrl Pts',(-9.95505955389538,38.3897431239352,26.0788606215348));
#51141=CARTESIAN_POINT('Ctrl Pts',(-9.91064735909992,38.3888632030355,26.076340266163));
#51142=CARTESIAN_POINT('Ctrl Pts',(-9.84684763951365,38.3863442141167,26.0726550445531));
#51143=CARTESIAN_POINT('Ctrl Pts',(-9.82743521529211,38.3854104829736,26.0715251189875));
#51144=CARTESIAN_POINT('Ctrl Pts',(-9.79311507733015,38.383463747946,26.0695105551651));
#51145=CARTESIAN_POINT('Ctrl Pts',(-9.7782043870701,38.3825190315678,26.0686295832056));
#51146=CARTESIAN_POINT('Ctrl Pts',(-9.74528999012911,38.3802150555544,26.0666718741739));
#51147=CARTESIAN_POINT('Ctrl Pts',(-9.72729081810735,38.3788105423087,26.0655928529111));
#51148=CARTESIAN_POINT('Ctrl Pts',(-9.67369492241274,38.3741973078412,26.0623563811923));
#51149=CARTESIAN_POINT('Ctrl Pts',(-9.63813786584196,38.3705693959921,26.060178313178));
#51150=CARTESIAN_POINT('Ctrl Pts',(-9.45997914560893,38.3495402762919,26.0491315355943));
#51151=CARTESIAN_POINT('Ctrl Pts',(-9.31853753500384,38.3236493436193,26.0399366963367));
#51152=CARTESIAN_POINT('Ctrl Pts',(-8.91465693344667,38.2228504292406,26.0131331119742));
#51153=CARTESIAN_POINT('Ctrl Pts',(-8.65901756661329,38.1251478362792,25.9955696647063));
#51154=CARTESIAN_POINT('Ctrl Pts',(-8.3750743612192,37.9752913099574,25.976099755814));
#51155=CARTESIAN_POINT('Ctrl Pts',(-8.33281000526718,37.9518163210347,25.9731990792327));
#51156=CARTESIAN_POINT('Ctrl Pts',(-8.26587317576551,37.9127409452949,25.9685988784394));
#51157=CARTESIAN_POINT('Ctrl Pts',(-8.24087608367216,37.8977126813187,25.9668795096363));
#51158=CARTESIAN_POINT('Ctrl Pts',(-8.19338814528815,37.8683219039009,25.9636093324775));
#51159=CARTESIAN_POINT('Ctrl Pts',(-8.17086694621227,37.8540128362286,25.9620567602209));
#51160=CARTESIAN_POINT('Ctrl Pts',(-8.1189902405869,37.8201861331183,25.958475246064));
#51161=CARTESIAN_POINT('Ctrl Pts',(-8.08976528343335,37.800473352958,25.9564536415056));
#51162=CARTESIAN_POINT('Ctrl Pts',(-7.99405206312668,37.733717409021,25.9498141826609));
#51163=CARTESIAN_POINT('Ctrl Pts',(-7.92894950392359,37.6847326214061,25.9452685852849));
#51164=CARTESIAN_POINT('Ctrl Pts',(-7.77122064623841,37.5568981807403,25.9341091572406));
#51165=CARTESIAN_POINT('Ctrl Pts',(-7.6809530164362,37.475320059597,25.927590194822));
#51166=CARTESIAN_POINT('Ctrl Pts',(-7.4657713371864,37.2587265325699,25.9113514605366));
#51167=CARTESIAN_POINT('Ctrl Pts',(-7.34710101386797,37.1180840911621,25.9017337902083));
#51168=CARTESIAN_POINT('Ctrl Pts',(-7.19535360780638,36.9053569488521,25.8874505685673));
#51169=CARTESIAN_POINT('Ctrl Pts',(-7.15247585933609,36.8406604867681,25.8831352834082));
#51170=CARTESIAN_POINT('Ctrl Pts',(-7.09892555608304,36.7535057648641,25.877281531557));
#51171=CARTESIAN_POINT('Ctrl Pts',(-7.08622326977071,36.732316508884,25.8758552874268));
#51172=CARTESIAN_POINT('Ctrl Pts',(-7.06659106432234,36.6987402591333,25.87358743745));
#51173=CARTESIAN_POINT('Ctrl Pts',(-7.05950515217262,36.6864449252258,25.8727553373451));
#51174=CARTESIAN_POINT('Ctrl Pts',(-7.04480873252465,36.6605697705818,25.8710000266439));
#51175=CARTESIAN_POINT('Ctrl Pts',(-7.03721426087042,36.6469814884838,25.8700757835793));
#51176=CARTESIAN_POINT('Ctrl Pts',(-7.01823479764693,36.6124667064079,25.8677229102746));
#51177=CARTESIAN_POINT('Ctrl Pts',(-7.00697644950711,36.591471821073,25.8662868511381));
#51178=CARTESIAN_POINT('Ctrl Pts',(-6.96084190222991,36.503217626561,25.8602355795365));
#51179=CARTESIAN_POINT('Ctrl Pts',(-6.92800649605403,36.4349213974346,25.8555178657469));
#51180=CARTESIAN_POINT('Ctrl Pts',(-6.83676988804999,36.2276388294385,25.8412141486208));
#51181=CARTESIAN_POINT('Ctrl Pts',(-6.78532081259013,36.0857978917837,25.831452983835));
#51182=CARTESIAN_POINT('Ctrl Pts',(-6.6875560973918,35.7474668904436,25.8087826760018));
#51183=CARTESIAN_POINT('Ctrl Pts',(-6.64898825076266,35.5493013221105,25.7959825536002));
#51184=CARTESIAN_POINT('Ctrl Pts',(-6.62279325577151,35.2961256535132,25.7804840904007));
#51185=CARTESIAN_POINT('Ctrl Pts',(-6.61857471691793,35.2432680108596,25.7772922963834));
#51186=CARTESIAN_POINT('Ctrl Pts',(-6.61388941396592,35.1599554438428,25.7723284545866));
#51187=CARTESIAN_POINT('Ctrl Pts',(-6.61259014418947,35.1295577247001,25.7705312779608));
#51188=CARTESIAN_POINT('Ctrl Pts',(-6.61092676477455,35.0727119073951,25.7671954272703));
#51189=CARTESIAN_POINT('Ctrl Pts',(-6.61046262321786,35.0462692668806,25.7656538022693));
#51190=CARTESIAN_POINT('Ctrl Pts',(-6.61011468628387,34.9867737796948,25.7622067123146));
#51191=CARTESIAN_POINT('Ctrl Pts',(-6.61040476393469,34.9537223719902,25.7603067180634));
#51192=CARTESIAN_POINT('Ctrl Pts',(-6.61277593008491,34.8524185078345,25.7545250526883));
#51193=CARTESIAN_POINT('Ctrl Pts',(-6.61643584820695,34.7842184120162,25.7506913925367));
#51194=CARTESIAN_POINT('Ctrl Pts',(-6.64315860307748,34.4661899715361,25.73301560677));
#51195=CARTESIAN_POINT('Ctrl Pts',(-6.69184675734686,34.2193182773196,25.7199448208357));
#51196=CARTESIAN_POINT('Ctrl Pts',(-6.81084275816068,33.842159700656,25.6988475975735));
#51197=CARTESIAN_POINT('Ctrl Pts',(-6.86313146312335,33.7071870752379,25.6910331903002));
#51198=CARTESIAN_POINT('Ctrl Pts',(-6.93575182762144,33.5503144797316,25.6811890543293));
#51199=CARTESIAN_POINT('Ctrl Pts',(-6.94795358343876,33.5247991560503,25.6795626933458));
#51200=CARTESIAN_POINT('Ctrl Pts',(-6.9677845409416,33.4846296516265,25.6769575101952));
#51201=CARTESIAN_POINT('Ctrl Pts',(-6.97520432366668,33.4698728894683,25.6759907662249));
#51202=CARTESIAN_POINT('Ctrl Pts',(-6.9897332507737,33.4414958443124,25.674111829048));
#51203=CARTESIAN_POINT('Ctrl Pts',(-6.9968276186201,33.4278687337668,25.6732004926753));
#51204=CARTESIAN_POINT('Ctrl Pts',(-7.01466685717736,33.3941638751519,25.6709246808398));
#51205=CARTESIAN_POINT('Ctrl Pts',(-7.02552179740678,33.3741454573063,25.6695537194397));
#51206=CARTESIAN_POINT('Ctrl Pts',(-7.06875424686307,33.2962994110933,25.6641511004625));
#51207=CARTESIAN_POINT('Ctrl Pts',(-7.10262141876041,33.239320147732,25.6600414748331));
#51208=CARTESIAN_POINT('Ctrl Pts',(-7.20200129245492,33.0827596500587,25.6483824669053));
#51209=CARTESIAN_POINT('Ctrl Pts',(-7.27112703209098,32.9855876497149,25.6407165603508));
#51210=CARTESIAN_POINT('Ctrl Pts',(-7.49992591407496,32.6974065492212,25.6170006440483));
#51211=CARTESIAN_POINT('Ctrl Pts',(-7.67563750068054,32.5201446055275,25.6010378242968));
#51212=CARTESIAN_POINT('Ctrl Pts',(-7.908718515938,32.33175534775,25.5828195237582));
#51213=CARTESIAN_POINT('Ctrl Pts',(-7.94895775156781,32.3007012237518,25.5797638550779));
#51214=CARTESIAN_POINT('Ctrl Pts',(-8.01399985670856,32.2528003961934,25.5749625457225));
#51215=CARTESIAN_POINT('Ctrl Pts',(-8.03835286149508,32.2353584640058,25.5731944251065));
#51216=CARTESIAN_POINT('Ctrl Pts',(-8.08468636664157,32.203094331023,25.5698846187334));
#51217=CARTESIAN_POINT('Ctrl Pts',(-8.10661562962621,32.1882028309092,25.5683404108251));
#51218=CARTESIAN_POINT('Ctrl Pts',(-8.15686931485316,32.1549315947795,25.5648507548753));
#51219=CARTESIAN_POINT('Ctrl Pts',(-8.18529842637698,32.1367146022925,25.562911379592));
#51220=CARTESIAN_POINT('Ctrl Pts',(-8.2754877120701,32.0808054553026,25.5568626564743));
#51221=CARTESIAN_POINT('Ctrl Pts',(-8.33818698640275,32.044662803327,25.5528083057104));
#51222=CARTESIAN_POINT('Ctrl Pts',(-8.49195106430681,31.9624685908534,25.5431756415221));
#51223=CARTESIAN_POINT('Ctrl Pts',(-8.58403203672346,31.9184670592111,25.5376595771576));
#51224=CARTESIAN_POINT('Ctrl Pts',(-8.7221275872218,31.8599764721752,25.5296368796231));
#51225=CARTESIAN_POINT('Ctrl Pts',(-8.76668633368025,31.8422091338516,25.5270846785267));
#51226=CARTESIAN_POINT('Ctrl Pts',(-9.00739032764444,31.752103231928,25.5134383882406));
#51227=CARTESIAN_POINT('Ctrl Pts',(-9.2095145713375,31.697088564832,25.5024973692784));
#51228=CARTESIAN_POINT('Ctrl Pts',(-9.46092523955007,31.6530700603128,25.4882441144485));
#51229=CARTESIAN_POINT('Ctrl Pts',(-9.50661157815093,31.6460308503453,25.485627614754));
#51230=CARTESIAN_POINT('Ctrl Pts',(-9.57084239733155,31.6374750519693,25.4818945626879));
#51231=CARTESIAN_POINT('Ctrl Pts',(-9.58927900799401,31.6351733317521,25.4808167729782));
#51232=CARTESIAN_POINT('Ctrl Pts',(-9.62272441959315,31.6312768016293,25.4788487452096));
#51233=CARTESIAN_POINT('Ctrl Pts',(-9.63772696093006,31.6296304222895,25.4779612606449));
#51234=CARTESIAN_POINT('Ctrl Pts',(-9.66936998301466,31.6263716353199,25.4760787322545));
#51235=CARTESIAN_POINT('Ctrl Pts',(-9.6860119969392,31.6247820723671,25.4750825663478));
#51236=CARTESIAN_POINT('Ctrl Pts',(-9.73177405669042,31.620752475635,25.4723278612193));
#51237=CARTESIAN_POINT('Ctrl Pts',(-9.76091430141407,31.6185658528079,25.4705565559212));
#51238=CARTESIAN_POINT('Ctrl Pts',(-9.82699099950323,31.6144659568371,25.4665066047314));
#51239=CARTESIAN_POINT('Ctrl Pts',(-9.86393755295473,31.6127799490557,25.464218470908));
#51240=CARTESIAN_POINT('Ctrl Pts',(-9.98615724706017,31.6092054067664,25.4565866189869));
#51241=CARTESIAN_POINT('Ctrl Pts',(-10.0714711667598,31.6099306859455,25.451159193638));
#51242=CARTESIAN_POINT('Ctrl Pts',(-10.4342489180101,31.6267149018692,25.4278699980286));
#51243=CARTESIAN_POINT('Ctrl Pts',(-10.7092551647009,31.6736468145872,25.4098054879696));
#51244=CARTESIAN_POINT('Ctrl Pts',(-11.0361669224451,31.7718765194759,25.3888701735249));
#51245=CARTESIAN_POINT('Ctrl Pts',(-11.0963527678074,31.7918175694263,25.3850331258267));
#51246=CARTESIAN_POINT('Ctrl Pts',(-11.1865500028866,31.8245372101359,25.3793069739075));
#51247=CARTESIAN_POINT('Ctrl Pts',(-11.2169921272335,31.836079155179,25.3773785525555));
#51248=CARTESIAN_POINT('Ctrl Pts',(-11.2718254583321,31.8577774121937,25.3739114891858));
#51249=CARTESIAN_POINT('Ctrl Pts',(-11.296272888264,31.8677836209125,25.3723680588408));
#51250=CARTESIAN_POINT('Ctrl Pts',(-11.3489653591365,31.8900729921109,25.3690455176644));
#51251=CARTESIAN_POINT('Ctrl Pts',(-11.377165145625,31.9024574601535,25.3672699444308));
#51252=CARTESIAN_POINT('Ctrl Pts',(-11.4564828926092,31.9385886951742,25.3622802668674));
#51253=CARTESIAN_POINT('Ctrl Pts',(-11.5071840482756,31.9632289608131,25.359096286936));
#51254=CARTESIAN_POINT('Ctrl Pts',(-11.6213290531763,32.0222656589352,25.3519220577914));
#51255=CARTESIAN_POINT('Ctrl Pts',(-11.6843367330153,32.057446631537,25.347957719094));
#51256=CARTESIAN_POINT('Ctrl Pts',(-11.911358391023,32.1938896874611,25.3335722052934));
#51257=CARTESIAN_POINT('Ctrl Pts',(-12.0677716748163,32.3070707873441,25.323480277421));
#51258=CARTESIAN_POINT('Ctrl Pts',(-12.3270273149047,32.5306409346461,25.3052358954368));
#51259=CARTESIAN_POINT('Ctrl Pts',(-12.4337280804593,32.63573508668,25.2971662840273));
#51260=CARTESIAN_POINT('Ctrl Pts',(-12.551936842087,32.7686719969475,25.2870362578449));
#51261=CARTESIAN_POINT('Ctrl Pts',(-12.5704798986837,32.7900589866139,25.2854085809478));
#51262=CARTESIAN_POINT('Ctrl Pts',(-12.5994186357054,32.8242930330407,25.2828017742787));
#51263=CARTESIAN_POINT('Ctrl Pts',(-12.6099923323982,32.8369886617042,25.281834748339));
#51264=CARTESIAN_POINT('Ctrl Pts',(-12.6302165842051,32.8616357319033,25.2799556937193));
#51265=CARTESIAN_POINT('Ctrl Pts',(-12.6398793801173,32.8735762776283,25.2790445276599));
#51266=CARTESIAN_POINT('Ctrl Pts',(-12.6636559223769,32.9033693451576,25.2767697680011));
#51267=CARTESIAN_POINT('Ctrl Pts',(-12.6776715465503,32.9212989626353,25.2753997013193));
#51268=CARTESIAN_POINT('Ctrl Pts',(-12.7317198872348,32.9918944756329,25.2700054156625));
#51269=CARTESIAN_POINT('Ctrl Pts',(-12.7703857646075,33.0455837486532,25.2659035212957));
#51270=CARTESIAN_POINT('Ctrl Pts',(-12.8788185821629,33.2058357150553,25.2537390742254));
#51271=CARTESIAN_POINT('Ctrl Pts',(-12.9441804209429,33.3152386766303,25.2455359813105));
#51272=CARTESIAN_POINT('Ctrl Pts',(-13.1084485820639,33.6290757093731,25.2227021709515));
#51273=CARTESIAN_POINT('Ctrl Pts',(-13.1932325883007,33.8401817121344,25.2081577404558));
#51274=CARTESIAN_POINT('Ctrl Pts',(-13.2711801538501,34.1096864905325,25.1910044784193));
#51275=CARTESIAN_POINT('Ctrl Pts',(-13.2848488903701,34.1615216174511,25.1877640333986));
#51276=CARTESIAN_POINT('Ctrl Pts',(-13.3050041541777,34.2460368784401,25.1825736372484));
#51277=CARTESIAN_POINT('Ctrl Pts',(-13.3122480302675,34.278525154762,25.1806003659227));
#51278=CARTESIAN_POINT('Ctrl Pts',(-13.3243904396943,34.3370267211086,25.177085183281));
#51279=CARTESIAN_POINT('Ctrl Pts',(-13.3294649444423,34.3630003087431,25.1755378702808));
#51280=CARTESIAN_POINT('Ctrl Pts',(-13.3387175006471,34.4134942070377,25.1725547367493));
#51281=CARTESIAN_POINT('Ctrl Pts',(-13.3429308486618,34.438006242891,25.1711179063616));
#51282=CARTESIAN_POINT('Ctrl Pts',(-13.3516007075619,34.4919975417983,25.1679767972371));
#51283=CARTESIAN_POINT('Ctrl Pts',(-13.3559388788068,34.5214938654338,25.1662762338235));
#51284=CARTESIAN_POINT('Ctrl Pts',(-13.3674687876274,34.6077812026211,25.161343445804));
#51285=CARTESIAN_POINT('Ctrl Pts',(-13.3736120216804,34.6647030477051,25.1581424529301));
#51286=CARTESIAN_POINT('Ctrl Pts',(-13.3860065433332,34.8151913438201,25.149793627205));
#51287=CARTESIAN_POINT('Ctrl Pts',(-13.3898226925466,34.9089085392964,25.1447108366345));
#51288=CARTESIAN_POINT('Ctrl Pts',(-13.3897489515612,35.0026660626174,25.139683636804));
#51289=CARTESIAN_POINT('Ctrl Pts',(-13.3897489540441,35.0026629038459,25.1396838061747));
#51290=CARTESIAN_POINT('Ctrl Pts',(-13.3895586151162,35.2449552355166,25.1266922911326));
#51291=CARTESIAN_POINT('Ctrl Pts',(-13.3633917304235,35.486518723814,25.114168333125));
#51292=CARTESIAN_POINT('Ctrl Pts',(-13.2975733377464,35.7879081937708,25.0971784745588));
#51293=CARTESIAN_POINT('Ctrl Pts',(-13.2815550038618,35.8521648037139,25.0934711323419));
#51294=CARTESIAN_POINT('Ctrl Pts',(-13.2575155904463,35.9378248654316,25.0883645600871));
#51295=CARTESIAN_POINT('Ctrl Pts',(-13.2511440960134,35.9596797938305,25.0870471058161));
#51296=CARTESIAN_POINT('Ctrl Pts',(-13.2401052720513,35.9961721115334,25.0848202522941));
#51297=CARTESIAN_POINT('Ctrl Pts',(-13.235557549218,36.01084538306,25.0839174652042));
#51298=CARTESIAN_POINT('Ctrl Pts',(-13.2259125759084,36.0412329325706,25.0820316066258));
#51299=CARTESIAN_POINT('Ctrl Pts',(-13.2207999761956,36.0569415572434,25.0810477592457));
#51300=CARTESIAN_POINT('Ctrl Pts',(-13.2066196900164,36.0994525038195,25.0783620751255));
#51301=CARTESIAN_POINT('Ctrl Pts',(-13.1973311007903,36.1261790988632,25.0766484626819));
#51302=CARTESIAN_POINT('Ctrl Pts',(-13.1847541388108,36.1609572133311,25.074388478803));
#51303=CARTESIAN_POINT('Ctrl Pts',(-13.1817676762443,36.1691171929711,25.07385603406));
#51304=CARTESIAN_POINT('Ctrl Pts',(-13.1787500684596,36.1772650783778,25.0733222522952));
#51305=CARTESIAN_POINT('Ctrl Pts',(-13.1787500473324,36.1772651354238,25.4139790685232));
#51306=CARTESIAN_POINT('Ctrl Pts',(-13.2129579337196,36.0848999432503,25.4192207709888));
#51307=CARTESIAN_POINT('Ctrl Pts',(-13.2431524082573,35.9910104588357,25.4244252688241));
#51308=CARTESIAN_POINT('Ctrl Pts',(-13.3114026221524,35.7419465658512,25.4381644453243));
#51309=CARTESIAN_POINT('Ctrl Pts',(-13.3426522696491,35.5852664646178,25.4467389538416));
#51310=CARTESIAN_POINT('Ctrl Pts',(-13.3663308409915,35.3987855749979,25.4574416608772));
#51311=CARTESIAN_POINT('Ctrl Pts',(-13.3695568188617,35.3705401434797,25.4590761898304));
#51312=CARTESIAN_POINT('Ctrl Pts',(-13.3740979390716,35.3257944389112,25.4616914500143));
#51313=CARTESIAN_POINT('Ctrl Pts',(-13.3756482038414,35.3093187639212,25.4626599435699));
#51314=CARTESIAN_POINT('Ctrl Pts',(-13.3783882017451,35.2777198903346,25.4645291472995));
#51315=CARTESIAN_POINT('Ctrl Pts',(-13.379597151546,35.2625990083102,25.4654288302341));
#51316=CARTESIAN_POINT('Ctrl Pts',(-13.3823498930941,35.2249937680228,25.4676785497845));
#51317=CARTESIAN_POINT('Ctrl Pts',(-13.383770993291,35.2025013577761,25.4690349730233));
#51318=CARTESIAN_POINT('Ctrl Pts',(-13.3881296066075,35.1205346874929,25.4740133933695));
#51319=CARTESIAN_POINT('Ctrl Pts',(-13.3897239751888,35.0610028093467,25.4776967957614));
#51320=CARTESIAN_POINT('Ctrl Pts',(-13.389794204842,34.898358979822,25.4878914648462));
#51321=CARTESIAN_POINT('Ctrl Pts',(-13.3851345436779,34.7953108227253,25.4944935619505));
#51322=CARTESIAN_POINT('Ctrl Pts',(-13.3515711501112,34.4266772184745,25.5183173666823));
#51323=CARTESIAN_POINT('Ctrl Pts',(-13.2960042092167,34.164459520482,25.5355549120409));
#51324=CARTESIAN_POINT('Ctrl Pts',(-13.1929876577644,33.8606521634231,25.5550979313356));
#51325=CARTESIAN_POINT('Ctrl Pts',(-13.174553782942,33.8102553022593,25.5583292040501));
#51326=CARTESIAN_POINT('Ctrl Pts',(-13.1437546594498,33.7318732161826,25.5633400842122));
#51327=CARTESIAN_POINT('Ctrl Pts',(-13.132194492935,33.7035831501014,25.5651456110598));
#51328=CARTESIAN_POINT('Ctrl Pts',(-13.1099245406714,33.651121543416,25.5684892082005));
#51329=CARTESIAN_POINT('Ctrl Pts',(-13.0993115773421,33.6269116764551,25.5700303504126));
#51330=CARTESIAN_POINT('Ctrl Pts',(-13.0748705108757,33.5728852696599,25.5734665162781));
#51331=CARTESIAN_POINT('Ctrl Pts',(-13.0608896749292,33.5431404945895,25.5753562265366));
#51332=CARTESIAN_POINT('Ctrl Pts',(-13.0169918116406,33.4531686515352,25.5810696311151));
#51333=CARTESIAN_POINT('Ctrl Pts',(-12.9857125403696,33.3936226256971,25.5848470208367));
#51334=CARTESIAN_POINT('Ctrl Pts',(-12.830387160293,33.1181641750318,25.6023726157613));
#51335=CARTESIAN_POINT('Ctrl Pts',(-12.6845745934833,32.9154228338062,25.6153580405207));
#51336=CARTESIAN_POINT('Ctrl Pts',(-12.4187424083374,32.6205022365624,25.6365240637188));
#51337=CARTESIAN_POINT('Ctrl Pts',(-12.3125292888982,32.5171541309261,25.6445139537417));
#51338=CARTESIAN_POINT('Ctrl Pts',(-12.1783851522986,32.4027237243424,25.6545545900013));
#51339=CARTESIAN_POINT('Ctrl Pts',(-12.1566265858284,32.3846285957447,25.6561818926817));
#51340=CARTESIAN_POINT('Ctrl Pts',(-12.121811194821,32.3564048616195,25.6587882374092));
#51341=CARTESIAN_POINT('Ctrl Pts',(-12.1089020140346,32.3460952782005,25.6597551829125));
#51342=CARTESIAN_POINT('Ctrl Pts',(-12.0838449647861,32.3263823742694,25.6616342032859));
#51343=CARTESIAN_POINT('Ctrl Pts',(-12.0717077185813,32.3169666158632,25.6625454171772));
#51344=CARTESIAN_POINT('Ctrl Pts',(-12.041428341085,32.2938046098369,25.6648204739112));
#51345=CARTESIAN_POINT('Ctrl Pts',(-12.023211104007,32.2801581059877,25.6661907934732));
#51346=CARTESIAN_POINT('Ctrl Pts',(-11.9514883757159,32.2275500026887,25.6715874359183));
#51347=CARTESIAN_POINT('Ctrl Pts',(-11.8969867100227,32.1899775592534,25.6756915169324));
#51348=CARTESIAN_POINT('Ctrl Pts',(-11.741586563053,32.0894293128611,25.6873282187567));
#51349=CARTESIAN_POINT('Ctrl Pts',(-11.638423302349,32.0301326571558,25.694976903951));
#51350=CARTESIAN_POINT('Ctrl Pts',(-11.3100242659808,31.8637007264316,25.7187055492107));
#51351=CARTESIAN_POINT('Ctrl Pts',(-11.0758988969106,31.7758698465472,25.7346992769268));
#51352=CARTESIAN_POINT('Ctrl Pts',(-10.7844414725703,31.7018648464897,25.7529783223421));
#51353=CARTESIAN_POINT('Ctrl Pts',(-10.7343688324649,31.690355492673,25.7560665249389));
#51354=CARTESIAN_POINT('Ctrl Pts',(-10.6548757687406,31.6739768239713,25.7608893422627));
#51355=CARTESIAN_POINT('Ctrl Pts',(-10.625621100955,31.6683501440244,25.7626473326219));
#51356=CARTESIAN_POINT('Ctrl Pts',(-10.5701750566453,31.6584420514336,25.7659484364741));
#51357=CARTESIAN_POINT('Ctrl Pts',(-10.5440003376274,31.6540811709684,25.7674939191911));
#51358=CARTESIAN_POINT('Ctrl Pts',(-10.484138444133,31.6448288295742,25.771000307956));
#51359=CARTESIAN_POINT('Ctrl Pts',(-10.4504231103753,31.6401364971965,25.7729549082072));
#51360=CARTESIAN_POINT('Ctrl Pts',(-10.3432343308713,31.6268610184773,25.779109450332));
#51361=CARTESIAN_POINT('Ctrl Pts',(-10.2695456274935,31.6201741715645,25.7832514883377));
#51362=CARTESIAN_POINT('Ctrl Pts',(-10.0905435619604,31.6098229612272,25.7931480676126));
#51363=CARTESIAN_POINT('Ctrl Pts',(-9.98516328836684,31.6086462331143,25.7988353102028));
#51364=CARTESIAN_POINT('Ctrl Pts',(-9.75584269178043,31.6167766142942,25.8110957658923));
#51365=CARTESIAN_POINT('Ctrl Pts',(-9.63212658365565,31.6279853995241,25.8176357061282));
#51366=CARTESIAN_POINT('Ctrl Pts',(-9.36614051087889,31.6668990869816,25.831943014208));
#51367=CARTESIAN_POINT('Ctrl Pts',(-9.22447753827665,31.6969867277509,25.8397195612678));
#51368=CARTESIAN_POINT('Ctrl Pts',(-9.05086008350839,31.7456476525079,25.8499003880931));
#51369=CARTESIAN_POINT('Ctrl Pts',(-9.01669091796208,31.7558084487553,25.8519364909765));
#51370=CARTESIAN_POINT('Ctrl Pts',(-8.96548551177221,31.7719185076869,25.8550455522482));
#51371=CARTESIAN_POINT('Ctrl Pts',(-8.94832512955932,31.7774683426617,25.8560973605369));
#51372=CARTESIAN_POINT('Ctrl Pts',(-8.91702917831271,31.7878663532101,25.8580350543435));
#51373=CARTESIAN_POINT('Ctrl Pts',(-8.90288022146633,31.7926714339753,25.85891853074));
#51374=CARTESIAN_POINT('Ctrl Pts',(-8.87006237815579,31.8040591563383,25.8609848857952));
#51375=CARTESIAN_POINT('Ctrl Pts',(-8.85141893561129,31.8107119286145,25.8621716271334));
#51376=CARTESIAN_POINT('Ctrl Pts',(-8.79028772894628,31.8331316613072,25.866102885363));
#51377=CARTESIAN_POINT('Ctrl Pts',(-8.7480594590841,31.8495868026729,25.8688823919999));
#51378=CARTESIAN_POINT('Ctrl Pts',(-8.64431589011256,31.8924278146832,25.8758486544061));
#51379=CARTESIAN_POINT('Ctrl Pts',(-8.58322888800214,31.9197982201372,25.8800727175986));
#51380=CARTESIAN_POINT('Ctrl Pts',(-8.27084611525887,32.0710221917836,25.9021821167578));
#51381=CARTESIAN_POINT('Ctrl Pts',(-8.03475747257198,32.2238980568496,25.9205163153555));
#51382=CARTESIAN_POINT('Ctrl Pts',(-7.75821702137178,32.4561133559638,25.9429012316555));
#51383=CARTESIAN_POINT('Ctrl Pts',(-7.69814022995364,32.5103427116435,25.9478387935537));
#51384=CARTESIAN_POINT('Ctrl Pts',(-7.61666981971402,32.5893561432938,25.9546427523748));
#51385=CARTESIAN_POINT('Ctrl Pts',(-7.5936096050873,32.6123752533962,25.9565816731046));
#51386=CARTESIAN_POINT('Ctrl Pts',(-7.55207611508749,32.6550477883394,25.9600990507351));
#51387=CARTESIAN_POINT('Ctrl Pts',(-7.53349887165762,32.6745958485019,25.9616819085535));
#51388=CARTESIAN_POINT('Ctrl Pts',(-7.4961647475416,32.7148317984209,25.9648836561149));
#51389=CARTESIAN_POINT('Ctrl Pts',(-7.47742625546472,32.7355339586796,25.9665017111061));
#51390=CARTESIAN_POINT('Ctrl Pts',(-7.43097144619379,32.7881492519174,25.9705429348604));
#51391=CARTESIAN_POINT('Ctrl Pts',(-7.40359182095877,32.8203541037486,25.9729523388893));
#51392=CARTESIAN_POINT('Ctrl Pts',(-7.2853011931341,32.9648844789227,25.9835000321336));
#51393=CARTESIAN_POINT('Ctrl Pts',(-7.20102027088682,33.0824485999414,25.9913804870382));
#51394=CARTESIAN_POINT('Ctrl Pts',(-7.0544243131109,33.3172941839943,26.0062215062889));
#51395=CARTESIAN_POINT('Ctrl Pts',(-6.99098718101669,33.4335526628433,26.0131925154303));
#51396=CARTESIAN_POINT('Ctrl Pts',(-6.87006374622918,33.6897699226011,26.0282563326832));
#51397=CARTESIAN_POINT('Ctrl Pts',(-6.81482011967634,33.8304597850349,26.0363522214827));
#51398=CARTESIAN_POINT('Ctrl Pts',(-6.75825135522711,34.0086542694434,26.0469047037303));
#51399=CARTESIAN_POINT('Ctrl Pts',(-6.74790804294664,34.0431309808567,26.0489600331863));
#51400=CARTESIAN_POINT('Ctrl Pts',(-6.73319074922079,34.0951850355616,26.0520926126476));
#51401=CARTESIAN_POINT('Ctrl Pts',(-6.72840514697019,34.1126444419263,26.0531482322971));
#51402=CARTESIAN_POINT('Ctrl Pts',(-6.71996337684894,34.1444395539839,26.0550809198817));
#51403=CARTESIAN_POINT('Ctrl Pts',(-6.71626087657103,34.1587620608372,26.0559554100279));
#51404=CARTESIAN_POINT('Ctrl Pts',(-6.70786679777396,34.1921331275623,26.058001848591));
#51405=CARTESIAN_POINT('Ctrl Pts',(-6.70324672044636,34.2111985814637,26.0591776031071));
#51406=CARTESIAN_POINT('Ctrl Pts',(-6.68874025775819,34.2734163312111,26.0630335521217));
#51407=CARTESIAN_POINT('Ctrl Pts',(-6.6795340658647,34.3167207793455,26.0657469992499));
#51408=CARTESIAN_POINT('Ctrl Pts',(-6.65895655273479,34.4237821639482,26.0725080880666));
#51409=CARTESIAN_POINT('Ctrl Pts',(-6.64855941210567,34.4877076438142,26.076590496555));
#51410=CARTESIAN_POINT('Ctrl Pts',(-6.60654240728267,34.8027565724484,26.0968175771035));
#51411=CARTESIAN_POINT('Ctrl Pts',(-6.60128346208668,35.0566153876587,26.1133720840391));
#51412=CARTESIAN_POINT('Ctrl Pts',(-6.63379318920325,35.4121208727315,26.1357404985384));
#51413=CARTESIAN_POINT('Ctrl Pts',(-6.64800037936982,35.5150667980796,26.1421316293458));
#51414=CARTESIAN_POINT('Ctrl Pts',(-6.67408507685431,35.6559314352732,26.1507496210035));
#51415=CARTESIAN_POINT('Ctrl Pts',(-6.6819305894342,35.6945298457562,26.153098003867));
#51416=CARTESIAN_POINT('Ctrl Pts',(-6.69630519163327,35.7594337216339,26.1570262752042));
#51417=CARTESIAN_POINT('Ctrl Pts',(-6.7024801308566,35.785812789735,26.1586170789532));
#51418=CARTESIAN_POINT('Ctrl Pts',(-6.71562102871583,35.8390651589678,26.1618177213325));
#51419=CARTESIAN_POINT('Ctrl Pts',(-6.72260219383413,35.8659325926269,26.1634269411565));
#51420=CARTESIAN_POINT('Ctrl Pts',(-6.74082624985918,35.9326890201371,26.1674129572905));
#51421=CARTESIAN_POINT('Ctrl Pts',(-6.75247223380295,35.9724638608133,26.1697767964274));
#51422=CARTESIAN_POINT('Ctrl Pts',(-6.80488256715277,36.1400061541793,26.1796987879973));
#51423=CARTESIAN_POINT('Ctrl Pts',(-6.85248213256192,36.2655140600372,26.1870379992449));
#51424=CARTESIAN_POINT('Ctrl Pts',(-6.96430389757298,36.5146853749286,26.201723588649));
#51425=CARTESIAN_POINT('Ctrl Pts',(-7.02895615940997,36.6378711519729,26.2090467066191));
#51426=CARTESIAN_POINT('Ctrl Pts',(-7.18221366117368,36.8907801638766,26.2247588664028));
#51427=CARTESIAN_POINT('Ctrl Pts',(-7.27263037198655,37.0190133497008,26.2331464385165));
#51428=CARTESIAN_POINT('Ctrl Pts',(-7.39421745692432,37.1683144089255,26.2440160394932));
#51429=CARTESIAN_POINT('Ctrl Pts',(-7.4172919551955,37.195747931581,26.2460631948066));
#51430=CARTESIAN_POINT('Ctrl Pts',(-7.45264856404106,37.236455324781,26.2491857770703));
#51431=CARTESIAN_POINT('Ctrl Pts',(-7.46460962529923,37.2500060831041,26.2502397784419));
#51432=CARTESIAN_POINT('Ctrl Pts',(-7.48665377646385,37.2745810622936,26.2521794078705));
#51433=CARTESIAN_POINT('Ctrl Pts',(-7.4967021865019,37.2856352025265,26.2530625900414));
#51434=CARTESIAN_POINT('Ctrl Pts',(-7.52019932325557,37.3111433178607,26.2551254537146));
#51435=CARTESIAN_POINT('Ctrl Pts',(-7.53370156374956,37.3255465624326,26.2563089514506));
#51436=CARTESIAN_POINT('Ctrl Pts',(-7.57839552027932,37.3723959333416,26.260217860343));
#51437=CARTESIAN_POINT('Ctrl Pts',(-7.61010650921456,37.4043376239366,26.2629777411421));
#51438=CARTESIAN_POINT('Ctrl Pts',(-7.69006533416638,37.481733210946,26.2698828199203));
#51439=CARTESIAN_POINT('Ctrl Pts',(-7.73902777517446,37.5264207101726,26.2740645587824));
#51440=CARTESIAN_POINT('Ctrl Pts',(-7.99505183746927,37.7466852990106,26.2955733697877));
#51441=CARTESIAN_POINT('Ctrl Pts',(-8.22139470643331,37.8983945138822,26.313337773136));
#51442=CARTESIAN_POINT('Ctrl Pts',(-8.54216823478973,38.0615253975093,26.3357254568321));
#51443=CARTESIAN_POINT('Ctrl Pts',(-8.62246219390565,38.0984839708911,26.3411317933336));
#51444=CARTESIAN_POINT('Ctrl Pts',(-8.73839695488934,38.1464486775011,26.3486612393622));
#51445=CARTESIAN_POINT('Ctrl Pts',(-8.77291099435185,38.1600687112666,26.3508691982686));
#51446=CARTESIAN_POINT('Ctrl Pts',(-8.83288062143889,38.1826033852236,26.354649423319));
#51447=CARTESIAN_POINT('Ctrl Pts',(-8.8582312656269,38.191785733906,26.3562303505633));
#51448=CARTESIAN_POINT('Ctrl Pts',(-8.91054623081791,38.2100318661549,26.3594589051295));
#51449=CARTESIAN_POINT('Ctrl Pts',(-8.93752054364175,38.2190606663059,26.3611052910412));
#51450=CARTESIAN_POINT('Ctrl Pts',(-9.00730300704421,38.2414454142642,26.3653194339785));
#51451=CARTESIAN_POINT('Ctrl Pts',(-9.05026896558488,38.2542936130639,26.3678708067969));
#51452=CARTESIAN_POINT('Ctrl Pts',(-9.28072868080194,38.3182551428436,26.3813462136432));
#51453=CARTESIAN_POINT('Ctrl Pts',(-9.47210794703533,38.3540288363337,26.3917753520011));
#51454=CARTESIAN_POINT('Ctrl Pts',(-9.86973041572493,38.3934567282657,26.412995158163));
#51455=CARTESIAN_POINT('Ctrl Pts',(-10.07534386208,38.3951181844919,26.4237347825941));
#51456=CARTESIAN_POINT('Ctrl Pts',(-10.330320705509,38.3739977296586,26.4379718293838));
#51457=CARTESIAN_POINT('Ctrl Pts',(-10.3807143463015,38.3686834943876,26.4408320903622));
#51458=CARTESIAN_POINT('Ctrl Pts',(-10.4520586662249,38.3595386863507,26.4449709989678));
#51459=CARTESIAN_POINT('Ctrl Pts',(-10.473123681416,38.3566368815892,26.4462041897912));
#51460=CARTESIAN_POINT('Ctrl Pts',(-10.5091094067904,38.3513342163538,26.4483320651295));
#51461=CARTESIAN_POINT('Ctrl Pts',(-10.524043731852,38.3490314389279,26.4492214522734));
#51462=CARTESIAN_POINT('Ctrl Pts',(-10.5558900069774,38.3439027089257,26.4511321462089));
#51463=CARTESIAN_POINT('Ctrl Pts',(-10.5727959563151,38.3410483072142,26.4521548561418));
#51464=CARTESIAN_POINT('Ctrl Pts',(-10.6204532656969,38.3326295037993,26.4550601781411));
#51465=CARTESIAN_POINT('Ctrl Pts',(-10.6511496003247,38.3267680580755,26.4569578319867));
#51466=CARTESIAN_POINT('Ctrl Pts',(-10.7213255682068,38.3123595776737,26.4613499278876));
#51467=CARTESIAN_POINT('Ctrl Pts',(-10.7607419275674,38.3035296281939,26.463856181457));
#51468=CARTESIAN_POINT('Ctrl Pts',(-10.8955562134225,38.2707882572896,26.4725431510995));
#51469=CARTESIAN_POINT('Ctrl Pts',(-10.9900630250911,38.243431824829,26.478830806825));
#51470=CARTESIAN_POINT('Ctrl Pts',(-11.3181996510314,38.1327685586388,26.5011022942915));
#51471=CARTESIAN_POINT('Ctrl Pts',(-11.5437887770378,38.0279755606158,26.5171499893163));
#51472=CARTESIAN_POINT('Ctrl Pts',(-11.8162686423876,37.8629613558772,26.5367632981696));
#51473=CARTESIAN_POINT('Ctrl Pts',(-11.8754458527532,37.8245501338669,26.5410443860709));
#51474=CARTESIAN_POINT('Ctrl Pts',(-11.96085853744,37.7652409659417,26.5472576389746));
#51475=CARTESIAN_POINT('Ctrl Pts',(-11.9880490017677,37.7457576532585,26.5492410059997));
#51476=CARTESIAN_POINT('Ctrl Pts',(-12.0362389623791,37.7101359715483,26.5527671777657));
#51477=CARTESIAN_POINT('Ctrl Pts',(-12.057345830883,37.6941481561563,26.5543155221304));
#51478=CARTESIAN_POINT('Ctrl Pts',(-12.1020838324438,37.6594280899437,26.5576068484293));
#51479=CARTESIAN_POINT('Ctrl Pts',(-12.1256568148076,37.6406244326859,26.5593468731566));
#51480=CARTESIAN_POINT('Ctrl Pts',(-12.1900805896896,37.5878131685234,26.564120984843));
#51481=CARTESIAN_POINT('Ctrl Pts',(-12.2303881051556,37.5531547766629,26.5671291195338));
#51482=CARTESIAN_POINT('Ctrl Pts',(-12.401246492321,37.3991066755484,26.5800027459003));
#51483=CARTESIAN_POINT('Ctrl Pts',(-12.5231588145027,37.2705451671547,26.5894906968189));
#51484=CARTESIAN_POINT('Ctrl Pts',(-12.761688705398,36.9759408040542,26.6096249915204));
#51485=CARTESIAN_POINT('Ctrl Pts',(-12.8745708830499,36.8077874637358,26.6202034269639));
#51486=CARTESIAN_POINT('Ctrl Pts',(-12.9979583017571,36.5829117761982,26.6344372282672));
#51487=CARTESIAN_POINT('Ctrl Pts',(-13.02297040449,36.5346051403349,26.6375009887625));
#51488=CARTESIAN_POINT('Ctrl Pts',(-13.0563437455481,36.4661655087397,26.6418786968314));
#51489=CARTESIAN_POINT('Ctrl Pts',(-13.0656906446513,36.4465196880605,26.643139522253));
#51490=CARTESIAN_POINT('Ctrl Pts',(-13.0812398412988,36.4130098169372,26.6452994370896));
#51491=CARTESIAN_POINT('Ctrl Pts',(-13.087539397919,36.3991912532366,26.6461928208042));
#51492=CARTESIAN_POINT('Ctrl Pts',(-13.1006589900603,36.369892340669,26.648093450725));
#51493=CARTESIAN_POINT('Ctrl Pts',(-13.1074562483596,36.354402759637,26.6491018937862));
#51494=CARTESIAN_POINT('Ctrl Pts',(-13.1260474341217,36.3111604802397,26.6519259102269));
#51495=CARTESIAN_POINT('Ctrl Pts',(-13.1375871096232,36.2833009619197,26.6537552772376));
#51496=CARTESIAN_POINT('Ctrl Pts',(-13.1590745903235,36.2294021419145,26.6573084803199));
#51497=CARTESIAN_POINT('Ctrl Pts',(-13.1690741828736,36.203391072613,26.6590294020481));
#51498=CARTESIAN_POINT('Ctrl Pts',(-13.178750052031,36.1772651227369,26.6607620761902));
#51499=CARTESIAN_POINT('Origin',(-10.,35.,23.));
#51500=CARTESIAN_POINT('',(-13.1787500671536,36.1772650819043,27.9134187897562));
#51501=CARTESIAN_POINT('',(-13.1787501041618,36.1772649819778,27.5681446579994));
#51502=CARTESIAN_POINT('',(-13.1787500671536,36.1772650819043,23.));
#51503=CARTESIAN_POINT('Ctrl Pts',(-13.1787501041618,36.1772649819778,27.5681446579994));
#51504=CARTESIAN_POINT('Ctrl Pts',(-13.1644020558965,36.2160063533906,27.5655716628728));
#51505=CARTESIAN_POINT('Ctrl Pts',(-13.1493430220709,36.2544928168724,27.5630170421175));
#51506=CARTESIAN_POINT('Ctrl Pts',(-13.1093020225905,36.3515541614008,27.556579647575));
#51507=CARTESIAN_POINT('Ctrl Pts',(-13.0833705559431,36.4097108027348,27.5527276911668));
#51508=CARTESIAN_POINT('Ctrl Pts',(-13.0418761164669,36.4961390268219,27.5470088494505));
#51509=CARTESIAN_POINT('Ctrl Pts',(-13.0275237023559,36.5249729946894,27.5451018466481));
#51510=CARTESIAN_POINT('Ctrl Pts',(-13.0018381810593,36.5747827436353,27.5418080492359));
#51511=CARTESIAN_POINT('Ctrl Pts',(-12.9906908813596,36.595851261887,27.5404149881501));
#51512=CARTESIAN_POINT('Ctrl Pts',(-12.9649640131329,36.6432588482702,27.5372799027834));
#51513=CARTESIAN_POINT('Ctrl Pts',(-12.9502538263333,36.669524988143,27.5355425833204));
#51514=CARTESIAN_POINT('Ctrl Pts',(-12.9094257063638,36.7402014748802,27.5308644442906));
#51515=CARTESIAN_POINT('Ctrl Pts',(-12.8826415826952,36.7842188798417,27.5279473063303));
#51516=CARTESIAN_POINT('Ctrl Pts',(-12.7245416510446,37.0311827472875,27.5115250320381));
#51517=CARTESIAN_POINT('Ctrl Pts',(-12.5728206912721,37.2202331862985,27.4987999017403));
#51518=CARTESIAN_POINT('Ctrl Pts',(-12.2768441758102,37.5175365248139,27.4765345234232));
#51519=CARTESIAN_POINT('Ctrl Pts',(-12.141715186843,37.6334485909179,27.4670550970074));
#51520=CARTESIAN_POINT('Ctrl Pts',(-11.9741515042845,37.7557236460611,27.4552633861233));
#51521=CARTESIAN_POINT('Ctrl Pts',(-11.949934296921,37.7729123834219,27.4535581017219));
#51522=CARTESIAN_POINT('Ctrl Pts',(-11.9116532624196,37.7993338030989,27.4508555624415));
#51523=CARTESIAN_POINT('Ctrl Pts',(-11.8977406619426,37.808784130316,27.4498719623093));
#51524=CARTESIAN_POINT('Ctrl Pts',(-11.871101514872,37.826590873707,27.4479847820681));
#51525=CARTESIAN_POINT('Ctrl Pts',(-11.8583881346318,37.8349656704456,27.4470823941857));
#51526=CARTESIAN_POINT('Ctrl Pts',(-11.8301034720192,37.8533258692491,27.4450715141246));
#51527=CARTESIAN_POINT('Ctrl Pts',(-11.8145060099757,37.8632700083236,27.4439605018109));
#51528=CARTESIAN_POINT('Ctrl Pts',(-11.7600716163884,37.8973511802993,27.4400779309422));
#51529=CARTESIAN_POINT('Ctrl Pts',(-11.7208298036602,37.920828703608,27.4372699301773));
#51530=CARTESIAN_POINT('Ctrl Pts',(-11.4992048062422,38.0474056708746,27.4214112109975));
#51531=CARTESIAN_POINT('Ctrl Pts',(-11.3080503659179,38.1342134899517,27.4077641496928));
#51532=CARTESIAN_POINT('Ctrl Pts',(-11.0645838020527,38.2186004079409,27.3912144752835));
#51533=CARTESIAN_POINT('Ctrl Pts',(-11.0187199333602,38.2334095201176,27.3881296922592));
#51534=CARTESIAN_POINT('Ctrl Pts',(-10.8748282411207,38.2765054320731,27.3785672738993));
#51535=CARTESIAN_POINT('Ctrl Pts',(-10.7758241659961,38.3013500076338,27.3721550159289));
#51536=CARTESIAN_POINT('Ctrl Pts',(-10.6049382725524,38.3361190669073,27.3614064551439));
#51537=CARTESIAN_POINT('Ctrl Pts',(-10.5335856677132,38.3482724294034,27.357010886608));
#51538=CARTESIAN_POINT('Ctrl Pts',(-10.4284455187394,38.3627339321608,27.3506668669819));
#51539=CARTESIAN_POINT('Ctrl Pts',(-10.3949288408948,38.3668347739969,27.3486640528557));
#51540=CARTESIAN_POINT('Ctrl Pts',(-10.3350003600284,38.3732599071995,27.3451165732695));
#51541=CARTESIAN_POINT('Ctrl Pts',(-10.308612400127,38.3757763682488,27.3435661023063));
#51542=CARTESIAN_POINT('Ctrl Pts',(-10.2523492683192,38.3804765962723,27.3402838494633));
#51543=CARTESIAN_POINT('Ctrl Pts',(-10.2224690707656,38.3825744288559,27.3385548398914));
#51544=CARTESIAN_POINT('Ctrl Pts',(-10.1418306003378,38.3871627334773,27.3339243424286));
#51545=CARTESIAN_POINT('Ctrl Pts',(-10.0910367157713,38.3889083780982,27.3310456980157));
#51546=CARTESIAN_POINT('Ctrl Pts',(-9.79136243130594,38.3924643930525,27.3142523352531));
#51547=CARTESIAN_POINT('Ctrl Pts',(-9.54293663192563,38.3680036328702,27.3011748964854));
#51548=CARTESIAN_POINT('Ctrl Pts',(-9.18283425269056,38.2919359188974,27.281630270654));
#51549=CARTESIAN_POINT('Ctrl Pts',(-9.06764192911394,38.2611818699293,27.2752712826042));
#51550=CARTESIAN_POINT('Ctrl Pts',(-8.89128049273529,38.2039877261241,27.2650607504209));
#51551=CARTESIAN_POINT('Ctrl Pts',(-8.82886298743505,38.1817028847309,27.2613505344467));
#51552=CARTESIAN_POINT('Ctrl Pts',(-8.74593118652872,38.1493229430602,27.2562405951232));
#51553=CARTESIAN_POINT('Ctrl Pts',(-8.72480409780817,38.1408277474417,27.254922785503));
#51554=CARTESIAN_POINT('Ctrl Pts',(-8.68956942559027,38.1262457988304,27.2526955086954));
#51555=CARTESIAN_POINT('Ctrl Pts',(-8.67541431211795,38.1202746407128,27.2517926594589));
#51556=CARTESIAN_POINT('Ctrl Pts',(-8.64612540167611,38.1076842607834,27.2499068766235));
#51557=CARTESIAN_POINT('Ctrl Pts',(-8.63099872219983,38.1010503654269,27.2489231695905));
#51558=CARTESIAN_POINT('Ctrl Pts',(-8.59010257490957,38.082757580974,27.2462382656024));
#51559=CARTESIAN_POINT('Ctrl Pts',(-8.56443012585635,38.0708865291867,27.2445253039196));
#51560=CARTESIAN_POINT('Ctrl Pts',(-8.40825395622129,37.9962836885627,27.2339485776098));
#51561=CARTESIAN_POINT('Ctrl Pts',(-8.28174240922741,37.925569108145,27.2247143727789));
#51562=CARTESIAN_POINT('Ctrl Pts',(-7.94957210869555,37.7109064032872,27.199276412934));
#51563=CARTESIAN_POINT('Ctrl Pts',(-7.754709114995,37.5518560222649,27.18305415216));
#51564=CARTESIAN_POINT('Ctrl Pts',(-7.53140634715714,37.3240277613018,27.1634394493117));
#51565=CARTESIAN_POINT('Ctrl Pts',(-7.48513013212041,37.2738711930842,27.1593025439933));
#51566=CARTESIAN_POINT('Ctrl Pts',(-7.41873522160689,37.1974004792366,27.1532546627517));
#51567=CARTESIAN_POINT('Ctrl Pts',(-7.39743910987483,37.172135735042,27.1512963435665));
#51568=CARTESIAN_POINT('Ctrl Pts',(-7.35976917236088,37.1260963179081,27.1477973367732));
#51569=CARTESIAN_POINT('Ctrl Pts',(-7.34326287312982,37.1054339870156,27.1462514517745));
#51570=CARTESIAN_POINT('Ctrl Pts',(-7.30828608078966,37.0605842001141,27.1429470045155));
#51571=CARTESIAN_POINT('Ctrl Pts',(-7.28989601099042,37.0363367904838,27.1411916524712));
#51572=CARTESIAN_POINT('Ctrl Pts',(-7.24034935172679,36.9691489487084,27.1364096485186));
#51573=CARTESIAN_POINT('Ctrl Pts',(-7.20986971395812,36.925718747619,27.1334085524622));
#51574=CARTESIAN_POINT('Ctrl Pts',(-7.07251277690084,36.7198880915861,27.11956664319));
#51575=CARTESIAN_POINT('Ctrl Pts',(-6.97871098069999,36.5491993506769,27.1091945254157));
#51576=CARTESIAN_POINT('Ctrl Pts',(-6.83692802185636,36.2287087902784,27.0906067793392));
#51577=CARTESIAN_POINT('Ctrl Pts',(-6.78373414418195,36.0818402906496,27.0823834686507));
#51578=CARTESIAN_POINT('Ctrl Pts',(-6.71963273670488,35.857642677158,27.0696259765021));
#51579=CARTESIAN_POINT('Ctrl Pts',(-6.70096005667042,35.7827477730105,27.0653298627126));
#51580=CARTESIAN_POINT('Ctrl Pts',(-6.6798598236318,35.6838484005066,27.0595364743564));
#51581=CARTESIAN_POINT('Ctrl Pts',(-6.67510809459823,35.6603583672449,27.0581516520363));
#51582=CARTESIAN_POINT('Ctrl Pts',(-6.66767612221192,35.6215028990293,27.055843560445));
#51583=CARTESIAN_POINT('Ctrl Pts',(-6.66485204885391,35.6061653332914,27.0549280146077));
#51584=CARTESIAN_POINT('Ctrl Pts',(-6.6596654951604,35.5768631031551,27.0531694597432));
#51585=CARTESIAN_POINT('Ctrl Pts',(-6.65728451619725,35.5629021427547,27.0523275780995));
#51586=CARTESIAN_POINT('Ctrl Pts',(-6.65101480283981,35.5246962456425,27.0500134413177));
#51587=CARTESIAN_POINT('Ctrl Pts',(-6.64730199089043,35.5004238046987,27.048532027761));
#51588=CARTESIAN_POINT('Ctrl Pts',(-6.63316837427889,35.4007953650909,27.0424113529431));
#51589=CARTESIAN_POINT('Ctrl Pts',(-6.62502265743839,35.3251436393476,27.0376703232025));
#51590=CARTESIAN_POINT('Ctrl Pts',(-6.60425543679456,35.0435211784401,27.0198233656105));
#51591=CARTESIAN_POINT('Ctrl Pts',(-6.60789997071299,34.8368009088116,27.0063621847826));
#51592=CARTESIAN_POINT('Ctrl Pts',(-6.64805835080242,34.4693865817426,26.9827704669739));
#51593=CARTESIAN_POINT('Ctrl Pts',(-6.67750363943818,34.3085569921706,26.9725548286115));
#51594=CARTESIAN_POINT('Ctrl Pts',(-6.72933214669909,34.108356458548,26.9600657074071));
#51595=CARTESIAN_POINT('Ctrl Pts',(-6.74104113193493,34.0664670484797,26.9574644075734));
#51596=CARTESIAN_POINT('Ctrl Pts',(-6.7616570037712,33.9978357704238,26.9532204217887));
#51597=CARTESIAN_POINT('Ctrl Pts',(-6.77009672206383,33.970959966283,26.9515630685122));
#51598=CARTESIAN_POINT('Ctrl Pts',(-6.78722021490882,33.9187184810189,26.9483494745553));
#51599=CARTESIAN_POINT('Ctrl Pts',(-6.79587182008135,33.8933445261088,26.9467923357216));
#51600=CARTESIAN_POINT('Ctrl Pts',(-6.81743898512195,33.8324651265856,26.9430639190352));
#51601=CARTESIAN_POINT('Ctrl Pts',(-6.83064903740939,33.797067361924,26.9409023837029));
#51602=CARTESIAN_POINT('Ctrl Pts',(-6.87815973904472,33.6759769178717,26.9335228035249));
#51603=CARTESIAN_POINT('Ctrl Pts',(-6.91536770855719,33.5914655413139,26.9283994021722));
#51604=CARTESIAN_POINT('Ctrl Pts',(-7.07326268086494,33.2692001819934,26.908798880377));
#51605=CARTESIAN_POINT('Ctrl Pts',(-7.21836034386465,33.044512635551,26.8950687975203));
#51606=CARTESIAN_POINT('Ctrl Pts',(-7.43027435690701,32.7883814668859,26.8770628614091));
#51607=CARTESIAN_POINT('Ctrl Pts',(-7.47374557193833,32.738853362478,26.8734501106726));
#51608=CARTESIAN_POINT('Ctrl Pts',(-7.54916476029074,32.6578171542213,26.8672543205111));
#51609=CARTESIAN_POINT('Ctrl Pts',(-7.58034570596083,32.6256187003126,26.8647119332045));
#51610=CARTESIAN_POINT('Ctrl Pts',(-7.62614447078359,32.5801645702481,26.8609881662972));
#51611=CARTESIAN_POINT('Ctrl Pts',(-7.64025517303491,32.5664022740476,26.8598422467316));
#51612=CARTESIAN_POINT('Ctrl Pts',(-7.66526850837877,32.5424286300922,26.8578116110175));
#51613=CARTESIAN_POINT('Ctrl Pts',(-7.67611985515543,32.5321650711385,26.8569308223012));
#51614=CARTESIAN_POINT('Ctrl Pts',(-7.7002698022037,32.509623794949,26.8549705735495));
#51615=CARTESIAN_POINT('Ctrl Pts',(-7.7135989559906,32.4973808002714,26.8538887874433));
#51616=CARTESIAN_POINT('Ctrl Pts',(-7.75370965331564,32.4611265245754,26.8506355712557));
#51617=CARTESIAN_POINT('Ctrl Pts',(-7.78077521148381,32.4374348864085,26.8484432202856));
#51618=CARTESIAN_POINT('Ctrl Pts',(-7.92315383763938,32.3167521704878,26.8369476919827));
#51619=CARTESIAN_POINT('Ctrl Pts',(-8.04445579568718,32.2271046456035,26.8272858989504));
#51620=CARTESIAN_POINT('Ctrl Pts',(-8.28214658929394,32.0748139401915,26.8090999242139));
#51621=CARTESIAN_POINT('Ctrl Pts',(-8.39703335282622,32.0103120277561,26.8006003611032));
#51622=CARTESIAN_POINT('Ctrl Pts',(-8.64608555148325,31.8889779129413,26.7829989476883));
#51623=CARTESIAN_POINT('Ctrl Pts',(-8.78076070155903,31.8337708493311,26.7739469410946));
#51624=CARTESIAN_POINT('Ctrl Pts',(-8.95869955993819,31.7738737774273,26.7626203361656));
#51625=CARTESIAN_POINT('Ctrl Pts',(-8.99906970610587,31.7611212124363,26.7600904282288));
#51626=CARTESIAN_POINT('Ctrl Pts',(-9.066459874619,31.7412136844828,26.755931283695));
#51627=CARTESIAN_POINT('Ctrl Pts',(-9.09334757402283,31.7336309357148,26.754288533611));
#51628=CARTESIAN_POINT('Ctrl Pts',(-9.14635961059223,31.7193857579464,26.7510813700159));
#51629=CARTESIAN_POINT('Ctrl Pts',(-9.17247571667746,31.7127009047677,26.7495163459103));
#51630=CARTESIAN_POINT('Ctrl Pts',(-9.23028925957285,31.6986352157932,26.7460834597176));
#51631=CARTESIAN_POINT('Ctrl Pts',(-9.2620190447602,31.6913978365864,26.74422021691));
#51632=CARTESIAN_POINT('Ctrl Pts',(-9.37273548814627,31.6678160766798,26.7377863170969));
#51633=CARTESIAN_POINT('Ctrl Pts',(-9.45220018262722,31.6538339571314,26.7332882871803));
#51634=CARTESIAN_POINT('Ctrl Pts',(-9.80991657497855,31.6039789706991,26.7134478247527));
#51635=CARTESIAN_POINT('Ctrl Pts',(-10.0914517082179,31.5998944838945,26.6990262943814));
#51636=CARTESIAN_POINT('Ctrl Pts',(-10.4368149127558,31.6378459149163,26.6802201487411));
#51637=CARTESIAN_POINT('Ctrl Pts',(-10.5031297741189,31.6471285602743,26.6765517865612));
#51638=CARTESIAN_POINT('Ctrl Pts',(-10.6138089800698,31.6659786474563,26.6702708847003));
#51639=CARTESIAN_POINT('Ctrl Pts',(-10.6583358528913,31.6744845002267,26.6677004662677));
#51640=CARTESIAN_POINT('Ctrl Pts',(-10.7220433493207,31.6879839402809,26.663942941532));
#51641=CARTESIAN_POINT('Ctrl Pts',(-10.7413733646851,31.6922571939079,26.6627921893773));
#51642=CARTESIAN_POINT('Ctrl Pts',(-10.7752265327717,31.7000526992554,26.6607563750533));
#51643=CARTESIAN_POINT('Ctrl Pts',(-10.789765552222,31.7035020513524,26.6598753163988));
#51644=CARTESIAN_POINT('Ctrl Pts',(-10.8218010626107,31.7113265117992,26.6579187244417));
#51645=CARTESIAN_POINT('Ctrl Pts',(-10.8392855209772,31.7157451255028,26.6568409254977));
#51646=CARTESIAN_POINT('Ctrl Pts',(-10.8912166009179,31.7293107361177,26.6536118402494));
#51647=CARTESIAN_POINT('Ctrl Pts',(-10.9255540988702,31.7388614436303,26.6514400695276));
#51648=CARTESIAN_POINT('Ctrl Pts',(-11.0983743354471,31.7898792294697,26.6403451902187));
#51649=CARTESIAN_POINT('Ctrl Pts',(-11.2342449603887,31.8396306714422,26.6310912161772));
#51650=CARTESIAN_POINT('Ctrl Pts',(-11.479837990415,31.9478173169895,26.613810137012));
#51651=CARTESIAN_POINT('Ctrl Pts',(-11.5903452339949,32.0039120087511,26.6058089420885));
#51652=CARTESIAN_POINT('Ctrl Pts',(-11.7889214257883,32.1188003005747,26.5911836653386));
#51653=CARTESIAN_POINT('Ctrl Pts',(-11.8777914198948,32.1759153843919,26.5845374430253));
#51654=CARTESIAN_POINT('Ctrl Pts',(-12.0242455723205,32.2800139207113,26.5734515681327));
#51655=CARTESIAN_POINT('Ctrl Pts',(-12.0832144217084,32.32490872108,26.5689474367798));
#51656=CARTESIAN_POINT('Ctrl Pts',(-12.1670755064744,32.39321102412,26.562479842034));
#51657=CARTESIAN_POINT('Ctrl Pts',(-12.1931580262123,32.4151164408063,26.5604589388141));
#51658=CARTESIAN_POINT('Ctrl Pts',(-12.238967626392,32.454782287719,26.5568914823136));
#51659=CARTESIAN_POINT('Ctrl Pts',(-12.2588242792995,32.4723880500339,26.5553388759454));
#51660=CARTESIAN_POINT('Ctrl Pts',(-12.3005195117641,32.5102406322092,26.5520642595093));
#51661=CARTESIAN_POINT('Ctrl Pts',(-12.3223022462479,32.5305457906186,26.5503448579249));
#51662=CARTESIAN_POINT('Ctrl Pts',(-12.3808844902312,32.5866150286782,26.5456944654271));
#51663=CARTESIAN_POINT('Ctrl Pts',(-12.4171447564691,32.6229325651388,26.542787159267));
#51664=CARTESIAN_POINT('Ctrl Pts',(-12.6250174268864,32.840810802125,26.525911791026));
#51665=CARTESIAN_POINT('Ctrl Pts',(-12.7769577450057,33.0400685591439,26.5127880365558));
#51666=CARTESIAN_POINT('Ctrl Pts',(-12.9667207683926,33.3559064274085,26.4932199779168));
#51667=CARTESIAN_POINT('Ctrl Pts',(-13.0224293008694,33.4607164814866,26.4868879854454));
#51668=CARTESIAN_POINT('Ctrl Pts',(-13.1004418297251,33.6281278219799,26.4767152722671));
#51669=CARTESIAN_POINT('Ctrl Pts',(-13.1265970956252,33.6888317132664,26.4730146313256));
#51670=CARTESIAN_POINT('Ctrl Pts',(-13.159347324168,33.7714044156547,26.4679159140815));
#51671=CARTESIAN_POINT('Ctrl Pts',(-13.1675215079674,33.7926350755546,26.4665992928365));
#51672=CARTESIAN_POINT('Ctrl Pts',(-13.1808552114007,33.8283340536788,26.4643734342631));
#51673=CARTESIAN_POINT('Ctrl Pts',(-13.1861313654338,33.8427585036431,26.4634707955934));
#51674=CARTESIAN_POINT('Ctrl Pts',(-13.1968803537048,33.8727759126454,26.4615847677718));
#51675=CARTESIAN_POINT('Ctrl Pts',(-13.2023374458677,33.8883737154046,26.4606005970039));
#51676=CARTESIAN_POINT('Ctrl Pts',(-13.2168363153487,33.9308081847432,26.4579131069085));
#51677=CARTESIAN_POINT('Ctrl Pts',(-13.2256559906663,33.957718687971,26.456197986378));
#51678=CARTESIAN_POINT('Ctrl Pts',(-13.2797922067914,34.1301702577487,26.4451521429408));
#51679=CARTESIAN_POINT('Ctrl Pts',(-13.3155812426581,34.2785062403407,26.4354107616784));
#51680=CARTESIAN_POINT('Ctrl Pts',(-13.3733889843741,34.6166149298027,26.4133312549766));
#51681=CARTESIAN_POINT('Ctrl Pts',(-13.3896100389236,34.8068893592864,26.4010053753037));
#51682=CARTESIAN_POINT('Ctrl Pts',(-13.3898250631782,35.1016684315265,26.3825327747888));
#51683=CARTESIAN_POINT('Ctrl Pts',(-13.3851018672738,35.2057648191004,26.3761237399455));
#51684=CARTESIAN_POINT('Ctrl Pts',(-13.3719934711717,35.3487387793943,26.3674865606486));
#51685=CARTESIAN_POINT('Ctrl Pts',(-13.3677102660867,35.3879258514924,26.3651361613135));
#51686=CARTESIAN_POINT('Ctrl Pts',(-13.3596408924418,35.4514698737382,26.3613509560353));
#51687=CARTESIAN_POINT('Ctrl Pts',(-13.3562709876614,35.4758750658002,26.3599034550229));
#51688=CARTESIAN_POINT('Ctrl Pts',(-13.3486063500042,35.5272436884008,26.3568692292508));
#51689=CARTESIAN_POINT('Ctrl Pts',(-13.3442513026037,35.5541964300205,26.3552844929365));
#51690=CARTESIAN_POINT('Ctrl Pts',(-13.3328778060978,35.6195603568914,26.3514575704157));
#51691=CARTESIAN_POINT('Ctrl Pts',(-13.3255203152845,35.6579090489232,26.3492260812221));
#51692=CARTESIAN_POINT('Ctrl Pts',(-13.2949466182526,35.8036135565192,26.3407912840509));
#51693=CARTESIAN_POINT('Ctrl Pts',(-13.2671795835836,35.9099498061325,26.3347291378396));
#51694=CARTESIAN_POINT('Ctrl Pts',(-13.2171490333955,36.069410151205,26.3256643244751));
#51695=CARTESIAN_POINT('Ctrl Pts',(-13.1986266460729,36.1235960409069,26.3225880933694));
#51696=CARTESIAN_POINT('Ctrl Pts',(-13.1787501361565,36.1772648955886,26.3195304627418));
#51697=CARTESIAN_POINT('',(-13.3897497681227,35.0012537990022,26.7339821967504));
#51698=CARTESIAN_POINT('Ctrl Pts',(-13.178750052031,36.1772651227369,26.6607620761902));
#51699=CARTESIAN_POINT('Ctrl Pts',(-13.2278569142916,36.0446709959331,26.6695557244977));
#51700=CARTESIAN_POINT('Ctrl Pts',(-13.2686255387752,35.9091174585747,26.6786460656091));
#51701=CARTESIAN_POINT('Ctrl Pts',(-13.3456145540687,35.5796817978736,26.7004496954122));
#51702=CARTESIAN_POINT('Ctrl Pts',(-13.3736350392072,35.3844071259962,26.7131248457753));
#51703=CARTESIAN_POINT('Ctrl Pts',(-13.3879876626213,35.125729936053,26.7292118644511));
#51704=CARTESIAN_POINT('Ctrl Pts',(-13.3897235886384,35.0635844579724,26.7330266693701));
#51705=CARTESIAN_POINT('Ctrl Pts',(-13.3897497009126,35.0014239601829,26.7367916060834));
#51706=CARTESIAN_POINT('Ctrl Pts',(-13.3897497681227,35.0012537990022,26.7339821967504));
#51707=CARTESIAN_POINT('Ctrl Pts',(-13.3897890807757,34.8949687755281,26.7401898647473));
#51708=CARTESIAN_POINT('Ctrl Pts',(-13.3848252223009,34.7887128798793,26.7463975327442));
#51709=CARTESIAN_POINT('Ctrl Pts',(-13.3748927040089,34.6829758701176,26.7526052007411));
#51710=CARTESIAN_POINT('Ctrl Pts',(-13.3649548482759,34.5771820404203,26.7588162045549));
#51711=CARTESIAN_POINT('Ctrl Pts',(-13.3500430541169,34.4719080519769,26.7650272083686));
#51712=CARTESIAN_POINT('Ctrl Pts',(-13.3302435188436,34.3676368387545,26.7712382121823));
#51713=CARTESIAN_POINT('Ctrl Pts',(-13.3101893565392,34.2620246713595,26.7775290910759));
#51714=CARTESIAN_POINT('Ctrl Pts',(-13.2851209399016,34.1574416688483,26.7838199699694));
#51715=CARTESIAN_POINT('Ctrl Pts',(-13.255180393362,34.0543755136568,26.790110848863));
#51716=CARTESIAN_POINT('Ctrl Pts',(-13.2255498660534,33.9523765564249,26.7963365888842));
#51717=CARTESIAN_POINT('Ctrl Pts',(-13.1911478357508,33.851863538394,26.8025623289055));
#51718=CARTESIAN_POINT('Ctrl Pts',(-13.1521609227585,33.7532896970288,26.8087880689268));
#51719=CARTESIAN_POINT('Ctrl Pts',(-13.1125621394815,33.6531688133423,26.8151115172565));
#51720=CARTESIAN_POINT('Ctrl Pts',(-13.0682335274196,33.555048882714,26.8214349655862));
#51721=CARTESIAN_POINT('Ctrl Pts',(-13.0194189846875,33.4593786781273,26.8277584139158));
#51722=CARTESIAN_POINT('Ctrl Pts',(-12.9706044419554,33.3637084735407,26.8340818622455));
#51723=CARTESIAN_POINT('Ctrl Pts',(-12.917304237297,33.270488333665,26.8404053105752));
#51724=CARTESIAN_POINT('Ctrl Pts',(-12.8598073032452,33.1801353756927,26.8467287589049));
#51725=CARTESIAN_POINT('Ctrl Pts',(-12.8043271157467,33.0929516130794,26.8528304077103));
#51726=CARTESIAN_POINT('Ctrl Pts',(-12.7447627250487,33.0081598725026,26.8589320565156));
#51727=CARTESIAN_POINT('Ctrl Pts',(-12.6813468174437,32.9261667600589,26.865033705321));
#51728=CARTESIAN_POINT('Ctrl Pts',(-12.6180143250755,32.8442814987073,26.8711273282146));
#51729=CARTESIAN_POINT('Ctrl Pts',(-12.5508406470161,32.7651878825775,26.8772209511081));
#51730=CARTESIAN_POINT('Ctrl Pts',(-12.4801026278488,32.6892650481206,26.8833145740017));
#51731=CARTESIAN_POINT('Ctrl Pts',(-12.4094374149311,32.6134203563214,26.8894019251077));
#51732=CARTESIAN_POINT('Ctrl Pts',(-12.3352154458944,32.5407402680369,26.8954892762138));
#51733=CARTESIAN_POINT('Ctrl Pts',(-12.2577542980673,32.4715715173139,26.9015766273198));
#51734=CARTESIAN_POINT('Ctrl Pts',(-12.1803482539564,32.4024519713253,26.9076596480527));
#51735=CARTESIAN_POINT('Ctrl Pts',(-12.0997079314063,32.3368390797548,26.9137426687857));
#51736=CARTESIAN_POINT('Ctrl Pts',(-12.0161876933347,32.2750427071703,26.9198256895186));
#51737=CARTESIAN_POINT('Ctrl Pts',(-11.9326983778282,32.2132692140986,26.9259064580717));
#51738=CARTESIAN_POINT('Ctrl Pts',(-11.8463316094188,32.1553096858483,26.9319872266247));
#51739=CARTESIAN_POINT('Ctrl Pts',(-11.7574741265875,32.101433154665,26.9380679951777));
#51740=CARTESIAN_POINT('Ctrl Pts',(-11.6686265213304,32.0475626125038,26.9441480877804));
#51741=CARTESIAN_POINT('Ctrl Pts',(-11.5772891179794,31.9977743866539,26.9502281803831));
#51742=CARTESIAN_POINT('Ctrl Pts',(-11.4838760926028,31.9522931892484,26.9563082729858));
#51743=CARTESIAN_POINT('Ctrl Pts',(-11.3904492502357,31.9068052645875,26.9623892649126));
#51744=CARTESIAN_POINT('Ctrl Pts',(-11.2949465605175,31.865625821324,26.9684702568394));
#51745=CARTESIAN_POINT('Ctrl Pts',(-11.1978043188601,31.8289323759623,26.9745512487661));
#51746=CARTESIAN_POINT('Ctrl Pts',(-11.1005612478569,31.7922008444289,26.9806385524933));
#51747=CARTESIAN_POINT('Ctrl Pts',(-11.0016756272462,31.759964761198,26.9867258562204));
#51748=CARTESIAN_POINT('Ctrl Pts',(-10.9016011111557,31.7323524518604,26.9928131599476));
#51749=CARTESIAN_POINT('Ctrl Pts',(-10.8014728282463,31.704725307317,26.9989037341872));
#51750=CARTESIAN_POINT('Ctrl Pts',(-10.7001547947215,31.6817269797083,27.0049943084269));
#51751=CARTESIAN_POINT('Ctrl Pts',(-10.598111160826,31.6634346849199,27.0110848826666));
#51752=CARTESIAN_POINT('Ctrl Pts',(-10.4959009341694,31.64511252679,27.0171854001583));
#51753=CARTESIAN_POINT('Ctrl Pts',(-10.3929631650667,31.6315118056855,27.0232859176501));
#51754=CARTESIAN_POINT('Ctrl Pts',(-10.2897676713137,31.6226578853836,27.0293864351419));
#51755=CARTESIAN_POINT('Ctrl Pts',(-10.208448759635,31.6156809221767,27.034193693919));
#51756=CARTESIAN_POINT('Ctrl Pts',(-10.1269699497371,31.6116504791971,27.0390009526962));
#51757=CARTESIAN_POINT('Ctrl Pts',(-10.0455599792816,31.6105561885779,27.0438082114734));
#51758=CARTESIAN_POINT('Ctrl Pts',(-9.94222969237447,31.6091672510434,27.0499098649429));
#51759=CARTESIAN_POINT('Ctrl Pts',(-9.83866121416243,31.6125054504178,27.0560115184124));
#51760=CARTESIAN_POINT('Ctrl Pts',(-9.73532216908929,31.6205990607322,27.0621131718819));
#51761=CARTESIAN_POINT('Ctrl Pts',(-9.63211905207604,31.6286820250342,27.0682067994797));
#51762=CARTESIAN_POINT('Ctrl Pts',(-9.52914519108828,31.6415079318196,27.0743004270775));
#51763=CARTESIAN_POINT('Ctrl Pts',(-9.42686944164642,31.6590530645367,27.0803940546753));
#51764=CARTESIAN_POINT('Ctrl Pts',(-9.32469895763911,31.6765801392486,27.0864814105189));
#51765=CARTESIAN_POINT('Ctrl Pts',(-9.2232255757606,31.6988167094296,27.0925687663625));
#51766=CARTESIAN_POINT('Ctrl Pts',(-9.1229133792418,31.7256872290224,27.0986561222062));
#51767=CARTESIAN_POINT('Ctrl Pts',(-9.0226725414854,31.7525386338207,27.1047391477072));
#51768=CARTESIAN_POINT('Ctrl Pts',(-8.92359165844345,31.7840173224317,27.1108221732082));
#51769=CARTESIAN_POINT('Ctrl Pts',(-8.82612414125007,31.8199967718972,27.1169051987092));
#51770=CARTESIAN_POINT('Ctrl Pts',(-8.72869271016785,31.8559629004282,27.1229859720472));
#51771=CARTESIAN_POINT('Ctrl Pts',(-8.63287385862828,31.8964263300735,27.1290667453853));
#51772=CARTESIAN_POINT('Ctrl Pts',(-8.53910459385463,31.9412110771086,27.1351475187233));
#51773=CARTESIAN_POINT('Ctrl Pts',(-8.4453457524782,31.9859908458684,27.1412276161222));
#51774=CARTESIAN_POINT('Ctrl Pts',(-8.35363643080694,32.0350907924778,27.1473077135211));
#51775=CARTESIAN_POINT('Ctrl Pts',(-8.26439160825895,32.0882876905474,27.15338781092));
#51776=CARTESIAN_POINT('Ctrl Pts',(-8.17513358518265,32.1414924571648,27.1594688076484));
#51777=CARTESIAN_POINT('Ctrl Pts',(-8.08834115292697,32.1987951601621,27.1655498043767));
#51778=CARTESIAN_POINT('Ctrl Pts',(-8.00440194284902,32.2599282022554,27.1716308011051));
#51779=CARTESIAN_POINT('Ctrl Pts',(-7.920375607953,32.3211246974736,27.1777181096123));
#51780=CARTESIAN_POINT('Ctrl Pts',(-7.8392087560508,32.3861592192928,27.1838054181196));
#51781=CARTESIAN_POINT('Ctrl Pts',(-7.76125739204368,32.4547226874423,27.1898927266268));
#51782=CARTESIAN_POINT('Ctrl Pts',(-7.68326414736911,32.5233229924559,27.1959833056418));
#51783=CARTESIAN_POINT('Ctrl Pts',(-7.60849013968793,32.5954557234185,27.2020738846569));
#51784=CARTESIAN_POINT('Ctrl Pts',(-7.53725438080866,32.6707750049311,27.2081644636719));
#51785=CARTESIAN_POINT('Ctrl Pts',(-7.46590232575739,32.7462172491839,27.2142649858817));
#51786=CARTESIAN_POINT('Ctrl Pts',(-7.39810033851056,32.8248561122507,27.2203655080915));
#51787=CARTESIAN_POINT('Ctrl Pts',(-7.33412717001587,32.906312555119,27.2264660303013));
#51788=CARTESIAN_POINT('Ctrl Pts',(-7.28371631591037,32.9705002287016,27.2312732415481));
#51789=CARTESIAN_POINT('Ctrl Pts',(-7.23568214943518,33.0364367761876,27.236080452795));
#51790=CARTESIAN_POINT('Ctrl Pts',(-7.19014138143131,33.1039252108223,27.2408876640418));
#51791=CARTESIAN_POINT('Ctrl Pts',(-7.13233799108828,33.1895860483931,27.2469892982554));
#51792=CARTESIAN_POINT('Ctrl Pts',(-7.07835764615036,33.278037335163,27.253090932469));
#51793=CARTESIAN_POINT('Ctrl Pts',(-7.0284803286951,33.3689034652884,27.2591925666825));
#51794=CARTESIAN_POINT('Ctrl Pts',(-6.97866861832966,33.4596500729001,27.265286174994));
#51795=CARTESIAN_POINT('Ctrl Pts',(-6.93294941010423,33.5528048372231,27.2713797833055));
#51796=CARTESIAN_POINT('Ctrl Pts',(-6.89155987761914,33.6479626232708,27.277473391617));
#51797=CARTESIAN_POINT('Ctrl Pts',(-6.85021294471852,33.7430224695278,27.2835607281693));
#51798=CARTESIAN_POINT('Ctrl Pts',(-6.81318699597916,33.8400808478651,27.2896480647216));
#51799=CARTESIAN_POINT('Ctrl Pts',(-6.78067324037895,33.9387082035143,27.2957354012739));
#51800=CARTESIAN_POINT('Ctrl Pts',(-6.74818261367836,34.0372653998673,27.3018184075545));
#51801=CARTESIAN_POINT('Ctrl Pts',(-6.7201979307338,34.1373889490011,27.3079014138351));
#51802=CARTESIAN_POINT('Ctrl Pts',(-6.69686191490677,34.2386302781784,27.3139844201157));
#51803=CARTESIAN_POINT('Ctrl Pts',(-6.67353453877915,34.3398341247513,27.3200651742832));
#51804=CARTESIAN_POINT('Ctrl Pts',(-6.65485250520525,34.4421545125211,27.3261459284507));
#51805=CARTESIAN_POINT('Ctrl Pts',(-6.64090817798173,34.5451294758395,27.3322266826183));
#51806=CARTESIAN_POINT('Ctrl Pts',(-6.62696540064945,34.648092993644,27.338306760919));
#51807=CARTESIAN_POINT('Ctrl Pts',(-6.61775933994476,34.7517105184419,27.3443868392198));
#51808=CARTESIAN_POINT('Ctrl Pts',(-6.61333077242632,34.855512611258,27.3504669175205));
#51809=CARTESIAN_POINT('Ctrl Pts',(-6.60890154979115,34.9593300594879,27.3565478952455));
#51810=CARTESIAN_POINT('Ctrl Pts',(-6.6092512426745,35.063331702573,27.3626288729705));
#51811=CARTESIAN_POINT('Ctrl Pts',(-6.61436852588733,35.1670466521595,27.3687098506955));
#51812=CARTESIAN_POINT('Ctrl Pts',(-6.61949112082979,35.2708692576538,27.3747971404631));
#51813=CARTESIAN_POINT('Ctrl Pts',(-6.62939116804803,35.3744041472782,27.3808844302306));
#51814=CARTESIAN_POINT('Ctrl Pts',(-6.64400531070665,35.4771841446809,27.3869717199982));
#51815=CARTESIAN_POINT('Ctrl Pts',(-6.65862730536355,35.5800193645063,27.3930622803914));
#51816=CARTESIAN_POINT('Ctrl Pts',(-6.67796836100029,35.682098463848,27.3991528407845));
#51817=CARTESIAN_POINT('Ctrl Pts',(-6.70191406814667,35.7829650366467,27.4052434011777));
#51818=CARTESIAN_POINT('Ctrl Pts',(-6.72589886957236,35.8839962863934,27.4113439051514));
#51819=CARTESIAN_POINT('Ctrl Pts',(-6.75450322260136,35.9838106434497,27.4174444091252));
#51820=CARTESIAN_POINT('Ctrl Pts',(-6.78756291115494,36.0819671957655,27.4235449130989));
#51821=CARTESIAN_POINT('Ctrl Pts',(-6.81361505145846,36.159317841961,27.4283523142694));
#51822=CARTESIAN_POINT('Ctrl Pts',(-6.84243293212115,36.2356392854295,27.4331597154398));
#51823=CARTESIAN_POINT('Ctrl Pts',(-6.87391576260421,36.3107259069712,27.4379671166102));
#51824=CARTESIAN_POINT('Ctrl Pts',(-6.91387445338392,36.4060274743921,27.444068774367));
#51825=CARTESIAN_POINT('Ctrl Pts',(-6.95826267810669,36.4996611620125,27.4501704321238));
#51826=CARTESIAN_POINT('Ctrl Pts',(-7.00691976467638,36.5911869052425,27.4562720898807));
#51827=CARTESIAN_POINT('Ctrl Pts',(-7.05551284871861,36.6825922573988,27.4623657216428));
#51828=CARTESIAN_POINT('Ctrl Pts',(-7.10836343232686,36.7718948029809,27.4684593534049));
#51829=CARTESIAN_POINT('Ctrl Pts',(-7.1652626800912,36.8586740945137,27.474552985167));
#51830=CARTESIAN_POINT('Ctrl Pts',(-7.22210336421032,36.9453640683166,27.4806403450485));
#51831=CARTESIAN_POINT('Ctrl Pts',(-7.28298419289195,37.0295355965252,27.4867277049301));
#51832=CARTESIAN_POINT('Ctrl Pts',(-7.34765071064495,37.1107932892062,27.4928150648116));
#51833=CARTESIAN_POINT('Ctrl Pts',(-7.41227122464338,37.1919931751722,27.4988980941459));
#51834=CARTESIAN_POINT('Ctrl Pts',(-7.4806718065959,37.2702830140263,27.5049811234801));
#51835=CARTESIAN_POINT('Ctrl Pts',(-7.55255551693585,37.3452975429183,27.5110641528144));
#51836=CARTESIAN_POINT('Ctrl Pts',(-7.62441261176841,37.4202842970929,27.5171449298594));
#51837=CARTESIAN_POINT('Ctrl Pts',(-7.69974997624432,37.4919978429857,27.5232257069043));
#51838=CARTESIAN_POINT('Ctrl Pts',(-7.77823186408501,37.5601076955341,27.5293064839493));
#51839=CARTESIAN_POINT('Ctrl Pts',(-7.85670502620347,37.6282099755372,27.5353865849253));
#51840=CARTESIAN_POINT('Ctrl Pts',(-7.93832169342656,37.6927090785546,27.5414666859013));
#51841=CARTESIAN_POINT('Ctrl Pts',(-8.02271159073161,37.7533135689697,27.5475467868772));
#51842=CARTESIAN_POINT('Ctrl Pts',(-8.1071139685944,37.8139270222806,27.5536277870491));
#51843=CARTESIAN_POINT('Ctrl Pts',(-8.19429004390403,37.8706444691265,27.559708787221));
#51844=CARTESIAN_POINT('Ctrl Pts',(-8.28383976907246,37.9232172557446,27.5657897873929));
#51845=CARTESIAN_POINT('Ctrl Pts',(-8.37348243910881,37.9758446083672,27.5718770991169));
#51846=CARTESIAN_POINT('Ctrl Pts',(-8.46550330951064,38.0243184927264,27.5779644108409));
#51847=CARTESIAN_POINT('Ctrl Pts',(-8.55947691538168,38.0684358075706,27.5840517225649));
#51848=CARTESIAN_POINT('Ctrl Pts',(-8.65350100824729,38.1125768242897,27.5901423046761));
#51849=CARTESIAN_POINT('Ctrl Pts',(-8.74947953108165,38.1523564454947,27.5962328867873));
#51850=CARTESIAN_POINT('Ctrl Pts',(-8.84696804158223,38.1876201726942,27.6023234688984));
#51851=CARTESIAN_POINT('Ctrl Pts',(-8.9446157035233,38.2229414684519,27.6084239939753));
#51852=CARTESIAN_POINT('Ctrl Pts',(-9.04377786880567,38.253732015688,27.6145245190522));
#51853=CARTESIAN_POINT('Ctrl Pts',(-9.14399575154938,38.2798874659254,27.6206250441291));
#51854=CARTESIAN_POINT('Ctrl Pts',(-9.22296680667401,38.3004977946009,27.6254322191456));
#51855=CARTESIAN_POINT('Ctrl Pts',(-9.30259308127847,38.3182310356037,27.6302393941621));
#51856=CARTESIAN_POINT('Ctrl Pts',(-9.38264738477849,38.3330587770064,27.6350465691787));
#51857=CARTESIAN_POINT('Ctrl Pts',(-9.48425923743688,38.351879430098,27.6411482518881));
#51858=CARTESIAN_POINT('Ctrl Pts',(-9.58690422830258,38.3660810321104,27.6472499345976));
#51859=CARTESIAN_POINT('Ctrl Pts',(-9.69012622107235,38.3755567398035,27.653351617307));
#51860=CARTESIAN_POINT('Ctrl Pts',(-9.79321244377338,38.3850199838981,27.6594452743442));
#51861=CARTESIAN_POINT('Ctrl Pts',(-9.89687373720429,38.3897696526902,27.6655389313814));
#51862=CARTESIAN_POINT('Ctrl Pts',(-10.0006439713222,38.3897499388304,27.6716325884186));
#51863=CARTESIAN_POINT('Ctrl Pts',(-10.1043074050542,38.3897302452602,27.6777199738605));
#51864=CARTESIAN_POINT('Ctrl Pts',(-10.208079131036,38.384950930002,27.6838073593023));
#51865=CARTESIAN_POINT('Ctrl Pts',(-10.3114889697607,38.3754080766949,27.6898947447441));
#51866=CARTESIAN_POINT('Ctrl Pts',(-10.4148252484858,38.3658720116422,27.6959777999589));
#51867=CARTESIAN_POINT('Ctrl Pts',(-10.5177997271705,38.351579186081,27.7020608551738));
#51868=CARTESIAN_POINT('Ctrl Pts',(-10.6199441358344,38.332577730668,27.7081439103886));
#51869=CARTESIAN_POINT('Ctrl Pts',(-10.7220507280278,38.3135833100795,27.714224713501));
#51870=CARTESIAN_POINT('Ctrl Pts',(-10.8233274408911,38.2898838024001,27.7203055166133));
#51871=CARTESIAN_POINT('Ctrl Pts',(-10.9233138194449,38.2615788589764,27.7263863197257));
#51872=CARTESIAN_POINT('Ctrl Pts',(-11.0232890839676,38.2332770618016,27.7324664469236));
#51873=CARTESIAN_POINT('Ctrl Pts',(-11.1219738878181,38.2003709633452,27.7385465741215));
#51874=CARTESIAN_POINT('Ctrl Pts',(-11.2189215086733,38.1630104992228,27.7446267013194));
#51875=CARTESIAN_POINT('Ctrl Pts',(-11.3158834691591,38.1256445090725,27.7507077278358));
#51876=CARTESIAN_POINT('Ctrl Pts',(-11.4111073369849,38.0838229981179,27.7567887543521));
#51877=CARTESIAN_POINT('Ctrl Pts',(-11.5041658512638,38.0377442542768,27.7628697808684));
#51878=CARTESIAN_POINT('Ctrl Pts',(-11.597320952198,37.9916176847017,27.7689571189621));
#51879=CARTESIAN_POINT('Ctrl Pts',(-11.6883058271688,37.9412252480255,27.7750444570557));
#51880=CARTESIAN_POINT('Ctrl Pts',(-11.7767173813687,37.8868114606331,27.7811317951494));
#51881=CARTESIAN_POINT('Ctrl Pts',(-11.86517643494,37.832368439271,27.7872224036837));
#51882=CARTESIAN_POINT('Ctrl Pts',(-11.9510590602153,37.7739000044431,27.7933130122179));
#51883=CARTESIAN_POINT('Ctrl Pts',(-12.03399240966,37.7116931869121,27.7994036207521));
#51884=CARTESIAN_POINT('Ctrl Pts',(-12.1170611458879,37.649384818184,27.8055041720646));
#51885=CARTESIAN_POINT('Ctrl Pts',(-12.1971706578459,37.5833261474703,27.811604723377));
#51886=CARTESIAN_POINT('Ctrl Pts',(-12.2739821794322,37.5138436924608,27.8177052746894));
#51887=CARTESIAN_POINT('Ctrl Pts',(-12.3345056451099,37.4590951483085,27.8225121903753));
#51888=CARTESIAN_POINT('Ctrl Pts',(-12.3929821821247,37.402221717251,27.8273191060612));
#51889=CARTESIAN_POINT('Ctrl Pts',(-12.4492635142395,37.3433978109393,27.8321260217471));
#51890=CARTESIAN_POINT('Ctrl Pts',(-12.5197884181869,37.2696868629828,27.8381494624564));
#51891=CARTESIAN_POINT('Ctrl Pts',(-12.5871173059483,37.1926485687336,27.8441729031657));
#51892=CARTESIAN_POINT('Ctrl Pts',(-12.6509144165922,37.1125950436379,27.8501963438749));
#51893=CARTESIAN_POINT('Ctrl Pts',(-12.7146125115311,37.0326657648623,27.8562104359597));
#51894=CARTESIAN_POINT('Ctrl Pts',(-12.7747894584714,36.9497309025452,27.8622245280446));
#51895=CARTESIAN_POINT('Ctrl Pts',(-12.8311464857577,36.8641391146269,27.8682386201294));
#51896=CARTESIAN_POINT('Ctrl Pts',(-12.887452973542,36.7786240831761,27.8742473189344));
#51897=CARTESIAN_POINT('Ctrl Pts',(-12.9399461035467,36.6904572226187,27.8802560177393));
#51898=CARTESIAN_POINT('Ctrl Pts',(-12.9883678913794,36.6000195024663,27.8862647165443));
#51899=CARTESIAN_POINT('Ctrl Pts',(-13.0367575357117,36.50964181696,27.8922694266363));
#51900=CARTESIAN_POINT('Ctrl Pts',(-13.0810810016637,36.4169966542195,27.8982741367283));
#51901=CARTESIAN_POINT('Ctrl Pts',(-13.1211247158629,36.3224921816516,27.9042788468204));
#51902=CARTESIAN_POINT('Ctrl Pts',(-13.1414419477865,36.2745428511419,27.9073254944656));
#51903=CARTESIAN_POINT('Ctrl Pts',(-13.160658162689,36.2261152885534,27.9103721421109));
#51904=CARTESIAN_POINT('Ctrl Pts',(-13.1787500671536,36.1772650819042,27.9134187897562));
#51905=CARTESIAN_POINT('Origin',(-10.,35.,23.));
#51906=CARTESIAN_POINT('',(-13.1787500528927,36.1772651204102,29.1634930667589));
#51907=CARTESIAN_POINT('',(-13.1787500671537,36.177265081904,28.8235277009158));
#51908=CARTESIAN_POINT('',(-13.1787500671536,36.1772650819043,23.));
#51909=CARTESIAN_POINT('',(-7.42676557298528,37.2065515280922,30.));
#51910=CARTESIAN_POINT('Ctrl Pts',(-7.42676557298526,37.2065515280922,30.));
#51911=CARTESIAN_POINT('Ctrl Pts',(-7.42044787186859,37.1991839566551,29.9994303932239));
#51912=CARTESIAN_POINT('Ctrl Pts',(-7.41416177089548,37.1917892038426,29.9988626237233));
#51913=CARTESIAN_POINT('Ctrl Pts',(-7.40027527655973,37.1753107133754,29.9976058906998));
#51914=CARTESIAN_POINT('Ctrl Pts',(-7.39269053096667,37.1662139038115,29.9969177930047));
#51915=CARTESIAN_POINT('Ctrl Pts',(-7.36359004725985,37.1309377951778,29.994270531793));
#51916=CARTESIAN_POINT('Ctrl Pts',(-7.34241906846593,37.1044754836715,29.9923291917595));
#51917=CARTESIAN_POINT('Ctrl Pts',(-7.2301273078817,36.9597207178191,29.9819237473292));
#51918=CARTESIAN_POINT('Ctrl Pts',(-7.14649535007684,36.8358152200063,29.9737735088464));
#51919=CARTESIAN_POINT('Ctrl Pts',(-6.99394268335336,36.5740487549211,29.9573004080105));
#51920=CARTESIAN_POINT('Ctrl Pts',(-6.92569854003083,36.4362028734202,29.9489953670567));
#51921=CARTESIAN_POINT('Ctrl Pts',(-6.83268627949556,36.2110431793853,29.9355077349894));
#51922=CARTESIAN_POINT('Ctrl Pts',(-6.80165808509507,36.1265474919904,29.9304643713169));
#51923=CARTESIAN_POINT('Ctrl Pts',(-6.76217732629905,36.0041907195728,29.923124350649));
#51924=CARTESIAN_POINT('Ctrl Pts',(-6.7509539859517,35.9672613470769,29.9209045127161));
#51925=CARTESIAN_POINT('Ctrl Pts',(-6.73224036891425,35.9016809286153,29.9169499801724));
#51926=CARTESIAN_POINT('Ctrl Pts',(-6.72449028298769,35.8731079678905,29.9152228946107));
#51927=CARTESIAN_POINT('Ctrl Pts',(-6.70890731199449,35.8125267203424,29.9115503843584));
#51928=CARTESIAN_POINT('Ctrl Pts',(-6.70116494633203,35.7804985172093,29.9096025428753));
#51929=CARTESIAN_POINT('Ctrl Pts',(-6.68142266347274,35.6932813309301,29.9042785794563));
#51930=CARTESIAN_POINT('Ctrl Pts',(-6.67033349861846,35.6378988872998,29.9008764684895));
#51931=CARTESIAN_POINT('Ctrl Pts',(-6.60768262401444,35.2785894246722,29.8786459957547));
#51932=CARTESIAN_POINT('Ctrl Pts',(-6.59641207396922,34.9691496330044,29.8585946837763));
#51933=CARTESIAN_POINT('Ctrl Pts',(-6.64229018594765,34.5106134504596,29.8287625927251));
#51934=CARTESIAN_POINT('Ctrl Pts',(-6.66773753543461,34.3598823643459,29.8189728421815));
#51935=CARTESIAN_POINT('Ctrl Pts',(-6.70996561949286,34.1833553682101,29.8078529773363));
#51936=CARTESIAN_POINT('Ctrl Pts',(-6.71702372747825,34.1554281587476,29.8061045002741));
#51937=CARTESIAN_POINT('Ctrl Pts',(-6.72873899736422,34.1114416756164,29.8033709372274));
#51938=CARTESIAN_POINT('Ctrl Pts',(-6.73316029745685,34.0953216995518,29.8023735063816));
#51939=CARTESIAN_POINT('Ctrl Pts',(-6.74176270860991,34.064843096824,29.8004966956275));
#51940=CARTESIAN_POINT('Ctrl Pts',(-6.7459197690407,34.0504787783796,29.7996161030741));
#51941=CARTESIAN_POINT('Ctrl Pts',(-6.75629356760114,34.0155015871302,29.7974812803449));
#51942=CARTESIAN_POINT('Ctrl Pts',(-6.76261179601755,33.9949197966454,29.7962329050143));
#51943=CARTESIAN_POINT('Ctrl Pts',(-6.78594519021965,33.9214143493779,29.7917978131322));
#51944=CARTESIAN_POINT('Ctrl Pts',(-6.80406637841891,33.8688482188654,29.7886696479653));
#51945=CARTESIAN_POINT('Ctrl Pts',(-6.89322020342415,33.6295081292945,29.7745239865511));
#51946=CARTESIAN_POINT('Ctrl Pts',(-6.97939137300909,33.4487857673895,29.7640987033258));
#51947=CARTESIAN_POINT('Ctrl Pts',(-7.14589102066328,33.1667610831271,29.7467532846791));
#51948=CARTESIAN_POINT('Ctrl Pts',(-7.21694898265522,33.060585862539,29.7399459310837));
#51949=CARTESIAN_POINT('Ctrl Pts',(-7.34395608773212,32.8922128759651,29.7283946348034));
#51950=CARTESIAN_POINT('Ctrl Pts',(-7.39651860311298,32.8276236744837,29.7237618910563));
#51951=CARTESIAN_POINT('Ctrl Pts',(-7.47418650544213,32.739056525246,29.7170706588259));
#51952=CARTESIAN_POINT('Ctrl Pts',(-7.49736585125607,32.7134258390944,29.7150918567539));
#51953=CARTESIAN_POINT('Ctrl Pts',(-7.53838042752792,32.6694445629033,29.711618665269));
#51954=CARTESIAN_POINT('Ctrl Pts',(-7.55603934628222,32.6509329866654,29.7101320156842));
#51955=CARTESIAN_POINT('Ctrl Pts',(-7.59302291324448,32.6130321216308,29.7070352759142));
#51956=CARTESIAN_POINT('Ctrl Pts',(-7.61237622756455,32.5936735464382,29.7054239456122));
#51957=CARTESIAN_POINT('Ctrl Pts',(-7.66334213201807,32.5439139874644,29.7012029078186));
#51958=CARTESIAN_POINT('Ctrl Pts',(-7.69531323036121,32.5138891612483,29.6985767347992));
#51959=CARTESIAN_POINT('Ctrl Pts',(-7.85832597731241,32.3666470804838,29.6852872972427));
#51960=CARTESIAN_POINT('Ctrl Pts',(-7.99774650970611,32.2591460760691,29.6742181312849));
#51961=CARTESIAN_POINT('Ctrl Pts',(-8.31022565522744,32.0548160388896,29.6501911371802));
#51962=CARTESIAN_POINT('Ctrl Pts',(-8.48473044029537,31.9613484769058,29.63721135416));
#51963=CARTESIAN_POINT('Ctrl Pts',(-8.72024718768592,31.8605620443076,29.6208810910153));
#51964=CARTESIAN_POINT('Ctrl Pts',(-8.77470449408973,31.8389100633464,29.617184874961));
#51965=CARTESIAN_POINT('Ctrl Pts',(-8.86804894544407,31.8045717551782,29.6110143771785));
#51966=CARTESIAN_POINT('Ctrl Pts',(-8.90665343930957,31.7911577639238,29.608509339066));
#51967=CARTESIAN_POINT('Ctrl Pts',(-8.96296752398051,31.7727245570946,29.6049324284727));
#51968=CARTESIAN_POINT('Ctrl Pts',(-8.98048881279557,31.7671467531446,29.6038302571288));
#51969=CARTESIAN_POINT('Ctrl Pts',(-9.01199194320197,31.7573995045647,29.6018688893715));
#51970=CARTESIAN_POINT('Ctrl Pts',(-9.02595653883095,31.7531773630961,29.6010066499992));
#51971=CARTESIAN_POINT('Ctrl Pts',(-9.05730530849841,31.7439196375393,29.5990862906916));
#51972=CARTESIAN_POINT('Ctrl Pts',(-9.07470368620323,31.7389327863549,29.5980309472168));
#51973=CARTESIAN_POINT('Ctrl Pts',(-9.1257739054026,31.7247362951594,29.5949614409659));
#51974=CARTESIAN_POINT('Ctrl Pts',(-9.1595500061878,31.7159068821048,29.5929672208399));
#51975=CARTESIAN_POINT('Ctrl Pts',(-9.33016597049147,31.6741109306034,29.5830459396973));
#51976=CARTESIAN_POINT('Ctrl Pts',(-9.4688406102282,31.6491653649432,29.5754687058191));
#51977=CARTESIAN_POINT('Ctrl Pts',(-9.8580781706075,31.6039280059719,29.5546030013781));
#51978=CARTESIAN_POINT('Ctrl Pts',(-10.1099113486465,31.6027422679523,29.5415006238399));
#51979=CARTESIAN_POINT('Ctrl Pts',(-10.4241097814455,31.636259587128,29.5239583435427));
#51980=CARTESIAN_POINT('Ctrl Pts',(-10.4884416191561,31.6449973609881,29.520307208312));
#51981=CARTESIAN_POINT('Ctrl Pts',(-10.5847409741776,31.660905480538,29.5147328332933));
#51982=CARTESIAN_POINT('Ctrl Pts',(-10.6169220393908,31.6667011372861,29.5128516084428));
#51983=CARTESIAN_POINT('Ctrl Pts',(-10.6727287650557,31.677587489654,29.5095551455745));
#51984=CARTESIAN_POINT('Ctrl Pts',(-10.69639347101,31.6824670356265,29.5081465433602));
#51985=CARTESIAN_POINT('Ctrl Pts',(-10.7497964823286,31.6940750379833,29.5049426189362));
#51986=CARTESIAN_POINT('Ctrl Pts',(-10.7794999355984,31.7009525041008,29.5031427660733));
#51987=CARTESIAN_POINT('Ctrl Pts',(-10.8598040498489,31.7206909797798,29.4982269605688));
#51988=CARTESIAN_POINT('Ctrl Pts',(-10.9102053492972,31.7343214438424,29.4950874658728));
#51989=CARTESIAN_POINT('Ctrl Pts',(-11.1668290533207,31.8101246808292,29.4788174245134));
#51990=CARTESIAN_POINT('Ctrl Pts',(-11.3670760940175,31.8906794914953,29.4651240321363));
#51991=CARTESIAN_POINT('Ctrl Pts',(-11.6765185520715,32.0508627371648,29.442757184862));
#51992=CARTESIAN_POINT('Ctrl Pts',(-11.7910317449351,32.1189701916702,29.4341939055577));
#51993=CARTESIAN_POINT('Ctrl Pts',(-11.9597299130344,32.2332593221212,29.4213828282598));
#51994=CARTESIAN_POINT('Ctrl Pts',(-12.0169651572732,32.2747021808372,29.4170001106056));
#51995=CARTESIAN_POINT('Ctrl Pts',(-12.0915185977888,32.3323211035021,29.4112841620895));
#51996=CARTESIAN_POINT('Ctrl Pts',(-12.1100199525093,32.3469307197105,29.4098651015657));
#51997=CARTESIAN_POINT('Ctrl Pts',(-12.1406319303622,32.3716263027181,29.4075182790486));
#51998=CARTESIAN_POINT('Ctrl Pts',(-12.1528271153108,32.3816056843917,29.4065836590477));
#51999=CARTESIAN_POINT('Ctrl Pts',(-12.1777639627951,32.4023036378329,29.4046739529542));
#52000=CARTESIAN_POINT('Ctrl Pts',(-12.190497105323,32.4130317503896,29.4036995700603));
#52001=CARTESIAN_POINT('Ctrl Pts',(-12.2247738913503,32.4423456633217,29.4010770272111));
#52002=CARTESIAN_POINT('Ctrl Pts',(-12.2461638773938,32.461109982511,29.399440930781));
#52003=CARTESIAN_POINT('Ctrl Pts',(-12.3796482556495,32.5812164500226,29.3892153702647));
#52004=CARTESIAN_POINT('Ctrl Pts',(-12.4851086121436,32.6897003778855,29.381062463495));
#52005=CARTESIAN_POINT('Ctrl Pts',(-12.7063310003824,32.9500104331378,29.3628440577734));
#52006=CARTESIAN_POINT('Ctrl Pts',(-12.8172205559896,33.1052832861524,29.3528527105587));
#52007=CARTESIAN_POINT('Ctrl Pts',(-12.9511161285198,33.3307290475532,29.3385974614388));
#52008=CARTESIAN_POINT('Ctrl Pts',(-12.9857814087657,33.3935565797701,29.334652146283));
#52009=CARTESIAN_POINT('Ctrl Pts',(-13.0439817218624,33.5074404343609,29.3275075610989));
#52010=CARTESIAN_POINT('Ctrl Pts',(-13.0682896832628,33.5580718805099,29.3243336039601));
#52011=CARTESIAN_POINT('Ctrl Pts',(-13.1039865417543,33.63741987352,29.3193506024849));
#52012=CARTESIAN_POINT('Ctrl Pts',(-13.1162601177284,33.6657287228074,29.3175711608442));
#52013=CARTESIAN_POINT('Ctrl Pts',(-13.1383771508478,33.7187118136351,29.3142357781199));
#52014=CARTESIAN_POINT('Ctrl Pts',(-13.1483203671356,33.7433419859982,29.3126833016252));
#52015=CARTESIAN_POINT('Ctrl Pts',(-13.169917480196,33.7987055062604,29.3091881646942));
#52016=CARTESIAN_POINT('Ctrl Pts',(-13.1814157677096,33.8294963087346,29.3072405698236));
#52017=CARTESIAN_POINT('Ctrl Pts',(-13.214881543688,33.9232510065904,29.3012970394068));
#52018=CARTESIAN_POINT('Ctrl Pts',(-13.2354395434981,33.9866975941466,29.2972565361413));
#52019=CARTESIAN_POINT('Ctrl Pts',(-13.3389887715299,34.3416569667822,29.2745422681367));
#52020=CARTESIAN_POINT('Ctrl Pts',(-13.3844515865375,34.6426550315855,29.2547080383822));
#52021=CARTESIAN_POINT('Ctrl Pts',(-13.3904139810993,35.0141741504821,29.2310163158062));
#52022=CARTESIAN_POINT('Ctrl Pts',(-13.3894334358754,35.0827635834291,29.2266835485809));
#52023=CARTESIAN_POINT('Ctrl Pts',(-13.3843135361265,35.1973720898942,29.2195582491029));
#52024=CARTESIAN_POINT('Ctrl Pts',(-13.3813134624638,35.2434205496467,29.2167264757905));
#52025=CARTESIAN_POINT('Ctrl Pts',(-13.375669953646,35.3092827603988,29.2127339396693));
#52026=CARTESIAN_POINT('Ctrl Pts',(-13.3737902332312,35.3291549280024,29.2115368530168));
#52027=CARTESIAN_POINT('Ctrl Pts',(-13.3701959684134,35.3638786139674,29.2094596887173));
#52028=CARTESIAN_POINT('Ctrl Pts',(-13.3685585447885,35.378737206747,29.2085755810229));
#52029=CARTESIAN_POINT('Ctrl Pts',(-13.364749816301,35.4113179805376,29.2066476681809));
#52030=CARTESIAN_POINT('Ctrl Pts',(-13.3625367351179,35.4290344314555,29.2056061203588));
#52031=CARTESIAN_POINT('Ctrl Pts',(-13.3555738011611,35.4814074092704,29.202545070484));
#52032=CARTESIAN_POINT('Ctrl Pts',(-13.3504272403609,35.5160098224672,29.2005459625742));
#52033=CARTESIAN_POINT('Ctrl Pts',(-13.3143118316057,35.7354299294076,29.1879827814945));
#52034=CARTESIAN_POINT('Ctrl Pts',(-13.2685943706197,35.917510735033,29.178059014632));
#52035=CARTESIAN_POINT('Ctrl Pts',(-13.1986388559469,36.1224812787303,29.1665818236184));
#52036=CARTESIAN_POINT('Ctrl Pts',(-13.1888698716654,36.1499404558964,29.1650380334421));
#52037=CARTESIAN_POINT('Ctrl Pts',(-13.1787500528927,36.1772651204102,29.1634930667589));
#52038=CARTESIAN_POINT('',(-12.5373008502128,37.2477787831567,30.));
#52039=CARTESIAN_POINT('Origin',(-10.,35.,30.));
#52040=CARTESIAN_POINT('Ctrl Pts',(-12.5373008502128,37.2477787831567,30.));
#52041=CARTESIAN_POINT('Ctrl Pts',(-12.5209396269508,37.2662473913687,29.9984867864796));
#52042=CARTESIAN_POINT('Ctrl Pts',(-12.5043772682535,37.2845367879542,29.9969623568916));
#52043=CARTESIAN_POINT('Ctrl Pts',(-12.3453284488148,37.4563621161872,29.9824055457391));
#52044=CARTESIAN_POINT('Ctrl Pts',(-12.1891050598384,37.5965540829986,29.9687575740533));
#52045=CARTESIAN_POINT('Ctrl Pts',(-11.889180987769,37.8192798357995,29.9447572538372));
#52046=CARTESIAN_POINT('Ctrl Pts',(-11.7504662075106,37.9074425883838,29.9343556202805));
#52047=CARTESIAN_POINT('Ctrl Pts',(-11.5488536037137,38.0159000158817,29.9203139605392));
#52048=CARTESIAN_POINT('Ctrl Pts',(-11.490941690947,38.0449456670797,29.9163937485696));
#52049=CARTESIAN_POINT('Ctrl Pts',(-11.4026183240444,38.0861196186118,29.9105799145652));
#52050=CARTESIAN_POINT('Ctrl Pts',(-11.3728079672304,38.0994952587838,29.9086451107208));
#52051=CARTESIAN_POINT('Ctrl Pts',(-11.3206255736704,38.1220084578819,29.905304492922));
#52052=CARTESIAN_POINT('Ctrl Pts',(-11.2983409675913,38.131341484563,29.9038923030429));
#52053=CARTESIAN_POINT('Ctrl Pts',(-11.2476965406407,38.1519182999373,29.9007145484011));
#52054=CARTESIAN_POINT('Ctrl Pts',(-11.2192806844991,38.1630191788191,29.8989537416988));
#52055=CARTESIAN_POINT('Ctrl Pts',(-11.141762425252,38.1921023863124,29.8942074610472));
#52056=CARTESIAN_POINT('Ctrl Pts',(-11.0923866097706,38.2093349739042,29.8912459757493));
#52057=CARTESIAN_POINT('Ctrl Pts',(-10.8409828617183,38.2906022717227,29.8764429922407));
#52058=CARTESIAN_POINT('Ctrl Pts',(-10.633663954766,38.3367342160331,29.8651626739669));
#52059=CARTESIAN_POINT('Ctrl Pts',(-10.2889264735885,38.3801317635053,29.8466594289939));
#52060=CARTESIAN_POINT('Ctrl Pts',(-10.1535860127577,38.3889787179865,29.8394465161247));
#52061=CARTESIAN_POINT('Ctrl Pts',(-9.94672665429997,38.3900825267069,29.8280696073382));
#52062=CARTESIAN_POINT('Ctrl Pts',(-9.87537613772187,38.388209722915,29.8240805287763));
#52063=CARTESIAN_POINT('Ctrl Pts',(-9.78052898184786,38.3827203578675,29.8186306161271));
#52064=CARTESIAN_POINT('Ctrl Pts',(-9.75693070932611,38.381106594221,29.8172624785278));
#52065=CARTESIAN_POINT('Ctrl Pts',(-9.71762699695598,38.3780052344146,29.8149606568456));
#52066=CARTESIAN_POINT('Ctrl Pts',(-9.70191116678088,38.3766546916441,29.814034078292));
#52067=CARTESIAN_POINT('Ctrl Pts',(-9.66965296072587,38.3736556218104,29.8121184567339));
#52068=CARTESIAN_POINT('Ctrl Pts',(-9.65311223514773,38.3719949991171,29.8111287971063));
#52069=CARTESIAN_POINT('Ctrl Pts',(-9.60841641350148,38.3671753800673,29.8084357371168));
#52070=CARTESIAN_POINT('Ctrl Pts',(-9.58028821460886,38.3637850182946,29.8067206857173));
#52071=CARTESIAN_POINT('Ctrl Pts',(-9.41608043113668,38.3419010329106,29.7966025993656));
#52072=CARTESIAN_POINT('Ctrl Pts',(-9.28119394985866,38.3155053374668,29.7878696586115));
#52073=CARTESIAN_POINT('Ctrl Pts',(-8.95383218171039,38.230526484566,29.7661553880092));
#52074=CARTESIAN_POINT('Ctrl Pts',(-8.76422704821641,38.1628539162094,29.7531416767803));
#52075=CARTESIAN_POINT('Ctrl Pts',(-8.5149303884167,38.0480127538378,29.7359279937534));
#52076=CARTESIAN_POINT('Ctrl Pts',(-8.44915074034565,38.0150756544054,29.7313715525671));
#52077=CARTESIAN_POINT('Ctrl Pts',(-8.33420404022636,37.9527615635442,29.7233906840237));
#52078=CARTESIAN_POINT('Ctrl Pts',(-8.28461295995801,37.9242306549314,29.7199408904801));
#52079=CARTESIAN_POINT('Ctrl Pts',(-8.20924299603481,37.8782910190496,29.7146852705358));
#52080=CARTESIAN_POINT('Ctrl Pts',(-8.18294343888853,37.8617608892065,29.7128488972518));
#52081=CARTESIAN_POINT('Ctrl Pts',(-8.13459468532429,37.8304368564147,29.7094672144109));
#52082=CARTESIAN_POINT('Ctrl Pts',(-8.11248512401191,37.8157410104619,29.7079185172302));
#52083=CARTESIAN_POINT('Ctrl Pts',(-8.06361086845244,37.7824207476384,29.7044888010652));
#52084=CARTESIAN_POINT('Ctrl Pts',(-8.03693747063544,37.763666712362,29.7026127608475));
#52085=CARTESIAN_POINT('Ctrl Pts',(-7.96934302950577,37.7146686871443,29.6978444695392));
#52086=CARTESIAN_POINT('Ctrl Pts',(-7.92882413539501,37.6838823968095,29.6949726764167));
#52087=CARTESIAN_POINT('Ctrl Pts',(-7.63999469295613,37.4539914695313,29.6743581788488));
#52088=CARTESIAN_POINT('Ctrl Pts',(-7.42015155987203,37.2217270340292,29.6580610057696));
#52089=CARTESIAN_POINT('Ctrl Pts',(-7.1957217566724,36.9055845152184,29.6371032174982));
#52090=CARTESIAN_POINT('Ctrl Pts',(-7.15726955445118,36.8477314318024,29.6333029118373));
#52091=CARTESIAN_POINT('Ctrl Pts',(-7.09605716183785,36.749196487882,29.6268188413329));
#52092=CARTESIAN_POINT('Ctrl Pts',(-7.07230938446741,36.7091517139359,29.6241806288692));
#52093=CARTESIAN_POINT('Ctrl Pts',(-7.03953556508414,36.6511985196832,29.6203399572476));
#52094=CARTESIAN_POINT('Ctrl Pts',(-7.02983111444626,36.6336777438702,29.6191759241695));
#52095=CARTESIAN_POINT('Ctrl Pts',(-7.01321621451732,36.6030431622358,29.6171338441503));
#52096=CARTESIAN_POINT('Ctrl Pts',(-7.00623558765716,36.5899683635448,29.6162601067456));
#52097=CARTESIAN_POINT('Ctrl Pts',(-6.99108621974016,36.5611399030567,29.6143283056083));
#52098=CARTESIAN_POINT('Ctrl Pts',(-6.98295542671353,36.5453678998681,29.6132681268058));
#52099=CARTESIAN_POINT('Ctrl Pts',(-6.95987361924039,36.4997176028676,29.6101916861547));
#52100=CARTESIAN_POINT('Ctrl Pts',(-6.94524042811648,36.4696819642634,29.6081579069329));
#52101=CARTESIAN_POINT('Ctrl Pts',(-6.84412820607362,36.2541059421147,29.5935180623731));
#52102=CARTESIAN_POINT('Ctrl Pts',(-6.7741746252472,36.0612955692302,29.5802282225884));
#52103=CARTESIAN_POINT('Ctrl Pts',(-6.68450100595008,35.7208313936711,29.5575489221594));
#52104=CARTESIAN_POINT('Ctrl Pts',(-6.65629286295052,35.5759866101405,29.5481261198815));
#52105=CARTESIAN_POINT('Ctrl Pts',(-6.62596082143454,35.3386692698542,29.5332252168921));
#52106=CARTESIAN_POINT('Ctrl Pts',(-6.61802418822,35.2471421473609,29.5276032278844));
#52107=CARTESIAN_POINT('Ctrl Pts',(-6.6121337200653,35.1187870857662,29.5198950418595));
#52108=CARTESIAN_POINT('Ctrl Pts',(-6.61104737133741,35.0821495119626,29.5177145840352));
#52109=CARTESIAN_POINT('Ctrl Pts',(-6.61019615423459,35.0187401145605,29.5139736436072));
#52110=CARTESIAN_POINT('Ctrl Pts',(-6.61015384111658,34.9919759570796,29.5124047494517));
#52111=CARTESIAN_POINT('Ctrl Pts',(-6.61071936862101,34.9368713382597,29.509194389416));
#52112=CARTESIAN_POINT('Ctrl Pts',(-6.6113657110771,34.9085333207337,29.5075542379979));
#52113=CARTESIAN_POINT('Ctrl Pts',(-6.61395421772528,34.8353333556793,29.5033436036199));
#52114=CARTESIAN_POINT('Ctrl Pts',(-6.61643248272675,34.7904951873941,29.5007897592267));
#52115=CARTESIAN_POINT('Ctrl Pts',(-6.63459402809224,34.5490717863472,29.4871554454963));
#52116=CARTESIAN_POINT('Ctrl Pts',(-6.66651870138317,34.3540840183654,29.4765897419547));
#52117=CARTESIAN_POINT('Ctrl Pts',(-6.75666823990741,34.0003116434927,29.4572284040476));
#52118=CARTESIAN_POINT('Ctrl Pts',(-6.81013619776005,33.8409742157929,29.4484213260463));
#52119=CARTESIAN_POINT('Ctrl Pts',(-6.89625318544574,33.636138897112,29.4362920852963));
#52120=CARTESIAN_POINT('Ctrl Pts',(-6.91852774618704,33.5865327733839,29.4332877382476));
#52121=CARTESIAN_POINT('Ctrl Pts',(-6.95880171285986,33.5023226884867,29.4280370032332));
#52122=CARTESIAN_POINT('Ctrl Pts',(-6.97622337510505,33.4674534258208,29.425817175743));
#52123=CARTESIAN_POINT('Ctrl Pts',(-7.00283920762476,33.4164034283052,29.4224881002581));
#52124=CARTESIAN_POINT('Ctrl Pts',(-7.01157216102883,33.3999843957678,29.4214050693375));
#52125=CARTESIAN_POINT('Ctrl Pts',(-7.02752378732178,33.370579566588,29.4194417385407));
#52126=CARTESIAN_POINT('Ctrl Pts',(-7.03469337341124,33.3575681535262,29.4185644181907));
#52127=CARTESIAN_POINT('Ctrl Pts',(-7.05120597351274,33.3280615392013,29.4165553827969));
#52128=CARTESIAN_POINT('Ctrl Pts',(-7.06060202136618,33.3115972300352,29.415420498807));
#52129=CARTESIAN_POINT('Ctrl Pts',(-7.09050791962363,33.2602006431111,29.4118361111738));
#52130=CARTESIAN_POINT('Ctrl Pts',(-7.11150544701686,33.2255578690523,29.4093592635796));
#52131=CARTESIAN_POINT('Ctrl Pts',(-7.24819545161236,33.0088970326594,29.3935193328223));
#52132=CARTESIAN_POINT('Ctrl Pts',(-7.38041216586462,32.8379013365208,29.3794691012816));
#52133=CARTESIAN_POINT('Ctrl Pts',(-7.56237680253748,32.6439594356501,29.3623812090118));
#52134=CARTESIAN_POINT('Ctrl Pts',(-7.5975981204726,32.6080553118372,29.3591605227291));
#52135=CARTESIAN_POINT('Ctrl Pts',(-7.7437955640887,32.4655117260328,29.3461577608832));
#52136=CARTESIAN_POINT('Ctrl Pts',(-7.86118405595141,32.3656944248076,29.3365537202643));
#52137=CARTESIAN_POINT('Ctrl Pts',(-8.01952131852312,32.2486446882893,29.3246683838735));
#52138=CARTESIAN_POINT('Ctrl Pts',(-8.05456221067293,32.2237572294516,29.3220989480786));
#52139=CARTESIAN_POINT('Ctrl Pts',(-8.1132847542766,32.1837080464183,29.3178905598686));
#52140=CARTESIAN_POINT('Ctrl Pts',(-8.13669787798292,32.1681631298337,29.3162375118986));
#52141=CARTESIAN_POINT('Ctrl Pts',(-8.18292643767467,32.1382917150435,29.3130209227098));
#52142=CARTESIAN_POINT('Ctrl Pts',(-8.20572464058836,32.1239425188523,29.3114566312738));
#52143=CARTESIAN_POINT('Ctrl Pts',(-8.25623278564863,32.0929870362857,29.3080377681723));
#52144=CARTESIAN_POINT('Ctrl Pts',(-8.28401411557813,32.0765019215338,29.3061876098534));
#52145=CARTESIAN_POINT('Ctrl Pts',(-8.38119318868305,32.0206996036542,29.2998156412589));
#52146=CARTESIAN_POINT('Ctrl Pts',(-8.45174213620083,31.9834348595183,29.2953645908614));
#52147=CARTESIAN_POINT('Ctrl Pts',(-8.77624245161622,31.8264168248332,29.2755445854091));
#52148=CARTESIAN_POINT('Ctrl Pts',(-9.04313207141249,31.7360136239522,29.2611013552682));
#52149=CARTESIAN_POINT('Ctrl Pts',(-9.38365250996888,31.6660835854944,29.2422781176924));
#52150=CARTESIAN_POINT('Ctrl Pts',(-9.44958218530448,31.6545669602589,29.2386105305425));
#52151=CARTESIAN_POINT('Ctrl Pts',(-9.56066917573313,31.638534825396,29.2323304537426));
#52152=CARTESIAN_POINT('Ctrl Pts',(-9.60565556225182,31.6329609817424,29.2297598276176));
#52153=CARTESIAN_POINT('Ctrl Pts',(-9.6704657282075,31.6262475505551,29.2260000929369));
#52154=CARTESIAN_POINT('Ctrl Pts',(-9.69021061456033,31.6243772541966,29.224847172381));
#52155=CARTESIAN_POINT('Ctrl Pts',(-9.72489391099103,31.6213988012479,29.2228070939141));
#52156=CARTESIAN_POINT('Ctrl Pts',(-9.73982503168357,31.6202162206567,29.2219239385905));
#52157=CARTESIAN_POINT('Ctrl Pts',(-9.7728035987184,31.6178240735557,29.2199620737127));
#52158=CARTESIAN_POINT('Ctrl Pts',(-9.79085294767274,31.6166599815685,29.2188810845482));
#52159=CARTESIAN_POINT('Ctrl Pts',(-9.84360728723493,31.6136813349682,29.2157021068948));
#52160=CARTESIAN_POINT('Ctrl Pts',(-9.8783309369857,31.6122560280276,29.2135850617306));
#52161=CARTESIAN_POINT('Ctrl Pts',(-10.0981263677544,31.6066174553222,29.2000541810209));
#52162=CARTESIAN_POINT('Ctrl Pts',(-10.2832483732874,31.6170376190416,29.1880914295951));
#52163=CARTESIAN_POINT('Ctrl Pts',(-10.6239784709893,31.6643877498171,29.1659230141077));
#52164=CARTESIAN_POINT('Ctrl Pts',(-10.7796569781257,31.6973040163098,29.1557331274996));
#52165=CARTESIAN_POINT('Ctrl Pts',(-11.0248254515854,31.7674518777504,29.1398229311888));
#52166=CARTESIAN_POINT('Ctrl Pts',(-11.1160301687483,31.7977954588283,29.1339328961468));
#52167=CARTESIAN_POINT('Ctrl Pts',(-11.2407477939109,31.8452661125389,29.1259222172468));
#52168=CARTESIAN_POINT('Ctrl Pts',(-11.2754448838168,31.8591336378877,29.1236981799086));
#52169=CARTESIAN_POINT('Ctrl Pts',(-11.3348213199839,31.8840111021375,29.1198987602241));
#52170=CARTESIAN_POINT('Ctrl Pts',(-11.3596107978847,31.894747464534,29.1183144979025));
#52171=CARTESIAN_POINT('Ctrl Pts',(-11.4070719875209,31.9159803041733,29.1152842291648));
#52172=CARTESIAN_POINT('Ctrl Pts',(-11.4297611101642,31.926433296835,29.113836889095));
#52173=CARTESIAN_POINT('Ctrl Pts',(-11.489709738225,31.9548594315303,29.1100149306547));
#52174=CARTESIAN_POINT('Ctrl Pts',(-11.5267599390454,31.9732657063701,29.1076551260102));
#52175=CARTESIAN_POINT('Ctrl Pts',(-11.6730874650145,32.0493309696961,29.0983330598165));
#52176=CARTESIAN_POINT('Ctrl Pts',(-11.7795182426047,32.112269338126,29.0915521627291));
#52177=CARTESIAN_POINT('Ctrl Pts',(-12.0757893280323,32.3100852188785,29.0723399803462));
#52178=CARTESIAN_POINT('Ctrl Pts',(-12.2554677453518,32.4588585975599,29.0602912873199));
#52179=CARTESIAN_POINT('Ctrl Pts',(-12.4834735946583,32.6910249054707,29.0426296952372));
#52180=CARTESIAN_POINT('Ctrl Pts',(-12.5457117965855,32.7598313137064,29.0375050969097));
#52181=CARTESIAN_POINT('Ctrl Pts',(-12.6212677042778,32.8505806660665,29.030753781437));
#52182=CARTESIAN_POINT('Ctrl Pts',(-12.6372701627646,32.8702455875169,29.0292912021241));
#52183=CARTESIAN_POINT('Ctrl Pts',(-12.6629383551474,32.9025213331412,29.026887933541));
#52184=CARTESIAN_POINT('Ctrl Pts',(-12.6727389390418,32.9150242249577,29.0259563015219));
#52185=CARTESIAN_POINT('Ctrl Pts',(-12.6909629300947,32.9386127466578,29.0241964444135));
#52186=CARTESIAN_POINT('Ctrl Pts',(-12.6994066599705,32.9496823254402,29.0233696789054));
#52187=CARTESIAN_POINT('Ctrl Pts',(-12.7217820403145,32.9793938529969,29.0211488899844));
#52188=CARTESIAN_POINT('Ctrl Pts',(-12.7355900635766,32.9981274729344,29.0197468853315));
#52189=CARTESIAN_POINT('Ctrl Pts',(-12.7872450041257,33.0697412089155,29.0143853882205));
#52190=CARTESIAN_POINT('Ctrl Pts',(-12.8237584255344,33.1235616294103,29.010352120052));
#52191=CARTESIAN_POINT('Ctrl Pts',(-12.9626053366071,33.3414582233969,28.9941076228168));
#52192=CARTESIAN_POINT('Ctrl Pts',(-13.0523665036986,33.5131081470561,28.9815183798047));
#52193=CARTESIAN_POINT('Ctrl Pts',(-13.1994628265299,33.8646252523959,28.9570765815282));
#52194=CARTESIAN_POINT('Ctrl Pts',(-13.2574225244727,34.0435197481613,28.9452567810019));
#52195=CARTESIAN_POINT('Ctrl Pts',(-13.31045493455,34.2697382096425,28.9312105266925));
#52196=CARTESIAN_POINT('Ctrl Pts',(-13.3197767551102,34.313358363635,28.9285407689065));
#52197=CARTESIAN_POINT('Ctrl Pts',(-13.3336175666805,34.3850167268999,28.92421618508));
#52198=CARTESIAN_POINT('Ctrl Pts',(-13.3386497105125,34.4129491582204,28.9225455342672));
#52199=CARTESIAN_POINT('Ctrl Pts',(-13.3477773477245,34.4675351162431,28.9193090562825));
#52200=CARTESIAN_POINT('Ctrl Pts',(-13.3519067643714,34.4941807368721,28.9177422826077));
#52201=CARTESIAN_POINT('Ctrl Pts',(-13.3609760471372,34.557700384283,28.9140369870926));
#52202=CARTESIAN_POINT('Ctrl Pts',(-13.3656277297902,34.5946124337918,28.9119075184641));
#52203=CARTESIAN_POINT('Ctrl Pts',(-13.3793601028952,34.7202175005973,28.9047350133045));
#52204=CARTESIAN_POINT('Ctrl Pts',(-13.3855497600678,34.809192343585,28.8997797086442));
#52205=CARTESIAN_POINT('Ctrl Pts',(-13.3963455872416,35.1689113805965,28.8800933739847));
#52206=CARTESIAN_POINT('Ctrl Pts',(-13.3720223036886,35.4394889413582,28.866159333191));
#52207=CARTESIAN_POINT('Ctrl Pts',(-13.302020701116,35.7690573393126,28.8479157063941));
#52208=CARTESIAN_POINT('Ctrl Pts',(-13.2863682651649,35.833410253715,28.8442859466476));
#52209=CARTESIAN_POINT('Ctrl Pts',(-13.2569379098682,35.9406290968532,28.8380642975009));
#52210=CARTESIAN_POINT('Ctrl Pts',(-13.244172277261,35.9837547873549,28.8355135626861));
#52211=CARTESIAN_POINT('Ctrl Pts',(-13.2245784949098,36.0454127285732,28.8317802351001));
#52212=CARTESIAN_POINT('Ctrl Pts',(-13.2184399656098,36.0641608853992,28.8306334098665));
#52213=CARTESIAN_POINT('Ctrl Pts',(-13.207368136938,36.0970039540344,28.8286021549514));
#52214=CARTESIAN_POINT('Ctrl Pts',(-13.2025048060993,36.1111215033851,28.8277216735734));
#52215=CARTESIAN_POINT('Ctrl Pts',(-13.1915487528986,36.1422557851853,28.8257632687472));
#52216=CARTESIAN_POINT('Ctrl Pts',(-13.1854131894937,36.15925601176,28.8246830364101));
#52217=CARTESIAN_POINT('Ctrl Pts',(-13.1790114989384,36.1765590056772,28.8235730107745));
#52218=CARTESIAN_POINT('Ctrl Pts',(-13.1788808123799,36.176912054873,28.8235503573816));
#52219=CARTESIAN_POINT('Ctrl Pts',(-13.1787500671537,36.177265081904,28.8235277009158));
#52220=CARTESIAN_POINT('Origin',(-10.,35.,23.));
#52221=CARTESIAN_POINT('',(-13.3897499995487,35.0000553150526,27.6441403738275));
#52222=CARTESIAN_POINT('Ctrl Pts',(-13.1787500671537,36.177265081904,28.8235277009158));
#52223=CARTESIAN_POINT('Ctrl Pts',(-13.166434766078,36.210517800194,28.8213936176659));
#52224=CARTESIAN_POINT('Ctrl Pts',(-13.1535989446877,36.2435738652805,28.8192322861915));
#52225=CARTESIAN_POINT('Ctrl Pts',(-13.0858169506057,36.4103309352554,28.8081469722261));
#52226=CARTESIAN_POINT('Ctrl Pts',(-13.022880744743,36.5406118917708,28.7988926786411));
#52227=CARTESIAN_POINT('Ctrl Pts',(-12.8184861727369,36.9026578936524,28.7721200136203));
#52228=CARTESIAN_POINT('Ctrl Pts',(-12.6572519859891,37.1220346140764,28.7546511910919));
#52229=CARTESIAN_POINT('Ctrl Pts',(-12.4383388202369,37.3552635424168,28.7352501428755));
#52230=CARTESIAN_POINT('Ctrl Pts',(-12.4043516353376,37.389948981851,28.7323361799766));
#52231=CARTESIAN_POINT('Ctrl Pts',(-12.3487390154015,37.4443165943742,28.7277198463628));
#52232=CARTESIAN_POINT('Ctrl Pts',(-12.3275847858441,37.4644690545115,28.7259973978757));
#52233=CARTESIAN_POINT('Ctrl Pts',(-12.2866205591494,37.5024953838658,28.7227243024674));
#52234=CARTESIAN_POINT('Ctrl Pts',(-12.2668549948662,37.5204137001373,28.7211718498571));
#52235=CARTESIAN_POINT('Ctrl Pts',(-12.2205451806129,37.5614099921634,28.717594812036));
#52236=CARTESIAN_POINT('Ctrl Pts',(-12.1938489277326,37.5843121059695,28.7155774902595));
#52237=CARTESIAN_POINT('Ctrl Pts',(-12.1045808818177,37.6585128069503,28.708972195594));
#52238=CARTESIAN_POINT('Ctrl Pts',(-12.0405269200284,37.7079886084641,28.7044553655199));
#52239=CARTESIAN_POINT('Ctrl Pts',(-11.8769317184796,37.8252468018461,28.6933885358282));
#52240=CARTESIAN_POINT('Ctrl Pts',(-11.7754341422537,37.8901087047309,28.6869311280284));
#52241=CARTESIAN_POINT('Ctrl Pts',(-11.4581549298229,38.0698302985159,28.667530135191));
#52242=CARTESIAN_POINT('Ctrl Pts',(-11.2332480888688,38.1668825137047,28.6548423315028));
#52243=CARTESIAN_POINT('Ctrl Pts',(-10.9661459976826,38.2493406884846,28.6390527818522));
#52244=CARTESIAN_POINT('Ctrl Pts',(-10.9322322711635,38.2592323921266,28.6370344486184));
#52245=CARTESIAN_POINT('Ctrl Pts',(-10.8808368575517,38.2733552626088,28.6339468710406));
#52246=CARTESIAN_POINT('Ctrl Pts',(-10.8634649382657,38.2779805542203,28.6328983228947));
#52247=CARTESIAN_POINT('Ctrl Pts',(-10.8315762262773,38.2861998845013,28.6309631796081));
#52248=CARTESIAN_POINT('Ctrl Pts',(-10.817071278103,38.2898363485813,28.6300789340397));
#52249=CARTESIAN_POINT('Ctrl Pts',(-10.7832176212011,38.2980859386765,28.6280059826253));
#52250=CARTESIAN_POINT('Ctrl Pts',(-10.7638518991496,38.3026248553185,28.6268133336086));
#52251=CARTESIAN_POINT('Ctrl Pts',(-10.699685028846,38.3170696670052,28.6228415648047));
#52252=CARTESIAN_POINT('Ctrl Pts',(-10.6547244550655,38.3262359758911,28.6200265089239));
#52253=CARTESIAN_POINT('Ctrl Pts',(-10.5425962849199,38.3467346868527,28.612949033971));
#52254=CARTESIAN_POINT('Ctrl Pts',(-10.4752477666643,38.3569602935189,28.6086479006761));
#52255=CARTESIAN_POINT('Ctrl Pts',(-10.1121661262008,38.4009425370305,28.5853366893942));
#52256=CARTESIAN_POINT('Ctrl Pts',(-9.81320160132118,38.3976679133283,28.5658578659115));
#52257=CARTESIAN_POINT('Ctrl Pts',(-9.4497784236149,38.3455166363152,28.5432673969683));
#52258=CARTESIAN_POINT('Ctrl Pts',(-9.38136995557253,38.3335451495908,28.5390552259866));
#52259=CARTESIAN_POINT('Ctrl Pts',(-9.28080837533687,38.3127442300193,28.5329208956245));
#52260=CARTESIAN_POINT('Ctrl Pts',(-9.24834326895999,38.30552918659,28.5309493985302));
#52261=CARTESIAN_POINT('Ctrl Pts',(-9.19024481020219,38.2917171506692,28.5274361100453));
#52262=CARTESIAN_POINT('Ctrl Pts',(-9.16457294883622,38.2852955678993,28.525888941759));
#52263=CARTESIAN_POINT('Ctrl Pts',(-9.10968953863327,38.2708820438247,28.522591511108));
#52264=CARTESIAN_POINT('Ctrl Pts',(-9.08050444941199,38.2627978914372,28.5208443241915));
#52265=CARTESIAN_POINT('Ctrl Pts',(-8.99979037213182,38.2392713803137,28.5160271820677));
#52266=CARTESIAN_POINT('Ctrl Pts',(-8.9485136156673,38.2229916540452,28.5129839885266));
#52267=CARTESIAN_POINT('Ctrl Pts',(-8.72554797795612,38.1463147910459,28.4997960289365));
#52268=CARTESIAN_POINT('Ctrl Pts',(-8.55849118790347,38.0733671443277,28.4900526261314));
#52269=CARTESIAN_POINT('Ctrl Pts',(-8.21039392337908,37.8867063059201,28.4690851937724));
#52270=CARTESIAN_POINT('Ctrl Pts',(-8.03262348458114,37.7686052114341,28.457938027921));
#52271=CARTESIAN_POINT('Ctrl Pts',(-7.83354885916886,37.6074433426528,28.4435819969441));
#52272=CARTESIAN_POINT('Ctrl Pts',(-7.80049643429137,37.579623041644,28.441128671115));
#52273=CARTESIAN_POINT('Ctrl Pts',(-7.75351541099053,37.5385195978483,28.4375242156927));
#52274=CARTESIAN_POINT('Ctrl Pts',(-7.73915287529624,37.5257365259102,28.4364059509919));
#52275=CARTESIAN_POINT('Ctrl Pts',(-7.71383564177686,37.5028144899695,28.4344038779858));
#52276=CARTESIAN_POINT('Ctrl Pts',(-7.70283798582009,37.4927243151097,28.4335235562481));
#52277=CARTESIAN_POINT('Ctrl Pts',(-7.67856540180816,37.4701575509501,28.4315565585262));
#52278=CARTESIAN_POINT('Ctrl Pts',(-7.66532432703466,37.457646514294,28.4304674450363));
#52279=CARTESIAN_POINT('Ctrl Pts',(-7.62579816065501,37.4196919142239,28.4271693389946));
#52280=CARTESIAN_POINT('Ctrl Pts',(-7.59982427665488,37.3939297394818,28.4249385988885));
#52281=CARTESIAN_POINT('Ctrl Pts',(-7.53947191510846,37.3320996870264,28.4196140352381));
#52282=CARTESIAN_POINT('Ctrl Pts',(-7.50546208284561,37.2956845470343,28.4165007860368));
#52283=CARTESIAN_POINT('Ctrl Pts',(-7.37794915451968,37.1529732608738,28.404427436929));
#52284=CARTESIAN_POINT('Ctrl Pts',(-7.29033809915329,37.0416106891168,28.3952751547634));
#52285=CARTESIAN_POINT('Ctrl Pts',(-7.08835706118761,36.7488794491795,28.3723617308675));
#52286=CARTESIAN_POINT('Ctrl Pts',(-6.98371889729,36.5615108978639,28.3587208858197));
#52287=CARTESIAN_POINT('Ctrl Pts',(-6.87617075894826,36.3171508286412,28.3424664533197));
#52288=CARTESIAN_POINT('Ctrl Pts',(-6.85602381318998,36.2683097565836,28.3392865892569));
#52289=CARTESIAN_POINT('Ctrl Pts',(-6.82610028714547,36.190667319821,28.3343370700035));
#52290=CARTESIAN_POINT('Ctrl Pts',(-6.81555615816321,36.1621727762971,28.3325425193558));
#52291=CARTESIAN_POINT('Ctrl Pts',(-6.79655229936173,36.1086150554803,28.3292092334463));
#52292=CARTESIAN_POINT('Ctrl Pts',(-6.78800015065401,36.0835873468427,28.3276675833656));
#52293=CARTESIAN_POINT('Ctrl Pts',(-6.76940491919353,36.0270133043127,28.3242174810881));
#52294=CARTESIAN_POINT('Ctrl Pts',(-6.75952921702349,35.9954145461676,28.3223145466611));
#52295=CARTESIAN_POINT('Ctrl Pts',(-6.7306186575016,35.8979170714287,28.3165126872897));
#52296=CARTESIAN_POINT('Ctrl Pts',(-6.71311909975902,35.8315793737517,28.3126622931271));
#52297=CARTESIAN_POINT('Ctrl Pts',(-6.67632132206091,35.6726792268013,28.3036306435247));
#52298=CARTESIAN_POINT('Ctrl Pts',(-6.65885818356737,35.5797501734478,28.2985010166764));
#52299=CARTESIAN_POINT('Ctrl Pts',(-6.61365159120521,35.2678376817111,28.2815899001262));
#52300=CARTESIAN_POINT('Ctrl Pts',(-6.60340128422791,35.0469117972492,28.2701381474515));
#52301=CARTESIAN_POINT('Ctrl Pts',(-6.61905258039951,34.7414046191699,28.2534839635711));
#52302=CARTESIAN_POINT('Ctrl Pts',(-6.62662742200177,34.6564417704503,28.2487592141704));
#52303=CARTESIAN_POINT('Ctrl Pts',(-6.64060342594177,34.5466740373212,28.2424332344298));
#52304=CARTESIAN_POINT('Ctrl Pts',(-6.64409321938054,34.5215239107456,28.2409685636642));
#52305=CARTESIAN_POINT('Ctrl Pts',(-6.65022631922119,34.4806985767634,28.2385627653547));
#52306=CARTESIAN_POINT('Ctrl Pts',(-6.65269800261716,34.4649981341706,28.2376307331641));
#52307=CARTESIAN_POINT('Ctrl Pts',(-6.65784846929929,34.433715457829,28.2357590394871));
#52308=CARTESIAN_POINT('Ctrl Pts',(-6.66052604122618,34.4181334416889,28.2348194596194));
#52309=CARTESIAN_POINT('Ctrl Pts',(-6.6677180458531,34.377965528228,28.2323795603338));
#52310=CARTESIAN_POINT('Ctrl Pts',(-6.67239553410521,34.3534102195046,28.2308707362243));
#52311=CARTESIAN_POINT('Ctrl Pts',(-6.69483918722206,34.2422887538044,28.2239711100712));
#52312=CARTESIAN_POINT('Ctrl Pts',(-6.71571365780099,34.1563916326028,28.2184404451808));
#52313=CARTESIAN_POINT('Ctrl Pts',(-6.79657066806341,33.8725181833984,28.1997033414331));
#52314=CARTESIAN_POINT('Ctrl Pts',(-6.87130623137782,33.6792222410189,28.1862135929335));
#52315=CARTESIAN_POINT('Ctrl Pts',(-7.02953877504176,33.3601639195086,28.1635501502474));
#52316=CARTESIAN_POINT('Ctrl Pts',(-7.10465536211101,33.2309067137465,28.1542355015247));
#52317=CARTESIAN_POINT('Ctrl Pts',(-7.21242016325755,33.0708275474554,28.1425801046868));
#52318=CARTESIAN_POINT('Ctrl Pts',(-7.23747603525473,33.035115955559,28.1399708178252));
#52319=CARTESIAN_POINT('Ctrl Pts',(-7.27985152129769,32.9771326576891,28.1357172856535));
#52320=CARTESIAN_POINT('Ctrl Pts',(-7.29677166386621,32.9545766537819,28.134058243212));
#52321=CARTESIAN_POINT('Ctrl Pts',(-7.33050206972609,32.9107608544167,28.1308258341812));
#52322=CARTESIAN_POINT('Ctrl Pts',(-7.34728971977179,32.8894864040244,28.1292517651311));
#52323=CARTESIAN_POINT('Ctrl Pts',(-7.38817006293192,32.8389385460768,28.1254992324593));
#52324=CARTESIAN_POINT('Ctrl Pts',(-7.41250252468886,32.8098631991498,28.123330435319));
#52325=CARTESIAN_POINT('Ctrl Pts',(-7.50301080324101,32.7053273949843,28.115486990426));
#52326=CARTESIAN_POINT('Ctrl Pts',(-7.57204378715094,32.6324044885922,28.1099279342807));
#52327=CARTESIAN_POINT('Ctrl Pts',(-7.88452936670291,32.3303765138965,28.0862607191016));
#52328=CARTESIAN_POINT('Ctrl Pts',(-8.15782883654959,32.1349604411043,28.0693995454902));
#52329=CARTESIAN_POINT('Ctrl Pts',(-8.48927744379643,31.9652703185237,28.0484302233606));
#52330=CARTESIAN_POINT('Ctrl Pts',(-8.52360118212731,31.9484244796703,28.0462509021404));
#52331=CARTESIAN_POINT('Ctrl Pts',(-8.57497476987081,31.9242803017925,28.0429669458511));
#52332=CARTESIAN_POINT('Ctrl Pts',(-8.59181253280937,31.9165349699536,28.0418871551777));
#52333=CARTESIAN_POINT('Ctrl Pts',(-8.62230909918148,31.9028085040565,28.039923725885));
#52334=CARTESIAN_POINT('Ctrl Pts',(-8.63594507271467,31.8967788486542,28.0390429581787));
#52335=CARTESIAN_POINT('Ctrl Pts',(-8.66721666144278,31.8831968837593,28.0370165559367));
#52336=CARTESIAN_POINT('Ctrl Pts',(-8.68487690848522,31.8757041899131,28.0358676033863));
#52337=CARTESIAN_POINT('Ctrl Pts',(-8.74120272284559,31.852369069814,28.0321908458046));
#52338=CARTESIAN_POINT('Ctrl Pts',(-8.78009670456377,31.8370920547107,28.0296337451941));
#52339=CARTESIAN_POINT('Ctrl Pts',(-8.87526239433176,31.8017286587729,28.023349752761));
#52340=CARTESIAN_POINT('Ctrl Pts',(-8.93180135754353,31.7824038135626,28.0195936690612));
#52341=CARTESIAN_POINT('Ctrl Pts',(-9.1851135692938,31.7032348191335,28.0027476023511));
#52342=CARTESIAN_POINT('Ctrl Pts',(-9.38658461972464,31.6598763903841,27.9893341662665));
#52343=CARTESIAN_POINT('Ctrl Pts',(-9.7402021627914,31.6168687271918,27.966658038071));
#52344=CARTESIAN_POINT('Ctrl Pts',(-9.89071545135332,31.6086671354038,27.9572633126712));
#52345=CARTESIAN_POINT('Ctrl Pts',(-10.0849832157498,31.6110337674961,27.9455280399593));
#52346=CARTESIAN_POINT('Ctrl Pts',(-10.1286615352161,31.612410776265,27.9429141082112));
#52347=CARTESIAN_POINT('Ctrl Pts',(-10.200475782283,31.6160658536245,27.9386551017424));
#52348=CARTESIAN_POINT('Ctrl Pts',(-10.2286305681341,31.6178514252808,27.9369951523507));
#52349=CARTESIAN_POINT('Ctrl Pts',(-10.2837708184416,31.6220401192642,27.9337624192067));
#52350=CARTESIAN_POINT('Ctrl Pts',(-10.3107561868358,31.6244156819909,27.93218891404));
#52351=CARTESIAN_POINT('Ctrl Pts',(-10.3753764693928,31.6308857994462,27.9284400918272));
#52352=CARTESIAN_POINT('Ctrl Pts',(-10.4129773641417,31.6352878504166,27.9262743922546));
#52353=CARTESIAN_POINT('Ctrl Pts',(-10.5495374420043,31.6535991142344,27.918458344247));
#52354=CARTESIAN_POINT('Ctrl Pts',(-10.647946512712,31.6712527819722,27.9129224842524));
#52355=CARTESIAN_POINT('Ctrl Pts',(-10.9116584652689,31.7307008266765,27.8981978993259));
#52356=CARTESIAN_POINT('Ctrl Pts',(-11.0748219585882,31.7806524029079,27.8892165004611));
#52357=CARTESIAN_POINT('Ctrl Pts',(-11.3902058864393,31.903869561698,27.8712460553602));
#52358=CARTESIAN_POINT('Ctrl Pts',(-11.5420849235255,31.9766477486335,27.8622788915445));
#52359=CARTESIAN_POINT('Ctrl Pts',(-11.7187326588042,32.0780784385183,27.8507760115731));
#52360=CARTESIAN_POINT('Ctrl Pts',(-11.7492646305123,32.0962540387456,27.8487463104989));
#52361=CARTESIAN_POINT('Ctrl Pts',(-11.7948351459586,32.1243615796153,27.8456450888389));
#52362=CARTESIAN_POINT('Ctrl Pts',(-11.810090325006,32.1339395488428,27.8445945598758));
#52363=CARTESIAN_POINT('Ctrl Pts',(-11.8378618705159,32.1516860818681,27.8426579999226));
#52364=CARTESIAN_POINT('Ctrl Pts',(-11.8504015771968,32.1598164834571,27.8417743567319));
#52365=CARTESIAN_POINT('Ctrl Pts',(-11.8794502638822,32.1789248830082,27.8397059805173));
#52366=CARTESIAN_POINT('Ctrl Pts',(-11.8959171003914,32.1899650506282,27.8385173577485));
#52367=CARTESIAN_POINT('Ctrl Pts',(-11.9498548729703,32.226817466587,27.8345730473586));
#52368=CARTESIAN_POINT('Ctrl Pts',(-11.9869015202532,32.2532387595667,27.8317820638421));
#52369=CARTESIAN_POINT('Ctrl Pts',(-12.0774044158213,32.3205735126223,27.8247799211133));
#52370=CARTESIAN_POINT('Ctrl Pts',(-12.1301943867381,32.3623483234418,27.82053100087));
#52371=CARTESIAN_POINT('Ctrl Pts',(-12.4002276476061,32.5894324375087,27.7980505522779));
#52372=CARTESIAN_POINT('Ctrl Pts',(-12.5946974596593,32.8001105182745,27.7793635235968));
#52373=CARTESIAN_POINT('Ctrl Pts',(-12.8060343545539,33.0966487722939,27.7568413044733));
#52374=CARTESIAN_POINT('Ctrl Pts',(-12.8493863001078,33.16218229632,27.752057380962));
#52375=CARTESIAN_POINT('Ctrl Pts',(-12.9084048960482,33.2585148320735,27.7452955753604));
#52376=CARTESIAN_POINT('Ctrl Pts',(-12.9259373587927,33.2881354221329,27.7432516162175));
#52377=CARTESIAN_POINT('Ctrl Pts',(-12.9562394189953,33.3411559015445,27.7396535727117));
#52378=CARTESIAN_POINT('Ctrl Pts',(-12.9691896438078,33.3644486664253,27.7380931861911));
#52379=CARTESIAN_POINT('Ctrl Pts',(-12.9957871453947,33.4136452135046,27.7348387981648));
#52380=CARTESIAN_POINT('Ctrl Pts',(-13.0093762668814,33.4395780406389,27.733146920061));
#52381=CARTESIAN_POINT('Ctrl Pts',(-13.0447510724429,33.5092670080002,27.7286607142981));
#52382=CARTESIAN_POINT('Ctrl Pts',(-13.0659296237242,33.5533245606395,27.7258872006604));
#52383=CARTESIAN_POINT('Ctrl Pts',(-13.1108486158215,33.6521901262051,27.7197899350797));
#52384=CARTESIAN_POINT('Ctrl Pts',(-13.1341085391091,33.7071988716986,27.7164816470441));
#52385=CARTESIAN_POINT('Ctrl Pts',(-13.2051817426865,33.8884948592549,27.7058098885118));
#52386=CARTESIAN_POINT('Ctrl Pts',(-13.2469075289949,34.0170309436269,27.69860806261));
#52387=CARTESIAN_POINT('Ctrl Pts',(-13.337171070746,34.3645000702773,27.679556706201));
#52388=CARTESIAN_POINT('Ctrl Pts',(-13.3718546197707,34.5863045927268,27.6678347172914));
#52389=CARTESIAN_POINT('Ctrl Pts',(-13.3862616624626,34.8427671081477,27.6532987185319));
#52390=CARTESIAN_POINT('Ctrl Pts',(-13.3876296810394,34.8756810358968,27.6514142305087));
#52391=CARTESIAN_POINT('Ctrl Pts',(-13.3889697175852,34.9253654300795,27.6485340617883));
#52392=CARTESIAN_POINT('Ctrl Pts',(-13.3892973536265,34.942125230214,27.6475564189619));
#52393=CARTESIAN_POINT('Ctrl Pts',(-13.3896044073129,34.967439442401,27.6460696673787));
#52394=CARTESIAN_POINT('Ctrl Pts',(-13.3896757778973,34.9759927583652,27.6455655660513));
#52395=CARTESIAN_POINT('Ctrl Pts',(-13.3897383420373,34.989715973186,27.6447538687426));
#52396=CARTESIAN_POINT('Ctrl Pts',(-13.3897500839088,34.9948856619753,27.6444474400273));
#52397=CARTESIAN_POINT('Ctrl Pts',(-13.3897499995487,35.0000553150526,27.6441403738275));
#52398=CARTESIAN_POINT('Ctrl Pts',(-13.3897499995573,35.0000547843624,27.6441404053493));
#52399=CARTESIAN_POINT('Ctrl Pts',(-13.3897499123479,35.0054508158919,27.6438198928052));
#52400=CARTESIAN_POINT('Ctrl Pts',(-13.3897369404911,35.0108468044594,27.6434986859644));
#52401=CARTESIAN_POINT('Ctrl Pts',(-13.3896570780152,35.0275134090258,27.6425044687922));
#52402=CARTESIAN_POINT('Ctrl Pts',(-13.3895468603506,35.0387836045129,27.6418291920736));
#52403=CARTESIAN_POINT('Ctrl Pts',(-13.3888732877613,35.0843952519037,27.6390848093052));
#52404=CARTESIAN_POINT('Ctrl Pts',(-13.3878442304446,35.1187265535147,27.6369928438969));
#52405=CARTESIAN_POINT('Ctrl Pts',(-13.3760311601969,35.3801214671601,27.620893719586));
#52406=CARTESIAN_POINT('Ctrl Pts',(-13.3429528571328,35.6055865388991,27.6060657679701));
#52407=CARTESIAN_POINT('Ctrl Pts',(-13.2576688564896,35.9450126906287,27.5835867882404));
#52408=CARTESIAN_POINT('Ctrl Pts',(-13.2213420677615,36.0622618086893,27.5757825549973));
#52409=CARTESIAN_POINT('Ctrl Pts',(-13.1787501041618,36.1772649819778,27.5681446579994));
#52410=CARTESIAN_POINT('',(-13.3897486873307,34.9970168406318,27.9839821967053));
#52411=CARTESIAN_POINT('Ctrl Pts',(-13.1787500671536,36.1772650819042,27.9134187897562));
#52412=CARTESIAN_POINT('Ctrl Pts',(-13.2144035502327,36.0809966089206,27.9194227790256));
#52413=CARTESIAN_POINT('Ctrl Pts',(-13.2456875617548,35.9830857988981,27.925426768295));
#52414=CARTESIAN_POINT('Ctrl Pts',(-13.2724606689644,35.8839718505592,27.9314307575644));
#52415=CARTESIAN_POINT('Ctrl Pts',(-13.2992339653125,35.7848572020301,27.937434789249));
#52416=CARTESIAN_POINT('Ctrl Pts',(-13.321496186599,35.6845398253861,27.9434388209335));
#52417=CARTESIAN_POINT('Ctrl Pts',(-13.3391564363488,35.5834718125927,27.9494428526181));
#52418=CARTESIAN_POINT('Ctrl Pts',(-13.3568325931257,35.4823127653216,27.9554522922836));
#52419=CARTESIAN_POINT('Ctrl Pts',(-13.3698984291381,35.3804021667328,27.9614617319492));
#52420=CARTESIAN_POINT('Ctrl Pts',(-13.3783146635796,35.2781997418099,27.9674711716147));
#52421=CARTESIAN_POINT('Ctrl Pts',(-13.3860225734551,35.1845988463221,27.9729748466449));
#52422=CARTESIAN_POINT('Ctrl Pts',(-13.3898311805857,35.0907535031083,27.9784785216751));
#52423=CARTESIAN_POINT('Ctrl Pts',(-13.3897486873307,34.9970168406318,27.9839821967053));
#52424=CARTESIAN_POINT('Ctrl Pts',(-13.1787500528927,36.1772651204102,29.1634930667589));
#52425=CARTESIAN_POINT('Ctrl Pts',(-13.1340997732529,36.2978259663116,29.1566764234979));
#52426=CARTESIAN_POINT('Ctrl Pts',(-13.0826198232573,36.41576798799,29.1498320161008));
#52427=CARTESIAN_POINT('Ctrl Pts',(-12.9813950356215,36.6158049004878,29.1376012013059));
#52428=CARTESIAN_POINT('Ctrl Pts',(-12.9346513179956,36.6992237348765,29.1322991726627));
#52429=CARTESIAN_POINT('Ctrl Pts',(-12.8649284543159,36.8121729879274,29.1247662297391));
#52430=CARTESIAN_POINT('Ctrl Pts',(-12.8448907318852,36.8434702479803,29.1226396230188));
#52431=CARTESIAN_POINT('Ctrl Pts',(-12.8094970446573,36.8968005226064,29.1189441170519));
#52432=CARTESIAN_POINT('Ctrl Pts',(-12.7943861046324,36.9189924709694,29.1173843508491));
#52433=CARTESIAN_POINT('Ctrl Pts',(-12.7628785646721,36.9641031262805,29.1141671402946));
#52434=CARTESIAN_POINT('Ctrl Pts',(-12.7464566298163,36.9870015003217,29.112508814953));
#52435=CARTESIAN_POINT('Ctrl Pts',(-12.703611945471,37.0451971554304,29.1082275934675));
#52436=CARTESIAN_POINT('Ctrl Pts',(-12.6767831641732,37.0801876290235,29.1055892428217));
#52437=CARTESIAN_POINT('Ctrl Pts',(-12.5489147893049,37.2403844470123,29.0932020505005));
#52438=CARTESIAN_POINT('Ctrl Pts',(-12.4397375318726,37.3588044030552,29.083135192241));
#52439=CARTESIAN_POINT('Ctrl Pts',(-12.1783483932242,37.604690743149,29.0602208107304));
#52440=CARTESIAN_POINT('Ctrl Pts',(-12.0225113048132,37.7274643236076,29.047303568469));
#52441=CARTESIAN_POINT('Ctrl Pts',(-11.7843239013872,37.8834195910559,29.0292318324245));
#52442=CARTESIAN_POINT('Ctrl Pts',(-11.7099957716762,37.9281115361742,29.0238068166022));
#52443=CARTESIAN_POINT('Ctrl Pts',(-11.6123415322459,37.9818404798989,29.0170234193192));
#52444=CARTESIAN_POINT('Ctrl Pts',(-11.5905219747764,37.9935360012297,29.0155291620398));
#52445=CARTESIAN_POINT('Ctrl Pts',(-11.5546660594003,38.0122524291996,29.0131108283773));
#52446=CARTESIAN_POINT('Ctrl Pts',(-11.5407058922779,38.0194166054924,29.0121783622819));
#52447=CARTESIAN_POINT('Ctrl Pts',(-11.5124972722046,38.0336463159682,29.0103131610728));
#52448=CARTESIAN_POINT('Ctrl Pts',(-11.498247964132,38.0407089682028,29.0093805753041));
#52449=CARTESIAN_POINT('Ctrl Pts',(-11.4610946009087,38.058799404492,29.0069724922851));
#52450=CARTESIAN_POINT('Ctrl Pts',(-11.4381148559781,38.0696704990969,29.005506114745));
#52451=CARTESIAN_POINT('Ctrl Pts',(-11.3372718719565,38.1159955572945,28.9991620347915));
#52452=CARTESIAN_POINT('Ctrl Pts',(-11.2581991612164,38.1487555447543,28.9944218014761));
#52453=CARTESIAN_POINT('Ctrl Pts',(-10.9923722884826,38.2472724304766,28.9789898181308));
#52454=CARTESIAN_POINT('Ctrl Pts',(-10.8011041296688,38.2996697364071,28.9686683052612));
#52455=CARTESIAN_POINT('Ctrl Pts',(-10.4494835159672,38.3635977653688,28.9495866759908));
#52456=CARTESIAN_POINT('Ctrl Pts',(-10.2908164197036,38.3810122252611,28.9409407273694));
#52457=CARTESIAN_POINT('Ctrl Pts',(-10.0873559290081,38.3889124561683,28.9294613299639));
#52458=CARTESIAN_POINT('Ctrl Pts',(-10.043161520813,38.3897633433184,28.9269452563885));
#52459=CARTESIAN_POINT('Ctrl Pts',(-9.97061338937728,38.3897411810286,28.9227720342434));
#52460=CARTESIAN_POINT('Ctrl Pts',(-9.94226416880182,38.389376838031,28.9211305507055));
#52461=CARTESIAN_POINT('Ctrl Pts',(-9.88683586167956,38.3879688829505,28.9178987169633));
#52462=CARTESIAN_POINT('Ctrl Pts',(-9.85975809258015,38.3869560697033,28.916309435822));
#52463=CARTESIAN_POINT('Ctrl Pts',(-9.79508235974244,38.3837600476191,28.9124872327553));
#52464=CARTESIAN_POINT('Ctrl Pts',(-9.75750355804307,38.3812747009975,28.9102452089159));
#52465=CARTESIAN_POINT('Ctrl Pts',(-9.62219348183156,38.3700584908048,28.9020929210222));
#52466=CARTESIAN_POINT('Ctrl Pts',(-9.52481804690792,38.3577122057406,28.8960746001056));
#52467=CARTESIAN_POINT('Ctrl Pts',(-9.26544685933983,38.3133178482844,28.8796442399029));
#52468=CARTESIAN_POINT('Ctrl Pts',(-9.1050346499253,38.2736329086204,28.8690476126876));
#52469=CARTESIAN_POINT('Ctrl Pts',(-8.78242301563198,38.1683289195128,28.8471837095783));
#52470=CARTESIAN_POINT('Ctrl Pts',(-8.62109057411236,38.1015189170032,28.8359452921324));
#52471=CARTESIAN_POINT('Ctrl Pts',(-8.43387924625587,38.0064824601605,28.8230213642665));
#52472=CARTESIAN_POINT('Ctrl Pts',(-8.40240727777856,37.9898777077718,28.8208535137542));
#52473=CARTESIAN_POINT('Ctrl Pts',(-8.35536573074415,37.9641034441352,28.8176269048468));
#52474=CARTESIAN_POINT('Ctrl Pts',(-8.33959935001169,37.9553004620166,28.8165478431187));
#52475=CARTESIAN_POINT('Ctrl Pts',(-8.31088455279339,37.9389655352719,28.8145879785283));
#52476=CARTESIAN_POINT('Ctrl Pts',(-8.29791504920588,37.9314733913885,28.8137049220446));
#52477=CARTESIAN_POINT('Ctrl Pts',(-8.2678448661108,37.9138357824356,28.811662177695));
#52478=CARTESIAN_POINT('Ctrl Pts',(-8.25078324390662,37.903625519335,28.8105065403981));
#52479=CARTESIAN_POINT('Ctrl Pts',(-8.19474615306908,37.8694177915735,28.8067189357706));
#52480=CARTESIAN_POINT('Ctrl Pts',(-8.15616533025121,37.8447801399108,28.8041240519016));
#52481=CARTESIAN_POINT('Ctrl Pts',(-8.06165447403324,37.7816948555124,28.7977693707605));
#52482=CARTESIAN_POINT('Ctrl Pts',(-8.00635648869059,37.7423340650285,28.7940529073192));
#52483=CARTESIAN_POINT('Ctrl Pts',(-7.71814109732992,37.5238549503901,28.7744865493603));
#52484=CARTESIAN_POINT('Ctrl Pts',(-7.50807853074206,37.3166918242718,28.7594026136538));
#52485=CARTESIAN_POINT('Ctrl Pts',(-7.28297096457466,37.0281430574878,28.7391799358052));
#52486=CARTESIAN_POINT('Ctrl Pts',(-7.24042011243293,36.969855039468,28.7351364129057));
#52487=CARTESIAN_POINT('Ctrl Pts',(-7.18075111425743,36.8823865114958,28.7291003182185));
#52488=CARTESIAN_POINT('Ctrl Pts',(-7.16215655099264,36.8542350715453,28.7271623450142));
#52489=CARTESIAN_POINT('Ctrl Pts',(-7.12970434838394,36.8034719152132,28.7236736095929));
#52490=CARTESIAN_POINT('Ctrl Pts',(-7.1156858742824,36.7809660417894,28.722128887862));
#52491=CARTESIAN_POINT('Ctrl Pts',(-7.08637570856987,36.7326563719046,28.7188162153526));
#52492=CARTESIAN_POINT('Ctrl Pts',(-7.07115966698711,36.7068095476301,28.7170457175915));
#52493=CARTESIAN_POINT('Ctrl Pts',(-7.03034491185258,36.6353261112097,28.712152665751));
#52494=CARTESIAN_POINT('Ctrl Pts',(-7.00545757521113,36.5892948255175,28.709005594645));
#52495=CARTESIAN_POINT('Ctrl Pts',(-6.9041052258938,36.390995958567,28.6954584094061));
#52496=CARTESIAN_POINT('Ctrl Pts',(-6.83812190722855,36.2336726590953,28.6847183628502));
#52497=CARTESIAN_POINT('Ctrl Pts',(-6.72459255235124,35.8931346448058,28.6617034042423));
#52498=CARTESIAN_POINT('Ctrl Pts',(-6.67997647958966,35.7095272700911,28.6494250784797));
#52499=CARTESIAN_POINT('Ctrl Pts',(-6.63987052987213,35.4527795868413,28.6330367752806));
#52500=CARTESIAN_POINT('Ctrl Pts',(-6.63109697931263,35.3820644678309,28.6286055876014));
#52501=CARTESIAN_POINT('Ctrl Pts',(-6.62235174607254,35.2871848434436,28.6228139225835));
#52502=CARTESIAN_POINT('Ctrl Pts',(-6.6204001168107,35.2632253085789,28.6213644529538));
#52503=CARTESIAN_POINT('Ctrl Pts',(-6.61771077589324,35.2252165336518,28.619087883612));
#52504=CARTESIAN_POINT('Ctrl Pts',(-6.61680539691678,35.2111804345761,28.6182521064136));
#52505=CARTESIAN_POINT('Ctrl Pts',(-6.61507480444282,35.1814737210962,28.6164942243093));
#52506=CARTESIAN_POINT('Ctrl Pts',(-6.61427098986582,35.1658022214602,28.6155733718771));
#52507=CARTESIAN_POINT('Ctrl Pts',(-6.61249248523683,35.1256839683633,28.6132314091921));
#52508=CARTESIAN_POINT('Ctrl Pts',(-6.61167356374995,35.1012307161939,28.6118185077685));
#52509=CARTESIAN_POINT('Ctrl Pts',(-6.60925192835746,34.9943317482969,28.6056974598744));
#52510=CARTESIAN_POINT('Ctrl Pts',(-6.61039300101457,34.9118463935938,28.6011184023175));
#52511=CARTESIAN_POINT('Ctrl Pts',(-6.62349217277806,34.6517805178474,28.5869136834067));
#52512=CARTESIAN_POINT('Ctrl Pts',(-6.64641977743063,34.4750543916973,28.5775920815758));
#52513=CARTESIAN_POINT('Ctrl Pts',(-6.72082339736006,34.1220268081602,28.558407957436));
#52514=CARTESIAN_POINT('Ctrl Pts',(-6.77293962969238,33.9464784832982,28.5485639389132));
#52515=CARTESIAN_POINT('Ctrl Pts',(-6.85511764533768,33.734249503145,28.5357410936755));
#52516=CARTESIAN_POINT('Ctrl Pts',(-6.87210824112787,33.6928266272056,28.5331938811931));
#52517=CARTESIAN_POINT('Ctrl Pts',(-6.90121583554541,33.6256822701297,28.5289856285119));
#52518=CARTESIAN_POINT('Ctrl Pts',(-6.91284511967554,33.5997545951006,28.5273409158588));
#52519=CARTESIAN_POINT('Ctrl Pts',(-6.93613455580945,33.5495312182144,28.524114986212));
#52520=CARTESIAN_POINT('Ctrl Pts',(-6.94776119364708,33.5252222697665,28.5225350004613));
#52521=CARTESIAN_POINT('Ctrl Pts',(-6.97608076226448,33.4677814289795,28.5187560223172));
#52522=CARTESIAN_POINT('Ctrl Pts',(-6.99302996320553,33.4347804181616,28.5165483558338));
#52523=CARTESIAN_POINT('Ctrl Pts',(-7.05495576317059,33.3189270482988,28.5086647420849));
#52524=CARTESIAN_POINT('Ctrl Pts',(-7.10283983064361,33.2376855484804,28.5028895216227));
#52525=CARTESIAN_POINT('Ctrl Pts',(-7.23758730060364,33.0294336322828,28.4874257376625));
#52526=CARTESIAN_POINT('Ctrl Pts',(-7.3298143872892,32.9061620302669,28.4775795336394));
#52527=CARTESIAN_POINT('Ctrl Pts',(-7.55611262699796,32.6430584241577,28.4552184612015));
#52528=CARTESIAN_POINT('Ctrl Pts',(-7.69445205054928,32.5075678686494,28.4427018649977));
#52529=CARTESIAN_POINT('Ctrl Pts',(-7.87029390474128,32.3625856290245,28.42867691504));
#52530=CARTESIAN_POINT('Ctrl Pts',(-7.89733100112303,32.3409802752037,28.4265686793645));
#52531=CARTESIAN_POINT('Ctrl Pts',(-7.93895651029983,32.308749339852,28.4234013367194));
#52532=CARTESIAN_POINT('Ctrl Pts',(-7.9533059718195,32.2978205149634,28.4223233064071));
#52533=CARTESIAN_POINT('Ctrl Pts',(-7.97969701894987,32.278051426867,28.4203668266139));
#52534=CARTESIAN_POINT('Ctrl Pts',(-7.9917103766311,32.2691757708859,28.4194861033334));
#52535=CARTESIAN_POINT('Ctrl Pts',(-8.01976187803375,32.2487361194797,28.417452028865));
#52536=CARTESIAN_POINT('Ctrl Pts',(-8.03584302472087,32.2372326595824,28.4163026635101));
#52537=CARTESIAN_POINT('Ctrl Pts',(-8.08899271888234,32.1999112934116,28.4125551998561));
#52538=CARTESIAN_POINT('Ctrl Pts',(-8.12647818199344,32.1746925838617,28.4099931820598));
#52539=CARTESIAN_POINT('Ctrl Pts',(-8.2204679809656,32.1141536069279,28.4037379308024));
#52540=CARTESIAN_POINT('Ctrl Pts',(-8.27753189213291,32.0797349234868,28.4000863663814));
#52541=CARTESIAN_POINT('Ctrl Pts',(-8.57608129324753,31.9114599425304,28.3815326206433));
#52542=CARTESIAN_POINT('Ctrl Pts',(-8.83224366531921,31.8057897946612,28.3673297398342));
#52543=CARTESIAN_POINT('Ctrl Pts',(-9.17958725809878,31.7099510199929,28.3475727265831));
#52544=CARTESIAN_POINT('Ctrl Pts',(-9.26158267448962,31.6905834830818,28.3428829923911));
#52545=CARTESIAN_POINT('Ctrl Pts',(-9.37664190367164,31.6678951903215,28.3362217466616));
#52546=CARTESIAN_POINT('Ctrl Pts',(-9.40916462110694,31.6619749513302,28.3343301857832));
#52547=CARTESIAN_POINT('Ctrl Pts',(-9.46848796849109,31.652070208988,28.3308615696132));
#52548=CARTESIAN_POINT('Ctrl Pts',(-9.49525993021783,31.6479295465497,28.3292894900063));
#52549=CARTESIAN_POINT('Ctrl Pts',(-9.54958058399104,31.6401935859481,28.3260848844295));
#52550=CARTESIAN_POINT('Ctrl Pts',(-9.57712954967957,31.6366152013296,28.3244519636475));
#52551=CARTESIAN_POINT('Ctrl Pts',(-9.64595472657706,31.6285343171899,28.3203520776345));
#52552=CARTESIAN_POINT('Ctrl Pts',(-9.68727468149272,31.6244509259057,28.3178724010656));
#52553=CARTESIAN_POINT('Ctrl Pts',(-9.86319511018777,31.6103235438391,28.3072335234283));
#52554=CARTESIAN_POINT('Ctrl Pts',(-9.99824260213392,31.6075654936302,28.2988570401372));
#52555=CARTESIAN_POINT('Ctrl Pts',(-10.2714192023481,31.6182987677193,28.2815427891607));
#52556=CARTESIAN_POINT('Ctrl Pts',(-10.4092872932831,31.6322036499239,28.2726120659514));
#52557=CARTESIAN_POINT('Ctrl Pts',(-10.7119507475226,31.6815916154419,28.2528520401303));
#52558=CARTESIAN_POINT('Ctrl Pts',(-10.8757576764483,31.7210113430549,28.2420520586333));
#52559=CARTESIAN_POINT('Ctrl Pts',(-11.0632901221813,31.7812048275565,28.2300109273435));
#52560=CARTESIAN_POINT('Ctrl Pts',(-11.0904971058809,31.7903201987758,28.2282725536309));
#52561=CARTESIAN_POINT('Ctrl Pts',(-11.1332663717901,31.8052561523624,28.2255569506633));
#52562=CARTESIAN_POINT('Ctrl Pts',(-11.1489066268253,31.8108473680556,28.2245675332994));
#52563=CARTESIAN_POINT('Ctrl Pts',(-11.1788958591213,31.8218174363999,28.2226782837185));
#52564=CARTESIAN_POINT('Ctrl Pts',(-11.1932503498736,31.8271789424723,28.2217775833855));
#52565=CARTESIAN_POINT('Ctrl Pts',(-11.2286286510776,31.840667045969,28.2195656129329));
#52566=CARTESIAN_POINT('Ctrl Pts',(-11.2496091217785,31.8489065107042,28.2182607486445));
#52567=CARTESIAN_POINT('Ctrl Pts',(-11.3301577382648,31.8814706509055,28.2132721469493));
#52568=CARTESIAN_POINT('Ctrl Pts',(-11.3891142118089,31.9072815072418,28.2096654236234));
#52569=CARTESIAN_POINT('Ctrl Pts',(-11.5499393493573,31.9832176724604,28.1998584665326));
#52570=CARTESIAN_POINT('Ctrl Pts',(-11.6500822268752,32.0368059221728,28.1937865090452));
#52571=CARTESIAN_POINT('Ctrl Pts',(-11.9698095288514,32.2291425492032,28.1739537020739));
#52572=CARTESIAN_POINT('Ctrl Pts',(-12.1761372084177,32.3880626871785,28.1603498002044));
#52573=CARTESIAN_POINT('Ctrl Pts',(-12.3981429066633,32.603791988108,28.1429838574218));
#52574=CARTESIAN_POINT('Ctrl Pts',(-12.4332053684795,32.6394039921987,28.1401503273009));
#52575=CARTESIAN_POINT('Ctrl Pts',(-12.4876955319896,32.6972524207712,28.1355904487289));
#52576=CARTESIAN_POINT('Ctrl Pts',(-12.5076427218605,32.7189907116535,28.1338861811608));
#52577=CARTESIAN_POINT('Ctrl Pts',(-12.5450267154039,32.7608145740583,28.1306229617614));
#52578=CARTESIAN_POINT('Ctrl Pts',(-12.5625158976558,32.7808504853694,28.1290663541624));
#52579=CARTESIAN_POINT('Ctrl Pts',(-12.6021888880244,32.8273949384578,28.1254643061819));
#52580=CARTESIAN_POINT('Ctrl Pts',(-12.6242063182923,32.8540408138312,28.1234123875122));
#52581=CARTESIAN_POINT('Ctrl Pts',(-12.6940337166738,32.9412289812792,28.1167284925802));
#52582=CARTESIAN_POINT('Ctrl Pts',(-12.7401830228991,33.0030645107109,28.1120334800256));
#52583=CARTESIAN_POINT('Ctrl Pts',(-12.8480817564917,33.15842867765,28.1003430847857));
#52584=CARTESIAN_POINT('Ctrl Pts',(-12.9073777637715,33.2535448074914,28.0932732335558));
#52585=CARTESIAN_POINT('Ctrl Pts',(-13.0535958821052,33.5162407491064,28.0740631072902));
#52586=CARTESIAN_POINT('Ctrl Pts',(-13.1314182896993,33.68843310281,28.0617804378806));
#52587=CARTESIAN_POINT('Ctrl Pts',(-13.2235449280478,33.9480032103652,28.0442983313558));
#52588=CARTESIAN_POINT('Ctrl Pts',(-13.249427069796,34.0308946335839,28.0388649674589));
#52589=CARTESIAN_POINT('Ctrl Pts',(-13.2787663606448,34.1393329772367,28.0320231382096));
#52590=CARTESIAN_POINT('Ctrl Pts',(-13.2851543917797,34.1640470831912,28.0304814613219));
#52591=CARTESIAN_POINT('Ctrl Pts',(-13.2950731792533,34.2042919250356,28.0280021316696));
#52592=CARTESIAN_POINT('Ctrl Pts',(-13.2987746104736,34.2197790766284,28.0270554746875));
#52593=CARTESIAN_POINT('Ctrl Pts',(-13.3059269514276,34.2506662337536,28.0251830800681));
#52594=CARTESIAN_POINT('Ctrl Pts',(-13.3093797099731,34.2660653598568,28.0242572714105));
#52595=CARTESIAN_POINT('Ctrl Pts',(-13.3179952213584,34.3057874969596,28.021887629523));
#52596=CARTESIAN_POINT('Ctrl Pts',(-13.3229982254408,34.3301446727635,28.0204523801437));
#52597=CARTESIAN_POINT('Ctrl Pts',(-13.3334405736123,34.3839825207823,28.0173147761501));
#52598=CARTESIAN_POINT('Ctrl Pts',(-13.3387578257398,34.4134849626792,28.0156182857639));
#52599=CARTESIAN_POINT('Ctrl Pts',(-13.3741761586187,34.626122980991,28.0035303339155));
#52600=CARTESIAN_POINT('Ctrl Pts',(-13.3895850560083,34.8113982025932,27.9937269914139));
#52601=CARTESIAN_POINT('Ctrl Pts',(-13.3897486828745,34.99701178137,27.9838867651182));
#52602=CARTESIAN_POINT('Origin',(-10.,35.,32.7603849714045));
#52603=CARTESIAN_POINT('',(-14.0849984180973,34.9964049836978,28.3853849713664));
#52604=CARTESIAN_POINT('Ctrl Pts',(-7.51282733495086,38.2405550657615,29.1925543226443));
#52605=CARTESIAN_POINT('Ctrl Pts',(-7.4182955070919,38.168000526969,29.1867402514207));
#52606=CARTESIAN_POINT('Ctrl Pts',(-7.326830655408,38.0912213338729,29.1809261801971));
#52607=CARTESIAN_POINT('Ctrl Pts',(-7.23882967629141,38.0105088346442,29.1751121089736));
#52608=CARTESIAN_POINT('Ctrl Pts',(-7.15090483531155,37.9298661675852,29.1693030680639));
#52609=CARTESIAN_POINT('Ctrl Pts',(-7.06643820360961,37.8452972399229,29.1634940271543));
#52610=CARTESIAN_POINT('Ctrl Pts',(-6.98579419832905,37.7571340890811,29.1576849862446));
#52611=CARTESIAN_POINT('Ctrl Pts',(-6.90519362828907,37.6690184233271,29.1518790741118));
#52612=CARTESIAN_POINT('Ctrl Pts',(-6.8284118645769,37.5773126851313,29.1460731619789));
#52613=CARTESIAN_POINT('Ctrl Pts',(-6.75577661811945,37.4823858782348,29.140267249846));
#52614=CARTESIAN_POINT('Ctrl Pts',(-6.68316100431293,37.3874847291966,29.1344629069987));
#52615=CARTESIAN_POINT('Ctrl Pts',(-6.6146899270105,37.289364566574,29.1286585641514));
#52616=CARTESIAN_POINT('Ctrl Pts',(-6.55065054055114,37.1884271307493,29.1228542213041));
#52617=CARTESIAN_POINT('Ctrl Pts',(-6.48661336469559,37.0874931792285,29.1170500788195));
#52618=CARTESIAN_POINT('Ctrl Pts',(-6.42700779398407,36.9837424926554,29.1112459363349));
#52619=CARTESIAN_POINT('Ctrl Pts',(-6.37207704802374,36.8776048717778,29.1054417938503));
#52620=CARTESIAN_POINT('Ctrl Pts',(-6.3171352472389,36.7714458906811,29.0996364832807));
#52621=CARTESIAN_POINT('Ctrl Pts',(-6.26687032970223,36.6628993824746,29.0938311727112));
#52622=CARTESIAN_POINT('Ctrl Pts',(-6.22147875497343,36.5524181784825,29.0880258621416));
#52623=CARTESIAN_POINT('Ctrl Pts',(-6.17603959747876,36.4418211600183,29.0822144660213));
#52624=CARTESIAN_POINT('Ctrl Pts',(-6.13548414107057,36.3292857734194,29.0764030699009));
#52625=CARTESIAN_POINT('Ctrl Pts',(-6.09996010488476,36.2152834305254,29.0705916737806));
#52626=CARTESIAN_POINT('Ctrl Pts',(-6.0644166719999,36.1012188405059,29.0647771045439));
#52627=CARTESIAN_POINT('Ctrl Pts',(-6.03391023664728,35.9856860929482,29.0589625353071));
#52628=CARTESIAN_POINT('Ctrl Pts',(-6.00853774778895,35.8691686195292,29.0531479660704));
#52629=CARTESIAN_POINT('Ctrl Pts',(-5.98312519279018,35.7524671513322,29.0473242149458));
#52630=CARTESIAN_POINT('Ctrl Pts',(-5.96286284996756,35.6347782530207,29.0415004638212));
#52631=CARTESIAN_POINT('Ctrl Pts',(-5.94779605265521,35.5165928465662,29.0356767126966));
#52632=CARTESIAN_POINT('Ctrl Pts',(-5.93586929503933,35.4230382133355,29.031066677356));
#52633=CARTESIAN_POINT('Ctrl Pts',(-5.92719713286778,35.3291726322501,29.0264566420155));
#52634=CARTESIAN_POINT('Ctrl Pts',(-5.92177888757647,35.2352393635917,29.021846606675));
#52635=CARTESIAN_POINT('Ctrl Pts',(-5.91493527095027,35.1165951818349,29.0160238148286));
#52636=CARTESIAN_POINT('Ctrl Pts',(-5.91326230607475,34.9974602544536,29.0102010229823));
#52637=CARTESIAN_POINT('Ctrl Pts',(-5.91681257285023,34.8783224146935,29.0043782311359));
#52638=CARTESIAN_POINT('Ctrl Pts',(-5.92035835323838,34.7593351265758,28.9985627974125));
#52639=CARTESIAN_POINT('Ctrl Pts',(-5.92911422513116,34.6403453380733,28.9927473636891));
#52640=CARTESIAN_POINT('Ctrl Pts',(-5.94308090843529,34.5218447067137,28.9869319299657));
#52641=CARTESIAN_POINT('Ctrl Pts',(-5.95703358566419,34.4034629102071,28.9811223280781));
#52642=CARTESIAN_POINT('Ctrl Pts',(-5.97618663134419,34.2855696983084,28.9753127261904));
#52643=CARTESIAN_POINT('Ctrl Pts',(-6.00048875566094,34.168654821145,28.9695031243027));
#52644=CARTESIAN_POINT('Ctrl Pts',(-6.02571561004793,34.0472911681807,28.9634724588778));
#52645=CARTESIAN_POINT('Ctrl Pts',(-6.05649117123816,33.9269822308918,28.957441793453));
#52646=CARTESIAN_POINT('Ctrl Pts',(-6.09269907735653,33.8082682768721,28.9514111280282));
#52647=CARTESIAN_POINT('Ctrl Pts',(-6.12754034506295,33.6940350859505,28.9456080852389));
#52648=CARTESIAN_POINT('Ctrl Pts',(-6.16741118247509,33.5812790842382,28.9398050424496));
#52649=CARTESIAN_POINT('Ctrl Pts',(-6.21215642369427,33.4704686856951,28.9340019996604));
#52650=CARTESIAN_POINT('Ctrl Pts',(-6.25689501143066,33.3596747643249,28.9281998197661));
#52651=CARTESIAN_POINT('Ctrl Pts',(-6.30650640866777,33.2508262494438,28.9223976398718));
#52652=CARTESIAN_POINT('Ctrl Pts',(-6.36078684226828,33.1443727226104,28.9165954599776));
#52653=CARTESIAN_POINT('Ctrl Pts',(-6.41507202504557,33.0379098818017,28.9107927724312));
#52654=CARTESIAN_POINT('Ctrl Pts',(-6.47402687083369,32.933842809575,28.9049900848848));
#52655=CARTESIAN_POINT('Ctrl Pts',(-6.53740137837309,32.8325969951328,28.8991873973384));
#52656=CARTESIAN_POINT('Ctrl Pts',(-6.60079639912306,32.7313184092058,28.8933828315644));
#52657=CARTESIAN_POINT('Ctrl Pts',(-6.66861371006093,32.6328632432358,28.8875782657903));
#52658=CARTESIAN_POINT('Ctrl Pts',(-6.74056004306344,32.5376279389326,28.8817737000163));
#52659=CARTESIAN_POINT('Ctrl Pts',(-6.81258604500554,32.4422871769168,28.8759627066235));
#52660=CARTESIAN_POINT('Ctrl Pts',(-6.88874994918451,32.3501737196662,28.8701517132307));
#52661=CARTESIAN_POINT('Ctrl Pts',(-6.96871816790781,32.2616509619065,28.8643407198379));
#52662=CARTESIAN_POINT('Ctrl Pts',(-7.04873889325022,32.1730700806722,28.8585259109842));
#52663=CARTESIAN_POINT('Ctrl Pts',(-7.13256862151863,32.0880848843044,28.8527111021304));
#52664=CARTESIAN_POINT('Ctrl Pts',(-7.21983808480828,32.0070207609612,28.8468962932767));
#52665=CARTESIAN_POINT('Ctrl Pts',(-7.30723262912441,31.925840450542,28.8410731502103));
#52666=CARTESIAN_POINT('Ctrl Pts',(-7.39807643854486,31.8485926939445,28.835250007144));
#52667=CARTESIAN_POINT('Ctrl Pts',(-7.49196839527695,31.7755616815156,28.8294268640776));
#52668=CARTESIAN_POINT('Ctrl Pts',(-7.5170126758887,31.7560817470006,28.8278736274206));
#52669=CARTESIAN_POINT('Ctrl Pts',(-7.54227367435121,31.7369015790538,28.8263203907635));
#52670=CARTESIAN_POINT('Ctrl Pts',(-7.56774346416096,31.7180260293737,28.8247671541065));
#52671=CARTESIAN_POINT('Ctrl Pts',(-7.66324135127727,31.6472529634761,28.8189433597193));
#52672=CARTESIAN_POINT('Ctrl Pts',(-7.76198471764007,31.5805374438546,28.8131195653321));
#52673=CARTESIAN_POINT('Ctrl Pts',(-7.86359415317665,31.5181908355484,28.8072957709449));
#52674=CARTESIAN_POINT('Ctrl Pts',(-7.96507542051418,31.4559228700618,28.8014793225805));
#52675=CARTESIAN_POINT('Ctrl Pts',(-8.06941522150667,31.3980130665553,28.7956628742162));
#52676=CARTESIAN_POINT('Ctrl Pts',(-8.17620253501886,31.3447315000498,28.7898464258519));
#52677=CARTESIAN_POINT('Ctrl Pts',(-8.28288297680706,31.2915032572274,28.7840357985335));
#52678=CARTESIAN_POINT('Ctrl Pts',(-8.39200569498173,31.2428942180532,28.7782251712152));
#52679=CARTESIAN_POINT('Ctrl Pts',(-8.50313276851186,31.1991299033909,28.7724145438969));
#52680=CARTESIAN_POINT('Ctrl Pts',(-8.61846075270562,31.1537111766191,28.7663842587986));
#52681=CARTESIAN_POINT('Ctrl Pts',(-8.73594724104708,31.11351092483,28.7603539737003));
#52682=CARTESIAN_POINT('Ctrl Pts',(-8.85507675928502,31.0787277864358,28.754323688602));
#52683=CARTESIAN_POINT('Ctrl Pts',(-8.96973771927774,31.0452493664872,28.7485196000048));
#52684=CARTESIAN_POINT('Ctrl Pts',(-9.08592024167654,31.0167891113456,28.7427155114076));
#52685=CARTESIAN_POINT('Ctrl Pts',(-9.20314733844475,30.9934739691633,28.7369114228103));
#52686=CARTESIAN_POINT('Ctrl Pts',(-9.32035712252227,30.9701622702791,28.7311081913903));
#52687=CARTESIAN_POINT('Ctrl Pts',(-9.4386107738259,30.9519942528622,28.7253049599702));
#52688=CARTESIAN_POINT('Ctrl Pts',(-9.5574204195789,30.9390458861255,28.7195017285501));
#52689=CARTESIAN_POINT('Ctrl Pts',(-9.6762405524279,30.9260963764617,28.7136979848901));
#52690=CARTESIAN_POINT('Ctrl Pts',(-9.79561637138188,30.9183674777574,28.7078942412301));
#52691=CARTESIAN_POINT('Ctrl Pts',(-9.91505482028812,30.9158832880972,28.7020904975701));
#52692=CARTESIAN_POINT('Ctrl Pts',(-10.0345319934913,30.9133982930138,28.6962848722221));
#52693=CARTESIAN_POINT('Ctrl Pts',(-10.1540714290248,30.9161613972532,28.6904792468742));
#52694=CARTESIAN_POINT('Ctrl Pts',(-10.273180652745,30.9241445890506,28.6846736215262));
#52695=CARTESIAN_POINT('Ctrl Pts',(-10.3924217429472,30.9321366190838,28.6788615687382));
#52696=CARTESIAN_POINT('Ctrl Pts',(-10.5112312629886,30.9453602451132,28.6730495159502));
#52697=CARTESIAN_POINT('Ctrl Pts',(-10.6291222796832,30.9637356185197,28.6672374631622));
#52698=CARTESIAN_POINT('Ctrl Pts',(-10.7470907118857,30.9821230584849,28.6614215937729));
#52699=CARTESIAN_POINT('Ctrl Pts',(-10.8641390401765,31.0056689028319,28.6556057243835));
#52700=CARTESIAN_POINT('Ctrl Pts',(-10.979792560757,31.0342426274562,28.6497898549941));
#52701=CARTESIAN_POINT('Ctrl Pts',(-11.0956116870234,31.0628572671452,28.6439656577905));
#52702=CARTESIAN_POINT('Ctrl Pts',(-11.2100316288698,31.0965140420848,28.6381414605868));
#52703=CARTESIAN_POINT('Ctrl Pts',(-11.3225946799007,31.1350332067793,28.6323172633832));
#52704=CARTESIAN_POINT('Ctrl Pts',(-11.3524195403347,31.1452392975038,28.6307740761015));
#52705=CARTESIAN_POINT('Ctrl Pts',(-11.3821141592751,31.1557864931314,28.6292308888198));
#52706=CARTESIAN_POINT('Ctrl Pts',(-11.4116702973451,31.1666709022582,28.6276877015381));
#52707=CARTESIAN_POINT('Ctrl Pts',(-11.5232093526256,31.2077465227747,28.6218640160785));
#52708=CARTESIAN_POINT('Ctrl Pts',(-11.6331339345893,31.2537606017622,28.6160403306189));
#52709=CARTESIAN_POINT('Ctrl Pts',(-11.7409756606022,31.3045665005049,28.6102166451593));
#52710=CARTESIAN_POINT('Ctrl Pts',(-11.8486813676145,31.3553083186006,28.6044003050186));
#52711=CARTESIAN_POINT('Ctrl Pts',(-11.9543090777373,31.4108297628885,28.598583964878));
#52712=CARTESIAN_POINT('Ctrl Pts',(-12.0574076135075,31.4709351221774,28.5927676247373));
#52713=CARTESIAN_POINT('Ctrl Pts',(-12.1604029821413,31.5309803361135,28.586957104807));
#52714=CARTESIAN_POINT('Ctrl Pts',(-12.260873860528,31.5956001353734,28.5811465848766));
#52715=CARTESIAN_POINT('Ctrl Pts',(-12.3583915891281,31.6645518873276,28.5753360649462));
#52716=CARTESIAN_POINT('Ctrl Pts',(-12.4595983087819,31.7361120100853,28.5693057392805));
#52717=CARTESIAN_POINT('Ctrl Pts',(-12.5576236322438,31.8123381126629,28.5632754136148));
#52718=CARTESIAN_POINT('Ctrl Pts',(-12.6520188398351,31.8929079393813,28.5572450879491));
#52719=CARTESIAN_POINT('Ctrl Pts',(-12.742871027128,31.9704536662669,28.551441103925));
#52720=CARTESIAN_POINT('Ctrl Pts',(-12.8303603536366,32.0520226312833,28.5456371199008));
#52721=CARTESIAN_POINT('Ctrl Pts',(-12.91411918878,32.1372854921274,28.5398331358767));
#52722=CARTESIAN_POINT('Ctrl Pts',(-12.9978656715284,32.2225357787692,28.5340300077993));
#52723=CARTESIAN_POINT('Ctrl Pts',(-13.0778824709313,32.3114785866766,28.5282268797219));
#52724=CARTESIAN_POINT('Ctrl Pts',(-13.1538386274584,32.4037475253836,28.5224237516445));
#52725=CARTESIAN_POINT('Ctrl Pts',(-13.2298015062869,32.4960246301124,28.5166201099764));
#52726=CARTESIAN_POINT('Ctrl Pts',(-13.3017027681857,32.5916281356603,28.5108164683083));
#52727=CARTESIAN_POINT('Ctrl Pts',(-13.3692519962592,32.6901588830175,28.5050128266402));
#52728=CARTESIAN_POINT('Ctrl Pts',(-13.4368231426422,32.788721601538,28.4992073018119));
#52729=CARTESIAN_POINT('Ctrl Pts',(-13.5000392159967,32.8902131142603,28.4934017769837));
#52730=CARTESIAN_POINT('Ctrl Pts',(-13.5586537021487,32.9942061850271,28.4875962521554));
#52731=CARTESIAN_POINT('Ctrl Pts',(-13.6173331091752,33.0983144375784,28.4817842971804));
#52732=CARTESIAN_POINT('Ctrl Pts',(-13.6714005549847,33.2049294228149,28.4759723422054));
#52733=CARTESIAN_POINT('Ctrl Pts',(-13.7206559180211,33.3136001246162,28.4701603872304));
#52734=CARTESIAN_POINT('Ctrl Pts',(-13.7699436385356,33.4223422157981,28.4643446141898));
#52735=CARTESIAN_POINT('Ctrl Pts',(-13.8144128288937,33.5331423349686,28.4585288411492));
#52736=CARTESIAN_POINT('Ctrl Pts',(-13.8539124552631,33.6455319172575,28.4527130681086));
#52737=CARTESIAN_POINT('Ctrl Pts',(-13.8934686622217,33.7580824901526,28.4468889643597));
#52738=CARTESIAN_POINT('Ctrl Pts',(-13.9280409789672,33.872226681134,28.4410648606108));
#52739=CARTESIAN_POINT('Ctrl Pts',(-13.9575288567085,33.9874831614638,28.4352407568619));
#52740=CARTESIAN_POINT('Ctrl Pts',(-13.9653471026424,34.0180416003109,28.4336965875645));
#52741=CARTESIAN_POINT('Ctrl Pts',(-13.9728082133453,34.0486781888914,28.4321524182671));
#52742=CARTESIAN_POINT('Ctrl Pts',(-13.9799109248485,34.0793838855029,28.4306082489697));
#52743=CARTESIAN_POINT('Ctrl Pts',(-14.015654940968,34.233908662999,28.4228372994904));
#52744=CARTESIAN_POINT('Ctrl Pts',(-14.0424112738778,34.3905837664468,28.4150663500111));
#52745=CARTESIAN_POINT('Ctrl Pts',(-14.0599741476013,34.5485191910954,28.4072954005318));
#52746=CARTESIAN_POINT('Ctrl Pts',(-14.0764805003541,34.6969537737527,28.399991924156));
#52747=CARTESIAN_POINT('Ctrl Pts',(-14.0848664953181,34.8465018450429,28.3926884477803));
#52748=CARTESIAN_POINT('Ctrl Pts',(-14.0849984180967,34.9964049829165,28.3853849714045));
#52749=CARTESIAN_POINT('Ctrl Pts',(-14.0849984180973,34.9964049836978,28.3853849713664));
#52750=CARTESIAN_POINT('Ctrl Pts',(-14.085102030525,35.1141392490068,28.3796488044156));
#52751=CARTESIAN_POINT('Ctrl Pts',(-14.0801115810811,35.2320158016211,28.3739126374648));
#52752=CARTESIAN_POINT('Ctrl Pts',(-14.0700169342151,35.3495527931545,28.368176470514));
#52753=CARTESIAN_POINT('Ctrl Pts',(-14.059929581389,35.4670048565564,28.3624444483174));
#52754=CARTESIAN_POINT('Ctrl Pts',(-14.0447454007801,35.5841174298377,28.3567124261208));
#52755=CARTESIAN_POINT('Ctrl Pts',(-14.0245063239988,35.7004097715579,28.3509804039242));
#52756=CARTESIAN_POINT('Ctrl Pts',(-14.0042749104805,35.8166580806968,28.3452505520831));
#52757=CARTESIAN_POINT('Ctrl Pts',(-13.9789924760443,35.9320863622645,28.3395207002421));
#52758=CARTESIAN_POINT('Ctrl Pts',(-13.9487526026871,36.0462207619676,28.3337908484011));
#52759=CARTESIAN_POINT('Ctrl Pts',(-13.9185165913529,36.1603405852314,28.3280617283363));
#52760=CARTESIAN_POINT('Ctrl Pts',(-13.8833245073619,36.2731664492456,28.3223326082715));
#52761=CARTESIAN_POINT('Ctrl Pts',(-13.8433204827315,36.3842372148646,28.3166034882066));
#52762=CARTESIAN_POINT('Ctrl Pts',(-13.8033115287939,36.495321666655,28.310873662198));
#52763=CARTESIAN_POINT('Ctrl Pts',(-13.7584895988473,36.6046501953671,28.3051438361894));
#52764=CARTESIAN_POINT('Ctrl Pts',(-13.7090476007998,36.7117800369793,28.2994140101808));
#52765=CARTESIAN_POINT('Ctrl Pts',(-13.6595570467352,36.8190150887092,28.2936785570223));
#52766=CARTESIAN_POINT('Ctrl Pts',(-13.6054375399421,36.9240467592881,28.2879431038639));
#52767=CARTESIAN_POINT('Ctrl Pts',(-13.5469287910702,37.0264553168223,28.2822076507054));
#52768=CARTESIAN_POINT('Ctrl Pts',(-13.4883905757711,37.1289154497938,28.2764693090334));
#52769=CARTESIAN_POINT('Ctrl Pts',(-13.4254589412614,37.2287494844963,28.2707309673615));
#52770=CARTESIAN_POINT('Ctrl Pts',(-13.358416910452,37.3255667815803,28.2649926256895));
#52771=CARTESIAN_POINT('Ctrl Pts',(-13.2912691757575,37.4225367286412,28.2592452364842));
#52772=CARTESIAN_POINT('Ctrl Pts',(-13.2199983543175,37.5164801034817,28.2534978472788));
#52773=CARTESIAN_POINT('Ctrl Pts',(-13.1449279379471,37.6070391759848,28.2477504580735));
#52774=CARTESIAN_POINT('Ctrl Pts',(-13.0830084573461,37.6817339892577,28.2430099041828));
#52775=CARTESIAN_POINT('Ctrl Pts',(-13.0185048127787,37.7541269409643,28.238269350292));
#52776=CARTESIAN_POINT('Ctrl Pts',(-12.9516163303101,37.8240371879008,28.2335287964012));
#52777=CARTESIAN_POINT('Ctrl Pts',(-12.8694458647662,37.9099197991524,28.2277051701839));
#52778=CARTESIAN_POINT('Ctrl Pts',(-12.7833914299211,37.9923515654202,28.2218815439666));
#52779=CARTESIAN_POINT('Ctrl Pts',(-12.6937743662288,38.0709615210629,28.2160579177493));
#52780=CARTESIAN_POINT('Ctrl Pts',(-12.6042703627787,38.1494723029516,28.2102416385769));
#52781=CARTESIAN_POINT('Ctrl Pts',(-12.511212974376,38.2241705973116,28.2044253594046));
#52782=CARTESIAN_POINT('Ctrl Pts',(-12.4149616736329,38.2947207946781,28.1986090802322));
#52783=CARTESIAN_POINT('Ctrl Pts',(-12.3188067164321,38.365200374236,28.1927986229129));
#52784=CARTESIAN_POINT('Ctrl Pts',(-12.2194645343185,38.431539876827,28.1869881655937));
#52785=CARTESIAN_POINT('Ctrl Pts',(-12.1173286397876,38.4934430625295,28.1811777082744));
#52786=CARTESIAN_POINT('Ctrl Pts',(-12.011327510028,38.5576889150802,28.175147359756));
#52787=CARTESIAN_POINT('Ctrl Pts',(-11.902317376978,38.6171557457961,28.1691170112376));
#52788=CARTESIAN_POINT('Ctrl Pts',(-11.7907727880757,38.6715606792599,28.1630866627192));
#52789=CARTESIAN_POINT('Ctrl Pts',(-11.6834165364236,38.723922786517,28.1572827450262));
#52790=CARTESIAN_POINT('Ctrl Pts',(-11.5737131275375,38.7715960814058,28.1514788273331));
#52791=CARTESIAN_POINT('Ctrl Pts',(-11.4621112314634,38.8143748828384,28.1456749096401));
#52792=CARTESIAN_POINT('Ctrl Pts',(-11.3505258184501,38.8571473660488,28.1398718491577));
#52793=CARTESIAN_POINT('Ctrl Pts',(-11.237042857048,38.8950266472981,28.1340687886753));
#52794=CARTESIAN_POINT('Ctrl Pts',(-11.122130356333,38.9278554534753,28.1282657281928));
#52795=CARTESIAN_POINT('Ctrl Pts',(-11.0072077091431,38.9606871583508,28.1224621553152));
#52796=CARTESIAN_POINT('Ctrl Pts',(-10.8908556643181,38.9884673893376,28.1166585824377));
#52797=CARTESIAN_POINT('Ctrl Pts',(-10.7735561008546,39.0110891237706,28.1108550095601));
#52798=CARTESIAN_POINT('Ctrl Pts',(-10.6562184984889,39.0337181941724,28.1050495546504));
#52799=CARTESIAN_POINT('Ctrl Pts',(-10.5379331671322,39.0511853638317,28.0992440997407));
#52800=CARTESIAN_POINT('Ctrl Pts',(-10.4191902130979,39.0634350696477,28.0934386448311));
#52801=CARTESIAN_POINT('Ctrl Pts',(-10.3003157660994,39.0756983404802,28.0876267611065));
#52802=CARTESIAN_POINT('Ctrl Pts',(-10.1809830913039,39.082732572781,28.0818148773819));
#52803=CARTESIAN_POINT('Ctrl Pts',(-10.0616855883498,39.0845342314871,28.0760029936573));
#52804=CARTESIAN_POINT('Ctrl Pts',(-9.94230973161859,39.0863370735102,28.0701872927276));
#52805=CARTESIAN_POINT('Ctrl Pts',(-9.8229694999585,39.0829005093515,28.0643715917978));
#52806=CARTESIAN_POINT('Ctrl Pts',(-9.70415479724293,39.0742730168713,28.0585558908681));
#52807=CARTESIAN_POINT('Ctrl Pts',(-9.58516991295967,39.0656331669962,28.0527318599499));
#52808=CARTESIAN_POINT('Ctrl Pts',(-9.46671246415969,39.0517875959597,28.0469078290317));
#52809=CARTESIAN_POINT('Ctrl Pts',(-9.34926391381397,39.0328361665378,28.0410837981136));
#52810=CARTESIAN_POINT('Ctrl Pts',(-9.31811080899898,39.0278093197573,28.03953898002));
#52811=CARTESIAN_POINT('Ctrl Pts',(-9.28702861156906,39.0224235141799,28.0379941619264));
#52812=CARTESIAN_POINT('Ctrl Pts',(-9.25602612783251,39.0166812018795,28.0364493438328));
#52813=CARTESIAN_POINT('Ctrl Pts',(-9.13915033330484,38.9950333455904,28.0306255574671));
#52814=CARTESIAN_POINT('Ctrl Pts',(-9.02303170445215,38.9682451382139,28.0248017711013));
#52815=CARTESIAN_POINT('Ctrl Pts',(-8.90815669635618,38.9363819936952,28.0189779847356));
#52816=CARTESIAN_POINT('Ctrl Pts',(-8.79342204162478,38.9045577793113,28.0131613138254));
#52817=CARTESIAN_POINT('Ctrl Pts',(-8.67992837610771,38.8676710665984,28.0073446429152));
#52818=CARTESIAN_POINT('Ctrl Pts',(-8.56815354267933,38.8258385646363,28.001527972005));
#52819=CARTESIAN_POINT('Ctrl Pts',(-8.45650821867766,38.7840545324699,27.9957180406594));
#52820=CARTESIAN_POINT('Ctrl Pts',(-8.34657814234692,38.7373362614064,27.9899081093138));
#52821=CARTESIAN_POINT('Ctrl Pts',(-8.23882666589127,38.6858504428726,27.9840981779682));
#52822=CARTESIAN_POINT('Ctrl Pts',(-8.13114729438493,38.6343990775311,27.9782921345026));
#52823=CARTESIAN_POINT('Ctrl Pts',(-8.02564399048193,38.5781866849026,27.972486091037));
#52824=CARTESIAN_POINT('Ctrl Pts',(-7.92276051150401,38.5174281950642,27.9666800475714));
#52825=CARTESIAN_POINT('Ctrl Pts',(-7.81992215509368,38.4566963526439,27.9608765505164));
#52826=CARTESIAN_POINT('Ctrl Pts',(-7.71970168852476,38.3914225871742,27.9550730534615));
#52827=CARTESIAN_POINT('Ctrl Pts',(-7.62251803980665,38.3218676266455,27.9492695564065));
#52828=CARTESIAN_POINT('Ctrl Pts',(-7.58550695103065,38.2953785530935,27.9470593724142));
#52829=CARTESIAN_POINT('Ctrl Pts',(-7.54893603282149,38.2682690112097,27.9448491884219));
#52830=CARTESIAN_POINT('Ctrl Pts',(-7.51282733495086,38.2405550657615,27.9426390044296));
#52831=CARTESIAN_POINT('',(-14.0849988977597,35.0030008835013,28.4896150285548));
#52832=CARTESIAN_POINT('Ctrl Pts',(-14.0849988977597,35.0030008835013,28.4896150285547));
#52833=CARTESIAN_POINT('Ctrl Pts',(-14.0848971430991,35.1415159828826,28.4828893615456));
#52834=CARTESIAN_POINT('Ctrl Pts',(-14.0777462435019,35.2797471812976,28.4761636945364));
#52835=CARTESIAN_POINT('Ctrl Pts',(-14.0636562889874,35.4170402438294,28.4694380275272));
#52836=CARTESIAN_POINT('Ctrl Pts',(-14.0494857339381,35.5551186810943,28.4626738868411));
#52837=CARTESIAN_POINT('Ctrl Pts',(-14.0282966187928,35.6922481018684,28.455909746155));
#52838=CARTESIAN_POINT('Ctrl Pts',(-14.0002502032237,35.8277821643456,28.4491456054689));
#52839=CARTESIAN_POINT('Ctrl Pts',(-13.9720233512023,35.9641881844296,28.4423379477228));
#52840=CARTESIAN_POINT('Ctrl Pts',(-13.93685076543,36.098978139626,28.4355302899768));
#52841=CARTESIAN_POINT('Ctrl Pts',(-13.8949451424515,36.2315142456721,28.4287226322307));
#52842=CARTESIAN_POINT('Ctrl Pts',(-13.8839506159381,36.2662869474801,28.4269365479713));
#52843=CARTESIAN_POINT('Ctrl Pts',(-13.8724928746765,36.3009046230714,28.4251504637118));
#52844=CARTESIAN_POINT('Ctrl Pts',(-13.86057629548,36.3353560075044,28.4233643794524));
#52845=CARTESIAN_POINT('Ctrl Pts',(-13.821720511137,36.4476898863606,28.4175405852529));
#52846=CARTESIAN_POINT('Ctrl Pts',(-13.7778950472024,36.5585074874179,28.4117167910535));
#52847=CARTESIAN_POINT('Ctrl Pts',(-13.7292372320862,36.6673375983352,28.405892996854));
#52848=CARTESIAN_POINT('Ctrl Pts',(-13.6806407930243,36.776030432994,28.4000765486791));
#52849=CARTESIAN_POINT('Ctrl Pts',(-13.6272242916691,36.8827403943895,28.3942601005043));
#52850=CARTESIAN_POINT('Ctrl Pts',(-13.5691744603437,36.9870124991127,28.3884436523295));
#52851=CARTESIAN_POINT('Ctrl Pts',(-13.5111827247524,37.0911802492783,28.3826330252022));
#52852=CARTESIAN_POINT('Ctrl Pts',(-13.4485670813968,37.1929146417315,28.3768223980748));
#52853=CARTESIAN_POINT('Ctrl Pts',(-13.3815616213169,37.2917822761415,28.3710117709475));
#52854=CARTESIAN_POINT('Ctrl Pts',(-13.3120231664601,37.3943873850987,28.3649814857782));
#52855=CARTESIAN_POINT('Ctrl Pts',(-13.2377566335247,37.4939043067719,28.3589512006089));
#52856=CARTESIAN_POINT('Ctrl Pts',(-13.1590752998962,37.589878037589,28.3529209154396));
#52857=CARTESIAN_POINT('Ctrl Pts',(-13.0833453131256,37.6822517815245,28.347116827036));
#52858=CARTESIAN_POINT('Ctrl Pts',(-13.0035260420673,37.7713430141043,28.3413127386323));
#52859=CARTESIAN_POINT('Ctrl Pts',(-12.9199394797829,37.8567776312491,28.3355086502287));
#52860=CARTESIAN_POINT('Ctrl Pts',(-12.8363652619942,37.9421996309679,28.3297054190029));
#52861=CARTESIAN_POINT('Ctrl Pts',(-12.7490251448956,38.023965797424,28.323902187777));
#52862=CARTESIAN_POINT('Ctrl Pts',(-12.6582788901612,38.1017379551025,28.3180989565512));
#52863=CARTESIAN_POINT('Ctrl Pts',(-12.5675246254377,38.1795169775727,28.3122952130858));
#52864=CARTESIAN_POINT('Ctrl Pts',(-12.4733639353473,38.2533010246102,28.3064914696205));
#52865=CARTESIAN_POINT('Ctrl Pts',(-12.3761901484246,38.3227918048728,28.3006877261551));
#52866=CARTESIAN_POINT('Ctrl Pts',(-12.2789848558491,38.3923051154131,28.294882101002));
#52867=CARTESIAN_POINT('Ctrl Pts',(-12.178764855543,38.4575221534938,28.2890764758488));
#52868=CARTESIAN_POINT('Ctrl Pts',(-12.075952419332,38.5181879643745,28.2832708506957));
#52869=CARTESIAN_POINT('Ctrl Pts',(-11.9730261588869,38.5789209387202,28.2774587981019));
#52870=CARTESIAN_POINT('Ctrl Pts',(-11.8675020854263,38.6350924205865,28.2716467455081));
#52871=CARTESIAN_POINT('Ctrl Pts',(-11.7598271671377,38.6864933665754,28.2658346929142));
#52872=CARTESIAN_POINT('Ctrl Pts',(-11.6520815419422,38.7379280660322,28.2600188237188));
#52873=CARTESIAN_POINT('Ctrl Pts',(-11.5421826340632,38.7845858316132,28.2542029545235));
#52874=CARTESIAN_POINT('Ctrl Pts',(-11.4305959321059,38.8263063493455,28.2483870853281));
#52875=CARTESIAN_POINT('Ctrl Pts',(-11.3188494477517,38.86808660721,28.2425628883167));
#52876=CARTESIAN_POINT('Ctrl Pts',(-11.2054107325405,38.9049153808315,28.2367386913053));
#52877=CARTESIAN_POINT('Ctrl Pts',(-11.0907590392455,38.9366825777937,28.230914494294));
#52878=CARTESIAN_POINT('Ctrl Pts',(-11.060380731773,38.9450996682798,28.2293713051573));
#52879=CARTESIAN_POINT('Ctrl Pts',(-11.0299173130036,38.9531616924201,28.2278281160206));
#52880=CARTESIAN_POINT('Ctrl Pts',(-10.9993777804663,38.960867209578,28.226284926884));
#52881=CARTESIAN_POINT('Ctrl Pts',(-10.884120738893,38.9899480447325,28.2204608883444));
#52882=CARTESIAN_POINT('Ctrl Pts',(-10.7674075153923,39.0140407957942,28.2146368498048));
#52883=CARTESIAN_POINT('Ctrl Pts',(-10.6497075664999,39.0330019933088,28.2088128112652));
#52884=CARTESIAN_POINT('Ctrl Pts',(-10.5321577796459,39.0519390000562,28.2029962030559));
#52885=CARTESIAN_POINT('Ctrl Pts',(-10.4136241710923,39.0657574111683,28.1971795948466));
#52886=CARTESIAN_POINT('Ctrl Pts',(-10.2945896878623,39.074363989116,28.1913629866373));
#52887=CARTESIAN_POINT('Ctrl Pts',(-10.171460887861,39.0832665994022,28.1853463100453));
#52888=CARTESIAN_POINT('Ctrl Pts',(-10.0477965568257,39.086592258203,28.1793296334533));
#52889=CARTESIAN_POINT('Ctrl Pts',(-9.92414171060296,39.0842955965417,28.1733129568613));
#52890=CARTESIAN_POINT('Ctrl Pts',(-9.80481591212125,39.0820793389913,28.1675069188412));
#52891=CARTESIAN_POINT('Ctrl Pts',(-9.68549939383176,39.0746278174157,28.1617008808211));
#52892=CARTESIAN_POINT('Ctrl Pts',(-9.56668511033785,39.0619531270556,28.1558948428009));
#52893=CARTESIAN_POINT('Ctrl Pts',(-9.44791893666366,39.0492835688821,28.1500911557392));
#52894=CARTESIAN_POINT('Ctrl Pts',(-9.32965499864144,39.0313950916617,28.1442874686775));
#52895=CARTESIAN_POINT('Ctrl Pts',(-9.21238261929791,39.0083517637074,28.1384837816158));
#52896=CARTESIAN_POINT('Ctrl Pts',(-9.09513005178673,38.9853123286608,28.1326810750209));
#52897=CARTESIAN_POINT('Ctrl Pts',(-8.97886910998498,38.9571198547666,28.126878368426));
#52898=CARTESIAN_POINT('Ctrl Pts',(-8.86407975983748,38.9238896783662,28.1210756618311));
#52899=CARTESIAN_POINT('Ctrl Pts',(-8.74928271508907,38.8906572744688,28.1152725662671));
#52900=CARTESIAN_POINT('Ctrl Pts',(-8.63595784977484,38.8523866115704,28.1094694707031));
#52901=CARTESIAN_POINT('Ctrl Pts',(-8.52457016431055,38.8092429431525,28.1036663751391));
#52902=CARTESIAN_POINT('Ctrl Pts',(-8.41310151663988,38.7660679157333,28.0978590615916));
#52903=CARTESIAN_POINT('Ctrl Pts',(-8.30357324099135,38.7180129588992,28.092051748044));
#52904=CARTESIAN_POINT('Ctrl Pts',(-8.19643051481694,38.6652915453094,28.0862444344965));
#52905=CARTESIAN_POINT('Ctrl Pts',(-8.08924103627097,38.6125471264144,28.0804345868929));
#52906=CARTESIAN_POINT('Ctrl Pts',(-7.9844395396861,38.5551323885469,28.0746247392892));
#52907=CARTESIAN_POINT('Ctrl Pts',(-7.88244548988597,38.4933061555918,28.0688148916856));
#52908=CARTESIAN_POINT('Ctrl Pts',(-7.78033800943058,38.4314111638206,28.0629985827754));
#52909=CARTESIAN_POINT('Ctrl Pts',(-7.68104454798937,38.3650951086807,28.0571822738652));
#52910=CARTESIAN_POINT('Ctrl Pts',(-7.5849545492095,38.2946593861302,28.0513659649551));
#52911=CARTESIAN_POINT('Ctrl Pts',(-7.5607063489003,38.2768850128238,28.0498982261133));
#52912=CARTESIAN_POINT('Ctrl Pts',(-7.53666197551205,38.2588484955234,28.0484304872715));
#52913=CARTESIAN_POINT('Ctrl Pts',(-7.51282733495086,38.2405550657615,28.0469627484298));
#52914=CARTESIAN_POINT('Ctrl Pts',(-7.51282733495086,38.2405550657615,29.2969304734038));
#52915=CARTESIAN_POINT('Ctrl Pts',(-7.41787327012908,38.1676764540214,29.291116388497));
#52916=CARTESIAN_POINT('Ctrl Pts',(-7.32614665447589,38.0906374940038,29.2853023035901));
#52917=CARTESIAN_POINT('Ctrl Pts',(-7.23801898436614,38.0097650853976,29.2794882186833));
#52918=CARTESIAN_POINT('Ctrl Pts',(-7.14979912665956,37.9288080786964,29.2736680518442));
#52919=CARTESIAN_POINT('Ctrl Pts',(-7.06518603454948,37.8440098891537,29.2678478850052));
#52920=CARTESIAN_POINT('Ctrl Pts',(-6.98451504536394,37.7557350178062,29.2620277181661));
#52921=CARTESIAN_POINT('Ctrl Pts',(-6.90380113162585,37.6674131759258,29.256204454451));
#52922=CARTESIAN_POINT('Ctrl Pts',(-6.82703376120211,37.5756112782869,29.2503811907358));
#52923=CARTESIAN_POINT('Ctrl Pts',(-6.75450747661353,37.4807263615003,29.2445579270207));
#52924=CARTESIAN_POINT('Ctrl Pts',(-6.68186468771735,37.38568902409,29.2387253089685));
#52925=CARTESIAN_POINT('Ctrl Pts',(-6.61347683034987,37.287559105778,29.2328926909164));
#52926=CARTESIAN_POINT('Ctrl Pts',(-6.54959499587365,37.1867625173987,29.2270600728643));
#52927=CARTESIAN_POINT('Ctrl Pts',(-6.49345283258686,37.0981780462428,29.2219341118182));
#52928=CARTESIAN_POINT('Ctrl Pts',(-6.44079037335608,37.0075344876291,29.2168081507722));
#52929=CARTESIAN_POINT('Ctrl Pts',(-6.39174780557274,36.9151347475859,29.2116821897262));
#52930=CARTESIAN_POINT('Ctrl Pts',(-6.33608961750155,36.8102707010749,29.2058647597498));
#52931=CARTESIAN_POINT('Ctrl Pts',(-6.28491498682052,36.7028056730188,29.2000473297733));
#52932=CARTESIAN_POINT('Ctrl Pts',(-6.23847551375534,36.5931599227265,29.1942298997969));
#52933=CARTESIAN_POINT('Ctrl Pts',(-6.19209531410575,36.4836541197182,29.1884198949466));
#52934=CARTESIAN_POINT('Ctrl Pts',(-6.15043841006421,36.3719735037468,29.1826098900963));
#52935=CARTESIAN_POINT('Ctrl Pts',(-6.11371091804858,36.2585635349498,29.176799885246));
#52936=CARTESIAN_POINT('Ctrl Pts',(-6.07702067142689,36.1452685753388,29.1709957723286));
#52937=CARTESIAN_POINT('Ctrl Pts',(-6.04525001802544,36.0302481386786,29.1651916594112));
#52938=CARTESIAN_POINT('Ctrl Pts',(-6.01855704784319,35.9139677339605,29.1593875464938));
#52939=CARTESIAN_POINT('Ctrl Pts',(-5.99081280959456,35.7931077760719,29.1533548461048));
#52940=CARTESIAN_POINT('Ctrl Pts',(-5.96855459914305,35.6708869823752,29.1473221457158));
#52941=CARTESIAN_POINT('Ctrl Pts',(-5.95190294454598,35.5478459907898,29.1412894453268));
#52942=CARTESIAN_POINT('Ctrl Pts',(-5.9359006682298,35.4296033300327,29.1354920071206));
#52943=CARTESIAN_POINT('Ctrl Pts',(-5.92507592136629,35.3106036875415,29.1296945689144));
#52944=CARTESIAN_POINT('Ctrl Pts',(-5.91948345438878,35.1913366692327,29.1238971307082));
#52945=CARTESIAN_POINT('Ctrl Pts',(-5.91389185178974,35.0720880849788,29.1181005885611));
#52946=CARTESIAN_POINT('Ctrl Pts',(-5.91353094007082,34.9525726158708,29.112304046414));
#52947=CARTESIAN_POINT('Ctrl Pts',(-5.91840344120809,34.8332830804685,29.1065075042668));
#52948=CARTESIAN_POINT('Ctrl Pts',(-5.92327634618274,34.7139836582398,29.100710481697));
#52949=CARTESIAN_POINT('Ctrl Pts',(-5.93338350962639,34.5949106159771,29.0949134591271));
#52950=CARTESIAN_POINT('Ctrl Pts',(-5.94867558759209,34.476554200105,29.0891164365572));
#52951=CARTESIAN_POINT('Ctrl Pts',(-5.96397256395702,34.3581598719899,29.0833175570696));
#52952=CARTESIAN_POINT('Ctrl Pts',(-5.98445770525062,34.2404830325342,29.077518677582));
#52953=CARTESIAN_POINT('Ctrl Pts',(-6.01003022317322,34.1240056050357,29.0717197980944));
#52954=CARTESIAN_POINT('Ctrl Pts',(-6.03563107169448,34.0073991376334,29.0659144942989));
#52955=CARTESIAN_POINT('Ctrl Pts',(-6.06633045893937,33.8919951345671,29.0601091905035));
#52956=CARTESIAN_POINT('Ctrl Pts',(-6.10197716192871,33.7782623219878,29.054303886708));
#52957=CARTESIAN_POINT('Ctrl Pts',(-6.1376472397103,33.664454930818,29.0484947761714));
#52958=CARTESIAN_POINT('Ctrl Pts',(-6.17827095449689,33.5523212964051,29.0426856656348));
#52959=CARTESIAN_POINT('Ctrl Pts',(-6.22364879898165,33.4423104909619,29.0368765550983));
#52960=CARTESIAN_POINT('Ctrl Pts',(-6.26909198485532,33.3321412765219,29.0310590797891));
#52961=CARTESIAN_POINT('Ctrl Pts',(-6.31930279186957,33.2241013619347,29.0252416044799));
#52962=CARTESIAN_POINT('Ctrl Pts',(-6.37403557954917,33.1186156635008,29.0194241291707));
#52963=CARTESIAN_POINT('Ctrl Pts',(-6.38915601188665,33.0894742761649,29.0178169984997));
#52964=CARTESIAN_POINT('Ctrl Pts',(-6.40462130285063,33.0605276540963,29.0162098678287));
#52965=CARTESIAN_POINT('Ctrl Pts',(-6.42042570108141,33.0317843516216,29.0146027371578));
#52966=CARTESIAN_POINT('Ctrl Pts',(-6.47770523441605,32.927610631863,29.0087780487706));
#52967=CARTESIAN_POINT('Ctrl Pts',(-6.53962822579674,32.8257718442912,29.0029533603834));
#52968=CARTESIAN_POINT('Ctrl Pts',(-6.60597959959592,32.7267093187098,28.9971286719963));
#52969=CARTESIAN_POINT('Ctrl Pts',(-6.67224730713684,32.6277717067568,28.9913113282932));
#52970=CARTESIAN_POINT('Ctrl Pts',(-6.74293206540356,32.5316037299637,28.9854939845902));
#52971=CARTESIAN_POINT('Ctrl Pts',(-6.81777285021209,32.43862236928,28.9796766408872));
#52972=CARTESIAN_POINT('Ctrl Pts',(-6.89253874937611,32.3457340456902,28.9738651180148));
#52973=CARTESIAN_POINT('Ctrl Pts',(-6.9714521476959,32.25602631111,28.9680535951424));
#52974=CARTESIAN_POINT('Ctrl Pts',(-7.05420899246627,32.1698868679974,28.96224207227));
#52975=CARTESIAN_POINT('Ctrl Pts',(-7.14007626075387,32.0805098661021,28.9562121227833));
#52976=CARTESIAN_POINT('Ctrl Pts',(-7.2300813083146,31.9949750204064,28.9501821732966));
#52977=CARTESIAN_POINT('Ctrl Pts',(-7.32383862184878,31.9136777099448,28.9441522238099));
#52978=CARTESIAN_POINT('Ctrl Pts',(-7.41409795379706,31.8354135121466,28.9383472450639));
#52979=CARTESIAN_POINT('Ctrl Pts',(-7.50783424477259,31.7610766086199,28.9325422663178));
#52980=CARTESIAN_POINT('Ctrl Pts',(-7.60466683284577,31.6909814116069,28.9267372875718));
#52981=CARTESIAN_POINT('Ctrl Pts',(-7.70148506252334,31.6208966083528,28.9209331695916));
#52982=CARTESIAN_POINT('Ctrl Pts',(-7.80139834570489,31.5550525000547,28.9151290516114));
#52983=CARTESIAN_POINT('Ctrl Pts',(-7.9039948635413,31.4937217070035,28.9093249336312));
#52984=CARTESIAN_POINT('Ctrl Pts',(-8.00660035487121,31.4323855497207,28.903520308));
#52985=CARTESIAN_POINT('Ctrl Pts',(-8.11188919711753,31.3755637019829,28.8977156823689));
#52986=CARTESIAN_POINT('Ctrl Pts',(-8.21942322233681,31.3234838040821,28.8919110567378));
#52987=CARTESIAN_POINT('Ctrl Pts',(-8.3269920032866,31.271387073603,28.8861045550121));
#52988=CARTESIAN_POINT('Ctrl Pts',(-8.43680704323431,31.2240355188569,28.8802980532863));
#52989=CARTESIAN_POINT('Ctrl Pts',(-8.54840896352329,31.1816091788791,28.8744915515606));
#52990=CARTESIAN_POINT('Ctrl Pts',(-8.66013417455606,31.1391359689639,28.868678635179));
#52991=CARTESIAN_POINT('Ctrl Pts',(-8.7736498245319,31.1015989798057,28.8628657187974));
#52992=CARTESIAN_POINT('Ctrl Pts',(-8.88847994430274,31.0691288286459,28.8570528024157));
#52993=CARTESIAN_POINT('Ctrl Pts',(-9.00338533099471,31.036637394496,28.8512360758812));
#52994=CARTESIAN_POINT('Ctrl Pts',(-9.11960650702794,31.0092195060462,28.8454193493466));
#52995=CARTESIAN_POINT('Ctrl Pts',(-9.23665747217893,30.986954624575,28.839602622812));
#52996=CARTESIAN_POINT('Ctrl Pts',(-9.35387569657673,30.9646579278403,28.8337775845024));
#52997=CARTESIAN_POINT('Ctrl Pts',(-9.47192567423361,30.9475289934098,28.8279525461927));
#52998=CARTESIAN_POINT('Ctrl Pts',(-9.59031631377747,30.9355954584659,28.822127507883));
#52999=CARTESIAN_POINT('Ctrl Pts',(-9.62150906658929,30.932451292617,28.8205927667851));
#53000=CARTESIAN_POINT('Ctrl Pts',(-9.65272546992431,30.9296675006439,28.8190580256872));
#53001=CARTESIAN_POINT('Ctrl Pts',(-9.68395656233487,30.927243986499,28.8175232845893));
#53002=CARTESIAN_POINT('Ctrl Pts',(-9.80248275775051,30.9180464244235,28.8116987357426));
#53003=CARTESIAN_POINT('Ctrl Pts',(-9.92160116571264,30.9140124436722,28.8058741868959));
#53004=CARTESIAN_POINT('Ctrl Pts',(-10.0408247702119,30.9152040028739,28.8000496380493));
#53005=CARTESIAN_POINT('Ctrl Pts',(-10.1598983591033,30.9163940627712,28.7942324180637));
#53006=CARTESIAN_POINT('Ctrl Pts',(-10.2790764766751,30.9227965806436,28.7884151980781));
#53007=CARTESIAN_POINT('Ctrl Pts',(-10.3978672944792,30.9344217365812,28.7825979780924));
#53008=CARTESIAN_POINT('Ctrl Pts',(-10.5165395726682,30.9460352919461,28.7767865630254));
#53009=CARTESIAN_POINT('Ctrl Pts',(-10.6348249160352,30.9628610779299,28.7709751479583));
#53010=CARTESIAN_POINT('Ctrl Pts',(-10.7522324076423,30.9848572372962,28.7651637328912));
#53011=CARTESIAN_POINT('Ctrl Pts',(-10.874055867381,31.0076807232449,28.7591337370216));
#53012=CARTESIAN_POINT('Ctrl Pts',(-10.9949336946401,31.0360711550509,28.753103741152));
#53013=CARTESIAN_POINT('Ctrl Pts',(-11.1143238744396,31.0699227357654,28.7470737452824));
#53014=CARTESIAN_POINT('Ctrl Pts',(-11.2292575272157,31.1025107244114,28.741268833583));
#53015=CARTESIAN_POINT('Ctrl Pts',(-11.3428121747645,31.1401593453216,28.7354639218835));
#53016=CARTESIAN_POINT('Ctrl Pts',(-11.4545162236956,31.1827224943677,28.7296590101841));
#53017=CARTESIAN_POINT('Ctrl Pts',(-11.5662040024583,31.2252794439107,28.7238549439946));
#53018=CARTESIAN_POINT('Ctrl Pts',(-11.6760413373258,31.2727493527382,28.7180508778052));
#53019=CARTESIAN_POINT('Ctrl Pts',(-11.7835745203653,31.324937152877,28.7122468116158));
#53020=CARTESIAN_POINT('Ctrl Pts',(-11.8911173938996,31.3771296559883,28.7064422223852));
#53021=CARTESIAN_POINT('Ctrl Pts',(-11.9963553355207,31.4340407175232,28.7006376331547));
#53022=CARTESIAN_POINT('Ctrl Pts',(-12.0988578243006,31.4954285806432,28.6948330439242));
#53023=CARTESIAN_POINT('Ctrl Pts',(-12.2013937171359,31.5568364491661,28.6890265630633));
#53024=CARTESIAN_POINT('Ctrl Pts',(-12.3011920342285,31.6227238111686,28.6832200822024));
#53025=CARTESIAN_POINT('Ctrl Pts',(-12.3978504501752,31.6928050830659,28.6774136013415));
#53026=CARTESIAN_POINT('Ctrl Pts',(-12.4946160366207,31.7629640579216,28.6716006825161));
#53027=CARTESIAN_POINT('Ctrl Pts',(-12.588234442121,31.8373259847854,28.6657877636907));
#53028=CARTESIAN_POINT('Ctrl Pts',(-12.6783355901023,31.9155643195567,28.6599748448653));
#53029=CARTESIAN_POINT('Ctrl Pts',(-12.76849600687,31.993854119723,28.6541581022857));
#53030=CARTESIAN_POINT('Ctrl Pts',(-12.855134262889,32.076025125808,28.6483413597061));
#53031=CARTESIAN_POINT('Ctrl Pts',(-12.9379175774703,32.1617143716689,28.6425246171265));
#53032=CARTESIAN_POINT('Ctrl Pts',(-13.020819468138,32.2475263559762,28.6366995428368));
#53033=CARTESIAN_POINT('Ctrl Pts',(-13.0998551268564,32.3368663338371,28.6308744685472));
#53034=CARTESIAN_POINT('Ctrl Pts',(-13.1747323336447,32.4293386824183,28.6250493942576));
#53035=CARTESIAN_POINT('Ctrl Pts',(-13.1944660811659,32.4537095965838,28.6235142068454));
#53036=CARTESIAN_POINT('Ctrl Pts',(-13.2139112289294,32.4782979258235,28.6219790194332));
#53037=CARTESIAN_POINT('Ctrl Pts',(-13.2330629426428,32.5030961154041,28.6204438320209));
#53038=CARTESIAN_POINT('Ctrl Pts',(-13.30569343614,32.5971401667112,28.6146218246001));
#53039=CARTESIAN_POINT('Ctrl Pts',(-13.3743387912988,32.6945133666739,28.6087998171793));
#53040=CARTESIAN_POINT('Ctrl Pts',(-13.4386788632778,32.7948440700834,28.6029778097585));
#53041=CARTESIAN_POINT('Ctrl Pts',(-13.5029393080696,32.8950506043481,28.5971630076463));
#53042=CARTESIAN_POINT('Ctrl Pts',(-13.5629048454414,32.9982070248374,28.5913482055341));
#53043=CARTESIAN_POINT('Ctrl Pts',(-13.6182957135303,33.1039089870346,28.5855334034219));
#53044=CARTESIAN_POINT('Ctrl Pts',(-13.6736310844335,33.2095050443844,28.5797244272729));
#53045=CARTESIAN_POINT('Ctrl Pts',(-13.7244007130429,33.3176412124539,28.5739154511238));
#53046=CARTESIAN_POINT('Ctrl Pts',(-13.7703686407808,33.4278850828846,28.5681064749747));
#53047=CARTESIAN_POINT('Ctrl Pts',(-13.8163013438007,33.5380444746485,28.5623019501802));
#53048=CARTESIAN_POINT('Ctrl Pts',(-13.8574395091137,33.6503079807764,28.5564974253857));
#53049=CARTESIAN_POINT('Ctrl Pts',(-13.8935938540381,33.7642201248616,28.5506929005912));
#53050=CARTESIAN_POINT('Ctrl Pts',(-13.9297310874388,33.8780783553618,28.5448911230257));
#53051=CARTESIAN_POINT('Ctrl Pts',(-13.9608890686761,33.9935832837857,28.5390893454601));
#53052=CARTESIAN_POINT('Ctrl Pts',(-13.9869274552809,34.1102615742101,28.5332875678946));
#53053=CARTESIAN_POINT('Ctrl Pts',(-14.012958527511,34.2269070888423,28.5274874200912));
#53054=CARTESIAN_POINT('Ctrl Pts',(-14.0338727805242,34.3447249111311,28.5216872722878));
#53055=CARTESIAN_POINT('Ctrl Pts',(-14.0495805146343,34.463229420055,28.5158871244843));
#53056=CARTESIAN_POINT('Ctrl Pts',(-14.0652908308943,34.5817534095995,28.510086023211));
#53057=CARTESIAN_POINT('Ctrl Pts',(-14.0757928630313,34.700963906997,28.5042849219377));
#53058=CARTESIAN_POINT('Ctrl Pts',(-14.081048575542,34.8203683656302,28.4984838206644));
#53059=CARTESIAN_POINT('Ctrl Pts',(-14.0837269073067,34.881217347334,28.4955275566415));
#53060=CARTESIAN_POINT('Ctrl Pts',(-14.0850436239649,34.9421166306784,28.4925712926185));
#53061=CARTESIAN_POINT('Ctrl Pts',(-14.0849988977603,35.0030008826619,28.4896150285955));
#53062=CARTESIAN_POINT('Origin',(130.,35.,23.));
#53063=CARTESIAN_POINT('',(126.610250000496,35.0000579986539,27.6441866060966));
#53064=CARTESIAN_POINT('Ctrl Pts',(126.821241918358,36.1772434416436,28.8235740826546));
#53065=CARTESIAN_POINT('Ctrl Pts',(126.833574096516,36.2105424260322,28.821437007519));
#53066=CARTESIAN_POINT('Ctrl Pts',(126.846428242073,36.2436442112275,28.819272610919));
#53067=CARTESIAN_POINT('Ctrl Pts',(126.914370492875,36.4107779264545,28.808161660815));
#53068=CARTESIAN_POINT('Ctrl Pts',(126.977489366515,36.54137167997,28.7988833094481));
#53069=CARTESIAN_POINT('Ctrl Pts',(127.181891381596,36.9031307712913,28.7721256404083));
#53070=CARTESIAN_POINT('Ctrl Pts',(127.342781788506,37.1219994400736,28.7546975621398));
#53071=CARTESIAN_POINT('Ctrl Pts',(127.561297458281,37.354888726488,28.7353266802008));
#53072=CARTESIAN_POINT('Ctrl Pts',(127.595340568098,37.3896410578469,28.7324073475024));
#53073=CARTESIAN_POINT('Ctrl Pts',(127.651025034136,37.4440901040894,28.7277844298354));
#53074=CARTESIAN_POINT('Ctrl Pts',(127.672192882417,37.4642593066907,28.7260606699848));
#53075=CARTESIAN_POINT('Ctrl Pts',(127.713169923754,37.5023039290061,28.7227862196759));
#53076=CARTESIAN_POINT('Ctrl Pts',(127.732934307613,37.5202241878357,28.721233706764));
#53077=CARTESIAN_POINT('Ctrl Pts',(127.779220503777,37.561206463623,28.7176581506043));
#53078=CARTESIAN_POINT('Ctrl Pts',(127.805893764433,37.584093279777,28.7156423451266));
#53079=CARTESIAN_POINT('Ctrl Pts',(127.894978973599,37.6581582332843,28.7090497772128));
#53080=CARTESIAN_POINT('Ctrl Pts',(127.958864831683,37.7075242034752,28.7045437604119));
#53081=CARTESIAN_POINT('Ctrl Pts',(128.12188887874,37.8244432791715,28.6935122432114));
#53082=CARTESIAN_POINT('Ctrl Pts',(128.222964918218,37.889105410943,28.6870785000955));
#53083=CARTESIAN_POINT('Ctrl Pts',(128.540674672581,38.06936184029,28.6676419050387));
#53084=CARTESIAN_POINT('Ctrl Pts',(128.766579897165,38.1669005061827,28.6549012043865));
#53085=CARTESIAN_POINT('Ctrl Pts',(129.034181054551,38.2494314344403,28.6390804729221));
#53086=CARTESIAN_POINT('Ctrl Pts',(129.067517663182,38.2591543963013,28.6370964543856));
#53087=CARTESIAN_POINT('Ctrl Pts',(129.118425341683,38.2731571817028,28.6340386777282));
#53088=CARTESIAN_POINT('Ctrl Pts',(129.135891951924,38.277811627241,28.6329845693424));
#53089=CARTESIAN_POINT('Ctrl Pts',(129.167868336798,38.2860592486628,28.6310443448697));
#53090=CARTESIAN_POINT('Ctrl Pts',(129.182365836565,38.2896964661152,28.6301606694589));
#53091=CARTESIAN_POINT('Ctrl Pts',(129.216088875176,38.2979204135607,28.6280959715622));
#53092=CARTESIAN_POINT('Ctrl Pts',(129.235330919935,38.3024349898655,28.6269111191426));
#53093=CARTESIAN_POINT('Ctrl Pts',(129.298619744966,38.3167010710799,28.6229943712998));
#53094=CARTESIAN_POINT('Ctrl Pts',(129.342820124311,38.3257411883443,28.6202278372197));
#53095=CARTESIAN_POINT('Ctrl Pts',(129.452582019679,38.3459168903911,28.6133024222603));
#53096=CARTESIAN_POINT('Ctrl Pts',(129.518315040751,38.3560102788485,28.6091067580621));
#53097=CARTESIAN_POINT('Ctrl Pts',(129.856441550266,38.3977917206956,28.5874072431919));
#53098=CARTESIAN_POINT('Ctrl Pts',(130.131704953603,38.3982765411878,28.5694624413171));
#53099=CARTESIAN_POINT('Ctrl Pts',(130.489228049749,38.3553577860524,28.5470864165132));
#53100=CARTESIAN_POINT('Ctrl Pts',(130.57402109284,38.3418964197762,28.541839332944));
#53101=CARTESIAN_POINT('Ctrl Pts',(130.690782750783,38.3187838572289,28.5346981223825));
#53102=CARTESIAN_POINT('Ctrl Pts',(130.723252208328,38.3118595170262,28.532721252984));
#53103=CARTESIAN_POINT('Ctrl Pts',(130.779656462399,38.2989618134617,28.5293018560984));
#53104=CARTESIAN_POINT('Ctrl Pts',(130.803637074221,38.2932022025586,28.5278527470299));
#53105=CARTESIAN_POINT('Ctrl Pts',(130.854017546788,38.2805188375112,28.5248174606695));
#53106=CARTESIAN_POINT('Ctrl Pts',(130.88040103618,38.2735369087089,28.5232332466146));
#53107=CARTESIAN_POINT('Ctrl Pts',(130.944230241851,38.2558181063316,28.5194120346597));
#53108=CARTESIAN_POINT('Ctrl Pts',(130.981581228048,38.2447528042198,28.5171856439566));
#53109=CARTESIAN_POINT('Ctrl Pts',(131.122653691527,38.20030080222,28.5088047971692));
#53110=CARTESIAN_POINT('Ctrl Pts',(131.224939304439,38.1625627722472,28.5027890182928));
#53111=CARTESIAN_POINT('Ctrl Pts',(131.510649137383,38.0412044530307,28.4859461301745));
#53112=CARTESIAN_POINT('Ctrl Pts',(131.688668891005,37.9460792807847,28.4754226666234));
#53113=CARTESIAN_POINT('Ctrl Pts',(131.972756390827,37.7600220255037,28.4572814280134));
#53114=CARTESIAN_POINT('Ctrl Pts',(132.083576931231,37.677347357494,28.4497979678272));
#53115=CARTESIAN_POINT('Ctrl Pts',(132.210561844483,37.5699448278629,28.4403258518178));
#53116=CARTESIAN_POINT('Ctrl Pts',(132.231861511741,37.551469021785,28.438704312997));
#53117=CARTESIAN_POINT('Ctrl Pts',(132.265256998767,37.5217628939599,28.436104913713));
#53118=CARTESIAN_POINT('Ctrl Pts',(132.277505987065,37.5107058405614,28.4351390354572));
#53119=CARTESIAN_POINT('Ctrl Pts',(132.301013279964,37.4891724410913,28.4332600638386));
#53120=CARTESIAN_POINT('Ctrl Pts',(132.312281799851,37.4787082119455,28.4323478046554));
#53121=CARTESIAN_POINT('Ctrl Pts',(132.340106719763,37.4525144521483,28.4300671027297));
#53122=CARTESIAN_POINT('Ctrl Pts',(132.356575955877,37.4366937230096,28.4286921179166));
#53123=CARTESIAN_POINT('Ctrl Pts',(132.420583871252,37.3739503793387,28.4232534288863));
#53124=CARTESIAN_POINT('Ctrl Pts',(132.466888591852,37.3257958111954,28.4191104930551));
#53125=CARTESIAN_POINT('Ctrl Pts',(132.592813814293,37.1868466740585,28.4073173935482));
#53126=CARTESIAN_POINT('Ctrl Pts',(132.669049190715,37.0931210438606,28.3995479409319));
#53127=CARTESIAN_POINT('Ctrl Pts',(132.884966326899,36.7966396200247,28.375907466975));
#53128=CARTESIAN_POINT('Ctrl Pts',(133.007750641083,36.5825347719095,28.3601290816689));
#53129=CARTESIAN_POINT('Ctrl Pts',(133.126738615134,36.3101613862715,28.3420566371341));
#53130=CARTESIAN_POINT('Ctrl Pts',(133.146137795041,36.2628676199947,28.3389830676894));
#53131=CARTESIAN_POINT('Ctrl Pts',(133.175222075742,36.1871271972444,28.3341601121192));
#53132=CARTESIAN_POINT('Ctrl Pts',(133.185610797525,36.1589608044419,28.3323879069868));
#53133=CARTESIAN_POINT('Ctrl Pts',(133.204464349062,36.1056743196671,28.3290741357947));
#53134=CARTESIAN_POINT('Ctrl Pts',(133.213011305906,36.0805858931559,28.3275299912826));
#53135=CARTESIAN_POINT('Ctrl Pts',(133.231747720515,36.0233990757995,28.3240453554249));
#53136=CARTESIAN_POINT('Ctrl Pts',(133.241754947344,35.9912436506845,28.3221108586675));
#53137=CARTESIAN_POINT('Ctrl Pts',(133.271595996234,35.8900680921034,28.3160972431502));
#53138=CARTESIAN_POINT('Ctrl Pts',(133.289717518608,35.8205615243723,28.3120721663896));
#53139=CARTESIAN_POINT('Ctrl Pts',(133.327957934295,35.6521358445925,28.302527182361));
#53140=CARTESIAN_POINT('Ctrl Pts',(133.345894348628,35.5527911204698,28.2970678938955));
#53141=CARTESIAN_POINT('Ctrl Pts',(133.376399624132,35.3264639920828,28.2848461073165));
#53142=CARTESIAN_POINT('Ctrl Pts',(133.386287257647,35.1992787054487,28.2781302437978));
#53143=CARTESIAN_POINT('Ctrl Pts',(133.392139470349,34.9231995487549,28.2634428995431));
#53144=CARTESIAN_POINT('Ctrl Pts',(133.385507710175,34.7745277664282,28.2554643235251));
#53145=CARTESIAN_POINT('Ctrl Pts',(133.365194750099,34.591154525106,28.2450493284386));
#53146=CARTESIAN_POINT('Ctrl Pts',(133.360682709541,34.5555882088104,28.2430019516411));
#53147=CARTESIAN_POINT('Ctrl Pts',(133.353048295232,34.5022058639237,28.2398789605673));
#53148=CARTESIAN_POINT('Ctrl Pts',(133.350345892762,34.4843312700863,28.2388247766148));
#53149=CARTESIAN_POINT('Ctrl Pts',(133.345148708232,34.4517222480562,28.2368847150788));
#53150=CARTESIAN_POINT('Ctrl Pts',(133.342699283756,34.4369814873771,28.2360012830928));
#53151=CARTESIAN_POINT('Ctrl Pts',(133.336786226334,34.4027958245229,28.2339376878709));
#53152=CARTESIAN_POINT('Ctrl Pts',(133.333250038459,34.383364542749,28.232753703952));
#53153=CARTESIAN_POINT('Ctrl Pts',(133.321094325853,34.3197311973542,28.2288426414629));
#53154=CARTESIAN_POINT('Ctrl Pts',(133.311764046651,34.2756715868186,28.2260810522973));
#53155=CARTESIAN_POINT('Ctrl Pts',(133.286527659243,34.167209116851,28.2191709669556));
#53156=CARTESIAN_POINT('Ctrl Pts',(133.26960368074,34.1030632157658,28.214985875343));
#53157=CARTESIAN_POINT('Ctrl Pts',(133.173709768274,33.7785245138152,28.1934336083411));
#53158=CARTESIAN_POINT('Ctrl Pts',(133.065458717479,33.527780728012,28.1756283372013));
#53159=CARTESIAN_POINT('Ctrl Pts',(132.884167711508,33.2168315288207,28.153242215087));
#53160=CARTESIAN_POINT('Ctrl Pts',(132.837014767794,33.1427271435099,28.1478709441991));
#53161=CARTESIAN_POINT('Ctrl Pts',(132.765949209058,33.0400759752863,28.1403789175242));
#53162=CARTESIAN_POINT('Ctrl Pts',(132.744365967886,33.0099666315855,28.1381745482307));
#53163=CARTESIAN_POINT('Ctrl Pts',(132.706230030744,32.9585664821669,28.134398104556));
#53164=CARTESIAN_POINT('Ctrl Pts',(132.689909176583,32.9371087107543,28.1328174253524));
#53165=CARTESIAN_POINT('Ctrl Pts',(132.655825604829,32.8933898564772,28.1295872998555));
#53166=CARTESIAN_POINT('Ctrl Pts',(132.638034824803,32.8711532993092,28.1279391223822));
#53167=CARTESIAN_POINT('Ctrl Pts',(132.591431823204,32.8143860376986,28.1237159343819));
#53168=CARTESIAN_POINT('Ctrl Pts',(132.562208408018,32.7801991920771,28.121157438277));
#53169=CARTESIAN_POINT('Ctrl Pts',(132.400390699791,32.5983524299034,28.1074441504082));
#53170=CARTESIAN_POINT('Ctrl Pts',(132.255700942443,32.4619670583649,28.0968078114157));
#53171=CARTESIAN_POINT('Ctrl Pts',(131.932718725283,32.2070883032422,28.0749666129233));
#53172=CARTESIAN_POINT('Ctrl Pts',(131.753499001965,32.0912235161095,28.0638198653989));
#53173=CARTESIAN_POINT('Ctrl Pts',(131.52631227605,31.9730146144893,28.0494653606025));
#53174=CARTESIAN_POINT('Ctrl Pts',(131.487630512196,31.9538179979563,28.0470130775307));
#53175=CARTESIAN_POINT('Ctrl Pts',(131.431210476031,31.9271493101097,28.0434096494183));
#53176=CARTESIAN_POINT('Ctrl Pts',(131.413757256599,31.9190804666867,28.0422913299573));
#53177=CARTESIAN_POINT('Ctrl Pts',(131.38263105902,31.9050106046708,28.0402888855845));
#53178=CARTESIAN_POINT('Ctrl Pts',(131.36898565294,31.8989507790011,28.0394082437586));
#53179=CARTESIAN_POINT('Ctrl Pts',(131.338590327462,31.8856921557224,28.0374401100009));
#53180=CARTESIAN_POINT('Ctrl Pts',(131.321822271987,31.8785382812092,28.0363501729915));
#53181=CARTESIAN_POINT('Ctrl Pts',(131.27118979176,31.8574177124802,28.0330482507067));
#53182=CARTESIAN_POINT('Ctrl Pts',(131.237156899003,31.8438647852612,28.0308144569166));
#53183=CARTESIAN_POINT('Ctrl Pts',(131.156252302406,31.8131557088708,28.0254814149447));
#53184=CARTESIAN_POINT('Ctrl Pts',(131.109208581425,31.7964782197383,28.0223626702654));
#53185=CARTESIAN_POINT('Ctrl Pts',(130.926970608384,31.7363682596789,28.0102561281204));
#53186=CARTESIAN_POINT('Ctrl Pts',(130.7894684363,31.7004085762799,28.0010753060825));
#53187=CARTESIAN_POINT('Ctrl Pts',(130.440615309178,31.6322362729187,27.9781757098992));
#53188=CARTESIAN_POINT('Ctrl Pts',(130.227682664944,31.6111714678352,27.9645769625097));
#53189=CARTESIAN_POINT('Ctrl Pts',(129.961316669213,31.6100588467737,27.9483596134753));
#53190=CARTESIAN_POINT('Ctrl Pts',(129.908474349767,31.6110737766308,27.9451785888353));
#53191=CARTESIAN_POINT('Ctrl Pts',(129.825310921066,31.6146178291803,27.9402272715984));
#53192=CARTESIAN_POINT('Ctrl Pts',(129.794964866568,31.616320139112,27.9384320690286));
#53193=CARTESIAN_POINT('Ctrl Pts',(129.738251764589,31.620267332518,27.9350975468225));
#53194=CARTESIAN_POINT('Ctrl Pts',(129.711880360391,31.6224132617813,27.9335553110492));
#53195=CARTESIAN_POINT('Ctrl Pts',(129.652561798925,31.6279400198095,27.9301038342263));
#53196=CARTESIAN_POINT('Ctrl Pts',(129.619633381831,31.6314954118846,27.9282001156446));
#53197=CARTESIAN_POINT('Ctrl Pts',(129.518648781878,31.64389878017,27.922395438506));
#53198=CARTESIAN_POINT('Ctrl Pts',(129.450802987556,31.6543314699426,27.9185430592683));
#53199=CARTESIAN_POINT('Ctrl Pts',(129.290322762465,31.6840224234511,27.9095060937393));
#53200=CARTESIAN_POINT('Ctrl Pts',(129.1980851807,31.7051125513866,27.9043732066077));
#53201=CARTESIAN_POINT('Ctrl Pts',(128.893629976027,31.7882709988625,27.8874389572777));
#53202=CARTESIAN_POINT('Ctrl Pts',(128.686634037005,31.8672187251832,27.8759683917868));
#53203=CARTESIAN_POINT('Ctrl Pts',(128.412862467222,32.0035692048123,27.8593137643252));
#53204=CARTESIAN_POINT('Ctrl Pts',(128.338371434693,32.0442274476537,27.8546121156365));
#53205=CARTESIAN_POINT('Ctrl Pts',(128.243701809941,32.1006095764349,27.8483124653107));
#53206=CARTESIAN_POINT('Ctrl Pts',(128.222060820479,32.1138294657378,27.8468495602163));
#53207=CARTESIAN_POINT('Ctrl Pts',(128.187103791365,32.1357261091945,27.8444457109528));
#53208=CARTESIAN_POINT('Ctrl Pts',(128.173696480614,32.1442561358848,27.8435138275415));
#53209=CARTESIAN_POINT('Ctrl Pts',(128.147059234748,32.1614676372031,27.8416414792382));
#53210=CARTESIAN_POINT('Ctrl Pts',(128.13382913687,32.1701481063337,27.8407010842539));
#53211=CARTESIAN_POINT('Ctrl Pts',(128.099816354184,32.1928066546411,27.8382573679144));
#53212=CARTESIAN_POINT('Ctrl Pts',(128.079127295868,32.2069227830563,27.8367454978581));
#53213=CARTESIAN_POINT('Ctrl Pts',(127.985713698667,32.272187555466,27.8298095856459));
#53214=CARTESIAN_POINT('Ctrl Pts',(127.914867325037,32.3259526462293,27.8242439687613));
#53215=CARTESIAN_POINT('Ctrl Pts',(127.684253361076,32.515705840765,27.8052821371633));
#53216=CARTESIAN_POINT('Ctrl Pts',(127.535002937455,32.6637221961105,27.7915971812811));
#53217=CARTESIAN_POINT('Ctrl Pts',(127.306577432178,32.9366902875799,27.7689661052399));
#53218=CARTESIAN_POINT('Ctrl Pts',(127.220108955343,33.0547527909872,27.7598556584501));
#53219=CARTESIAN_POINT('Ctrl Pts',(127.118191512677,33.2146514210372,27.7484050943926));
#53220=CARTESIAN_POINT('Ctrl Pts',(127.095562389508,33.2517059357571,27.7458085595277));
#53221=CARTESIAN_POINT('Ctrl Pts',(127.059439203084,33.3134947010813,27.7415699269521));
#53222=CARTESIAN_POINT('Ctrl Pts',(127.045531039314,33.3379797969184,27.7399132440909));
#53223=CARTESIAN_POINT('Ctrl Pts',(127.018823445137,33.3863929932172,27.7366813475991));
#53224=CARTESIAN_POINT('Ctrl Pts',(127.006003069917,33.4103070519976,27.7351054849422));
#53225=CARTESIAN_POINT('Ctrl Pts',(126.97588557156,33.4681427520691,27.7313419316012));
#53226=CARTESIAN_POINT('Ctrl Pts',(126.958869956927,33.5022073137825,27.7291640518083));
#53227=CARTESIAN_POINT('Ctrl Pts',(126.898556323856,33.6282200685959,27.7212408916887));
#53228=CARTESIAN_POINT('Ctrl Pts',(126.858823561132,33.7218191899794,27.7156144660151));
#53229=CARTESIAN_POINT('Ctrl Pts',(126.76417014344,33.9760016402912,27.7008517446808));
#53230=CARTESIAN_POINT('Ctrl Pts',(126.716995332061,34.1391570156289,27.6919145493355));
#53231=CARTESIAN_POINT('Ctrl Pts',(126.648215593138,34.4675707085868,27.67410429333));
#53232=CARTESIAN_POINT('Ctrl Pts',(126.626176428229,34.6322456405921,27.6652534687727));
#53233=CARTESIAN_POINT('Ctrl Pts',(126.614173352631,34.8331639056892,27.6538934721961));
#53234=CARTESIAN_POINT('Ctrl Pts',(126.612616790041,34.8685041737009,27.6518740875299));
#53235=CARTESIAN_POINT('Ctrl Pts',(126.611111539139,34.9215561476712,27.6488023239765));
#53236=CARTESIAN_POINT('Ctrl Pts',(126.610748103906,34.9392546862154,27.6477708333819));
#53237=CARTESIAN_POINT('Ctrl Pts',(126.610410290085,34.9658549347967,27.646209363987));
#53238=CARTESIAN_POINT('Ctrl Pts',(126.610332318059,34.9747553592404,27.6456850120307));
#53239=CARTESIAN_POINT('Ctrl Pts',(126.610263040683,34.9891233453301,27.6448353861475));
#53240=CARTESIAN_POINT('Ctrl Pts',(126.61024990695,34.9945906917616,27.6445113526269));
#53241=CARTESIAN_POINT('Ctrl Pts',(126.610250000496,35.0000579986539,27.6441866060966));
#53242=CARTESIAN_POINT('Ctrl Pts',(126.610250000487,35.0000574599859,27.6441866380923));
#53243=CARTESIAN_POINT('Ctrl Pts',(126.610250090869,35.0053893568261,27.6438699346801));
#53244=CARTESIAN_POINT('Ctrl Pts',(126.610262761436,35.0107212118073,27.6435525533915));
#53245=CARTESIAN_POINT('Ctrl Pts',(126.610341021443,35.0272464228444,27.6425668195178));
#53246=CARTESIAN_POINT('Ctrl Pts',(126.610449474336,35.0384393661142,27.6418962240595));
#53247=CARTESIAN_POINT('Ctrl Pts',(126.6111108585,35.0836060713677,27.6391788960502));
#53248=CARTESIAN_POINT('Ctrl Pts',(126.612119143323,35.1175699816628,27.6371097940641));
#53249=CARTESIAN_POINT('Ctrl Pts',(126.624079589182,35.3848921680719,27.6206508155777));
#53250=CARTESIAN_POINT('Ctrl Pts',(126.658618390739,35.6165549798459,27.6053930793298));
#53251=CARTESIAN_POINT('Ctrl Pts',(126.74576514076,35.9560478668779,27.5828983791518));
#53252=CARTESIAN_POINT('Ctrl Pts',(126.780662504909,36.0676720844525,27.5754697298841));
#53253=CARTESIAN_POINT('Ctrl Pts',(126.821241849407,36.1772432554656,27.5681926079129));
#53254=CARTESIAN_POINT('',(126.610251311732,34.9970179063717,27.9839821967168));
#53255=CARTESIAN_POINT('Ctrl Pts',(126.821241918358,36.1772434416438,27.913420165303));
#53256=CARTESIAN_POINT('Ctrl Pts',(126.78558888443,36.0809741691002,27.9194241936204));
#53257=CARTESIAN_POINT('Ctrl Pts',(126.754305384126,35.983062571326,27.9254282219378));
#53258=CARTESIAN_POINT('Ctrl Pts',(126.72753284865,35.8839478524425,27.9314322502553));
#53259=CARTESIAN_POINT('Ctrl Pts',(126.700760124204,35.7848324339714,27.9374363209513));
#53260=CARTESIAN_POINT('Ctrl Pts',(126.678498535277,35.6845143046025,27.9434403916474));
#53261=CARTESIAN_POINT('Ctrl Pts',(126.660838976721,35.5834455613996,27.9494444623435));
#53262=CARTESIAN_POINT('Ctrl Pts',(126.643163513312,35.4822857919401,27.9554539405282));
#53263=CARTESIAN_POINT('Ctrl Pts',(126.630098428797,35.380374493645,27.9614634187129));
#53264=CARTESIAN_POINT('Ctrl Pts',(126.621683002323,35.2781713962731,27.9674728968976));
#53265=CARTESIAN_POINT('Ctrl Pts',(126.613976687149,35.1845802654455,27.9729759968373));
#53266=CARTESIAN_POINT('Ctrl Pts',(126.610168856573,35.0907447639098,27.978479096777));
#53267=CARTESIAN_POINT('Ctrl Pts',(126.610251311732,34.9970179063717,27.9839821967168));
#53268=CARTESIAN_POINT('Ctrl Pts',(126.821241934448,36.17724348509,29.1634527466974));
#53269=CARTESIAN_POINT('Ctrl Pts',(126.865650457316,36.2971540660655,29.1566721127873));
#53270=CARTESIAN_POINT('Ctrl Pts',(126.916815953089,36.4144761966767,29.1498639293176));
#53271=CARTESIAN_POINT('Ctrl Pts',(127.017822426018,36.6143887349965,29.1376463261198));
#53272=CARTESIAN_POINT('Ctrl Pts',(127.064767641159,36.6982469982982,29.132318279004));
#53273=CARTESIAN_POINT('Ctrl Pts',(127.134768480411,36.8116956160826,29.1247531624993));
#53274=CARTESIAN_POINT('Ctrl Pts',(127.154849794449,36.8430715716172,29.1226214602806));
#53275=CARTESIAN_POINT('Ctrl Pts',(127.190309125222,36.8965139603084,29.1189184872974));
#53276=CARTESIAN_POINT('Ctrl Pts',(127.205440417,36.9187403912989,29.1173564039352));
#53277=CARTESIAN_POINT('Ctrl Pts',(127.23697945629,36.9639036958967,29.1141356107022));
#53278=CARTESIAN_POINT('Ctrl Pts',(127.253412192638,36.9868204740305,29.1124760341176));
#53279=CARTESIAN_POINT('Ctrl Pts',(127.296261535642,37.0450297329475,29.1081940013818));
#53280=CARTESIAN_POINT('Ctrl Pts',(127.323083530223,37.0800159206566,29.1055561301045));
#53281=CARTESIAN_POINT('Ctrl Pts',(127.450381060313,37.2395192722143,29.093223471913));
#53282=CARTESIAN_POINT('Ctrl Pts',(127.558898350999,37.3573320943317,29.0832148366242));
#53283=CARTESIAN_POINT('Ctrl Pts',(127.81990481958,37.6032786160111,29.06032154642));
#53284=CARTESIAN_POINT('Ctrl Pts',(127.976187864314,37.7265466963254,29.0473620849306));
#53285=CARTESIAN_POINT('Ctrl Pts',(128.214994438526,37.8830018466142,29.029240114234));
#53286=CARTESIAN_POINT('Ctrl Pts',(128.289432491016,37.9277817013019,29.023806283354));
#53287=CARTESIAN_POINT('Ctrl Pts',(128.387226810324,37.9816072824505,29.0170125257965));
#53288=CARTESIAN_POINT('Ctrl Pts',(128.409071128837,37.9933200219717,29.0155164482157));
#53289=CARTESIAN_POINT('Ctrl Pts',(128.444967151292,38.0120631894446,29.0130952337504));
#53290=CARTESIAN_POINT('Ctrl Pts',(128.458942445982,38.0192372319407,29.0121616944514));
#53291=CARTESIAN_POINT('Ctrl Pts',(128.487168252057,38.0334795481558,29.0102952467849));
#53292=CARTESIAN_POINT('Ctrl Pts',(128.501419540881,38.04054513151,29.0093624804291));
#53293=CARTESIAN_POINT('Ctrl Pts',(128.538582721673,38.0586453338267,29.0069536391171));
#53294=CARTESIAN_POINT('Ctrl Pts',(128.561570399773,38.0695231074417,29.0054866950883));
#53295=CARTESIAN_POINT('Ctrl Pts',(128.662514647195,38.1159068561669,28.9991360347455));
#53296=CARTESIAN_POINT('Ctrl Pts',(128.741684139075,38.1487118071384,28.9943901677296));
#53297=CARTESIAN_POINT('Ctrl Pts',(129.008138199996,38.2474627509051,28.9789226807803));
#53298=CARTESIAN_POINT('Ctrl Pts',(129.199965139118,38.299962968452,28.9685732098983));
#53299=CARTESIAN_POINT('Ctrl Pts',(129.551444970943,38.3636868144409,28.9494982576423));
#53300=CARTESIAN_POINT('Ctrl Pts',(129.709378818467,38.3809943068604,28.9408905818149));
#53301=CARTESIAN_POINT('Ctrl Pts',(129.912060243996,38.3888968272813,28.9294548975422));
#53302=CARTESIAN_POINT('Ctrl Pts',(129.956213899416,38.3897548040091,28.9269411093992));
#53303=CARTESIAN_POINT('Ctrl Pts',(130.028707639274,38.3897468838245,28.9227709955705));
#53304=CARTESIAN_POINT('Ctrl Pts',(130.057043132898,38.3893884514982,28.9211303033685));
#53305=CARTESIAN_POINT('Ctrl Pts',(130.112453006022,38.3879925218593,28.9178995463875));
#53306=CARTESIAN_POINT('Ctrl Pts',(130.139526057678,38.3869855952781,28.9163105440226));
#53307=CARTESIAN_POINT('Ctrl Pts',(130.204203437771,38.3838032891687,28.9124882492052));
#53308=CARTESIAN_POINT('Ctrl Pts',(130.241788651226,38.3813254532137,28.9102458398722));
#53309=CARTESIAN_POINT('Ctrl Pts',(130.377189888425,38.3701299864737,28.902088019353));
#53310=CARTESIAN_POINT('Ctrl Pts',(130.47465010442,38.3577898616422,28.8960642659392));
#53311=CARTESIAN_POINT('Ctrl Pts',(130.734308539463,38.3133821432914,28.8796147203478));
#53312=CARTESIAN_POINT('Ctrl Pts',(130.894919538314,38.2736556264363,28.8690036366284));
#53313=CARTESIAN_POINT('Ctrl Pts',(131.217728518421,38.1682712559772,28.8471232641739));
#53314=CARTESIAN_POINT('Ctrl Pts',(131.37906738404,38.1014492754746,28.8358830053645));
#53315=CARTESIAN_POINT('Ctrl Pts',(131.566289529084,38.0063946240017,28.8229572808464));
#53316=CARTESIAN_POINT('Ctrl Pts',(131.597767082269,37.9897846227255,28.8207888902099));
#53317=CARTESIAN_POINT('Ctrl Pts',(131.644809219965,37.9640063358149,28.8175620463634));
#53318=CARTESIAN_POINT('Ctrl Pts',(131.66057077583,37.9552048422108,28.8164832550982));
#53319=CARTESIAN_POINT('Ctrl Pts',(131.689276889293,37.9388727231796,28.8145238841537));
#53320=CARTESIAN_POINT('Ctrl Pts',(131.702242517314,37.9313818782885,28.813641050877));
#53321=CARTESIAN_POINT('Ctrl Pts',(131.732300127542,37.9137495200397,28.8115990653595));
#53322=CARTESIAN_POINT('Ctrl Pts',(131.749353108451,37.9035433078895,28.810443959665));
#53323=CARTESIAN_POINT('Ctrl Pts',(131.805326947851,37.8693707981458,28.8066604578366));
#53324=CARTESIAN_POINT('Ctrl Pts',(131.843854383611,37.8447663517038,28.8040690405227));
#53325=CARTESIAN_POINT('Ctrl Pts',(131.938202052553,37.7817915546806,28.7977250920237));
#53326=CARTESIAN_POINT('Ctrl Pts',(131.993393393891,37.7425125615829,28.7940157131865));
#53327=CARTESIAN_POINT('Ctrl Pts',(132.279839238729,37.525433561398,28.774570146116));
#53328=CARTESIAN_POINT('Ctrl Pts',(132.488591531801,37.3200007649064,28.7595919516378));
#53329=CARTESIAN_POINT('Ctrl Pts',(132.713969482376,37.0322937362579,28.7394161866236));
#53330=CARTESIAN_POINT('Ctrl Pts',(132.757555444751,36.9727481030679,28.7352847121568));
#53331=CARTESIAN_POINT('Ctrl Pts',(132.818349626506,36.883737726,28.7291421063803));
#53332=CARTESIAN_POINT('Ctrl Pts',(132.837112617516,36.8553582709199,28.7271884753924));
#53333=CARTESIAN_POINT('Ctrl Pts',(132.869752327104,36.8043368710607,28.7236821375369));
#53334=CARTESIAN_POINT('Ctrl Pts',(132.88379627074,36.7818049761453,28.722135705659));
#53335=CARTESIAN_POINT('Ctrl Pts',(132.913058461344,36.7336048557974,28.7188307241416));
#53336=CARTESIAN_POINT('Ctrl Pts',(132.928205284585,36.707896109656,28.7170697782943));
#53337=CARTESIAN_POINT('Ctrl Pts',(132.968585365462,36.6372423590641,28.7122337770239));
#53338=CARTESIAN_POINT('Ctrl Pts',(132.993135267547,36.5919178522079,28.7091351631451));
#53339=CARTESIAN_POINT('Ctrl Pts',(133.091666410476,36.3996649932213,28.6960014977137));
#53340=CARTESIAN_POINT('Ctrl Pts',(133.155927427618,36.2480278867025,28.6856509776992));
#53341=CARTESIAN_POINT('Ctrl Pts',(133.288738733609,35.8578743804535,28.6592596571671));
#53342=CARTESIAN_POINT('Ctrl Pts',(133.342617059639,35.615361432157,28.6430347130332));
#53343=CARTESIAN_POINT('Ctrl Pts',(133.37333134148,35.3349934103167,28.6256826190535));
#53344=CARTESIAN_POINT('Ctrl Pts',(133.376552849037,35.3007922489946,28.6235904640387));
#53345=CARTESIAN_POINT('Ctrl Pts',(133.380669138672,35.2486063073163,28.6204413940224));
#53346=CARTESIAN_POINT('Ctrl Pts',(133.381941371965,35.2306545246443,28.6193659068443));
#53347=CARTESIAN_POINT('Ctrl Pts',(133.384008576429,35.197773809985,28.6174113110888));
#53348=CARTESIAN_POINT('Ctrl Pts',(133.384847820655,35.1828490307917,28.6165299727953));
#53349=CARTESIAN_POINT('Ctrl Pts',(133.386571858428,35.1480887839398,28.6144905617265));
#53350=CARTESIAN_POINT('Ctrl Pts',(133.387381156365,35.128250470195,28.6133365440452));
#53351=CARTESIAN_POINT('Ctrl Pts',(133.389477131792,35.0627446876347,28.6095553858785));
#53352=CARTESIAN_POINT('Ctrl Pts',(133.39001498757,35.0170565173093,28.6069652563475));
#53353=CARTESIAN_POINT('Ctrl Pts',(133.389057286393,34.9036732441961,28.6006240965911));
#53354=CARTESIAN_POINT('Ctrl Pts',(133.386457595868,34.8360060684183,28.5969162730125));
#53355=CARTESIAN_POINT('Ctrl Pts',(133.361924339353,34.4776791621796,28.5774854715992));
#53356=CARTESIAN_POINT('Ctrl Pts',(133.30459925731,34.1906867837349,28.5625212117561));
#53357=CARTESIAN_POINT('Ctrl Pts',(133.18987109863,33.8512655145781,28.5427470261242));
#53358=CARTESIAN_POINT('Ctrl Pts',(133.166612476095,33.7886234360696,28.5390117054158));
#53359=CARTESIAN_POINT('Ctrl Pts',(133.129074041698,33.696006747606,28.533336134345));
#53360=CARTESIAN_POINT('Ctrl Pts',(133.116179705843,33.6654863461253,28.5314404835134));
#53361=CARTESIAN_POINT('Ctrl Pts',(133.09292065392,33.6126089708988,28.5281092990482));
#53362=CARTESIAN_POINT('Ctrl Pts',(133.082755557594,33.5901666182129,28.5266804988298));
#53363=CARTESIAN_POINT('Ctrl Pts',(133.060818402026,33.5431059307594,28.5236516882624));
#53364=CARTESIAN_POINT('Ctrl Pts',(133.048991941846,33.5185150379379,28.5220499082525));
#53365=CARTESIAN_POINT('Ctrl Pts',(133.019547383566,33.4591369079057,28.5181343105906));
#53366=CARTESIAN_POINT('Ctrl Pts',(133.001623730231,33.4245063434621,28.51581013273));
#53367=CARTESIAN_POINT('Ctrl Pts',(132.931143928456,33.2939013083417,28.5068858758715));
#53368=CARTESIAN_POINT('Ctrl Pts',(132.874553595752,33.2001902360918,28.5001479255731));
#53369=CARTESIAN_POINT('Ctrl Pts',(132.700212762543,32.9407431501739,28.4805317591112));
#53370=CARTESIAN_POINT('Ctrl Pts',(132.571962248077,32.7826398048713,28.4673550572921));
#53371=CARTESIAN_POINT('Ctrl Pts',(132.335491832914,32.5394316512585,28.4455599674143));
#53372=CARTESIAN_POINT('Ctrl Pts',(132.234843370349,32.4476676254561,28.4369021200079));
#53373=CARTESIAN_POINT('Ctrl Pts',(132.107047144835,32.34452469855,28.4268678493928));
#53374=CARTESIAN_POINT('Ctrl Pts',(132.084931879327,32.327125906852,28.4251638857455));
#53375=CARTESIAN_POINT('Ctrl Pts',(132.049522107146,32.2999748418779,28.4224899792002));
#53376=CARTESIAN_POINT('Ctrl Pts',(132.036369167066,32.2900410773152,28.4215084137486));
#53377=CARTESIAN_POINT('Ctrl Pts',(132.010802278945,32.271022928489,28.4196236910182));
#53378=CARTESIAN_POINT('Ctrl Pts',(131.99839817806,32.2619265182791,28.4187197965125));
#53379=CARTESIAN_POINT('Ctrl Pts',(131.96740642698,32.2395218537389,28.4164863234166));
#53380=CARTESIAN_POINT('Ctrl Pts',(131.948744868507,32.2263163223643,28.4151634437478));
#53381=CARTESIAN_POINT('Ctrl Pts',(131.874886732048,32.1751652958098,28.410007598271));
#53382=CARTESIAN_POINT('Ctrl Pts',(131.818700958593,32.1386682529056,28.406258413104));
#53383=CARTESIAN_POINT('Ctrl Pts',(131.657826647824,32.0408226405472,28.3958935495562));
#53384=CARTESIAN_POINT('Ctrl Pts',(131.550871247584,31.9833923826728,28.3894243154397));
#53385=CARTESIAN_POINT('Ctrl Pts',(131.219207146427,31.8276166196265,28.3699716943244));
#53386=CARTESIAN_POINT('Ctrl Pts',(130.986726819905,31.7477943755422,28.3570805717256));
#53387=CARTESIAN_POINT('Ctrl Pts',(130.697720302912,31.68243840353,28.3404823472541));
#53388=CARTESIAN_POINT('Ctrl Pts',(130.647513972822,31.6722749756741,28.3375817021378));
#53389=CARTESIAN_POINT('Ctrl Pts',(130.567519916183,31.6579603368981,28.3329234675449));
#53390=CARTESIAN_POINT('Ctrl Pts',(130.537873072096,31.6530610343861,28.3311891878952));
#53391=CARTESIAN_POINT('Ctrl Pts',(130.484579097376,31.6449802864875,28.328055865857));
#53392=CARTESIAN_POINT('Ctrl Pts',(130.460955878357,31.6416531127989,28.3266614686194));
#53393=CARTESIAN_POINT('Ctrl Pts',(130.405248885379,31.634405987085,28.3233594725153));
#53394=CARTESIAN_POINT('Ctrl Pts',(130.373140699676,31.6306950822682,28.3214455231618));
#53395=CARTESIAN_POINT('Ctrl Pts',(130.277084163365,31.6209832038168,28.315685690669));
#53396=CARTESIAN_POINT('Ctrl Pts',(130.21301596426,31.61634022,28.3117988519883));
#53397=CARTESIAN_POINT('Ctrl Pts',(129.896301421753,31.602418573742,28.2923553739511));
#53398=CARTESIAN_POINT('Ctrl Pts',(129.643324707481,31.6196063153522,28.27602309344));
#53399=CARTESIAN_POINT('Ctrl Pts',(129.248223399285,31.6913166453197,28.2501853300543));
#53400=CARTESIAN_POINT('Ctrl Pts',(129.103686967136,31.7275109423525,28.2406823804366));
#53401=CARTESIAN_POINT('Ctrl Pts',(128.93503823822,31.7817609048842,28.2298562266376));
#53402=CARTESIAN_POINT('Ctrl Pts',(128.908198448345,31.7907670833852,28.2281416562374));
#53403=CARTESIAN_POINT('Ctrl Pts',(128.865870964788,31.8055627122895,28.2254544641373));
#53404=CARTESIAN_POINT('Ctrl Pts',(128.850307962199,31.8111308435338,28.2244700586326));
#53405=CARTESIAN_POINT('Ctrl Pts',(128.820353738658,31.8220956655272,28.2225832317353));
#53406=CARTESIAN_POINT('Ctrl Pts',(128.805957589125,31.8274767157732,28.2216800333339));
#53407=CARTESIAN_POINT('Ctrl Pts',(128.770317979797,31.8410751869875,28.2194520079547));
#53408=CARTESIAN_POINT('Ctrl Pts',(128.749119364781,31.8494093344111,28.2181338009025));
#53409=CARTESIAN_POINT('Ctrl Pts',(128.666574782292,31.8828258809621,28.2130225573489));
#53410=CARTESIAN_POINT('Ctrl Pts',(128.605882259017,31.90949289428,28.209311459649));
#53411=CARTESIAN_POINT('Ctrl Pts',(128.438353390463,31.9890421331644,28.1990980972361));
#53412=CARTESIAN_POINT('Ctrl Pts',(128.333464171249,32.0458048586648,28.1927372108013));
#53413=CARTESIAN_POINT('Ctrl Pts',(128.019115313631,32.238002050537,28.173171193243));
#53414=CARTESIAN_POINT('Ctrl Pts',(127.821462669881,32.391072875728,28.160074203684));
#53415=CARTESIAN_POINT('Ctrl Pts',(127.605609359429,32.6000171651751,28.1432371133889));
#53416=CARTESIAN_POINT('Ctrl Pts',(127.569650312907,32.6364382469302,28.1403374054098));
#53417=CARTESIAN_POINT('Ctrl Pts',(127.514109692311,32.6953004851045,28.1356959956543));
#53418=CARTESIAN_POINT('Ctrl Pts',(127.493974950627,32.7172102930258,28.1339778050777));
#53419=CARTESIAN_POINT('Ctrl Pts',(127.456424337209,32.7591669160105,28.1307035064515));
#53420=CARTESIAN_POINT('Ctrl Pts',(127.438950427376,32.7791589229117,28.1291499781799));
#53421=CARTESIAN_POINT('Ctrl Pts',(127.399558010848,32.8253112444638,28.1255775324848));
#53422=CARTESIAN_POINT('Ctrl Pts',(127.377796382142,32.8516011121898,28.1235525109746));
#53423=CARTESIAN_POINT('Ctrl Pts',(127.309828184662,32.936283692104,28.1170587617667));
#53424=CARTESIAN_POINT('Ctrl Pts',(127.265149364582,32.995869238157,28.1125319500083));
#53425=CARTESIAN_POINT('Ctrl Pts',(127.161516698363,33.144003102298,28.1013756354379));
#53426=CARTESIAN_POINT('Ctrl Pts',(127.10470030721,33.2339454659358,28.0946805491506));
#53427=CARTESIAN_POINT('Ctrl Pts',(126.956433718969,33.4950950151653,28.0755308302079));
#53428=CARTESIAN_POINT('Ctrl Pts',(126.875319596041,33.6716910429383,28.0628946674612));
#53429=CARTESIAN_POINT('Ctrl Pts',(126.77924151185,33.9392129151538,28.0448296209382));
#53430=CARTESIAN_POINT('Ctrl Pts',(126.752132136427,34.0253660160909,28.0391708453404));
#53431=CARTESIAN_POINT('Ctrl Pts',(126.721709489226,34.1375107555842,28.032090434298));
#53432=CARTESIAN_POINT('Ctrl Pts',(126.715212603212,34.162594353656,28.0305248767131));
#53433=CARTESIAN_POINT('Ctrl Pts',(126.705167702483,34.2032933536749,28.0280166594166));
#53434=CARTESIAN_POINT('Ctrl Pts',(126.70144171656,34.2188632495394,28.0270646289969));
#53435=CARTESIAN_POINT('Ctrl Pts',(126.694277203055,34.2497675106689,28.0251906422662));
#53436=CARTESIAN_POINT('Ctrl Pts',(126.690834745472,34.2651004605382,28.0242685122559));
#53437=CARTESIAN_POINT('Ctrl Pts',(126.682291777531,34.3044290235944,28.0219215344808));
#53438=CARTESIAN_POINT('Ctrl Pts',(126.677344789056,34.328457554312,28.0205049468539));
#53439=CARTESIAN_POINT('Ctrl Pts',(126.667033082523,34.3814499865233,28.0174147237341));
#53440=CARTESIAN_POINT('Ctrl Pts',(126.661784110045,34.4104345885619,28.0157466677298));
#53441=CARTESIAN_POINT('Ctrl Pts',(126.62602528337,34.6237113359987,28.0036111025836));
#53442=CARTESIAN_POINT('Ctrl Pts',(126.610416088327,34.8101883435728,27.9937443927268));
#53443=CARTESIAN_POINT('Ctrl Pts',(126.61025131837,34.9970103699449,27.9838400398653));
#53444=CARTESIAN_POINT('Origin',(130.,35.,32.7603849714045));
#53445=CARTESIAN_POINT('',(125.915001580773,34.9964062680618,28.3853849713761));
#53446=CARTESIAN_POINT('Ctrl Pts',(132.487160689988,38.2405642567579,29.1925548573102));
#53447=CARTESIAN_POINT('Ctrl Pts',(132.581690765635,38.1680116179144,29.1867409038837));
#53448=CARTESIAN_POINT('Ctrl Pts',(132.67315408253,38.0912344395281,29.1809269504572));
#53449=CARTESIAN_POINT('Ctrl Pts',(132.761153744737,38.0105240404164,29.1751129970307));
#53450=CARTESIAN_POINT('Ctrl Pts',(132.849077229458,37.9298835087917,29.1693040764911));
#53451=CARTESIAN_POINT('Ctrl Pts',(132.933542725555,37.845316805426,29.1634951559516));
#53452=CARTESIAN_POINT('Ctrl Pts',(133.014185814076,37.7571559401356,29.1576862354121));
#53453=CARTESIAN_POINT('Ctrl Pts',(133.094785419096,37.6690426120001,29.1518804470963));
#53454=CARTESIAN_POINT('Ctrl Pts',(133.171566440987,37.5773392769486,29.1460746587805));
#53455=CARTESIAN_POINT('Ctrl Pts',(133.244201165315,37.4824149127345,29.1402688704647));
#53456=CARTESIAN_POINT('Ctrl Pts',(133.316816230649,37.3875162403308,29.134464653518));
#53457=CARTESIAN_POINT('Ctrl Pts',(133.385286982042,37.2893985962056,29.1286604365713));
#53458=CARTESIAN_POINT('Ctrl Pts',(133.449326260106,37.1884636966017,29.1228562196246));
#53459=CARTESIAN_POINT('Ctrl Pts',(133.513363305932,37.0875323153176,29.1170522049974));
#53460=CARTESIAN_POINT('Ctrl Pts',(133.572968967077,36.98378421861,29.1112481903701));
#53461=CARTESIAN_POINT('Ctrl Pts',(133.627900017705,36.8776491848945,29.1054441757429));
#53462=CARTESIAN_POINT('Ctrl Pts',(133.682842106129,36.7714928245,29.0996389948621));
#53463=CARTESIAN_POINT('Ctrl Pts',(133.733107528507,36.6629489357843,29.0938338139814));
#53464=CARTESIAN_POINT('Ctrl Pts',(133.778499818206,36.5524703294487,29.0880286331006));
#53465=CARTESIAN_POINT('Ctrl Pts',(133.823939675865,36.4418759492238,29.0822173687943));
#53466=CARTESIAN_POINT('Ctrl Pts',(133.864496046327,36.3293431803229,29.0764061044881));
#53467=CARTESIAN_POINT('Ctrl Pts',(133.900021202843,36.2153434154088,29.0705948401819));
#53468=CARTESIAN_POINT('Ctrl Pts',(133.935565748714,36.1012814303058,29.0647804041326));
#53469=CARTESIAN_POINT('Ctrl Pts',(133.966073505789,35.9857512485749,29.0589659680832));
#53470=CARTESIAN_POINT('Ctrl Pts',(133.99144751717,35.8692362841478,29.0531515320339));
#53471=CARTESIAN_POINT('Ctrl Pts',(134.016861593775,35.7525373441513,29.0473279150679));
#53472=CARTESIAN_POINT('Ctrl Pts',(134.037125660968,35.6348509173009,29.0415042981019));
#53473=CARTESIAN_POINT('Ctrl Pts',(134.052194377336,35.5166679090954,29.0356806811359));
#53474=CARTESIAN_POINT('Ctrl Pts',(134.064126351656,35.4230861742918,29.0310693229823));
#53475=CARTESIAN_POINT('Ctrl Pts',(134.072801833475,35.3291932530324,29.0264579648287));
#53476=CARTESIAN_POINT('Ctrl Pts',(134.078221501167,35.235232624052,29.021846606675));
#53477=CARTESIAN_POINT('Ctrl Pts',(134.085065207076,35.1165834838716,29.016023596698));
#53478=CARTESIAN_POINT('Ctrl Pts',(134.086737820651,34.9974437193359,29.0102005867211));
#53479=CARTESIAN_POINT('Ctrl Pts',(134.083186794953,34.8783012016325,29.0043775767441));
#53480=CARTESIAN_POINT('Ctrl Pts',(134.079640254598,34.7593091742895,28.9985619218818));
#53481=CARTESIAN_POINT('Ctrl Pts',(134.07088321031,34.6403148053383,28.9927462670194));
#53482=CARTESIAN_POINT('Ctrl Pts',(134.05691497557,34.5218097857627,28.986930612157));
#53483=CARTESIAN_POINT('Ctrl Pts',(134.042960741383,34.4034235453878,28.981120786405));
#53484=CARTESIAN_POINT('Ctrl Pts',(134.023805755227,34.2855260819284,28.975310960653));
#53485=CARTESIAN_POINT('Ctrl Pts',(133.999501340222,34.1686071749385,28.9695011349009));
#53486=CARTESIAN_POINT('Ctrl Pts',(133.97427342688,34.0472456834969,28.9634705523678));
#53487=CARTESIAN_POINT('Ctrl Pts',(133.943497010083,33.9269390362428,28.9574399698347));
#53488=CARTESIAN_POINT('Ctrl Pts',(133.907288468512,33.8082274445867,28.9514093873016));
#53489=CARTESIAN_POINT('Ctrl Pts',(133.872444733883,33.6939904436618,28.9456061152471));
#53490=CARTESIAN_POINT('Ctrl Pts',(133.832571097199,33.5812308562466,28.9398028431925));
#53491=CARTESIAN_POINT('Ctrl Pts',(133.787822753732,33.4704171201558,28.9339995711379));
#53492=CARTESIAN_POINT('Ctrl Pts',(133.743081051571,33.3596198304379,28.9281971603735));
#53493=CARTESIAN_POINT('Ctrl Pts',(133.69346623428,33.2507681963479,28.922394749609));
#53494=CARTESIAN_POINT('Ctrl Pts',(133.639182103552,33.1443118211332,28.9165923388446));
#53495=CARTESIAN_POINT('Ctrl Pts',(133.584893210769,33.0378461070718,28.9107894190658));
#53496=CARTESIAN_POINT('Ctrl Pts',(133.525934375693,32.933776433535,28.9049864992869));
#53497=CARTESIAN_POINT('Ctrl Pts',(133.462555627298,32.832528309788,28.8991835795081));
#53498=CARTESIAN_POINT('Ctrl Pts',(133.399156352903,32.7312473955718,28.8933787803813));
#53499=CARTESIAN_POINT('Ctrl Pts',(133.331334534987,32.6327901944861,28.8875739812544));
#53500=CARTESIAN_POINT('Ctrl Pts',(133.259383468629,32.5375531671871,28.8817691821275));
#53501=CARTESIAN_POINT('Ctrl Pts',(133.187352725038,32.4422106762284,28.8759579548773));
#53502=CARTESIAN_POINT('Ctrl Pts',(133.111183851963,32.3500958030861,28.8701467276271));
#53503=CARTESIAN_POINT('Ctrl Pts',(133.031210463438,32.2615719607152,28.8643355003769));
#53504=CARTESIAN_POINT('Ctrl Pts',(132.951184559165,32.1729899878093,28.8585204570954));
#53505=CARTESIAN_POINT('Ctrl Pts',(132.867349450225,32.0880040319731,28.852705413814));
#53506=CARTESIAN_POINT('Ctrl Pts',(132.780074430544,32.0069394993355,28.8468903705325));
#53507=CARTESIAN_POINT('Ctrl Pts',(132.692674341008,31.92575879681,28.8410669939775));
#53508=CARTESIAN_POINT('Ctrl Pts',(132.601824811626,31.8485109975396,28.8352436174225));
#53509=CARTESIAN_POINT('Ctrl Pts',(132.507926985996,31.7754803097343,28.8294202408675));
#53510=CARTESIAN_POINT('Ctrl Pts',(132.482917742351,31.7560289299747,28.8278692119472));
#53511=CARTESIAN_POINT('Ctrl Pts',(132.457692403287,31.7368764672564,28.8263181830269));
#53512=CARTESIAN_POINT('Ctrl Pts',(132.432258861009,31.7180277525484,28.8247671541066));
#53513=CARTESIAN_POINT('Ctrl Pts',(132.336762586141,31.6472557766668,28.8189434476609));
#53514=CARTESIAN_POINT('Ctrl Pts',(132.238020892333,31.5805411803083,28.8131197412152));
#53515=CARTESIAN_POINT('Ctrl Pts',(132.136413171174,31.5181953297125,28.8072960347695));
#53516=CARTESIAN_POINT('Ctrl Pts',(132.034933632443,31.4559281310388,28.8014796751753));
#53517=CARTESIAN_POINT('Ctrl Pts',(131.930595602701,31.398018927822,28.7956633155811));
#53518=CARTESIAN_POINT('Ctrl Pts',(131.823810085798,31.3447377972379,28.7898469559869));
#53519=CARTESIAN_POINT('Ctrl Pts',(131.717131453584,31.2915099972665,28.7840364181539));
#53520=CARTESIAN_POINT('Ctrl Pts',(131.608010570973,31.2429012356439,28.778225880321));
#53521=CARTESIAN_POINT('Ctrl Pts',(131.496885342853,31.1991370360993,28.772415342488));
#53522=CARTESIAN_POINT('Ctrl Pts',(131.381556861378,31.1537174787061,28.7663850241151));
#53523=CARTESIAN_POINT('Ctrl Pts',(131.264069795977,31.1135164398812,28.7603547057422));
#53524=CARTESIAN_POINT('Ctrl Pts',(131.14493963677,31.078732573752,28.7543243873693));
#53525=CARTESIAN_POINT('Ctrl Pts',(131.030280484246,31.0452541612459,28.7485203894674));
#53526=CARTESIAN_POINT('Ctrl Pts',(130.914099774573,31.0167937561008,28.7427163915656));
#53527=CARTESIAN_POINT('Ctrl Pts',(130.796874481907,30.9934783090459,28.7369123936637));
#53528=CARTESIAN_POINT('Ctrl Pts',(130.679666507778,30.97016630655,28.7311092532284));
#53529=CARTESIAN_POINT('Ctrl Pts',(130.561414657923,30.9519978301704,28.725306112793));
#53530=CARTESIAN_POINT('Ctrl Pts',(130.442606791871,30.9390488518342,28.7195029723576));
#53531=CARTESIAN_POINT('Ctrl Pts',(130.32378844262,30.9260987309244,28.713699319873));
#53532=CARTESIAN_POINT('Ctrl Pts',(130.204414385562,30.9183690679873,28.7078956673884));
#53533=CARTESIAN_POINT('Ctrl Pts',(130.084977664052,30.9158839638653,28.7020920149038));
#53534=CARTESIAN_POINT('Ctrl Pts',(129.965502220096,30.9133980540505,28.6962864808235));
#53535=CARTESIAN_POINT('Ctrl Pts',(129.845964479303,30.916160093121,28.6904809467431));
#53536=CARTESIAN_POINT('Ctrl Pts',(129.72685690328,30.9241420720646,28.6846754126628));
#53537=CARTESIAN_POINT('Ctrl Pts',(129.607617453919,30.932132888483,28.6788634508204));
#53538=CARTESIAN_POINT('Ctrl Pts',(129.488809527649,30.9453551536462,28.6730514889781));
#53539=CARTESIAN_POINT('Ctrl Pts',(129.370920045251,30.963729021667,28.6672395271357));
#53540=CARTESIAN_POINT('Ctrl Pts',(129.252953145497,30.982114955703,28.6614237486109));
#53541=CARTESIAN_POINT('Ctrl Pts',(129.135906290161,31.0056591496562,28.655607970086));
#53542=CARTESIAN_POINT('Ctrl Pts',(129.020254170505,31.034231082175,28.6497921915611));
#53543=CARTESIAN_POINT('Ctrl Pts',(128.904436428454,31.0628439318158,28.643968084411));
#53544=CARTESIAN_POINT('Ctrl Pts',(128.790017799052,31.0964987762113,28.6381439772608));
#53545=CARTESIAN_POINT('Ctrl Pts',(128.677455975987,31.1350158726654,28.6323198701107));
#53546=CARTESIAN_POINT('Ctrl Pts',(128.64761418646,31.1452273196222,28.6307758139198));
#53547=CARTESIAN_POINT('Ctrl Pts',(128.61790278324,31.1557802566211,28.629231757729));
#53548=CARTESIAN_POINT('Ctrl Pts',(128.588330019733,31.1666707854902,28.6276877015381));
#53549=CARTESIAN_POINT('Ctrl Pts',(128.476791316995,31.2077462657013,28.6218640312394));
#53550=CARTESIAN_POINT('Ctrl Pts',(128.366867061984,31.253760178499,28.6160403609406));
#53551=CARTESIAN_POINT('Ctrl Pts',(128.259025636051,31.3045658896317,28.6102166906419));
#53552=CARTESIAN_POINT('Ctrl Pts',(128.151320237252,31.3553075163439,28.6044003661027));
#53553=CARTESIAN_POINT('Ctrl Pts',(128.045692808213,31.4108287471307,28.5985840415635));
#53554=CARTESIAN_POINT('Ctrl Pts',(127.942594525573,31.470933875117,28.5927677170243));
#53555=CARTESIAN_POINT('Ctrl Pts',(127.839599417534,31.5309788534823,28.5869572131151));
#53556=CARTESIAN_POINT('Ctrl Pts',(127.73912877147,31.5955983987234,28.581146709206));
#53557=CARTESIAN_POINT('Ctrl Pts',(127.641611246505,31.6645498823413,28.5753362052969));
#53558=CARTESIAN_POINT('Ctrl Pts',(127.540404360988,31.736109993319,28.5693058737833));
#53559=CARTESIAN_POINT('Ctrl Pts',(127.442378864502,31.8123361035121,28.5632755422696));
#53560=CARTESIAN_POINT('Ctrl Pts',(127.347983481711,31.8929059578566,28.557245210756));
#53561=CARTESIAN_POINT('Ctrl Pts',(127.257131479608,31.9704514093396,28.5514412437063));
#53562=CARTESIAN_POINT('Ctrl Pts',(127.16964231007,32.0520200861198,28.5456372766565));
#53563=CARTESIAN_POINT('Ctrl Pts',(127.085883603764,32.1372826494414,28.5398333096068));
#53564=CARTESIAN_POINT('Ctrl Pts',(127.002137254553,32.2225326338013,28.5340301988283));
#53565=CARTESIAN_POINT('Ctrl Pts',(126.922120560146,32.3114751297278,28.5282270880498));
#53566=CARTESIAN_POINT('Ctrl Pts',(126.846164480396,32.4037437500732,28.5224239772712));
#53567=CARTESIAN_POINT('Ctrl Pts',(126.770201682356,32.496020531548,28.5166203532095));
#53568=CARTESIAN_POINT('Ctrl Pts',(126.698300472598,32.5916237071096,28.5108167291477));
#53569=CARTESIAN_POINT('Ctrl Pts',(126.63075126853,32.6901541208372,28.5050131050859));
#53570=CARTESIAN_POINT('Ctrl Pts',(126.563180149476,32.7887165007823,28.4992075981547));
#53571=CARTESIAN_POINT('Ctrl Pts',(126.499964074872,32.8902076709954,28.4934020912234));
#53572=CARTESIAN_POINT('Ctrl Pts',(126.441349559543,32.9942003981873,28.4875965842922));
#53573=CARTESIAN_POINT('Ctrl Pts',(126.382670126589,33.09830830096,28.481784647559));
#53574=CARTESIAN_POINT('Ctrl Pts',(126.32860262635,33.2049229350681,28.4759727108259));
#53575=CARTESIAN_POINT('Ctrl Pts',(126.279347181127,33.3135932870715,28.4701607740928));
#53576=CARTESIAN_POINT('Ctrl Pts',(126.230059380157,33.4223350242861,28.4643450195168));
#53577=CARTESIAN_POINT('Ctrl Pts',(126.185590081203,33.5331347906707,28.4585292649407));
#53578=CARTESIAN_POINT('Ctrl Pts',(126.146090318909,33.6455240238415,28.4527135103647));
#53579=CARTESIAN_POINT('Ctrl Pts',(126.106533976932,33.7580742439836,28.446889425269));
#53580=CARTESIAN_POINT('Ctrl Pts',(126.071961497484,33.8722180857994,28.4410653401734));
#53581=CARTESIAN_POINT('Ctrl Pts',(126.042473430204,33.9874742228666,28.4352412550777));
#53582=CARTESIAN_POINT('Ctrl Pts',(126.034654268134,34.0180359550677,28.4336969197083));
#53583=CARTESIAN_POINT('Ctrl Pts',(126.027192318522,34.0486758547276,28.432152584339));
#53584=CARTESIAN_POINT('Ctrl Pts',(126.020088845761,34.0793848771795,28.4306082489696));
#53585=CARTESIAN_POINT('Ctrl Pts',(125.984344514023,34.2339111944862,28.4228372280037));
#53586=CARTESIAN_POINT('Ctrl Pts',(125.957588052264,34.3905878428019,28.4150662070378));
#53587=CARTESIAN_POINT('Ctrl Pts',(125.940025229609,34.5485247916084,28.407295186072));
#53588=CARTESIAN_POINT('Ctrl Pts',(125.923519238259,34.6969579883735,28.3999917811828));
#53589=CARTESIAN_POINT('Ctrl Pts',(125.915133455108,34.8465046131736,28.3926883762936));
#53590=CARTESIAN_POINT('Ctrl Pts',(125.915001580773,34.9964062674799,28.3853849714045));
#53591=CARTESIAN_POINT('Ctrl Pts',(125.915001580773,34.9964062680618,28.3853849713761));
#53592=CARTESIAN_POINT('Ctrl Pts',(125.914898004711,35.1141412731948,28.3796487677559));
#53593=CARTESIAN_POINT('Ctrl Pts',(125.919888554547,35.2320185491245,28.3739125641357));
#53594=CARTESIAN_POINT('Ctrl Pts',(125.929983362015,35.3495562422898,28.3681763605155));
#53595=CARTESIAN_POINT('Ctrl Pts',(125.940070876034,35.4670090150511,28.3624443012741));
#53596=CARTESIAN_POINT('Ctrl Pts',(125.955255278668,35.5841222759973,28.3567122420327));
#53597=CARTESIAN_POINT('Ctrl Pts',(125.975494634492,35.700415278957,28.3509801827913));
#53598=CARTESIAN_POINT('Ctrl Pts',(125.995726327814,35.8166642540619,28.3452502936742));
#53599=CARTESIAN_POINT('Ctrl Pts',(126.021009099457,35.9320931751257,28.3395204045571));
#53600=CARTESIAN_POINT('Ctrl Pts',(126.051249363658,36.0462281835202,28.33379051544));
#53601=CARTESIAN_POINT('Ctrl Pts',(126.0814857669,36.1603486195975,28.3280613578931));
#53602=CARTESIAN_POINT('Ctrl Pts',(126.116678296784,36.2731750655389,28.3223322003461));
#53603=CARTESIAN_POINT('Ctrl Pts',(126.156682817604,36.3842463781795,28.3166030427991));
#53604=CARTESIAN_POINT('Ctrl Pts',(126.196692269025,36.495331380479,28.3108731791273));
#53605=CARTESIAN_POINT('Ctrl Pts',(126.24151474706,36.6046604246836,28.3051433154555));
#53606=CARTESIAN_POINT('Ctrl Pts',(126.290957340198,36.7117907429857,28.2994134517837));
#53607=CARTESIAN_POINT('Ctrl Pts',(126.340448490637,36.8190262733863,28.2936779608442));
#53608=CARTESIAN_POINT('Ctrl Pts',(126.394568641031,36.9240583837005,28.2879424699047));
#53609=CARTESIAN_POINT('Ctrl Pts',(126.453078077212,37.0264673384101,28.2822069789652));
#53610=CARTESIAN_POINT('Ctrl Pts',(126.511616981188,37.1289278705461,28.2764685993929));
#53611=CARTESIAN_POINT('Ctrl Pts',(126.574549348282,37.2287622617238,28.2707302198206));
#53612=CARTESIAN_POINT('Ctrl Pts',(126.641592152127,37.3255798690533,28.2649918402483));
#53613=CARTESIAN_POINT('Ctrl Pts',(126.708740659179,37.4225501241103,28.2592444132453));
#53614=CARTESIAN_POINT('Ctrl Pts',(126.780012293326,37.5164937607468,28.2534969862422));
#53615=CARTESIAN_POINT('Ctrl Pts',(126.855083559348,37.6070530453589,28.2477495592392));
#53616=CARTESIAN_POINT('Ctrl Pts',(126.916999420102,37.6817428215291,28.2430093049598));
#53617=CARTESIAN_POINT('Ctrl Pts',(126.981499109161,37.754131023783,28.2382690506805));
#53618=CARTESIAN_POINT('Ctrl Pts',(127.04838334079,37.8240368441422,28.2335287964012));
#53619=CARTESIAN_POINT('Ctrl Pts',(127.130553566367,37.9099192246102,28.2277051851563));
#53620=CARTESIAN_POINT('Ctrl Pts',(127.21660774636,37.9923507865766,28.2218815739113));
#53621=CARTESIAN_POINT('Ctrl Pts',(127.306224543499,38.0709605647014,28.2160579626664));
#53622=CARTESIAN_POINT('Ctrl Pts',(127.395728278124,38.1494711670094,28.2102416986169));
#53623=CARTESIAN_POINT('Ctrl Pts',(127.488785385822,38.2241693087236,28.2044254345674));
#53624=CARTESIAN_POINT('Ctrl Pts',(127.585036396985,38.2947193804804,28.1986091705178));
#53625=CARTESIAN_POINT('Ctrl Pts',(127.681191062474,38.3651988327794,28.1927987284527));
#53626=CARTESIAN_POINT('Ctrl Pts',(127.780532943856,38.4315382352989,28.1869882863875));
#53627=CARTESIAN_POINT('Ctrl Pts',(127.882668531465,38.4934413480623,28.1811778443223));
#53628=CARTESIAN_POINT('Ctrl Pts',(127.988669720613,38.5576873539699,28.1751474901353));
#53629=CARTESIAN_POINT('Ctrl Pts',(128.097679927859,38.617154333157,28.1691171359482));
#53630=CARTESIAN_POINT('Ctrl Pts',(128.209224603579,38.6715594070603,28.1630867817611));
#53631=CARTESIAN_POINT('Ctrl Pts',(128.316580551466,38.72392146057,28.1572828795518));
#53632=CARTESIAN_POINT('Ctrl Pts',(128.426283651319,38.77159472813,28.1514789773425));
#53633=CARTESIAN_POINT('Ctrl Pts',(128.53788523552,38.8143735285746,28.1456750751332));
#53634=CARTESIAN_POINT('Ctrl Pts',(128.649470335548,38.857146010353,28.1398720301924));
#53635=CARTESIAN_POINT('Ctrl Pts',(128.762952981085,38.8950253166028,28.1340689852517));
#53636=CARTESIAN_POINT('Ctrl Pts',(128.877865165376,38.9278541740908,28.1282659403109));
#53637=CARTESIAN_POINT('Ctrl Pts',(128.992787495324,38.9606859300563,28.1224623830162));
#53638=CARTESIAN_POINT('Ctrl Pts',(129.109139222327,38.988466238516,28.1166588257215));
#53639=CARTESIAN_POINT('Ctrl Pts',(129.226438469627,39.0110880766603,28.1108552684268));
#53640=CARTESIAN_POINT('Ctrl Pts',(129.343775755335,39.0337172507317,28.1050498291244));
#53641=CARTESIAN_POINT('Ctrl Pts',(129.462060771685,39.0511845503497,28.099244389822));
#53642=CARTESIAN_POINT('Ctrl Pts',(129.580803414552,39.0634344122613,28.0934389505196));
#53643=CARTESIAN_POINT('Ctrl Pts',(129.699677551255,39.0756978394876,28.0876270823602));
#53644=CARTESIAN_POINT('Ctrl Pts',(129.819009919609,39.08273225427,28.0818152142007));
#53645=CARTESIAN_POINT('Ctrl Pts',(129.938307122138,39.0845341213927,28.0760033460413));
#53646=CARTESIAN_POINT('Ctrl Pts',(130.057682678586,39.0863371719744,28.0701876606704));
#53647=CARTESIAN_POINT('Ctrl Pts',(130.177022615984,39.0829008423141,28.0643719752995));
#53648=CARTESIAN_POINT('Ctrl Pts',(130.295837032635,39.0742736101202,28.0585562899286));
#53649=CARTESIAN_POINT('Ctrl Pts',(130.414821633508,39.0656340206817,28.0527322744416));
#53650=CARTESIAN_POINT('Ctrl Pts',(130.533278807089,39.0517887356762,28.0469082589546));
#53651=CARTESIAN_POINT('Ctrl Pts',(130.650727092607,39.0328376177262,28.0410842434676));
#53652=CARTESIAN_POINT('Ctrl Pts',(130.681883203419,39.0278103571897,28.0395392769226));
#53653=CARTESIAN_POINT('Ctrl Pts',(130.712968393572,39.0224240687474,28.0379943103777));
#53654=CARTESIAN_POINT('Ctrl Pts',(130.743973854194,39.0166812052085,28.0364493438327));
#53655=CARTESIAN_POINT('Ctrl Pts',(130.860849615099,38.995033355688,28.0306255587031));
#53656=CARTESIAN_POINT('Ctrl Pts',(130.976968212525,38.9682451577193,28.0248017735734));
#53657=CARTESIAN_POINT('Ctrl Pts',(131.091843191552,38.9363820247865,28.0189779884437));
#53658=CARTESIAN_POINT('Ctrl Pts',(131.20657781608,38.9045578222985,28.0131613188273));
#53659=CARTESIAN_POINT('Ctrl Pts',(131.320071453772,38.8676711237568,28.007344649211));
#53660=CARTESIAN_POINT('Ctrl Pts',(131.431846261862,38.8258386377879,28.0015279795946));
#53661=CARTESIAN_POINT('Ctrl Pts',(131.543491558863,38.7840546222295,27.9957180496294));
#53662=CARTESIAN_POINT('Ctrl Pts',(131.653421610726,38.7373363697412,27.9899081196642));
#53663=CARTESIAN_POINT('Ctrl Pts',(131.761173065314,38.685850571308,27.984098189699));
#53664=CARTESIAN_POINT('Ctrl Pts',(131.868852414126,38.6343992264558,27.9782921476582));
#53665=CARTESIAN_POINT('Ctrl Pts',(131.974355697965,38.5781868559141,27.9724861056175));
#53666=CARTESIAN_POINT('Ctrl Pts',(132.07723915953,38.517428389337,27.9666800635767));
#53667=CARTESIAN_POINT('Ctrl Pts',(132.180077496822,38.4566965711794,27.9608765680427));
#53668=CARTESIAN_POINT('Ctrl Pts',(132.280297947008,38.3914228312968,27.9550730725086));
#53669=CARTESIAN_POINT('Ctrl Pts',(132.377481582068,38.3218678972719,27.9492695769746));
#53670=CARTESIAN_POINT('Ctrl Pts',(132.414488708325,38.295381666091,27.9470596298799));
#53671=CARTESIAN_POINT('Ctrl Pts',(132.451055758543,38.2682750994043,27.9448496827852));
#53672=CARTESIAN_POINT('Ctrl Pts',(132.487160689988,38.2405642567579,27.9426397356904));
#53673=CARTESIAN_POINT('',(125.915001103447,35.0030025254734,28.4896150285558));
#53674=CARTESIAN_POINT('Ctrl Pts',(125.915001103447,35.0030025254734,28.4896150285558));
#53675=CARTESIAN_POINT('Ctrl Pts',(125.915102919105,35.1415248644931,28.4828889783069));
#53676=CARTESIAN_POINT('Ctrl Pts',(125.922254616048,35.2797632987396,28.4761629280581));
#53677=CARTESIAN_POINT('Ctrl Pts',(125.936346099466,35.4170635163571,28.4694368778092));
#53678=CARTESIAN_POINT('Ctrl Pts',(125.950518218314,35.5551494044232,28.4626723392097));
#53679=CARTESIAN_POINT('Ctrl Pts',(125.971709663148,35.6922861909673,28.4559078006102));
#53680=CARTESIAN_POINT('Ctrl Pts',(125.999759168527,35.8278274519563,28.4491432620107));
#53681=CARTESIAN_POINT('Ctrl Pts',(126.027989137381,35.9642407513876,28.4423352020683));
#53682=CARTESIAN_POINT('Ctrl Pts',(126.063165613499,36.0990378158406,28.4355271421258));
#53683=CARTESIAN_POINT('Ctrl Pts',(126.10507589336,36.2315807742544,28.4287190821834));
#53684=CARTESIAN_POINT('Ctrl Pts',(126.116063707408,36.2663301814467,28.4269341812731));
#53685=CARTESIAN_POINT('Ctrl Pts',(126.12751412061,36.3009247684037,28.4251492803627));
#53686=CARTESIAN_POINT('Ctrl Pts',(126.139422765552,36.3353532929025,28.4233643794524));
#53687=CARTESIAN_POINT('Ctrl Pts',(126.178277840155,36.4476853755434,28.4175406725268));
#53688=CARTESIAN_POINT('Ctrl Pts',(126.222102451514,36.558501283174,28.4117169656011));
#53689=CARTESIAN_POINT('Ctrl Pts',(126.270759287032,36.667329812827,28.4058932586755));
#53690=CARTESIAN_POINT('Ctrl Pts',(126.319354739941,36.7760210507917,28.4000768985968));
#53691=CARTESIAN_POINT('Ctrl Pts',(126.372770126904,36.8827295279913,28.3942605385182));
#53692=CARTESIAN_POINT('Ctrl Pts',(126.430818730963,36.9870002689362,28.3884441784395));
#53693=CARTESIAN_POINT('Ctrl Pts',(126.488809232551,37.0911666423827,28.3826336401182));
#53694=CARTESIAN_POINT('Ctrl Pts',(126.551423527991,37.1928997789442,28.3768231017969));
#53695=CARTESIAN_POINT('Ctrl Pts',(126.61842754107,37.2917662849882,28.3710125634756));
#53696=CARTESIAN_POINT('Ctrl Pts',(126.687965937794,37.3943723529533,28.3649822452843));
#53697=CARTESIAN_POINT('Ctrl Pts',(126.762232502365,37.493890242639,28.358951927093));
#53698=CARTESIAN_POINT('Ctrl Pts',(126.840913953207,37.5898649287092,28.3529216089017));
#53699=CARTESIAN_POINT('Ctrl Pts',(126.916642463719,37.6822376537309,28.3471176105049));
#53700=CARTESIAN_POINT('Ctrl Pts',(126.996460165988,37.771327993409,28.3413136121082));
#53701=CARTESIAN_POINT('Ctrl Pts',(127.080045079766,37.8567618493323,28.3355096137114));
#53702=CARTESIAN_POINT('Ctrl Pts',(127.163617644965,37.94218308352,28.3297064727796));
#53703=CARTESIAN_POINT('Ctrl Pts',(127.250956029385,38.0239486164502,28.3239033318477));
#53704=CARTESIAN_POINT('Ctrl Pts',(127.341700483724,38.1017202778081,28.3181001909158));
#53705=CARTESIAN_POINT('Ctrl Pts',(127.432452945057,38.1794988014839,28.3122965379338));
#53706=CARTESIAN_POINT('Ctrl Pts',(127.526611763807,38.2532824871939,28.3064928849517));
#53707=CARTESIAN_POINT('Ctrl Pts',(127.623783623465,38.3227730485074,28.3006892319696));
#53708=CARTESIAN_POINT('Ctrl Pts',(127.72098698711,38.3922861392827,28.2948836973912));
#53709=CARTESIAN_POINT('Ctrl Pts',(127.821205002449,38.4575031001514,28.2890781628129));
#53710=CARTESIAN_POINT('Ctrl Pts',(127.92401540947,38.518168981144,28.2832726282346));
#53711=CARTESIAN_POINT('Ctrl Pts',(128.026939645913,38.578902030066,28.2774606658961));
#53712=CARTESIAN_POINT('Ctrl Pts',(128.132461651413,38.6350737334926,28.2716487035575));
#53713=CARTESIAN_POINT('Ctrl Pts',(128.240134469473,38.6864750527383,28.2658367412189));
#53714=CARTESIAN_POINT('Ctrl Pts',(128.347877995648,38.7379101269329,28.2600209621984));
#53715=CARTESIAN_POINT('Ctrl Pts',(128.457774772286,38.7845684189146,28.2542051831778));
#53716=CARTESIAN_POINT('Ctrl Pts',(128.56935932259,38.82628961948,28.2483894041572));
#53717=CARTESIAN_POINT('Ctrl Pts',(128.68110367013,38.8680705678554,28.2425652965157));
#53718=CARTESIAN_POINT('Ctrl Pts',(128.794540228585,38.9049001872796,28.2367411888743));
#53719=CARTESIAN_POINT('Ctrl Pts',(128.909189757158,38.9366683901633,28.2309170812329));
#53720=CARTESIAN_POINT('Ctrl Pts',(128.939584932126,38.9450905799192,28.2293730297833));
#53721=CARTESIAN_POINT('Ctrl Pts',(128.970065315596,38.953157306727,28.2278289783336));
#53722=CARTESIAN_POINT('Ctrl Pts',(129.000621894753,38.9608671276318,28.226284926884));
#53723=CARTESIAN_POINT('Ctrl Pts',(129.115878570033,38.9899478804179,28.2204609033366));
#53724=CARTESIAN_POINT('Ctrl Pts',(129.232591433716,39.0140405845588,28.2146368797891));
#53725=CARTESIAN_POINT('Ctrl Pts',(129.350291032808,39.0330017676603,28.2088128562417));
#53726=CARTESIAN_POINT('Ctrl Pts',(129.467840460985,39.0519387585109,28.2029962634668));
#53727=CARTESIAN_POINT('Ctrl Pts',(129.586373720696,39.0657571869573,28.1971796706919));
#53728=CARTESIAN_POINT('Ctrl Pts',(129.705407868,39.0743638123962,28.1913630779171));
#53729=CARTESIAN_POINT('Ctrl Pts',(129.828536064991,39.0832664533314,28.1853464297768));
#53730=CARTESIAN_POINT('Ctrl Pts',(129.952199804614,39.0865921982106,28.1793297816366));
#53731=CARTESIAN_POINT('Ctrl Pts',(130.075854077224,39.0842956747729,28.1733131334963));
#53732=CARTESIAN_POINT('Ctrl Pts',(130.19517954854,39.082079546403,28.1675071119176));
#53733=CARTESIAN_POINT('Ctrl Pts',(130.314495756203,39.0746281826785,28.1617010903388));
#53734=CARTESIAN_POINT('Ctrl Pts',(130.433309747874,39.0619536755602,28.1558950687601));
#53735=CARTESIAN_POINT('Ctrl Pts',(130.552075622451,39.049284301343,28.1500913984944));
#53736=CARTESIAN_POINT('Ctrl Pts',(130.670339280224,39.0313960340944,28.1442877282288));
#53737=CARTESIAN_POINT('Ctrl Pts',(130.787611400039,39.0083529388677,28.1384840579631));
#53738=CARTESIAN_POINT('Ctrl Pts',(130.904863701188,38.9853137378605,28.1326813685017));
#53739=CARTESIAN_POINT('Ctrl Pts',(131.021124397455,38.9571215213546,28.1268786790403));
#53740=CARTESIAN_POINT('Ctrl Pts',(131.13591352441,38.9238916224918,28.1210759895789));
#53741=CARTESIAN_POINT('Ctrl Pts',(131.250710339632,38.8906594979799,28.115272911469));
#53742=CARTESIAN_POINT('Ctrl Pts',(131.364034997925,38.852389135171,28.1094698333591));
#53743=CARTESIAN_POINT('Ctrl Pts',(131.475422500075,38.8092457844398,28.1036667552492));
#53744=CARTESIAN_POINT('Ctrl Pts',(131.586890956033,38.7660710781394,28.0978594595991));
#53745=CARTESIAN_POINT('Ctrl Pts',(131.696419063995,38.7180164607688,28.0920521639489));
#53746=CARTESIAN_POINT('Ctrl Pts',(131.803561647476,38.6652954019771,28.0862448682988));
#53747=CARTESIAN_POINT('Ctrl Pts',(131.910750978871,38.6125513401973,28.0804350388386));
#53748=CARTESIAN_POINT('Ctrl Pts',(132.015552353511,38.5551369751747,28.0746252093783));
#53749=CARTESIAN_POINT('Ctrl Pts',(132.117546307303,38.4933111279171,28.068815379918));
#53750=CARTESIAN_POINT('Ctrl Pts',(132.219653685798,38.4314165258152,28.0629990895044));
#53751=CARTESIAN_POINT('Ctrl Pts',(132.318947071591,38.3651008737315,28.0571827990907));
#53752=CARTESIAN_POINT('Ctrl Pts',(132.415037021597,38.294665564866,28.051366508677));
#53753=CARTESIAN_POINT('Ctrl Pts',(132.439284017914,38.2768921694744,28.0498988466351));
#53754=CARTESIAN_POINT('Ctrl Pts',(132.463327209055,38.2588566565333,28.0484311845931));
#53755=CARTESIAN_POINT('Ctrl Pts',(132.487160689988,38.2405642567579,28.0469635225512));
#53756=CARTESIAN_POINT('Ctrl Pts',(132.487160689988,38.2405642567579,29.2969312480094));
#53757=CARTESIAN_POINT('Ctrl Pts',(132.582108042264,38.1676913545445,29.2911177030164));
#53758=CARTESIAN_POINT('Ctrl Pts',(132.673828553593,38.09065861231,29.2853041580235));
#53759=CARTESIAN_POINT('Ctrl Pts',(132.761950750955,38.0097928582048,29.2794906130305));
#53760=CARTESIAN_POINT('Ctrl Pts',(132.85016499061,37.9288426410506,29.2736709958783));
#53761=CARTESIAN_POINT('Ctrl Pts',(132.934773108887,37.8440516908564,29.2678513787261));
#53762=CARTESIAN_POINT('Ctrl Pts',(133.015439789088,37.7557844397532,29.2620317615739));
#53763=CARTESIAN_POINT('Ctrl Pts',(133.096149315893,37.6674703049552,29.2562090532962));
#53764=CARTESIAN_POINT('Ctrl Pts',(133.172912972251,37.5756765022524,29.2503863450185));
#53765=CARTESIAN_POINT('Ctrl Pts',(133.245436233957,37.4808000022812,29.2445636367407));
#53766=CARTESIAN_POINT('Ctrl Pts',(133.318075930572,37.3857711796431,29.2387315802002));
#53767=CARTESIAN_POINT('Ctrl Pts',(133.386461396551,37.287650104556,29.2328995236597));
#53768=CARTESIAN_POINT('Ctrl Pts',(133.450341557546,37.1868626240052,29.2270674671192));
#53769=CARTESIAN_POINT('Ctrl Pts',(133.506514652462,37.0982350341065,29.2219390413216));
#53770=CARTESIAN_POINT('Ctrl Pts',(133.559204577721,37.0075461828279,29.2168106155239));
#53771=CARTESIAN_POINT('Ctrl Pts',(133.608270922278,36.915099462545,29.2116821897262));
#53772=CARTESIAN_POINT('Ctrl Pts',(133.663941025846,36.8102104894807,29.2058635374938));
#53773=CARTESIAN_POINT('Ctrl Pts',(133.71512506242,36.7027201243151,29.2000448852614));
#53774=CARTESIAN_POINT('Ctrl Pts',(133.761571509473,36.5930488941413,29.194226233029));
#53775=CARTESIAN_POINT('Ctrl Pts',(133.807958816077,36.4835173087863,29.1884149897099));
#53776=CARTESIAN_POINT('Ctrl Pts',(133.849620372773,36.3718107547191,29.1826037463907));
#53777=CARTESIAN_POINT('Ctrl Pts',(133.886350153383,36.2583749382828,29.1767925030716));
#53778=CARTESIAN_POINT('Ctrl Pts',(133.923042786988,36.1450538462129,29.1709871370074));
#53779=CARTESIAN_POINT('Ctrl Pts',(133.954813441367,36.0300073578089,29.1651817709432));
#53780=CARTESIAN_POINT('Ctrl Pts',(133.981504125685,35.9137012078085,29.159376404879));
#53781=CARTESIAN_POINT('Ctrl Pts',(134.009237865327,35.7928498858889,29.153344168724));
#53782=CARTESIAN_POINT('Ctrl Pts',(134.031486323361,35.6706388565263,29.1473119325689));
#53783=CARTESIAN_POINT('Ctrl Pts',(134.048129187758,35.5476085090839,29.1412796964139));
#53784=CARTESIAN_POINT('Ctrl Pts',(134.064127785092,35.4293408274173,29.1354809760156));
#53785=CARTESIAN_POINT('Ctrl Pts',(134.074946651782,35.3103165242915,29.1296822556173));
#53786=CARTESIAN_POINT('Ctrl Pts',(134.080531129495,35.1910253941776,29.123883535219));
#53787=CARTESIAN_POINT('Ctrl Pts',(134.08611475254,35.071752520806,29.1180857022776));
#53788=CARTESIAN_POINT('Ctrl Pts',(134.086465560523,34.9522133102423,29.1122878693363));
#53789=CARTESIAN_POINT('Ctrl Pts',(134.081580924464,34.8329007568704,29.1064900363949));
#53790=CARTESIAN_POINT('Ctrl Pts',(134.07669587751,34.7135781669593,29.1006917157415));
#53791=CARTESIAN_POINT('Ctrl Pts',(134.066574527684,34.5944826809788,29.094893395088));
#53792=CARTESIAN_POINT('Ctrl Pts',(134.051266311449,34.4761047111119,29.0890950744346));
#53793=CARTESIAN_POINT('Ctrl Pts',(134.035953176953,34.3576887084832,29.0832948908826));
#53794=CARTESIAN_POINT('Ctrl Pts',(134.015449914474,34.2399910859764,29.0774947073306));
#53795=CARTESIAN_POINT('Ctrl Pts',(133.989857403606,34.1234939253545,29.0716945237786));
#53796=CARTESIAN_POINT('Ctrl Pts',(133.964236535414,34.0068676821355,29.0658879134368));
#53797=CARTESIAN_POINT('Ctrl Pts',(133.933515250763,33.8914449557314,29.0600813030951));
#53798=CARTESIAN_POINT('Ctrl Pts',(133.897844862505,33.7776946257816,29.0542746927534));
#53799=CARTESIAN_POINT('Ctrl Pts',(133.862151070597,33.6638696632573,29.0484642726444));
#53800=CARTESIAN_POINT('Ctrl Pts',(133.82150184772,33.5517196660969,29.0426538525354));
#53801=CARTESIAN_POINT('Ctrl Pts',(133.77609679007,33.4416938580555,29.0368434324265));
#53802=CARTESIAN_POINT('Ctrl Pts',(133.730626409303,33.3315097586448,29.0310246530119));
#53803=CARTESIAN_POINT('Ctrl Pts',(133.680386709373,33.2234563175936,29.0252058735973));
#53804=CARTESIAN_POINT('Ctrl Pts',(133.625623418858,33.1179586017766,29.0193870941828));
#53805=CARTESIAN_POINT('Ctrl Pts',(133.610614135122,33.0890442481051,29.0177923085078));
#53806=CARTESIAN_POINT('Ctrl Pts',(133.595265301974,33.0603217062284,29.0161975228328));
#53807=CARTESIAN_POINT('Ctrl Pts',(133.579582536377,33.0317993330807,29.0146027371578));
#53808=CARTESIAN_POINT('Ctrl Pts',(133.522308781787,32.9276350904959,29.0087785499115));
#53809=CARTESIAN_POINT('Ctrl Pts',(133.460392278334,32.8258050587369,29.0029543626652));
#53810=CARTESIAN_POINT('Ctrl Pts',(133.394048002963,32.7267505298394,28.9971301754189));
#53811=CARTESIAN_POINT('Ctrl Pts',(133.327787445879,32.6278209955326,28.9913133375782));
#53812=CARTESIAN_POINT('Ctrl Pts',(133.257110455119,32.5316603341817,28.9854964997374));
#53813=CARTESIAN_POINT('Ctrl Pts',(133.182277960134,32.4386854967721,28.9796796618966));
#53814=CARTESIAN_POINT('Ctrl Pts',(133.107520401396,32.345803763106,28.9738686489585));
#53815=CARTESIAN_POINT('Ctrl Pts',(133.028615871292,32.2561018229628,28.9680576360204));
#53816=CARTESIAN_POINT('Ctrl Pts',(132.945868332009,32.1699673552296,28.9622466230823));
#53817=CARTESIAN_POINT('Ctrl Pts',(132.86000048458,32.0805848624353,28.9562164839784));
#53818=CARTESIAN_POINT('Ctrl Pts',(132.769994341324,31.9950445607963,28.9501863448745));
#53819=CARTESIAN_POINT('Ctrl Pts',(132.676235460261,31.9137419483712,28.9441562057706));
#53820=CARTESIAN_POINT('Ctrl Pts',(132.585985493001,31.8354820755325,28.9383517438303));
#53821=CARTESIAN_POINT('Ctrl Pts',(132.492258968244,31.7611486928278,28.93254728189));
#53822=CARTESIAN_POINT('Ctrl Pts',(132.395436469808,31.6910561928139,28.9267428199497));
#53823=CARTESIAN_POINT('Ctrl Pts',(132.298628356826,31.6209741068308,28.9209392204105));
#53824=CARTESIAN_POINT('Ctrl Pts',(132.198725515535,31.5551318898012,28.9151356208712));
#53825=CARTESIAN_POINT('Ctrl Pts',(132.096139689627,31.4938021445485,28.909332021332));
#53826=CARTESIAN_POINT('Ctrl Pts',(131.993544909283,31.4324670459909,28.9035279152125));
#53827=CARTESIAN_POINT('Ctrl Pts',(131.888267029112,31.3756454118286,28.897723809093));
#53828=CARTESIAN_POINT('Ctrl Pts',(131.780744144132,31.3235648661862,28.8919197029735));
#53829=CARTESIAN_POINT('Ctrl Pts',(131.673186513296,31.2714674907951,28.8861137212659));
#53830=CARTESIAN_POINT('Ctrl Pts',(131.563382802075,31.2241144287547,28.8803077395584));
#53831=CARTESIAN_POINT('Ctrl Pts',(131.45179231755,31.1816857035201,28.8745017578509));
#53832=CARTESIAN_POINT('Ctrl Pts',(131.34007850799,31.1392100878714,28.8686893596204));
#53833=CARTESIAN_POINT('Ctrl Pts',(131.226574365335,31.1016698172517,28.86287696139));
#53834=CARTESIAN_POINT('Ctrl Pts',(131.111755787906,31.0691954935335,28.8570645631596));
#53835=CARTESIAN_POINT('Ctrl Pts',(130.996861934853,31.0366998794891,28.8512483542924));
#53836=CARTESIAN_POINT('Ctrl Pts',(130.880652327236,31.0092769203217,28.8454321454251));
#53837=CARTESIAN_POINT('Ctrl Pts',(130.763612893707,30.9870060617333,28.8396159365578));
#53838=CARTESIAN_POINT('Ctrl Pts',(130.646406108926,30.9647033586978,28.8337914112642));
#53839=CARTESIAN_POINT('Ctrl Pts',(130.528367532529,30.9475675185305,28.8279668859706));
#53840=CARTESIAN_POINT('Ctrl Pts',(130.409988183316,30.9356261626738,28.8221423606769));
#53841=CARTESIAN_POINT('Ctrl Pts',(130.37869503388,30.932469508783,28.8206026686477));
#53842=CARTESIAN_POINT('Ctrl Pts',(130.347378069137,30.929675557665,28.8190629766185));
#53843=CARTESIAN_POINT('Ctrl Pts',(130.316046338524,30.9272442116049,28.8175232845893));
#53844=CARTESIAN_POINT('Ctrl Pts',(130.197522854099,30.9180467749729,28.8116988484452));
#53845=CARTESIAN_POINT('Ctrl Pts',(130.078407074767,30.9140126755592,28.8058744123011));
#53846=CARTESIAN_POINT('Ctrl Pts',(129.959185995004,30.9152038952971,28.8000499761569));
#53847=CARTESIAN_POINT('Ctrl Pts',(129.840114987407,30.9163936155608,28.7942328716504));
#53848=CARTESIAN_POINT('Ctrl Pts',(129.720939347617,30.9227955683593,28.7884157671439));
#53849=CARTESIAN_POINT('Ctrl Pts',(129.602150885732,30.9344199574629,28.7825986626374));
#53850=CARTESIAN_POINT('Ctrl Pts',(129.483481017092,30.9460327412809,28.7767873656756));
#53851=CARTESIAN_POINT('Ctrl Pts',(129.365197961308,30.962857549474,28.7709760687138));
#53852=CARTESIAN_POINT('Ctrl Pts',(129.247792619923,30.9848525484912,28.765164771752));
#53853=CARTESIAN_POINT('Ctrl Pts',(129.125968040959,31.0076754581049,28.7591347325965));
#53854=CARTESIAN_POINT('Ctrl Pts',(129.005088998645,31.0360654235347,28.753104693441));
#53855=CARTESIAN_POINT('Ctrl Pts',(128.885697539091,31.0699166642917,28.7470746542856));
#53856=CARTESIAN_POINT('Ctrl Pts',(128.770765933651,31.1025033958794,28.7412698665429));
#53857=CARTESIAN_POINT('Ctrl Pts',(128.657213194814,31.1401505878394,28.7354650788002));
#53858=CARTESIAN_POINT('Ctrl Pts',(128.545510905086,31.1827121574636,28.7296602910574));
#53859=CARTESIAN_POINT('Ctrl Pts',(128.433824923314,31.225267513319,28.7238563507837));
#53860=CARTESIAN_POINT('Ctrl Pts',(128.323989234738,31.2727356746992,28.7180524105099));
#53861=CARTESIAN_POINT('Ctrl Pts',(128.216457538374,31.3249215943634,28.7122484702361));
#53862=CARTESIAN_POINT('Ctrl Pts',(128.108916185418,31.3771122004423,28.7064440087553));
#53863=CARTESIAN_POINT('Ctrl Pts',(128.003679603309,31.4340212289403,28.7006395472745));
#53864=CARTESIAN_POINT('Ctrl Pts',(127.901178305706,31.4954069429446,28.6948350857936));
#53865=CARTESIAN_POINT('Ctrl Pts',(127.798643633902,31.5568126440047,28.6890287343927));
#53866=CARTESIAN_POINT('Ctrl Pts',(127.698846367849,31.6226977198201,28.6832223829917));
#53867=CARTESIAN_POINT('Ctrl Pts',(127.602188827012,31.6927766058683,28.6774160315907));
#53868=CARTESIAN_POINT('Ctrl Pts',(127.505424146079,31.7629331708897,28.6716032441369));
#53869=CARTESIAN_POINT('Ctrl Pts',(127.411806467881,31.8372925854792,28.6657904566831));
#53870=CARTESIAN_POINT('Ctrl Pts',(127.321705864026,31.9155283238118,28.6599776692293));
#53871=CARTESIAN_POINT('Ctrl Pts',(127.231546010086,31.9938155099036,28.6541610592911));
#53872=CARTESIAN_POINT('Ctrl Pts',(127.144908132067,32.0759838160554,28.6483444493528));
#53873=CARTESIAN_POINT('Ctrl Pts',(127.062125006479,32.1616702935631,28.6425278394146));
#53874=CARTESIAN_POINT('Ctrl Pts',(126.979223314766,32.2474794955207,28.6367028986373));
#53875=CARTESIAN_POINT('Ctrl Pts',(126.900187664572,32.3368166215831,28.6308779578601));
#53876=CARTESIAN_POINT('Ctrl Pts',(126.825310272269,32.4292860655764,28.6250530170828));
#53877=CARTESIAN_POINT('Ctrl Pts',(126.805560500196,32.4536759433008,28.6235166220622));
#53878=CARTESIAN_POINT('Ctrl Pts',(126.78609978188,32.478283584601,28.6219802270415));
#53879=CARTESIAN_POINT('Ctrl Pts',(126.766932963214,32.5031014166276,28.6204438320209));
#53880=CARTESIAN_POINT('Ctrl Pts',(126.694299734928,32.5971493277878,28.6146216174838));
#53881=CARTESIAN_POINT('Ctrl Pts',(126.625652059009,32.6945265269436,28.6087994029467));
#53882=CARTESIAN_POINT('Ctrl Pts',(126.561310074298,32.7948613207151,28.6029771884095));
#53883=CARTESIAN_POINT('Ctrl Pts',(126.497047686161,32.8950719917106,28.5971621764529));
#53884=CARTESIAN_POINT('Ctrl Pts',(126.437080616818,32.9982326428979,28.5913471644963));
#53885=CARTESIAN_POINT('Ctrl Pts',(126.381688619243,33.1039388849808,28.5855321525397));
#53886=CARTESIAN_POINT('Ctrl Pts',(126.326352094297,33.209539266951,28.5797229640596));
#53887=CARTESIAN_POINT('Ctrl Pts',(126.275581717512,33.3176798110937,28.5739137755795));
#53888=CARTESIAN_POINT('Ctrl Pts',(126.229613436349,33.4279280675994,28.5681045870994));
#53889=CARTESIAN_POINT('Ctrl Pts',(126.183680361098,33.5380918878319,28.5622998477258));
#53890=CARTESIAN_POINT('Ctrl Pts',(126.142542221637,33.6503598341763,28.5564951083521));
#53891=CARTESIAN_POINT('Ctrl Pts',(126.106388287917,33.7642763919362,28.5506903689784));
#53892=CARTESIAN_POINT('Ctrl Pts',(126.070251448661,33.8781390871565,28.5448883742277));
#53893=CARTESIAN_POINT('Ctrl Pts',(126.039094251164,33.9936484553415,28.5390863794771));
#53894=CARTESIAN_POINT('Ctrl Pts',(126.013057024121,34.1103311250293,28.5332843847264));
#53895=CARTESIAN_POINT('Ctrl Pts',(125.987027103937,34.2269810499178,28.5274840181966));
#53896=CARTESIAN_POINT('Ctrl Pts',(125.966114381374,34.3448032226732,28.5216836516667));
#53897=CARTESIAN_POINT('Ctrl Pts',(125.950408541689,34.4633119893528,28.5158832851369));
#53898=CARTESIAN_POINT('Ctrl Pts',(125.934700116696,34.5818402635305,28.51008196382));
#53899=CARTESIAN_POINT('Ctrl Pts',(125.924200342196,34.7010549531536,28.5042806425031));
#53900=CARTESIAN_POINT('Ctrl Pts',(125.91894723897,34.8204634808992,28.4984793211861));
#53901=CARTESIAN_POINT('Ctrl Pts',(125.91627169654,34.8812813572605,28.4955245569893));
#53902=CARTESIAN_POINT('Ctrl Pts',(125.914956375683,34.9421494485323,28.4925697927924));
#53903=CARTESIAN_POINT('Ctrl Pts',(125.915001103446,35.0030025246561,28.4896150285955));
#53904=CARTESIAN_POINT('Origin',(-10.,-35.,23.));
#53905=CARTESIAN_POINT('',(-13.3897499995485,-34.9999446770898,27.6441405118761));
#53906=CARTESIAN_POINT('Ctrl Pts',(-13.1787501240208,-33.8227350716437,
28.823527842849));
#53907=CARTESIAN_POINT('Ctrl Pts',(-13.1664347419393,-33.7894821296968,
28.8213937451837));
#53908=CARTESIAN_POINT('Ctrl Pts',(-13.1535988325558,-33.7564258435817,
28.8192323989357));
#53909=CARTESIAN_POINT('Ctrl Pts',(-13.085816098104,-33.5896670296809,28.80814696636));
#53910=CARTESIAN_POINT('Ctrl Pts',(-13.022879052973,-33.4593846333745,28.7988925620819));
#53911=CARTESIAN_POINT('Ctrl Pts',(-12.8184844407376,-33.097339935892,28.7721199648883));
#53912=CARTESIAN_POINT('Ctrl Pts',(-12.6572518256493,-32.8779655398593,
28.7546513287065));
#53913=CARTESIAN_POINT('Ctrl Pts',(-12.4383404821078,-32.6447381700147,
28.7352504188843));
#53914=CARTESIAN_POINT('Ctrl Pts',(-12.4043530459316,-32.6100524293014,
28.7323364318189));
#53915=CARTESIAN_POINT('Ctrl Pts',(-12.3487401089221,-32.5556844553309,
28.7277200690391));
#53916=CARTESIAN_POINT('Ctrl Pts',(-12.327585824062,-32.5355319249923,28.7259976151087));
#53917=CARTESIAN_POINT('Ctrl Pts',(-12.2866215554542,-32.4975055266092,
28.7227245147918));
#53918=CARTESIAN_POINT('Ctrl Pts',(-12.2668560063183,-32.4795872096751,
28.7211720626376));
#53919=CARTESIAN_POINT('Ctrl Pts',(-12.2205463282811,-32.4385910048228,
28.7175950336669));
#53920=CARTESIAN_POINT('Ctrl Pts',(-12.1938501992873,-32.4156889754949,
28.7155777201542));
#53921=CARTESIAN_POINT('Ctrl Pts',(-12.1045830844938,-32.3414889675122,
28.70897249035));
#53922=CARTESIAN_POINT('Ctrl Pts',(-12.0405299715053,-32.2920137210762,
28.7044557148758));
#53923=CARTESIAN_POINT('Ctrl Pts',(-11.8769376434677,-32.1747572331746,
28.6933890627615));
#53924=CARTESIAN_POINT('Ctrl Pts',(-11.7754421846986,-32.1098963324565,
28.6869317737568));
#53925=CARTESIAN_POINT('Ctrl Pts',(-11.4581608150141,-31.9301720579015,
28.6675306025401));
#53926=CARTESIAN_POINT('Ctrl Pts',(-11.233248967079,-31.8331174030263,28.6548425334432));
#53927=CARTESIAN_POINT('Ctrl Pts',(-10.9661423848162,-31.7506582474366,
28.6390527099184));
#53928=CARTESIAN_POINT('Ctrl Pts',(-10.9322295454276,-31.7407668383586,
28.6370344285241));
#53929=CARTESIAN_POINT('Ctrl Pts',(-10.8808352001012,-31.726644292384,28.6339469142761));
#53930=CARTESIAN_POINT('Ctrl Pts',(-10.8634634546689,-31.7220190559795,
28.6328983763595));
#53931=CARTESIAN_POINT('Ctrl Pts',(-10.8315748877775,-31.7137997766585,
28.6309632414602));
#53932=CARTESIAN_POINT('Ctrl Pts',(-10.817069909998,-31.710163311502,28.6300789938724));
#53933=CARTESIAN_POINT('Ctrl Pts',(-10.7832159560899,-31.7019136642517,
28.6280060237918));
#53934=CARTESIAN_POINT('Ctrl Pts',(-10.763849965576,-31.6973746958279,28.6268133578898));
#53935=CARTESIAN_POINT('Ctrl Pts',(-10.6996812680255,-31.6829295177165,
28.6228414746318));
#53936=CARTESIAN_POINT('Ctrl Pts',(-10.6547191234464,-31.6737629527302,
28.620026318491));
#53937=CARTESIAN_POINT('Ctrl Pts',(-10.5425860673905,-31.6532635887739,
28.6129485295212));
#53938=CARTESIAN_POINT('Ctrl Pts',(-10.4752342145489,-31.6430377202951,
28.6086471784615));
#53939=CARTESIAN_POINT('Ctrl Pts',(-10.1120966137231,-31.599050548723,28.5853323537151));
#53940=CARTESIAN_POINT('Ctrl Pts',(-9.8130786471456,-31.6023342153103,28.5658500816704));
#53941=CARTESIAN_POINT('Ctrl Pts',(-9.4496437434001,-31.6545063114903,28.5432592343292));
#53942=CARTESIAN_POINT('Ctrl Pts',(-9.38127345527458,-31.6664735580105,
28.5390494595316));
#53943=CARTESIAN_POINT('Ctrl Pts',(-9.2807563734005,-31.6872671276796,28.5329178761918));
#53944=CARTESIAN_POINT('Ctrl Pts',(-9.24829796176518,-31.6944811842009,
28.5309467941138));
#53945=CARTESIAN_POINT('Ctrl Pts',(-9.19020673427615,-31.7082922203206,
28.5274339545297));
#53946=CARTESIAN_POINT('Ctrl Pts',(-9.16453544904484,-31.7147139724268,
28.5258868258147));
#53947=CARTESIAN_POINT('Ctrl Pts',(-9.10964819946747,-31.7291291655765,
28.5225891741485));
#53948=CARTESIAN_POINT('Ctrl Pts',(-9.08045873089549,-31.7372149497202,
28.5208417308572));
#53949=CARTESIAN_POINT('Ctrl Pts',(-8.99971853060223,-31.7607504226347,
28.5160230464574));
#53950=CARTESIAN_POINT('Ctrl Pts',(-8.94842032282783,-31.7770384009335,
28.512978596222));
#53951=CARTESIAN_POINT('Ctrl Pts',(-8.72526038916927,-31.8537909843778,
28.4997792099716));
#53952=CARTESIAN_POINT('Ctrl Pts',(-8.55804144064753,-31.926832853801,28.4900265194022));
#53953=CARTESIAN_POINT('Ctrl Pts',(-8.2094493043554,-32.1138486150595,28.4690274416487));
#53954=CARTESIAN_POINT('Ctrl Pts',(-8.03137366801509,-32.2322511425002,
28.4578582595488));
#53955=CARTESIAN_POINT('Ctrl Pts',(-7.83560566151058,-32.3909205510743,
28.4437285522146));
#53956=CARTESIAN_POINT('Ctrl Pts',(-7.80600363805133,-32.4157635299367,
28.4415360098675));
#53957=CARTESIAN_POINT('Ctrl Pts',(-7.76256052289224,-32.4535068891171,
28.4382227911626));
#53958=CARTESIAN_POINT('Ctrl Pts',(-7.74839133873374,-32.4660266420265,
28.4371265850077));
#53959=CARTESIAN_POINT('Ctrl Pts',(-7.72304488023586,-32.4888029641643,
28.4351357902192));
#53960=CARTESIAN_POINT('Ctrl Pts',(-7.71183010523102,-32.4990174538065,
28.434244187484));
#53961=CARTESIAN_POINT('Ctrl Pts',(-7.68852743559765,-32.5205296158759,
28.4323681017364));
#53962=CARTESIAN_POINT('Ctrl Pts',(-7.67645319261137,-32.5318409673775,
28.4313826781284));
#53963=CARTESIAN_POINT('Ctrl Pts',(-7.64386740223262,-32.5628188953921,
28.4286879622769));
#53964=CARTESIAN_POINT('Ctrl Pts',(-7.62352001762466,-32.5826553135429,
28.4269667644949));
#53965=CARTESIAN_POINT('Ctrl Pts',(-7.49095166150049,-32.7151860271487,
28.4155098764389));
#53966=CARTESIAN_POINT('Ctrl Pts',(-7.38654065519599,-32.8353939064203,
28.4053276982853));
#53967=CARTESIAN_POINT('Ctrl Pts',(-7.1294576219205,-33.1772041027171,28.3777820827545));
#53968=CARTESIAN_POINT('Ctrl Pts',(-6.9940278645292,-33.4104163243334,28.3604840768473));
#53969=CARTESIAN_POINT('Ctrl Pts',(-6.86818528590019,-33.7021043720864,
28.3412107000448));
#53970=CARTESIAN_POINT('Ctrl Pts',(-6.8497867398924,-33.7474213582024,28.3382752064751));
#53971=CARTESIAN_POINT('Ctrl Pts',(-6.821949819122,-33.820483401488,28.3336337200535));
#53972=CARTESIAN_POINT('Ctrl Pts',(-6.81187988924761,-33.8479789071961,
28.3319072409461));
#53973=CARTESIAN_POINT('Ctrl Pts',(-6.79332876434943,-33.9007390510442,
28.3286318459368));
#53974=CARTESIAN_POINT('Ctrl Pts',(-6.78478681449628,-33.9259798517561,
28.3270810492658));
#53975=CARTESIAN_POINT('Ctrl Pts',(-6.7657166710736,-33.9845980595745,28.3235155446851));
#53976=CARTESIAN_POINT('Ctrl Pts',(-6.75540588451315,-34.0180433268239,
28.3215079593414));
#53977=CARTESIAN_POINT('Ctrl Pts',(-6.72327730335093,-34.1282959067011,
28.3149720740905));
#53978=CARTESIAN_POINT('Ctrl Pts',(-6.70365412882489,-34.205717375016,28.3105128326565));
#53979=CARTESIAN_POINT('Ctrl Pts',(-6.66185766426764,-34.399062555541,28.2996307381464));
#53980=CARTESIAN_POINT('Ctrl Pts',(-6.6429674047542,-34.515588303047,28.293296213856));
#53981=CARTESIAN_POINT('Ctrl Pts',(-6.60310749272352,-34.8814508267982,
28.2737057227833));
#53982=CARTESIAN_POINT('Ctrl Pts',(-6.60361725714158,-35.1322368507821,
28.2607399063069));
#53983=CARTESIAN_POINT('Ctrl Pts',(-6.63549774844189,-35.4143420090158,
28.2446869956881));
#53984=CARTESIAN_POINT('Ctrl Pts',(-6.63981038557455,-35.4479735188258,
28.2427484127442));
#53985=CARTESIAN_POINT('Ctrl Pts',(-6.64716905914354,-35.4992495088584,
28.2397471785014));
#53986=CARTESIAN_POINT('Ctrl Pts',(-6.64985173843999,-35.5169448564233,
28.2387031183569));
#53987=CARTESIAN_POINT('Ctrl Pts',(-6.65503356128081,-35.5493890656727,
28.2367721788914));
#53988=CARTESIAN_POINT('Ctrl Pts',(-6.65749037941416,-35.5641438026397,
28.2358875785823));
#53989=CARTESIAN_POINT('Ctrl Pts',(-6.66345765598603,-35.5985730059391,
28.2338085276069));
#53990=CARTESIAN_POINT('Ctrl Pts',(-6.66704453521932,-35.6182331953278,
28.2326100459078));
#53991=CARTESIAN_POINT('Ctrl Pts',(-6.67954720466424,-35.683488621804,28.2285971216631));
#53992=CARTESIAN_POINT('Ctrl Pts',(-6.68922614790436,-35.7289303884995,
28.22574575664));
#53993=CARTESIAN_POINT('Ctrl Pts',(-6.71566829159229,-35.8416510562581,
28.2185538255722));
#53994=CARTESIAN_POINT('Ctrl Pts',(-6.73356735854304,-35.9086407933472,
28.214173060421));
#53995=CARTESIAN_POINT('Ctrl Pts',(-6.84517293719294,-36.2802461910706,
28.1894291968761));
#53996=CARTESIAN_POINT('Ctrl Pts',(-6.97945000499741,-36.5710859836512,
28.1685799872428));
#53997=CARTESIAN_POINT('Ctrl Pts',(-7.18196389076624,-36.8846881545117,
28.1458237051035));
#53998=CARTESIAN_POINT('Ctrl Pts',(-7.21263918001192,-36.9297660808519,
28.1425389127532));
#53999=CARTESIAN_POINT('Ctrl Pts',(-7.26229310237735,-36.9990775583663,
28.1374642901982));
#54000=CARTESIAN_POINT('Ctrl Pts',(-7.28053594663425,-37.0238244729718,
28.1356474544839));
#54001=CARTESIAN_POINT('Ctrl Pts',(-7.31507781192188,-37.0693708927981,
28.1322931276101));
#54002=CARTESIAN_POINT('Ctrl Pts',(-7.33128811514864,-37.090234432301,28.1307524030424));
#54003=CARTESIAN_POINT('Ctrl Pts',(-7.36805899127428,-37.136435376639,28.1273299518131));
#54004=CARTESIAN_POINT('Ctrl Pts',(-7.38874495738245,-37.161669910167,28.1254533369255));
#54005=CARTESIAN_POINT('Ctrl Pts',(-7.45232472404222,-37.2369852839618,
28.1198262986822));
#54006=CARTESIAN_POINT('Ctrl Pts',(-7.4963195580903,-37.2861184359444,28.1161200621157));
#54007=CARTESIAN_POINT('Ctrl Pts',(-7.60328320952698,-37.3987804986427,
28.1075033630551));
#54008=CARTESIAN_POINT('Ctrl Pts',(-7.66738850552402,-37.4611631984061,
28.1026378628716));
#54009=CARTESIAN_POINT('Ctrl Pts',(-7.83832518800311,-37.6148207464233,
28.0902757237925));
#54010=CARTESIAN_POINT('Ctrl Pts',(-7.94849654350741,-37.7021213735162,
28.0828776112622));
#54011=CARTESIAN_POINT('Ctrl Pts',(-8.20191219381496,-37.8784739635882,
28.0664724638875));
#54012=CARTESIAN_POINT('Ctrl Pts',(-8.34701326926217,-37.9641785485708,
28.0574602499881));
#54013=CARTESIAN_POINT('Ctrl Pts',(-8.52358290915223,-38.051462123326,28.0462496381849));
#54014=CARTESIAN_POINT('Ctrl Pts',(-8.54946691244673,-38.0638508715059,
28.0446002030662));
#54015=CARTESIAN_POINT('Ctrl Pts',(-8.59057299499792,-38.0828876642906,
28.0419665171148));
#54016=CARTESIAN_POINT('Ctrl Pts',(-8.60569256655494,-38.0897552635778,
28.0409947958848));
#54017=CARTESIAN_POINT('Ctrl Pts',(-8.63485571349489,-38.1027440791559,
28.0391136219904));
#54018=CARTESIAN_POINT('Ctrl Pts',(-8.64889127286791,-38.108881618297,28.0382051265547));
#54019=CARTESIAN_POINT('Ctrl Pts',(-8.68366834833717,-38.1238091365963,
28.0359471032101));
#54020=CARTESIAN_POINT('Ctrl Pts',(-8.70445663342249,-38.132487807545,28.034591307251));
#54021=CARTESIAN_POINT('Ctrl Pts',(-8.78486662299587,-38.1651199693079,
28.0293281096639));
#54022=CARTESIAN_POINT('Ctrl Pts',(-8.84507517890134,-38.1875823311257,
28.0253475628698));
#54023=CARTESIAN_POINT('Ctrl Pts',(-9.01305746573739,-38.2448685785511,
28.01420063812));
#54024=CARTESIAN_POINT('Ctrl Pts',(-9.12199280763895,-38.2760232947801,
28.0069281239153));
#54025=CARTESIAN_POINT('Ctrl Pts',(-9.48522498506772,-38.3604841774746,
27.9829007361708));
#54026=CARTESIAN_POINT('Ctrl Pts',(-9.74413799887095,-38.3900477324314,
27.9662071153393));
#54027=CARTESIAN_POINT('Ctrl Pts',(-10.0540330706947,-38.3896898622973,
27.9473877283307));
#54028=CARTESIAN_POINT('Ctrl Pts',(-10.1041460406995,-38.3885204646458,
27.9443769768559));
#54029=CARTESIAN_POINT('Ctrl Pts',(-10.1837181311802,-38.3848965786457,
27.9396460148026));
#54030=CARTESIAN_POINT('Ctrl Pts',(-10.2132013754226,-38.3831675181686,
27.937903914336));
#54031=CARTESIAN_POINT('Ctrl Pts',(-10.2691769407077,-38.3791501389735,
27.9346160004409));
#54032=CARTESIAN_POINT('Ctrl Pts',(-10.2956721313698,-38.3769349915463,
27.9330680621092));
#54033=CARTESIAN_POINT('Ctrl Pts',(-10.3564852158984,-38.3711294488342,
27.9295331155057));
#54034=CARTESIAN_POINT('Ctrl Pts',(-10.3907801338895,-38.3673263105263,
27.9275528074438));
#54035=CARTESIAN_POINT('Ctrl Pts',(-10.5011727091637,-38.3533750288404,
27.921216074775));
#54036=CARTESIAN_POINT('Ctrl Pts',(-10.5769879324629,-38.3411651099419,
27.9169227465679));
#54037=CARTESIAN_POINT('Ctrl Pts',(-10.7614770837294,-38.3049855625242,
27.9065624743554));
#54038=CARTESIAN_POINT('Ctrl Pts',(-10.86951169189,-38.2782203349786,27.9005722860236));
#54039=CARTESIAN_POINT('Ctrl Pts',(-11.1859260865101,-38.1830832972969,
27.882951953015));
#54040=CARTESIAN_POINT('Ctrl Pts',(-11.3891806596632,-38.0997746908322,
27.8715545986186));
#54041=CARTESIAN_POINT('Ctrl Pts',(-11.6385461628331,-37.9680841716859,
27.8560008211231));
#54042=CARTESIAN_POINT('Ctrl Pts',(-11.6933054711164,-37.9371879023392,
27.8524775299477));
#54043=CARTESIAN_POINT('Ctrl Pts',(-11.7668766783237,-37.892936343102,27.8475515907463));
#54044=CARTESIAN_POINT('Ctrl Pts',(-11.7864610685216,-37.8808836613223,
27.8462211614423));
#54045=CARTESIAN_POINT('Ctrl Pts',(-11.8188283880511,-37.8605071219958,
27.8439876874902));
#54046=CARTESIAN_POINT('Ctrl Pts',(-11.8316808914577,-37.8522943052936,
27.843091576731));
#54047=CARTESIAN_POINT('Ctrl Pts',(-11.8582286660767,-37.8350767043949,
27.8412204692755));
#54048=CARTESIAN_POINT('Ctrl Pts',(-11.8719146905146,-37.8260589275569,
27.8402447020276));
#54049=CARTESIAN_POINT('Ctrl Pts',(-11.9085456035975,-37.8015398435209,
27.8376040333474));
#54050=CARTESIAN_POINT('Ctrl Pts',(-11.9313663563749,-37.7858563685581,
27.8359279845345));
#54051=CARTESIAN_POINT('Ctrl Pts',(-12.0634906679487,-37.6926507652265,
27.826054018356));
#54052=CARTESIAN_POINT('Ctrl Pts',(-12.1683034294526,-37.6089874577042,
27.8175367606907));
#54053=CARTESIAN_POINT('Ctrl Pts',(-12.4839926721803,-37.324808943195,27.7902588940564));
#54054=CARTESIAN_POINT('Ctrl Pts',(-12.67421994575,-37.1032261240233,27.7714091509572));
#54055=CARTESIAN_POINT('Ctrl Pts',(-12.8619574118325,-36.8172044970381,
27.7506137814449));
#54056=CARTESIAN_POINT('Ctrl Pts',(-12.8891095031233,-36.7737190080863,
27.7475325195256));
#54057=CARTESIAN_POINT('Ctrl Pts',(-12.9304541467555,-36.7040333202694,
27.7427179377951));
#54058=CARTESIAN_POINT('Ctrl Pts',(-12.9453047393154,-36.6782345306933,
27.7409613767008));
#54059=CARTESIAN_POINT('Ctrl Pts',(-12.9727492137851,-36.6290707297088,
27.7376614990967));
#54060=CARTESIAN_POINT('Ctrl Pts',(-12.9854121699783,-36.6057470425886,
27.7361158348853));
#54061=CARTESIAN_POINT('Ctrl Pts',(-13.0137066887149,-36.5521399070339,
27.7326070554025));
#54062=CARTESIAN_POINT('Ctrl Pts',(-13.0291582335005,-36.5217643750974,
27.730650279473));
#54063=CARTESIAN_POINT('Ctrl Pts',(-13.0767917358651,-36.424522305688,27.7244804309158));
#54064=CARTESIAN_POINT('Ctrl Pts',(-13.1072384853675,-36.3568276497573,
27.7203256902728));
#54065=CARTESIAN_POINT('Ctrl Pts',(-13.1756517811604,-36.1903097389848,
27.7103905806528));
#54066=CARTESIAN_POINT('Ctrl Pts',(-13.2112600960353,-36.0906017298781,
27.7046782686266));
#54067=CARTESIAN_POINT('Ctrl Pts',(-13.3039133994116,-35.7869837233182,
27.6877200675271));
#54068=CARTESIAN_POINT('Ctrl Pts',(-13.346586441733,-35.5792549246931,27.6767111850404));
#54069=CARTESIAN_POINT('Ctrl Pts',(-13.377918515725,-35.2930745769432,27.6609627759639));
#54070=CARTESIAN_POINT('Ctrl Pts',(-13.3836585457924,-35.2169778751103,
27.6567169058938));
#54071=CARTESIAN_POINT('Ctrl Pts',(-13.3878253891392,-35.1167180987123,
27.6509730333547));
#54072=CARTESIAN_POINT('Ctrl Pts',(-13.3885684869205,-35.0926688788554,
27.6495839276084));
#54073=CARTESIAN_POINT('Ctrl Pts',(-13.389334991484,-35.0548091612999,27.6473764827574));
#54074=CARTESIAN_POINT('Ctrl Pts',(-13.3895301311732,-35.0410024856843,
27.6465671551311));
#54075=CARTESIAN_POINT('Ctrl Pts',(-13.3897137852033,-35.0181116961334,
27.6452176133072));
#54076=CARTESIAN_POINT('Ctrl Pts',(-13.389750147796,-35.0090281067772,27.644680047935));
#54077=CARTESIAN_POINT('Ctrl Pts',(-13.3897499995485,-34.9999446770898,
27.6441405118761));
#54078=CARTESIAN_POINT('Ctrl Pts',(-13.3897499995572,-34.999945207804,27.6441405433994));
#54079=CARTESIAN_POINT('Ctrl Pts',(-13.3897499123749,-34.994551631023,27.6438201766608));
#54080=CARTESIAN_POINT('Ctrl Pts',(-13.3897369522656,-34.989158097162,27.6434991162569));
#54081=CARTESIAN_POINT('Ctrl Pts',(-13.3896571545376,-34.9724974592523,
27.6425052569258));
#54082=CARTESIAN_POINT('Ctrl Pts',(-13.3895470131806,-34.9612307753627,
27.6418301927998));
#54083=CARTESIAN_POINT('Ctrl Pts',(-13.3888739786967,-34.9156392667992,
27.639087033885));
#54084=CARTESIAN_POINT('Ctrl Pts',(-13.3878458534473,-34.8813245789518,
27.6369961020113));
#54085=CARTESIAN_POINT('Ctrl Pts',(-13.3760246063147,-34.6196327011655,
27.6208789136258));
#54086=CARTESIAN_POINT('Ctrl Pts',(-13.3428736881132,-34.3938588597364,
27.6060295639237));
#54087=CARTESIAN_POINT('Ctrl Pts',(-13.2574968510191,-34.0544322309172,
27.583549957105));
#54088=CARTESIAN_POINT('Ctrl Pts',(-13.2212412264666,-33.9374659252775,
27.5757646113467));
#54089=CARTESIAN_POINT('Ctrl Pts',(-13.1787501609633,-33.8227351713926,
27.5681448070208));
#54090=CARTESIAN_POINT('',(-13.3897486873357,-35.0029831537265,27.9839821967052));
#54091=CARTESIAN_POINT('Ctrl Pts',(-13.1787501240207,-33.8227350716434,
27.9134187994658));
#54092=CARTESIAN_POINT('Ctrl Pts',(-13.2144036035584,-33.9190035493433,
27.9194227889449));
#54093=CARTESIAN_POINT('Ctrl Pts',(-13.2456876111846,-34.016914363963,27.925426778424));
#54094=CARTESIAN_POINT('Ctrl Pts',(-13.2724607141584,-34.1160283167489,
27.9314307679031));
#54095=CARTESIAN_POINT('Ctrl Pts',(-13.2992340062708,-34.2151429697253,
27.9374347997973));
#54096=CARTESIAN_POINT('Ctrl Pts',(-13.3214962229816,-34.3154603506665,
27.9434388316916));
#54097=CARTESIAN_POINT('Ctrl Pts',(-13.3391564678312,-34.4165283675782,
27.9494428635859));
#54098=CARTESIAN_POINT('Ctrl Pts',(-13.3568326196948,-34.5176874189217,
27.9554523034583));
#54099=CARTESIAN_POINT('Ctrl Pts',(-13.3698984504733,-34.6195980214031,
27.9614617433308));
#54100=CARTESIAN_POINT('Ctrl Pts',(-13.3783146793759,-34.7218004500127,
27.9674711832033));
#54101=CARTESIAN_POINT('Ctrl Pts',(-13.3860225785033,-34.8154012799579,
27.9729748543706));
#54102=CARTESIAN_POINT('Ctrl Pts',(-13.3898311803767,-34.9092465570969,
27.9784785255379));
#54103=CARTESIAN_POINT('Ctrl Pts',(-13.3897486873357,-35.0029831537265,
27.9839821967052));
#54104=CARTESIAN_POINT('Ctrl Pts',(-13.1787501097524,-33.8227350331175,
29.1634929519179));
#54105=CARTESIAN_POINT('Ctrl Pts',(-13.1341008506572,-33.7021769249243,
29.1566764597228));
#54106=CARTESIAN_POINT('Ctrl Pts',(-13.0826222281607,-33.5842375125987,
29.1498322043012));
#54107=CARTESIAN_POINT('Ctrl Pts',(-12.9813983847272,-33.3842011618824,
29.1376014467608));
#54108=CARTESIAN_POINT('Ctrl Pts',(-12.9346538431717,-33.3007805148027,
29.1322993107299));
#54109=CARTESIAN_POINT('Ctrl Pts',(-12.8649298389742,-33.1878291933825,
29.1247662346228));
#54110=CARTESIAN_POINT('Ctrl Pts',(-12.8448919349152,-33.1565316009532,
29.122639606394));
#54111=CARTESIAN_POINT('Ctrl Pts',(-12.8094979716464,-33.1032008479741,
29.1189440686014));
#54112=CARTESIAN_POINT('Ctrl Pts',(-12.7943869442591,-33.081008749247,29.1173842923023));
#54113=CARTESIAN_POINT('Ctrl Pts',(-12.7628792651954,-33.0358978577039,
29.1141670656781));
#54114=CARTESIAN_POINT('Ctrl Pts',(-12.7464572799425,-33.0129993968743,
29.1125087344198));
#54115=CARTESIAN_POINT('Ctrl Pts',(-12.7036125563011,-32.9548036521409,
29.1082275071958));
#54116=CARTESIAN_POINT('Ctrl Pts',(-12.6767837881576,-32.9198131740124,
29.1055891568768));
#54117=CARTESIAN_POINT('Ctrl Pts',(-12.5489175186532,-32.7596188946876,
29.0932021646422));
#54118=CARTESIAN_POINT('Ctrl Pts',(-12.4397427093475,-32.6412011765305,
29.0831355219448));
#54119=CARTESIAN_POINT('Ctrl Pts',(-12.1783550529947,-32.3953146486059,
29.0602212240801));
#54120=CARTESIAN_POINT('Ctrl Pts',(-12.02251638337,-32.2725392724793,29.0473038315074));
#54121=CARTESIAN_POINT('Ctrl Pts',(-11.7843267739212,-32.116582171182,29.029231915516));
#54122=CARTESIAN_POINT('Ctrl Pts',(-11.7099982471548,-32.0718898943673,
29.0238068675787));
#54123=CARTESIAN_POINT('Ctrl Pts',(-11.6123434904894,-32.0181605779497,
29.0170234316381));
#54124=CARTESIAN_POINT('Ctrl Pts',(-11.5905238328035,-32.0064649849654,
29.0155291669482));
#54125=CARTESIAN_POINT('Ctrl Pts',(-11.5546677528406,-31.9877484444146,
29.013110821397));
#54126=CARTESIAN_POINT('Ctrl Pts',(-11.540707522233,-31.9805842258255,29.0121783507766));
#54127=CARTESIAN_POINT('Ctrl Pts',(-11.5124988338076,-31.9663544625593,
29.0103131445429));
#54128=CARTESIAN_POINT('Ctrl Pts',(-11.498249521214,-31.9592917989708,29.009380558242));
#54129=CARTESIAN_POINT('Ctrl Pts',(-11.4610961217925,-31.9412013216437,
29.0069724723049));
#54130=CARTESIAN_POINT('Ctrl Pts',(-11.4381163447554,-31.9303301980402,
29.0055060924296));
#54131=CARTESIAN_POINT('Ctrl Pts',(-11.3372728856087,-31.8840048638483,
28.9991619815716));
#54132=CARTESIAN_POINT('Ctrl Pts',(-11.2581997154204,-31.8512446629565,
28.9944217215085));
#54133=CARTESIAN_POINT('Ctrl Pts',(-10.9923698373936,-31.7527266557703,
28.9789895680065));
#54134=CARTESIAN_POINT('Ctrl Pts',(-10.8010989965715,-31.7003288552688,
28.9686679209581));
#54135=CARTESIAN_POINT('Ctrl Pts',(-10.4494790577306,-31.6364018067372,
28.9495863238047));
#54136=CARTESIAN_POINT('Ctrl Pts',(-10.2908154804733,-31.6189878608985,
28.9409405588369));
#54137=CARTESIAN_POINT('Ctrl Pts',(-10.0873587375544,-31.6110876188855,
28.9294613717095));
#54138=CARTESIAN_POINT('Ctrl Pts',(-10.0431645338026,-31.6102366977027,
28.9269453096083));
#54139=CARTESIAN_POINT('Ctrl Pts',(-9.97061668238919,-31.6102587910637,
28.9227721034821));
#54140=CARTESIAN_POINT('Ctrl Pts',(-9.94226753781605,-31.6106231052204,
28.9211306243353));
#54141=CARTESIAN_POINT('Ctrl Pts',(-9.88683934256462,-31.6120310010794,
28.9178987971465));
#54142=CARTESIAN_POINT('Ctrl Pts',(-9.8597616093796,-31.6130437849761,28.9163095181377));
#54143=CARTESIAN_POINT('Ctrl Pts',(-9.79508590705522,-31.6162397375263,
28.9124873169503));
#54144=CARTESIAN_POINT('Ctrl Pts',(-9.75750709968905,-31.6187250449724,
28.9102452928013));
#54145=CARTESIAN_POINT('Ctrl Pts',(-9.62219673189963,-31.6299411367559,
28.902092987353));
#54146=CARTESIAN_POINT('Ctrl Pts',(-9.52482100973745,-31.642287366852,28.8960746481012));
#54147=CARTESIAN_POINT('Ctrl Pts',(-9.26544890108731,-31.6866816681431,
28.8796442261479));
#54148=CARTESIAN_POINT('Ctrl Pts',(-9.10503606589438,-31.7263666729971,
28.869047553));
#54149=CARTESIAN_POINT('Ctrl Pts',(-8.78242321748637,-31.8316709683176,
28.8471835559908));
#54150=CARTESIAN_POINT('Ctrl Pts',(-8.62109019404132,-31.8984812166077,
28.8359450909284));
#54151=CARTESIAN_POINT('Ctrl Pts',(-8.43387832991036,-31.9935180171217,
28.8230211210226));
#54152=CARTESIAN_POINT('Ctrl Pts',(-8.40240636232595,-32.0101227813293,
28.8208532698331));
#54153=CARTESIAN_POINT('Ctrl Pts',(-8.35536484955722,-32.0358970450037,
28.8176266623488));
#54154=CARTESIAN_POINT('Ctrl Pts',(-8.33959850175203,-32.0447000147807,
28.8165476025892));
#54155=CARTESIAN_POINT('Ctrl Pts',(-8.31088376206896,-32.0610349193159,
28.8145877414521));
#54156=CARTESIAN_POINT('Ctrl Pts',(-8.29791428321023,-32.0685270535017,
28.8137046864572));
#54157=CARTESIAN_POINT('Ctrl Pts',(-8.26784417326212,-32.0861646297984,
28.811661946619));
#54158=CARTESIAN_POINT('Ctrl Pts',(-8.2507825991845,-32.0963748694272,28.8105063123233));
#54159=CARTESIAN_POINT('Ctrl Pts',(-8.19474583146499,-32.1305824158147,
28.8067187287056));
#54160=CARTESIAN_POINT('Ctrl Pts',(-8.15616527750445,-32.1552198993775,
28.8041238623235));
#54161=CARTESIAN_POINT('Ctrl Pts',(-8.06165523712683,-32.2183046290798,
28.797769234912));
#54162=CARTESIAN_POINT('Ctrl Pts',(-8.00635778306566,-32.2576650105475,
28.7940528068173));
#54163=CARTESIAN_POINT('Ctrl Pts',(-7.71815124300348,-32.4761371130312,
28.7744870534131));
#54164=CARTESIAN_POINT('Ctrl Pts',(-7.50809522385788,-32.6832915669291,
28.7594036472472));
#54165=CARTESIAN_POINT('Ctrl Pts',(-7.28298630627063,-32.9718361012953,
28.7391812061063));
#54166=CARTESIAN_POINT('Ctrl Pts',(-7.24043029172502,-33.0301304032548,
28.7351372438304));
#54167=CARTESIAN_POINT('Ctrl Pts',(-7.18075567495961,-33.1176066325867,
28.7291006171509));
#54168=CARTESIAN_POINT('Ctrl Pts',(-7.16216026879386,-33.1457592127428,
28.72716256565));
#54169=CARTESIAN_POINT('Ctrl Pts',(-7.129707135741,-33.196523646232,28.7236737431847));
#54170=CARTESIAN_POINT('Ctrl Pts',(-7.11568854195321,-33.2190296354606,
28.722129013886));
#54171=CARTESIAN_POINT('Ctrl Pts',(-7.0863786463198,-33.2673387021508,28.7188163836387));
#54172=CARTESIAN_POINT('Ctrl Pts',(-7.07116297257799,-33.2931847944357,
28.7170459364889));
#54173=CARTESIAN_POINT('Ctrl Pts',(-7.03035050290647,-33.3646638671613,
28.7121531846486));
#54174=CARTESIAN_POINT('Ctrl Pts',(-7.00546493573918,-33.4106914410072,
28.7090063679964));
#54175=CARTESIAN_POINT('Ctrl Pts',(-6.90412754409968,-33.6089582018583,
28.6954613785215));
#54176=CARTESIAN_POINT('Ctrl Pts',(-6.8381532885114,-33.7662512326336,28.6847234058602));
#54177=CARTESIAN_POINT('Ctrl Pts',(-6.72464210624342,-34.106696775112,28.6617145854371));
#54178=CARTESIAN_POINT('Ctrl Pts',(-6.68002961627969,-34.2902406705934,
28.6494403593251));
#54179=CARTESIAN_POINT('Ctrl Pts',(-6.63989810842761,-34.5470030944697,
28.6330502692425));
#54180=CARTESIAN_POINT('Ctrl Pts',(-6.63111087840936,-34.6177979345041,
28.6286139039283));
#54181=CARTESIAN_POINT('Ctrl Pts',(-6.62235577805131,-34.7127669700333,
28.6228166986049));
#54182=CARTESIAN_POINT('Ctrl Pts',(-6.62040309298162,-34.736735642969,28.6213666593028));
#54183=CARTESIAN_POINT('Ctrl Pts',(-6.61771264564724,-34.7747552808034,
28.6190894204333));
#54184=CARTESIAN_POINT('Ctrl Pts',(-6.61680704249519,-34.7887930896588,
28.6182535348629));
#54185=CARTESIAN_POINT('Ctrl Pts',(-6.61507624842204,-34.8184995194161,
28.6164956566593));
#54186=CARTESIAN_POINT('Ctrl Pts',(-6.61427240748996,-34.8341690214957,
28.6155749141646));
#54187=CARTESIAN_POINT('Ctrl Pts',(-6.61249405559459,-34.8742755966487,
28.6132336131238));
#54188=CARTESIAN_POINT('Ctrl Pts',(-6.61167513142788,-34.8987191630877,
28.6118212541202));
#54189=CARTESIAN_POINT('Ctrl Pts',(-6.60925421008101,-35.0055033773342,
28.605706686524));
#54190=CARTESIAN_POINT('Ctrl Pts',(-6.61038854584917,-35.0878836361065,
28.6011332281708));
#54191=CARTESIAN_POINT('Ctrl Pts',(-6.62343024225929,-35.3473797153306,
28.5869589228742));
#54192=CARTESIAN_POINT('Ctrl Pts',(-6.64624164788816,-35.5236479487111,
28.5776606781066));
#54193=CARTESIAN_POINT('Ctrl Pts',(-6.72047610361767,-35.8767883349627,
28.5584740101881));
#54194=CARTESIAN_POINT('Ctrl Pts',(-6.77269752704192,-36.0528739573895,
28.5486025110094));
#54195=CARTESIAN_POINT('Ctrl Pts',(-6.85507095372378,-36.265635354014,28.5357479975101));
#54196=CARTESIAN_POINT('Ctrl Pts',(-6.87206954965174,-36.3070816308171,
28.5331994250152));
#54197=CARTESIAN_POINT('Ctrl Pts',(-6.90118750153499,-36.374253946467,28.5289895089035));
#54198=CARTESIAN_POINT('Ctrl Pts',(-6.91281835599816,-36.4001865002447,
28.5273445186338));
#54199=CARTESIAN_POINT('Ctrl Pts',(-6.93610801114565,-36.4504126634799,
28.5241184661231));
#54200=CARTESIAN_POINT('Ctrl Pts',(-6.9477331276999,-36.4747195976138,28.5225386408883));
#54201=CARTESIAN_POINT('Ctrl Pts',(-6.97604373195173,-36.5321451187126,
28.5187607463818));
#54202=CARTESIAN_POINT('Ctrl Pts',(-6.9929850987164,-36.5651330280031,28.516554016426));
#54203=CARTESIAN_POINT('Ctrl Pts',(-7.05484667928038,-36.6808755104915,
28.5086782201529));
#54204=CARTESIAN_POINT('Ctrl Pts',(-7.10266663729085,-36.7620236677082,
28.5029101450212));
#54205=CARTESIAN_POINT('Ctrl Pts',(-7.23715489530556,-36.969935621708,28.4874737473239));
#54206=CARTESIAN_POINT('Ctrl Pts',(-7.3291601632739,-37.0929803967567,28.4776485274617));
#54207=CARTESIAN_POINT('Ctrl Pts',(-7.55541247795924,-37.3562489256483,
28.4552818605003));
#54208=CARTESIAN_POINT('Ctrl Pts',(-7.69401412460238,-37.4920586855317,
28.4427375133697));
#54209=CARTESIAN_POINT('Ctrl Pts',(-7.87019009517371,-37.6373309861613,
28.428684892285));
#54210=CARTESIAN_POINT('Ctrl Pts',(-7.89725291093571,-37.65895841271,28.4265745383328));
#54211=CARTESIAN_POINT('Ctrl Pts',(-7.93891017733314,-37.691215223772,28.4234046817938));
#54212=CARTESIAN_POINT('Ctrl Pts',(-7.95326509800031,-37.7021485730608,
28.4223262128984));
#54213=CARTESIAN_POINT('Ctrl Pts',(-7.97966099617803,-37.721921831851,28.4203693311496));
#54214=CARTESIAN_POINT('Ctrl Pts',(-7.99167367271867,-37.7307972322945,
28.419488637862));
#54215=CARTESIAN_POINT('Ctrl Pts',(-8.01971669637135,-37.7512312923336,
28.4174551325651));
#54216=CARTESIAN_POINT('Ctrl Pts',(-8.03578995516797,-37.7627295428876,
28.4163062980315));
#54217=CARTESIAN_POINT('Ctrl Pts',(-8.08888515917287,-37.8000143910725,
28.4125625485804));
#54218=CARTESIAN_POINT('Ctrl Pts',(-8.12632284978902,-37.8252035086741,
28.4100036156142));
#54219=CARTESIAN_POINT('Ctrl Pts',(-8.22016284563578,-37.8856555154309,
28.4037577383386));
#54220=CARTESIAN_POINT('Ctrl Pts',(-8.27712235126746,-37.9200208119295,
28.40011230084));
#54221=CARTESIAN_POINT('Ctrl Pts',(-8.57418272803949,-38.0875250714524,
28.3816478870716));
#54222=CARTESIAN_POINT('Ctrl Pts',(-8.82879785374734,-38.1928139604689,
28.3675222665316));
#54223=CARTESIAN_POINT('Ctrl Pts',(-9.17584074389774,-38.2891486536877,
28.3477866805065));
#54224=CARTESIAN_POINT('Ctrl Pts',(-9.2591826939759,-38.3089160558987,28.3430213134391));
#54225=CARTESIAN_POINT('Ctrl Pts',(-9.37573350284544,-38.3319360008063,
28.3362743725662));
#54226=CARTESIAN_POINT('Ctrl Pts',(-9.40837939797173,-38.3378872249599,
28.3343758139665));
#54227=CARTESIAN_POINT('Ctrl Pts',(-9.46542756567714,-38.3474236978603,
28.3310404631353));
#54228=CARTESIAN_POINT('Ctrl Pts',(-9.48979167137738,-38.3512237339599,
28.3296104314202));
#54229=CARTESIAN_POINT('Ctrl Pts',(-9.54120745208911,-38.3586692984014,
28.3265799304701));
#54230=CARTESIAN_POINT('Ctrl Pts',(-9.56826594492124,-38.3622545559208,
28.3249777016695));
#54231=CARTESIAN_POINT('Ctrl Pts',(-9.63405956671405,-38.3701649272472,
28.3210627840895));
#54232=CARTESIAN_POINT('Ctrl Pts',(-9.67283100420665,-38.3741494181034,
28.3187397692326));
#54233=CARTESIAN_POINT('Ctrl Pts',(-9.82042713161933,-38.3867498966942,
28.3098324414982));
#54234=CARTESIAN_POINT('Ctrl Pts',(-9.9295679435339,-38.3907752388314,28.3031111114502));
#54235=CARTESIAN_POINT('Ctrl Pts',(-10.2409523380736,-38.3872195929405,
28.2835720651901));
#54236=CARTESIAN_POINT('Ctrl Pts',(-10.4425764903608,-38.3668128946524,
28.2704593358006));
#54237=CARTESIAN_POINT('Ctrl Pts',(-10.7756025125774,-38.3026643305676,
28.2486687382601));
#54238=CARTESIAN_POINT('Ctrl Pts',(-10.9083670477982,-38.2686429996786,
28.2399553930302));
#54239=CARTESIAN_POINT('Ctrl Pts',(-11.0655311581706,-38.2180493717434,
28.2298674715829));
#54240=CARTESIAN_POINT('Ctrl Pts',(-11.0922349017072,-38.2090842057795,
28.2281617377294));
#54241=CARTESIAN_POINT('Ctrl Pts',(-11.1343968820166,-38.1943420161088,
28.2254852114822));
#54242=CARTESIAN_POINT('Ctrl Pts',(-11.1499294545838,-38.1887833849867,
28.224502784887));
#54243=CARTESIAN_POINT('Ctrl Pts',(-11.1798643120017,-38.1778234429967,
28.2226172704239));
#54244=CARTESIAN_POINT('Ctrl Pts',(-11.194271320391,-38.1724371782705,28.2217134377073));
#54245=CARTESIAN_POINT('Ctrl Pts',(-11.2299946806446,-38.158803653946,28.2194802901512));
#54246=CARTESIAN_POINT('Ctrl Pts',(-11.2512656695106,-38.1504383384015,
28.2181576685891));
#54247=CARTESIAN_POINT('Ctrl Pts',(-11.3345206370969,-38.1167201179939,
28.2130028053058));
#54248=CARTESIAN_POINT('Ctrl Pts',(-11.3958358477449,-38.0897464442777,
28.20925430883));
#54249=CARTESIAN_POINT('Ctrl Pts',(-11.5658273270964,-38.0088697802057,
28.1988916781526));
#54250=CARTESIAN_POINT('Ctrl Pts',(-11.6724706396187,-37.9509249117669,
28.1924239175614));
#54251=CARTESIAN_POINT('Ctrl Pts',(-11.9849633252903,-37.7587374229869,
28.1729478360663));
#54252=CARTESIAN_POINT('Ctrl Pts',(-12.1795245139706,-37.6077525295176,
28.1600322001831));
#54253=CARTESIAN_POINT('Ctrl Pts',(-12.3927020634508,-37.4016616550794,
28.1434190878654));
#54254=CARTESIAN_POINT('Ctrl Pts',(-12.4285344539276,-37.3654221391915,
28.1405327830202));
#54255=CARTESIAN_POINT('Ctrl Pts',(-12.4841305742579,-37.3065990912556,
28.1358927807155));
#54256=CARTESIAN_POINT('Ctrl Pts',(-12.5044355110543,-37.2845364443238,
28.1341620910076));
#54257=CARTESIAN_POINT('Ctrl Pts',(-12.542132053673,-37.2424700906363,28.1308784278349));
#54258=CARTESIAN_POINT('Ctrl Pts',(-12.5595869853624,-37.2225260157992,
28.1293282543901));
#54259=CARTESIAN_POINT('Ctrl Pts',(-12.5987131319049,-37.1767480402325,
28.1257839539075));
#54260=CARTESIAN_POINT('Ctrl Pts',(-12.6202360861217,-37.1507916455033,
28.1237840618344));
#54261=CARTESIAN_POINT('Ctrl Pts',(-12.6865471837808,-37.0683485251447,
28.1174600344297));
#54262=CARTESIAN_POINT('Ctrl Pts',(-12.729920631706,-37.0107544767929,28.1130820268668));
#54263=CARTESIAN_POINT('Ctrl Pts',(-12.8298413340573,-36.8688756876391,
28.1023878040694));
#54264=CARTESIAN_POINT('Ctrl Pts',(-12.8845020854608,-36.7833517200597,
28.096013140807));
#54265=CARTESIAN_POINT('Ctrl Pts',(-13.0347698264456,-36.523210528921,28.07689198148));
#54266=CARTESIAN_POINT('Ctrl Pts',(-13.1189289791171,-36.3424889285501,
28.0639261820548));
#54267=CARTESIAN_POINT('Ctrl Pts',(-13.218543037923,-36.0677477931313,28.0453344477974));
#54268=CARTESIAN_POINT('Ctrl Pts',(-13.2467056778762,-35.9787796896697,
28.0394813346878));
#54269=CARTESIAN_POINT('Ctrl Pts',(-13.2780155784685,-35.8635402341408,
28.032202702615));
#54270=CARTESIAN_POINT('Ctrl Pts',(-13.2845751589283,-35.8382445854423,
28.0306234205127));
#54271=CARTESIAN_POINT('Ctrl Pts',(-13.2946914175318,-35.79728993047,28.0280989113837));
#54272=CARTESIAN_POINT('Ctrl Pts',(-13.2984303802658,-35.7816775676792,
28.0271440964218));
#54273=CARTESIAN_POINT('Ctrl Pts',(-13.3055989806115,-35.7507768688988,
28.0252699906278));
#54274=CARTESIAN_POINT('Ctrl Pts',(-13.3090337880532,-35.7354902664808,
28.024350464316));
#54275=CARTESIAN_POINT('Ctrl Pts',(-13.3175298447815,-35.6964139050986,
28.0220180350336));
#54276=CARTESIAN_POINT('Ctrl Pts',(-13.3224413731803,-35.6725919957669,
28.0206131949169));
#54277=CARTESIAN_POINT('Ctrl Pts',(-13.3326711587271,-35.6201262843258,
28.0175525224743));
#54278=CARTESIAN_POINT('Ctrl Pts',(-13.3378774649339,-35.5914624221048,
28.0159020993239));
#54279=CARTESIAN_POINT('Ctrl Pts',(-13.373848976752,-35.3777869694156,28.0037368074046));
#54280=CARTESIAN_POINT('Ctrl Pts',(-13.3895833277203,-35.1905621689522,
27.9938307688362));
#54281=CARTESIAN_POINT('Ctrl Pts',(-13.3897486828724,-35.0029882209942,
27.9838866141078));
#54282=CARTESIAN_POINT('Origin',(-10.,-35.,32.7603849714045));
#54283=CARTESIAN_POINT('',(-14.0849984181033,-35.0035950095037,28.3853849713664));
#54284=CARTESIAN_POINT('Ctrl Pts',(-7.5128274573098,-31.7594448403263,29.1925543292906));
#54285=CARTESIAN_POINT('Ctrl Pts',(-7.41829563611702,-31.8319993683303,
29.1867402586116));
#54286=CARTESIAN_POINT('Ctrl Pts',(-7.32683078998923,-31.9087785501752,
29.1809261879325));
#54287=CARTESIAN_POINT('Ctrl Pts',(-7.23882981532482,-31.9894910378375,
29.1751121172534));
#54288=CARTESIAN_POINT('Ctrl Pts',(-7.1509049789919,-32.070133693158,29.1693030769008));
#54289=CARTESIAN_POINT('Ctrl Pts',(-7.06643835081943,-32.1547026087496,
29.1634940365483));
#54290=CARTESIAN_POINT('Ctrl Pts',(-6.98579434796882,-32.2428657473269,
29.1576849961958));
#54291=CARTESIAN_POINT('Ctrl Pts',(-6.90519378059777,-32.3309814005604,
29.151879084637));
#54292=CARTESIAN_POINT('Ctrl Pts',(-6.82841201843355,-32.4226871260208,
29.1460731730783));
#54293=CARTESIAN_POINT('Ctrl Pts',(-6.75577677243,-32.5176139200972,29.1402672615195));
#54294=CARTESIAN_POINT('Ctrl Pts',(-6.68316115920835,-32.6125150561474,
29.1344629192567));
#54295=CARTESIAN_POINT('Ctrl Pts',(-6.61469008138252,-32.7106352056854,
29.1286585769939));
#54296=CARTESIAN_POINT('Ctrl Pts',(-6.55065069332656,-32.8115726284495,
29.122854234731));
#54297=CARTESIAN_POINT('Ctrl Pts',(-6.48661351598212,-32.9125065667405,
29.1170500928406));
#54298=CARTESIAN_POINT('Ctrl Pts',(-6.42700794269385,-33.016257240098,29.1112459509502));
#54299=CARTESIAN_POINT('Ctrl Pts',(-6.37207719311032,-33.1223948478847,
29.1054418090597));
#54300=CARTESIAN_POINT('Ctrl Pts',(-6.31713538878711,-33.2285538157227,
29.0996364990935));
#54301=CARTESIAN_POINT('Ctrl Pts',(-6.26687046665079,-33.3371003107878,
29.0938311891273));
#54302=CARTESIAN_POINT('Ctrl Pts',(-6.22147888630712,-33.4475815018568,
29.0880258791611));
#54303=CARTESIAN_POINT('Ctrl Pts',(-6.17603972326924,-33.5581785071956,
29.0822144836547));
#54304=CARTESIAN_POINT('Ctrl Pts',(-6.13548426028394,-33.6707138808813,
29.0764030881482));
#54305=CARTESIAN_POINT('Ctrl Pts',(-6.09996021653626,-33.7847162111671,
29.0705916926418));
#54306=CARTESIAN_POINT('Ctrl Pts',(-6.06441677612587,-33.8987807884415,
29.0647771240259));
#54307=CARTESIAN_POINT('Ctrl Pts',(-6.03391033225052,-34.014313523556,29.05896255541));
#54308=CARTESIAN_POINT('Ctrl Pts',(-6.00853783392326,-34.1308309849183,
29.0531479867942));
#54309=CARTESIAN_POINT('Ctrl Pts',(-5.98312526945627,-34.2475324409677,
29.047324236295));
#54310=CARTESIAN_POINT('Ctrl Pts',(-5.96286291620998,-34.3652213275178,
29.0415004857958));
#54311=CARTESIAN_POINT('Ctrl Pts',(-5.94779610757038,-34.4834067226742,
29.0356767352966));
#54312=CARTESIAN_POINT('Ctrl Pts',(-5.9358693202173,-34.5769615098881,29.0310666924227));
#54313=CARTESIAN_POINT('Ctrl Pts',(-5.92719713908413,-34.6708272463293,
29.0264566495489));
#54314=CARTESIAN_POINT('Ctrl Pts',(-5.92177888561108,-34.7647606704813,
29.021846606675));
#54315=CARTESIAN_POINT('Ctrl Pts',(-5.91493526854366,-34.8834048771292,
29.0160238137307));
#54316=CARTESIAN_POINT('Ctrl Pts',(-5.91326230543851,-35.0025398287942,
29.0102010207864));
#54317=CARTESIAN_POINT('Ctrl Pts',(-5.91681257603086,-35.1216776920402,
29.0043782278421));
#54318=CARTESIAN_POINT('Ctrl Pts',(-5.92035836024105,-35.2406650039495,
28.9985627930058));
#54319=CARTESIAN_POINT('Ctrl Pts',(-5.92911423802636,-35.359654815448,28.9927473581695));
#54320=CARTESIAN_POINT('Ctrl Pts',(-5.94308092912631,-35.4781554688398,
28.9869319233332));
#54321=CARTESIAN_POINT('Ctrl Pts',(-5.95703361417853,-35.5965372876561,
28.981122320319));
#54322=CARTESIAN_POINT('Ctrl Pts',(-5.97618666960746,-35.7144305209006,
28.9753127173048));
#54323=CARTESIAN_POINT('Ctrl Pts',(-6.00048880543195,-35.8313454182979,
28.9695031142906));
#54324=CARTESIAN_POINT('Ctrl Pts',(-6.02571566512785,-35.9527090603374,
28.9634724492829));
#54325=CARTESIAN_POINT('Ctrl Pts',(-6.05649123059984,-36.0730179860591,
28.9574417842752));
#54326=CARTESIAN_POINT('Ctrl Pts',(-6.09269913988917,-36.1917319281521,
28.9514111192676));
#54327=CARTESIAN_POINT('Ctrl Pts',(-6.12754041998201,-36.305965138204,28.9456080753249));
#54328=CARTESIAN_POINT('Ctrl Pts',(-6.16741127144981,-36.4187211579221,
28.9398050313822));
#54329=CARTESIAN_POINT('Ctrl Pts',(-6.21215652824688,-36.5295315732267,
28.9340019874395));
#54330=CARTESIAN_POINT('Ctrl Pts',(-6.25689513162165,-36.6403255115113,
28.9281998063839));
#54331=CARTESIAN_POINT('Ctrl Pts',(-6.30650654603254,-36.7491740420576,
28.9223976253283));
#54332=CARTESIAN_POINT('Ctrl Pts',(-6.36078699819927,-36.8556275831978,
28.9165954442726));
#54333=CARTESIAN_POINT('Ctrl Pts',(-6.41507219960668,-36.9620904384367,
28.9107927555581));
#54334=CARTESIAN_POINT('Ctrl Pts',(-6.47402706542833,-37.0661575237296,
28.9049900668436));
#54335=CARTESIAN_POINT('Ctrl Pts',(-6.53740159426591,-37.1674033497731,
28.899187378129));
#54336=CARTESIAN_POINT('Ctrl Pts',(-6.60079663637736,-37.2686819473953,
28.8933828111813));
#54337=CARTESIAN_POINT('Ctrl Pts',(-6.66861396995011,-37.3671371235897,
28.8875782442336));
#54338=CARTESIAN_POINT('Ctrl Pts',(-6.74056032672592,-37.4623724365512,
28.8817736772859));
#54339=CARTESIAN_POINT('Ctrl Pts',(-6.81258635248139,-37.557713207253,28.875962682717));
#54340=CARTESIAN_POINT('Ctrl Pts',(-6.88875028161634,-37.649826671619,28.8701516881482));
#54341=CARTESIAN_POINT('Ctrl Pts',(-6.96871852630632,-37.7383494348314,
28.8643406935793));
#54342=CARTESIAN_POINT('Ctrl Pts',(-7.04873927766027,-37.8269303215528,
28.8585258835466));
#54343=CARTESIAN_POINT('Ctrl Pts',(-7.13256903295501,-37.9119155217405,
28.852711073514));
#54344=CARTESIAN_POINT('Ctrl Pts',(-7.2198385241554,-37.9929796471459,28.8468962634814));
#54345=CARTESIAN_POINT('Ctrl Pts',(-7.30723309632454,-38.0741599595394,
28.841073119241));
#54346=CARTESIAN_POINT('Ctrl Pts',(-7.3980769344774,-38.1514077163572,28.8352499750006));
#54347=CARTESIAN_POINT('Ctrl Pts',(-7.49196892069193,-38.2244387271624,
28.8294268307601));
#54348=CARTESIAN_POINT('Ctrl Pts',(-7.51701302504882,-38.2439185180331,
28.8278736052089));
#54349=CARTESIAN_POINT('Ctrl Pts',(-7.5422738441232,-38.2630985466123,28.8263203796577));
#54350=CARTESIAN_POINT('Ctrl Pts',(-7.56774345158431,-38.2819739613058,
28.8247671541065));
#54351=CARTESIAN_POINT('Ctrl Pts',(-7.66324133017982,-38.3527470214556,
28.8189433601848));
#54352=CARTESIAN_POINT('Ctrl Pts',(-7.76198468770386,-38.4194625362104,
28.8131195662631));
#54353=CARTESIAN_POINT('Ctrl Pts',(-7.86359411418139,-38.4818091405244,
28.8072957723414));
#54354=CARTESIAN_POINT('Ctrl Pts',(-7.96507537238453,-38.5440771019707,
28.8014793244469));
#54355=CARTESIAN_POINT('Ctrl Pts',(-8.06941516401801,-38.6019869023167,
28.7956628765524));
#54356=CARTESIAN_POINT('Ctrl Pts',(-8.17620246803788,-38.65526846653,28.789846428658));
#54357=CARTESIAN_POINT('Ctrl Pts',(-8.2828829002652,-38.7084967070236,28.7840358018133));
#54358=CARTESIAN_POINT('Ctrl Pts',(-8.39200560874236,-38.7571057447421,
28.7782251749687));
#54359=CARTESIAN_POINT('Ctrl Pts',(-8.50313267252363,-38.8008700588068,
28.772414548124));
#54360=CARTESIAN_POINT('Ctrl Pts',(-8.61846065936954,-38.8462887899873,
28.7663842628496));
#54361=CARTESIAN_POINT('Ctrl Pts',(-8.73594715078625,-38.8864890459525,
28.7603539775752));
#54362=CARTESIAN_POINT('Ctrl Pts',(-8.85507667243839,-38.9212721882069,
28.7543236923007));
#54363=CARTESIAN_POINT('Ctrl Pts',(-8.96973762288422,-38.954750608124,28.7485196041836));
#54364=CARTESIAN_POINT('Ctrl Pts',(-9.08592013570892,-38.9832108640657,
28.7427155160664));
#54365=CARTESIAN_POINT('Ctrl Pts',(-9.20314722294913,-39.006526007866,28.7369114279493));
#54366=CARTESIAN_POINT('Ctrl Pts',(-9.32035699746757,-39.0298377083614,
28.7311081970108));
#54367=CARTESIAN_POINT('Ctrl Pts',(-9.43861063925757,-39.04800572821,28.7253049660724));
#54368=CARTESIAN_POINT('Ctrl Pts',(-9.55742027561235,-39.0609540981844,
28.7195017351339));
#54369=CARTESIAN_POINT('Ctrl Pts',(-9.67624039904241,-39.0739036110841,
28.7136979919565));
#54370=CARTESIAN_POINT('Ctrl Pts',(-9.79561620869263,-39.0816325138321,
28.7078942487792));
#54371=CARTESIAN_POINT('Ctrl Pts',(-9.91505464847786,-39.0841167083293,
28.7020905056018));
#54372=CARTESIAN_POINT('Ctrl Pts',(-10.03453181255,-39.0866017082512,28.696284880737));
#54373=CARTESIAN_POINT('Ctrl Pts',(-10.1540712391352,-39.0838386096445,
28.6904792558721));
#54374=CARTESIAN_POINT('Ctrl Pts',(-10.2731804541561,-39.0758554242597,
28.6846736310073));
#54375=CARTESIAN_POINT('Ctrl Pts',(-10.392421535695,-39.067863400643,28.6788615787007));
#54376=CARTESIAN_POINT('Ctrl Pts',(-10.5112310473222,-39.0546397818076,
28.6730495263942));
#54377=CARTESIAN_POINT('Ctrl Pts',(-10.6291220559173,-39.0362644163581,
28.6672374740876));
#54378=CARTESIAN_POINT('Ctrl Pts',(-10.7470904800299,-39.0178769843528,
28.6614216051793));
#54379=CARTESIAN_POINT('Ctrl Pts',(-10.8641388005456,-38.9943311487283,
28.6556057362709));
#54380=CARTESIAN_POINT('Ctrl Pts',(-10.979792313732,-38.9657574335745,28.6497898673626));
#54381=CARTESIAN_POINT('Ctrl Pts',(-11.0956114326921,-38.9371428033454,
28.6439656706357));
#54382=CARTESIAN_POINT('Ctrl Pts',(-11.2100313676118,-38.9034860386072,
28.6381414739088));
#54383=CARTESIAN_POINT('Ctrl Pts',(-11.3225944121625,-38.8649668848409,
28.6323172771819));
#54384=CARTESIAN_POINT('Ctrl Pts',(-11.3524193622157,-38.8547607657566,
28.6307740853006));
#54385=CARTESIAN_POINT('Ctrl Pts',(-11.382114070009,-38.8442135397309,28.6292308934194));
#54386=CARTESIAN_POINT('Ctrl Pts',(-11.4116702960911,-38.8333290982035,
28.6276877015381));
#54387=CARTESIAN_POINT('Ctrl Pts',(-11.5232093497215,-38.7922534783362,
28.6218640161485));
#54388=CARTESIAN_POINT('Ctrl Pts',(-11.6331339301567,-38.7462394001181,
28.616040330759));
#54389=CARTESIAN_POINT('Ctrl Pts',(-11.7409756547684,-38.6954335022435,
28.6102166453694));
#54390=CARTESIAN_POINT('Ctrl Pts',(-11.8486813603392,-38.6446916850346,
28.604400305301));
#54391=CARTESIAN_POINT('Ctrl Pts',(-11.9543090691492,-38.5891702417359,
28.5985839652326));
#54392=CARTESIAN_POINT('Ctrl Pts',(-12.0574076037386,-38.5290648835178,
28.5927676251642));
#54393=CARTESIAN_POINT('Ctrl Pts',(-12.1604029711546,-38.4690196706737,
28.5869571053081));
#54394=CARTESIAN_POINT('Ctrl Pts',(-12.2608738484572,-38.4043998725906,
28.581146585452));
#54395=CARTESIAN_POINT('Ctrl Pts',(-12.3583915761085,-38.3354481218781,
28.575336065596));
#54396=CARTESIAN_POINT('Ctrl Pts',(-12.4595982965265,-38.2638879991726,
28.5693057399032));
#54397=CARTESIAN_POINT('Ctrl Pts',(-12.5576236207883,-38.1876618965559,
28.5632754142105));
#54398=CARTESIAN_POINT('Ctrl Pts',(-12.6520188291916,-38.1070920697033,
28.5572450885177));
#54399=CARTESIAN_POINT('Ctrl Pts',(-12.7428710156203,-38.0295463440933,
28.5514411045726));
#54400=CARTESIAN_POINT('Ctrl Pts',(-12.8303603413976,-37.9479773804106,
28.5456371206276));
#54401=CARTESIAN_POINT('Ctrl Pts',(-12.9141191759421,-37.862714520941,28.5398331366825));
#54402=CARTESIAN_POINT('Ctrl Pts',(-12.9978656580678,-37.7774642356977,
28.5340300086858));
#54403=CARTESIAN_POINT('Ctrl Pts',(-13.0778824569824,-37.688521429232,28.5282268806891));
#54404=CARTESIAN_POINT('Ctrl Pts',(-13.1538386131533,-37.5962524919937,
28.5224237526924));
#54405=CARTESIAN_POINT('Ctrl Pts',(-13.2298014916053,-37.5039753887585,
28.5166201111066));
#54406=CARTESIAN_POINT('Ctrl Pts',(-13.301702753262,-37.408371884733,28.5108164695208));
#54407=CARTESIAN_POINT('Ctrl Pts',(-13.3692519812247,-37.3098411389126,
28.5050128279349));
#54408=CARTESIAN_POINT('Ctrl Pts',(-13.4368231274801,-37.2112784219538,
28.4992073031904));
#54409=CARTESIAN_POINT('Ctrl Pts',(-13.5000392008406,-37.109786910809,28.4934017784459));
#54410=CARTESIAN_POINT('Ctrl Pts',(-13.5586536871284,-37.0057938416217,
28.4875962537014));
#54411=CARTESIAN_POINT('Ctrl Pts',(-13.6173330942738,-36.9016855906822,
28.4817842988119));
#54412=CARTESIAN_POINT('Ctrl Pts',(-13.6714005403349,-36.7950706070611,
28.4759723439225));
#54413=CARTESIAN_POINT('Ctrl Pts',(-13.7206559037518,-36.6863999068659,
28.470160389033));
#54414=CARTESIAN_POINT('Ctrl Pts',(-13.7699436246378,-36.5776578173114,
28.464344616079));
#54415=CARTESIAN_POINT('Ctrl Pts',(-13.814412815498,-36.46685769976,28.4585288431251));
#54416=CARTESIAN_POINT('Ctrl Pts',(-13.8539124424957,-36.35446811907,28.4527130701712));
#54417=CARTESIAN_POINT('Ctrl Pts',(-13.8934686500774,-36.2419175477936,
28.44688896651));
#54418=CARTESIAN_POINT('Ctrl Pts',(-13.9280409675739,-36.1277733584114,
28.4410648628488));
#54419=CARTESIAN_POINT('Ctrl Pts',(-13.9575288461897,-36.0125168796503,
28.4352407591876));
#54420=CARTESIAN_POINT('Ctrl Pts',(-13.9653470963981,-35.9819584254174,
28.4336965891149));
#54421=CARTESIAN_POINT('Ctrl Pts',(-13.972808211015,-35.9513218213683,28.4321524190423));
#54422=CARTESIAN_POINT('Ctrl Pts',(-13.9799109260694,-35.9206161092189,
28.4306082489697));
#54423=CARTESIAN_POINT('Ctrl Pts',(-14.0156549436737,-35.7660913243706,
28.4228372991516));
#54424=CARTESIAN_POINT('Ctrl Pts',(-14.0424112771735,-35.6094162135617,
28.4150663493335));
#54425=CARTESIAN_POINT('Ctrl Pts',(-14.0599741506301,-35.451480781668,28.4072953995154));
#54426=CARTESIAN_POINT('Ctrl Pts',(-14.0764805016467,-35.3030462055577,
28.3999919234785));
#54427=CARTESIAN_POINT('Ctrl Pts',(-14.0848664955798,-35.1534981411174,
28.3926884474415));
#54428=CARTESIAN_POINT('Ctrl Pts',(-14.0849984181026,-35.0035950102863,
28.3853849714045));
#54429=CARTESIAN_POINT('Ctrl Pts',(-14.0849984181033,-35.0035950095037,
28.3853849713664));
#54430=CARTESIAN_POINT('Ctrl Pts',(-14.0851020303385,-34.885860740221,28.3796488042185));
#54431=CARTESIAN_POINT('Ctrl Pts',(-14.0801115803583,-34.7679841837216,
28.3739126370707));
#54432=CARTESIAN_POINT('Ctrl Pts',(-14.0700169326326,-34.6504471884196,
28.3681764699229));
#54433=CARTESIAN_POINT('Ctrl Pts',(-14.0599295789436,-34.5329951212077,
28.3624444475273));
#54434=CARTESIAN_POINT('Ctrl Pts',(-14.0447453971451,-34.4158825442329,
28.3567124251316));
#54435=CARTESIAN_POINT('Ctrl Pts',(-14.024506318868,-34.2995901989612,28.350980402736));
#54436=CARTESIAN_POINT('Ctrl Pts',(-14.0042749038498,-34.1833418862451,
28.3452505506947));
#54437=CARTESIAN_POINT('Ctrl Pts',(-13.9789924676054,-34.0679136012425,
28.3395206986534));
#54438=CARTESIAN_POINT('Ctrl Pts',(-13.948752592152,-33.9537791982699,28.3337908466121));
#54439=CARTESIAN_POINT('Ctrl Pts',(-13.9185165787158,-33.8396593717141,
28.3280617263459));
#54440=CARTESIAN_POINT('Ctrl Pts',(-13.8833244923329,-33.726833504574,28.3223326060797));
#54441=CARTESIAN_POINT('Ctrl Pts',(-13.8433204650405,-33.6157627360163,
28.3166034858135));
#54442=CARTESIAN_POINT('Ctrl Pts',(-13.8033115084338,-33.5046782812685,
28.3108736596025));
#54443=CARTESIAN_POINT('Ctrl Pts',(-13.7584895755464,-33.3953497497871,
28.3051438333915));
#54444=CARTESIAN_POINT('Ctrl Pts',(-13.7090475743058,-33.2882199056139,
28.2994140071806));
#54445=CARTESIAN_POINT('Ctrl Pts',(-13.659557017041,-33.1809848513123,28.2936785538191));
#54446=CARTESIAN_POINT('Ctrl Pts',(-13.6054375067942,-33.0759531783709,
28.2879431004577));
#54447=CARTESIAN_POINT('Ctrl Pts',(-13.5469287542339,-32.9735446187027,
28.2822076470962));
#54448=CARTESIAN_POINT('Ctrl Pts',(-13.4883905352389,-32.8710844835864,
28.2764693052206));
#54449=CARTESIAN_POINT('Ctrl Pts',(-13.4254588967976,-32.7712504469683,
28.270730963345));
#54450=CARTESIAN_POINT('Ctrl Pts',(-13.3584168618395,-32.6744331482169,
28.2649926214694));
#54451=CARTESIAN_POINT('Ctrl Pts',(-13.2912691229998,-32.5774631995006,
28.259245232061));
#54452=CARTESIAN_POINT('Ctrl Pts',(-13.2199982971978,-32.4835198232529,
28.2534978426526));
#54453=CARTESIAN_POINT('Ctrl Pts',(-13.1449278762672,-32.3929607496093,
28.2477504532441));
#54454=CARTESIAN_POINT('Ctrl Pts',(-13.0830084151193,-32.3182659633999,
28.2430099009632));
#54455=CARTESIAN_POINT('Ctrl Pts',(-13.0185047918086,-32.2458730372111,
28.2382693486822));
#54456=CARTESIAN_POINT('Ctrl Pts',(-12.9516163321836,-32.1759628140574,
28.2335287964012));
#54457=CARTESIAN_POINT('Ctrl Pts',(-12.8694458679809,-32.0900802040935,
28.2277051702677));
#54458=CARTESIAN_POINT('Ctrl Pts',(-12.7833914345599,-32.0076484389653,
28.2218815441341));
#54459=CARTESIAN_POINT('Ctrl Pts',(-12.6937743723571,-31.9290384843127,
28.2160579180006));
#54460=CARTESIAN_POINT('Ctrl Pts',(-12.604270370409,-31.8505277034256,28.2102416389128));
#54461=CARTESIAN_POINT('Ctrl Pts',(-12.5112129835747,-31.7758294099165,
28.204425359825));
#54462=CARTESIAN_POINT('Ctrl Pts',(-12.4149616844493,-31.7052792132501,
28.1986090807372));
#54463=CARTESIAN_POINT('Ctrl Pts',(-12.318806728878,-31.6347996344013,28.1927986235032));
#54464=CARTESIAN_POINT('Ctrl Pts',(-12.2194645484442,-31.5684601323676,
28.1869881662693));
#54465=CARTESIAN_POINT('Ctrl Pts',(-12.1173286556274,-31.5065569470708,
28.1811777090354));
#54466=CARTESIAN_POINT('Ctrl Pts',(-12.0113275255331,-31.44231109366,28.1751473604853));
#54467=CARTESIAN_POINT('Ctrl Pts',(-11.9023173920652,-31.3828442621115,
28.1691170119352));
#54468=CARTESIAN_POINT('Ctrl Pts',(-11.7907728026743,-31.3284393278604,
28.1630866633851));
#54469=CARTESIAN_POINT('Ctrl Pts',(-11.6834165527187,-31.2760772209023,
28.1572827457787));
#54470=CARTESIAN_POINT('Ctrl Pts',(-11.5737131455584,-31.2284039261651,
28.1514788281722));
#54471=CARTESIAN_POINT('Ctrl Pts',(-11.4621112512257,-31.1856251247368,
28.1456749105658));
#54472=CARTESIAN_POINT('Ctrl Pts',(-11.3505258399602,-31.1428526415333,
28.1398718501704));
#54473=CARTESIAN_POINT('Ctrl Pts',(-11.2370428803218,-31.1049733601433,
28.1340687897749));
#54474=CARTESIAN_POINT('Ctrl Pts',(-11.1221303813735,-31.0721445536784,
28.1282657293794));
#54475=CARTESIAN_POINT('Ctrl Pts',(-11.0072077359545,-31.0393128485164,
28.122462156589));
#54476=CARTESIAN_POINT('Ctrl Pts',(-10.8908556929035,-31.0115326170957,
28.1166585837986));
#54477=CARTESIAN_POINT('Ctrl Pts',(-10.7735561312046,-30.9889108820826,
28.1108550110081));
#54478=CARTESIAN_POINT('Ctrl Pts',(-10.6562185306065,-30.9662818111008,
28.1050495561858));
#54479=CARTESIAN_POINT('Ctrl Pts',(-10.5379332010082,-30.9488146407147,
28.0992441013634));
#54480=CARTESIAN_POINT('Ctrl Pts',(-10.4191902487106,-30.9365649340262,
28.0934386465411));
#54481=CARTESIAN_POINT('Ctrl Pts',(-10.3003158034443,-30.9243016623195,
28.0876267629036));
#54482=CARTESIAN_POINT('Ctrl Pts',(-10.1809831303593,-30.9172674289987,
28.0818148792661));
#54483=CARTESIAN_POINT('Ctrl Pts',(-10.0616856290819,-30.915465769128,28.0760029956286));
#54484=CARTESIAN_POINT('Ctrl Pts',(-9.94230977402666,-30.9136629259396,
28.0701872947859));
#54485=CARTESIAN_POINT('Ctrl Pts',(-9.82296954400879,-30.917099488788,28.0643715939433));
#54486=CARTESIAN_POINT('Ctrl Pts',(-9.70415484288956,-30.9257269798142,
28.0585558931006));
#54487=CARTESIAN_POINT('Ctrl Pts',(-9.58516996018755,-30.9343668282343,
28.0527318622688));
#54488=CARTESIAN_POINT('Ctrl Pts',(-9.46671251292297,-30.9482123976731,
28.0469078314369));
#54489=CARTESIAN_POINT('Ctrl Pts',(-9.3492639640545,-30.9671638253554,28.0410838006051));
#54490=CARTESIAN_POINT('Ctrl Pts',(-9.31811084242144,-30.9721906744514,
28.039538981681));
#54491=CARTESIAN_POINT('Ctrl Pts',(-9.2870286282477,-30.9775764827311,28.0379941627569));
#54492=CARTESIAN_POINT('Ctrl Pts',(-9.25602612785593,-30.9833187981162,
28.0364493438328));
#54493=CARTESIAN_POINT('Ctrl Pts',(-9.13915033347081,-31.0049666543782,
28.0306255574719));
#54494=CARTESIAN_POINT('Ctrl Pts',(-9.02303170475046,-31.0317548617166,
28.0248017711111));
#54495=CARTESIAN_POINT('Ctrl Pts',(-8.90815669677599,-31.0636180061883,
28.0189779847502));
#54496=CARTESIAN_POINT('Ctrl Pts',(-8.79342204217191,-31.0954422205237,
28.0131613138452));
#54497=CARTESIAN_POINT('Ctrl Pts',(-8.67992837677122,-31.1323289331788,
28.0073446429401));
#54498=CARTESIAN_POINT('Ctrl Pts',(-8.56815354344793,-31.1741614350761,
28.0015279720351));
#54499=CARTESIAN_POINT('Ctrl Pts',(-8.45650821956137,-31.2159454671738,
27.9957180406952));
#54500=CARTESIAN_POINT('Ctrl Pts',(-8.34657814333416,-31.2626637381606,
27.9899081093553));
#54501=CARTESIAN_POINT('Ctrl Pts',(-8.23882666697027,-31.3141495566118,
27.9840981780154));
#54502=CARTESIAN_POINT('Ctrl Pts',(-8.13114729556032,-31.3656009218686,
27.9782921345557));
#54503=CARTESIAN_POINT('Ctrl Pts',(-8.02564399174177,-31.421813314406,27.972486091096));
#54504=CARTESIAN_POINT('Ctrl Pts',(-7.9227605128364,-31.4825718041489,27.9666800476364));
#54505=CARTESIAN_POINT('Ctrl Pts',(-7.81992215651057,-31.5433036464668,
27.960876550588));
#54506=CARTESIAN_POINT('Ctrl Pts',(-7.71970169001365,-31.6085774118287,
27.9550730535397));
#54507=CARTESIAN_POINT('Ctrl Pts',(-7.6225180413552,-31.6781323722462,27.9492695564913));
#54508=CARTESIAN_POINT('Ctrl Pts',(-7.58550699385698,-31.7046214162293,
27.9470593749652));
#54509=CARTESIAN_POINT('Ctrl Pts',(-7.5489361159424,-31.7317309271604,27.944849193439));
#54510=CARTESIAN_POINT('Ctrl Pts',(-7.5128274573098,-31.7594448403263,27.9426390119128));
#54511=CARTESIAN_POINT('',(-14.0849988977546,-34.9969991094922,28.4896150285548));
#54512=CARTESIAN_POINT('Ctrl Pts',(-14.0849988977546,-34.9969991094922,
28.4896150285548));
#54513=CARTESIAN_POINT('Ctrl Pts',(-14.0848971428309,-34.8584839753713,
28.4828893597099));
#54514=CARTESIAN_POINT('Ctrl Pts',(-14.0777462394372,-34.7202527422421,
28.476163690865));
#54515=CARTESIAN_POINT('Ctrl Pts',(-14.0636562776183,-34.5829596453898,
28.4694380220201));
#54516=CARTESIAN_POINT('Ctrl Pts',(-14.0494857150941,-34.4448811723539,
28.4626738794264));
#54517=CARTESIAN_POINT('Ctrl Pts',(-14.028296588798,-34.3077517162237,28.4559097368326));
#54518=CARTESIAN_POINT('Ctrl Pts',(-14.0002501584321,-34.1722176191994,
28.4491455942389));
#54519=CARTESIAN_POINT('Ctrl Pts',(-13.9720232914753,-34.0358115641359,
28.4423379345624));
#54520=CARTESIAN_POINT('Ctrl Pts',(-13.9368506870528,-33.9010215747836,
28.4355302748859));
#54521=CARTESIAN_POINT('Ctrl Pts',(-13.8949450417453,-33.7684854358214,
28.4287226152095));
#54522=CARTESIAN_POINT('Ctrl Pts',(-13.8839505474168,-33.733712845698,28.4269365366238));
#54523=CARTESIAN_POINT('Ctrl Pts',(-13.8724928412928,-33.6990952808039,
28.4251504580381));
#54524=CARTESIAN_POINT('Ctrl Pts',(-13.8605763001412,-33.6646440059715,
28.4233643794524));
#54525=CARTESIAN_POINT('Ctrl Pts',(-13.8217205192481,-33.5523101358198,
28.417540585677));
#54526=CARTESIAN_POINT('Ctrl Pts',(-13.7778950594556,-33.441492542968,28.4117167919016));
#54527=CARTESIAN_POINT('Ctrl Pts',(-13.7292372490971,-33.3326624397121,
28.4058929981261));
#54528=CARTESIAN_POINT('Ctrl Pts',(-13.6806408148247,-33.2239696127895,
28.4000765503793));
#54529=CARTESIAN_POINT('Ctrl Pts',(-13.6272243188804,-33.1172596585844,
28.3942601026325));
#54530=CARTESIAN_POINT('Ctrl Pts',(-13.5691744935128,-33.0129875604673,
28.3884436548858));
#54531=CARTESIAN_POINT('Ctrl Pts',(-13.5111827639121,-32.9088198169708,
28.3826330281899));
#54532=CARTESIAN_POINT('Ctrl Pts',(-13.4485671270989,-32.8070854306003,
28.3768224014941));
#54533=CARTESIAN_POINT('Ctrl Pts',(-13.3815616740415,-32.7082178016544,
28.3710117747983));
#54534=CARTESIAN_POINT('Ctrl Pts',(-13.3120232194584,-32.6056126880183,
28.3649814894685));
#54535=CARTESIAN_POINT('Ctrl Pts',(-13.237756686359,-32.5060957616236,28.3589512041388));
#54536=CARTESIAN_POINT('Ctrl Pts',(-13.1590753521491,-32.410122026148,28.352920918809));
#54537=CARTESIAN_POINT('Ctrl Pts',(-13.0833453725403,-32.317748287147,28.3471168308427));
#54538=CARTESIAN_POINT('Ctrl Pts',(-13.003526109092,-32.2286570588905,28.3413127428765));
#54539=CARTESIAN_POINT('Ctrl Pts',(-12.9199395548036,-32.1432224454303,
28.3355086549102));
#54540=CARTESIAN_POINT('Ctrl Pts',(-12.8363653450308,-32.0578004494171,
28.3297054241231));
#54541=CARTESIAN_POINT('Ctrl Pts',(-12.749025236336,-31.9760342860264,28.323902193336));
#54542=CARTESIAN_POINT('Ctrl Pts',(-12.6582789903332,-31.8982621307478,
28.3180989625489));
#54543=CARTESIAN_POINT('Ctrl Pts',(-12.5675247343561,-31.8204831106898,
28.3122952195232));
#54544=CARTESIAN_POINT('Ctrl Pts',(-12.473364053341,-31.7466990653977,28.3064914764975));
#54545=CARTESIAN_POINT('Ctrl Pts',(-12.3761902757642,-31.6772082861901,
28.3006877334718));
#54546=CARTESIAN_POINT('Ctrl Pts',(-12.2789849925427,-31.6076949767088,
28.2948821087588));
#54547=CARTESIAN_POINT('Ctrl Pts',(-12.1787650018617,-31.5424779389958,
28.2890764840458));
#54548=CARTESIAN_POINT('Ctrl Pts',(-12.0759525754898,-31.4818121277684,
28.2832708593327));
#54549=CARTESIAN_POINT('Ctrl Pts',(-11.9730263248589,-31.4210791530546,
28.2774588071775));
#54550=CARTESIAN_POINT('Ctrl Pts',(-11.8675022614251,-31.3649076701075,
28.2716467550223));
#54551=CARTESIAN_POINT('Ctrl Pts',(-11.7598273533192,-31.3135067223024,
28.265834702867));
#54552=CARTESIAN_POINT('Ctrl Pts',(-11.6520817383006,-31.2620720210222,
28.2600188341098));
#54553=CARTESIAN_POINT('Ctrl Pts',(-11.5421828407542,-31.2154142528824,
28.2542029653526));
#54554=CARTESIAN_POINT('Ctrl Pts',(-11.4305961492278,-31.1736937318329,
28.2483870965954));
#54555=CARTESIAN_POINT('Ctrl Pts',(-11.3188496752328,-31.1319134706142,
28.2425629000184));
#54556=CARTESIAN_POINT('Ctrl Pts',(-11.2054109704769,-31.0950846928856,
28.2367387034413));
#54557=CARTESIAN_POINT('Ctrl Pts',(-11.0907592876752,-31.0633174910402,
28.2309145068642));
#54558=CARTESIAN_POINT('Ctrl Pts',(-11.0603808982341,-31.0549003757783,
28.2293713135375));
#54559=CARTESIAN_POINT('Ctrl Pts',(-11.0299173970239,-31.046838328789,28.2278281202107));
#54560=CARTESIAN_POINT('Ctrl Pts',(-10.9993777816479,-31.0391327907201,
28.226284926884));
#54561=CARTESIAN_POINT('Ctrl Pts',(-10.884120741644,-31.010051955925,28.2204608884079));
#54562=CARTESIAN_POINT('Ctrl Pts',(-10.767407519683,-30.9859592050703,28.2146368499319));
#54563=CARTESIAN_POINT('Ctrl Pts',(-10.6497075722854,-30.9669980076232,
28.2088128114558));
#54564=CARTESIAN_POINT('Ctrl Pts',(-10.532157786967,-30.9480610009502,28.2029962033121));
#54565=CARTESIAN_POINT('Ctrl Pts',(-10.4136241799048,-30.9342425897698,
28.1971795951684));
#54566=CARTESIAN_POINT('Ctrl Pts',(-10.2945896981088,-30.9256360116249,
28.1913629870247));
#54567=CARTESIAN_POINT('Ctrl Pts',(-10.1714609044516,-30.9167334014861,
28.185346310738));
#54568=CARTESIAN_POINT('Ctrl Pts',(-10.0477965797414,-30.9134077422541,
28.1793296344514));
#54569=CARTESIAN_POINT('Ctrl Pts',(-9.92414173974794,-30.915704402917,28.1733129581648));
#54570=CARTESIAN_POINT('Ctrl Pts',(-9.80481594266389,-30.9179206595896,
28.1675069202149));
#54571=CARTESIAN_POINT('Ctrl Pts',(-9.68549942568355,-30.9253721801646,
28.1617008822649));
#54572=CARTESIAN_POINT('Ctrl Pts',(-9.56668514340063,-30.9380468694173,
28.155894844315));
#54573=CARTESIAN_POINT('Ctrl Pts',(-9.44791897097225,-30.9507164264802,
28.1500911573251));
#54574=CARTESIAN_POINT('Ctrl Pts',(-9.32965503409748,-30.9686049024805,
28.1442874703353));
#54575=CARTESIAN_POINT('Ctrl Pts',(-9.21238265579534,-30.9916482291211,
28.1384837833455));
#54576=CARTESIAN_POINT('Ctrl Pts',(-9.09513008935856,-31.0146876628477,
28.1326810768241));
#54577=CARTESIAN_POINT('Ctrl Pts',(-8.97886914852464,-31.0428801353257,
28.1268783703028));
#54578=CARTESIAN_POINT('Ctrl Pts',(-8.86407979923247,-31.0761103102294,
28.1210756637814));
#54579=CARTESIAN_POINT('Ctrl Pts',(-8.74928275537019,-31.1093427126212,
28.1152725682924));
#54580=CARTESIAN_POINT('Ctrl Pts',(-8.6359578908288,-31.1476133739308,28.1094694728035));
#54581=CARTESIAN_POINT('Ctrl Pts',(-8.52457020601974,-31.1907570406923,
28.1036663773146));
#54582=CARTESIAN_POINT('Ctrl Pts',(-8.41310155905027,-31.2339320664363,
28.0978590638446));
#54583=CARTESIAN_POINT('Ctrl Pts',(-8.30357328398359,-31.2819870215234,
28.0920517503745));
#54584=CARTESIAN_POINT('Ctrl Pts',(-8.19643055826853,-31.3347084333095,
28.0862444369045));
#54585=CARTESIAN_POINT('Ctrl Pts',(-8.08924108020353,-31.3874528503895,
28.0804345893796));
#54586=CARTESIAN_POINT('Ctrl Pts',(-7.98443958397608,-31.4448675863832,
28.0746247418546));
#54587=CARTESIAN_POINT('Ctrl Pts',(-7.88244553440794,-31.5066938174201,
28.0688148943297));
#54588=CARTESIAN_POINT('Ctrl Pts',(-7.78033805422457,-31.5685888072469,
28.0629985855006));
#54589=CARTESIAN_POINT('Ctrl Pts',(-7.68104459292747,-31.6349048603944,
28.0571822766715));
#54590=CARTESIAN_POINT('Ctrl Pts',(-7.58495459416272,-31.7053405809182,
28.0513659678423));
#54591=CARTESIAN_POINT('Ctrl Pts',(-7.56070642011141,-31.7231149344685,
28.0498982306102));
#54592=CARTESIAN_POINT('Ctrl Pts',(-7.53666207253144,-31.741151431443,28.048430493378));
#54593=CARTESIAN_POINT('Ctrl Pts',(-7.5128274573098,-31.7594448403263,28.0469627561459));
#54594=CARTESIAN_POINT('Ctrl Pts',(-7.51282745730978,-31.7594448403263,
29.2969304815276));
#54595=CARTESIAN_POINT('Ctrl Pts',(-7.41787341740872,-31.832323427242,29.2911163987806));
#54596=CARTESIAN_POINT('Ctrl Pts',(-7.32614682414379,-31.9093623605148,
29.2853023160336));
#54597=CARTESIAN_POINT('Ctrl Pts',(-7.23801917381052,-31.9902347407544,
29.2794882332866));
#54598=CARTESIAN_POINT('Ctrl Pts',(-7.1497993364812,-32.0711917185269,29.273668068648));
#54599=CARTESIAN_POINT('Ctrl Pts',(-7.06518626208406,-32.155989877465,29.2678479040093));
#54600=CARTESIAN_POINT('Ctrl Pts',(-6.9845152878803,-32.2442647168183,29.2620277393706));
#54601=CARTESIAN_POINT('Ctrl Pts',(-6.90380138944867,-32.332586526341,29.2562044778799));
#54602=CARTESIAN_POINT('Ctrl Pts',(-6.82703403156669,-32.4243883902038,
29.2503812163892));
#54603=CARTESIAN_POINT('Ctrl Pts',(-6.75450775669891,-32.5192732720688,
29.2445579548984));
#54604=CARTESIAN_POINT('Ctrl Pts',(-6.68186497780587,-32.6143105741523,
29.2387253390957));
#54605=CARTESIAN_POINT('Ctrl Pts',(-6.61347712758057,-32.7124404559656,
29.232892723293));
#54606=CARTESIAN_POINT('Ctrl Pts',(-6.54959529733578,-32.8132370069364,
29.2270601074902));
#54607=CARTESIAN_POINT('Ctrl Pts',(-6.49345298970209,-32.9018216788428,
29.2219341349022));
#54608=CARTESIAN_POINT('Ctrl Pts',(-6.44079040224357,-32.9924654483701,
29.2168081623142));
#54609=CARTESIAN_POINT('Ctrl Pts',(-6.39174772339236,-33.0848654072479,
29.2116821897262));
#54610=CARTESIAN_POINT('Ctrl Pts',(-6.33608948362485,-33.1897295620249,
29.2058647544224));
#54611=CARTESIAN_POINT('Ctrl Pts',(-6.28491481213769,-33.2971947001416,
29.2000473191185));
#54612=CARTESIAN_POINT('Ctrl Pts',(-6.2384753088229,-33.4068405611286,29.1942298838146));
#54613=CARTESIAN_POINT('Ctrl Pts',(-6.19209507835399,-33.5163464761266,
29.1884198735675));
#54614=CARTESIAN_POINT('Ctrl Pts',(-6.15043815414528,-33.6280272047772,
29.1826098633204));
#54615=CARTESIAN_POINT('Ctrl Pts',(-6.11371065222675,-33.7414372858756,
29.1767998530732));
#54616=CARTESIAN_POINT('Ctrl Pts',(-6.0770203952809,-33.8547323590058,29.1709957346963));
#54617=CARTESIAN_POINT('Ctrl Pts',(-6.04524974191319,-33.9697529088491,
29.1651916163193));
#54618=CARTESIAN_POINT('Ctrl Pts',(-6.01855678169613,-34.086033425435,29.1593874979423));
#54619=CARTESIAN_POINT('Ctrl Pts',(-5.99081258920605,-34.2068933453828,
29.1533547995763));
#54620=CARTESIAN_POINT('Ctrl Pts',(-5.96855442122842,-34.329114096242,29.1473221012103));
#54621=CARTESIAN_POINT('Ctrl Pts',(-5.9519028048853,-34.45215504118,29.1412894028443));
#54622=CARTESIAN_POINT('Ctrl Pts',(-5.93590054455395,-34.570397810635,29.1354919590548));
#54623=CARTESIAN_POINT('Ctrl Pts',(-5.92507582323453,-34.6893975602768,
29.1296945152653));
#54624=CARTESIAN_POINT('Ctrl Pts',(-5.91948339096502,-34.8086646833706,
29.1238970714758));
#54625=CARTESIAN_POINT('Ctrl Pts',(-5.91389182303259,-34.9279133731616,
29.1181005237088));
#54626=CARTESIAN_POINT('Ctrl Pts',(-5.91353095520818,-35.0474289454461,
29.1123039759419));
#54627=CARTESIAN_POINT('Ctrl Pts',(-5.91840350906871,-35.1667185809002,
29.106507428175));
#54628=CARTESIAN_POINT('Ctrl Pts',(-5.92327646679649,-35.2860181038135,
29.1007103999545));
#54629=CARTESIAN_POINT('Ctrl Pts',(-5.93338369187788,-35.4050912436341,
29.0949133717341));
#54630=CARTESIAN_POINT('Ctrl Pts',(-5.94867583996883,-35.5234477532168,
29.0891163435136));
#54631=CARTESIAN_POINT('Ctrl Pts',(-5.9639728865431,-35.6418421755495,29.0833174583502));
#54632=CARTESIAN_POINT('Ctrl Pts',(-5.9844581065806,-35.7595191053679,29.0775185731868));
#54633=CARTESIAN_POINT('Ctrl Pts',(-6.01003071138977,-35.8759966186848,
29.0717196880234));
#54634=CARTESIAN_POINT('Ctrl Pts',(-6.03563164690813,-35.9926031720654,
29.0659143785427));
#54635=CARTESIAN_POINT('Ctrl Pts',(-6.06633112931651,-36.1080072565552,
29.0601090690619));
#54636=CARTESIAN_POINT('Ctrl Pts',(-6.10197793524993,-36.2217401453344,
29.0543037595812));
#54637=CARTESIAN_POINT('Ctrl Pts',(-6.13764811609673,-36.3355476129251,
29.0484946433469));
#54638=CARTESIAN_POINT('Ctrl Pts',(-6.17827194175445,-36.4476813185244,
29.0426855271125));
#54639=CARTESIAN_POINT('Ctrl Pts',(-6.22364990453442,-36.5576921892585,
29.0368764108782));
#54640=CARTESIAN_POINT('Ctrl Pts',(-6.26909320861608,-36.6678614684592,
29.031058929896));
#54641=CARTESIAN_POINT('Ctrl Pts',(-6.31930414123014,-36.7759014419196,
29.0252414489138));
#54642=CARTESIAN_POINT('Ctrl Pts',(-6.37403706152266,-36.8813871926822,
29.0194239679316));
#54643=CARTESIAN_POINT('Ctrl Pts',(-6.38915701008606,-36.9105275914985,
29.017816891007));
#54644=CARTESIAN_POINT('Ctrl Pts',(-6.4046217940718,-36.9394732379555,29.0162098140824));
#54645=CARTESIAN_POINT('Ctrl Pts',(-6.42042566271007,-36.9682155785928,
29.0146027371578));
#54646=CARTESIAN_POINT('Ctrl Pts',(-6.47770516985146,-37.0723892555243,
29.0087780510453));
#54647=CARTESIAN_POINT('Ctrl Pts',(-6.53962813183109,-37.1742280035309,
29.0029533649328));
#54648=CARTESIAN_POINT('Ctrl Pts',(-6.60597947346715,-37.2732904929801,
28.9971286788204));
#54649=CARTESIAN_POINT('Ctrl Pts',(-6.67224714861135,-37.3722280684371,
28.9913113374133));
#54650=CARTESIAN_POINT('Ctrl Pts',(-6.74293187168987,-37.468396012181,28.9854939960061));
#54651=CARTESIAN_POINT('Ctrl Pts',(-6.81777261894665,-37.5613773433983,
28.979676654599));
#54652=CARTESIAN_POINT('Ctrl Pts',(-6.89253848033271,-37.6542656372235,
28.9738651340407));
#54653=CARTESIAN_POINT('Ctrl Pts',(-6.97145183848653,-37.7439733456366,
28.9680536134824));
#54654=CARTESIAN_POINT('Ctrl Pts',(-7.05420864111179,-37.8301127662868,
28.9622420929242));
#54655=CARTESIAN_POINT('Ctrl Pts',(-7.14007591211693,-37.9194897932207,
28.9562121425769));
#54656=CARTESIAN_POINT('Ctrl Pts',(-7.23008096474498,-38.0050246637825,
28.9501821922296));
#54657=CARTESIAN_POINT('Ctrl Pts',(-7.32383828549135,-38.0863219983984,
28.9441522418823));
#54658=CARTESIAN_POINT('Ctrl Pts',(-7.41409757504367,-38.1645861766676,
28.938347265481));
#54659=CARTESIAN_POINT('Ctrl Pts',(-7.50783382180515,-38.2389230643019,
28.9325422890797));
#54660=CARTESIAN_POINT('Ctrl Pts',(-7.60466636419906,-38.3090182491489,
28.9267373126784));
#54661=CARTESIAN_POINT('Ctrl Pts',(-7.70148454807795,-38.3791030401476,
28.9209331970501));
#54662=CARTESIAN_POINT('Ctrl Pts',(-7.80139778398777,-38.4449471399261,
28.9151290814219));
#54663=CARTESIAN_POINT('Ctrl Pts',(-7.90399425341895,-38.5062779282737,
28.9093249657936));
#54664=CARTESIAN_POINT('Ctrl Pts',(-8.00659969626102,-38.5676140808055,
28.9035203425191));
#54665=CARTESIAN_POINT('Ctrl Pts',(-8.11188848888147,-38.6244359276154,
28.8977157192445));
#54666=CARTESIAN_POINT('Ctrl Pts',(-8.21942246366639,-38.6765158284855,
28.89191109597));
#54667=CARTESIAN_POINT('Ctrl Pts',(-8.32699119414061,-38.7286125619227,
28.886104596603));
#54668=CARTESIAN_POINT('Ctrl Pts',(-8.4368061828024,-38.7759641235285,28.8802980972359));
#54669=CARTESIAN_POINT('Ctrl Pts',(-8.5484080513187,-38.8183904743391,28.8744915978689));
#54670=CARTESIAN_POINT('Ctrl Pts',(-8.66013321073938,-38.8608636951818,
28.8686786838373));
#54671=CARTESIAN_POINT('Ctrl Pts',(-8.77364880862195,-38.89840069923,28.8628657698056));
#54672=CARTESIAN_POINT('Ctrl Pts',(-8.88847887613864,-38.9308708693125,
28.857052855774));
#54673=CARTESIAN_POINT('Ctrl Pts',(-9.0033842106199,-38.9633623224196,28.851236131587));
#54674=CARTESIAN_POINT('Ctrl Pts',(-9.11960533428275,-38.9907802338579,
28.8454194074));
#54675=CARTESIAN_POINT('Ctrl Pts',(-9.23665624722748,-39.0130451424203,
28.839602683213));
#54676=CARTESIAN_POINT('Ctrl Pts',(-9.35387441984046,-39.0353418663793,
28.8337776472296));
#54677=CARTESIAN_POINT('Ctrl Pts',(-9.47192434588376,-39.0524708321049,
28.8279526112462));
#54678=CARTESIAN_POINT('Ctrl Pts',(-9.59031493431379,-39.0644044024868,
28.8221275752628));
#54679=CARTESIAN_POINT('Ctrl Pts',(-9.62150814260123,-39.0675486249412,
28.820592811705));
#54680=CARTESIAN_POINT('Ctrl Pts',(-9.65272500215769,-39.0703324629713,
28.8190580481471));
#54681=CARTESIAN_POINT('Ctrl Pts',(-9.68395655113767,-39.0727560126321,
28.8175232845893));
#54682=CARTESIAN_POINT('Ctrl Pts',(-9.8024827349867,-39.0819535741379,28.811698736222));
#54683=CARTESIAN_POINT('Ctrl Pts',(-9.92160113173807,-39.0859875553614,
28.8058741878547));
#54684=CARTESIAN_POINT('Ctrl Pts',(-10.0408247254744,-39.0847959975732,
28.8000496394874));
#54685=CARTESIAN_POINT('Ctrl Pts',(-10.1598983033553,-39.0836059390902,
28.7942324199933));
#54686=CARTESIAN_POINT('Ctrl Pts',(-10.2790764103628,-39.0772034235936,
28.7884152004993));
#54687=CARTESIAN_POINT('Ctrl Pts',(-10.397867218127,-39.0655782708909,28.7825979810052));
#54688=CARTESIAN_POINT('Ctrl Pts',(-10.5165394860414,-39.0539647187814,
28.7767865664411));
#54689=CARTESIAN_POINT('Ctrl Pts',(-10.6348248196585,-39.0371389369318,
28.7709751518771));
#54690=CARTESIAN_POINT('Ctrl Pts',(-10.7522323021061,-39.0151427824759,
28.765163737313));
#54691=CARTESIAN_POINT('Ctrl Pts',(-10.8740557666081,-38.9923192989492,
28.7591337412592));
#54692=CARTESIAN_POINT('Ctrl Pts',(-10.9949335990444,-38.9639288690956,
28.7531037452054));
#54693=CARTESIAN_POINT('Ctrl Pts',(-11.1143237843018,-38.9300772897921,
28.7470737491515));
#54694=CARTESIAN_POINT('Ctrl Pts',(-11.2292574283504,-38.8974893064685,
28.7412688379809));
#54695=CARTESIAN_POINT('Ctrl Pts',(-11.3428120677675,-38.8598406916114,
28.7354639268102));
#54696=CARTESIAN_POINT('Ctrl Pts',(-11.4545161092082,-38.817277549256,28.7296590156396));
#54697=CARTESIAN_POINT('Ctrl Pts',(-11.5662038803135,-38.7747206064668,
28.7238549499876));
#54698=CARTESIAN_POINT('Ctrl Pts',(-11.6760412081702,-38.7272507050453,
28.7180508843356));
#54699=CARTESIAN_POINT('Ctrl Pts',(-11.7835743848829,-38.675062912875,28.7122468186836));
#54700=CARTESIAN_POINT('Ctrl Pts',(-11.8911172519402,-38.6228704178056,
28.7064422299986));
#54701=CARTESIAN_POINT('Ctrl Pts',(-11.9963551877746,-38.5659593648881,
28.7006376413137));
#54702=CARTESIAN_POINT('Ctrl Pts',(-12.098857671488,-38.5045715108749,28.6948330526287));
#54703=CARTESIAN_POINT('Ctrl Pts',(-12.201393559125,-38.4431636515397,28.689026572321));
#54704=CARTESIAN_POINT('Ctrl Pts',(-12.301191871747,-38.3772762992261,28.6832200920132));
#54705=CARTESIAN_POINT('Ctrl Pts',(-12.3978502839748,-38.3071950374361,
28.6774136117054));
#54706=CARTESIAN_POINT('Ctrl Pts',(-12.4946158665635,-38.237036072796,28.6716006934418));
#54707=CARTESIAN_POINT('Ctrl Pts',(-12.5882342689691,-38.1626741565788,
28.6657877751782));
#54708=CARTESIAN_POINT('Ctrl Pts',(-12.6783354146374,-38.0844358328062,
28.6599748569146));
#54709=CARTESIAN_POINT('Ctrl Pts',(-12.7684958290091,-38.0061460437169,
28.6541581149023));
#54710=CARTESIAN_POINT('Ctrl Pts',(-12.8551340834213,-37.9239750490683,
28.6483413728901));
#54711=CARTESIAN_POINT('Ctrl Pts',(-12.9379173972012,-37.8382858149282,
28.6425246308779));
#54712=CARTESIAN_POINT('Ctrl Pts',(-13.0208192870192,-37.7524738424073,
28.6366995571598));
#54713=CARTESIAN_POINT('Ctrl Pts',(-13.0998549457001,-37.663133876622,28.6308744834417));
#54714=CARTESIAN_POINT('Ctrl Pts',(-13.1747321532766,-37.5706615403338,
28.6250494097237));
#54715=CARTESIAN_POINT('Ctrl Pts',(-13.1944659692104,-37.546290545176,28.6235142171561));
#54716=CARTESIAN_POINT('Ctrl Pts',(-13.2139111834488,-37.5217021334563,
28.6219790245885));
#54717=CARTESIAN_POINT('Ctrl Pts',(-13.2330629616497,-37.4969038599851,
28.6204438320209));
#54718=CARTESIAN_POINT('Ctrl Pts',(-13.3056934675164,-37.4028597911819,
28.6146218236613));
#54719=CARTESIAN_POINT('Ctrl Pts',(-13.3743388331657,-37.3054865730966,
28.6087998153017));
#54720=CARTESIAN_POINT('Ctrl Pts',(-13.4386789137847,-37.205155851157,28.6029778069421));
#54721=CARTESIAN_POINT('Ctrl Pts',(-13.5029393673578,-37.1049492981481,
28.5971630038786));
#54722=CARTESIAN_POINT('Ctrl Pts',(-13.5629049116448,-37.0017928584942,
28.591348200815));
#54723=CARTESIAN_POINT('Ctrl Pts',(-13.6182957848243,-36.8960908769156,
28.5855333977514));
#54724=CARTESIAN_POINT('Ctrl Pts',(-13.6736311609314,-36.7904947999777,
28.5797244206395));
#54725=CARTESIAN_POINT('Ctrl Pts',(-13.7244007929045,-36.6823586120928,
28.5739154435275));
#54726=CARTESIAN_POINT('Ctrl Pts',(-13.7703687222174,-36.5721147218077,
28.5681064664156));
#54727=CARTESIAN_POINT('Ctrl Pts',(-13.8163014268996,-36.4619553099924,
28.5623019406478));
#54728=CARTESIAN_POINT('Ctrl Pts',(-13.8574395920708,-36.349691783766,28.55649741488));
#54729=CARTESIAN_POINT('Ctrl Pts',(-13.8935939351083,-36.235779619709,28.5506928891122));
#54730=CARTESIAN_POINT('Ctrl Pts',(-13.9297311667015,-36.1219213689992,
28.5448911105612));
#54731=CARTESIAN_POINT('Ctrl Pts',(-13.9608891443664,-36.0064164204851,
28.5390893320103));
#54732=CARTESIAN_POINT('Ctrl Pts',(-13.9869275256978,-35.889738110251,28.5332875534593));
#54733=CARTESIAN_POINT('Ctrl Pts',(-14.0129585926891,-35.7730925756662,
28.5274874046633));
#54734=CARTESIAN_POINT('Ctrl Pts',(-14.0338728387506,-35.6552747337021,
28.5216872558673));
#54735=CARTESIAN_POINT('Ctrl Pts',(-14.0495805642629,-35.5367702055292,
28.5158871070713));
#54736=CARTESIAN_POINT('Ctrl Pts',(-14.0652908719406,-35.4182461966059,
28.5100860047991));
#54737=CARTESIAN_POINT('Ctrl Pts',(-14.0757928938376,-35.2990356802547,
28.5042849025269));
#54738=CARTESIAN_POINT('Ctrl Pts',(-14.081048594519,-35.1796312032315,28.4984838002547));
#54739=CARTESIAN_POINT('Ctrl Pts',(-14.0837269136306,-35.1187823626656,
28.495527543035));
#54740=CARTESIAN_POINT('Ctrl Pts',(-14.0850436239602,-35.0578832208542,
28.4925712858152));
#54741=CARTESIAN_POINT('Ctrl Pts',(-14.0849988977552,-34.9969991103314,
28.4896150285955));
#54742=CARTESIAN_POINT('Origin',(130.,-35.,23.));
#54743=CARTESIAN_POINT('',(126.610250000496,-34.9999420099749,27.6441864590851));
#54744=CARTESIAN_POINT('Ctrl Pts',(126.821241915871,-33.8227565650717,28.8235739384178));
#54745=CARTESIAN_POINT('Ctrl Pts',(126.833574063551,-33.7894576627623,28.8214368686364));
#54746=CARTESIAN_POINT('Ctrl Pts',(126.846428176058,-33.7563559586685,28.8192724775167));
#54747=CARTESIAN_POINT('Ctrl Pts',(126.914370105375,-33.5892229961455,28.8081615787155));
#54748=CARTESIAN_POINT('Ctrl Pts',(126.977488607444,-33.4586298771998,28.798883276182));
#54749=CARTESIAN_POINT('Ctrl Pts',(127.181890612654,-33.0968701903928,28.7721255757395));
#54750=CARTESIAN_POINT('Ctrl Pts',(127.342781726071,-32.8780004792562,28.7546974138192));
#54751=CARTESIAN_POINT('Ctrl Pts',(127.561298209235,-32.6451104996121,28.7353264702612));
#54752=CARTESIAN_POINT('Ctrl Pts',(127.595341200996,-32.6103583090058,28.7324071488727));
#54753=CARTESIAN_POINT('Ctrl Pts',(127.651025511273,-32.5559094379489,28.7277842454063));
#54754=CARTESIAN_POINT('Ctrl Pts',(127.672193326602,-32.5357402743224,28.7260604886461));
#54755=CARTESIAN_POINT('Ctrl Pts',(127.713170329732,-32.4976957000816,28.7227860420401));
#54756=CARTESIAN_POINT('Ctrl Pts',(127.732934709085,-32.4797754511263,28.7212335297737));
#54757=CARTESIAN_POINT('Ctrl Pts',(127.779220933771,-32.4387931629945,28.7176579720437));
#54758=CARTESIAN_POINT('Ctrl Pts',(127.805894228396,-32.4159063257433,28.7156421643936));
#54759=CARTESIAN_POINT('Ctrl Pts',(127.894979746538,-32.3418411441775,28.7090495750105));
#54760=CARTESIAN_POINT('Ctrl Pts',(127.958865893956,-32.2924749854509,28.7045435396024));
#54761=CARTESIAN_POINT('Ctrl Pts',(128.121890932563,-32.1755553209706,28.6935119610474));
#54762=CARTESIAN_POINT('Ctrl Pts',(128.222967706627,-32.110892840549,28.6870781766475));
#54763=CARTESIAN_POINT('Ctrl Pts',(128.540676710504,-31.9306373441203,28.6676416436425));
#54764=CARTESIAN_POINT('Ctrl Pts',(128.766580194337,-31.833099526583,28.6549010351605));
#54765=CARTESIAN_POINT('Ctrl Pts',(129.034179783342,-31.7505689400022,28.6390803993295));
#54766=CARTESIAN_POINT('Ctrl Pts',(129.06751669369,-31.7408458776975,28.6370963631631));
#54767=CARTESIAN_POINT('Ctrl Pts',(129.118424733512,-31.7268429817674,28.6340385651005));
#54768=CARTESIAN_POINT('Ctrl Pts',(129.135891400908,-31.722188517689,28.6329844533612));
#54769=CARTESIAN_POINT('Ctrl Pts',(129.167867824993,-31.7139408810249,28.6310442266637));
#54770=CARTESIAN_POINT('Ctrl Pts',(129.182365306507,-31.7103036657101,28.6301605524467));
#54771=CARTESIAN_POINT('Ctrl Pts',(129.216088215963,-31.7020797438125,28.6280958626424));
#54772=CARTESIAN_POINT('Ctrl Pts',(129.235330149403,-31.6975651892273,28.626911017215));
#54773=CARTESIAN_POINT('Ctrl Pts',(129.298618259288,-31.6832992514724,28.6229943141593));
#54774=CARTESIAN_POINT('Ctrl Pts',(129.342818030257,-31.6742592338015,28.620227818892));
#54775=CARTESIAN_POINT('Ctrl Pts',(129.45257805719,-31.6540837830903,28.6133025239753));
#54776=CARTESIAN_POINT('Ctrl Pts',(129.518309811019,-31.6439904968777,28.6091069424881));
#54777=CARTESIAN_POINT('Ctrl Pts',(129.856418489977,-31.6022105947466,28.5874085795202));
#54778=CARTESIAN_POINT('Ctrl Pts',(130.131665077691,-31.6017232560519,28.5694648690226));
#54779=CARTESIAN_POINT('Ctrl Pts',(130.489187791843,-31.6446359471021,28.547088761069));
#54780=CARTESIAN_POINT('Ctrl Pts',(130.573996323768,-31.6580989268164,28.5418407029634));
#54781=CARTESIAN_POINT('Ctrl Pts',(130.690774407546,-31.6812143947729,28.5346984816899));
#54782=CARTESIAN_POINT('Ctrl Pts',(130.723244998124,-31.688138896954,28.5327215419536));
#54783=CARTESIAN_POINT('Ctrl Pts',(130.779650631762,-31.7010368067049,28.5293020596601));
#54784=CARTESIAN_POINT('Ctrl Pts',(130.803631495735,-31.7067964342686,28.5278529346695));
#54785=CARTESIAN_POINT('Ctrl Pts',(130.854011927271,-31.7194797021652,28.5248176494911));
#54786=CARTESIAN_POINT('Ctrl Pts',(130.880395126734,-31.7264615045877,28.523233452141));
#54787=CARTESIAN_POINT('Ctrl Pts',(130.944222511583,-31.7441796710833,28.5194123474784));
#54788=CARTESIAN_POINT('Ctrl Pts',(130.981571980668,-31.7552444176918,28.5171860458989));
#54789=CARTESIAN_POINT('Ctrl Pts',(131.122629814511,-31.7996912944836,28.508806063024));
#54790=CARTESIAN_POINT('Ctrl Pts',(131.224902737554,-31.8374235430999,28.5027910199424));
#54791=CARTESIAN_POINT('Ctrl Pts',(131.510552545927,-31.958751105075,28.4859516864678));
#54792=CARTESIAN_POINT('Ctrl Pts',(131.688528669577,-32.053843998535,28.4754308592064));
#54793=CARTESIAN_POINT('Ctrl Pts',(131.972640357157,-32.2398916211758,28.4572891109635));
#54794=CARTESIAN_POINT('Ctrl Pts',(132.083518499994,-32.3226036463769,28.4498021488128));
#54795=CARTESIAN_POINT('Ctrl Pts',(132.210556912132,-32.4300509138175,28.4403260785439));
#54796=CARTESIAN_POINT('Ctrl Pts',(132.231857693392,-32.4485276223424,28.4387044597264));
#54797=CARTESIAN_POINT('Ctrl Pts',(132.26525450511,-32.4782348640848,28.4361049623113));
#54798=CARTESIAN_POINT('Ctrl Pts',(132.277503724703,-32.4892921052566,28.4351390674826));
#54799=CARTESIAN_POINT('Ctrl Pts',(132.301011118523,-32.5108255619939,28.4332600906378));
#54800=CARTESIAN_POINT('Ctrl Pts',(132.312279512588,-32.5212896555105,28.4323478431613));
#54801=CARTESIAN_POINT('Ctrl Pts',(132.340103641754,-32.5474826196449,28.4300672100993));
#54802=CARTESIAN_POINT('Ctrl Pts',(132.356572224356,-32.5633026769439,28.4286922832698));
#54803=CARTESIAN_POINT('Ctrl Pts',(132.420574008729,-32.6260397841033,28.4232541322682));
#54804=CARTESIAN_POINT('Ctrl Pts',(132.466873568129,-32.6741884779096,28.4191116954963));
#54805=CARTESIAN_POINT('Ctrl Pts',(132.592778907574,-32.8131132428913,28.4073206183791));
#54806=CARTESIAN_POINT('Ctrl Pts',(132.669001151531,-32.9068190616157,28.3995527310962));
#54807=CARTESIAN_POINT('Ctrl Pts',(132.88493735272,-33.2033082280161,28.3759111475075));
#54808=CARTESIAN_POINT('Ctrl Pts',(133.00774475201,-33.4174476411746,28.3601300090901));
#54809=CARTESIAN_POINT('Ctrl Pts',(133.126745709506,-33.689855706075,28.342055373861));
#54810=CARTESIAN_POINT('Ctrl Pts',(133.146143090254,-33.7371457392357,28.3389820605837));
#54811=CARTESIAN_POINT('Ctrl Pts',(133.175225334764,-33.812881542665,28.3341594122556));
#54812=CARTESIAN_POINT('Ctrl Pts',(133.185613668949,-33.8410471117028,28.3323872630832));
#54813=CARTESIAN_POINT('Ctrl Pts',(133.204466835758,-33.8943328847204,28.3290735426164));
#54814=CARTESIAN_POINT('Ctrl Pts',(133.213013770499,-33.9194214324476,28.3275293936847));
#54815=CARTESIAN_POINT('Ctrl Pts',(133.23175051388,-33.9766097001116,28.3240446763439));
#54816=CARTESIAN_POINT('Ctrl Pts',(133.241758054909,-34.0087664656775,28.3221101037009));
#54817=CARTESIAN_POINT('Ctrl Pts',(133.271601419392,-34.1099511904523,28.3160959606109));
#54818=CARTESIAN_POINT('Ctrl Pts',(133.289724486876,-34.1794657058512,28.3120704463795));
#54819=CARTESIAN_POINT('Ctrl Pts',(133.327968512637,-34.3479156109979,28.3025241585312));
#54820=CARTESIAN_POINT('Ctrl Pts',(133.345906057418,-34.4472767692154,28.2970640277362));
#54821=CARTESIAN_POINT('Ctrl Pts',(133.376405108925,-34.6736006892021,28.2848425324381));
#54822=CARTESIAN_POINT('Ctrl Pts',(133.38628910921,-34.8007657868358,28.2781277359795));
#54823=CARTESIAN_POINT('Ctrl Pts',(133.392138767068,-35.0768172722747,28.2634418490839));
#54824=CARTESIAN_POINT('Ctrl Pts',(133.385506759669,-35.2254816572142,28.2554636453605));
#54825=CARTESIAN_POINT('Ctrl Pts',(133.365194542982,-35.4088471412835,28.2450490854384));
#54826=CARTESIAN_POINT('Ctrl Pts',(133.360682542202,-35.4444130213191,28.2430017329154));
#54827=CARTESIAN_POINT('Ctrl Pts',(133.353048190738,-35.497794836456,28.23987877211));
#54828=CARTESIAN_POINT('Ctrl Pts',(133.350345799082,-35.5156693352137,28.2388245935552));
#54829=CARTESIAN_POINT('Ctrl Pts',(133.345148625611,-35.5482782558593,28.2368845377422));
#54830=CARTESIAN_POINT('Ctrl Pts',(133.34269919995,-35.5630190100192,28.2360011060033));
#54831=CARTESIAN_POINT('Ctrl Pts',(133.336786124291,-35.5972047483972,28.2339375059085));
#54832=CARTESIAN_POINT('Ctrl Pts',(133.333249917837,-35.6166361119619,28.2327535167855));
#54833=CARTESIAN_POINT('Ctrl Pts',(133.321094071103,-35.6802700831552,28.2288424149936));
#54834=CARTESIAN_POINT('Ctrl Pts',(133.311763656093,-35.7243302334475,28.2260807907919));
#54835=CARTESIAN_POINT('Ctrl Pts',(133.286526800118,-35.8327943668122,28.2191705954585));
#54836=CARTESIAN_POINT('Ctrl Pts',(133.269602443916,-35.8969413793448,28.214985427496));
#54837=CARTESIAN_POINT('Ctrl Pts',(133.173703284366,-36.2214957508718,28.1934320970228));
#54838=CARTESIAN_POINT('Ctrl Pts',(133.065443947851,-36.4722528640407,28.1756258173543));
#54839=CARTESIAN_POINT('Ctrl Pts',(132.884147298716,-36.7832008180712,28.1532397239967));
#54840=CARTESIAN_POINT('Ctrl Pts',(132.837000973545,-36.8572932845562,28.1478693089175));
#54841=CARTESIAN_POINT('Ctrl Pts',(132.765943672843,-36.959931809334,28.1403782003703));
#54842=CARTESIAN_POINT('Ctrl Pts',(132.744361227893,-36.9900398771756,28.1381739233098));
#54843=CARTESIAN_POINT('Ctrl Pts',(132.706226242686,-37.0414385359868,28.1343975875296));
#54844=CARTESIAN_POINT('Ctrl Pts',(132.689905509209,-37.0628960678669,28.1328169252894));
#54845=CARTESIAN_POINT('Ctrl Pts',(132.655821739017,-37.1066150234773,28.1295867909048));
#54846=CARTESIAN_POINT('Ctrl Pts',(132.638030625693,-37.128851910383,28.1279385881348));
#54847=CARTESIAN_POINT('Ctrl Pts',(132.591425718131,-37.1856212492617,28.1237152429296));
#54848=CARTESIAN_POINT('Ctrl Pts',(132.562200668219,-37.2198097891668,28.1211566173981));
#54849=CARTESIAN_POINT('Ctrl Pts',(132.400324077677,-37.4017211869068,28.1074384328021));
#54850=CARTESIAN_POINT('Ctrl Pts',(132.255566357925,-37.5381592034005,28.0967978208873));
#54851=CARTESIAN_POINT('Ctrl Pts',(131.932366639642,-37.7931679873723,28.0749434529271));
#54852=CARTESIAN_POINT('Ctrl Pts',(131.752988760412,-37.9090961702754,28.0637879604533));
#54853=CARTESIAN_POINT('Ctrl Pts',(131.525782287855,-38.0272500903273,28.0494316278816));
#54854=CARTESIAN_POINT('Ctrl Pts',(131.487253482213,-38.0463636396839,28.0469889181108));
#54855=CARTESIAN_POINT('Ctrl Pts',(131.431015780375,-38.0729411767222,28.0433970359435));
#54856=CARTESIAN_POINT('Ctrl Pts',(131.41358924603,-38.080996437068,28.0422803975341));
#54857=CARTESIAN_POINT('Ctrl Pts',(131.382491333171,-38.0950518027564,28.0402797299016));
#54858=CARTESIAN_POINT('Ctrl Pts',(131.368847325059,-38.1011102745544,28.0393991576625));
#54859=CARTESIAN_POINT('Ctrl Pts',(131.338430368373,-38.114376738193,28.0374295816383));
#54860=CARTESIAN_POINT('Ctrl Pts',(131.321639112141,-38.1215394186853,28.0363381096993));
#54861=CARTESIAN_POINT('Ctrl Pts',(131.270863821115,-38.1427156241531,28.0330267861333));
#54862=CARTESIAN_POINT('Ctrl Pts',(131.236709926645,-38.1563118773537,28.0307849513599));
#54863=CARTESIAN_POINT('Ctrl Pts',(131.155458911971,-38.1871357451455,28.0254288223517));
#54864=CARTESIAN_POINT('Ctrl Pts',(131.108187739638,-38.2038787484316,28.0222948190829));
#54865=CARTESIAN_POINT('Ctrl Pts',(130.924509054455,-38.2643847731338,28.0100921214553));
#54866=CARTESIAN_POINT('Ctrl Pts',(130.785753795227,-38.3005322689072,28.0008278114887));
#54867=CARTESIAN_POINT('Ctrl Pts',(130.437288270604,-38.3680865832329,27.97796250853));
#54868=CARTESIAN_POINT('Ctrl Pts',(130.226098857396,-38.38882440937,27.9644806993655));
#54869=CARTESIAN_POINT('Ctrl Pts',(129.961456414662,-38.3899432452389,27.9483678954458));
#54870=CARTESIAN_POINT('Ctrl Pts',(129.908581967943,-38.3889296286348,27.9451848810891));
#54871=CARTESIAN_POINT('Ctrl Pts',(129.825379583772,-38.3853857744695,27.940231192331));
#54872=CARTESIAN_POINT('Ctrl Pts',(129.79502668014,-38.383683667258,27.9384355684792));
#54873=CARTESIAN_POINT('Ctrl Pts',(129.738307450002,-38.3797369738032,27.9351006612185));
#54874=CARTESIAN_POINT('Ctrl Pts',(129.71193675565,-38.3775915425938,27.9335584555133));
#54875=CARTESIAN_POINT('Ctrl Pts',(129.652628559471,-38.3720667623539,27.930107556462));
#54876=CARTESIAN_POINT('Ctrl Pts',(129.619709768729,-38.3685131168181,27.9282043773497));
#54877=CARTESIAN_POINT('Ctrl Pts',(129.518788811183,-38.3561201829704,27.9224032998985));
#54878=CARTESIAN_POINT('Ctrl Pts',(129.450996586785,-38.3456991824849,27.9185538895824));
#54879=CARTESIAN_POINT('Ctrl Pts',(129.290672756162,-38.3160494238967,27.9095255495407));
#54880=CARTESIAN_POINT('Ctrl Pts',(129.198536670883,-38.2949942421069,27.9043981749614));
#54881=CARTESIAN_POINT('Ctrl Pts',(128.89490598293,-38.2121158915519,27.887509774008));
#54882=CARTESIAN_POINT('Ctrl Pts',(128.688587700696,-38.1335459414615,27.8760771398493));
#54883=CARTESIAN_POINT('Ctrl Pts',(128.414656411637,-37.9974034243499,27.859426531554));
#54884=CARTESIAN_POINT('Ctrl Pts',(128.339431767106,-37.9563918011335,27.8546816818741));
#54885=CARTESIAN_POINT('Ctrl Pts',(128.243997620173,-37.8995701974791,27.8483322501311));
#54886=CARTESIAN_POINT('Ctrl Pts',(128.222296141297,-37.8863160943402,27.8468654561853));
#54887=CARTESIAN_POINT('Ctrl Pts',(128.18726627644,-37.8643768094663,27.8444568225998));
#54888=CARTESIAN_POINT('Ctrl Pts',(128.173845914495,-37.8558395075002,27.843524111636));
#54889=CARTESIAN_POINT('Ctrl Pts',(128.147207344192,-37.8386289605609,27.8416518134364));
#54890=CARTESIAN_POINT('Ctrl Pts',(128.133988757082,-37.82995707004,27.8407123166043));
#54891=CARTESIAN_POINT('Ctrl Pts',(128.10004244536,-37.8073457742072,27.8382736025057));
#54892=CARTESIAN_POINT('Ctrl Pts',(128.07940761048,-37.7932693745054,27.8367658989528));
#54893=CARTESIAN_POINT('Ctrl Pts',(127.986697023176,-37.7285123345843,27.8298833731564));
#54894=CARTESIAN_POINT('Ctrl Pts',(127.916463262321,-37.6752645928473,27.8243695214119));
#54895=CARTESIAN_POINT('Ctrl Pts',(127.689682256208,-37.4889797805725,27.805740958767));
#54896=CARTESIAN_POINT('Ctrl Pts',(127.543151642975,-37.3444590254826,27.792345641333));
#54897=CARTESIAN_POINT('Ctrl Pts',(127.31325831958,-37.0723359830616,27.769667198596));
#54898=CARTESIAN_POINT('Ctrl Pts',(127.223705754414,-36.9507324731433,27.7602541048155));
#54899=CARTESIAN_POINT('Ctrl Pts',(127.119024550753,-36.7866999832605,27.7485000919317));
#54900=CARTESIAN_POINT('Ctrl Pts',(127.096220091915,-36.7493938614791,27.7458846883742));
#54901=CARTESIAN_POINT('Ctrl Pts',(127.059893240694,-36.6872977410977,27.7416236174423));
#54902=CARTESIAN_POINT('Ctrl Pts',(127.045948027024,-36.6627622909291,27.7399630554176));
#54903=CARTESIAN_POINT('Ctrl Pts',(127.01921739195,-36.6143339870321,27.736729338175));
#54904=CARTESIAN_POINT('Ctrl Pts',(127.006408884253,-36.5904563723308,27.7351554585054));
#54905=CARTESIAN_POINT('Ctrl Pts',(126.976393484072,-36.5328541678085,27.7314060545317));
#54906=CARTESIAN_POINT('Ctrl Pts',(126.959462393848,-36.4989894900393,27.7292401466531));
#54907=CARTESIAN_POINT('Ctrl Pts',(126.899928201952,-36.374751302794,27.72142502383));
#54908=CARTESIAN_POINT('Ctrl Pts',(126.86075670556,-36.282786136086,27.7158902365737));
#54909=CARTESIAN_POINT('Ctrl Pts',(126.765709302514,-36.0290828060731,27.7011331877452));
#54910=CARTESIAN_POINT('Ctrl Pts',(126.717917927243,-35.8646316876755,27.6921206186954));
#54911=CARTESIAN_POINT('Ctrl Pts',(126.648436028572,-35.5340743001795,27.6741926342898));
#54912=CARTESIAN_POINT('Ctrl Pts',(126.626225508301,-35.3685797852238,27.6652999999467));
#54913=CARTESIAN_POINT('Ctrl Pts',(126.614173178845,-35.1668323622302,27.653893111756));
#54914=CARTESIAN_POINT('Ctrl Pts',(126.612616692744,-35.1314930595958,27.6518737807094));
#54915=CARTESIAN_POINT('Ctrl Pts',(126.611111507407,-35.0784424023675,27.6488020920364));
#54916=CARTESIAN_POINT('Ctrl Pts',(126.610748086028,-35.0607442141275,27.6477706215128));
#54917=CARTESIAN_POINT('Ctrl Pts',(126.610410284175,-35.0341444448989,27.6462091799433));
#54918=CARTESIAN_POINT('Ctrl Pts',(126.610332314739,-35.0252441494281,27.6456848355043));
#54919=CARTESIAN_POINT('Ctrl Pts',(126.610263040116,-35.0108764159749,27.644835224476));
#54920=CARTESIAN_POINT('Ctrl Pts',(126.610249906966,-35.0054091932058,27.6445111982693));
#54921=CARTESIAN_POINT('Ctrl Pts',(126.610250000496,-34.9999420099749,27.6441864590851));
#54922=CARTESIAN_POINT('Ctrl Pts',(126.610250000487,-34.9999425486175,27.6441864910793));
#54923=CARTESIAN_POINT('Ctrl Pts',(126.610250211739,-34.9874782475485,27.6434461379204));
#54924=CARTESIAN_POINT('Ctrl Pts',(126.610319170897,-34.9750142253258,27.6427020834383));
#54925=CARTESIAN_POINT('Ctrl Pts',(126.610721397634,-34.938608265017,27.6405184802462));
#54926=CARTESIAN_POINT('Ctrl Pts',(126.611239599136,-34.9146696669379,27.6390696402569));
#54927=CARTESIAN_POINT('Ctrl Pts',(126.614490498641,-34.8138647903812,27.6329193133682));
#54928=CARTESIAN_POINT('Ctrl Pts',(126.619585242127,-34.7371021297444,27.6281154409567));
#54929=CARTESIAN_POINT('Ctrl Pts',(126.648696526434,-34.44782777585,27.6097103485302));
#54930=CARTESIAN_POINT('Ctrl Pts',(126.690190415604,-34.2375741406169,27.5957488678196));
#54931=CARTESIAN_POINT('Ctrl Pts',(126.772269698362,-33.9619227091561,27.5774401648129));
#54932=CARTESIAN_POINT('Ctrl Pts',(126.795624121705,-33.8919289802302,27.5727865041634));
#54933=CARTESIAN_POINT('Ctrl Pts',(126.821241909639,-33.8227565818973,27.5681924492054));
#54934=CARTESIAN_POINT('',(126.610251311733,-35.0029820949929,27.9839821967168));
#54935=CARTESIAN_POINT('Ctrl Pts',(126.821241915871,-33.8227565650715,27.9134201656876));
#54936=CARTESIAN_POINT('Ctrl Pts',(126.785588882404,-33.919025836993,27.9194241939558));
#54937=CARTESIAN_POINT('Ctrl Pts',(126.754305382504,-34.0169374341092,27.925428222224));
#54938=CARTESIAN_POINT('Ctrl Pts',(126.727532847368,-34.1160521523038,27.9314322504923));
#54939=CARTESIAN_POINT('Ctrl Pts',(126.700760123262,-34.2151675700899,27.9374363211393));
#54940=CARTESIAN_POINT('Ctrl Pts',(126.678498534611,-34.3154856987428,27.9434403917864));
#54941=CARTESIAN_POINT('Ctrl Pts',(126.660838976266,-34.4165544412042,27.9494444624335));
#54942=CARTESIAN_POINT('Ctrl Pts',(126.643163513067,-34.5177142099312,27.9554539405697));
#54943=CARTESIAN_POINT('Ctrl Pts',(126.630098428695,-34.6196255074683,27.9614634187059));
#54944=CARTESIAN_POINT('Ctrl Pts',(126.621683002295,-34.7218286040624,27.9674728968422));
#54945=CARTESIAN_POINT('Ctrl Pts',(126.613976687101,-34.8154197352465,27.9729759968004));
#54946=CARTESIAN_POINT('Ctrl Pts',(126.610168856536,-34.9092552371277,27.9784790967586));
#54947=CARTESIAN_POINT('Ctrl Pts',(126.610251311733,-35.0029820949929,27.9839821967168));
#54948=CARTESIAN_POINT('Ctrl Pts',(126.821241931958,-33.822756521634,29.1634528404117));
#54949=CARTESIAN_POINT('Ctrl Pts',(126.865650864581,-33.702844833472,29.1566721449487));
#54950=CARTESIAN_POINT('Ctrl Pts',(126.916816893519,-33.5855216471383,29.1498638995743));
#54951=CARTESIAN_POINT('Ctrl Pts',(127.017823728585,-33.3856089084275,29.137646274305));
#54952=CARTESIAN_POINT('Ctrl Pts',(127.064768592437,-33.3017514046476,29.1323182721239));
#54953=CARTESIAN_POINT('Ctrl Pts',(127.134768948841,-33.188303646206,29.124753211007));
#54954=CARTESIAN_POINT('Ctrl Pts',(127.154850188462,-33.15692782321,29.1226215173715));
#54955=CARTESIAN_POINT('Ctrl Pts',(127.190309408356,-33.1034856211516,29.1189185568259));
#54956=CARTESIAN_POINT('Ctrl Pts',(127.205440666592,-33.0812592460935,29.1173564772224));
#54957=CARTESIAN_POINT('Ctrl Pts',(127.23697965579,-33.0360960238724,29.1141356895905));
#54958=CARTESIAN_POINT('Ctrl Pts',(127.253412376225,-33.0131792726201,29.1124761148223));
#54959=CARTESIAN_POINT('Ctrl Pts',(127.2962617206,-32.9549700219748,29.1081940823907));
#54960=CARTESIAN_POINT('Ctrl Pts',(127.323083733854,-32.9199838167422,29.1055562095267));
#54961=CARTESIAN_POINT('Ctrl Pts',(127.450382364417,-32.7604791208009,29.0932234457836));
#54962=CARTESIAN_POINT('Ctrl Pts',(127.558900920604,-32.6426651286359,29.0832146986985));
#54963=CARTESIAN_POINT('Ctrl Pts',(127.819908092753,-32.3967187414527,29.0603213707334));
#54964=CARTESIAN_POINT('Ctrl Pts',(127.976190247168,-32.273451629026,29.0473619932687));
#54965=CARTESIAN_POINT('Ctrl Pts',(128.214995589976,-32.1169974486217,29.0292401220475));
#54966=CARTESIAN_POINT('Ctrl Pts',(128.289433426241,-32.0722177603212,29.0238063083829));
#54967=CARTESIAN_POINT('Ctrl Pts',(128.387227475203,-32.0183923583476,29.0170125706348));
#54968=CARTESIAN_POINT('Ctrl Pts',(128.409071749994,-32.0066796483224,29.0155164962485));
#54969=CARTESIAN_POINT('Ctrl Pts',(128.444967702716,-31.9879365260305,29.0130952867612));
#54970=CARTESIAN_POINT('Ctrl Pts',(128.458942971785,-31.9807624998397,29.0121617492703));
#54971=CARTESIAN_POINT('Ctrl Pts',(128.487168747003,-31.9665202050456,29.010295303811));
#54972=CARTESIAN_POINT('Ctrl Pts',(128.501420030712,-31.9594546271057,29.009362537866));
#54973=CARTESIAN_POINT('Ctrl Pts',(128.538583192545,-31.941354441335,29.0069536979618));
#54974=CARTESIAN_POINT('Ctrl Pts',(128.561570856652,-31.9304766786006,29.0054867549124));
#54975=CARTESIAN_POINT('Ctrl Pts',(128.662514955512,-31.8840930157107,28.9991361042091));
#54976=CARTESIAN_POINT('Ctrl Pts',(128.74168430787,-31.8512881295849,28.9943902453128));
#54977=CARTESIAN_POINT('Ctrl Pts',(129.00813747748,-31.7525375185348,28.9789228088012));
#54978=CARTESIAN_POINT('Ctrl Pts',(129.199963624613,-31.7000374467142,28.9685733775538));
#54979=CARTESIAN_POINT('Ctrl Pts',(129.55144366072,-31.6363133107145,28.9494984156279));
#54980=CARTESIAN_POINT('Ctrl Pts',(129.709378552225,-31.6190056667288,28.9408906852994));
#54981=CARTESIAN_POINT('Ctrl Pts',(129.912061082677,-31.6111031502578,28.9294549390198));
#54982=CARTESIAN_POINT('Ctrl Pts',(129.956214791871,-31.6102451837655,28.9269411478639));
#54983=CARTESIAN_POINT('Ctrl Pts',(130.028708600315,-31.6102531241889,28.922771030121));
#54984=CARTESIAN_POINT('Ctrl Pts',(130.057044108881,-31.6106115648018,28.9211303370611));
#54985=CARTESIAN_POINT('Ctrl Pts',(130.112453997717,-31.6120075110482,28.9178995791691));
#54986=CARTESIAN_POINT('Ctrl Pts',(130.13952705016,-31.6130144455984,28.9163105767614));
#54987=CARTESIAN_POINT('Ctrl Pts',(130.204204410876,-31.6161967697733,28.9124882831013));
#54988=CARTESIAN_POINT('Ctrl Pts',(130.241789604117,-31.6186746151426,28.9102458749964));
#54989=CARTESIAN_POINT('Ctrl Pts',(130.377190647787,-31.6298701035138,28.9020880662825));
#54990=CARTESIAN_POINT('Ctrl Pts',(130.474650690925,-31.6422102262792,28.8960643239744));
#54991=CARTESIAN_POINT('Ctrl Pts',(130.734308518476,-31.6866178739626,28.8796148188599));
#54992=CARTESIAN_POINT('Ctrl Pts',(130.894919092059,-31.7263442737321,28.8690037658878));
#54993=CARTESIAN_POINT('Ctrl Pts',(131.217727904092,-31.8317284950796,28.8471234106422));
#54994=CARTESIAN_POINT('Ctrl Pts',(131.3790669967,-31.8985505391931,28.8358831378486));
#54995=CARTESIAN_POINT('Ctrl Pts',(131.566289333661,-31.9936052744687,28.8229574015941));
#54996=CARTESIAN_POINT('Ctrl Pts',(131.597766866808,-32.0102152624157,28.8207890125636));
#54997=CARTESIAN_POINT('Ctrl Pts',(131.644808987484,-32.0359935351618,28.8175621701658));
#54998=CARTESIAN_POINT('Ctrl Pts',(131.660570545962,-32.0447950286094,28.8164833788081));
#54999=CARTESIAN_POINT('Ctrl Pts',(131.689276664858,-32.0611271478006,28.8145240076353));
#55000=CARTESIAN_POINT('Ctrl Pts',(131.702242295708,-32.0686179930126,28.8136411742244));
#55001=CARTESIAN_POINT('Ctrl Pts',(131.732299918191,-32.0862503554271,28.8115991880103));
#55002=CARTESIAN_POINT('Ctrl Pts',(131.749352908455,-32.0964565715465,28.8104440817585));
#55003=CARTESIAN_POINT('Ctrl Pts',(131.805326829381,-32.1306291259969,28.8066605746648));
#55004=CARTESIAN_POINT('Ctrl Pts',(131.843854335682,-32.1552336159002,28.8040691527834));
#55005=CARTESIAN_POINT('Ctrl Pts',(131.938202223027,-32.2182085597067,28.7977251899512));
#55006=CARTESIAN_POINT('Ctrl Pts',(131.993393707962,-32.2574876622457,28.794015801596));
#55007=CARTESIAN_POINT('Ctrl Pts',(132.279841935849,-32.474568543669,28.7745700720025));
#55008=CARTESIAN_POINT('Ctrl Pts',(132.488595995966,-32.6800036646978,28.7595917353172));
#55009=CARTESIAN_POINT('Ctrl Pts',(132.713973584988,-32.9677118219575,28.7394159075654));
#55010=CARTESIAN_POINT('Ctrl Pts',(132.757558151112,-33.0272557618188,28.7352845515418));
#55011=CARTESIAN_POINT('Ctrl Pts',(132.81835081605,-33.1162640606414,28.7291420893276));
#55012=CARTESIAN_POINT('Ctrl Pts',(132.837113579737,-33.144643207469,28.7271884795051));
#55013=CARTESIAN_POINT('Ctrl Pts',(132.869753033185,-33.1956642527425,28.723682165818));
#55014=CARTESIAN_POINT('Ctrl Pts',(132.883796939454,-33.2181961069571,28.7221357366294));
#55015=CARTESIAN_POINT('Ctrl Pts',(132.913059183982,-33.2663963551876,28.7188307460978));
#55016=CARTESIAN_POINT('Ctrl Pts',(132.928206093067,-33.2921052731478,28.7170697883524));
#55017=CARTESIAN_POINT('Ctrl Pts',(132.968586724072,-33.3627600730744,28.7122337149015));
#55018=CARTESIAN_POINT('Ctrl Pts',(132.993137055083,-33.4080854766099,28.7091350395298));
#55019=CARTESIAN_POINT('Ctrl Pts',(133.091671751514,-33.6003459356898,28.6960008542175));
#55020=CARTESIAN_POINT('Ctrl Pts',(133.155934954993,-33.751990174415,28.6856498456774));
#55021=CARTESIAN_POINT('Ctrl Pts',(133.288741422585,-34.1421396210965,28.6592588276333));
#55022=CARTESIAN_POINT('Ctrl Pts',(133.342616393357,-34.3846400963994,28.6430347561294));
#55023=CARTESIAN_POINT('Ctrl Pts',(133.373330469998,-34.6649975792445,28.6256832696096));
#55024=CARTESIAN_POINT('Ctrl Pts',(133.376552272186,-34.6992010139932,28.6235909713055));
#55025=CARTESIAN_POINT('Ctrl Pts',(133.380668847835,-34.7513897036637,28.6204417316801));
#55026=CARTESIAN_POINT('Ctrl Pts',(133.381941134373,-34.7693419549542,28.6193662152861));
#55027=CARTESIAN_POINT('Ctrl Pts',(133.384008393886,-34.8022230716624,28.6174115938886));
#55028=CARTESIAN_POINT('Ctrl Pts',(133.384847648285,-34.8171477837951,28.6165302587124));
#55029=CARTESIAN_POINT('Ctrl Pts',(133.386571681928,-34.8519072724532,28.6144908902231));
#55030=CARTESIAN_POINT('Ctrl Pts',(133.387380976814,-34.8717448945619,28.6133369114024));
#55031=CARTESIAN_POINT('Ctrl Pts',(133.389476902568,-34.9372459026435,28.6095560235844));
#55032=CARTESIAN_POINT('Ctrl Pts',(133.390014864614,-34.9829299873729,28.6069661183035));
#55033=CARTESIAN_POINT('Ctrl Pts',(133.389057858057,-35.0963006264341,28.6006256429669));
#55034=CARTESIAN_POINT('Ctrl Pts',(133.386459103189,-35.1639592691376,28.5969182674979));
#55035=CARTESIAN_POINT('Ctrl Pts',(133.361939831642,-35.5221489653176,28.5774948197096));
#55036=CARTESIAN_POINT('Ctrl Pts',(133.304660383949,-35.8090170149409,28.5625369696971));
#55037=CARTESIAN_POINT('Ctrl Pts',(133.187667351783,-36.1552834848121,28.5423659962037));
#55038=CARTESIAN_POINT('Ctrl Pts',(133.161635691132,-36.2247292532434,28.5382147262456));
#55039=CARTESIAN_POINT('Ctrl Pts',(133.120353455634,-36.3247489047332,28.5320493436718));
#55040=CARTESIAN_POINT('Ctrl Pts',(133.106884190087,-36.3560368202566,28.5300934798964));
#55041=CARTESIAN_POINT('Ctrl Pts',(133.082089169933,-36.4113239616813,28.5265860795067));
#55042=CARTESIAN_POINT('Ctrl Pts',(133.07094869315,-36.4354034420038,28.5250408761394));
#55043=CARTESIAN_POINT('Ctrl Pts',(133.046713591717,-36.4862123551714,28.5217417350145));
#55044=CARTESIAN_POINT('Ctrl Pts',(133.033547332127,-36.5129049453734,28.5199854463282));
#55045=CARTESIAN_POINT('Ctrl Pts',(132.996750929229,-36.585092063633,28.5151710481448));
#55046=CARTESIAN_POINT('Ctrl Pts',(132.972438231204,-36.6302280558076,28.5120896792608));
#55047=CARTESIAN_POINT('Ctrl Pts',(132.866770448989,-36.8161702651956,28.499090100135));
#55048=CARTESIAN_POINT('Ctrl Pts',(132.776369540242,-36.9515655272575,28.4888637184202));
#55049=CARTESIAN_POINT('Ctrl Pts',(132.522589336101,-37.2781481025811,28.4623892693826));
#55050=CARTESIAN_POINT('Ctrl Pts',(132.347023545526,-37.4586385631106,28.4459352946881));
#55051=CARTESIAN_POINT('Ctrl Pts',(132.127078864026,-37.6395224514217,28.4284255514894));
#55052=CARTESIAN_POINT('Ctrl Pts',(132.10070214109,-37.6605627159295,28.4263716321593));
#55053=CARTESIAN_POINT('Ctrl Pts',(132.059888610862,-37.6921335252834,28.4232685241094));
#55054=CARTESIAN_POINT('Ctrl Pts',(132.045676094596,-37.7029490106906,28.4222015073409));
#55055=CARTESIAN_POINT('Ctrl Pts',(132.019399273316,-37.7226192444384,28.4202545856474));
#55056=CARTESIAN_POINT('Ctrl Pts',(132.007361298214,-37.7315068376044,28.4193725793892));
#55057=CARTESIAN_POINT('Ctrl Pts',(131.979065934881,-37.7521091136718,28.4173220355156));
#55058=CARTESIAN_POINT('Ctrl Pts',(131.96276301018,-37.7637597501321,28.416157714943));
#55059=CARTESIAN_POINT('Ctrl Pts',(131.908077242125,-37.8021121334996,28.4123055047588));
#55060=CARTESIAN_POINT('Ctrl Pts',(131.869243843123,-37.8281653188411,28.4096565257023));
#55061=CARTESIAN_POINT('Ctrl Pts',(131.770993777703,-37.8911727889326,28.4031350224538));
#55062=CARTESIAN_POINT('Ctrl Pts',(131.710947557345,-37.9271075331202,28.399308913883));
#55063=CARTESIAN_POINT('Ctrl Pts',(131.404640359588,-38.0977685712417,28.3803647875889));
#55064=CARTESIAN_POINT('Ctrl Pts',(131.143439428503,-38.2033948837027,28.3659218698166));
#55065=CARTESIAN_POINT('Ctrl Pts',(130.796968171429,-38.2956498261437,28.3461864791395));
#55066=CARTESIAN_POINT('Ctrl Pts',(130.721073707885,-38.3130827807271,28.3418376679014));
#55067=CARTESIAN_POINT('Ctrl Pts',(130.610438711454,-38.3345140538044,28.335425624827));
#55068=CARTESIAN_POINT('Ctrl Pts',(130.57612818682,-38.3406130544841,28.3334272493346));
#55069=CARTESIAN_POINT('Ctrl Pts',(130.515353065313,-38.3504522518076,28.3298673356849));
#55070=CARTESIAN_POINT('Ctrl Pts',(130.488926526695,-38.3544105093142,28.3283127184016));
#55071=CARTESIAN_POINT('Ctrl Pts',(130.433632686867,-38.3620253306843,28.3250448191752));
#55072=CARTESIAN_POINT('Ctrl Pts',(130.404759665552,-38.3656234438039,28.3233298578134));
#55073=CARTESIAN_POINT('Ctrl Pts',(130.328182370857,-38.3741667642635,28.3187574235033));
#55074=CARTESIAN_POINT('Ctrl Pts',(130.280414655935,-38.3784718868008,28.3158805496174));
#55075=CARTESIAN_POINT('Ctrl Pts',(130.02593310052,-38.3959733109343,28.300416783084));
#55076=CARTESIAN_POINT('Ctrl Pts',(129.818454706349,-38.391213019506,28.2872895231079));
#55077=CARTESIAN_POINT('Ctrl Pts',(129.40037926935,-38.3431350981244,28.2602121526972));
#55078=CARTESIAN_POINT('Ctrl Pts',(129.190795683427,-38.298681060548,28.2463138403642));
#55079=CARTESIAN_POINT('Ctrl Pts',(128.955398940729,-38.2249489121988,28.2311599191909));
#55080=CARTESIAN_POINT('Ctrl Pts',(128.92415540516,-38.21466101476,28.2291589720985));
#55081=CARTESIAN_POINT('Ctrl Pts',(128.876346244365,-38.1981432417472,28.2261183644967));
#55082=CARTESIAN_POINT('Ctrl Pts',(128.859672197048,-38.1922359702146,28.2250619347378));
#55083=CARTESIAN_POINT('Ctrl Pts',(128.829081779952,-38.1811281419797,28.2231322082853));
#55084=CARTESIAN_POINT('Ctrl Pts',(128.81515278015,-38.1759664369078,28.2222568734248));
#55085=CARTESIAN_POINT('Ctrl Pts',(128.782334326936,-38.1635588560237,28.2202018837192));
#55086=CARTESIAN_POINT('Ctrl Pts',(128.763475192099,-38.1562352209384,28.2190267065331));
#55087=CARTESIAN_POINT('Ctrl Pts',(128.700148423394,-38.1309885696127,28.2150963704062));
#55088=CARTESIAN_POINT('Ctrl Pts',(128.655993923941,-38.1122904248296,28.2123823065342));
#55089=CARTESIAN_POINT('Ctrl Pts',(128.54609179637,-38.0629746996909,28.2056584663242));
#55090=CARTESIAN_POINT('Ctrl Pts',(128.480900897326,-38.0311717335472,28.2016988991137));
#55091=CARTESIAN_POINT('Ctrl Pts',(128.27496513587,-37.9223931250671,28.1891346521279));
#55092=CARTESIAN_POINT('Ctrl Pts',(128.138644685991,-37.8375140776417,28.1807224070989));
#55093=CARTESIAN_POINT('Ctrl Pts',(127.869299741438,-37.6420166906638,28.1629959554046));
#55094=CARTESIAN_POINT('Ctrl Pts',(127.737702033916,-37.5302440323514,28.1536826941632));
#55095=CARTESIAN_POINT('Ctrl Pts',(127.583536982917,-37.377623746849,28.1414567674077));
#55096=CARTESIAN_POINT('Ctrl Pts',(127.552511254712,-37.3456740560293,28.1389224963165));
#55097=CARTESIAN_POINT('Ctrl Pts',(127.502753839617,-37.2923726811027,28.1347288901729));
#55098=CARTESIAN_POINT('Ctrl Pts',(127.483644651331,-37.2713798851415,28.1330856096267));
#55099=CARTESIAN_POINT('Ctrl Pts',(127.446875756158,-37.2299531195062,28.1298575183643));
#55100=CARTESIAN_POINT('Ctrl Pts',(127.429192116281,-37.2095431839829,28.1282738731182));
#55101=CARTESIAN_POINT('Ctrl Pts',(127.387654791971,-37.1604282943073,28.1244777296392));
#55102=CARTESIAN_POINT('Ctrl Pts',(127.364028005377,-37.1315368580672,28.1222563839726));
#55103=CARTESIAN_POINT('Ctrl Pts',(127.281966709627,-37.02773889171,28.1143138125225));
#55104=CARTESIAN_POINT('Ctrl Pts',(127.226213281078,-36.9507779503513,28.1084918287921));
#55105=CARTESIAN_POINT('Ctrl Pts',(127.087448715858,-36.7412329788623,28.0928172146615));
#55106=CARTESIAN_POINT('Ctrl Pts',(127.010256594028,-36.6050776682874,28.0828006059806));
#55107=CARTESIAN_POINT('Ctrl Pts',(126.860896257594,-36.2931896405955,28.0605166503736));
#55108=CARTESIAN_POINT('Ctrl Pts',(126.793520836425,-36.1157119601657,28.0482568228123));
#55109=CARTESIAN_POINT('Ctrl Pts',(126.731823219316,-35.9003426565637,28.0344717635883));
#55110=CARTESIAN_POINT('Ctrl Pts',(126.722824778079,-35.8670173767127,28.0323692334853));
#55111=CARTESIAN_POINT('Ctrl Pts',(126.709903117556,-35.8160837043503,28.0292079662754));
#55112=CARTESIAN_POINT('Ctrl Pts',(126.705609054892,-35.7985727526427,28.0281304448739));
#55113=CARTESIAN_POINT('Ctrl Pts',(126.698010715842,-35.7664823968006,28.0261738528277));
#55114=CARTESIAN_POINT('Ctrl Pts',(126.694662980902,-35.7519146888537,28.0252925238941));
#55115=CARTESIAN_POINT('Ctrl Pts',(126.687101650162,-35.7179848072703,28.023255393623));
#55116=CARTESIAN_POINT('Ctrl Pts',(126.68296131409,-35.6986072266556,28.0221036095574));
#55117=CARTESIAN_POINT('Ctrl Pts',(126.674518282434,-35.6573239027156,28.0196723419892));
#55118=CARTESIAN_POINT('Ctrl Pts',(126.670261568484,-35.6354096292043,28.0183952069511));
#55119=CARTESIAN_POINT('Ctrl Pts',(126.65909154854,-35.5747068683642,28.0148907004978));
#55120=CARTESIAN_POINT('Ctrl Pts',(126.652637350317,-35.5358365371097,28.0126839168103));
#55121=CARTESIAN_POINT('Ctrl Pts',(126.622634442689,-35.3333576298257,28.0013415814903));
#55122=CARTESIAN_POINT('Ctrl Pts',(126.610397109784,-35.1682933274947,27.9926037001798));
#55123=CARTESIAN_POINT('Ctrl Pts',(126.610251318367,-35.0029896261394,27.9838401394632));
#55124=CARTESIAN_POINT('Origin',(130.,-35.,32.7603849714045));
#55125=CARTESIAN_POINT('',(125.915001580774,-35.0035937335827,28.3853849713762));
#55126=CARTESIAN_POINT('Ctrl Pts',(132.487160670875,-31.7594357285724,29.1925548588025));
#55127=CARTESIAN_POINT('Ctrl Pts',(132.581690749928,-31.8319883691446,29.1867409052004));
#55128=CARTESIAN_POINT('Ctrl Pts',(132.673154069962,-31.9087655494671,29.1809269515982));
#55129=CARTESIAN_POINT('Ctrl Pts',(132.761153735035,-31.9894759506853,29.1751129979961));
#55130=CARTESIAN_POINT('Ctrl Pts',(132.849077222675,-32.0701164844653,29.1693040772775));
#55131=CARTESIAN_POINT('Ctrl Pts',(132.933542721414,-32.1546831901611,29.1634951565588));
#55132=CARTESIAN_POINT('Ctrl Pts',(133.014185812298,-32.242844057921,29.1576862358402));
#55133=CARTESIAN_POINT('Ctrl Pts',(133.094785419747,-32.3309573885969,29.1518804473406));
#55134=CARTESIAN_POINT('Ctrl Pts',(133.171566443781,-32.4226607263339,29.146074658841));
#55135=CARTESIAN_POINT('Ctrl Pts',(133.244201169967,-32.5175850933451,29.1402688703414));
#55136=CARTESIAN_POINT('Ctrl Pts',(133.316816237194,-32.6124837685916,29.1344646532081));
#55137=CARTESIAN_POINT('Ctrl Pts',(133.385286990192,-32.7106014156742,29.1286604360748));
#55138=CARTESIAN_POINT('Ctrl Pts',(133.449326269572,-32.8115363183187,29.1228562189416));
#55139=CARTESIAN_POINT('Ctrl Pts',(133.513363316744,-32.9124677026887,29.1170522041251));
#55140=CARTESIAN_POINT('Ctrl Pts',(133.572968978944,-33.0162158025678,29.1112481893086));
#55141=CARTESIAN_POINT('Ctrl Pts',(133.627900030336,-33.122350839511,29.1054441744922));
#55142=CARTESIAN_POINT('Ctrl Pts',(133.682842119548,-33.2285072031775,29.0996389934198));
#55143=CARTESIAN_POINT('Ctrl Pts',(133.733107542422,-33.3370510952233,29.0938338123474));
#55144=CARTESIAN_POINT('Ctrl Pts',(133.778499832327,-33.4475297049192,29.088028631275));
#55145=CARTESIAN_POINT('Ctrl Pts',(133.823939690213,-33.5581240885591,29.0822173667742));
#55146=CARTESIAN_POINT('Ctrl Pts',(133.864496060608,-33.6706568609073,29.0764061022734));
#55147=CARTESIAN_POINT('Ctrl Pts',(133.900021216767,-33.7846566292745,29.0705948377726));
#55148=CARTESIAN_POINT('Ctrl Pts',(133.935565762292,-33.8987186178653,29.064780401527));
#55149=CARTESIAN_POINT('Ctrl Pts',(133.966073518727,-34.0142488030906,29.0589659652814));
#55150=CARTESIAN_POINT('Ctrl Pts',(133.991447529178,-34.1307637709937,29.0531515290358));
#55151=CARTESIAN_POINT('Ctrl Pts',(134.016861604858,-34.2474627144958,29.047327911872));
#55152=CARTESIAN_POINT('Ctrl Pts',(134.037125670834,-34.3651491448337,29.0415042947082));
#55153=CARTESIAN_POINT('Ctrl Pts',(134.052194385697,-34.4833321564844,29.0356806775443));
#55154=CARTESIAN_POINT('Ctrl Pts',(134.064126355323,-34.5769138665417,29.0310693205879));
#55155=CARTESIAN_POINT('Ctrl Pts',(134.07280183418,-34.6708067628457,29.0264579636314));
#55156=CARTESIAN_POINT('Ctrl Pts',(134.078221500643,-34.7647673668643,29.021846606675));
#55157=CARTESIAN_POINT('Ctrl Pts',(134.085065206428,-34.8834165002981,29.016023596994));
#55158=CARTESIAN_POINT('Ctrl Pts',(134.086737820478,-35.0025562582525,29.0102005873129));
#55159=CARTESIAN_POINT('Ctrl Pts',(134.08318679581,-35.1216987695917,29.0043775776319));
#55160=CARTESIAN_POINT('Ctrl Pts',(134.079640256487,-35.2406907904865,28.9985619230695));
#55161=CARTESIAN_POINT('Ctrl Pts',(134.070883213792,-35.3596851532059,28.9927462685072));
#55162=CARTESIAN_POINT('Ctrl Pts',(134.056914981161,-35.4781901668116,28.9869306139449));
#55163=CARTESIAN_POINT('Ctrl Pts',(134.042960749089,-35.5965764011404,28.9811207884966));
#55164=CARTESIAN_POINT('Ctrl Pts',(134.02380576557,-35.7144738588157,28.9753109630483));
#55165=CARTESIAN_POINT('Ctrl Pts',(133.999501353679,-35.8313927603236,28.9695011376001));
#55166=CARTESIAN_POINT('Ctrl Pts',(133.97427344178,-35.9527542546836,28.9634705549545));
#55167=CARTESIAN_POINT('Ctrl Pts',(133.943497026151,-36.0730609050317,28.957439972309));
#55168=CARTESIAN_POINT('Ctrl Pts',(133.90728848545,-36.1917724998812,28.9514093896634));
#55169=CARTESIAN_POINT('Ctrl Pts',(133.872444754176,-36.3060094956231,28.94560611792));
#55170=CARTESIAN_POINT('Ctrl Pts',(133.8325711213,-36.418769078161,28.9398028461766));
#55171=CARTESIAN_POINT('Ctrl Pts',(133.787822782052,-36.5295828097124,28.9339995744332));
#55172=CARTESIAN_POINT('Ctrl Pts',(133.743081084127,-36.6403800948486,28.9281971639822));
#55173=CARTESIAN_POINT('Ctrl Pts',(133.693466271488,-36.7492317246963,28.9223947535311));
#55174=CARTESIAN_POINT('Ctrl Pts',(133.639182145788,-36.8556880960374,28.9165923430801));
#55175=CARTESIAN_POINT('Ctrl Pts',(133.584893258051,-36.9621538061911,28.9107894236165));
#55176=CARTESIAN_POINT('Ctrl Pts',(133.525934428401,-37.0662234761904,28.9049865041529));
#55177=CARTESIAN_POINT('Ctrl Pts',(133.462555685773,-37.1674715967975,28.8991835846894));
#55178=CARTESIAN_POINT('Ctrl Pts',(133.399156417163,-37.2687525078477,28.8933787858793));
#55179=CARTESIAN_POINT('Ctrl Pts',(133.331334605376,-37.3672097061665,28.8875739870693));
#55180=CARTESIAN_POINT('Ctrl Pts',(133.259383545455,-37.4624467311234,28.8817691882592));
#55181=CARTESIAN_POINT('Ctrl Pts',(133.187352808312,-37.5577892197313,28.8759579613266));
#55182=CARTESIAN_POINT('Ctrl Pts',(133.111183941995,-37.649904090949,28.8701467343939));
#55183=CARTESIAN_POINT('Ctrl Pts',(133.0312105605,-37.7384279318461,28.8643355074612));
#55184=CARTESIAN_POINT('Ctrl Pts',(132.951184663269,-37.8270099032683,28.8585204644981));
#55185=CARTESIAN_POINT('Ctrl Pts',(132.867349561646,-37.911995858073,28.8527054215349));
#55186=CARTESIAN_POINT('Ctrl Pts',(132.780074549519,-37.9930603901556,28.8468903785718));
#55187=CARTESIAN_POINT('Ctrl Pts',(132.692674467523,-38.074241092149,28.8410670023339));
#55188=CARTESIAN_POINT('Ctrl Pts',(132.601824945918,-38.1514888913627,28.835243626096));
#55189=CARTESIAN_POINT('Ctrl Pts',(132.507927128268,-38.2245195796111,28.829420249858));
#55190=CARTESIAN_POINT('Ctrl Pts',(132.482917837064,-38.2439709981313,28.8278692179409));
#55191=CARTESIAN_POINT('Ctrl Pts',(132.457692449597,-38.2631234984578,28.8263181860237));
#55192=CARTESIAN_POINT('Ctrl Pts',(132.432258858119,-38.2819722495937,28.8247671541066));
#55193=CARTESIAN_POINT('Ctrl Pts',(132.336762581187,-38.3527442268744,28.8189434475485));
#55194=CARTESIAN_POINT('Ctrl Pts',(132.238020885238,-38.4194588244185,28.8131197409904));
#55195=CARTESIAN_POINT('Ctrl Pts',(132.136413161883,-38.481804675988,28.8072960344323));
#55196=CARTESIAN_POINT('Ctrl Pts',(132.03493362094,-38.5440718756469,28.8014796747247));
#55197=CARTESIAN_POINT('Ctrl Pts',(131.93059558893,-38.6019810796357,28.7956633150171));
#55198=CARTESIAN_POINT('Ctrl Pts',(131.823810069726,-38.6552622107813,28.7898469553094));
#55199=CARTESIAN_POINT('Ctrl Pts',(131.717131435195,-38.708490011323,28.7840364173621));
#55200=CARTESIAN_POINT('Ctrl Pts',(131.608010550233,-38.7570987733044,28.7782258794148));
#55201=CARTESIAN_POINT('Ctrl Pts',(131.496885319749,-38.8008629729996,28.7724153414675));
#55202=CARTESIAN_POINT('Ctrl Pts',(131.381556838905,-38.846282529335,28.7663850231371));
#55203=CARTESIAN_POINT('Ctrl Pts',(131.264069774235,-38.8864835671572,28.7603547048067));
#55204=CARTESIAN_POINT('Ctrl Pts',(131.144939615841,-38.9212674323589,28.7543243864763));
#55205=CARTESIAN_POINT('Ctrl Pts',(131.030280461001,-38.954745844877,28.7485203884586));
#55206=CARTESIAN_POINT('Ctrl Pts',(130.914099749006,-38.9832062498323,28.7427163904408));
#55207=CARTESIAN_POINT('Ctrl Pts',(130.796874454028,-39.006521696499,28.7369123924231));
#55208=CARTESIAN_POINT('Ctrl Pts',(130.67966647758,-39.0298336986083,28.7311092518715));
#55209=CARTESIAN_POINT('Ctrl Pts',(130.561414625417,-39.0480021744022,28.7253061113198));
#55210=CARTESIAN_POINT('Ctrl Pts',(130.442606757085,-39.0609511519572,28.7195029707682));
#55211=CARTESIAN_POINT('Ctrl Pts',(130.323788405549,-39.0739012720862,28.7136993181671));
#55212=CARTESIAN_POINT('Ctrl Pts',(130.204414346232,-39.0816309340465,28.707895665566));
#55213=CARTESIAN_POINT('Ctrl Pts',(130.084977622509,-39.084116036999,28.7020920129649));
#55214=CARTESIAN_POINT('Ctrl Pts',(129.965502176336,-39.0866019456441,28.696286478768));
#55215=CARTESIAN_POINT('Ctrl Pts',(129.845964433371,-39.0838399052112,28.690480944571));
#55216=CARTESIAN_POINT('Ctrl Pts',(129.726856855235,-39.0758579247157,28.6846754103741));
#55217=CARTESIAN_POINT('Ctrl Pts',(129.607617403772,-39.0678671067446,28.6788634484156));
#55218=CARTESIAN_POINT('Ctrl Pts',(129.488809475458,-39.0546448398398,28.673051486457));
#55219=CARTESIAN_POINT('Ctrl Pts',(129.370919991094,-39.0362709698922,28.6672395244985));
#55220=CARTESIAN_POINT('Ctrl Pts',(129.252953089375,-39.0178850339287,28.6614237458575));
#55221=CARTESIAN_POINT('Ctrl Pts',(129.13590623215,-38.9943408378627,28.6556079672166));
#55222=CARTESIAN_POINT('Ctrl Pts',(129.020254110698,-38.9657689030496,28.6497921885756));
#55223=CARTESIAN_POINT('Ctrl Pts',(128.904436366872,-38.937156051117,28.6439680813105));
#55224=CARTESIAN_POINT('Ctrl Pts',(128.790017735786,-38.9035012042496,28.6381439740453));
#55225=CARTESIAN_POINT('Ctrl Pts',(128.677455911146,-38.8649841051469,28.6323198667801));
#55226=CARTESIAN_POINT('Ctrl Pts',(128.647614143248,-38.8547726650319,28.6307758116994));
#55227=CARTESIAN_POINT('Ctrl Pts',(128.617902761471,-38.844219735367,28.6292317566188));
#55228=CARTESIAN_POINT('Ctrl Pts',(128.588330019206,-38.8333292143154,28.6276877015381));
#55229=CARTESIAN_POINT('Ctrl Pts',(128.476791315952,-38.792253733897,28.6218640312169));
#55230=CARTESIAN_POINT('Ctrl Pts',(128.366867060462,-38.7462398208537,28.6160403608958));
#55231=CARTESIAN_POINT('Ctrl Pts',(128.259025634089,-38.6954341094438,28.6102166905746));
#55232=CARTESIAN_POINT('Ctrl Pts',(128.151320234839,-38.6446924824491,28.6044003660123));
#55233=CARTESIAN_POINT('Ctrl Pts',(128.045692805387,-38.5891712513471,28.5985840414501));
#55234=CARTESIAN_POINT('Ctrl Pts',(127.942594522375,-38.529066123019,28.5927677168878));
#55235=CARTESIAN_POINT('Ctrl Pts',(127.839599413955,-38.469021144306,28.5869572129551));
#55236=CARTESIAN_POINT('Ctrl Pts',(127.73912876755,-38.4044015986898,28.5811467090223));
#55237=CARTESIAN_POINT('Ctrl Pts',(127.641611242286,-38.3354501146752,28.5753362050896));
#55238=CARTESIAN_POINT('Ctrl Pts',(127.540404357014,-38.2638900036794,28.5693058735846));
#55239=CARTESIAN_POINT('Ctrl Pts',(127.442378860784,-38.1876638934963,28.5632755420796));
#55240=CARTESIAN_POINT('Ctrl Pts',(127.347983478252,-38.1070940391907,28.5572452105746));
#55241=CARTESIAN_POINT('Ctrl Pts',(127.257131475877,-38.029548587301,28.5514412434999));
#55242=CARTESIAN_POINT('Ctrl Pts',(127.169642306108,-37.9479799100945,28.5456372764253));
#55243=CARTESIAN_POINT('Ctrl Pts',(127.085883599613,-37.8627173463325,28.5398333093506));
#55244=CARTESIAN_POINT('Ctrl Pts',(127.002137250205,-37.7774673615257,28.5340301985467));
#55245=CARTESIAN_POINT('Ctrl Pts',(126.922120555643,-37.6885248651375,28.5282270877429));
#55246=CARTESIAN_POINT('Ctrl Pts',(126.846164475781,-37.5962562443202,28.522423976939));
#55247=CARTESIAN_POINT('Ctrl Pts',(126.770201677622,-37.5039794623669,28.5166203528514));
#55248=CARTESIAN_POINT('Ctrl Pts',(126.698300467788,-37.4083762863162,28.5108167287639));
#55249=CARTESIAN_POINT('Ctrl Pts',(126.630751263683,-37.3098458720934,28.5050131046763));
#55250=CARTESIAN_POINT('Ctrl Pts',(126.563180144589,-37.2112834916462,28.4992075977189));
#55251=CARTESIAN_POINT('Ctrl Pts',(126.499964069986,-37.1097923209244,28.4934020907615));
#55252=CARTESIAN_POINT('Ctrl Pts',(126.4413495547,-37.0057995932215,28.487596583804));
#55253=CARTESIAN_POINT('Ctrl Pts',(126.382670121785,-36.9016916899297,28.4817846470443));
#55254=CARTESIAN_POINT('Ctrl Pts',(126.328602621627,-36.7950770552998,28.4759727102845));
#55255=CARTESIAN_POINT('Ctrl Pts',(126.279347176525,-36.6864067027756,28.4701607735248));
#55256=CARTESIAN_POINT('Ctrl Pts',(126.230059375674,-36.5776649650346,28.4643450189218));
#55257=CARTESIAN_POINT('Ctrl Pts',(126.185590076881,-36.4668651981246,28.4585292643189));
#55258=CARTESIAN_POINT('Ctrl Pts',(126.146090314788,-36.3544759644327,28.4527135097159));
#55259=CARTESIAN_POINT('Ctrl Pts',(126.106533973011,-36.2419257437652,28.4468894245931));
#55260=CARTESIAN_POINT('Ctrl Pts',(126.071961493804,-36.1277819014283,28.4410653394703));
#55261=CARTESIAN_POINT('Ctrl Pts',(126.042473426805,-36.0125257638479,28.4352412543474));
#55262=CARTESIAN_POINT('Ctrl Pts',(126.034654266078,-35.981964036471,28.4336969192215));
#55263=CARTESIAN_POINT('Ctrl Pts',(126.027192317697,-35.9513241416612,28.4321525840956));
#55264=CARTESIAN_POINT('Ctrl Pts',(126.020088846053,-35.920615124081,28.4306082489697));
#55265=CARTESIAN_POINT('Ctrl Pts',(125.984344514774,-35.766088808985,28.4228372281072));
#55266=CARTESIAN_POINT('Ctrl Pts',(125.957588053208,-35.6094121628919,28.4150662072447));
#55267=CARTESIAN_POINT('Ctrl Pts',(125.940025230487,-35.4514752162833,28.4072951863823));
#55268=CARTESIAN_POINT('Ctrl Pts',(125.923519238621,-35.3030420175071,28.3999917813897));
#55269=CARTESIAN_POINT('Ctrl Pts',(125.915133455172,-35.1534953906131,28.3926883763971));
#55270=CARTESIAN_POINT('Ctrl Pts',(125.915001580775,-35.0035937341642,28.3853849714045));
#55271=CARTESIAN_POINT('Ctrl Pts',(125.915001580774,-35.0035937335827,28.3853849713762));
#55272=CARTESIAN_POINT('Ctrl Pts',(125.914898004666,-34.885858729381,28.3796487678021));
#55273=CARTESIAN_POINT('Ctrl Pts',(125.919888554375,-34.7679814543618,28.373912564228));
#55274=CARTESIAN_POINT('Ctrl Pts',(125.92998336164,-34.6504437620797,28.3681763606539));
#55275=CARTESIAN_POINT('Ctrl Pts',(125.940070875455,-34.5329909902111,28.3624443014591));
#55276=CARTESIAN_POINT('Ctrl Pts',(125.955255277809,-34.4158777301303,28.3567122422643));
#55277=CARTESIAN_POINT('Ctrl Pts',(125.975494633281,-34.2995847280028,28.3509801830696));
#55278=CARTESIAN_POINT('Ctrl Pts',(125.995726326249,-34.183335753736,28.3452502939994));
#55279=CARTESIAN_POINT('Ctrl Pts',(126.021009097467,-34.067906833477,28.3395204049292));
#55280=CARTESIAN_POINT('Ctrl Pts',(126.051249361176,-33.9537718258485,28.333790515859));
#55281=CARTESIAN_POINT('Ctrl Pts',(126.081485763923,-33.8396513905425,28.3280613583592));
#55282=CARTESIAN_POINT('Ctrl Pts',(126.116678293246,-33.7268249453335,28.3223322008594));
#55283=CARTESIAN_POINT('Ctrl Pts',(126.156682813441,-33.6157536333813,28.3166030433596));
#55284=CARTESIAN_POINT('Ctrl Pts',(126.196692264234,-33.5046686317747,28.3108731797352));
#55285=CARTESIAN_POINT('Ctrl Pts',(126.241514741578,-33.3953395882188,28.3051433161108));
#55286=CARTESIAN_POINT('Ctrl Pts',(126.290957333967,-33.2882092705167,28.2994134524864));
#55287=CARTESIAN_POINT('Ctrl Pts',(126.340448483654,-33.1809737407183,28.2936779615944));
#55288=CARTESIAN_POINT('Ctrl Pts',(126.394568633237,-33.0759416309574,28.2879424707024));
#55289=CARTESIAN_POINT('Ctrl Pts',(126.453078068552,-32.9735326767475,28.2822069798104));
#55290=CARTESIAN_POINT('Ctrl Pts',(126.51161697166,-32.8710721451136,28.2764686002858));
#55291=CARTESIAN_POINT('Ctrl Pts',(126.574549337832,-32.7712377543844,28.2707302207612));
#55292=CARTESIAN_POINT('Ctrl Pts',(126.641592140703,-32.674420147445,28.2649918412366));
#55293=CARTESIAN_POINT('Ctrl Pts',(126.708740646782,-32.5774498927753,28.2592444142811));
#55294=CARTESIAN_POINT('Ctrl Pts',(126.780012279904,-32.4835062564679,28.2534969873256));
#55295=CARTESIAN_POINT('Ctrl Pts',(126.855083544856,-32.3929469721224,28.2477495603701));
#55296=CARTESIAN_POINT('Ctrl Pts',(126.916999410163,-32.3182571896145,28.2430093057138));
#55297=CARTESIAN_POINT('Ctrl Pts',(126.981499104198,-32.2458689813848,28.2382690510575));
#55298=CARTESIAN_POINT('Ctrl Pts',(127.048383341174,-32.1759631554559,28.2335287964012));
#55299=CARTESIAN_POINT('Ctrl Pts',(127.130553567039,-32.0900807747109,28.2277051851384));
#55300=CARTESIAN_POINT('Ctrl Pts',(127.216607747338,-32.0076492124992,28.2218815738755));
#55301=CARTESIAN_POINT('Ctrl Pts',(127.306224544795,-31.9290394341611,28.2160579626127));
#55302=CARTESIAN_POINT('Ctrl Pts',(127.395728279743,-31.8505288316373,28.210241698545));
#55303=CARTESIAN_POINT('Ctrl Pts',(127.488785387778,-31.7758306897397,28.2044254344774));
#55304=CARTESIAN_POINT('Ctrl Pts',(127.585036399288,-31.7052806178318,28.1986091704098));
#55305=CARTESIAN_POINT('Ctrl Pts',(127.681191065126,-31.6348011653795,28.1927987283263));
#55306=CARTESIAN_POINT('Ctrl Pts',(127.78053294687,-31.5684617627394,28.1869882862429));
#55307=CARTESIAN_POINT('Ctrl Pts',(127.882668534847,-31.5065586498879,28.1811778441594));
#55308=CARTESIAN_POINT('Ctrl Pts',(127.988669723925,-31.4423126441632,28.1751474899792));
#55309=CARTESIAN_POINT('Ctrl Pts',(128.097679931082,-31.3828456651534,28.1691171357989));
#55310=CARTESIAN_POINT('Ctrl Pts',(128.209224606699,-31.3284405914178,28.1630867816186));
#55311=CARTESIAN_POINT('Ctrl Pts',(128.316580554951,-31.2760785378433,28.1572828793908));
#55312=CARTESIAN_POINT('Ctrl Pts',(128.426283655175,-31.2284052702501,28.1514789771629));
#55313=CARTESIAN_POINT('Ctrl Pts',(128.53788523975,-31.185626469804,28.1456750749351));
#55314=CARTESIAN_POINT('Ctrl Pts',(128.649470340154,-31.1428539880237,28.1398720299757));
#55315=CARTESIAN_POINT('Ctrl Pts',(128.762952986069,-31.1049746818036,28.1340689850164));
#55316=CARTESIAN_POINT('Ctrl Pts',(128.877865170739,-31.0721458243769,28.128265940057));
#55317=CARTESIAN_POINT('Ctrl Pts',(128.992787501069,-31.0393140684723,28.1224623827437));
#55318=CARTESIAN_POINT('Ctrl Pts',(129.109139228453,-31.0115337601051,28.1166588254303));
#55319=CARTESIAN_POINT('Ctrl Pts',(129.226438476133,-30.988911922085,28.1108552681169));
#55320=CARTESIAN_POINT('Ctrl Pts',(129.343775762221,-30.9662827481377,28.1050498287958));
#55321=CARTESIAN_POINT('Ctrl Pts',(129.462060778949,-30.9488154486754,28.0992443894748));
#55322=CARTESIAN_POINT('Ctrl Pts',(129.58080342219,-30.9365655869509,28.0934389501537));
#55323=CARTESIAN_POINT('Ctrl Pts',(129.699677559264,-30.924302159912,28.0876270819757));
#55324=CARTESIAN_POINT('Ctrl Pts',(129.819009927986,-30.9172677453482,28.0818152137976));
#55325=CARTESIAN_POINT('Ctrl Pts',(129.938307130876,-30.9154658784753,28.0760033456196));
#55326=CARTESIAN_POINT('Ctrl Pts',(130.057682687685,-30.9136628281436,28.0701876602301));
#55327=CARTESIAN_POINT('Ctrl Pts',(130.177022625436,-30.917099158085,28.0643719748406));
#55328=CARTESIAN_POINT('Ctrl Pts',(130.29583704243,-30.9257263905911,28.0585562894511));
#55329=CARTESIAN_POINT('Ctrl Pts',(130.414821643643,-30.9343659803418,28.0527322739456));
#55330=CARTESIAN_POINT('Ctrl Pts',(130.533278817554,-30.9482112656903,28.0469082584401));
#55331=CARTESIAN_POINT('Ctrl Pts',(130.65072710339,-30.9671623840138,28.0410842429346));
#55332=CARTESIAN_POINT('Ctrl Pts',(130.681883210605,-30.9721896440553,28.0395392765673));
#55333=CARTESIAN_POINT('Ctrl Pts',(130.712968397176,-30.97757593192,28.0379943102001));
#55334=CARTESIAN_POINT('Ctrl Pts',(130.743973854237,-30.9833187947993,28.0364493438328));
#55335=CARTESIAN_POINT('Ctrl Pts',(130.860849615195,-31.0049666443311,28.030625558701));
#55336=CARTESIAN_POINT('Ctrl Pts',(130.976968212671,-31.0317548423152,28.0248017735693));
#55337=CARTESIAN_POINT('Ctrl Pts',(131.091843191745,-31.0636179752671,28.0189779884375));
#55338=CARTESIAN_POINT('Ctrl Pts',(131.206577816322,-31.0954421777747,28.013161318819));
#55339=CARTESIAN_POINT('Ctrl Pts',(131.320071454059,-31.1323288763398,28.0073446492004));
#55340=CARTESIAN_POINT('Ctrl Pts',(131.431846262191,-31.1741613623352,28.0015279795818));
#55341=CARTESIAN_POINT('Ctrl Pts',(131.543491559234,-31.2159453779204,27.9957180496144));
#55342=CARTESIAN_POINT('Ctrl Pts',(131.653421611136,-31.2626636304388,27.989908119647));
#55343=CARTESIAN_POINT('Ctrl Pts',(131.761173065759,-31.3141494289046,27.9840981896796));
#55344=CARTESIAN_POINT('Ctrl Pts',(131.868852414607,-31.3656007737898,27.9782921476365));
#55345=CARTESIAN_POINT('Ctrl Pts',(131.974355698478,-31.4218131443671,27.9724861055935));
#55346=CARTESIAN_POINT('Ctrl Pts',(132.07723916007,-31.4825716109819,27.9666800635504));
#55347=CARTESIAN_POINT('Ctrl Pts',(132.18007749739,-31.5433034291775,27.9608765680141));
#55348=CARTESIAN_POINT('Ctrl Pts',(132.2802979476,-31.6085771691,27.9550730724778));
#55349=CARTESIAN_POINT('Ctrl Pts',(132.377481582681,-31.6781321031665,27.9492695769414));
#55350=CARTESIAN_POINT('Ctrl Pts',(132.414488702198,-31.7046183295344,27.9470596302487));
#55351=CARTESIAN_POINT('Ctrl Pts',(132.451055745837,-31.7317248911822,27.944849683556));
#55352=CARTESIAN_POINT('Ctrl Pts',(132.487160670875,-31.7594357285724,27.9426397368634));
#55353=CARTESIAN_POINT('',(125.915001103444,-34.9969974781416,28.4896150285558));
#55354=CARTESIAN_POINT('Ctrl Pts',(125.915001103444,-34.9969974781416,28.4896150285558));
#55355=CARTESIAN_POINT('Ctrl Pts',(125.915102918969,-34.8584751532076,28.4828889790542));
#55356=CARTESIAN_POINT('Ctrl Pts',(125.922254614347,-34.7202367330429,28.4761629295526));
#55357=CARTESIAN_POINT('Ctrl Pts',(125.936346094775,-34.5829365293537,28.4694368800511));
#55358=CARTESIAN_POINT('Ctrl Pts',(125.950518210567,-34.4448506557737,28.4626723422266));
#55359=CARTESIAN_POINT('Ctrl Pts',(125.971709650854,-34.3077138835539,28.455907804402));
#55360=CARTESIAN_POINT('Ctrl Pts',(125.999759150207,-34.1721726365672,28.4491432665776));
#55361=CARTESIAN_POINT('Ctrl Pts',(126.027989112987,-34.0357593512738,28.4423352074174));
#55362=CARTESIAN_POINT('Ctrl Pts',(126.063165581529,-33.9009623006317,28.4355271482572));
#55363=CARTESIAN_POINT('Ctrl Pts',(126.105075852321,-33.7684193555327,28.428719089097));
#55364=CARTESIAN_POINT('Ctrl Pts',(126.116063679441,-33.7336699029727,28.4269341858821));
#55365=CARTESIAN_POINT('Ctrl Pts',(126.127514106913,-33.6990752710491,28.4251492826673));
#55366=CARTESIAN_POINT('Ctrl Pts',(126.139422767306,-33.6646467020292,28.4233643794524));
#55367=CARTESIAN_POINT('Ctrl Pts',(126.178277843269,-33.5523146159319,28.4175406723593));
#55368=CARTESIAN_POINT('Ctrl Pts',(126.222102456264,-33.4414987050422,28.4117169652662));
#55369=CARTESIAN_POINT('Ctrl Pts',(126.270759293661,-33.3326701723455,28.4058932581732));
#55370=CARTESIAN_POINT('Ctrl Pts',(126.319354748462,-33.2239789313076,28.4000768979255));
#55371=CARTESIAN_POINT('Ctrl Pts',(126.372770137565,-33.1172704512509,28.3942605376778));
#55372=CARTESIAN_POINT('Ctrl Pts',(126.430818743981,-33.0129997076801,28.3884441774302));
#55373=CARTESIAN_POINT('Ctrl Pts',(126.488809247939,-32.9088333315831,28.3826336389385));
#55374=CARTESIAN_POINT('Ctrl Pts',(126.551423545968,-32.8071001926032,28.3768231004468));
#55375=CARTESIAN_POINT('Ctrl Pts',(126.618427561826,-32.7082336843857,28.3710125619551));
#55376=CARTESIAN_POINT('Ctrl Pts',(126.687965958665,-32.6056276182515,28.3649822438272));
#55377=CARTESIAN_POINT('Ctrl Pts',(126.76223252318,-32.5061097304143,28.3589519256992));
#55378=CARTESIAN_POINT('Ctrl Pts',(126.840913973803,-32.4101350461686,28.3529216075712));
#55379=CARTESIAN_POINT('Ctrl Pts',(126.916642487152,-32.3177623191844,28.3471176090018));
#55380=CARTESIAN_POINT('Ctrl Pts',(126.996460192436,-32.2286719777861,28.3413136104324));
#55381=CARTESIAN_POINT('Ctrl Pts',(127.080045109383,-32.1432381203957,28.335509611863));
#55382=CARTESIAN_POINT('Ctrl Pts',(127.163617677759,-32.0578168847325,28.3297064707579));
#55383=CARTESIAN_POINT('Ctrl Pts',(127.25095606551,-31.9760513505808,28.3239033296529));
#55384=CARTESIAN_POINT('Ctrl Pts',(127.34170052331,-31.898279688265,28.3181001885478));
#55385=CARTESIAN_POINT('Ctrl Pts',(127.43245298811,-31.8205011636266,28.3122965353921));
#55386=CARTESIAN_POINT('Ctrl Pts',(127.526611810458,-31.7467174772185,28.3064928822365));
#55387=CARTESIAN_POINT('Ctrl Pts',(127.623783673822,-31.6772269154805,28.3006892290808));
#55388=CARTESIAN_POINT('Ctrl Pts',(127.720987041176,-31.6077138242792,28.2948836943288));
#55389=CARTESIAN_POINT('Ctrl Pts',(127.821205060333,-31.5424968632586,28.2890781595767));
#55390=CARTESIAN_POINT('Ctrl Pts',(127.924015471257,-31.4818309823975,28.2832726248247));
#55391=CARTESIAN_POINT('Ctrl Pts',(128.026939711592,-31.4210979336155,28.277460662313));
#55392=CARTESIAN_POINT('Ctrl Pts',(128.132461721069,-31.3649262306117,28.2716486998013));
#55393=CARTESIAN_POINT('Ctrl Pts',(128.240134543168,-31.3135249120806,28.2658367372897));
#55394=CARTESIAN_POINT('Ctrl Pts',(128.347878073381,-31.2620898386033,28.2600209580961));
#55395=CARTESIAN_POINT('Ctrl Pts',(128.457774854118,-31.2154315476308,28.2542051789026));
#55396=CARTESIAN_POINT('Ctrl Pts',(128.569359408562,-31.1737103483754,28.248389399709));
#55397=CARTESIAN_POINT('Ctrl Pts',(128.681103760212,-31.1319294013248,28.2425652918962));
#55398=CARTESIAN_POINT('Ctrl Pts',(128.794540322816,-31.0950997835242,28.2367411840834));
#55399=CARTESIAN_POINT('Ctrl Pts',(128.909189855554,-31.0633315825721,28.2309170762706));
#55400=CARTESIAN_POINT('Ctrl Pts',(128.93958499817,-31.0549094025986,28.229373026475));
#55401=CARTESIAN_POINT('Ctrl Pts',(128.970065349101,-31.0468426848124,28.2278289766795));
#55402=CARTESIAN_POINT('Ctrl Pts',(129.000621895564,-31.0391328721638,28.226284926884));
#55403=CARTESIAN_POINT('Ctrl Pts',(129.115878571649,-31.0100521191993,28.2204609033032));
#55404=CARTESIAN_POINT('Ctrl Pts',(129.232591436126,-30.9859594149578,28.2146368797225));
#55405=CARTESIAN_POINT('Ctrl Pts',(129.35029103599,-30.9669982318272,28.2088128561417));
#55406=CARTESIAN_POINT('Ctrl Pts',(129.467840464957,-30.9480612409445,28.2029962633326));
#55407=CARTESIAN_POINT('Ctrl Pts',(129.586373725437,-30.9342428125389,28.1971796705235));
#55408=CARTESIAN_POINT('Ctrl Pts',(129.705407873483,-30.9256361872074,28.1913630777144));
#55409=CARTESIAN_POINT('Ctrl Pts',(129.8285360694,-30.9167335465165,28.1853464296288));
#55410=CARTESIAN_POINT('Ctrl Pts',(129.952199807902,-30.9134078017856,28.1793297815431));
#55411=CARTESIAN_POINT('Ctrl Pts',(130.075854079365,-30.9157043252669,28.1733131334575));
#55412=CARTESIAN_POINT('Ctrl Pts',(130.195179551404,-30.9179204537128,28.1675071118425));
#55413=CARTESIAN_POINT('Ctrl Pts',(130.314495759763,-30.9253718175763,28.1617010902274));
#55414=CARTESIAN_POINT('Ctrl Pts',(130.433309752101,-30.9380463248907,28.1558950686124));
#55415=CARTESIAN_POINT('Ctrl Pts',(130.552075627358,-30.9507156993055,28.1500913983097));
#55416=CARTESIAN_POINT('Ctrl Pts',(130.670339285781,-30.9686039668099,28.1442877280071));
#55417=CARTESIAN_POINT('Ctrl Pts',(130.787611406211,-30.9916470623451,28.1384840577044));
#55418=CARTESIAN_POINT('Ctrl Pts',(130.904863707988,-31.0146862636632,28.1326813682054));
#55419=CARTESIAN_POINT('Ctrl Pts',(131.021124404848,-31.0428784805336,28.1268786787064));
#55420=CARTESIAN_POINT('Ctrl Pts',(131.135913532358,-31.0761083798088,28.1210759892074));
#55421=CARTESIAN_POINT('Ctrl Pts',(131.250710348146,-31.1093405047367,28.1152729110592));
#55422=CARTESIAN_POINT('Ctrl Pts',(131.364035006966,-31.1476108680104,28.1094698329111));
#55423=CARTESIAN_POINT('Ctrl Pts',(131.475422509601,-31.1907542192498,28.1036667547629));
#55424=CARTESIAN_POINT('Ctrl Pts',(131.586890966057,-31.2339289260635,28.0978594590739));
#55425=CARTESIAN_POINT('Ctrl Pts',(131.696419074474,-31.2819835439919,28.0920521633849));
#55426=CARTESIAN_POINT('Ctrl Pts',(131.803561658364,-31.3347046033805,28.0862448676959));
#55427=CARTESIAN_POINT('Ctrl Pts',(131.910750990177,-31.3874486657615,28.0804350381962));
#55428=CARTESIAN_POINT('Ctrl Pts',(132.01555236519,-31.4448630314251,28.0746252086966));
#55429=CARTESIAN_POINT('Ctrl Pts',(132.117546319305,-31.5066888793585,28.068815379197));
#55430=CARTESIAN_POINT('Ctrl Pts',(132.219653698128,-31.5685834821392,28.0629990887437));
#55431=CARTESIAN_POINT('Ctrl Pts',(132.318947084202,-31.6348991349368,28.0571827982904));
#55432=CARTESIAN_POINT('Ctrl Pts',(132.415037034438,-31.7053344445462,28.0513665078371));
#55433=CARTESIAN_POINT('Ctrl Pts',(132.439284019921,-31.7231078321418,28.0498988464445));
#55434=CARTESIAN_POINT('Ctrl Pts',(132.463327200408,-31.7411433370532,28.0484311850518));
#55435=CARTESIAN_POINT('Ctrl Pts',(132.487160670875,-31.7594357285724,28.0469635236591));
#55436=CARTESIAN_POINT('Ctrl Pts',(132.487160670875,-31.7594357285724,29.296931249476));
#55437=CARTESIAN_POINT('Ctrl Pts',(132.582108041547,-31.832308644015,29.2911177031239));
#55438=CARTESIAN_POINT('Ctrl Pts',(132.673828569789,-31.9093414008505,29.2853041567717));
#55439=CARTESIAN_POINT('Ctrl Pts',(132.761950782513,-31.9902071707547,29.2794906104196));
#55440=CARTESIAN_POINT('Ctrl Pts',(132.850165037886,-32.0711574040362,29.2736709918844));
#55441=CARTESIAN_POINT('Ctrl Pts',(132.934773170299,-32.155948371588,29.2678513733491));
#55442=CARTESIAN_POINT('Ctrl Pts',(133.015439862989,-32.2442156411106,29.2620317548139));
#55443=CARTESIAN_POINT('Ctrl Pts',(133.096149402472,-32.3325297945371,29.2562090451393));
#55444=CARTESIAN_POINT('Ctrl Pts',(133.172913069843,-32.4243236169473,29.2503863354646));
#55445=CARTESIAN_POINT('Ctrl Pts',(133.245436340838,-32.5192001375429,29.24456362579));
#55446=CARTESIAN_POINT('Ctrl Pts',(133.318076046915,-32.6142289810455,29.2387315678376));
#55447=CARTESIAN_POINT('Ctrl Pts',(133.386461520609,-32.7123500779307,29.2328995098852));
#55448=CARTESIAN_POINT('Ctrl Pts',(133.450341687516,-32.8131375810553,29.2270674519329));
#55449=CARTESIAN_POINT('Ctrl Pts',(133.506514718584,-32.901765081867,29.2219390311973));
#55450=CARTESIAN_POINT('Ctrl Pts',(133.55920458717,-32.9924538395889,29.2168106104618));
#55451=CARTESIAN_POINT('Ctrl Pts',(133.608270882691,-33.0849004628673,29.2116821897262));
#55452=CARTESIAN_POINT('Ctrl Pts',(133.663940960201,-33.1897893816007,29.2058635401457));
#55453=CARTESIAN_POINT('Ctrl Pts',(133.715124976196,-33.2972796915462,29.2000448905651));
#55454=CARTESIAN_POINT('Ctrl Pts',(133.761571407974,-33.4069508661956,29.1942262409846));
#55455=CARTESIAN_POINT('Ctrl Pts',(133.807958699009,-33.516482395355,29.1884150003534));
#55456=CARTESIAN_POINT('Ctrl Pts',(133.849620245492,-33.6281888928937,29.1826037597221));
#55457=CARTESIAN_POINT('Ctrl Pts',(133.886350021045,-33.7416246530066,29.1767925190909));
#55458=CARTESIAN_POINT('Ctrl Pts',(133.923042649375,-33.8549456881204,29.1709871557472));
#55459=CARTESIAN_POINT('Ctrl Pts',(133.954813303684,-33.9699921197517,29.1651817924034));
#55460=CARTESIAN_POINT('Ctrl Pts',(133.981503992919,-34.086298213656,29.1593764290597));
#55461=CARTESIAN_POINT('Ctrl Pts',(134.009237755298,-34.2071495541052,29.1533441918971));
#55462=CARTESIAN_POINT('Ctrl Pts',(134.031486234473,-34.3293606044579,29.1473119547345));
#55463=CARTESIAN_POINT('Ctrl Pts',(134.048129117943,-34.452390974814,29.141279717572));
#55464=CARTESIAN_POINT('Ctrl Pts',(134.064127723253,-34.5706586019449,29.135480999959));
#55465=CARTESIAN_POINT('Ctrl Pts',(134.07494660272,-34.68968285133,29.1296822823461));
#55466=CARTESIAN_POINT('Ctrl Pts',(134.080531097806,-34.8089739289099,29.1238835647332));
#55467=CARTESIAN_POINT('Ctrl Pts',(134.086114738203,-34.9282467493494,29.1180857345965));
#55468=CARTESIAN_POINT('Ctrl Pts',(134.086465568167,-35.0477859081848,29.1122879044598));
#55469=CARTESIAN_POINT('Ctrl Pts',(134.081580958514,-35.1670984114157,29.1064900743232));
#55470=CARTESIAN_POINT('Ctrl Pts',(134.076695937982,-35.2864209508477,29.1006917564909));
#55471=CARTESIAN_POINT('Ctrl Pts',(134.066574619032,-35.4055163879374,29.0948934386586));
#55472=CARTESIAN_POINT('Ctrl Pts',(134.051266437924,-35.5238943108626,29.0890951208262));
#55473=CARTESIAN_POINT('Ctrl Pts',(134.035953338598,-35.6423102662757,29.083294940109));
#55474=CARTESIAN_POINT('Ctrl Pts',(134.015450115566,-35.7600078435198,29.0774947593917));
#55475=CARTESIAN_POINT('Ctrl Pts',(133.989857648217,-35.8765049611768,29.0716945786744));
#55476=CARTESIAN_POINT('Ctrl Pts',(133.964236823605,-35.993131161322,29.0658879711735));
#55477=CARTESIAN_POINT('Ctrl Pts',(133.933515586623,-36.108553846956,29.0600813636727));
#55478=CARTESIAN_POINT('Ctrl Pts',(133.897845249922,-36.2223041387726,29.0542747561719));
#55479=CARTESIAN_POINT('Ctrl Pts',(133.862151509636,-36.3361290630372,29.0484643389108));
#55480=CARTESIAN_POINT('Ctrl Pts',(133.821502342285,-36.4482790245809,29.0426539216498));
#55481=CARTESIAN_POINT('Ctrl Pts',(133.776097343868,-36.5583047999775,29.0368435043888));
#55482=CARTESIAN_POINT('Ctrl Pts',(133.730627022299,-36.6684888669866,29.0310247278109));
#55483=CARTESIAN_POINT('Ctrl Pts',(133.680387385259,-36.776542278605,29.0252059512331));
#55484=CARTESIAN_POINT('Ctrl Pts',(133.625624161131,-36.8820399682843,29.0193871746552));
#55485=CARTESIAN_POINT('Ctrl Pts',(133.610614635819,-36.9109548152251,29.0177923621561));
#55486=CARTESIAN_POINT('Ctrl Pts',(133.595265549603,-36.9396778439786,29.0161975496569));
#55487=CARTESIAN_POINT('Ctrl Pts',(133.579582519736,-36.9682006971849,29.0146027371578));
#55488=CARTESIAN_POINT('Ctrl Pts',(133.522308753151,-37.0723649594993,29.0087785488726));
#55489=CARTESIAN_POINT('Ctrl Pts',(133.460392236228,-37.1741950094874,29.0029543605875));
#55490=CARTESIAN_POINT('Ctrl Pts',(133.394047946116,-37.2732495550351,28.9971301723023));
#55491=CARTESIAN_POINT('Ctrl Pts',(133.327787374183,-37.3721791061615,28.9913133334128));
#55492=CARTESIAN_POINT('Ctrl Pts',(133.25711036729,-37.4683397827467,28.9854964945232));
#55493=CARTESIAN_POINT('Ctrl Pts',(133.182277855087,-37.5613146337429,28.9796796556337));
#55494=CARTESIAN_POINT('Ctrl Pts',(133.107520279024,-37.6541963811351,28.9738686416383));
#55495=CARTESIAN_POINT('Ctrl Pts',(133.028615730497,-37.7438983333498,28.9680576276429));
#55496=CARTESIAN_POINT('Ctrl Pts',(132.945868171882,-37.8300328114511,28.9622466136476));
#55497=CARTESIAN_POINT('Ctrl Pts',(132.860000325613,-37.9194152929151,28.9562164749368));
#55498=CARTESIAN_POINT('Ctrl Pts',(132.769994184585,-38.0049555832903,28.950186336226));
#55499=CARTESIAN_POINT('Ctrl Pts',(132.676235306726,-38.0862581847653,28.9441561975153));
#55500=CARTESIAN_POINT('Ctrl Pts',(132.585985320004,-38.1645180666153,28.9383517345033));
#55501=CARTESIAN_POINT('Ctrl Pts',(132.492258774949,-38.2388514566586,28.9325472714912));
#55502=CARTESIAN_POINT('Ctrl Pts',(132.395436255544,-38.3089439622979,28.9267428084792));
#55503=CARTESIAN_POINT('Ctrl Pts',(132.298628121535,-38.3790260539491,28.9209392078648));
#55504=CARTESIAN_POINT('Ctrl Pts',(132.198725258541,-38.4448682749289,28.9151356072503));
#55505=CARTESIAN_POINT('Ctrl Pts',(132.09613941041,-38.5061980223776,28.9093320066359));
#55506=CARTESIAN_POINT('Ctrl Pts',(131.993544607804,-38.5675331231544,28.903527899439));
#55507=CARTESIAN_POINT('Ctrl Pts',(131.888266704849,-38.6243547577782,28.897723792242));
#55508=CARTESIAN_POINT('Ctrl Pts',(131.780743796715,-38.6764353020911,28.8919196850451));
#55509=CARTESIAN_POINT('Ctrl Pts',(131.673186142703,-38.7285326761596,28.8861137022589));
#55510=CARTESIAN_POINT('Ctrl Pts',(131.563382407934,-38.7758857350839,28.8803077194728));
#55511=CARTESIAN_POINT('Ctrl Pts',(131.45179189964,-38.818314455377,28.8745017366867));
#55512=CARTESIAN_POINT('Ctrl Pts',(131.34007806638,-38.8607900660422,28.8686893373815));
#55513=CARTESIAN_POINT('Ctrl Pts',(131.226573899806,-38.8983303298574,28.8628769380763));
#55514=CARTESIAN_POINT('Ctrl Pts',(131.111755298385,-38.9308046449186,28.8570645387711));
#55515=CARTESIAN_POINT('Ctrl Pts',(130.996861421357,-38.9633002502909,28.85124832883));
#55516=CARTESIAN_POINT('Ctrl Pts',(130.880651789694,-38.9907231989341,28.8454321188889));
#55517=CARTESIAN_POINT('Ctrl Pts',(130.763612332195,-39.0129940451139,28.8396159089478));
#55518=CARTESIAN_POINT('Ctrl Pts',(130.646405523634,-39.0352967356807,28.8337913825899));
#55519=CARTESIAN_POINT('Ctrl Pts',(130.528366923537,-39.0524325615092,28.827966856232));
#55520=CARTESIAN_POINT('Ctrl Pts',(130.409987550855,-39.0643739011247,28.8221423298741));
#55521=CARTESIAN_POINT('Ctrl Pts',(130.378694609615,-39.067530529095,28.8206026481125));
#55522=CARTESIAN_POINT('Ctrl Pts',(130.347377853411,-39.0703244591297,28.8190629663509));
#55523=CARTESIAN_POINT('Ctrl Pts',(130.316046331496,-39.0727557889405,28.8175232845893));
#55524=CARTESIAN_POINT('Ctrl Pts',(130.197522841049,-39.081953225834,28.8116988481941));
#55525=CARTESIAN_POINT('Ctrl Pts',(130.078407055875,-39.0859873249673,28.8058744117989));
#55526=CARTESIAN_POINT('Ctrl Pts',(129.959185970498,-39.0847961044581,28.8000499754037));
#55527=CARTESIAN_POINT('Ctrl Pts',(129.840114957166,-39.0836063834226,28.7942328706402));
#55528=CARTESIAN_POINT('Ctrl Pts',(129.720939311869,-39.0772044293515,28.7884157658766));
#55529=CARTESIAN_POINT('Ctrl Pts',(129.602150844744,-39.0655800385261,28.782598661113));
#55530=CARTESIAN_POINT('Ctrl Pts',(129.483480970749,-39.0539672529762,28.7767873638884));
#55531=CARTESIAN_POINT('Ctrl Pts',(129.365197909877,-39.0371424425923,28.7709760666639));
#55532=CARTESIAN_POINT('Ctrl Pts',(129.247792563708,-39.0151474409774,28.7651647694393));
#55533=CARTESIAN_POINT('Ctrl Pts',(129.125967987234,-38.9923245300647,28.7591347303802));
#55534=CARTESIAN_POINT('Ctrl Pts',(129.005088947621,-38.9639345635799,28.7531046913211));
#55535=CARTESIAN_POINT('Ctrl Pts',(128.885697490909,-38.9300833220473,28.747074652262));
#55536=CARTESIAN_POINT('Ctrl Pts',(128.770765880917,-38.8974965876467,28.741269864244));
#55537=CARTESIAN_POINT('Ctrl Pts',(128.657213137834,-38.8598493924904,28.735465076226));
#55538=CARTESIAN_POINT('Ctrl Pts',(128.54551084419,-38.8172878193335,28.7296602882079));
#55539=CARTESIAN_POINT('Ctrl Pts',(128.433824858422,-38.7747324599148,28.7238563476546));
#55540=CARTESIAN_POINT('Ctrl Pts',(128.323989166181,-38.7272642946276,28.7180524071013));
#55541=CARTESIAN_POINT('Ctrl Pts',(128.216457466505,-38.6750783707582,28.7122484665481));
#55542=CARTESIAN_POINT('Ctrl Pts',(128.108916110165,-38.6228877604385,28.7064440047837));
#55543=CARTESIAN_POINT('Ctrl Pts',(128.003679525028,-38.5659787273951,28.7006395430194));
#55544=CARTESIAN_POINT('Ctrl Pts',(127.90117822477,-38.5045930085844,28.6948350812551));
#55545=CARTESIAN_POINT('Ctrl Pts',(127.798643550248,-38.4431873026791,28.6890287295671));
#55546=CARTESIAN_POINT('Ctrl Pts',(127.698846281852,-38.3773022217518,28.683222377879));
#55547=CARTESIAN_POINT('Ctrl Pts',(127.602188739063,-38.3072233303669,28.677416026191));
#55548=CARTESIAN_POINT('Ctrl Pts',(127.505424056115,-38.2370667599581,28.6716032384461));
#55549=CARTESIAN_POINT('Ctrl Pts',(127.411806376296,-38.1627073397506,28.6657904507012));
#55550=CARTESIAN_POINT('Ctrl Pts',(127.321705771227,-38.0844715956094,28.6599776629563));
#55551=CARTESIAN_POINT('Ctrl Pts',(127.231545916034,-38.0061844036722,28.6541610527243));
#55552=CARTESIAN_POINT('Ctrl Pts',(127.144908037172,-37.9240160914809,28.6483444424924));
#55553=CARTESIAN_POINT('Ctrl Pts',(127.062124911162,-37.8383296077776,28.6425278322604));
#55554=CARTESIAN_POINT('Ctrl Pts',(126.979223219008,-37.7525203995956,28.6367028911876));
#55555=CARTESIAN_POINT('Ctrl Pts',(126.900187568794,-37.6631832671508,28.6308779501148));
#55556=CARTESIAN_POINT('Ctrl Pts',(126.825310176905,-37.5707138166536,28.625053009042));
#55557=CARTESIAN_POINT('Ctrl Pts',(126.805560440396,-37.5463239809995,28.6235166167016));
#55558=CARTESIAN_POINT('Ctrl Pts',(126.786099756637,-37.5217163825431,28.6219802243613));
#55559=CARTESIAN_POINT('Ctrl Pts',(126.766932971494,-37.4968985940935,28.6204438320209));
#55560=CARTESIAN_POINT('Ctrl Pts',(126.694299748913,-37.4028506909643,28.6146216179148));
#55561=CARTESIAN_POINT('Ctrl Pts',(126.625652077838,-37.3054735001323,28.6087994038087));
#55562=CARTESIAN_POINT('Ctrl Pts',(126.561310097123,-37.2051387148773,28.6029771897026));
#55563=CARTESIAN_POINT('Ctrl Pts',(126.497047713044,-37.1049280524929,28.5971621781826));
#55564=CARTESIAN_POINT('Ctrl Pts',(126.437080646904,-37.0017674101151,28.5913471666625));
#55565=CARTESIAN_POINT('Ctrl Pts',(126.381688651695,-36.8960611769474,28.5855321551425));
#55566=CARTESIAN_POINT('Ctrl Pts',(126.326352129164,-36.790460803983,28.5797229671041));
#55567=CARTESIAN_POINT('Ctrl Pts',(126.27558175395,-36.6823202689564,28.5739137790656));
#55568=CARTESIAN_POINT('Ctrl Pts',(126.229613473537,-36.5720720215907,28.5681045910272));
#55569=CARTESIAN_POINT('Ctrl Pts',(126.183680399074,-36.461908210584,28.5622998520997));
#55570=CARTESIAN_POINT('Ctrl Pts',(126.142542259572,-36.3496402734931,28.5564951131722));
#55571=CARTESIAN_POINT('Ctrl Pts',(126.106388325008,-36.2357237249349,28.5506903742447));
#55572=CARTESIAN_POINT('Ctrl Pts',(126.070251484944,-36.1218610390188,28.5448883799455));
#55573=CARTESIAN_POINT('Ctrl Pts',(126.039094285826,-36.0063516800894,28.5390863856462));
#55574=CARTESIAN_POINT('Ctrl Pts',(126.01305705638,-35.8896690195346,28.533284391347));
#55575=CARTESIAN_POINT('Ctrl Pts',(125.987027133808,-35.7730191038418,28.5274840252717));
#55576=CARTESIAN_POINT('Ctrl Pts',(125.966114408067,-35.655196940161,28.5216836591964));
#55577=CARTESIAN_POINT('Ctrl Pts',(125.950408564446,-35.5366881823662,28.5158832931211));
#55578=CARTESIAN_POINT('Ctrl Pts',(125.934700135524,-35.418159917126,28.5100819722613));
#55579=CARTESIAN_POINT('Ctrl Pts',(125.92420035633,-35.2989452362512,28.5042806514015));
#55580=CARTESIAN_POINT('Ctrl Pts',(125.918947247676,-35.179536717001,28.4984793305417));
#55581=CARTESIAN_POINT('Ctrl Pts',(125.916271699447,-35.1187187759861,28.4955245632263));
#55582=CARTESIAN_POINT('Ctrl Pts',(125.914956375687,-35.0578506198813,28.4925697959109));
#55583=CARTESIAN_POINT('Ctrl Pts',(125.915001103444,-34.9969974789589,28.4896150285955));
#55584=CARTESIAN_POINT('Origin',(130.,-35.,17.));
#55585=CARTESIAN_POINT('Ctrl Pts',(133.378768828602,-35.2726284383002,17.));
#55586=CARTESIAN_POINT('Ctrl Pts',(133.398288246238,-35.1664583073869,17.0000000000001));
#55587=CARTESIAN_POINT('Ctrl Pts',(133.412279037496,-35.0595484327477,17.0000000000002));
#55588=CARTESIAN_POINT('Ctrl Pts',(133.420978754548,-34.9522469234893,17.0000000000001));
#55589=CARTESIAN_POINT('Ctrl Pts',(133.4296784716,-34.8449454142309,17.));
#55590=CARTESIAN_POINT('Ctrl Pts',(133.433086995943,-34.7372515853272,17.));
#55591=CARTESIAN_POINT('Ctrl Pts',(133.431392639095,-34.6294944550508,17.));
#55592=CARTESIAN_POINT('Ctrl Pts',(133.430532659945,-34.5748017936812,17.));
#55593=CARTESIAN_POINT('Ctrl Pts',(133.428357343707,-34.5200925845888,17.0000000000001));
#55594=CARTESIAN_POINT('Ctrl Pts',(133.424886608819,-34.465408836506,17.));
#55595=CARTESIAN_POINT('Ctrl Pts',(133.423593739603,-34.4450388178326,17.));
#55596=CARTESIAN_POINT('Ctrl Pts',(133.422121635848,-34.4246812381163,17.));
#55597=CARTESIAN_POINT('Ctrl Pts',(133.420471959324,-34.4043410098082,17.));
#55598=CARTESIAN_POINT('Ctrl Pts',(133.411386307087,-34.2923164776353,16.9999999999999));
#55599=CARTESIAN_POINT('Ctrl Pts',(133.396916955542,-34.1807930555395,17.0000000000002));
#55600=CARTESIAN_POINT('Ctrl Pts',(133.377281863082,-34.0701359071285,17.0000000000002));
#55601=CARTESIAN_POINT('Ctrl Pts',(133.360260736019,-33.9742102379531,17.0000000000002));
#55602=CARTESIAN_POINT('Ctrl Pts',(133.339356815858,-33.8789349316622,17.0000000000003));
#55603=CARTESIAN_POINT('Ctrl Pts',(133.314680668356,-33.7845430961811,17.0000000000002));
#55604=CARTESIAN_POINT('Ctrl Pts',(133.305738882743,-33.7503387473677,17.0000000000001));
#55605=CARTESIAN_POINT('Ctrl Pts',(133.296301499474,-33.7162503957036,16.9999999999999));
#55606=CARTESIAN_POINT('Ctrl Pts',(133.286372866255,-33.6822891544893,17.));
#55607=CARTESIAN_POINT('Ctrl Pts',(133.279074612109,-33.6573252179607,17.0000000000002));
#55608=CARTESIAN_POINT('Ctrl Pts',(133.271509097602,-33.6324245812173,17.));
#55609=CARTESIAN_POINT('Ctrl Pts',(133.263688075278,-33.6076228894364,17.));
#55610=CARTESIAN_POINT('Ctrl Pts',(133.229059460988,-33.4978101075652,17.));
#55611=CARTESIAN_POINT('Ctrl Pts',(133.189399626582,-33.3898390969386,17.0000000000001));
#55612=CARTESIAN_POINT('Ctrl Pts',(133.144933359838,-33.2840773063132,17.));
#55613=CARTESIAN_POINT('Ctrl Pts',(133.099802502295,-33.176734804779,17.));
#55614=CARTESIAN_POINT('Ctrl Pts',(133.049720392207,-33.0716671799564,16.9999999999999));
#55615=CARTESIAN_POINT('Ctrl Pts',(132.994868514162,-32.9692566318156,17.));
#55616=CARTESIAN_POINT('Ctrl Pts',(132.940479847808,-32.8677109175681,17.0000000000001));
#55617=CARTESIAN_POINT('Ctrl Pts',(132.881401361892,-32.768776718664,17.0000000000001));
#55618=CARTESIAN_POINT('Ctrl Pts',(132.817760633728,-32.6728378225391,17.0000000000001));
#55619=CARTESIAN_POINT('Ctrl Pts',(132.780118924681,-32.616092651352,17.0000000000001));
#55620=CARTESIAN_POINT('Ctrl Pts',(132.740880248093,-32.5603956288563,17.));
#55621=CARTESIAN_POINT('Ctrl Pts',(132.700063340168,-32.5058299364338,16.9999999999999));
#55622=CARTESIAN_POINT('Ctrl Pts',(132.678441129705,-32.476924491469,16.9999999999999));
#55623=CARTESIAN_POINT('Ctrl Pts',(132.65637594081,-32.4483365778201,17.0000000000002));
#55624=CARTESIAN_POINT('Ctrl Pts',(132.633869936992,-32.4200789995526,17.));
#55625=CARTESIAN_POINT('Ctrl Pts',(132.623920095448,-32.4075864029794,17.));
#55626=CARTESIAN_POINT('Ctrl Pts',(132.613884890735,-32.3951594678565,16.9999999999999));
#55627=CARTESIAN_POINT('Ctrl Pts',(132.603772440782,-32.3828086916134,16.9999999999999));
#55628=CARTESIAN_POINT('Ctrl Pts',(132.528293751701,-32.2906232761805,17.));
#55629=CARTESIAN_POINT('Ctrl Pts',(132.448401459479,-32.202535222033,17.0000000000001));
#55630=CARTESIAN_POINT('Ctrl Pts',(132.364286473895,-32.1189321572606,17.0000000000001));
#55631=CARTESIAN_POINT('Ctrl Pts',(132.340801349937,-32.095589962932,17.0000000000001));
#55632=CARTESIAN_POINT('Ctrl Pts',(132.316986747461,-32.0725974700126,16.9999999999999));
#55633=CARTESIAN_POINT('Ctrl Pts',(132.292846130803,-32.0499633408993,16.9999999999999));
#55634=CARTESIAN_POINT('Ctrl Pts',(132.208772055331,-31.9711358815073,16.9999999999999));
#55635=CARTESIAN_POINT('Ctrl Pts',(132.120747300731,-31.8966525443055,16.9999999999999));
#55636=CARTESIAN_POINT('Ctrl Pts',(132.029197860355,-31.8265245910536,16.9999999999999));
#55637=CARTESIAN_POINT('Ctrl Pts',(131.937648419978,-31.7563966378017,17.));
#55638=CARTESIAN_POINT('Ctrl Pts',(131.842573618672,-31.6906237914098,17.));
#55639=CARTESIAN_POINT('Ctrl Pts',(131.744359117884,-31.629251345085,17.));
#55640=CARTESIAN_POINT('Ctrl Pts',(131.6882846066,-31.5942114079436,17.));
#55641=CARTESIAN_POINT('Ctrl Pts',(131.63118595824,-31.5606065213418,17.));
#55642=CARTESIAN_POINT('Ctrl Pts',(131.573130353031,-31.528450628799,17.));
#55643=CARTESIAN_POINT('Ctrl Pts',(131.556946837447,-31.5194868881541,17.));
#55644=CARTESIAN_POINT('Ctrl Pts',(131.540688943071,-31.5106357689599,17.));
#55645=CARTESIAN_POINT('Ctrl Pts',(131.524358087669,-31.5018976324805,17.));
#55646=CARTESIAN_POINT('Ctrl Pts',(131.511363461925,-31.4949446094788,17.));
#55647=CARTESIAN_POINT('Ctrl Pts',(131.498323714352,-31.4880637401771,17.));
#55648=CARTESIAN_POINT('Ctrl Pts',(131.485248425713,-31.4812596596424,17.));
#55649=CARTESIAN_POINT('Ctrl Pts',(131.379202552098,-31.426075817483,17.0000000000001));
#55650=CARTESIAN_POINT('Ctrl Pts',(131.270666658491,-31.375856441141,17.));
#55651=CARTESIAN_POINT('Ctrl Pts',(131.160094992004,-31.3306020577967,17.));
#55652=CARTESIAN_POINT('Ctrl Pts',(131.047641736312,-31.2845775842305,17.0000000000001));
#55653=CARTESIAN_POINT('Ctrl Pts',(130.933082172006,-31.243688134086,17.));
#55654=CARTESIAN_POINT('Ctrl Pts',(130.816854357636,-31.2079719988663,17.));
#55655=CARTESIAN_POINT('Ctrl Pts',(130.69920023221,-31.1718175665076,17.));
#55656=CARTESIAN_POINT('Ctrl Pts',(130.579835885835,-31.1409637990667,17.));
#55657=CARTESIAN_POINT('Ctrl Pts',(130.459186272896,-31.1154946922679,17.));
#55658=CARTESIAN_POINT('Ctrl Pts',(130.384595675,-31.0997486334307,17.));
#55659=CARTESIAN_POINT('Ctrl Pts',(130.309513284361,-31.0860616069785,17.));
#55660=CARTESIAN_POINT('Ctrl Pts',(130.234036026462,-31.0744627946408,17.));
#55661=CARTESIAN_POINT('Ctrl Pts',(130.197795458841,-31.0688935999647,17.));
#55662=CARTESIAN_POINT('Ctrl Pts',(130.161463827202,-31.0638059443293,17.));
#55663=CARTESIAN_POINT('Ctrl Pts',(130.125051741993,-31.0592036806989,17.));
#55664=CARTESIAN_POINT('Ctrl Pts',(130.107528311351,-31.0569888268377,17.));
#55665=CARTESIAN_POINT('Ctrl Pts',(130.089984287133,-31.0548861776152,17.));
#55666=CARTESIAN_POINT('Ctrl Pts',(130.072427070294,-31.052896897432,17.));
#55667=CARTESIAN_POINT('Ctrl Pts',(129.946714827881,-31.0386533601501,17.));
#55668=CARTESIAN_POINT('Ctrl Pts',(129.820703894979,-31.0302595130221,17.));
#55669=CARTESIAN_POINT('Ctrl Pts',(129.69485817944,-31.0277503025434,17.));
#55670=CARTESIAN_POINT('Ctrl Pts',(129.568768654346,-31.0252362307988,17.));
#55671=CARTESIAN_POINT('Ctrl Pts',(129.442844100505,-31.02862930582,17.));
#55672=CARTESIAN_POINT('Ctrl Pts',(129.317528571408,-31.0380119206155,17.));
#55673=CARTESIAN_POINT('Ctrl Pts',(129.194473966571,-31.047225255661,17.));
#55674=CARTESIAN_POINT('Ctrl Pts',(129.072005730894,-31.0622138114403,17.));
#55675=CARTESIAN_POINT('Ctrl Pts',(128.950535741321,-31.0831042418908,17.));
#55676=CARTESIAN_POINT('Ctrl Pts',(128.859102153225,-31.0988290066634,17.));
#55677=CARTESIAN_POINT('Ctrl Pts',(128.768233909816,-31.1178987055077,17.));
#55678=CARTESIAN_POINT('Ctrl Pts',(128.678107868388,-31.1403868954586,17.));
#55679=CARTESIAN_POINT('Ctrl Pts',(128.630400840111,-31.1522907214436,17.));
#55680=CARTESIAN_POINT('Ctrl Pts',(128.582901820088,-31.1651527026015,17.));
#55681=CARTESIAN_POINT('Ctrl Pts',(128.535626875521,-31.178955003241,17.));
#55682=CARTESIAN_POINT('Ctrl Pts',(126.824949217806,-32.429732011932,17.));
#55683=CARTESIAN_POINT('Ctrl Pts',(126.754722564964,-32.5331868396527,17.0000000000001));
#55684=CARTESIAN_POINT('Ctrl Pts',(126.689770328881,-32.6399361026362,17.0000000000001));
#55685=CARTESIAN_POINT('Ctrl Pts',(126.630097033085,-32.7495483500992,17.0000000000001));
#55686=CARTESIAN_POINT('Ctrl Pts',(126.569576097871,-32.8607176032622,17.));
#55687=CARTESIAN_POINT('Ctrl Pts',(126.51448500206,-32.9748326342131,17.0000000000002));
#55688=CARTESIAN_POINT('Ctrl Pts',(126.464879563014,-33.0914584109723,17.0000000000001));
#55689=CARTESIAN_POINT('Ctrl Pts',(126.443235134053,-33.1423459424326,17.0000000000001));
#55690=CARTESIAN_POINT('Ctrl Pts',(126.422635756764,-33.1937115953365,17.0000000000003));
#55691=CARTESIAN_POINT('Ctrl Pts',(126.403089154084,-33.2455194506075,17.0000000000001));
#55692=CARTESIAN_POINT('Ctrl Pts',(126.392820709654,-33.2727357444875,16.9999999999999));
#55693=CARTESIAN_POINT('Ctrl Pts',(126.382841496993,-33.3000781943394,17.));
#55694=CARTESIAN_POINT('Ctrl Pts',(126.37316194691,-33.3275147827857,17.));
#55695=CARTESIAN_POINT('Ctrl Pts',(126.331490200439,-33.4456329337216,16.9999999999999));
#55696=CARTESIAN_POINT('Ctrl Pts',(126.295333265067,-33.5655832581459,17.0000000000001));
#55697=CARTESIAN_POINT('Ctrl Pts',(126.264731200303,-33.686937606849,17.0000000000001));
#55698=CARTESIAN_POINT('Ctrl Pts',(126.239067787757,-33.7887074298646,17.));
#55699=CARTESIAN_POINT('Ctrl Pts',(126.217311899518,-33.8914651743243,17.0000000000002));
#55700=CARTESIAN_POINT('Ctrl Pts',(126.199515422177,-33.9949584531853,17.0000000000001));
#55701=CARTESIAN_POINT('Ctrl Pts',(126.191672483203,-34.0405681238387,17.));
#55702=CARTESIAN_POINT('Ctrl Pts',(126.184598869754,-34.0863206118168,16.9999999999998));
#55703=CARTESIAN_POINT('Ctrl Pts',(126.178300615437,-34.1321940133029,17.));
#55704=CARTESIAN_POINT('Ctrl Pts',(126.175607336728,-34.1518105370754,17.0000000000001));
#55705=CARTESIAN_POINT('Ctrl Pts',(126.173055853477,-34.1714491679886,17.));
#55706=CARTESIAN_POINT('Ctrl Pts',(126.170646691963,-34.1911081767111,17.));
#55707=CARTESIAN_POINT('Ctrl Pts',(126.168408134718,-34.2093750368465,16.9999999999999));
#55708=CARTESIAN_POINT('Ctrl Pts',(126.166292933428,-34.2276559610749,17.0000000000003));
#55709=CARTESIAN_POINT('Ctrl Pts',(126.164302324029,-34.2459397516365,17.0000000000002));
#55710=CARTESIAN_POINT('Ctrl Pts',(126.151067617198,-34.3675008213213,17.0000000000001));
#55711=CARTESIAN_POINT('Ctrl Pts',(126.143320213443,-34.4893160661783,17.));
#55712=CARTESIAN_POINT('Ctrl Pts',(126.141093992317,-34.6109885614732,17.));
#55713=CARTESIAN_POINT('Ctrl Pts',(126.138877610836,-34.7321232781618,16.9999999999999));
#55714=CARTESIAN_POINT('Ctrl Pts',(126.14213377111,-34.8531173504601,17.));
#55715=CARTESIAN_POINT('Ctrl Pts',(126.150946782328,-34.973572328076,17.0000000000001));
#55716=CARTESIAN_POINT('Ctrl Pts',(126.159510425353,-35.0906189768731,17.0000000000001));
#55717=CARTESIAN_POINT('Ctrl Pts',(126.173321132798,-35.2071572701507,17.0000000000001));
#55718=CARTESIAN_POINT('Ctrl Pts',(126.192501970979,-35.322804279403,17.0000000000002));
#55719=CARTESIAN_POINT('Ctrl Pts',(126.204193875272,-35.3932982667441,17.0000000000002));
#55720=CARTESIAN_POINT('Ctrl Pts',(126.217882010487,-35.4634607028539,16.9999999999999));
#55721=CARTESIAN_POINT('Ctrl Pts',(126.233602445872,-35.5332000053698,16.9999999999999));
#55722=CARTESIAN_POINT('Ctrl Pts',(126.243155310077,-35.5755786081459,16.9999999999999));
#55723=CARTESIAN_POINT('Ctrl Pts',(126.253458751899,-35.6178008839807,17.));
#55724=CARTESIAN_POINT('Ctrl Pts',(126.264521983881,-35.6598454466932,16.9999999999999));
#55725=CARTESIAN_POINT('Ctrl Pts',(126.269462009858,-35.6786194570633,16.9999999999999));
#55726=CARTESIAN_POINT('Ctrl Pts',(126.274554024022,-35.6973594264633,17.));
#55727=CARTESIAN_POINT('Ctrl Pts',(126.279792975253,-35.7160432617782,17.));
#55728=CARTESIAN_POINT('Ctrl Pts',(126.311062580707,-35.8275610318175,16.9999999999999));
#55729=CARTESIAN_POINT('Ctrl Pts',(126.34760531646,-35.937246500656,16.9999999999999));
#55730=CARTESIAN_POINT('Ctrl Pts',(126.3894966474,-36.0447443535775,16.9999999999999));
#55731=CARTESIAN_POINT('Ctrl Pts',(126.402466834512,-36.0780273081938,16.9999999999999));
#55732=CARTESIAN_POINT('Ctrl Pts',(126.415950090396,-36.1111004102563,17.));
#55733=CARTESIAN_POINT('Ctrl Pts',(126.429949578689,-36.1439526727213,17.));
#55734=CARTESIAN_POINT('Ctrl Pts',(126.475866127408,-36.2517039332289,17.0000000000001));
#55735=CARTESIAN_POINT('Ctrl Pts',(126.527332973336,-36.3570819762472,17.0000000000002));
#55736=CARTESIAN_POINT('Ctrl Pts',(126.58400504888,-36.45981771484,17.));
#55737=CARTESIAN_POINT('Ctrl Pts',(126.641107329219,-36.5633333332401,16.9999999999998));
#55738=CARTESIAN_POINT('Ctrl Pts',(126.703494928383,-36.6641669871817,17.));
#55739=CARTESIAN_POINT('Ctrl Pts',(126.770850629467,-36.7620050500939,16.9999999999999));
#55740=CARTESIAN_POINT('Ctrl Pts',(126.804493487409,-36.8108732527689,16.9999999999999));
#55741=CARTESIAN_POINT('Ctrl Pts',(126.839376275211,-36.8589934594567,17.0000000000001));
#55742=CARTESIAN_POINT('Ctrl Pts',(126.87546185721,-36.9063223196442,17.0000000000001));
#55743=CARTESIAN_POINT('Ctrl Pts',(126.886663998762,-36.9210147414354,17.0000000000001));
#55744=CARTESIAN_POINT('Ctrl Pts',(126.897982060954,-36.9356308801713,17.));
#55745=CARTESIAN_POINT('Ctrl Pts',(126.909414956083,-36.9501693775893,17.0000000000001));
#55746=CARTESIAN_POINT('Ctrl Pts',(126.919260361815,-36.9626891640644,17.0000000000001));
#55747=CARTESIAN_POINT('Ctrl Pts',(126.929187993614,-36.9751475918217,17.0000000000001));
#55748=CARTESIAN_POINT('Ctrl Pts',(126.93919204257,-36.9875378873469,17.));
#55749=CARTESIAN_POINT('Ctrl Pts',(127.01206530898,-37.0777934739326,16.9999999999999));
#55750=CARTESIAN_POINT('Ctrl Pts',(127.089068527172,-37.1645366085542,16.9999999999999));
#55751=CARTESIAN_POINT('Ctrl Pts',(127.169856641689,-37.2475215103742,16.9999999999999));
#55752=CARTESIAN_POINT('Ctrl Pts',(127.25039235393,-37.3302471466052,17.));
#55753=CARTESIAN_POINT('Ctrl Pts',(127.334690166794,-37.4092384879766,17.0000000000001));
#55754=CARTESIAN_POINT('Ctrl Pts',(127.422439583585,-37.4842112339295,17.));
#55755=CARTESIAN_POINT('Ctrl Pts',(127.509315422489,-37.558437598478,16.9999999999999));
#55756=CARTESIAN_POINT('Ctrl Pts',(127.599575260046,-37.6287253893366,16.9999999999999));
#55757=CARTESIAN_POINT('Ctrl Pts',(127.692936664564,-37.6947520496931,17.0000000000001));
#55758=CARTESIAN_POINT('Ctrl Pts',(127.745228885034,-37.7317339342105,17.0000000000001));
#55759=CARTESIAN_POINT('Ctrl Pts',(127.798494396841,-37.7673781515159,17.));
#55760=CARTESIAN_POINT('Ctrl Pts',(127.852684844814,-37.8016208067591,17.));
#55761=CARTESIAN_POINT('Ctrl Pts',(127.881422150523,-37.8197797570693,17.0000000000001));
#55762=CARTESIAN_POINT('Ctrl Pts',(127.910419576427,-37.8375444684963,16.9999999999999));
#55763=CARTESIAN_POINT('Ctrl Pts',(127.939669941168,-37.8549047719967,16.9999999999999));
#55764=CARTESIAN_POINT('Ctrl Pts',(127.956236675144,-37.8647372486984,17.));
#55765=CARTESIAN_POINT('Ctrl Pts',(127.972886345269,-37.8744409183027,17.));
#55766=CARTESIAN_POINT('Ctrl Pts',(127.989598062667,-37.8840029632689,17.));
#55767=CARTESIAN_POINT('Ctrl Pts',(128.08642888323,-37.9394072426899,17.0000000000001));
#55768=CARTESIAN_POINT('Ctrl Pts',(128.18548331692,-37.9901465489129,16.9999999999999));
#55769=CARTESIAN_POINT('Ctrl Pts',(128.286476552124,-38.0359637356346,16.9999999999999));
#55770=CARTESIAN_POINT('Ctrl Pts',(128.385961066845,-38.0810964673239,16.9999999999999));
#55771=CARTESIAN_POINT('Ctrl Pts',(128.487327606991,-38.1214533278655,17.));
#55772=CARTESIAN_POINT('Ctrl Pts',(128.590315969054,-38.1567401839697,17.));
#55773=CARTESIAN_POINT('Ctrl Pts',(128.690232540977,-38.1909745540018,17.));
#55774=CARTESIAN_POINT('Ctrl Pts',(128.7916762279,-38.220436955216,17.));
#55775=CARTESIAN_POINT('Ctrl Pts',(128.89441127067,-38.2448103330173,17.));
#55776=CARTESIAN_POINT('Ctrl Pts',(128.959370040939,-38.2602214781005,17.));
#55777=CARTESIAN_POINT('Ctrl Pts',(129.024845096459,-38.2735970799981,17.));
#55778=CARTESIAN_POINT('Ctrl Pts',(129.090775666099,-38.2848462111391,17.));
#55779=CARTESIAN_POINT('Ctrl Pts',(129.131408328244,-38.2917789912983,17.));
#55780=CARTESIAN_POINT('Ctrl Pts',(129.172213989212,-38.2979038932228,17.));
#55781=CARTESIAN_POINT('Ctrl Pts',(129.213170804443,-38.3032244865145,17.));
#55782=CARTESIAN_POINT('Ctrl Pts',(132.56705599117,-32.7956090760829,29.9966206630762));
#55783=CARTESIAN_POINT('Ctrl Pts',(133.295540663306,-33.6438478316206,29.9308808351505));
#55784=CARTESIAN_POINT('Ctrl Pts',(133.832377684159,-36.1047329053186,29.7994478563687));
#55785=CARTESIAN_POINT('Ctrl Pts',(131.173363843183,-38.8159059974858,29.6023217267306));
#55786=CARTESIAN_POINT('Ctrl Pts',(127.452981180699,-38.0706344938751,29.4052422741622));
#55787=CARTESIAN_POINT('Ctrl Pts',(126.035010329987,-34.5541540104475,29.2081628215937));
#55788=CARTESIAN_POINT('Ctrl Pts',(128.199728320707,-31.4388221268633,29.0110833690253));
#55789=CARTESIAN_POINT('Ctrl Pts',(131.991478820009,-31.5424762882451,28.8140039164569));
#55790=CARTESIAN_POINT('Ctrl Pts',(133.983498939676,-34.7701917247564,28.6169244638884));
#55791=CARTESIAN_POINT('Ctrl Pts',(132.375780338592,-38.2057763622061,28.41984501132));
#55792=CARTESIAN_POINT('Ctrl Pts',(128.621113687997,-38.744292389259,28.2227655587515));
#55793=CARTESIAN_POINT('Ctrl Pts',(126.112518759346,-35.8992392442492,28.0256861061831));
#55794=CARTESIAN_POINT('Ctrl Pts',(127.116930427117,-32.2415456859938,27.8286066536146));
#55795=CARTESIAN_POINT('Ctrl Pts',(130.726696025998,-31.0766031807178,27.6315272010462));
#55796=CARTESIAN_POINT('Ctrl Pts',(133.679765074078,-33.4571226309144,27.4344477484778));
#55797=CARTESIAN_POINT('Ctrl Pts',(133.307530867572,-37.2319009861223,27.2373682959093));
#55798=CARTESIAN_POINT('Ctrl Pts',(129.946370573864,-38.9897698055861,27.0402888433409));
#55799=CARTESIAN_POINT('Ctrl Pts',(126.633673858793,-37.1421925771597,26.8432093907724));
#55800=CARTESIAN_POINT('Ctrl Pts',(126.363034610644,-33.3587738001739,26.646129938204));
#55801=CARTESIAN_POINT('Ctrl Pts',(129.379022256961,-31.058486712473,26.4490504856355));
#55802=CARTESIAN_POINT('Ctrl Pts',(132.956170614085,-32.3200380901321,26.2519710330671));
#55803=CARTESIAN_POINT('Ctrl Pts',(133.86190786446,-36.0033983074205,26.0548915804986));
#55804=CARTESIAN_POINT('Ctrl Pts',(131.277743838984,-38.780014704575,25.8578121279302));
#55805=CARTESIAN_POINT('Ctrl Pts',(127.538917403056,-38.1407344615195,25.6607326753618));
#55806=CARTESIAN_POINT('Ctrl Pts',(126.024104482112,-34.6632577640359,25.4636532227933));
#55807=CARTESIAN_POINT('Ctrl Pts',(128.102200381387,-31.4900858832021,25.2665737702249));
#55808=CARTESIAN_POINT('Ctrl Pts',(131.895286263836,-31.488728082256,25.0694943176564));
#55809=CARTESIAN_POINT('Ctrl Pts',(133.975653413485,-34.6604113703016,24.872414865088));
#55810=CARTESIAN_POINT('Ctrl Pts',(132.463330526414,-38.1389716817721,24.6753354125196));
#55811=CARTESIAN_POINT('Ctrl Pts',(128.724962730802,-38.7809285187328,24.4782559599511));
#55812=CARTESIAN_POINT('Ctrl Pts',(126.138811493571,-36.0061629188847,24.2811765073827));
#55813=CARTESIAN_POINT('Ctrl Pts',(127.041911464645,-32.3221552101542,24.0840970548142));
#55814=CARTESIAN_POINT('Ctrl Pts',(130.618155722524,-31.0580431250146,23.8870176022458));
#55815=CARTESIAN_POINT('Ctrl Pts',(133.63578943908,-33.3561704296975,23.6899381496773));
#55816=CARTESIAN_POINT('Ctrl Pts',(133.367858964113,-37.1397818812582,23.4928586971089));
#55817=CARTESIAN_POINT('Ctrl Pts',(130.056485792592,-38.9897305493931,23.2957792445405));
#55818=CARTESIAN_POINT('Ctrl Pts',(126.694067944094,-37.2342680553723,23.098699791972));
#55819=CARTESIAN_POINT('Ctrl Pts',(126.31913112674,-33.4597581880133,22.9016203394036));
#55820=CARTESIAN_POINT('Ctrl Pts',(129.27049556151,-31.0771230231173,22.7045408868351));
#55821=CARTESIAN_POINT('Ctrl Pts',(132.881093348709,-32.239485262215,22.5074614342667));
#55822=CARTESIAN_POINT('Ctrl Pts',(133.888125308583,-35.8964497120742,22.3103819816983));
#55823=CARTESIAN_POINT('Ctrl Pts',(131.381564003476,-38.743316898943,22.1133025291298));
#55824=CARTESIAN_POINT('Ctrl Pts',(127.626520822797,-38.207450248518,21.9162230765614));
#55825=CARTESIAN_POINT('Ctrl Pts',(126.016326326165,-34.7730979022514,21.7191436239929));
#55826=CARTESIAN_POINT('Ctrl Pts',(128.006069557745,-31.5437908203244,21.5220641714245));
#55827=CARTESIAN_POINT('Ctrl Pts',(131.797673587636,-31.4377661261477,21.324984718856));
#55828=CARTESIAN_POINT('Ctrl Pts',(133.964768809745,-34.550835455637,21.1279052662876));
#55829=CARTESIAN_POINT('Ctrl Pts',(132.549010115704,-38.0698025892216,20.9308258137191));
#55830=CARTESIAN_POINT('Ctrl Pts',(128.829780195416,-38.8146724753018,20.7337463611507));
#55831=CARTESIAN_POINT('Ctrl Pts',(126.168046135565,-36.1123264348889,20.5366669085822));
#55832=CARTESIAN_POINT('Ctrl Pts',(126.969144734657,-32.4048011832485,20.3395874560138));
#55833=CARTESIAN_POINT('Ctrl Pts',(130.5091449328,-31.0424866657829,20.1425080034454));
#55834=CARTESIAN_POINT('Ctrl Pts',(133.589044692203,-33.2564694210485,19.9454285508769));
#55835=CARTESIAN_POINT('Ctrl Pts',(133.425622193847,-37.0460335558426,19.7483490983085));
#55836=CARTESIAN_POINT('Ctrl Pts',(130.166557987812,-38.9866524370216,19.5512696457401));
#55837=CARTESIAN_POINT('Ctrl Pts',(126.75697974509,-37.3246423548653,19.3541901931716));
#55838=CARTESIAN_POINT('Ctrl Pts',(126.278031065997,-33.5619148736047,19.1571107406032));
#55839=CARTESIAN_POINT('Ctrl Pts',(129.162524195305,-31.0987484069462,18.9600312880347));
#55840=CARTESIAN_POINT('Ctrl Pts',(132.803822405259,-32.1610318275282,18.7629518354663));
#55841=CARTESIAN_POINT('Ctrl Pts',(133.911380504042,-35.7888245479408,18.5658723828978));
#55842=CARTESIAN_POINT('Ctrl Pts',(131.484334257128,-38.703755495549,18.3687929303294));
#55843=CARTESIAN_POINT('Ctrl Pts',(127.715927155011,-38.2717496145793,18.171713477761));
#55844=CARTESIAN_POINT('Ctrl Pts',(126.011591817358,-34.8830563622797,17.9746340251925));
#55845=CARTESIAN_POINT('Ctrl Pts',(127.911437163445,-31.6002406871,17.7775545726241));
#55846=CARTESIAN_POINT('Ctrl Pts',(131.698733465358,-31.3892839246133,17.5804751200556));
#55847=CARTESIAN_POINT('Ctrl Pts',(133.950778614665,-34.4420841751546,17.3833956674872));
#55848=CARTESIAN_POINT('Ctrl Pts',(132.632927369956,-37.9972978706467,17.1863162149187));
#55849=CARTESIAN_POINT('Ctrl Pts',(128.935134434648,-38.8475943936263,16.9892367623503));
#55850=CARTESIAN_POINT('Ctrl Pts',(126.201080798138,-36.2134083112296,16.7921573097818));
#55851=CARTESIAN_POINT('Ctrl Pts',(126.667056273216,-33.7394457916199,16.6607710080696));
#55852=CARTESIAN_POINT('Ctrl Pts',(127.370067526471,-32.8710163360532,16.5950778572134));
#55853=CARTESIAN_POINT('Ctrl Pts',(132.745392735114,-32.6424671496488,30.1323365993077));
#55854=CARTESIAN_POINT('Ctrl Pts',(133.524486192134,-33.5496341631874,30.066596771382));
#55855=CARTESIAN_POINT('Ctrl Pts',(134.098617984373,-36.1814801480512,29.9351637926001));
#55856=CARTESIAN_POINT('Ctrl Pts',(131.254878967113,-39.0810019880405,29.7380376629621));
#55857=CARTESIAN_POINT('Ctrl Pts',(127.276036445345,-38.2839554963636,29.5409582103937));
#55858=CARTESIAN_POINT('Ctrl Pts',(125.759557301321,-34.5231805052529,29.3438787578252));
#55859=CARTESIAN_POINT('Ctrl Pts',(128.074661087812,-31.1914224329392,29.1467993052568));
#55860=CARTESIAN_POINT('Ctrl Pts',(132.129829463554,-31.3022775847555,28.9497198526884));
#55861=CARTESIAN_POINT('Ctrl Pts',(134.260237831562,-34.7542266427015,28.7526404001199));
#55862=CARTESIAN_POINT('Ctrl Pts',(132.540828912276,-38.4284858473968,28.5555609475515));
#55863=CARTESIAN_POINT('Ctrl Pts',(128.525320648812,-39.0044132885975,28.358481494983));
#55864=CARTESIAN_POINT('Ctrl Pts',(125.842450342846,-35.961710573039,28.1614020424146));
#55865=CARTESIAN_POINT('Ctrl Pts',(126.916639805502,-32.0499122497264,27.9643225898461));
#55866=CARTESIAN_POINT('Ctrl Pts',(130.77718055129,-30.8040396619014,27.7672431372777));
#55867=CARTESIAN_POINT('Ctrl Pts',(133.935403176266,-33.3499369180767,27.5701636847093));
#55868=CARTESIAN_POINT('Ctrl Pts',(133.537309371604,-37.3869540726307,27.3730842321408));
#55869=CARTESIAN_POINT('Ctrl Pts',(129.942644867347,-39.2669443427457,27.1760047795724));
#55870=CARTESIAN_POINT('Ctrl Pts',(126.399810770048,-37.2910135029307,26.9789253270039));
#55871=CARTESIAN_POINT('Ctrl Pts',(126.110369858646,-33.2447556651743,26.7818458744355));
#55872=CARTESIAN_POINT('Ctrl Pts',(129.335882119334,-30.7846646188652,26.584766421867));
#55873=CARTESIAN_POINT('Ctrl Pts',(133.161539660835,-32.1338576240479,26.3876869692986));
#55874=CARTESIAN_POINT('Ctrl Pts',(134.130199665,-36.0731057028338,26.1906075167301));
#55875=CARTESIAN_POINT('Ctrl Pts',(131.366510378016,-39.0426172799742,25.9935280641617));
#55876=CARTESIAN_POINT('Ctrl Pts',(127.367942769692,-38.3589254006293,25.7964486115933));
#55877=CARTESIAN_POINT('Ctrl Pts',(125.747893809902,-34.6398638395882,25.5993691590248));
#55878=CARTESIAN_POINT('Ctrl Pts',(127.970357754733,-31.2462475496142,25.4022897064564));
#55879=CARTESIAN_POINT('Ctrl Pts',(132.026954284439,-31.2447954204569,25.2052102538879));
#55880=CARTESIAN_POINT('Ctrl Pts',(134.251847266385,-34.6368197031509,25.0081308013195));
#55881=CARTESIAN_POINT('Ctrl Pts',(132.634461326385,-38.3570401582626,24.8110513487511));
#55882=CARTESIAN_POINT('Ctrl Pts',(128.636384220719,-39.0435945779991,24.6139718961826));
#55883=CARTESIAN_POINT('Ctrl Pts',(125.870569667775,-36.0760623754797,24.4168924436142));
#55884=CARTESIAN_POINT('Ctrl Pts',(126.836409177391,-32.1361218231724,24.2198129910457));
#55885=CARTESIAN_POINT('Ctrl Pts',(130.661099810687,-30.7841902148048,24.0227335384773));
#55886=CARTESIAN_POINT('Ctrl Pts',(133.888372496271,-33.241971435139,23.8256540859088));
#55887=CARTESIAN_POINT('Ctrl Pts',(133.601828540075,-37.2884353328256,23.6285746333404));
#55888=CARTESIAN_POINT('Ctrl Pts',(130.060409934631,-39.2669023593734,23.431495180772));
#55889=CARTESIAN_POINT('Ctrl Pts',(126.464400511604,-37.3894855852837,23.2344157282035));
#55890=CARTESIAN_POINT('Ctrl Pts',(126.063416342178,-33.3527555707813,23.0373362756351));
#55891=CARTESIAN_POINT('Ctrl Pts',(129.21981593212,-30.8045956184337,22.8402568230666));
#55892=CARTESIAN_POINT('Ctrl Pts',(133.081246679441,-32.0477086856073,22.6431773704982));
#55893=CARTESIAN_POINT('Ctrl Pts',(134.158238469326,-35.958727248408,22.4460979179297));
#55894=CARTESIAN_POINT('Ctrl Pts',(131.477543065397,-39.0033700296909,22.2490184653613));
#55895=CARTESIAN_POINT('Ctrl Pts',(127.46163211381,-38.4302760207844,22.0519390127928));
#55896=CARTESIAN_POINT('Ctrl Pts',(125.739575295267,-34.7573347161559,21.8548595602244));
#55897=CARTESIAN_POINT('Ctrl Pts',(127.86754859679,-31.3036834391011,21.657780107656));
#55898=CARTESIAN_POINT('Ctrl Pts',(131.922560327698,-31.1902930704699,21.4607006550875));
#55899=CARTESIAN_POINT('Ctrl Pts',(134.240206494958,-34.5196314060906,21.2636212025191));
#55900=CARTESIAN_POINT('Ctrl Pts',(132.726093189031,-38.2830657982036,21.0665417499506));
#55901=CARTESIAN_POINT('Ctrl Pts',(128.748483491969,-39.079682771454,20.8694622973822));
#55902=CARTESIAN_POINT('Ctrl Pts',(125.901835278662,-36.1896012100724,20.6723828448137));
#55903=CARTESIAN_POINT('Ctrl Pts',(126.758587247308,-32.2245093203287,20.4753033922453));
#55904=CARTESIAN_POINT('Ctrl Pts',(130.544515898538,-30.7675530279628,20.2782239396769));
#55905=CARTESIAN_POINT('Ctrl Pts',(133.838380330569,-33.1353440667567,20.0811444871084));
#55906=CARTESIAN_POINT('Ctrl Pts',(133.66360465708,-37.1881741883823,19.88406503454));
#55907=CARTESIAN_POINT('Ctrl Pts',(130.178128989507,-39.2636104065015,19.6869855819715));
#55908=CARTESIAN_POINT('Ctrl Pts',(126.531682877863,-37.4861383058019,19.4899061294031));
#55909=CARTESIAN_POINT('Ctrl Pts',(126.019461006351,-33.4620092152014,19.2928266768347));
#55910=CARTESIAN_POINT('Ctrl Pts',(129.104343653605,-30.8277233460182,19.0957472242662));
#55911=CARTESIAN_POINT('Ctrl Pts',(132.998607622283,-31.9638049879963,18.8986677716978));
#55912=CARTESIAN_POINT('Ctrl Pts',(134.183109233691,-35.8436252230749,18.7015883191293));
#55913=CARTESIAN_POINT('Ctrl Pts',(131.587452903254,-38.9610602437561,18.5045088665609));
#55914=CARTESIAN_POINT('Ctrl Pts',(127.557249621093,-38.4990423480732,18.3074294139925));
#55915=CARTESIAN_POINT('Ctrl Pts',(125.734511873928,-34.8749321345075,18.110349961424));
#55916=CARTESIAN_POINT('Ctrl Pts',(127.766341966037,-31.3640549521016,17.9132705088556));
#55917=CARTESIAN_POINT('Ctrl Pts',(131.816746705461,-31.138442746857,17.7161910562871));
#55918=CARTESIAN_POINT('Ctrl Pts',(134.225244382692,-34.4033250316298,17.5191116037187));
#55919=CARTESIAN_POINT('Ctrl Pts',(132.815840284911,-38.2055240818087,17.3220321511502));
#55920=CARTESIAN_POINT('Ctrl Pts',(128.861156828271,-39.11489181859,17.1249526985818));
#55921=CARTESIAN_POINT('Ctrl Pts',(125.937164902537,-36.2977053768346,16.9278732460134));
#55922=CARTESIAN_POINT('Ctrl Pts',(126.435512304549,-33.651873438753,16.7964869443011));
#55923=CARTESIAN_POINT('Ctrl Pts',(127.187362670894,-32.7231130507938,16.7307937934449));
#55924=CARTESIAN_POINT('Ctrl Pts',(132.923729479057,-32.4893252232149,30.2680525355392));
#55925=CARTESIAN_POINT('Ctrl Pts',(133.753431720963,-33.4554204947541,30.2023127076135));
#55926=CARTESIAN_POINT('Ctrl Pts',(134.364858284588,-36.2582273907838,30.0708797288316));
#55927=CARTESIAN_POINT('Ctrl Pts',(131.336394091043,-39.3460979785953,29.8737535991936));
#55928=CARTESIAN_POINT('Ctrl Pts',(127.09909170999,-38.497276498852,29.6766741466252));
#55929=CARTESIAN_POINT('Ctrl Pts',(125.484104272656,-34.4922070000582,29.4795946940567));
#55930=CARTESIAN_POINT('Ctrl Pts',(127.949593854918,-30.9440227390151,29.2825152414883));
#55931=CARTESIAN_POINT('Ctrl Pts',(132.268180107098,-31.0620788812659,29.0854357889198));
#55932=CARTESIAN_POINT('Ctrl Pts',(134.536976723449,-34.7382615606466,28.8883563363514));
#55933=CARTESIAN_POINT('Ctrl Pts',(132.70587748596,-38.6511953325875,28.691276883783));
#55934=CARTESIAN_POINT('Ctrl Pts',(128.429527609628,-39.2645341879362,28.4941974312145));
#55935=CARTESIAN_POINT('Ctrl Pts',(125.572381926345,-36.0241819018289,28.2971179786461));
#55936=CARTESIAN_POINT('Ctrl Pts',(126.716349183886,-31.858278813459,28.1000385260776));
#55937=CARTESIAN_POINT('Ctrl Pts',(130.827665076582,-30.5314761430851,27.9029590735092));
#55938=CARTESIAN_POINT('Ctrl Pts',(134.191041278453,-33.2427512052388,27.7058796209408));
#55939=CARTESIAN_POINT('Ctrl Pts',(133.767087875637,-37.5420071591392,27.5088001683723));
#55940=CARTESIAN_POINT('Ctrl Pts',(129.93891916083,-39.5441188799051,27.3117207158039));
#55941=CARTESIAN_POINT('Ctrl Pts',(126.165947681302,-37.4398344287019,27.1146412632354));
#55942=CARTESIAN_POINT('Ctrl Pts',(125.857705106647,-33.1307375301746,26.917561810667));
#55943=CARTESIAN_POINT('Ctrl Pts',(129.292741981707,-30.5108425252575,26.7204823580985));
#55944=CARTESIAN_POINT('Ctrl Pts',(133.366908707584,-31.9476771579637,26.5234029055301));
#55945=CARTESIAN_POINT('Ctrl Pts',(134.398491465541,-36.142813098247,26.3263234529617));
#55946=CARTESIAN_POINT('Ctrl Pts',(131.455276917049,-39.3052198553734,26.1292440003932));
#55947=CARTESIAN_POINT('Ctrl Pts',(127.196968136327,-38.5771163397391,25.9321645478248));
#55948=CARTESIAN_POINT('Ctrl Pts',(125.471683137692,-34.6164699151406,25.7350850952563));
#55949=CARTESIAN_POINT('Ctrl Pts',(127.83851512808,-31.0024092160264,25.5380056426879));
#55950=CARTESIAN_POINT('Ctrl Pts',(132.158622305042,-31.0008627586579,25.3409261901194));
#55951=CARTESIAN_POINT('Ctrl Pts',(134.528041119285,-34.6132280360003,25.143846737551));
#55952=CARTESIAN_POINT('Ctrl Pts',(132.805592126357,-38.5751086347531,24.9467672849826));
#55953=CARTESIAN_POINT('Ctrl Pts',(128.547805710636,-39.3062606372654,24.7496878324141));
#55954=CARTESIAN_POINT('Ctrl Pts',(125.602327841979,-36.1459618320745,24.5526083798457));
#55955=CARTESIAN_POINT('Ctrl Pts',(126.630906890138,-31.9500884361906,24.3555289272772));
#55956=CARTESIAN_POINT('Ctrl Pts',(130.704043898852,-30.510337304595,24.1584494747088));
#55957=CARTESIAN_POINT('Ctrl Pts',(134.140955553463,-33.1277724405804,23.9613700221403));
#55958=CARTESIAN_POINT('Ctrl Pts',(133.835798116036,-37.4370887843932,23.7642905695719));
#55959=CARTESIAN_POINT('Ctrl Pts',(130.064334076669,-39.5440741693538,23.5672111170034));
#55960=CARTESIAN_POINT('Ctrl Pts',(126.234733079114,-37.5447031151951,23.370131664435));
#55961=CARTESIAN_POINT('Ctrl Pts',(125.807701557615,-33.2457529535492,23.1730522118666));
#55962=CARTESIAN_POINT('Ctrl Pts',(129.169136302732,-30.5320682137501,22.9759727592981));
#55963=CARTESIAN_POINT('Ctrl Pts',(133.281400010173,-31.8559321089998,22.7788933067297));
#55964=CARTESIAN_POINT('Ctrl Pts',(134.428351630069,-36.0210047847419,22.5818138541613));
#55965=CARTESIAN_POINT('Ctrl Pts',(131.573522127316,-39.2634231604387,22.3847344015928));
#55966=CARTESIAN_POINT('Ctrl Pts',(127.296743404824,-38.6531017930509,22.1876549490244));
#55967=CARTESIAN_POINT('Ctrl Pts',(125.462824264368,-34.7415715300603,21.9905754964559));
#55968=CARTESIAN_POINT('Ctrl Pts',(127.729027635835,-31.0635760578779,21.7934960438875));
#55969=CARTESIAN_POINT('Ctrl Pts',(132.047447067761,-30.9428200147922,21.596416591319));
#55970=CARTESIAN_POINT('Ctrl Pts',(134.515644180173,-34.4884273565441,21.3993371387506));
#55971=CARTESIAN_POINT('Ctrl Pts',(132.903176262356,-38.4963290071856,21.2022576861821));
#55972=CARTESIAN_POINT('Ctrl Pts',(128.667186788521,-39.3446930676061,21.0051782336137));
#55973=CARTESIAN_POINT('Ctrl Pts',(125.635624421759,-36.2668759852559,20.8080987810452));
#55974=CARTESIAN_POINT('Ctrl Pts',(126.548029759958,-32.044217457409,20.6110193284768));
#55975=CARTESIAN_POINT('Ctrl Pts',(130.579886864277,-30.4926193901429,20.4139398759084));
#55976=CARTESIAN_POINT('Ctrl Pts',(134.087715968934,-33.0142187124648,20.2168604233399));
#55977=CARTESIAN_POINT('Ctrl Pts',(133.901587120311,-37.3303148209218,20.0197809707715));
#55978=CARTESIAN_POINT('Ctrl Pts',(130.189699991202,-39.5405683759814,19.822701518203));
#55979=CARTESIAN_POINT('Ctrl Pts',(126.306386010636,-37.6476342567385,19.6256220656346));
#55980=CARTESIAN_POINT('Ctrl Pts',(125.760890946705,-33.362103556798,19.4285426130662));
#55981=CARTESIAN_POINT('Ctrl Pts',(129.046163111905,-30.5566982850902,19.2314631604977));
#55982=CARTESIAN_POINT('Ctrl Pts',(133.193392839307,-31.7665781484643,19.0343837079293));
#55983=CARTESIAN_POINT('Ctrl Pts',(134.45483796334,-35.898425898209,18.8373042553608));
#55984=CARTESIAN_POINT('Ctrl Pts',(131.690571549381,-39.2183649919633,18.6402248027924));
#55985=CARTESIAN_POINT('Ctrl Pts',(127.398572087175,-38.726335081567,18.443145350224));
#55986=CARTESIAN_POINT('Ctrl Pts',(125.4574319305,-34.8668079067353,18.2460658976555));
#55987=CARTESIAN_POINT('Ctrl Pts',(127.62124676863,-31.1278692171032,18.0489864450871));
#55988=CARTESIAN_POINT('Ctrl Pts',(131.934759945563,-30.8876015691007,17.8519069925186));
#55989=CARTESIAN_POINT('Ctrl Pts',(134.499710150719,-34.364565888105,17.6548275399502));
#55990=CARTESIAN_POINT('Ctrl Pts',(132.998753199867,-38.4137502929707,17.4577480873817));
#55991=CARTESIAN_POINT('Ctrl Pts',(128.787179221893,-39.3821892435537,17.2606686348133));
#55992=CARTESIAN_POINT('Ctrl Pts',(125.673249006936,-36.3820024424398,17.0635891822449));
#55993=CARTESIAN_POINT('Ctrl Pts',(126.203968335883,-33.5643010858862,16.9322028805325));
#55994=CARTESIAN_POINT('Ctrl Pts',(127.004657815318,-32.5752097655344,16.8665097296764));
#55995=CARTESIAN_POINT('Ctrl Pts',(133.102066223001,-32.3361832967811,30.4037684717707));
#55996=CARTESIAN_POINT('Ctrl Pts',(133.98237724979,-33.3612068263209,30.338028643845));
#55997=CARTESIAN_POINT('Ctrl Pts',(134.631098584803,-36.3349746335164,30.2065956650631));
#55998=CARTESIAN_POINT('Ctrl Pts',(131.417909214973,-39.61119396915,30.0094695354251));
#55999=CARTESIAN_POINT('Ctrl Pts',(126.922146974635,-38.7105975013405,29.8123900828567));
#56000=CARTESIAN_POINT('Ctrl Pts',(125.20865124399,-34.4612334948636,29.6153106302882));
#56001=CARTESIAN_POINT('Ctrl Pts',(127.824526622024,-30.696623045091,29.4182311777198));
#56002=CARTESIAN_POINT('Ctrl Pts',(132.406530750643,-30.8218801777763,29.2211517251513));
#56003=CARTESIAN_POINT('Ctrl Pts',(134.813715615336,-34.7222964785918,29.0240722725829));
#56004=CARTESIAN_POINT('Ctrl Pts',(132.870926059646,-38.8739048177783,28.8269928200145));
#56005=CARTESIAN_POINT('Ctrl Pts',(128.333734570443,-39.5246550872747,28.629913367446));
#56006=CARTESIAN_POINT('Ctrl Pts',(125.302313509846,-36.0866532306186,28.4328339148776));
#56007=CARTESIAN_POINT('Ctrl Pts',(126.516058562272,-31.6666453771916,28.2357544623091));
#56008=CARTESIAN_POINT('Ctrl Pts',(130.878149601875,-30.2589126242688,28.0386750097407));
#56009=CARTESIAN_POINT('Ctrl Pts',(134.446679380639,-33.1355654924012,27.8415955571722));
#56010=CARTESIAN_POINT('Ctrl Pts',(133.996866379668,-37.6970602456476,27.6445161046038));
#56011=CARTESIAN_POINT('Ctrl Pts',(129.935193454313,-39.8212934170647,27.4474366520353));
#56012=CARTESIAN_POINT('Ctrl Pts',(125.932084592557,-37.5886553544729,27.2503571994669));
#56013=CARTESIAN_POINT('Ctrl Pts',(125.605040354648,-33.0167193951749,27.0532777468985));
#56014=CARTESIAN_POINT('Ctrl Pts',(129.24960184408,-30.2370204316497,26.85619829433));
#56015=CARTESIAN_POINT('Ctrl Pts',(133.572277754333,-31.7614966918794,26.6591188417616));
#56016=CARTESIAN_POINT('Ctrl Pts',(134.666783266082,-36.2125204936603,26.4620393891931));
#56017=CARTESIAN_POINT('Ctrl Pts',(131.544043456082,-39.5678224307725,26.2649599366247));
#56018=CARTESIAN_POINT('Ctrl Pts',(127.025993502963,-38.7953072788489,26.0678804840562));
#56019=CARTESIAN_POINT('Ctrl Pts',(125.195472465481,-34.5930759906928,25.8708010314878));
#56020=CARTESIAN_POINT('Ctrl Pts',(127.706672501426,-30.7585708824386,25.6737215789194));
#56021=CARTESIAN_POINT('Ctrl Pts',(132.290290325646,-30.7569300968589,25.4766421263509));
#56022=CARTESIAN_POINT('Ctrl Pts',(134.804234972186,-34.5896363688495,25.2795626737825));
#56023=CARTESIAN_POINT('Ctrl Pts',(132.976722926327,-38.7931771112437,25.0824832212141));
#56024=CARTESIAN_POINT('Ctrl Pts',(128.459227200554,-39.5689266965317,24.8854037686456));
#56025=CARTESIAN_POINT('Ctrl Pts',(125.334086016183,-36.2158612886693,24.6883243160772));
#56026=CARTESIAN_POINT('Ctrl Pts',(126.425404602883,-31.7640550492089,24.4912448635087));
#56027=CARTESIAN_POINT('Ctrl Pts',(130.746987987015,-30.2364843943852,24.2941654109403));
#56028=CARTESIAN_POINT('Ctrl Pts',(134.393538610655,-33.013573446022,24.0970859583718));
#56029=CARTESIAN_POINT('Ctrl Pts',(134.069767691998,-37.5857422359606,23.9000065058034));
#56030=CARTESIAN_POINT('Ctrl Pts',(130.068258218707,-39.8212459793342,23.702927053235));
#56031=CARTESIAN_POINT('Ctrl Pts',(126.005065646623,-37.6999206451065,23.5058476006665));
#56032=CARTESIAN_POINT('Ctrl Pts',(125.551986773052,-33.1387503363173,23.308768148098));
#56033=CARTESIAN_POINT('Ctrl Pts',(129.118456673342,-30.2595408090666,23.1116886955297));
#56034=CARTESIAN_POINT('Ctrl Pts',(133.481553340905,-31.6641555323922,22.9146092429611));
#56035=CARTESIAN_POINT('Ctrl Pts',(134.698464790813,-36.0832823210757,22.7175297903928));
#56036=CARTESIAN_POINT('Ctrl Pts',(131.669501189237,-39.5234762911866,22.5204503378243));
#56037=CARTESIAN_POINT('Ctrl Pts',(127.131854695836,-38.8759275653174,22.3233708852559));
#56038=CARTESIAN_POINT('Ctrl Pts',(125.186073233471,-34.7258083439647,22.1262914326874));
#56039=CARTESIAN_POINT('Ctrl Pts',(127.590506674879,-30.8234686766545,21.929211980119));
#56040=CARTESIAN_POINT('Ctrl Pts',(132.172333807822,-30.6953469591144,21.7321325275505));
#56041=CARTESIAN_POINT('Ctrl Pts',(134.791081865386,-34.4572233069978,21.5350530749821));
#56042=CARTESIAN_POINT('Ctrl Pts',(133.080259335682,-38.7095922161676,21.3379736224136));
#56043=CARTESIAN_POINT('Ctrl Pts',(128.585890085073,-39.6097033637582,21.1408941698452));
#56044=CARTESIAN_POINT('Ctrl Pts',(125.369413564855,-36.3441507604394,20.9438147172767));
#56045=CARTESIAN_POINT('Ctrl Pts',(126.337472272608,-31.8639255944892,20.7467352647083));
#56046=CARTESIAN_POINT('Ctrl Pts',(130.615257830015,-30.2176857523228,20.5496558121399));
#56047=CARTESIAN_POINT('Ctrl Pts',(134.337051607298,-32.893093358173,20.3525763595714));
#56048=CARTESIAN_POINT('Ctrl Pts',(134.139569583543,-37.4724554534615,20.155496907003));
#56049=CARTESIAN_POINT('Ctrl Pts',(130.201270992896,-39.8175263454613,19.9584174544345));
#56050=CARTESIAN_POINT('Ctrl Pts',(126.08108914341,-37.8091302076751,19.7613380018661));
#56051=CARTESIAN_POINT('Ctrl Pts',(125.502320887058,-33.2621978983947,19.5642585492976));
#56052=CARTESIAN_POINT('Ctrl Pts',(128.987982570204,-30.2856732241622,19.3671790967292));
#56053=CARTESIAN_POINT('Ctrl Pts',(133.388178056331,-31.5693513089325,19.1700996441607));
#56054=CARTESIAN_POINT('Ctrl Pts',(134.726566692989,-35.953226573343,18.9730201915924));
#56055=CARTESIAN_POINT('Ctrl Pts',(131.793690195508,-39.4756697401704,18.7759407390239));
#56056=CARTESIAN_POINT('Ctrl Pts',(127.239894553259,-38.9536278150609,18.5788612864555));
#56057=CARTESIAN_POINT('Ctrl Pts',(125.18035198707,-34.8586836789633,18.381781833887));
#56058=CARTESIAN_POINT('Ctrl Pts',(127.476151571223,-30.8916834821048,18.1847023813186));
#56059=CARTESIAN_POINT('Ctrl Pts',(132.052773185665,-30.6367603913443,17.9876229287501));
#56060=CARTESIAN_POINT('Ctrl Pts',(134.774175918744,-34.3258067445803,17.7905434761817));
#56061=CARTESIAN_POINT('Ctrl Pts',(133.181666114823,-38.6219765041328,17.5934640236132));
#56062=CARTESIAN_POINT('Ctrl Pts',(128.713201615517,-39.6494866685174,17.3963845710448));
#56063=CARTESIAN_POINT('Ctrl Pts',(125.409333111335,-36.4662995080448,17.1993051184764));
#56064=CARTESIAN_POINT('Ctrl Pts',(125.972424367217,-33.4767287330193,17.067918816764));
#56065=CARTESIAN_POINT('Ctrl Pts',(126.821952959743,-32.4273064802751,17.0022256659079));
#56066=CARTESIAN_POINT('Ctrl Pts',(132.573234427015,-32.7934484719078,30.));
#56067=CARTESIAN_POINT('Ctrl Pts',(132.649853057503,-32.8663667566396,29.9999999999999));
#56068=CARTESIAN_POINT('Ctrl Pts',(132.722535071741,-32.9429224736587,29.9999999999998));
#56069=CARTESIAN_POINT('Ctrl Pts',(132.791284600853,-33.022699725554,29.9999999999998));
#56070=CARTESIAN_POINT('Ctrl Pts',(132.861753079838,-33.1044716543404,29.9999999999998));
#56071=CARTESIAN_POINT('Ctrl Pts',(132.928090363081,-33.1896286377168,30.));
#56072=CARTESIAN_POINT('Ctrl Pts',(132.990274682848,-33.2777711046078,30.));
#56073=CARTESIAN_POINT('Ctrl Pts',(133.054246634771,-33.3684474306573,30.));
#56074=CARTESIAN_POINT('Ctrl Pts',(133.113823916719,-33.462283857259,30.));
#56075=CARTESIAN_POINT('Ctrl Pts',(133.168948488249,-33.5588888786663,30.));
#56076=CARTESIAN_POINT('Ctrl Pts',(133.221605685532,-33.651169862074,30.));
#56077=CARTESIAN_POINT('Ctrl Pts',(133.270199903795,-33.7459780039061,30.));
#56078=CARTESIAN_POINT('Ctrl Pts',(133.314646378775,-33.8430003949785,30.));
#56079=CARTESIAN_POINT('Ctrl Pts',(133.321660120829,-33.8583107210449,30.));
#56080=CARTESIAN_POINT('Ctrl Pts',(133.328571263663,-33.8736779522171,29.9999999999999));
#56081=CARTESIAN_POINT('Ctrl Pts',(133.335376993632,-33.8890954660849,29.9999999999999));
#56082=CARTESIAN_POINT('Ctrl Pts',(133.381245007221,-33.9930036050855,30.));
#56083=CARTESIAN_POINT('Ctrl Pts',(133.422184804746,-34.0988655926642,30.));
#56084=CARTESIAN_POINT('Ctrl Pts',(133.458173581916,-34.2062509409393,30.));
#56085=CARTESIAN_POINT('Ctrl Pts',(133.494910039186,-34.3158672593755,30.));
#56086=CARTESIAN_POINT('Ctrl Pts',(133.52648809981,-34.4270715662737,30.));
#56087=CARTESIAN_POINT('Ctrl Pts',(133.552844216446,-34.5394441670278,30.));
#56088=CARTESIAN_POINT('Ctrl Pts',(133.57918140631,-34.651736071123,30.));
#56089=CARTESIAN_POINT('Ctrl Pts',(133.600304510595,-34.7651954321151,30.0000000000001));
#56090=CARTESIAN_POINT('Ctrl Pts',(133.616105145657,-34.8794295532343,30.));
#56091=CARTESIAN_POINT('Ctrl Pts',(133.629438458493,-34.9758256327184,29.9999999999999));
#56092=CARTESIAN_POINT('Ctrl Pts',(133.638981116824,-35.0727741182234,30.0000000000001));
#56093=CARTESIAN_POINT('Ctrl Pts',(133.644640126762,-35.1700467953132,30.));
#56094=CARTESIAN_POINT('Ctrl Pts',(133.645721269348,-35.1886305466821,30.));
#56095=CARTESIAN_POINT('Ctrl Pts',(133.646660581927,-35.207226141285,30.0000000000001));
#56096=CARTESIAN_POINT('Ctrl Pts',(133.647457301671,-35.2258319984673,30.0000000000001));
#56097=CARTESIAN_POINT('Ctrl Pts',(133.648146506942,-35.2419270619067,30.0000000000002));
#56098=CARTESIAN_POINT('Ctrl Pts',(133.64872875084,-35.2580246317189,30.0000000000001));
#56099=CARTESIAN_POINT('Ctrl Pts',(133.649203597933,-35.2741159296301,30.0000000000001));
#56100=CARTESIAN_POINT('Ctrl Pts',(133.652701975148,-35.3926665764815,30.0000000000001));
#56101=CARTESIAN_POINT('Ctrl Pts',(133.650380391952,-35.5110020020146,29.9999999999999));
#56102=CARTESIAN_POINT('Ctrl Pts',(133.642173844882,-35.6286939927366,29.9999999999999));
#56103=CARTESIAN_POINT('Ctrl Pts',(133.633997658714,-35.7459505707316,29.9999999999999));
#56104=CARTESIAN_POINT('Ctrl Pts',(133.619980289647,-35.8625693524084,30.));
#56105=CARTESIAN_POINT('Ctrl Pts',(133.600009193167,-35.9781441488548,29.9999999999999));
#56106=CARTESIAN_POINT('Ctrl Pts',(133.59650213025,-35.9984398839037,29.9999999999998));
#56107=CARTESIAN_POINT('Ctrl Pts',(133.592811339928,-36.0187034486169,30.0000000000002));
#56108=CARTESIAN_POINT('Ctrl Pts',(133.588936046823,-36.038932666806,30.0000000000002));
#56109=CARTESIAN_POINT('Ctrl Pts',(133.567332076941,-36.1517064386639,30.0000000000001));
#56110=CARTESIAN_POINT('Ctrl Pts',(133.539998383114,-36.2634130820552,30.0000000000001));
#56111=CARTESIAN_POINT('Ctrl Pts',(133.507233683019,-36.3737930037498,30.0000000000001));
#56112=CARTESIAN_POINT('Ctrl Pts',(133.486428152307,-36.4438840726162,30.0000000000002));
#56113=CARTESIAN_POINT('Ctrl Pts',(133.463431616385,-36.5134401519788,30.));
#56114=CARTESIAN_POINT('Ctrl Pts',(133.438309961509,-36.5823930508116,29.9999999999999));
#56115=CARTESIAN_POINT('Ctrl Pts',(133.432144353763,-36.5993161607454,29.9999999999998));
#56116=CARTESIAN_POINT('Ctrl Pts',(133.425850700818,-36.6162029277894,29.9999999999999));
#56117=CARTESIAN_POINT('Ctrl Pts',(133.419429906065,-36.6330523228395,29.9999999999999));
#56118=CARTESIAN_POINT('Ctrl Pts',(133.413621254329,-36.6482953373861,29.9999999999998));
#56119=CARTESIAN_POINT('Ctrl Pts',(133.407710252341,-36.6635031939445,30.0000000000001));
#56120=CARTESIAN_POINT('Ctrl Pts',(133.401700786121,-36.6786677684889,30.0000000000001));
#56121=CARTESIAN_POINT('Ctrl Pts',(133.358822804144,-36.786868119445,30.));
#56122=CARTESIAN_POINT('Ctrl Pts',(133.310892795036,-36.8929797564497,30.));
#56123=CARTESIAN_POINT('Ctrl Pts',(133.258267581598,-36.9967501880808,29.9999999999999));
#56124=CARTESIAN_POINT('Ctrl Pts',(133.2037780914,-37.1041967435974,29.9999999999999));
#56125=CARTESIAN_POINT('Ctrl Pts',(133.14425472734,-37.2091339535983,30.0000000000001));
#56126=CARTESIAN_POINT('Ctrl Pts',(133.080037568562,-37.3112779782923,30.0000000000001));
#56127=CARTESIAN_POINT('Ctrl Pts',(133.015111946839,-37.4145488864843,30.0000000000001));
#56128=CARTESIAN_POINT('Ctrl Pts',(132.945388009163,-37.5149653945738,30.0000000000001));
#56129=CARTESIAN_POINT('Ctrl Pts',(132.87116509564,-37.6122196498687,30.));
#56130=CARTESIAN_POINT('Ctrl Pts',(132.817181793609,-37.682953949941,30.));
#56131=CARTESIAN_POINT('Ctrl Pts',(132.760817487172,-37.7520152103035,30.0000000000001));
#56132=CARTESIAN_POINT('Ctrl Pts',(132.702172154835,-37.8192767143393,29.9999999999999));
#56133=CARTESIAN_POINT('Ctrl Pts',(132.682391535084,-37.8419635025653,29.9999999999999));
#56134=CARTESIAN_POINT('Ctrl Pts',(132.662351312549,-37.8644454683242,29.9999999999999));
#56135=CARTESIAN_POINT('Ctrl Pts',(132.642055030732,-37.8867175151918,30.));
#56136=CARTESIAN_POINT('Ctrl Pts',(132.629127618235,-37.9009033616246,30.));
#56137=CARTESIAN_POINT('Ctrl Pts',(132.616095858353,-37.9150044443019,29.9999999999998));
#56138=CARTESIAN_POINT('Ctrl Pts',(132.602971661464,-37.9290079434914,29.9999999999998));
#56139=CARTESIAN_POINT('Ctrl Pts',(132.517322557525,-38.0203954141101,29.9999999999999));
#56140=CARTESIAN_POINT('Ctrl Pts',(132.427632644473,-38.1077482657667,29.9999999999999));
#56141=CARTESIAN_POINT('Ctrl Pts',(132.334235165115,-38.1907540095518,29.9999999999999));
#56142=CARTESIAN_POINT('Ctrl Pts',(132.250200410151,-38.2654387589431,29.9999999999998));
#56143=CARTESIAN_POINT('Ctrl Pts',(132.163163235718,-38.3366044655783,30.0000000000001));
#56144=CARTESIAN_POINT('Ctrl Pts',(132.073335782034,-38.4040052793126,30.));
#56145=CARTESIAN_POINT('Ctrl Pts',(132.035647403083,-38.4322842442108,29.9999999999999));
#56146=CARTESIAN_POINT('Ctrl Pts',(131.997467518359,-38.4599002091719,30.));
#56147=CARTESIAN_POINT('Ctrl Pts',(131.958810486488,-38.4868338044422,30.0000000000001));
#56148=CARTESIAN_POINT('Ctrl Pts',(131.94120789347,-38.4990980961665,30.0000000000001));
#56149=CARTESIAN_POINT('Ctrl Pts',(131.923504399256,-38.5112222027607,29.9999999999999));
#56150=CARTESIAN_POINT('Ctrl Pts',(131.905707729789,-38.5231999316637,29.9999999999999));
#56151=CARTESIAN_POINT('Ctrl Pts',(131.800671774011,-38.5938924961189,29.9999999999999));
#56152=CARTESIAN_POINT('Ctrl Pts',(131.692537688031,-38.659393354725,29.9999999999999));
#56153=CARTESIAN_POINT('Ctrl Pts',(131.581620730744,-38.7193732400858,29.9999999999999));
#56154=CARTESIAN_POINT('Ctrl Pts',(131.471353175383,-38.7790019523351,29.9999999999999));
#56155=CARTESIAN_POINT('Ctrl Pts',(131.358334664968,-38.8331748755337,30.));
#56156=CARTESIAN_POINT('Ctrl Pts',(131.242839107679,-38.8815321227036,30.));
#56157=CARTESIAN_POINT('Ctrl Pts',(131.228328557671,-38.8876075966851,30.));
#56158=CARTESIAN_POINT('Ctrl Pts',(131.21377886806,-38.8935912160834,30.));
#56159=CARTESIAN_POINT('Ctrl Pts',(131.199190548796,-38.899482217298,30.));
#56160=CARTESIAN_POINT('Ctrl Pts',(131.153580177004,-38.9179004292087,30.));
#56161=CARTESIAN_POINT('Ctrl Pts',(131.107592245152,-38.935413389631,30.));
#56162=CARTESIAN_POINT('Ctrl Pts',(131.061251415332,-38.9520280711437,30.));
#56163=CARTESIAN_POINT('Ctrl Pts',(128.941097447709,-38.949361204357,29.9977747858503));
#56164=CARTESIAN_POINT('Ctrl Pts',(127.636979705122,-38.599701212612,29.9320816349942));
#56165=CARTESIAN_POINT('Ctrl Pts',(125.424202616686,-36.5120753779567,29.8006953332819));
#56166=CARTESIAN_POINT('Ctrl Pts',(126.226060557691,-31.9948456048335,29.6036158807134));
#56167=CARTESIAN_POINT('Ctrl Pts',(130.445077406051,-30.199627076779,29.406536428145));
#56168=CARTESIAN_POINT('Ctrl Pts',(134.258668325894,-32.7392435465971,29.2094569755765));
#56169=CARTESIAN_POINT('Ctrl Pts',(134.225374578973,-37.3233447428259,29.0123775230081));
#56170=CARTESIAN_POINT('Ctrl Pts',(130.372971341113,-39.8071763851411,28.8152980704396));
#56171=CARTESIAN_POINT('Ctrl Pts',(126.183888210242,-37.9472442087612,28.6182186178712));
#56172=CARTESIAN_POINT('Ctrl Pts',(125.443145605471,-33.4237977850877,28.4211391653028));
#56173=CARTESIAN_POINT('Ctrl Pts',(128.820393714243,-30.3248045440124,28.2240597127343));
#56174=CARTESIAN_POINT('Ctrl Pts',(133.263578832371,-31.4506188224813,28.0269802601659));
#56175=CARTESIAN_POINT('Ctrl Pts',(134.757576278224,-35.7839316709174,27.8299008075974));
#56176=CARTESIAN_POINT('Ctrl Pts',(131.952271604642,-39.4088174824048,27.632821355029));
#56177=CARTESIAN_POINT('Ctrl Pts',(127.382756745135,-39.0495791332309,27.4357419024605));
#56178=CARTESIAN_POINT('Ctrl Pts',(125.178371298366,-35.0308439142191,27.2386624498921));
#56179=CARTESIAN_POINT('Ctrl Pts',(127.33116187244,-30.9842369354514,27.0415829973237));
#56180=CARTESIAN_POINT('Ctrl Pts',(131.895708468177,-30.5665654892088,26.8445035447552));
#56181=CARTESIAN_POINT('Ctrl Pts',(134.747155050647,-34.1552686718858,26.6474240921868));
#56182=CARTESIAN_POINT('Ctrl Pts',(133.308726393028,-38.5073324998802,26.4503446396183));
#56183=CARTESIAN_POINT('Ctrl Pts',(128.880291597111,-39.6899152415161,26.2532651870499));
#56184=CARTESIAN_POINT('Ctrl Pts',(125.463706852098,-36.634348899534,26.0561857344814));
#56185=CARTESIAN_POINT('Ctrl Pts',(126.146447062293,-32.1018658487985,25.859106281913));
#56186=CARTESIAN_POINT('Ctrl Pts',(130.311538417948,-30.1883479294121,25.6620268293445));
#56187=CARTESIAN_POINT('Ctrl Pts',(134.195100967925,-32.6229893359297,25.4649473767761));
#56188=CARTESIAN_POINT('Ctrl Pts',(134.287664683484,-37.2056707337862,25.2678679242077));
#56189=CARTESIAN_POINT('Ctrl Pts',(130.505582250638,-39.7951473820333,25.0707884716392));
#56190=CARTESIAN_POINT('Ctrl Pts',(126.266618865874,-38.0513795460382,24.8737090190708));
#56191=CARTESIAN_POINT('Ctrl Pts',(125.40141063766,-33.5501628702343,24.6766295665024));
#56192=CARTESIAN_POINT('Ctrl Pts',(128.6918227481,-30.3591246402977,24.4795501139339));
#56193=CARTESIAN_POINT('Ctrl Pts',(133.164399119471,-31.3619194567416,24.2824706613655));
#56194=CARTESIAN_POINT('Ctrl Pts',(134.777393931214,-35.6523488733214,24.085391208797));
#56195=CARTESIAN_POINT('Ctrl Pts',(132.073187570514,-39.3532683266752,23.8883117562286));
#56196=CARTESIAN_POINT('Ctrl Pts',(127.49549789673,-39.1202573998797,23.6912323036602));
#56197=CARTESIAN_POINT('Ctrl Pts',(125.18105876756,-35.1638817404141,23.4941528510917));
#56198=CARTESIAN_POINT('Ctrl Pts',(127.221365978803,-31.0594106021052,23.2970733985233));
#56199=CARTESIAN_POINT('Ctrl Pts',(131.772649305235,-30.5159431016996,23.0999939459548));
#56200=CARTESIAN_POINT('Ctrl Pts',(134.72203758824,-34.0245960622412,22.9029144933864));
#56201=CARTESIAN_POINT('Ctrl Pts',(133.404248722819,-38.4146950756628,22.7058350408179));
#56202=CARTESIAN_POINT('Ctrl Pts',(129.010132724007,-39.7190268702816,22.5087555882495));
#56203=CARTESIAN_POINT('Ctrl Pts',(125.51053290411,-36.7589022205524,22.3116761356811));
#56204=CARTESIAN_POINT('Ctrl Pts',(126.067942593805,-32.2093053945169,22.1145966831126));
#56205=CARTESIAN_POINT('Ctrl Pts',(130.178645792201,-30.1815835062547,21.9175172305442));
#56206=CARTESIAN_POINT('Ctrl Pts',(134.127911639003,-32.5081337661877,21.7204377779757));
#56207=CARTESIAN_POINT('Ctrl Pts',(134.346895825177,-37.086515878837,21.5233583254073));
#56208=CARTESIAN_POINT('Ctrl Pts',(130.637708287566,-39.7793702476217,21.3262788728388));
#56209=CARTESIAN_POINT('Ctrl Pts',(126.352241086956,-38.1532375014412,21.1291994202704));
#56210=CARTESIAN_POINT('Ctrl Pts',(125.363154565577,-33.6776096448007,20.932119967702));
#56211=CARTESIAN_POINT('Ctrl Pts',(128.564259358348,-30.3969900486762,20.7350405151335));
#56212=CARTESIAN_POINT('Ctrl Pts',(133.062803979689,-31.2759855490205,20.5379610625651));
#56213=CARTESIAN_POINT('Ctrl Pts',(134.793575818518,-35.520271806098,20.3408816099966));
#56214=CARTESIAN_POINT('Ctrl Pts',(132.192523336302,-39.294402522867,20.1438021574282));
#56215=CARTESIAN_POINT('Ctrl Pts',(127.610147083839,-39.187798363185,19.9467227048597));
#56216=CARTESIAN_POINT('Ctrl Pts',(125.187415948436,-35.2967943807173,19.7496432522913));
#56217=CARTESIAN_POINT('Ctrl Pts',(127.113686487097,-31.1375856971393,19.5525637997228));
#56218=CARTESIAN_POINT('Ctrl Pts',(131.648239873017,-30.4687352753939,19.3554843471544));
#56219=CARTESIAN_POINT('Ctrl Pts',(134.693324263192,-33.8946671216466,19.158404894586));
#56220=CARTESIAN_POINT('Ctrl Pts',(133.49717767076,-38.3194554298236,18.9613254420175));
#56221=CARTESIAN_POINT('Ctrl Pts',(129.140729238591,-39.7445478885119,18.7642459894491));
#56222=CARTESIAN_POINT('Ctrl Pts',(125.560774958467,-36.8821090746942,18.5671665368806));
#56223=CARTESIAN_POINT('Ctrl Pts',(125.992439189035,-32.3188845814651,18.3700870843122));
#56224=CARTESIAN_POINT('Ctrl Pts',(130.045603765049,-30.1784591994005,18.1730076317438));
#56225=CARTESIAN_POINT('Ctrl Pts',(134.057606144223,-32.3952370556287,17.9759281791753));
#56226=CARTESIAN_POINT('Ctrl Pts',(134.40275932918,-36.9656456212823,17.7788487266069));
#56227=CARTESIAN_POINT('Ctrl Pts',(130.769466728782,-39.7602144993633,17.5817692740384));
#56228=CARTESIAN_POINT('Ctrl Pts',(126.440397046927,-38.2521535123727,17.38468982147));
#56229=CARTESIAN_POINT('Ctrl Pts',(125.32893397472,-33.8071813688381,17.1876103689015));
#56230=CARTESIAN_POINT('Ctrl Pts',(128.436718489661,-30.4360408883912,16.9905309163331));
#56231=CARTESIAN_POINT('Ctrl Pts',(132.961968787017,-31.197894221067,16.7934047948872));
#56232=CARTESIAN_POINT('Ctrl Pts',(134.185068371337,-33.9850287565488,16.6619718242975));
#56233=CARTESIAN_POINT('Ctrl Pts',(134.075375726175,-35.3317236383559,16.5962320045639));
#56234=CARTESIAN_POINT('Ctrl Pts',(129.001973251084,-38.7223143098011,30.1334903656045));
#56235=CARTESIAN_POINT('Ctrl Pts',(127.772828616367,-38.3927561044383,30.0677972147483));
#56236=CARTESIAN_POINT('Ctrl Pts',(125.687263028798,-36.4251468846801,29.9364109130361));
#56237=CARTESIAN_POINT('Ctrl Pts',(126.4430225387,-32.1676104996552,29.7393314604676));
#56238=CARTESIAN_POINT('Ctrl Pts',(130.419490117967,-30.4755982297153,29.5422520078992));
#56239=CARTESIAN_POINT('Ctrl Pts',(134.013839512243,-32.8692133583039,29.3451725553307));
#56240=CARTESIAN_POINT('Ctrl Pts',(133.982459806977,-37.189776760171,29.1480931027623));
#56241=CARTESIAN_POINT('Ctrl Pts',(130.351529396359,-39.5308141044197,28.9510136501938));
#56242=CARTESIAN_POINT('Ctrl Pts',(126.403274659419,-37.7778085429733,28.7539341976254));
#56243=CARTESIAN_POINT('Ctrl Pts',(125.705116994181,-33.5144128996771,28.5568547450569));
#56244=CARTESIAN_POINT('Ctrl Pts',(128.888208717764,-30.5935793039794,28.3597752924885));
#56245=CARTESIAN_POINT('Ctrl Pts',(133.075957239742,-31.654671055805,28.1626958399201));
#56246=CARTESIAN_POINT('Ctrl Pts',(134.484065484026,-35.7388638125433,27.9656163873516));
#56247=CARTESIAN_POINT('Ctrl Pts',(131.840036439958,-39.1553566652632,27.7685369347832));
#56248=CARTESIAN_POINT('Ctrl Pts',(127.533220813264,-38.8167707576779,27.5714574822147));
#56249=CARTESIAN_POINT('Ctrl Pts',(125.455564435879,-35.0290707122816,27.3743780296463));
#56250=CARTESIAN_POINT('Ctrl Pts',(127.484592105225,-31.2151012413225,27.1772985770779));
#56251=CARTESIAN_POINT('Ctrl Pts',(131.786725091269,-30.8214415275873,26.9802191245094));
#56252=CARTESIAN_POINT('Ctrl Pts',(134.474243367857,-34.2038318735932,26.783139671941));
#56253=CARTESIAN_POINT('Ctrl Pts',(133.118509288641,-38.3056976250062,26.5860602193725));
#56254=CARTESIAN_POINT('Ctrl Pts',(128.944663099876,-39.42029424809,26.3889807668041));
#56255=CARTESIAN_POINT('Ctrl Pts',(125.724496184533,-36.540390959741,26.1919013142356));
#56256=CARTESIAN_POINT('Ctrl Pts',(126.367985985233,-32.2684782007685,25.9948218616672));
#56257=CARTESIAN_POINT('Ctrl Pts',(130.293628222687,-30.4649675151582,25.7977424090988));
#56258=CARTESIAN_POINT('Ctrl Pts',(133.953926611407,-32.7596425468358,25.6006629565303));
#56259=CARTESIAN_POINT('Ctrl Pts',(134.041168883048,-37.0788677738628,25.4035835039619));
#56260=CARTESIAN_POINT('Ctrl Pts',(130.476516567858,-39.5194766429712,25.2065040513934));
#56261=CARTESIAN_POINT('Ctrl Pts',(126.481249169064,-37.87595718931,25.009424598825));
#56262=CARTESIAN_POINT('Ctrl Pts',(125.665781349791,-33.6335133162664,24.8123451462565));
#56263=CARTESIAN_POINT('Ctrl Pts',(128.767029235226,-30.625926354276,24.6152656936881));
#56264=CARTESIAN_POINT('Ctrl Pts',(132.982479321297,-31.5710709743541,24.4181862411197));
#56265=CARTESIAN_POINT('Ctrl Pts',(134.502743829583,-35.6148456473082,24.2211067885512));
#56266=CARTESIAN_POINT('Ctrl Pts',(131.954001004545,-39.1030010040384,24.0240273359828));
#56267=CARTESIAN_POINT('Ctrl Pts',(127.639480529752,-38.883385764441,23.8269478834143));
#56268=CARTESIAN_POINT('Ctrl Pts',(125.458097403749,-35.1544602572147,23.6298684308459));
#56269=CARTESIAN_POINT('Ctrl Pts',(127.381108325217,-31.2859532096857,23.4327889782775));
#56270=CARTESIAN_POINT('Ctrl Pts',(131.670740540991,-30.7737293970246,23.235709525709));
#56271=CARTESIAN_POINT('Ctrl Pts',(134.450569896401,-34.0806715700376,23.0386300731406));
#56272=CARTESIAN_POINT('Ctrl Pts',(133.208540085189,-38.2183858821837,22.8415506205721));
#56273=CARTESIAN_POINT('Ctrl Pts',(129.06703972223,-39.4477322631838,22.6444711680036));
#56274=CARTESIAN_POINT('Ctrl Pts',(125.768630229117,-36.6577837696589,22.4473917154353));
#56275=CARTESIAN_POINT('Ctrl Pts',(126.293994701247,-32.369741098177,22.2503122628668));
#56276=CARTESIAN_POINT('Ctrl Pts',(130.168375530697,-30.4585919754662,22.0532328102984));
#56277=CARTESIAN_POINT('Ctrl Pts',(133.890599965003,-32.6513899690925,21.8561533577299));
#56278=CARTESIAN_POINT('Ctrl Pts',(134.096994854616,-36.9665630747711,21.6590739051615));
#56279=CARTESIAN_POINT('Ctrl Pts',(130.601046741853,-39.5046065285022,21.461994452593));
#56280=CARTESIAN_POINT('Ctrl Pts',(126.561949009437,-37.9719593793719,21.2649150000246));
#56281=CARTESIAN_POINT('Ctrl Pts',(125.629724601071,-33.753633236466,21.0678355474561));
#56282=CARTESIAN_POINT('Ctrl Pts',(128.646799403992,-30.6616148983622,20.8707560948877));
#56283=CARTESIAN_POINT('Ctrl Pts',(132.886724837712,-31.4900773660575,20.6736766423193));
#56284=CARTESIAN_POINT('Ctrl Pts',(134.517995427894,-35.4903616277712,20.4765971897508));
#56285=CARTESIAN_POINT('Ctrl Pts',(132.066476213998,-39.0475193672533,20.2795177371824));
#56286=CARTESIAN_POINT('Ctrl Pts',(127.747538589701,-38.9470438299358,20.0824382846139));
#56287=CARTESIAN_POINT('Ctrl Pts',(125.464089113325,-35.2797318131331,19.8853588320455));
#56288=CARTESIAN_POINT('Ctrl Pts',(127.279619276201,-31.3596340557411,19.688279379477));
#56289=CARTESIAN_POINT('Ctrl Pts',(131.553483347775,-30.729235526168,19.4911999269086));
#56290=CARTESIAN_POINT('Ctrl Pts',(134.423507286734,-33.9582121823526,19.2941204743402));
#56291=CARTESIAN_POINT('Ctrl Pts',(133.296126592175,-38.1286215182213,19.0970410217717));
#56292=CARTESIAN_POINT('Ctrl Pts',(129.190128305394,-39.4717860902317,18.8999615692033));
#56293=CARTESIAN_POINT('Ctrl Pts',(125.8159838917,-36.7739075204394,18.7028821166348));
#56294=CARTESIAN_POINT('Ctrl Pts',(126.222831951255,-32.4730206298602,18.5058026640664));
#56295=CARTESIAN_POINT('Ctrl Pts',(130.042982026317,-30.455647283525,18.308723211498));
#56296=CARTESIAN_POINT('Ctrl Pts',(133.824336299632,-32.5449836366508,18.1116437589295));
#56297=CARTESIAN_POINT('Ctrl Pts',(134.149646792382,-36.8526415907527,17.9145643063611));
#56298=CARTESIAN_POINT('Ctrl Pts',(130.725230453043,-39.4865520350872,17.7174848537926));
#56299=CARTESIAN_POINT('Ctrl Pts',(126.645036925259,-38.0651887559485,17.5204054012242));
#56300=CARTESIAN_POINT('Ctrl Pts',(125.597471335683,-33.8757559438036,17.3233259486557));
#56301=CARTESIAN_POINT('Ctrl Pts',(128.526590799099,-30.6984207239018,17.1262464960873));
#56302=CARTESIAN_POINT('Ctrl Pts',(132.791686612239,-31.4164754713532,16.9291203746415));
#56303=CARTESIAN_POINT('Ctrl Pts',(133.944470784019,-34.0433789699035,16.7976874040518));
#56304=CARTESIAN_POINT('Ctrl Pts',(133.84108431678,-35.3126530043869,16.7319475843182));
#56305=CARTESIAN_POINT('Ctrl Pts',(129.06284905446,-38.4952674152452,30.2692059453588));
#56306=CARTESIAN_POINT('Ctrl Pts',(127.908677527612,-38.1858109962646,30.2035127945026));
#56307=CARTESIAN_POINT('Ctrl Pts',(125.95032344091,-36.3382183914036,30.0721264927903));
#56308=CARTESIAN_POINT('Ctrl Pts',(126.65998451971,-32.3403753944769,29.8750470402219));
#56309=CARTESIAN_POINT('Ctrl Pts',(130.393902829884,-30.7515693826514,29.6779675876535));
#56310=CARTESIAN_POINT('Ctrl Pts',(133.769010698594,-32.9991831700107,29.480888135085));
#56311=CARTESIAN_POINT('Ctrl Pts',(133.739545034979,-37.0562087775161,29.2838086825166));
#56312=CARTESIAN_POINT('Ctrl Pts',(130.330087451605,-39.2544518236982,29.0867292299481));
#56313=CARTESIAN_POINT('Ctrl Pts',(126.622661108597,-37.6083728771854,28.8896497773797));
#56314=CARTESIAN_POINT('Ctrl Pts',(125.967088382891,-33.6050280142665,28.6925703248112));
#56315=CARTESIAN_POINT('Ctrl Pts',(128.956023721286,-30.8623540639465,28.4954908722428));
#56316=CARTESIAN_POINT('Ctrl Pts',(132.888335647114,-31.8587232891287,28.2984114196744));
#56317=CARTESIAN_POINT('Ctrl Pts',(134.210554689826,-35.6937959541694,28.1013319671059));
#56318=CARTESIAN_POINT('Ctrl Pts',(131.727801275276,-38.9018958481215,27.9042525145375));
#56319=CARTESIAN_POINT('Ctrl Pts',(127.683684881391,-38.5839623821248,27.707173061969));
#56320=CARTESIAN_POINT('Ctrl Pts',(125.732757573393,-35.0272975103442,27.5100936094006));
#56321=CARTESIAN_POINT('Ctrl Pts',(127.638022338009,-31.4459655471936,27.3130141568322));
#56322=CARTESIAN_POINT('Ctrl Pts',(131.67774171436,-31.0763175659658,27.1159347042637));
#56323=CARTESIAN_POINT('Ctrl Pts',(134.201331685068,-34.2523950753005,26.9188552516953));
#56324=CARTESIAN_POINT('Ctrl Pts',(132.928292184253,-38.1040627501321,26.7217757991268));
#56325=CARTESIAN_POINT('Ctrl Pts',(129.00903460264,-39.1506732546641,26.5246963465584));
#56326=CARTESIAN_POINT('Ctrl Pts',(125.985285516968,-36.4464330199479,26.32761689399));
#56327=CARTESIAN_POINT('Ctrl Pts',(126.589524908172,-32.4350905527384,26.1305374414215));
#56328=CARTESIAN_POINT('Ctrl Pts',(130.275718027424,-30.7415871009042,25.9334579888531));
#56329=CARTESIAN_POINT('Ctrl Pts',(133.71275225489,-32.896295757742,25.7363785362846));
#56330=CARTESIAN_POINT('Ctrl Pts',(133.794673082611,-36.9520648139394,25.5392990837162));
#56331=CARTESIAN_POINT('Ctrl Pts',(130.447450885079,-39.2438059039089,25.3422196311477));
#56332=CARTESIAN_POINT('Ctrl Pts',(126.695879472254,-37.7005348325817,25.1451401785793));
#56333=CARTESIAN_POINT('Ctrl Pts',(125.930152061922,-33.7168637622985,24.9480607260108));
#56334=CARTESIAN_POINT('Ctrl Pts',(128.842235722353,-30.8927280682542,24.7509812734424));
#56335=CARTESIAN_POINT('Ctrl Pts',(132.800559523124,-31.7802224919666,24.553901820874));
#56336=CARTESIAN_POINT('Ctrl Pts',(134.228093727952,-35.5773424212951,24.3568223683055));
#56337=CARTESIAN_POINT('Ctrl Pts',(131.834814438577,-38.8527336814015,24.1597429157371));
#56338=CARTESIAN_POINT('Ctrl Pts',(127.783463162773,-38.6465141290025,23.9626634631686));
#56339=CARTESIAN_POINT('Ctrl Pts',(125.735136039938,-35.1450387740152,23.7655840106002));
#56340=CARTESIAN_POINT('Ctrl Pts',(127.540850671631,-31.5124958172661,23.5685045580317));
#56341=CARTESIAN_POINT('Ctrl Pts',(131.568831776746,-31.0315156923496,23.3714251054633));
#56342=CARTESIAN_POINT('Ctrl Pts',(134.179102204562,-34.1367470778341,23.1743456528949));
#56343=CARTESIAN_POINT('Ctrl Pts',(133.01283144756,-38.0220766887047,22.9772662003264));
#56344=CARTESIAN_POINT('Ctrl Pts',(129.123946720453,-39.1764376560859,22.780186747758));
#56345=CARTESIAN_POINT('Ctrl Pts',(126.026727554125,-36.5566653187652,22.5831072951895));
#56346=CARTESIAN_POINT('Ctrl Pts',(126.520046808689,-32.5301768018372,22.3860278426211));
#56347=CARTESIAN_POINT('Ctrl Pts',(130.158105269193,-30.7356004446776,22.1889483900526));
#56348=CARTESIAN_POINT('Ctrl Pts',(133.653288291002,-32.7946461719973,21.9918689374842));
#56349=CARTESIAN_POINT('Ctrl Pts',(133.847093884055,-36.8466102707053,21.7947894849158));
#56350=CARTESIAN_POINT('Ctrl Pts',(130.564385196142,-39.2298428093826,21.5977100323473));
#56351=CARTESIAN_POINT('Ctrl Pts',(126.771656931919,-37.7906812573025,21.4006305797789));
#56352=CARTESIAN_POINT('Ctrl Pts',(125.896294636564,-33.8296568281313,21.2035511272104));
#56353=CARTESIAN_POINT('Ctrl Pts',(128.729339449638,-30.926239748048,21.006471674642));
#56354=CARTESIAN_POINT('Ctrl Pts',(132.710645695734,-31.7041691830945,20.8093922220735));
#56355=CARTESIAN_POINT('Ctrl Pts',(134.24241503727,-35.4604514494443,20.6123127695051));
#56356=CARTESIAN_POINT('Ctrl Pts',(131.940429091694,-38.8006362116395,20.4152333169367));
#56357=CARTESIAN_POINT('Ctrl Pts',(127.884930095563,-38.7062892966865,20.2181538643682));
#56358=CARTESIAN_POINT('Ctrl Pts',(125.740762278213,-35.262669245549,20.0210744117998));
#56359=CARTESIAN_POINT('Ctrl Pts',(127.445552065305,-31.5816824143429,19.8239949592313));
#56360=CARTESIAN_POINT('Ctrl Pts',(131.458726822532,-30.9897357769423,19.6269155066629));
#56361=CARTESIAN_POINT('Ctrl Pts',(134.153690310275,-34.0217572430586,19.4298360540945));
#56362=CARTESIAN_POINT('Ctrl Pts',(133.09507551359,-37.9377876066188,19.232756601526));
#56363=CARTESIAN_POINT('Ctrl Pts',(129.239527372196,-39.1990242919515,19.0356771489576));
#56364=CARTESIAN_POINT('Ctrl Pts',(126.071192824932,-36.6657059661847,18.8385976963891));
#56365=CARTESIAN_POINT('Ctrl Pts',(126.453224713474,-32.6271566782553,18.6415182438207));
#56366=CARTESIAN_POINT('Ctrl Pts',(130.040360287586,-30.7328353676494,18.4444387912522));
#56367=CARTESIAN_POINT('Ctrl Pts',(133.59106645504,-32.694730217673,18.2473593386838));
#56368=CARTESIAN_POINT('Ctrl Pts',(133.896534255584,-36.7396375602231,18.0502798861154));
#56369=CARTESIAN_POINT('Ctrl Pts',(130.680994177302,-39.2128895708112,17.8532004335469));
#56370=CARTESIAN_POINT('Ctrl Pts',(126.849676803589,-37.8782239995245,17.6561209809785));
#56371=CARTESIAN_POINT('Ctrl Pts',(125.866008696645,-33.9443305187691,17.45904152841));
#56372=CARTESIAN_POINT('Ctrl Pts',(128.616463108536,-30.9608005594124,17.2619620758416));
#56373=CARTESIAN_POINT('Ctrl Pts',(132.62140443746,-31.6350567216393,17.0648359543957));
#56374=CARTESIAN_POINT('Ctrl Pts',(133.703873196701,-34.1017291832583,16.933402983806));
#56375=CARTESIAN_POINT('Ctrl Pts',(133.606792907386,-35.293582370418,16.8676631640724));
#56376=CARTESIAN_POINT('Ctrl Pts',(129.123724857835,-38.2682205206892,30.4049215251131));
#56377=CARTESIAN_POINT('Ctrl Pts',(128.044526438856,-37.9788658880908,30.3392283742569));
#56378=CARTESIAN_POINT('Ctrl Pts',(126.213383853024,-36.251289898127,30.2078420725446));
#56379=CARTESIAN_POINT('Ctrl Pts',(126.876946500719,-32.5131402892986,30.0107626199762));
#56380=CARTESIAN_POINT('Ctrl Pts',(130.368315541801,-31.0275405355875,29.8136831674077));
#56381=CARTESIAN_POINT('Ctrl Pts',(133.524181884943,-33.1291529817175,29.6166037148393));
#56382=CARTESIAN_POINT('Ctrl Pts',(133.496630262981,-36.9226407948612,29.4195242622709));
#56383=CARTESIAN_POINT('Ctrl Pts',(130.30864550685,-38.9780895429767,29.2224448097024));
#56384=CARTESIAN_POINT('Ctrl Pts',(126.842047557774,-37.4389372113975,29.025365357134));
#56385=CARTESIAN_POINT('Ctrl Pts',(126.2290597716,-33.6956431288561,28.8282859045656));
#56386=CARTESIAN_POINT('Ctrl Pts',(129.023838724806,-31.1311288239135,28.6312064519971));
#56387=CARTESIAN_POINT('Ctrl Pts',(132.700714054484,-32.0627755224524,28.4341269994287));
#56388=CARTESIAN_POINT('Ctrl Pts',(133.937043895626,-35.6487280957953,28.2370475468602));
#56389=CARTESIAN_POINT('Ctrl Pts',(131.615566110593,-38.6484350309798,28.0399680942918));
#56390=CARTESIAN_POINT('Ctrl Pts',(127.83414894952,-38.3511540065717,27.8428886417233));
#56391=CARTESIAN_POINT('Ctrl Pts',(126.009950710905,-35.0255243084067,27.6458091891549));
#56392=CARTESIAN_POINT('Ctrl Pts',(127.791452570794,-31.6768298530648,27.4487297365864));
#56393=CARTESIAN_POINT('Ctrl Pts',(131.568758337451,-31.3311936043443,27.251650284018));
#56394=CARTESIAN_POINT('Ctrl Pts',(133.928420002278,-34.3009582770079,27.0545708314495));
#56395=CARTESIAN_POINT('Ctrl Pts',(132.738075079866,-37.9024278752581,26.8574913788811));
#56396=CARTESIAN_POINT('Ctrl Pts',(129.073406105405,-38.8810522612381,26.6604119263127));
#56397=CARTESIAN_POINT('Ctrl Pts',(126.246074849402,-36.3524750801548,26.4633324737443));
#56398=CARTESIAN_POINT('Ctrl Pts',(126.811063831112,-32.6017029047084,26.2662530211758));
#56399=CARTESIAN_POINT('Ctrl Pts',(130.257807832163,-31.0182066866501,26.0691735686074));
#56400=CARTESIAN_POINT('Ctrl Pts',(133.471577898372,-33.0329489686482,25.8720941160389));
#56401=CARTESIAN_POINT('Ctrl Pts',(133.548177282174,-36.8252618540159,25.6750146634705));
#56402=CARTESIAN_POINT('Ctrl Pts',(130.418385202298,-38.9681351648467,25.477935210902));
#56403=CARTESIAN_POINT('Ctrl Pts',(126.910509775443,-37.5251124758535,25.2808557583336));
#56404=CARTESIAN_POINT('Ctrl Pts',(126.194522774053,-33.8002142083307,25.0837763057651));
#56405=CARTESIAN_POINT('Ctrl Pts',(128.917442209478,-31.1595297822324,24.8866968531967));
#56406=CARTESIAN_POINT('Ctrl Pts',(132.61863972495,-31.9893740095791,24.6896174006282));
#56407=CARTESIAN_POINT('Ctrl Pts',(133.953443626322,-35.5398391952819,24.4925379480598));
#56408=CARTESIAN_POINT('Ctrl Pts',(131.715627872607,-38.6024663587646,24.2954584954914));
#56409=CARTESIAN_POINT('Ctrl Pts',(127.927445795795,-38.4096424935639,24.0983790429229));
#56410=CARTESIAN_POINT('Ctrl Pts',(126.012174676128,-35.1356172908157,23.9012995903545));
#56411=CARTESIAN_POINT('Ctrl Pts',(127.700593018045,-31.7390384248466,23.704220137786));
#56412=CARTESIAN_POINT('Ctrl Pts',(131.466923012502,-31.2893019876745,23.5071406852176));
#56413=CARTESIAN_POINT('Ctrl Pts',(133.907634512722,-34.1928225856305,23.3100612326491));
#56414=CARTESIAN_POINT('Ctrl Pts',(132.81712280993,-37.8257674952256,23.1129817800807));
#56415=CARTESIAN_POINT('Ctrl Pts',(129.180853718675,-38.9051430489881,22.9159023275123));
#56416=CARTESIAN_POINT('Ctrl Pts',(126.284824879133,-36.4555468678715,22.7188228749439));
#56417=CARTESIAN_POINT('Ctrl Pts',(126.74609891613,-32.6906125054973,22.5217434223754));
#56418=CARTESIAN_POINT('Ctrl Pts',(130.147835007688,-31.012608913889,22.324663969807));
#56419=CARTESIAN_POINT('Ctrl Pts',(133.415976617003,-32.9379023749022,22.1275845172385));
#56420=CARTESIAN_POINT('Ctrl Pts',(133.597192913494,-36.7266574666393,21.9305050646701));
#56421=CARTESIAN_POINT('Ctrl Pts',(130.527723650431,-38.9550790902631,21.7334256121016));
#56422=CARTESIAN_POINT('Ctrl Pts',(126.981364854401,-37.609403135233,21.5363461595332));
#56423=CARTESIAN_POINT('Ctrl Pts',(126.162864672058,-33.9056804197966,21.3392667069647));
#56424=CARTESIAN_POINT('Ctrl Pts',(128.811879495282,-31.1908645977338,21.1421872543962));
#56425=CARTESIAN_POINT('Ctrl Pts',(132.534566553757,-31.9182610001316,20.9451078018278));
#56426=CARTESIAN_POINT('Ctrl Pts',(133.966834646645,-35.4305412711174,20.7480283492594));
#56427=CARTESIAN_POINT('Ctrl Pts',(131.814381969389,-38.5537530560258,20.550948896691));
#56428=CARTESIAN_POINT('Ctrl Pts',(128.022321601425,-38.4655347634374,20.3538694441225));
#56429=CARTESIAN_POINT('Ctrl Pts',(126.017435443101,-35.2456066779649,20.1567899915541));
#56430=CARTESIAN_POINT('Ctrl Pts',(127.61148485441,-31.8037307729446,19.9597105389856));
#56431=CARTESIAN_POINT('Ctrl Pts',(131.36397029729,-31.2502360277164,19.7626310864172));
#56432=CARTESIAN_POINT('Ctrl Pts',(133.883873333817,-34.0853023037645,19.5655516338488));
#56433=CARTESIAN_POINT('Ctrl Pts',(132.894024435006,-37.7469536950163,19.3684721812803));
#56434=CARTESIAN_POINT('Ctrl Pts',(129.288926438999,-38.9262624936712,19.1713927287119));
#56435=CARTESIAN_POINT('Ctrl Pts',(126.326401758165,-36.5575044119299,18.9743132761434));
#56436=CARTESIAN_POINT('Ctrl Pts',(126.683617475693,-32.7812927266503,18.777233823575));
#56437=CARTESIAN_POINT('Ctrl Pts',(130.037738548853,-31.0100234517737,18.5801543710065));
#56438=CARTESIAN_POINT('Ctrl Pts',(133.357796610448,-32.844476798695,18.3830749184381));
#56439=CARTESIAN_POINT('Ctrl Pts',(133.643421718785,-36.6266335296934,18.1859954658697));
#56440=CARTESIAN_POINT('Ctrl Pts',(130.636757901562,-38.9392271065351,17.9889160133012));
#56441=CARTESIAN_POINT('Ctrl Pts',(127.054316681922,-37.6912592431004,17.7918365607328));
#56442=CARTESIAN_POINT('Ctrl Pts',(126.134546057608,-34.0129050937345,17.5947571081642));
#56443=CARTESIAN_POINT('Ctrl Pts',(128.706335417974,-31.223180394923,17.3976776555959));
#56444=CARTESIAN_POINT('Ctrl Pts',(132.451122262682,-31.8536379719255,17.20055153415));
#56445=CARTESIAN_POINT('Ctrl Pts',(133.463275609383,-34.160079396613,17.0691185635602));
#56446=CARTESIAN_POINT('Ctrl Pts',(133.372501497992,-35.274511736449,17.0033787438267));
#56447=CARTESIAN_POINT('',(127.424194268159,-32.7919560716439,30.0017032878335));
#56448=CARTESIAN_POINT('Ctrl Pts',(127.426413829439,-32.7938587340794,30.0017032878335));
#56449=CARTESIAN_POINT('Ctrl Pts',(127.438461137846,-32.7798048805081,30.0011355252223));
#56450=CARTESIAN_POINT('Ctrl Pts',(127.450623566855,-32.7658497111731,30.0005677626112));
#56451=CARTESIAN_POINT('Ctrl Pts',(127.462899484434,-32.7519950986681,30.));
#56452=CARTESIAN_POINT('Ctrl Pts',(128.942095577027,-38.9456385074984,30.));
#56453=CARTESIAN_POINT('Ctrl Pts',(128.82630386935,-38.9038806817832,30.));
#56454=CARTESIAN_POINT('Ctrl Pts',(128.712884526443,-38.8565769348122,30.));
#56455=CARTESIAN_POINT('Ctrl Pts',(128.602063029409,-38.8040859693868,30.));
#56456=CARTESIAN_POINT('Ctrl Pts',(128.48644207688,-38.7493217261301,30.));
#56457=CARTESIAN_POINT('Ctrl Pts',(128.373648076022,-38.6889108098624,29.9999999999999));
#56458=CARTESIAN_POINT('Ctrl Pts',(128.263966932901,-38.6232096796844,29.9999999999999));
#56459=CARTESIAN_POINT('Ctrl Pts',(128.15428578978,-38.5575085495065,29.9999999999999));
#56460=CARTESIAN_POINT('Ctrl Pts',(128.047716901034,-38.4865164045163,30.));
#56461=CARTESIAN_POINT('Ctrl Pts',(127.944585645469,-38.4105498139686,30.));
#56462=CARTESIAN_POINT('Ctrl Pts',(127.85193017975,-38.3422997011609,30.0000000000001));
#56463=CARTESIAN_POINT('Ctrl Pts',(127.762049656311,-38.2700334897146,29.9999999999999));
#56464=CARTESIAN_POINT('Ctrl Pts',(127.675213227679,-38.1939612063097,29.9999999999999));
#56465=CARTESIAN_POINT('Ctrl Pts',(127.658100651142,-38.1789698853557,29.9999999999999));
#56466=CARTESIAN_POINT('Ctrl Pts',(127.641106400836,-38.1638307099299,30.0000000000001));
#56467=CARTESIAN_POINT('Ctrl Pts',(127.624232699747,-38.1485452275119,30.));
#56468=CARTESIAN_POINT('Ctrl Pts',(127.613106149663,-38.1384659517932,30.));
#56469=CARTESIAN_POINT('Ctrl Pts',(127.602033315642,-38.1283241907556,30.0000000000001));
#56470=CARTESIAN_POINT('Ctrl Pts',(127.59102153458,-38.1181267915428,30.0000000000001));
#56471=CARTESIAN_POINT('Ctrl Pts',(127.500544559117,-38.0343410866547,29.9999999999998));
#56472=CARTESIAN_POINT('Ctrl Pts',(127.414055491681,-37.9466844892944,30.0000000000001));
#56473=CARTESIAN_POINT('Ctrl Pts',(127.331810952627,-37.855473172009,30.0000000000001));
#56474=CARTESIAN_POINT('Ctrl Pts',(127.25026281251,-37.7650341791259,30.));
#56475=CARTESIAN_POINT('Ctrl Pts',(127.172887189515,-37.671099663786,29.9999999999999));
#56476=CARTESIAN_POINT('Ctrl Pts',(127.099976041161,-37.5739493940444,30.));
#56477=CARTESIAN_POINT('Ctrl Pts',(127.027475603359,-37.4773463745078,30.0000000000001));
#56478=CARTESIAN_POINT('Ctrl Pts',(126.959389056289,-37.3775630490853,30.0000000000001));
#56479=CARTESIAN_POINT('Ctrl Pts',(126.896051405949,-37.2748568041853,29.9999999999999));
#56480=CARTESIAN_POINT('Ctrl Pts',(126.843495295564,-37.1896335488993,29.9999999999998));
#56481=CARTESIAN_POINT('Ctrl Pts',(126.794209667284,-37.1023972880374,30.0000000000002));
#56482=CARTESIAN_POINT('Ctrl Pts',(126.748414412018,-37.0132907019563,30.0000000000001));
#56483=CARTESIAN_POINT('Ctrl Pts',(126.738572960238,-36.9941415965499,30.0000000000001));
#56484=CARTESIAN_POINT('Ctrl Pts',(126.728892803937,-36.9749061092015,29.9999999999999));
#56485=CARTESIAN_POINT('Ctrl Pts',(126.719376295068,-36.9555856509566,30.));
#56486=CARTESIAN_POINT('Ctrl Pts',(126.712231453978,-36.9410801630899,30.));
#56487=CARTESIAN_POINT('Ctrl Pts',(126.705179730846,-36.9265284390521,30.));
#56488=CARTESIAN_POINT('Ctrl Pts',(126.698226860057,-36.9119414822678,30.));
#56489=CARTESIAN_POINT('Ctrl Pts',(126.647942792783,-36.8064467106005,30.0000000000001));
#56490=CARTESIAN_POINT('Ctrl Pts',(126.602751084607,-36.6989610097156,30.0000000000001));
#56491=CARTESIAN_POINT('Ctrl Pts',(126.562915840835,-36.5897363849447,30.0000000000001));
#56492=CARTESIAN_POINT('Ctrl Pts',(126.523317774394,-36.4811620789004,30.0000000000001));
#56493=CARTESIAN_POINT('Ctrl Pts',(126.489012229666,-36.3708688756739,30.));
#56494=CARTESIAN_POINT('Ctrl Pts',(126.460308487673,-36.2590933458545,29.9999999999999));
#56495=CARTESIAN_POINT('Ctrl Pts',(126.452959393802,-36.2304751656402,29.9999999999998));
#56496=CARTESIAN_POINT('Ctrl Pts',(126.445977784055,-36.2017597851064,29.9999999999999));
#56497=CARTESIAN_POINT('Ctrl Pts',(126.439369421695,-36.1729511329457,29.9999999999999));
#56498=CARTESIAN_POINT('Ctrl Pts',(126.412872256441,-36.0574387600593,29.9999999999999));
#56499=CARTESIAN_POINT('Ctrl Pts',(126.392371897484,-35.9404260397136,30.));
#56500=CARTESIAN_POINT('Ctrl Pts',(126.377781991937,-35.8223498160256,29.9999999999999));
#56501=CARTESIAN_POINT('Ctrl Pts',(126.369641629914,-35.7564698002806,29.9999999999999));
#56502=CARTESIAN_POINT('Ctrl Pts',(126.363342135217,-35.6902588634788,30.0000000000001));
#56503=CARTESIAN_POINT('Ctrl Pts',(126.358875193738,-35.6237950595802,29.9999999999999));
#56504=CARTESIAN_POINT('Ctrl Pts',(126.357510944051,-35.6034963330169,29.9999999999998));
#56505=CARTESIAN_POINT('Ctrl Pts',(126.356317658871,-35.5831740353541,29.9999999999999));
#56506=CARTESIAN_POINT('Ctrl Pts',(126.355295185526,-35.5628304336442,30.));
#56507=CARTESIAN_POINT('Ctrl Pts',(126.35456734149,-35.5483489126842,30.0000000000001));
#56508=CARTESIAN_POINT('Ctrl Pts',(126.353926172819,-35.5338582350463,30.0000000000001));
#56509=CARTESIAN_POINT('Ctrl Pts',(126.353371824647,-35.5193686343449,30.0000000000001));
#56510=CARTESIAN_POINT('Ctrl Pts',(126.348947576412,-35.403727249526,30.0000000000001));
#56511=CARTESIAN_POINT('Ctrl Pts',(126.350040249793,-35.2879868021222,29.9999999999999));
#56512=CARTESIAN_POINT('Ctrl Pts',(126.356503368941,-35.1725471859202,30.0000000000001));
#56513=CARTESIAN_POINT('Ctrl Pts',(126.363113237002,-35.0544864454716,30.0000000000002));
#56514=CARTESIAN_POINT('Ctrl Pts',(126.375340363165,-34.9367393586674,30.0000000000002));
#56515=CARTESIAN_POINT('Ctrl Pts',(126.393082724363,-34.8197437025802,30.0000000000002));
#56516=CARTESIAN_POINT('Ctrl Pts',(126.410825085562,-34.702748046493,30.0000000000002));
#56517=CARTESIAN_POINT('Ctrl Pts',(126.434083043154,-34.5865028570309,30.));
#56518=CARTESIAN_POINT('Ctrl Pts',(126.462804329437,-34.4714705833518,29.9999999999999));
#56519=CARTESIAN_POINT('Ctrl Pts',(126.481403635652,-34.3969780811092,29.9999999999998));
#56520=CARTESIAN_POINT('Ctrl Pts',(126.502295031583,-34.3229947638336,30.0000000000002));
#56521=CARTESIAN_POINT('Ctrl Pts',(126.525474385826,-34.2496546116183,30.0000000000001));
#56522=CARTESIAN_POINT('Ctrl Pts',(126.53257453879,-34.2271895207573,30.));
#56523=CARTESIAN_POINT('Ctrl Pts',(126.539889419495,-34.2047848317409,30.0000000000002));
#56524=CARTESIAN_POINT('Ctrl Pts',(126.547419047006,-34.1824445482406,30.0000000000001));
#56525=CARTESIAN_POINT('Ctrl Pts',(126.553170483406,-34.1653801291155,30.0000000000001));
#56526=CARTESIAN_POINT('Ctrl Pts',(126.559046987838,-34.1483541612293,30.));
#56527=CARTESIAN_POINT('Ctrl Pts',(126.565044083677,-34.1313805413347,30.));
#56528=CARTESIAN_POINT('Ctrl Pts',(126.602641717811,-34.0249677095538,30.0000000000001));
#56529=CARTESIAN_POINT('Ctrl Pts',(126.645018327222,-33.9204820438248,29.9999999999998));
#56530=CARTESIAN_POINT('Ctrl Pts',(126.69210907066,-33.8183255357337,30.));
#56531=CARTESIAN_POINT('Ctrl Pts',(126.732414546534,-33.7308886772017,30.0000000000001));
#56532=CARTESIAN_POINT('Ctrl Pts',(126.776174342542,-33.6451582292905,29.9999999999999));
#56533=CARTESIAN_POINT('Ctrl Pts',(126.823370536012,-33.5614064352205,29.9999999999999));
#56534=CARTESIAN_POINT('Ctrl Pts',(126.844837231283,-33.5233128071232,29.9999999999999));
#56535=CARTESIAN_POINT('Ctrl Pts',(126.867015116863,-33.4856288122295,29.9999999999999));
#56536=CARTESIAN_POINT('Ctrl Pts',(126.889903809861,-33.448381667042,30.));
#56537=CARTESIAN_POINT('Ctrl Pts',(126.903889653885,-33.4256222738776,30.0000000000001));
#56538=CARTESIAN_POINT('Ctrl Pts',(126.9181432011,-33.4030226799343,29.9999999999998));
#56539=CARTESIAN_POINT('Ctrl Pts',(126.932649322486,-33.3806120942224,29.9999999999998));
#56540=CARTESIAN_POINT('Ctrl Pts',(126.991212030765,-33.2901382481445,29.9999999999998));
#56541=CARTESIAN_POINT('Ctrl Pts',(127.053930677688,-33.2026705753962,29.9999999999999));
#56542=CARTESIAN_POINT('Ctrl Pts',(127.120768947966,-33.1185902784384,30.));
#56543=CARTESIAN_POINT('Ctrl Pts',(127.187607218243,-33.0345099814805,30.));
#56544=CARTESIAN_POINT('Ctrl Pts',(127.258565397579,-32.9538164052713,29.9999999999999));
#56545=CARTESIAN_POINT('Ctrl Pts',(127.333638398083,-32.8769328424591,30.));
#56546=CARTESIAN_POINT('Ctrl Pts',(127.362444874375,-32.8474316301123,30.));
#56547=CARTESIAN_POINT('Ctrl Pts',(127.391857525546,-32.8184918975039,29.9999999999999));
#56548=CARTESIAN_POINT('Ctrl Pts',(127.421855683173,-32.7901223422051,29.9999999999999));
#56549=CARTESIAN_POINT('Origin',(-10.,-35.,17.));
#56550=CARTESIAN_POINT('Ctrl Pts',(-6.62123117139838,-35.2726284383003,
17.));
#56551=CARTESIAN_POINT('Ctrl Pts',(-6.60195936274602,-35.1678051036246,
17.));
#56552=CARTESIAN_POINT('Ctrl Pts',(-6.58807248374327,-35.0622614892112,
17.));
#56553=CARTESIAN_POINT('Ctrl Pts',(-6.57934242661586,-34.9563326165135,
17.));
#56554=CARTESIAN_POINT('Ctrl Pts',(-6.57037153216212,-34.8474814689544,
17.));
#56555=CARTESIAN_POINT('Ctrl Pts',(-6.56684579918875,-34.7382228961907,
17.));
#56556=CARTESIAN_POINT('Ctrl Pts',(-6.56856914163975,-34.6289004249964,
17.));
#56557=CARTESIAN_POINT('Ctrl Pts',(-6.56942711098046,-34.5744740232787,
17.));
#56558=CARTESIAN_POINT('Ctrl Pts',(-6.57158689612088,-34.5200315365156,
17.));
#56559=CARTESIAN_POINT('Ctrl Pts',(-6.57502897084565,-34.465614347352,17.));
#56560=CARTESIAN_POINT('Ctrl Pts',(-6.57632076661394,-34.4451918114384,
17.));
#56561=CARTESIAN_POINT('Ctrl Pts',(-6.57779265782301,-34.4247816698274,
17.));
#56562=CARTESIAN_POINT('Ctrl Pts',(-6.57944296507798,-34.4043890422814,
17.));
#56563=CARTESIAN_POINT('Ctrl Pts',(-6.58842189201816,-34.2934376347159,
17.));
#56564=CARTESIAN_POINT('Ctrl Pts',(-6.60267989553898,-34.1829782686288,
17.));
#56565=CARTESIAN_POINT('Ctrl Pts',(-6.62200581466125,-34.0733656510403,
17.));
#56566=CARTESIAN_POINT('Ctrl Pts',(-6.64170770786029,-33.9616205862218,
17.));
#56567=CARTESIAN_POINT('Ctrl Pts',(-6.66667661424612,-33.8507547385056,
17.));
#56568=CARTESIAN_POINT('Ctrl Pts',(-6.69674188079343,-33.7411363045331,
17.));
#56569=CARTESIAN_POINT('Ctrl Pts',(-6.70213413683576,-33.7214760543234,
17.));
#56570=CARTESIAN_POINT('Ctrl Pts',(-6.7076904628942,-33.7018559288903,17.));
#56571=CARTESIAN_POINT('Ctrl Pts',(-6.71341005038338,-33.6822780588274,
17.));
#56572=CARTESIAN_POINT('Ctrl Pts',(-6.7206963490438,-33.6573374125511,17.));
#56573=CARTESIAN_POINT('Ctrl Pts',(-6.72824940271889,-33.6324599742726,
17.));
#56574=CARTESIAN_POINT('Ctrl Pts',(-6.7360574985804,-33.6076813199021,17.));
#56575=CARTESIAN_POINT('Ctrl Pts',(-6.77081749559188,-33.4973719734054,
17.));
#56576=CARTESIAN_POINT('Ctrl Pts',(-6.81065448189253,-33.3889213989467,
17.));
#56577=CARTESIAN_POINT('Ctrl Pts',(-6.85534159827004,-33.2827019280528,
17.));
#56578=CARTESIAN_POINT('Ctrl Pts',(-6.90044356785989,-33.1754963678275,
17.));
#56579=CARTESIAN_POINT('Ctrl Pts',(-6.95048625969968,-33.0705626493514,
17.));
#56580=CARTESIAN_POINT('Ctrl Pts',(-7.00528986546843,-32.9682816440293,
17.));
#56581=CARTESIAN_POINT('Ctrl Pts',(-7.05981998464246,-32.8665110519083,
17.));
#56582=CARTESIAN_POINT('Ctrl Pts',(-7.11906386156907,-32.7673658768366,
17.));
#56583=CARTESIAN_POINT('Ctrl Pts',(-7.18289409730164,-32.671232657024,17.));
#56584=CARTESIAN_POINT('Ctrl Pts',(-7.22018368206598,-32.6150716886722,
17.));
#56585=CARTESIAN_POINT('Ctrl Pts',(-7.25903945429618,-32.5599389460292,
17.));
#56586=CARTESIAN_POINT('Ctrl Pts',(-7.29944343578837,-32.5059151540895,
17.));
#56587=CARTESIAN_POINT('Ctrl Pts',(-7.32106075068243,-32.4770108412222,
17.));
#56588=CARTESIAN_POINT('Ctrl Pts',(-7.34312134161498,-32.448424027476,17.));
#56589=CARTESIAN_POINT('Ctrl Pts',(-7.36562307324715,-32.4201675125236,
17.));
#56590=CARTESIAN_POINT('Ctrl Pts',(-7.37557070373355,-32.4076757908119,
17.));
#56591=CARTESIAN_POINT('Ctrl Pts',(-7.3856037462521,-32.39524973087,17.));
#56592=CARTESIAN_POINT('Ctrl Pts',(-7.39571409769092,-32.3828998151529,
17.));
#56593=CARTESIAN_POINT('Ctrl Pts',(-7.47117758841242,-32.2907202548503,
17.));
#56594=CARTESIAN_POINT('Ctrl Pts',(-7.55105817840693,-32.2026374053398,
17.));
#56595=CARTESIAN_POINT('Ctrl Pts',(-7.63516588800145,-32.1190387156275,
17.));
#56596=CARTESIAN_POINT('Ctrl Pts',(-7.65864346748547,-32.0957032224611,
17.));
#56597=CARTESIAN_POINT('Ctrl Pts',(-7.68245071568654,-32.0727172019008,
17.));
#56598=CARTESIAN_POINT('Ctrl Pts',(-7.70658419094811,-32.0500893063318,
17.));
#56599=CARTESIAN_POINT('Ctrl Pts',(-7.79064406788299,-31.9712735495372,
17.));
#56600=CARTESIAN_POINT('Ctrl Pts',(-7.87865820844732,-31.8968001233851,
17.));
#56601=CARTESIAN_POINT('Ctrl Pts',(-7.97020004902603,-31.8266803948519,
17.));
#56602=CARTESIAN_POINT('Ctrl Pts',(-8.06174188960474,-31.7565606663187,
17.));
#56603=CARTESIAN_POINT('Ctrl Pts',(-8.15681210589746,-31.6907943583393,
17.));
#56604=CARTESIAN_POINT('Ctrl Pts',(-8.2550244894812,-31.6294268457453,17.));
#56605=CARTESIAN_POINT('Ctrl Pts',(-8.31110600223239,-31.5943845953236,
17.));
#56606=CARTESIAN_POINT('Ctrl Pts',(-8.36821275697467,-31.5607772919423,
17.));
#56607=CARTESIAN_POINT('Ctrl Pts',(-8.4262774446775,-31.5286188972515,17.));
#56608=CARTESIAN_POINT('Ctrl Pts',(-8.44233628183896,-31.5197249129016,
17.));
#56609=CARTESIAN_POINT('Ctrl Pts',(-8.45846840796252,-31.5109417802214,
17.));
#56610=CARTESIAN_POINT('Ctrl Pts',(-8.47467243570209,-31.5022698523055,
17.));
#56611=CARTESIAN_POINT('Ctrl Pts',(-8.48766853586036,-31.495314714634,17.));
#56612=CARTESIAN_POINT('Ctrl Pts',(-8.50071001765182,-31.4884316194093,
17.));
#56613=CARTESIAN_POINT('Ctrl Pts',(-8.51378706273541,-31.4816253310382,
17.));
#56614=CARTESIAN_POINT('Ctrl Pts',(-8.61982624789618,-31.4264344780416,
17.));
#56615=CARTESIAN_POINT('Ctrl Pts',(-8.72835801098144,-31.3762061453459,
17.));
#56616=CARTESIAN_POINT('Ctrl Pts',(-8.83892749372354,-31.3309409256438,
17.));
#56617=CARTESIAN_POINT('Ctrl Pts',(-8.95138481870543,-31.2849028562219,
17.));
#56618=CARTESIAN_POINT('Ctrl Pts',(-9.06595070186539,-31.2439984397476,
17.));
#56619=CARTESIAN_POINT('Ctrl Pts',(-9.18218640297054,-31.208266008192,17.));
#56620=CARTESIAN_POINT('Ctrl Pts',(-9.29985863077184,-31.1720919688398,
17.));
#56621=CARTESIAN_POINT('Ctrl Pts',(-9.41924298093842,-31.1412181424403,
17.));
#56622=CARTESIAN_POINT('Ctrl Pts',(-9.53991371679841,-31.1157285615814,
17.));
#56623=CARTESIAN_POINT('Ctrl Pts',(-9.61457871346185,-31.0999568878925,
17.));
#56624=CARTESIAN_POINT('Ctrl Pts',(-9.68973674093548,-31.0862474736742,
17.));
#56625=CARTESIAN_POINT('Ctrl Pts',(-9.76529045541688,-31.0746295822446,
17.));
#56626=CARTESIAN_POINT('Ctrl Pts',(-9.80157333625044,-31.0690503652177,
17.));
#56627=CARTESIAN_POINT('Ctrl Pts',(-9.83794749841506,-31.0639535993401,
17.));
#56628=CARTESIAN_POINT('Ctrl Pts',(-9.87440228076019,-31.0593431503807,
17.));
#56629=CARTESIAN_POINT('Ctrl Pts',(-9.89072382555558,-31.0572789589529,
17.));
#56630=CARTESIAN_POINT('Ctrl Pts',(-9.90706204440871,-31.0553121984509,
17.));
#56631=CARTESIAN_POINT('Ctrl Pts',(-9.9234144236545,-31.0534434210371,17.));
#56632=CARTESIAN_POINT('Ctrl Pts',(-10.0491353854642,-31.0390758179906,
17.));
#56633=CARTESIAN_POINT('Ctrl Pts',(-10.1751595106833,-31.0305566396611,
17.));
#56634=CARTESIAN_POINT('Ctrl Pts',(-10.3010219327232,-31.0279204753263,
17.));
#56635=CARTESIAN_POINT('Ctrl Pts',(-10.4271451736567,-31.0252788481897,
17.));
#56636=CARTESIAN_POINT('Ctrl Pts',(-10.5531069280695,-31.0285443279939,
17.));
#56637=CARTESIAN_POINT('Ctrl Pts',(-10.6784621466317,-31.0377989166891,
17.));
#56638=CARTESIAN_POINT('Ctrl Pts',(-10.8015650460913,-31.04688722362,17.));
#56639=CARTESIAN_POINT('Ctrl Pts',(-10.924083889428,-31.061751209596,17.));
#56640=CARTESIAN_POINT('Ctrl Pts',(-11.0456058942539,-31.0825171502249,
17.));
#56641=CARTESIAN_POINT('Ctrl Pts',(-11.1383505538559,-31.0983655564268,
17.));
#56642=CARTESIAN_POINT('Ctrl Pts',(-11.2305148677362,-31.1176525692725,
17.));
#56643=CARTESIAN_POINT('Ctrl Pts',(-11.3219141163422,-31.1404548077392,
17.));
#56644=CARTESIAN_POINT('Ctrl Pts',(-11.3696276429971,-31.152358354316,17.));
#56645=CARTESIAN_POINT('Ctrl Pts',(-11.4171326273164,-31.165220183099,17.));
#56646=CARTESIAN_POINT('Ctrl Pts',(-11.4644130279462,-31.1790224515809,
17.));
#56647=CARTESIAN_POINT('Ctrl Pts',(-13.1750507821944,-32.4297320119321,
17.));
#56648=CARTESIAN_POINT('Ctrl Pts',(-13.2457830379296,-32.5339316716807,
17.));
#56649=CARTESIAN_POINT('Ctrl Pts',(-13.3111684320266,-32.6414695796738,
17.));
#56650=CARTESIAN_POINT('Ctrl Pts',(-13.3712014634247,-32.7519056634986,
17.));
#56651=CARTESIAN_POINT('Ctrl Pts',(-13.4312344948227,-32.8623417473234,
17.));
#56652=CARTESIAN_POINT('Ctrl Pts',(-13.4859151823647,-32.9756769087957,
17.));
#56653=CARTESIAN_POINT('Ctrl Pts',(-13.5351879905628,-33.0914857757907,
17.));
#56654=CARTESIAN_POINT('Ctrl Pts',(-13.5568745982239,-33.1424571239651,
17.));
#56655=CARTESIAN_POINT('Ctrl Pts',(-13.577512952621,-33.1939077821244,17.));
#56656=CARTESIAN_POINT('Ctrl Pts',(-13.5970952298849,-33.2458016998049,
17.));
#56657=CARTESIAN_POINT('Ctrl Pts',(-13.6073220395261,-33.2729032064631,
17.));
#56658=CARTESIAN_POINT('Ctrl Pts',(-13.6172620907691,-33.3001296513874,
17.));
#56659=CARTESIAN_POINT('Ctrl Pts',(-13.6269050370344,-33.3274493235186,
17.));
#56660=CARTESIAN_POINT('Ctrl Pts',(-13.6685917972946,-33.4455531261519,
17.));
#56661=CARTESIAN_POINT('Ctrl Pts',(-13.7047654844905,-33.5654872367405,
17.));
#56662=CARTESIAN_POINT('Ctrl Pts',(-13.7353853470909,-33.686824179545,17.));
#56663=CARTESIAN_POINT('Ctrl Pts',(-13.7610632945821,-33.7885778577618,
17.));
#56664=CARTESIAN_POINT('Ctrl Pts',(-13.7828345727888,-33.8913185884214,
17.));
#56665=CARTESIAN_POINT('Ctrl Pts',(-13.8006468889342,-33.9947943925399,
17.));
#56666=CARTESIAN_POINT('Ctrl Pts',(-13.8084972326622,-34.0403988284389,
17.));
#56667=CARTESIAN_POINT('Ctrl Pts',(-13.8155782548013,-34.0861460076211,
17.));
#56668=CARTESIAN_POINT('Ctrl Pts',(-13.8218838856489,-34.1320140579904,
17.));
#56669=CARTESIAN_POINT('Ctrl Pts',(-13.8245828861217,-34.151646969055,17.));
#56670=CARTESIAN_POINT('Ctrl Pts',(-13.8271398150965,-34.1713020216297,
17.));
#56671=CARTESIAN_POINT('Ctrl Pts',(-13.8295541419123,-34.1909774839374,
17.));
#56672=CARTESIAN_POINT('Ctrl Pts',(-13.8317972215008,-34.20925737364,17.));
#56673=CARTESIAN_POINT('Ctrl Pts',(-13.833916727226,-34.2275513035412,17.));
#56674=CARTESIAN_POINT('Ctrl Pts',(-13.835911424144,-34.2458481127575,17.));
#56675=CARTESIAN_POINT('Ctrl Pts',(-13.8491700107784,-34.3674655013118,
17.));
#56676=CARTESIAN_POINT('Ctrl Pts',(-13.8569344264697,-34.4893371723603,
17.));
#56677=CARTESIAN_POINT('Ctrl Pts',(-13.8591700411928,-34.611066101442,17.));
#56678=CARTESIAN_POINT('Ctrl Pts',(-13.8613878458839,-34.7318252766074,
17.));
#56679=CARTESIAN_POINT('Ctrl Pts',(-13.8581645033039,-34.8524448082591,
17.));
#56680=CARTESIAN_POINT('Ctrl Pts',(-13.8494158248468,-34.9725303958732,
17.));
#56681=CARTESIAN_POINT('Ctrl Pts',(-13.840878077774,-35.0897207097202,17.));
#56682=CARTESIAN_POINT('Ctrl Pts',(-13.8270780176714,-35.2064031908734,
17.));
#56683=CARTESIAN_POINT('Ctrl Pts',(-13.8078915167199,-35.3221939954455,
17.));
#56684=CARTESIAN_POINT('Ctrl Pts',(-13.7961959663632,-35.3927768072427,
17.));
#56685=CARTESIAN_POINT('Ctrl Pts',(-13.7824980530838,-35.4630279096876,
17.));
#56686=CARTESIAN_POINT('Ctrl Pts',(-13.7667614148585,-35.532855489557,17.));
#56687=CARTESIAN_POINT('Ctrl Pts',(-13.757216255672,-35.5752098574922,17.));
#56688=CARTESIAN_POINT('Ctrl Pts',(-13.7469209067431,-35.6174083281479,
17.));
#56689=CARTESIAN_POINT('Ctrl Pts',(-13.7358661344643,-35.6594295784058,
17.));
#56690=CARTESIAN_POINT('Ctrl Pts',(-13.7309267403395,-35.6782051362742,
17.));
#56691=CARTESIAN_POINT('Ctrl Pts',(-13.7258352371277,-35.6969467100214,
17.));
#56692=CARTESIAN_POINT('Ctrl Pts',(-13.7205966738498,-35.7156322006019,
17.));
#56693=CARTESIAN_POINT('Ctrl Pts',(-13.6893367538286,-35.8271335627347,
17.));
#56694=CARTESIAN_POINT('Ctrl Pts',(-13.6528018180032,-35.9368053180647,
17.));
#56695=CARTESIAN_POINT('Ctrl Pts',(-13.6109158237098,-36.0442928075802,
17.));
#56696=CARTESIAN_POINT('Ctrl Pts',(-13.5979435125947,-36.0775822442643,
17.));
#56697=CARTESIAN_POINT('Ctrl Pts',(-13.5844575975254,-36.1106620277172,
17.));
#56698=CARTESIAN_POINT('Ctrl Pts',(-13.5704548945751,-36.1435211813812,
17.));
#56699=CARTESIAN_POINT('Ctrl Pts',(-13.5245394274593,-36.2512677639423,
17.));
#56700=CARTESIAN_POINT('Ctrl Pts',(-13.4730705027225,-36.3566445855268,
17.));
#56701=CARTESIAN_POINT('Ctrl Pts',(-13.4163937309752,-36.4593820470852,
17.));
#56702=CARTESIAN_POINT('Ctrl Pts',(-13.3593202829442,-36.5628385600856,
17.));
#56703=CARTESIAN_POINT('Ctrl Pts',(-13.2969650692165,-36.6636192426463,
17.));
#56704=CARTESIAN_POINT('Ctrl Pts',(-13.2296453006718,-36.7614105285874,
17.));
#56705=CARTESIAN_POINT('Ctrl Pts',(-13.1959565268153,-36.8103481376796,
17.));
#56706=CARTESIAN_POINT('Ctrl Pts',(-13.1610239983712,-36.8585364607721,
17.));
#56707=CARTESIAN_POINT('Ctrl Pts',(-13.1248850662753,-36.9059319156406,
17.));
#56708=CARTESIAN_POINT('Ctrl Pts',(-13.1136839868388,-36.9206218974448,
17.));
#56709=CARTESIAN_POINT('Ctrl Pts',(-13.1023670038866,-36.9352356893667,
17.));
#56710=CARTESIAN_POINT('Ctrl Pts',(-13.0909352063088,-36.9497719323387,
17.));
#56711=CARTESIAN_POINT('Ctrl Pts',(-13.0810899908133,-36.9622907373281,
17.));
#56712=CARTESIAN_POINT('Ctrl Pts',(-13.0711625418207,-36.9747482535312,
17.));
#56713=CARTESIAN_POINT('Ctrl Pts',(-13.0611586777581,-36.9871376957437,
17.));
#56714=CARTESIAN_POINT('Ctrl Pts',(-12.9882938384087,-37.0773782978546,
17.));
#56715=CARTESIAN_POINT('Ctrl Pts',(-12.9112998416349,-37.1641103597806,
17.));
#56716=CARTESIAN_POINT('Ctrl Pts',(-12.8305219931231,-37.2470878105587,
17.));
#56717=CARTESIAN_POINT('Ctrl Pts',(-12.7496930685579,-37.3301177282046,
17.));
#56718=CARTESIAN_POINT('Ctrl Pts',(-12.6650746977764,-37.409388808979,17.));
#56719=CARTESIAN_POINT('Ctrl Pts',(-12.5769811318078,-37.4846132121967,
17.));
#56720=CARTESIAN_POINT('Ctrl Pts',(-12.4904409634934,-37.5585111461063,
17.));
#56721=CARTESIAN_POINT('Ctrl Pts',(-12.4005462848826,-37.6285042016323,
17.));
#56722=CARTESIAN_POINT('Ctrl Pts',(-12.3075763963486,-37.694273447211,17.));
#56723=CARTESIAN_POINT('Ctrl Pts',(-12.2551724160701,-37.731345345463,17.));
#56724=CARTESIAN_POINT('Ctrl Pts',(-12.2017911097264,-37.767074392327,17.));
#56725=CARTESIAN_POINT('Ctrl Pts',(-12.1474812222069,-37.8013962232141,
17.));
#56726=CARTESIAN_POINT('Ctrl Pts',(-12.1187449086064,-37.8195565056371,
17.));
#56727=CARTESIAN_POINT('Ctrl Pts',(-12.08974861503,-37.8373227245847,17.));
#56728=CARTESIAN_POINT('Ctrl Pts',(-12.0604995325634,-37.8546847045796,
17.));
#56729=CARTESIAN_POINT('Ctrl Pts',(-12.0426076402161,-37.8653051634387,
17.));
#56730=CARTESIAN_POINT('Ctrl Pts',(-12.024619808101,-37.8757749838419,17.));
#56731=CARTESIAN_POINT('Ctrl Pts',(-12.0065599568337,-37.8860794595539,
17.));
#56732=CARTESIAN_POINT('Ctrl Pts',(-11.9096687237166,-37.9413630465328,
17.));
#56733=CARTESIAN_POINT('Ctrl Pts',(-11.8105593158835,-37.9919798651834,
17.));
#56734=CARTESIAN_POINT('Ctrl Pts',(-11.7095166454714,-38.0376717971112,
17.));
#56735=CARTESIAN_POINT('Ctrl Pts',(-11.6099952290825,-38.0826758114,17.));
#56736=CARTESIAN_POINT('Ctrl Pts',(-11.5085976071889,-38.1229024009533,
17.));
#56737=CARTESIAN_POINT('Ctrl Pts',(-11.4055841475048,-38.1580565561197,
17.));
#56738=CARTESIAN_POINT('Ctrl Pts',(-11.3056451647854,-38.1921615217861,
17.));
#56739=CARTESIAN_POINT('Ctrl Pts',(-11.2041847596975,-38.2214924163805,
17.));
#56740=CARTESIAN_POINT('Ctrl Pts',(-11.101438968834,-38.2457313749553,17.));
#56741=CARTESIAN_POINT('Ctrl Pts',(-11.0378253219427,-38.2607385936338,
17.));
#56742=CARTESIAN_POINT('Ctrl Pts',(-10.9737189501175,-38.2737929603252,
17.));
#56743=CARTESIAN_POINT('Ctrl Pts',(-10.9091769854019,-38.2848089949374,
17.));
#56744=CARTESIAN_POINT('Ctrl Pts',(-10.8685412172475,-38.2917447154481,
17.));
#56745=CARTESIAN_POINT('Ctrl Pts',(-10.8277327929855,-38.2978722505483,
17.));
#56746=CARTESIAN_POINT('Ctrl Pts',(-10.7867735403064,-38.3031951868165,
17.));
#56747=CARTESIAN_POINT('Ctrl Pts',(-7.43281991866731,-32.7955655913445,
29.9966885573452));
#56748=CARTESIAN_POINT('Ctrl Pts',(-6.70433287707855,-33.6438343820474,
29.9309496672087));
#56749=CARTESIAN_POINT('Ctrl Pts',(-6.16680494687376,-36.1040434535625,
29.7995176262159));
#56750=CARTESIAN_POINT('Ctrl Pts',(-8.82688604484989,-38.8162402853805,
29.602392434367));
#56751=CARTESIAN_POINT('Ctrl Pts',(-12.5469213771536,-38.0704890626947,
29.4053129817986));
#56752=CARTESIAN_POINT('Ctrl Pts',(-13.9650986146378,-34.5542581135541,
29.2082335292301));
#56753=CARTESIAN_POINT('Ctrl Pts',(-11.8002655329401,-31.4387142292477,
29.0111540766617));
#56754=CARTESIAN_POINT('Ctrl Pts',(-8.00850995998504,-31.5424701940952,
28.8140746240932));
#56755=CARTESIAN_POINT('Ctrl Pts',(-6.01644574177587,-34.7701684626168,
28.6169951715248));
#56756=CARTESIAN_POINT('Ctrl Pts',(-7.62419332014188,-38.2058271295203,
28.4199157189564));
#56757=CARTESIAN_POINT('Ctrl Pts',(-11.378901931472,-38.7443323602222,28.2228362663879));
#56758=CARTESIAN_POINT('Ctrl Pts',(-13.8875297661741,-35.8992536493971,
28.0257568138195));
#56759=CARTESIAN_POINT('Ctrl Pts',(-12.8831047926849,-32.2415099196181,
27.828677361251));
#56760=CARTESIAN_POINT('Ctrl Pts',(-9.27329515907125,-31.0765558017924,
27.6315979086826));
#56761=CARTESIAN_POINT('Ctrl Pts',(-6.32018953277514,-33.4571031196912,
27.4345184561141));
#56762=CARTESIAN_POINT('Ctrl Pts',(-6.6924284169921,-37.2319287467791,27.2374390035457));
#56763=CARTESIAN_POINT('Ctrl Pts',(-10.0536300734982,-38.9898188142619,
27.0403595509773));
#56764=CARTESIAN_POINT('Ctrl Pts',(-13.3663676160112,-37.142219039571,26.8432800984088));
#56765=CARTESIAN_POINT('Ctrl Pts',(-13.6370101893174,-33.3587535440872,
26.6462006458404));
#56766=CARTESIAN_POINT('Ctrl Pts',(-10.6209853939007,-31.0584381780949,
26.4491211932719));
#56767=CARTESIAN_POINT('Ctrl Pts',(-7.04379296919064,-32.3200050661253,
26.2520417407035));
#56768=CARTESIAN_POINT('Ctrl Pts',(-6.13804456209019,-36.0034106733504,
26.0549622881351));
#56769=CARTESIAN_POINT('Ctrl Pts',(-8.72224042076868,-38.7800612666714,
25.8578828355666));
#56770=CARTESIAN_POINT('Ctrl Pts',(-12.4611129143278,-38.14077315272,25.6608033829982));
#56771=CARTESIAN_POINT('Ctrl Pts',(-13.9759444957377,-34.6632536150714,
25.4637239304297));
#56772=CARTESIAN_POINT('Ctrl Pts',(-11.8978229970468,-31.490042645999,25.2666444778613));
#56773=CARTESIAN_POINT('Ctrl Pts',(-8.10469038869652,-31.4886848277523,
25.0695650252928));
#56774=CARTESIAN_POINT('Ctrl Pts',(-6.02429761163027,-34.6604071871109,
24.8724855727244));
#56775=CARTESIAN_POINT('Ctrl Pts',(-7.53663912855336,-38.1390103497744,
24.6754061201559));
#56776=CARTESIAN_POINT('Ctrl Pts',(-11.2750529760013,-38.7809750948868,
24.4783266675875));
#56777=CARTESIAN_POINT('Ctrl Pts',(-13.861236071256,-36.0061753134915,24.2812472150191));
#56778=CARTESIAN_POINT('Ctrl Pts',(-12.958124975163,-32.3221222225917,24.0841677624506));
#56779=CARTESIAN_POINT('Ctrl Pts',(-9.38183666260023,-31.0579945652231,
23.8870883098822));
#56780=CARTESIAN_POINT('Ctrl Pts',(-6.36416577271778,-33.3561501798544,
23.6900088573138));
#56781=CARTESIAN_POINT('Ctrl Pts',(-6.63209954823897,-37.1398082405902,
23.4929294047453));
#56782=CARTESIAN_POINT('Ctrl Pts',(-9.94351351157651,-38.9897796976916,
23.2958499521769));
#56783=CARTESIAN_POINT('Ctrl Pts',(-13.305972780694,-37.2342955786512,23.0987704996084));
#56784=CARTESIAN_POINT('Ctrl Pts',(-13.6809142167823,-33.459739214237,22.90169104704));
#56785=CARTESIAN_POINT('Ctrl Pts',(-10.7295134250377,-31.0770746983652,
22.7046115944715));
#56786=CARTESIAN_POINT('Ctrl Pts',(-7.11887115996344,-32.2394512562663,
22.5075321419031));
#56787=CARTESIAN_POINT('Ctrl Pts',(-6.11182679476447,-35.8964607551567,
22.3104526893346));
#56788=CARTESIAN_POINT('Ctrl Pts',(-8.61841897744962,-38.7433630117707,
22.1133732367662));
#56789=CARTESIAN_POINT('Ctrl Pts',(-12.3735084153843,-38.2074897600872,
21.9162937841978));
#56790=CARTESIAN_POINT('Ctrl Pts',(-13.9837227475169,-34.7730951072122,
21.7192143316293));
#56791=CARTESIAN_POINT('Ctrl Pts',(-11.9939550048957,-31.5437482441223,
21.5221348790609));
#56792=CARTESIAN_POINT('Ctrl Pts',(-8.20230426734218,-31.4377222444328,
21.3250554264924));
#56793=CARTESIAN_POINT('Ctrl Pts',(-6.0351823494922,-34.5508299217764,21.127975973924));
#56794=CARTESIAN_POINT('Ctrl Pts',(-7.45095848371802,-38.0698404066318,
20.9308965213555));
#56795=CARTESIAN_POINT('Ctrl Pts',(-11.1702342203526,-38.814719464341,20.7338170687871));
#56796=CARTESIAN_POINT('Ctrl Pts',(-13.8320010687388,-36.112340142663,20.5367376162187));
#56797=CARTESIAN_POINT('Ctrl Pts',(-13.0308926023777,-32.4047692034324,
20.3396581636502));
#56798=CARTESIAN_POINT('Ctrl Pts',(-9.49084879340863,-31.0424379342625,
20.1425787110818));
#56799=CARTESIAN_POINT('Ctrl Pts',(-6.41091109924001,-33.2564479047973,
19.9454992585133));
#56800=CARTESIAN_POINT('Ctrl Pts',(-6.5743355988234,-37.0460588334994,19.7484198059449));
#56801=CARTESIAN_POINT('Ctrl Pts',(-9.8334399776528,-38.9867014077275,19.5513403533764));
#56802=CARTESIAN_POINT('Ctrl Pts',(-13.2430601681256,-37.3246712570463,
19.354260900808));
#56803=CARTESIAN_POINT('Ctrl Pts',(-13.7220148613169,-33.561896655278,19.1571814482396));
#56804=CARTESIAN_POINT('Ctrl Pts',(-10.8374859573864,-31.0987012965605,
18.9601019956711));
#56805=CARTESIAN_POINT('Ctrl Pts',(-7.1961434015981,-32.1609950784182,18.7630225431027));
#56806=CARTESIAN_POINT('Ctrl Pts',(-6.08857058207861,-35.7888375735615,
18.5659430905342));
#56807=CARTESIAN_POINT('Ctrl Pts',(-8.51564899808879,-38.7037950083057,
18.3688636379658));
#56808=CARTESIAN_POINT('Ctrl Pts',(-12.2840977384796,-38.2718011072648,
18.1717841853974));
#56809=CARTESIAN_POINT('Ctrl Pts',(-13.9884641375675,-34.8830346755273,
17.9747047328289));
#56810=CARTESIAN_POINT('Ctrl Pts',(-12.0885742245895,-31.6002349130302,
17.7776252802605));
#56811=CARTESIAN_POINT('Ctrl Pts',(-8.30127573310404,-31.3891762442465,
17.580545827692));
#56812=CARTESIAN_POINT('Ctrl Pts',(-6.04910953722514,-34.4421851523227,
17.3834663751236));
#56813=CARTESIAN_POINT('Ctrl Pts',(-7.36717415028043,-37.9971552563352,
17.1863869225551));
#56814=CARTESIAN_POINT('Ctrl Pts',(-11.0646063138124,-38.8479214732267,
16.9893074699867));
#56815=CARTESIAN_POINT('Ctrl Pts',(-13.7997685140726,-36.2127299742061,
16.7922280174183));
#56816=CARTESIAN_POINT('Ctrl Pts',(-13.3330643605671,-33.7394001666604,
16.660841715706));
#56817=CARTESIAN_POINT('Ctrl Pts',(-12.6300276622661,-32.8709392788408,
16.5951485648498));
#56818=CARTESIAN_POINT('Ctrl Pts',(-7.2545283688926,-32.642466854737,30.1323684526006));
#56819=CARTESIAN_POINT('Ctrl Pts',(-6.47544764882367,-33.5496482080684,
30.066629562464));
#56820=CARTESIAN_POINT('Ctrl Pts',(-5.90058821685929,-36.180719655511,29.9351975214714));
#56821=CARTESIAN_POINT('Ctrl Pts',(-8.74541287253645,-39.0812795008765,
29.7380723296225));
#56822=CARTESIAN_POINT('Ctrl Pts',(-12.7238059528751,-38.283735596327,29.5409928770541));
#56823=CARTESIAN_POINT('Ctrl Pts',(-14.2404760928887,-34.5233011844661,
29.3439134244856));
#56824=CARTESIAN_POINT('Ctrl Pts',(-11.9252946005181,-31.1913816934919,
29.1468339719172));
#56825=CARTESIAN_POINT('Ctrl Pts',(-7.87020028386335,-31.3023435461948,
28.9497545193487));
#56826=CARTESIAN_POINT('Ctrl Pts',(-5.73978651265714,-34.7542065823867,
28.7526750667803));
#56827=CARTESIAN_POINT('Ctrl Pts',(-7.45919271967868,-38.428472938978,28.5555956142119));
#56828=CARTESIAN_POINT('Ctrl Pts',(-11.474667150335,-39.0043775452991,28.3585161616434));
#56829=CARTESIAN_POINT('Ctrl Pts',(-14.1575200609129,-35.9617071281995,
28.161436709075));
#56830=CARTESIAN_POINT('Ctrl Pts',(-13.0833374235737,-32.0499318238524,
27.9643572565065));
#56831=CARTESIAN_POINT('Ctrl Pts',(-9.22282525504695,-30.8040712372542,
27.7672778039381));
#56832=CARTESIAN_POINT('Ctrl Pts',(-6.06462541561428,-33.3499483945774,
27.5701983513697));
#56833=CARTESIAN_POINT('Ctrl Pts',(-6.46271641984263,-37.3869369747346,
27.3731188988012));
#56834=CARTESIAN_POINT('Ctrl Pts',(-10.0573547007607,-39.2669131189769,
27.1760394462328));
#56835=CARTESIAN_POINT('Ctrl Pts',(-13.6001630181079,-37.2909968971508,
26.9789599936643));
#56836=CARTESIAN_POINT('Ctrl Pts',(-13.8896018122872,-33.2447684067318,
26.7818805410959));
#56837=CARTESIAN_POINT('Ctrl Pts',(-10.664113045549,-30.7846953382877,26.5848010885274));
#56838=CARTESIAN_POINT('Ctrl Pts',(-6.83848336243165,-32.1338784855931,
26.387721635959));
#56839=CARTESIAN_POINT('Ctrl Pts',(-5.86983041334672,-36.0730978937028,
26.1906421833905));
#56840=CARTESIAN_POINT('Ctrl Pts',(-8.63349957345641,-39.0425878367312,
25.9935627308221));
#56841=CARTESIAN_POINT('Ctrl Pts',(-12.6320380624531,-38.3589009408566,
25.7964832782536));
#56842=CARTESIAN_POINT('Ctrl Pts',(-14.2520752242043,-34.6398664614834,
25.5994038256852));
#56843=CARTESIAN_POINT('Ctrl Pts',(-12.0296274644475,-31.2462748866438,
25.4023243731168));
#56844=CARTESIAN_POINT('Ctrl Pts',(-7.97306047681017,-31.2448227674474,
25.2052449205483));
#56845=CARTESIAN_POINT('Ctrl Pts',(-5.74818369760461,-34.6368223481107,
25.0081654679799));
#56846=CARTESIAN_POINT('Ctrl Pts',(-7.3655578590241,-38.357015710633,24.8110860154114));
#56847=CARTESIAN_POINT('Ctrl Pts',(-11.3636058487777,-39.0435651306342,
24.614006562843));
#56848=CARTESIAN_POINT('Ctrl Pts',(-14.129400259735,-36.0760545390636,24.4169271102746));
#56849=CARTESIAN_POINT('Ctrl Pts',(-13.1635677838246,-32.1361426793127,
24.2198476577061));
#56850=CARTESIAN_POINT('Ctrl Pts',(-9.33890500375777,-30.7842209163476,
24.0227682051376));
#56851=CARTESIAN_POINT('Ctrl Pts',(-6.11165582072035,-33.2419842379472,
23.8256887525693));
#56852=CARTESIAN_POINT('Ctrl Pts',(-6.39819769016606,-37.288418667342,23.6286093000008));
#56853=CARTESIAN_POINT('Ctrl Pts',(-9.93959050530377,-39.2668712857472,
23.4315298474324));
#56854=CARTESIAN_POINT('Ctrl Pts',(-13.5355737404665,-37.3894681839036,
23.2344503948639));
#56855=CARTESIAN_POINT('Ctrl Pts',(-13.936554989734,-33.3527675668065,23.0373709422955));
#56856=CARTESIAN_POINT('Ctrl Pts',(-10.7801783862054,-30.8046261713746,
22.840291489727));
#56857=CARTESIAN_POINT('Ctrl Pts',(-6.91877575967346,-32.0477301856145,
22.6432120371586));
#56858=CARTESIAN_POINT('Ctrl Pts',(-5.84179181295901,-35.9587202664826,
22.4461325845901));
#56859=CARTESIAN_POINT('Ctrl Pts',(-8.52246769477921,-39.0033408752603,
22.2490531320217));
#56860=CARTESIAN_POINT('Ctrl Pts',(-12.5383494005802,-38.4302510398163,
22.0519736794533));
#56861=CARTESIAN_POINT('Ctrl Pts',(-14.2603936782757,-34.7573364834676,
21.8548942268848));
#56862=CARTESIAN_POINT('Ctrl Pts',(-12.132435873686,-31.303710357241,21.6578147743164));
#56863=CARTESIAN_POINT('Ctrl Pts',(-8.0774536732878,-31.1903208149863,21.4607353217479));
#56864=CARTESIAN_POINT('Ctrl Pts',(-5.75982438429787,-34.5196349035768,
21.2636558691795));
#56865=CARTESIAN_POINT('Ctrl Pts',(-7.27392666359651,-38.2830418908748,
21.066576416611));
#56866=CARTESIAN_POINT('Ctrl Pts',(-11.2515073940825,-39.0796530582867,
20.8694969640426));
#56867=CARTESIAN_POINT('Ctrl Pts',(-14.0981348761221,-36.1895925525558,
20.6724175114742));
#56868=CARTESIAN_POINT('Ctrl Pts',(-13.2413891480653,-32.2245295217257,
20.4753380589057));
#56869=CARTESIAN_POINT('Ctrl Pts',(-9.45548806497633,-30.7675838719546,
20.2782586063373));
#56870=CARTESIAN_POINT('Ctrl Pts',(-6.16164762643231,-33.1353576052008,
20.0811791537688));
#56871=CARTESIAN_POINT('Ctrl Pts',(-6.33642201436741,-37.1881583313131,
19.8840997012004));
#56872=CARTESIAN_POINT('Ctrl Pts',(-9.82187232615428,-39.2635792074742,
19.6870202486319));
#56873=CARTESIAN_POINT('Ctrl Pts',(-13.4682918250679,-37.4861204846052,
19.4899407960635));
#56874=CARTESIAN_POINT('Ctrl Pts',(-13.9805100883304,-33.4620198776685,
19.2928613434951));
#56875=CARTESIAN_POINT('Ctrl Pts',(-10.8956496484897,-30.8277547443384,
19.0957818909266));
#56876=CARTESIAN_POINT('Ctrl Pts',(-7.00141458537276,-31.9638251989198,
18.8987024383582));
#56877=CARTESIAN_POINT('Ctrl Pts',(-5.81692044821127,-35.8436226174832,
18.7016229857897));
#56878=CARTESIAN_POINT('Ctrl Pts',(-8.4125603045979,-38.9610248601888,18.5045435332213));
#56879=CARTESIAN_POINT('Ctrl Pts',(-12.4427291210584,-38.4990288324294,
18.3074640806529));
#56880=CARTESIAN_POINT('Ctrl Pts',(-14.2654643595148,-34.8749113930502,
18.1103846280844));
#56881=CARTESIAN_POINT('Ctrl Pts',(-12.2336264311057,-31.3641200449563,
17.913305175516));
#56882=CARTESIAN_POINT('Ctrl Pts',(-8.18329874177914,-31.138403278198,17.7162257229475));
#56883=CARTESIAN_POINT('Ctrl Pts',(-5.77471882006415,-34.4034447170867,
17.5191462703791));
#56884=CARTESIAN_POINT('Ctrl Pts',(-7.18432347905296,-38.205308731603,17.3220668178106));
#56885=CARTESIAN_POINT('Ctrl Pts',(-11.1385435926851,-39.1151609582406,
17.1249873652422));
#56886=CARTESIAN_POINT('Ctrl Pts',(-14.0636637593207,-36.2969544928254,
16.9279079126738));
#56887=CARTESIAN_POINT('Ctrl Pts',(-13.564546839987,-33.6518510696702,16.7965216109615));
#56888=CARTESIAN_POINT('Ctrl Pts',(-12.8126839984014,-32.7230752710526,
16.7308284601053));
#56889=CARTESIAN_POINT('Ctrl Pts',(-7.07623681911788,-32.4893681181295,
30.268048347856));
#56890=CARTESIAN_POINT('Ctrl Pts',(-6.24656242056877,-33.4554620340893,
30.2023094577194));
#56891=CARTESIAN_POINT('Ctrl Pts',(-5.63437148684482,-36.2573958574595,
30.0708774167267));
#56892=CARTESIAN_POINT('Ctrl Pts',(-8.663939700223,-39.3463187163724,29.8737522248779));
#56893=CARTESIAN_POINT('Ctrl Pts',(-12.9006905285965,-38.4969821299593,
29.6766727723095));
#56894=CARTESIAN_POINT('Ctrl Pts',(-14.5158535711396,-34.4923442553782,
29.479593319741));
#56895=CARTESIAN_POINT('Ctrl Pts',(-12.0503236680962,-30.9440491577359,
29.2825138671726));
#56896=CARTESIAN_POINT('Ctrl Pts',(-7.73189060774165,-31.0622168982944,
29.0854344146041));
#56897=CARTESIAN_POINT('Ctrl Pts',(-5.46312728353841,-34.7382447021567,
28.8883549620357));
#56898=CARTESIAN_POINT('Ctrl Pts',(-7.29419211921549,-38.6511187484357,
28.6912755094673));
#56899=CARTESIAN_POINT('Ctrl Pts',(-11.5704323691979,-39.2644227303759,
28.4941960568988));
#56900=CARTESIAN_POINT('Ctrl Pts',(-14.4275103556515,-36.0241606070019,
28.2971166043304));
#56901=CARTESIAN_POINT('Ctrl Pts',(-13.2835700544625,-31.8583537280866,
28.1000371517619));
#56902=CARTESIAN_POINT('Ctrl Pts',(-9.17235535102264,-30.5315866727159,
27.9029576991935));
#56903=CARTESIAN_POINT('Ctrl Pts',(-5.8090612984534,-33.2427936694637,27.7058782466251));
#56904=CARTESIAN_POINT('Ctrl Pts',(-6.23300442269314,-37.5419452026901,
27.5087987940566));
#56905=CARTESIAN_POINT('Ctrl Pts',(-10.0610793280231,-39.5440074236919,
27.3117193414882));
#56906=CARTESIAN_POINT('Ctrl Pts',(-13.8339584202047,-37.4397747547305,
27.1146398889197));
#56907=CARTESIAN_POINT('Ctrl Pts',(-14.1421934352571,-33.1307832693763,
26.9175604363513));
#56908=CARTESIAN_POINT('Ctrl Pts',(-10.7072406971973,-30.5109524984806,
26.7204809837828));
#56909=CARTESIAN_POINT('Ctrl Pts',(-6.63317375567267,-31.9477519050608,
26.5234015312144));
#56910=CARTESIAN_POINT('Ctrl Pts',(-5.60161626460324,-36.1427851140552,
26.3263220786459));
#56911=CARTESIAN_POINT('Ctrl Pts',(-8.54475872614412,-39.3051144067911,
26.1292426260775));
#56912=CARTESIAN_POINT('Ctrl Pts',(-12.8029632105785,-38.577028728993,25.9321631735091));
#56913=CARTESIAN_POINT('Ctrl Pts',(-14.5282059526709,-34.6164793078955,
25.7350837209406));
#56914=CARTESIAN_POINT('Ctrl Pts',(-12.1614319318481,-31.0025071272885,
25.5380042683722));
#56915=CARTESIAN_POINT('Ctrl Pts',(-7.84143056492381,-31.0009607071424,
25.3409248158037));
#56916=CARTESIAN_POINT('Ctrl Pts',(-5.47206978357895,-34.6132375091107,
25.1438453632353));
#56917=CARTESIAN_POINT('Ctrl Pts',(-7.19447658949484,-38.5750210714917,
24.9467659106668));
#56918=CARTESIAN_POINT('Ctrl Pts',(-11.452158721554,-39.3061551663815,24.7496864580984));
#56919=CARTESIAN_POINT('Ctrl Pts',(-14.3975644482142,-36.1459337646356,
24.55260700553));
#56920=CARTESIAN_POINT('Ctrl Pts',(-13.3690105924863,-31.9501631360336,
24.3555275529615));
#56921=CARTESIAN_POINT('Ctrl Pts',(-9.29597334491533,-30.5104472674722,
24.1584481003931));
#56922=CARTESIAN_POINT('Ctrl Pts',(-5.8591458687229,-33.1278182960401,23.9613686478246));
#56923=CARTESIAN_POINT('Ctrl Pts',(-6.16429583209316,-37.4370290940937,
23.7642891952562));
#56924=CARTESIAN_POINT('Ctrl Pts',(-9.93566749903101,-39.5439628738029,
23.5672097426877));
#56925=CARTESIAN_POINT('Ctrl Pts',(-13.7651747002391,-37.544640789156,23.3701302901193));
#56926=CARTESIAN_POINT('Ctrl Pts',(-14.1921957626856,-33.245795919376,23.1730508375509));
#56927=CARTESIAN_POINT('Ctrl Pts',(-10.8308433473732,-30.532177644384,22.9759713849824));
#56928=CARTESIAN_POINT('Ctrl Pts',(-6.71868035938346,-31.8560091149627,
22.778891932414));
#56929=CARTESIAN_POINT('Ctrl Pts',(-5.57175683115357,-36.0209797778084,
22.5818124798456));
#56930=CARTESIAN_POINT('Ctrl Pts',(-8.42651641210876,-39.2633187387499,
22.3847330272771));
#56931=CARTESIAN_POINT('Ctrl Pts',(-12.7031903857762,-38.6530123195454,
22.1876535747087));
#56932=CARTESIAN_POINT('Ctrl Pts',(-14.5370646090343,-34.7415778597228,
21.9905741221402));
#56933=CARTESIAN_POINT('Ctrl Pts',(-12.2709167424762,-31.0636724703596,
21.7934946695718));
#56934=CARTESIAN_POINT('Ctrl Pts',(-7.95260307923342,-30.9429193855399,
21.5964152170033));
#56935=CARTESIAN_POINT('Ctrl Pts',(-5.48446641910354,-34.4884398853772,
21.3993357644349));
#56936=CARTESIAN_POINT('Ctrl Pts',(-7.09689484347499,-38.496243375118,21.2022563118664));
#56937=CARTESIAN_POINT('Ctrl Pts',(-11.3327805678125,-39.3445866522322,
21.005176859298));
#56938=CARTESIAN_POINT('Ctrl Pts',(-14.3642686835055,-36.2668449624488,
20.8080974067296));
#56939=CARTESIAN_POINT('Ctrl Pts',(-13.451885693753,-32.0442898400189,20.6110179541611));
#56940=CARTESIAN_POINT('Ctrl Pts',(-9.420127336544,-30.4927298096469,20.4139385015927));
#56941=CARTESIAN_POINT('Ctrl Pts',(-5.91238415362461,-33.0142673056043,
20.2168590490242));
#56942=CARTESIAN_POINT('Ctrl Pts',(-6.09850842991144,-37.3302578291269,
20.0197795964558));
#56943=CARTESIAN_POINT('Ctrl Pts',(-9.81030467465576,-39.5404570072207,
19.8227001438873));
#56944=CARTESIAN_POINT('Ctrl Pts',(-13.6935234820103,-37.6475697121639,
19.6256206913189));
#56945=CARTESIAN_POINT('Ctrl Pts',(-14.2390053153439,-33.3621431000591,
19.4285412387505));
#56946=CARTESIAN_POINT('Ctrl Pts',(-10.9538133395929,-30.5568081921163,
19.231461786182));
#56947=CARTESIAN_POINT('Ctrl Pts',(-6.80668576914744,-31.7666553194215,
19.0343823336136));
#56948=CARTESIAN_POINT('Ctrl Pts',(-5.54527031434392,-35.8984076614049,
18.8373028810451));
#56949=CARTESIAN_POINT('Ctrl Pts',(-8.30947161110702,-39.2182547120721,
18.6402234284767));
#56950=CARTESIAN_POINT('Ctrl Pts',(-12.6013605036371,-38.7262565575938,
18.4431439759083));
#56951=CARTESIAN_POINT('Ctrl Pts',(-14.5424645814622,-34.8667881105732,
18.2460645233398));
#56952=CARTESIAN_POINT('Ctrl Pts',(-12.3786786376218,-31.1280051768823,
18.0489850707714));
#56953=CARTESIAN_POINT('Ctrl Pts',(-8.06532175045426,-30.8876303121494,
17.8519056182029));
#56954=CARTESIAN_POINT('Ctrl Pts',(-5.50032810290316,-34.3647042818508,
17.6548261656345));
#56955=CARTESIAN_POINT('Ctrl Pts',(-7.00147280782552,-38.4134622068707,
17.457746713066));
#56956=CARTESIAN_POINT('Ctrl Pts',(-11.2124808715576,-39.3824004432543,
17.2606672604976));
#56957=CARTESIAN_POINT('Ctrl Pts',(-14.3275590045687,-36.3811790114449,
17.0635878079291));
#56958=CARTESIAN_POINT('Ctrl Pts',(-13.796029319407,-33.5643019726801,16.9322015062168));
#56959=CARTESIAN_POINT('Ctrl Pts',(-12.9953403345368,-32.5752112632643,
16.8665083553607));
#56960=CARTESIAN_POINT('Ctrl Pts',(-6.89794526934316,-32.3362693815221,
30.4037282431115));
#56961=CARTESIAN_POINT('Ctrl Pts',(-6.01767719231387,-33.3612758601103,
30.3379893529749));
#56962=CARTESIAN_POINT('Ctrl Pts',(-5.36815475683035,-36.3340720594079,
30.2065573119822));
#56963=CARTESIAN_POINT('Ctrl Pts',(-8.58246652790955,-39.6113579318683,
30.0094321201333));
#56964=CARTESIAN_POINT('Ctrl Pts',(-13.077575104318,-38.7102286635917,29.8123526675649));
#56965=CARTESIAN_POINT('Ctrl Pts',(-14.7912310493905,-34.4613873262902,
29.6152732149964));
#56966=CARTESIAN_POINT('Ctrl Pts',(-12.1753527356742,-30.69671662198,29.418193762428));
#56967=CARTESIAN_POINT('Ctrl Pts',(-7.59358093161996,-30.822090250394,29.2211143098595));
#56968=CARTESIAN_POINT('Ctrl Pts',(-5.18646805441968,-34.7222828219266,
29.0240348572911));
#56969=CARTESIAN_POINT('Ctrl Pts',(-7.12919151875231,-38.8737645578935,
28.8269554047226));
#56970=CARTESIAN_POINT('Ctrl Pts',(-11.6661975880609,-39.5244679154526,
28.6298759521542));
#56971=CARTESIAN_POINT('Ctrl Pts',(-14.6975006503904,-36.0866140858044,
28.4327964995858));
#56972=CARTESIAN_POINT('Ctrl Pts',(-13.4838026853514,-31.6667756323208,
28.2357170470173));
#56973=CARTESIAN_POINT('Ctrl Pts',(-9.12188544699834,-30.2591021081778,
28.0386375944489));
#56974=CARTESIAN_POINT('Ctrl Pts',(-5.55349718129253,-33.1356389443498,
27.8415581418804));
#56975=CARTESIAN_POINT('Ctrl Pts',(-6.00329242554367,-37.6969534306456,
27.644478689312));
#56976=CARTESIAN_POINT('Ctrl Pts',(-10.0648039552855,-39.8211017284068,
27.4473992367436));
#56977=CARTESIAN_POINT('Ctrl Pts',(-14.0677538223015,-37.5885526123103,
27.2503197841751));
#56978=CARTESIAN_POINT('Ctrl Pts',(-14.394785058227,-33.0167981320208,27.0532403316067));
#56979=CARTESIAN_POINT('Ctrl Pts',(-10.7503683488455,-30.2372096586735,
26.8561608790382));
#56980=CARTESIAN_POINT('Ctrl Pts',(-6.42786414891367,-31.7616253245286,
26.6590814264698));
#56981=CARTESIAN_POINT('Ctrl Pts',(-5.33340211585977,-36.2124723344077,
26.4620019739013));
#56982=CARTESIAN_POINT('Ctrl Pts',(-8.45601787883186,-39.5676409768508,
26.2649225213329));
#56983=CARTESIAN_POINT('Ctrl Pts',(-12.9738883587037,-38.7951565171297,
26.0678430687645));
#56984=CARTESIAN_POINT('Ctrl Pts',(-14.8043366811376,-34.5930921543075,
25.870763616196));
#56985=CARTESIAN_POINT('Ctrl Pts',(-12.2932363992487,-30.7587393679332,
25.6736841636276));
#56986=CARTESIAN_POINT('Ctrl Pts',(-7.70980065303747,-30.7570986468375,
25.4766047110591));
#56987=CARTESIAN_POINT('Ctrl Pts',(-5.19595586955329,-34.5896526701106,
25.2795252584907));
#56988=CARTESIAN_POINT('Ctrl Pts',(-7.02339531996559,-38.7930264323505,
25.0824458059222));
#56989=CARTESIAN_POINT('Ctrl Pts',(-11.5407115943303,-39.5687452021288,
24.8853663533538));
#56990=CARTESIAN_POINT('Ctrl Pts',(-14.6657286366932,-36.2158129902076,
24.6882869007854));
#56991=CARTESIAN_POINT('Ctrl Pts',(-13.5744534011479,-31.7641835927545,
24.4912074482169));
#56992=CARTESIAN_POINT('Ctrl Pts',(-9.25304168607287,-30.2366736185969,
24.2941279956485));
#56993=CARTESIAN_POINT('Ctrl Pts',(-5.60663591672545,-33.0136523541329,
24.09704854308));
#56994=CARTESIAN_POINT('Ctrl Pts',(-5.93039397402027,-37.5856395208455,
23.8999690905116));
#56995=CARTESIAN_POINT('Ctrl Pts',(-9.93174449275826,-39.8210544618584,
23.7028896379431));
#56996=CARTESIAN_POINT('Ctrl Pts',(-13.9947756600116,-37.6998133944084,
23.5058101853747));
#56997=CARTESIAN_POINT('Ctrl Pts',(-14.4478365356373,-33.1388242719455,
23.3087307328062));
#56998=CARTESIAN_POINT('Ctrl Pts',(-10.881508308541,-30.2597291173932,23.1116512802378));
#56999=CARTESIAN_POINT('Ctrl Pts',(-6.51858495909347,-31.664288044311,22.9145718276693));
#57000=CARTESIAN_POINT('Ctrl Pts',(-5.30172184934813,-36.0832392891341,
22.717492375101));
#57001=CARTESIAN_POINT('Ctrl Pts',(-8.33056512943833,-39.5232966022396,
22.5204129225325));
#57002=CARTESIAN_POINT('Ctrl Pts',(-12.8680313709721,-38.8757735992743,
22.3233334699641));
#57003=CARTESIAN_POINT('Ctrl Pts',(-14.8137355397931,-34.7258192359782,
22.1262540173956));
#57004=CARTESIAN_POINT('Ctrl Pts',(-12.4093976112665,-30.8236345834782,
21.9291745648272));
#57005=CARTESIAN_POINT('Ctrl Pts',(-7.82775248517904,-30.6955179560935,
21.7320951122587));
#57006=CARTESIAN_POINT('Ctrl Pts',(-5.2091084539092,-34.4572448671776,21.5350156596903));
#57007=CARTESIAN_POINT('Ctrl Pts',(-6.91986302335349,-38.709444859361,21.3379362071218));
#57008=CARTESIAN_POINT('Ctrl Pts',(-11.4140537415424,-39.6095202461779,
21.1408567545534));
#57009=CARTESIAN_POINT('Ctrl Pts',(-14.6304024908889,-36.3440973723417,
20.943777301985));
#57010=CARTESIAN_POINT('Ctrl Pts',(-13.6623822394406,-31.8640501583123,
20.7466978494165));
#57011=CARTESIAN_POINT('Ctrl Pts',(-9.38476660811169,-30.2178757473391,
20.5496183968481));
#57012=CARTESIAN_POINT('Ctrl Pts',(-5.66312068081691,-32.8931770060079,
20.3525389442796));
#57013=CARTESIAN_POINT('Ctrl Pts',(-5.86059484545545,-37.4723573269407,
20.1554594917112));
#57014=CARTESIAN_POINT('Ctrl Pts',(-9.79873702315724,-39.8173348069675,
19.9583800391427));
#57015=CARTESIAN_POINT('Ctrl Pts',(-13.9187551389525,-37.8090189397228,
19.7613005865743));
#57016=CARTESIAN_POINT('Ctrl Pts',(-14.4975005423574,-33.2622663224496,
19.5642211340059));
#57017=CARTESIAN_POINT('Ctrl Pts',(-11.0119770306961,-30.2858616398942,
19.3671416814374));
#57018=CARTESIAN_POINT('Ctrl Pts',(-6.61195695292212,-31.5694854399232,
19.170062228869));
#57019=CARTESIAN_POINT('Ctrl Pts',(-5.27362018047655,-35.9531927053267,
18.9729827763005));
#57020=CARTESIAN_POINT('Ctrl Pts',(-8.20638291761613,-39.4754845639552,
18.7759033237321));
#57021=CARTESIAN_POINT('Ctrl Pts',(-12.7599918862159,-38.9534842827584,
18.5788238711636));
#57022=CARTESIAN_POINT('Ctrl Pts',(-14.8194648034095,-34.8586648280961,
18.3817444185952));
#57023=CARTESIAN_POINT('Ctrl Pts',(-12.523730844138,-30.8918903088085,18.1846649660268));
#57024=CARTESIAN_POINT('Ctrl Pts',(-7.94734475912938,-30.6368573461008,
17.9875855134583));
#57025=CARTESIAN_POINT('Ctrl Pts',(-5.22593738574218,-34.325963846615,17.7905060608899));
#57026=CARTESIAN_POINT('Ctrl Pts',(-6.81862213659804,-38.6216156821384,
17.5934266083214));
#57027=CARTESIAN_POINT('Ctrl Pts',(-11.2864181504302,-39.6496399282681,
17.396347155753));
#57028=CARTESIAN_POINT('Ctrl Pts',(-14.5914542498167,-36.4654035300642,
17.1992677031845));
#57029=CARTESIAN_POINT('Ctrl Pts',(-14.0275117988269,-33.4767528756898,
17.0678814014722));
#57030=CARTESIAN_POINT('Ctrl Pts',(-13.177996670672,-32.4273472554761,17.0021882506161));
#57031=CARTESIAN_POINT('Ctrl Pts',(-7.42676557298524,-32.7934484719077,
30.));
#57032=CARTESIAN_POINT('Ctrl Pts',(-7.348473680774,-32.8679592071175,30.));
#57033=CARTESIAN_POINT('Ctrl Pts',(-7.27428894791241,-32.9462643748986,
30.));
#57034=CARTESIAN_POINT('Ctrl Pts',(-7.20420784983133,-33.0279214358029,
30.));
#57035=CARTESIAN_POINT('Ctrl Pts',(-7.13363401900521,-33.1101526188153,
30.));
#57036=CARTESIAN_POINT('Ctrl Pts',(-7.06722139480313,-33.1957835701515,
30.));
#57037=CARTESIAN_POINT('Ctrl Pts',(-7.00499327507605,-33.2844116565263,
30.));
#57038=CARTESIAN_POINT('Ctrl Pts',(-6.94120691731623,-33.3752590555778,
30.));
#57039=CARTESIAN_POINT('Ctrl Pts',(-6.88181677124198,-33.4692561008207,
30.));
#57040=CARTESIAN_POINT('Ctrl Pts',(-6.82688246489709,-33.5660125152163,
30.));
#57041=CARTESIAN_POINT('Ctrl Pts',(-6.77575465411374,-33.6560645059748,
30.));
#57042=CARTESIAN_POINT('Ctrl Pts',(-6.72848667230412,-33.748507616239,30.));
#57043=CARTESIAN_POINT('Ctrl Pts',(-6.68515790161883,-33.8430529558883,
30.));
#57044=CARTESIAN_POINT('Ctrl Pts',(-6.67815310128406,-33.8583377474102,
30.));
#57045=CARTESIAN_POINT('Ctrl Pts',(-6.67125055154478,-33.8736792804882,
30.));
#57046=CARTESIAN_POINT('Ctrl Pts',(-6.66445311748837,-33.8890708261453,
30.));
#57047=CARTESIAN_POINT('Ctrl Pts',(-6.61779557045972,-33.9947183042054,
30.));
#57048=CARTESIAN_POINT('Ctrl Pts',(-6.5762333697332,-34.1023850035639,30.));
#57049=CARTESIAN_POINT('Ctrl Pts',(-6.53979147597588,-34.2116192879216,
30.));
#57050=CARTESIAN_POINT('Ctrl Pts',(-6.50328868698427,-34.3210361052559,
30.));
#57051=CARTESIAN_POINT('Ctrl Pts',(-6.47192296745121,-34.4320265565667,
30.));
#57052=CARTESIAN_POINT('Ctrl Pts',(-6.44575876679422,-34.5441747920789,
30.));
#57053=CARTESIAN_POINT('Ctrl Pts',(-6.41958697740395,-34.6563555553591,
30.));
#57054=CARTESIAN_POINT('Ctrl Pts',(-6.39861935723561,-34.7696956037716,
30.));
#57055=CARTESIAN_POINT('Ctrl Pts',(-6.38296523648734,-34.8838044926981,
30.));
#57056=CARTESIAN_POINT('Ctrl Pts',(-6.36739851537545,-34.9972762921604,
30.));
#57057=CARTESIAN_POINT('Ctrl Pts',(-6.35708579723688,-35.1115092190907,
30.));
#57058=CARTESIAN_POINT('Ctrl Pts',(-6.3521840433183,-35.2261322552398,30.));
#57059=CARTESIAN_POINT('Ctrl Pts',(-6.35142083329213,-35.2439792242782,
30.));
#57060=CARTESIAN_POINT('Ctrl Pts',(-6.35078926352373,-35.2618281998695,
30.));
#57061=CARTESIAN_POINT('Ctrl Pts',(-6.35028981819732,-35.2796697579982,
30.));
#57062=CARTESIAN_POINT('Ctrl Pts',(-6.34696896251305,-35.3982998393995,
30.));
#57063=CARTESIAN_POINT('Ctrl Pts',(-6.34948085220682,-35.5167089537285,
30.));
#57064=CARTESIAN_POINT('Ctrl Pts',(-6.3578921072129,-35.6344688667497,30.));
#57065=CARTESIAN_POINT('Ctrl Pts',(-6.36625711786001,-35.7515813458642,
30.));
#57066=CARTESIAN_POINT('Ctrl Pts',(-6.38045650012585,-35.8680526311929,
30.));
#57067=CARTESIAN_POINT('Ctrl Pts',(-6.40060399470209,-35.9834785326489,
30.));
#57068=CARTESIAN_POINT('Ctrl Pts',(-6.40380951972359,-36.0018431294897,
30.));
#57069=CARTESIAN_POINT('Ctrl Pts',(-6.4071657188688,-36.0201812828735,30.));
#57070=CARTESIAN_POINT('Ctrl Pts',(-6.41067317161291,-36.0384913817355,
30.));
#57071=CARTESIAN_POINT('Ctrl Pts',(-6.43232735026095,-36.1515335752435,
30.));
#57072=CARTESIAN_POINT('Ctrl Pts',(-6.45974222332004,-36.2635067659136,
30.));
#57073=CARTESIAN_POINT('Ctrl Pts',(-6.49261646094871,-36.3741489668983,
30.));
#57074=CARTESIAN_POINT('Ctrl Pts',(-6.51335838631696,-36.4439584116473,
30.));
#57075=CARTESIAN_POINT('Ctrl Pts',(-6.5362747620185,-36.5132379695589,30.));
#57076=CARTESIAN_POINT('Ctrl Pts',(-6.56130037757764,-36.5819201363282,
30.));
#57077=CARTESIAN_POINT('Ctrl Pts',(-6.56744767501135,-36.5987912381209,
30.));
#57078=CARTESIAN_POINT('Ctrl Pts',(-6.57372227837194,-36.6156262842334,
30.));
#57079=CARTESIAN_POINT('Ctrl Pts',(-6.58012329087647,-36.632424253444,30.));
#57080=CARTESIAN_POINT('Ctrl Pts',(-6.58592196118508,-36.6476415155939,
30.));
#57081=CARTESIAN_POINT('Ctrl Pts',(-6.5918227230537,-36.6628239282595,30.));
#57082=CARTESIAN_POINT('Ctrl Pts',(-6.59782163563458,-36.6779632135072,
30.));
#57083=CARTESIAN_POINT('Ctrl Pts',(-6.64115230666265,-36.787315596931,30.));
#57084=CARTESIAN_POINT('Ctrl Pts',(-6.68964474891968,-36.8945375462831,
30.));
#57085=CARTESIAN_POINT('Ctrl Pts',(-6.74293042168715,-36.9993679579068,
30.));
#57086=CARTESIAN_POINT('Ctrl Pts',(-6.79720023807432,-37.1061345031175,
30.));
#57087=CARTESIAN_POINT('Ctrl Pts',(-6.8564422422142,-37.2104210176384,30.));
#57088=CARTESIAN_POINT('Ctrl Pts',(-6.92032223600451,-37.3119481519295,
30.));
#57089=CARTESIAN_POINT('Ctrl Pts',(-6.98529990584252,-37.4152198684739,
30.));
#57090=CARTESIAN_POINT('Ctrl Pts',(-7.05507665614285,-37.5156373235829,
30.));
#57091=CARTESIAN_POINT('Ctrl Pts',(-7.12935272067387,-37.6128920097048,
30.));
#57092=CARTESIAN_POINT('Ctrl Pts',(-7.18304873196466,-37.6831998370926,
30.));
#57093=CARTESIAN_POINT('Ctrl Pts',(-7.23909729085682,-37.7518544742134,
30.));
#57094=CARTESIAN_POINT('Ctrl Pts',(-7.2974000200836,-37.8187312516186,30.));
#57095=CARTESIAN_POINT('Ctrl Pts',(-7.3176529320871,-37.8419625738196,30.));
#57096=CARTESIAN_POINT('Ctrl Pts',(-7.33817775201689,-37.8649790685653,
30.));
#57097=CARTESIAN_POINT('Ctrl Pts',(-7.35897141037825,-37.8877760628998,
30.));
#57098=CARTESIAN_POINT('Ctrl Pts',(-7.37199172460619,-37.9020508011171,
30.));
#57099=CARTESIAN_POINT('Ctrl Pts',(-7.38511665917092,-37.9162385040998,
30.));
#57100=CARTESIAN_POINT('Ctrl Pts',(-7.3983354919303,-37.9303276817975,30.));
#57101=CARTESIAN_POINT('Ctrl Pts',(-7.48411062168129,-38.0217503563337,
30.));
#57102=CARTESIAN_POINT('Ctrl Pts',(-7.57393021067795,-38.1091313263961,
30.));
#57103=CARTESIAN_POINT('Ctrl Pts',(-7.66746004992797,-38.1921567632245,
30.));
#57104=CARTESIAN_POINT('Ctrl Pts',(-7.73941550489948,-38.2560308501373,
30.));
#57105=CARTESIAN_POINT('Ctrl Pts',(-7.81356806356869,-38.3173268123056,
30.));
#57106=CARTESIAN_POINT('Ctrl Pts',(-7.88978351495984,-38.3758912604165,
30.));
#57107=CARTESIAN_POINT('Ctrl Pts',(-7.92789124065542,-38.405173484472,30.));
#57108=CARTESIAN_POINT('Ctrl Pts',(-7.96651491739015,-38.4337726638739,
30.));
#57109=CARTESIAN_POINT('Ctrl Pts',(-8.00563904546686,-38.4616684950285,
30.));
#57110=CARTESIAN_POINT('Ctrl Pts',(-8.02949698067293,-38.4786794027451,
30.));
#57111=CARTESIAN_POINT('Ctrl Pts',(-8.05354236869358,-38.4954296697472,
30.));
#57112=CARTESIAN_POINT('Ctrl Pts',(-8.07776857551838,-38.5119122904479,
30.));
#57113=CARTESIAN_POINT('Ctrl Pts',(-8.09327041768187,-38.5224591740931,
30.));
#57114=CARTESIAN_POINT('Ctrl Pts',(-8.1088447591175,-38.5328953980027,30.));
#57115=CARTESIAN_POINT('Ctrl Pts',(-8.12448498934949,-38.5432161517883,
30.));
#57116=CARTESIAN_POINT('Ctrl Pts',(-8.2313653964011,-38.613744932332,30.));
#57117=CARTESIAN_POINT('Ctrl Pts',(-8.34138274960732,-38.6789276717489,
30.));
#57118=CARTESIAN_POINT('Ctrl Pts',(-8.45421422908593,-38.7384194582944,
30.));
#57119=CARTESIAN_POINT('Ctrl Pts',(-8.56704570856451,-38.7979112448399,
30.));
#57120=CARTESIAN_POINT('Ctrl Pts',(-8.68269189967889,-38.8517129044718,
30.));
#57121=CARTESIAN_POINT('Ctrl Pts',(-8.80086736442083,-38.8994392928682,
30.));
#57122=CARTESIAN_POINT('Ctrl Pts',(-8.84648289711551,-38.9178615993515,
30.));
#57123=CARTESIAN_POINT('Ctrl Pts',(-8.89247562661289,-38.9353782311179,
30.));
#57124=CARTESIAN_POINT('Ctrl Pts',(-8.93882090860579,-38.9519961826432,
30.));
#57125=CARTESIAN_POINT('Ctrl Pts',(-11.0588859861567,-38.9492994180788,
29.9978117181351));
#57126=CARTESIAN_POINT('Ctrl Pts',(-12.3629833263098,-38.5996448966335,
29.932118567279));
#57127=CARTESIAN_POINT('Ctrl Pts',(-14.5759069292524,-36.5132512939394,
29.8007322655667));
#57128=CARTESIAN_POINT('Ctrl Pts',(-13.7737241750814,-31.9945004802153,
29.6036528129982));
#57129=CARTESIAN_POINT('Ctrl Pts',(-9.55494350084833,-30.2000838007241,
29.4065733604298));
#57130=CARTESIAN_POINT('Ctrl Pts',(-5.74151352522334,-32.7391832451362,
29.2094939078613));
#57131=CARTESIAN_POINT('Ctrl Pts',(-5.77477598136472,-37.3233360369277,
29.0124144552929));
#57132=CARTESIAN_POINT('Ctrl Pts',(-9.62705482091557,-39.8069425790181,
28.8153350027244));
#57133=CARTESIAN_POINT('Ctrl Pts',(-13.8159543550122,-37.9471529628393,
28.618255550156));
#57134=CARTESIAN_POINT('Ctrl Pts',(-14.5566802618819,-33.4238465177708,
28.4211760975876));
#57135=CARTESIAN_POINT('Ctrl Pts',(-11.1795571712635,-30.3249950720552,
28.2240966450191));
#57136=CARTESIAN_POINT('Ctrl Pts',(-6.73655089324582,-31.4507544203241,
28.0270171924506));
#57137=CARTESIAN_POINT('Ctrl Pts',(-5.24260955293931,-35.7839028674565,
27.8299377398823));
#57138=CARTESIAN_POINT('Ctrl Pts',(-8.04780553591408,-39.4086433897224,
27.6328582873138));
#57139=CARTESIAN_POINT('Ctrl Pts',(-12.617140242138,-39.0494207196498,27.4357788347454));
#57140=CARTESIAN_POINT('Ctrl Pts',(-14.8214395921059,-35.0308424199595,
27.2386993821769));
#57141=CARTESIAN_POINT('Ctrl Pts',(-12.6687332871507,-30.9843947121075,
27.0416199296085));
#57142=CARTESIAN_POINT('Ctrl Pts',(-8.10436598692081,-30.5667394360589,
26.84454047704));
#57143=CARTESIAN_POINT('Ctrl Pts',(-5.25303126404637,-34.1553018695318,
26.6474610244716));
#57144=CARTESIAN_POINT('Ctrl Pts',(-6.69140349521391,-38.5071948075579,
26.4503815719031));
#57145=CARTESIAN_POINT('Ctrl Pts',(-11.1196644450027,-39.6897311610149,
26.2533021193347));
#57146=CARTESIAN_POINT('Ctrl Pts',(-14.5361150902314,-36.6342847416972,
26.0562226667663));
#57147=CARTESIAN_POINT('Ctrl Pts',(-13.8534016741551,-32.1019796107692,
25.8591432141978));
#57148=CARTESIAN_POINT('Ctrl Pts',(-9.68847381165508,-30.1885367975724,
25.6620637616294));
#57149=CARTESIAN_POINT('Ctrl Pts',(-5.80506369999907,-32.6230826404,25.4649843090609));
#57150=CARTESIAN_POINT('Ctrl Pts',(-5.7125036185332,-37.205584155207,25.2679048564925));
#57151=CARTESIAN_POINT('Ctrl Pts',(-9.49443759462431,-39.794959160471,25.070825403924));
#57152=CARTESIAN_POINT('Ctrl Pts',(-13.7332345894671,-38.0512597715136,
24.8737459513556));
#57153=CARTESIAN_POINT('Ctrl Pts',(-14.598408855951,-33.550219780088,24.6766664987872));
#57154=CARTESIAN_POINT('Ctrl Pts',(-11.3081259026265,-30.3593068064588,
24.4795870462187));
#57155=CARTESIAN_POINT('Ctrl Pts',(-6.83572509125078,-31.3620622606893,
24.2825075936503));
#57156=CARTESIAN_POINT('Ctrl Pts',(-5.22279359367999,-35.6523232669585,
24.0854281410818));
#57157=CARTESIAN_POINT('Ctrl Pts',(-7.92689380738031,-39.3530974498007,
23.8883486885134));
#57158=CARTESIAN_POINT('Ctrl Pts',(-12.5044037951801,-39.1200956692727,
23.6912692359449));
#57159=CARTESIAN_POINT('Ctrl Pts',(-14.8187520767123,-35.1638753076392,
23.4941897833765));
#57160=CARTESIAN_POINT('Ctrl Pts',(-12.7785249527297,-31.0595652802824,
23.2971103308081));
#57161=CARTESIAN_POINT('Ctrl Pts',(-8.2274202757673,-30.5161191123635,23.1000308782396));
#57162=CARTESIAN_POINT('Ctrl Pts',(-5.27814776377262,-34.0246343493302,
22.9029514256712));
#57163=CARTESIAN_POINT('Ctrl Pts',(-6.59588490261864,-38.4145610401807,
22.7058719731027));
#57164=CARTESIAN_POINT('Ctrl Pts',(-10.989828421184,-39.7188416364419,22.5087925205343));
#57165=CARTESIAN_POINT('Ctrl Pts',(-14.4892908728541,-36.7588331791699,
22.3117130679658));
#57166=CARTESIAN_POINT('Ctrl Pts',(-13.9319030629373,-32.2094149363679,
22.1146336153974));
#57167=CARTESIAN_POINT('Ctrl Pts',(-9.8213612200649,-30.1817726414334,21.917554162829));
#57168=CARTESIAN_POINT('Ctrl Pts',(-5.8722503921224,-32.5082315781925,21.7204747102605));
#57169=CARTESIAN_POINT('Ctrl Pts',(-5.65327480142373,-37.0864339779578,
21.5233952576921));
#57170=CARTESIAN_POINT('Ctrl Pts',(-9.36231674438557,-39.7791826447939,
21.3263158051236));
#57171=CARTESIAN_POINT('Ctrl Pts',(-13.6476157286711,-38.1531137295354,
21.1292363525552));
#57172=CARTESIAN_POINT('Ctrl Pts',(-14.6366634274731,-33.6776615506337,
20.9321568999867));
#57173=CARTESIAN_POINT('Ctrl Pts',(-11.4356842831145,-30.3971707311702,
20.7350774474183));
#57174=CARTESIAN_POINT('Ctrl Pts',(-6.9373162471913,-31.2761317210392,20.5379979948499));
#57175=CARTESIAN_POINT('Ctrl Pts',(-5.20661233371697,-35.5202513937734,
20.3409185422814));
#57176=CARTESIAN_POINT('Ctrl Pts',(-7.80756274108455,-39.294233938127,20.143839089713));
#57177=CARTESIAN_POINT('Ctrl Pts',(-12.38975907867,-39.1876340166796,19.9467596371445));
#57178=CARTESIAN_POINT('Ctrl Pts',(-14.8123952029925,-35.2967826638352,
19.7496801845761));
#57179=CARTESIAN_POINT('Ctrl Pts',(-12.8862001060391,-31.1377374333175,
19.5526007320077));
#57180=CARTESIAN_POINT('Ctrl Pts',(-8.35182504074954,-30.4689129009811,
19.3555212794392));
#57181=CARTESIAN_POINT('Ctrl Pts',(-5.30685954432354,-33.8947109540756,
19.1584418268708));
#57182=CARTESIAN_POINT('Ctrl Pts',(-6.50296040670598,-38.3193243056809,
18.9613623743023));
#57183=CARTESIAN_POINT('Ctrl Pts',(-10.8592354868165,-39.7443631764007,
18.7642829217339));
#57184=CARTESIAN_POINT('Ctrl Pts',(-14.4390537541248,-36.8820324187471,
18.5672034691654));
#57185=CARTESIAN_POINT('Ctrl Pts',(-14.0073978409461,-32.3189948263819,
18.370124016597));
#57186=CARTESIAN_POINT('Ctrl Pts',(-9.95440880910246,-30.1786395849428,
18.1730445640285));
#57187=CARTESIAN_POINT('Ctrl Pts',(-5.94253267211965,-32.3953547057049,
17.9759651114601));
#57188=CARTESIAN_POINT('Ctrl Pts',(-5.59745211347252,-36.9655424623781,
17.7788856588917));
#57189=CARTESIAN_POINT('Ctrl Pts',(-9.23049091074666,-39.7600697589106,
17.5818062063232));
#57190=CARTESIAN_POINT('Ctrl Pts',(-13.5595986838708,-38.2519619715973,
17.3847267537548));
#57191=CARTESIAN_POINT('Ctrl Pts',(-14.6706288037252,-33.8073150519438,
17.1876473011863));
#57192=CARTESIAN_POINT('Ctrl Pts',(-11.5636788830593,-30.4361277555464,
16.9905678486179));
#57193=CARTESIAN_POINT('Ctrl Pts',(-7.03690775456509,-31.1981823891181,
16.7934426556376));
#57194=CARTESIAN_POINT('Ctrl Pts',(-5.81501521204634,-33.9850050967667,
16.6620106135137));
#57195=CARTESIAN_POINT('Ctrl Pts',(-5.92468338351297,-35.3316613902157,
16.5962717222458));
#57196=CARTESIAN_POINT('Ctrl Pts',(-10.9980261717899,-38.7223121573106,
30.1334916522396));
#57197=CARTESIAN_POINT('Ctrl Pts',(-12.2271700957341,-38.3927541425204,
30.0677985013834));
#57198=CARTESIAN_POINT('Ctrl Pts',(-14.3129051992123,-36.4262766866223,
29.9364121996711));
#57199=CARTESIAN_POINT('Ctrl Pts',(-13.5568281581637,-32.1672425367211,
29.7393327471027));
#57200=CARTESIAN_POINT('Ctrl Pts',(-9.58052326701321,-30.4759605359757,
29.5422532945342));
#57201=CARTESIAN_POINT('Ctrl Pts',(-5.986271412028,-32.8691244189901,29.3451738419658));
#57202=CARTESIAN_POINT('Ctrl Pts',(-6.01762209774973,-37.1898015471262,
29.1480943893974));
#57203=CARTESIAN_POINT('Ctrl Pts',(-9.6484899656477,-39.5306620003194,28.9510149368289));
#57204=CARTESIAN_POINT('Ctrl Pts',(-13.5966311448511,-37.7777643935561,
28.7539354842605));
#57205=CARTESIAN_POINT('Ctrl Pts',(-14.2947835907645,-33.5144364486947,
28.5568560316921));
#57206=CARTESIAN_POINT('Ctrl Pts',(-11.1117617415225,-30.5936924916062,
28.3597765791236));
#57207=CARTESIAN_POINT('Ctrl Pts',(-6.9241186856516,-31.6547484574022,28.1626971265552));
#57208=CARTESIAN_POINT('Ctrl Pts',(-5.51604210683472,-35.7388477967325,
27.9656176739867));
#57209=CARTESIAN_POINT('Ctrl Pts',(-8.16000854383523,-39.1552551856891,
27.7685382214183));
#57210=CARTESIAN_POINT('Ctrl Pts',(-12.4667192606622,-38.816678954707,27.5714587688498));
#57211=CARTESIAN_POINT('Ctrl Pts',(-14.5443257928935,-35.0290697419017,
27.3743793162814));
#57212=CARTESIAN_POINT('Ctrl Pts',(-12.5153469787341,-31.2151929241783,
27.177299863713));
#57213=CARTESIAN_POINT('Ctrl Pts',(-8.2133181646357,-30.8215425201386,26.9802204111445));
#57214=CARTESIAN_POINT('Ctrl Pts',(-5.52586482672684,-34.2038511676513,
26.7831409585761));
#57215=CARTESIAN_POINT('Ctrl Pts',(-6.88156614891665,-38.3056176522011,
26.5860615060077));
#57216=CARTESIAN_POINT('Ctrl Pts',(-11.0553113690653,-39.4201873464575,
26.3889820534392));
#57217=CARTESIAN_POINT('Ctrl Pts',(-14.2754004090027,-36.540353697843,26.1919026008708));
#57218=CARTESIAN_POINT('Ctrl Pts',(-13.6319261672203,-32.2685442695009,
25.9948231483023));
#57219=CARTESIAN_POINT('Ctrl Pts',(-9.70637888003917,-30.465077200563,25.7977436957339));
#57220=CARTESIAN_POINT('Ctrl Pts',(-6.04616901996426,-32.7596967340437,
25.6006642431654));
#57221=CARTESIAN_POINT('Ctrl Pts',(-5.9589288591031,-37.0788174928738,25.403584790597));
#57222=CARTESIAN_POINT('Ctrl Pts',(-9.52349495730953,-39.5193673326274,
25.2065053380285));
#57223=CARTESIAN_POINT('Ctrl Pts',(-13.5186657245719,-37.8758876297465,
25.0094258854601));
#57224=CARTESIAN_POINT('Ctrl Pts',(-14.3341138203995,-33.6335463669068,
24.8123464328917));
#57225=CARTESIAN_POINT('Ctrl Pts',(-11.2329409434872,-30.6260321479827,
24.6152669803232));
#57226=CARTESIAN_POINT('Ctrl Pts',(-7.01759281456559,-31.5711539083146,
24.4181875277548));
#57227=CARTESIAN_POINT('Ctrl Pts',(-5.49736507623987,-35.6148307763096,
24.2211080751863));
#57228=CARTESIAN_POINT('Ctrl Pts',(-8.04604625598683,-39.1029017666212,
24.0240286226179));
#57229=CARTESIAN_POINT('Ctrl Pts',(-12.3604623774382,-38.8832918387528,
23.8269491700494));
#57230=CARTESIAN_POINT('Ctrl Pts',(-14.5417927433158,-35.1544565213557,
23.629869717481));
#57231=CARTESIAN_POINT('Ctrl Pts',(-12.6188283328409,-31.2860430396466,
23.4327902649126));
#57232=CARTESIAN_POINT('Ctrl Pts',(-8.32929986845024,-30.7738316159119,
23.2357108123441));
#57233=CARTESIAN_POINT('Ctrl Pts',(-5.54953774751175,-34.0806938054149,
23.0386313597757));
#57234=CARTESIAN_POINT('Ctrl Pts',(-6.79153751830967,-38.2183080405503,
22.8415519072072));
#57235=CARTESIAN_POINT('Ctrl Pts',(-10.9329377126885,-39.4476246878987,
22.6444724546388));
#57236=CARTESIAN_POINT('Ctrl Pts',(-14.2312674286564,-36.6577436736085,
22.4473930020703));
#57237=CARTESIAN_POINT('Ctrl Pts',(-13.7059156633048,-32.3698047150298,
22.2503135495019));
#57238=CARTESIAN_POINT('Ctrl Pts',(-9.83162854169131,-30.4587018164847,
22.0532340969334));
#57239=CARTESIAN_POINT('Ctrl Pts',(-6.10949413523795,-32.651446773765,21.856154644365));
#57240=CARTESIAN_POINT('Ctrl Pts',(-5.90310423740425,-36.9665155105805,
21.6590751917966));
#57241=CARTESIAN_POINT('Ctrl Pts',(-9.39896779564977,-39.5044975772889,
21.4619957392281));
#57242=CARTESIAN_POINT('Ctrl Pts',(-13.4379678354787,-37.971887498604,21.2649162866597));
#57243=CARTESIAN_POINT('Ctrl Pts',(-14.3701696980567,-33.7536633804914,
21.0678368340912));
#57244=CARTESIAN_POINT('Ctrl Pts',(-11.35316786482,-30.6617198313809,20.8707573815228));
#57245=CARTESIAN_POINT('Ctrl Pts',(-7.11334498597645,-31.4901622542101,
20.6736779289544));
#57246=CARTESIAN_POINT('Ctrl Pts',(-5.48211383942423,-35.4903497767315,
20.4765984763859));
#57247=CARTESIAN_POINT('Ctrl Pts',(-7.93357378130328,-39.0474214543101,
20.2795190238175));
#57248=CARTESIAN_POINT('Ctrl Pts',(-12.2524069030715,-38.946948397809,20.082439571249));
#57249=CARTESIAN_POINT('Ctrl Pts',(-14.5358012329681,-35.2797249842885,
19.8853601186806));
#57250=CARTESIAN_POINT('Ctrl Pts',(-12.720314821905,-31.3597222229148,19.6882806661121));
#57251=CARTESIAN_POINT('Ctrl Pts',(-8.44655442934804,-30.7293385967893,
19.4912012135437));
#57252=CARTESIAN_POINT('Ctrl Pts',(-5.57659930919367,-33.9582377993036,
19.2941217609752));
#57253=CARTESIAN_POINT('Ctrl Pts',(-6.70395388783986,-38.1285450681538,
19.0970423084068));
#57254=CARTESIAN_POINT('Ctrl Pts',(-10.8098506494414,-39.4716793690978,
18.8999628558384));
#57255=CARTESIAN_POINT('Ctrl Pts',(-14.1839177045665,-36.7738619970635,
18.7028834032699));
#57256=CARTESIAN_POINT('Ctrl Pts',(-13.7770713545418,-32.4730864654405,
18.5058039507015));
#57257=CARTESIAN_POINT('Ctrl Pts',(-9.95702917753784,-30.4557488334288,
18.3087244981331));
#57258=CARTESIAN_POINT('Ctrl Pts',(-6.17573691847179,-32.5450575360141,
18.1116450455646));
#57259=CARTESIAN_POINT('Ctrl Pts',(-5.85048997648918,-36.8525722739401,
17.9145655929962));
#57260=CARTESIAN_POINT('Ctrl Pts',(-9.27471869441539,-39.4864832107005,
17.7174861404277));
#57261=CARTESIAN_POINT('Ctrl Pts',(-13.3550095987821,-38.0650544059981,
17.5204066878593));
#57262=CARTESIAN_POINT('Ctrl Pts',(-14.4021829033284,-33.8758650048999,
17.3233272352908));
#57263=CARTESIAN_POINT('Ctrl Pts',(-11.4738059337554,-30.6984377881871,
17.1262477827224));
#57264=CARTESIAN_POINT('Ctrl Pts',(-7.20721243926833,-31.4166930853403,
16.9291225897422));
#57265=CARTESIAN_POINT('Ctrl Pts',(-6.05554856563953,-34.0433422569536,
16.7976905476182));
#57266=CARTESIAN_POINT('Ctrl Pts',(-6.15891352349801,-35.3125990445948,
16.7319516563503));
#57267=CARTESIAN_POINT('Ctrl Pts',(-10.9371663574229,-38.4953248965424,
30.2691715863441));
#57268=CARTESIAN_POINT('Ctrl Pts',(-12.0913568651584,-38.1858633884072,
30.2034784354879));
#57269=CARTESIAN_POINT('Ctrl Pts',(-14.0499034691722,-36.3393020793051,
30.0720921337757));
#57270=CARTESIAN_POINT('Ctrl Pts',(-13.3399321412461,-32.3399845932268,
29.8750126812072));
#57271=CARTESIAN_POINT('Ctrl Pts',(-9.60610303317808,-30.7518372712273,
29.6779332286388));
#57272=CARTESIAN_POINT('Ctrl Pts',(-6.23102929883268,-32.9990655928438,
29.4808537760703));
#57273=CARTESIAN_POINT('Ctrl Pts',(-6.26046821413472,-37.0562670573248,
29.2837743235019));
#57274=CARTESIAN_POINT('Ctrl Pts',(-9.66992511037984,-39.2543814216206,
29.0866948709334));
#57275=CARTESIAN_POINT('Ctrl Pts',(-13.3773079346899,-37.6083758242728,
28.889615418365));
#57276=CARTESIAN_POINT('Ctrl Pts',(-14.032886919647,-33.6050263796185,28.6925359657965));
#57277=CARTESIAN_POINT('Ctrl Pts',(-11.0439663117815,-30.8623899111572,
28.4954565132281));
#57278=CARTESIAN_POINT('Ctrl Pts',(-7.11168647805739,-31.8587424944803,
28.2983770606597));
#57279=CARTESIAN_POINT('Ctrl Pts',(-5.78947466073016,-35.6937927260083,
28.1012976080912));
#57280=CARTESIAN_POINT('Ctrl Pts',(-8.27221155175637,-38.9018669816557,
27.9042181555228));
#57281=CARTESIAN_POINT('Ctrl Pts',(-12.3162982791864,-38.5839371897643,
27.7071387029544));
#57282=CARTESIAN_POINT('Ctrl Pts',(-14.267211993681,-35.0272970638439,27.5100592503859));
#57283=CARTESIAN_POINT('Ctrl Pts',(-12.3619606703174,-31.4459911362492,
27.3129797978175));
#57284=CARTESIAN_POINT('Ctrl Pts',(-8.32227034235058,-31.0763456042183,
27.115900345249));
#57285=CARTESIAN_POINT('Ctrl Pts',(-5.7986983894073,-34.2524004657706,26.9188208926806));
#57286=CARTESIAN_POINT('Ctrl Pts',(-7.07172880261939,-38.1040404968445,
26.7217414401122));
#57287=CARTESIAN_POINT('Ctrl Pts',(-10.990958293128,-39.1506435319003,26.5246619875437));
#57288=CARTESIAN_POINT('Ctrl Pts',(-14.0146857277741,-36.4464226539888,
26.3275825349753));
#57289=CARTESIAN_POINT('Ctrl Pts',(-13.4104506602856,-32.4351089282327,
26.1305030824068));
#57290=CARTESIAN_POINT('Ctrl Pts',(-9.72428394842326,-30.7416176035536,
25.9334236298383));
#57291=CARTESIAN_POINT('Ctrl Pts',(-6.28727433992944,-32.8963108276873,
25.7363441772699));
#57292=CARTESIAN_POINT('Ctrl Pts',(-6.205354099673,-36.9520508305407,25.5392647247015));
#57293=CARTESIAN_POINT('Ctrl Pts',(-9.55255231999473,-39.2437755047836,
25.342185272133));
#57294=CARTESIAN_POINT('Ctrl Pts',(-13.3040968596768,-37.7005154879794,
25.1451058195646));
#57295=CARTESIAN_POINT('Ctrl Pts',(-14.0698187848481,-33.7168729537256,
24.9480263669962));
#57296=CARTESIAN_POINT('Ctrl Pts',(-11.1577559843479,-30.8927574895067,
24.7509469144277));
#57297=CARTESIAN_POINT('Ctrl Pts',(-7.1994605378804,-31.7802455559398,24.5538674618593));
#57298=CARTESIAN_POINT('Ctrl Pts',(-5.77193655879976,-35.5773382856607,
24.3567880092908));
#57299=CARTESIAN_POINT('Ctrl Pts',(-8.1651987045933,-38.8527060834415,24.1597085567224));
#57300=CARTESIAN_POINT('Ctrl Pts',(-12.2165209596964,-38.6464880082329,
23.9626291041539));
#57301=CARTESIAN_POINT('Ctrl Pts',(-14.2648334099194,-35.1450377350721,
23.7655496515855));
#57302=CARTESIAN_POINT('Ctrl Pts',(-12.4591317129521,-31.5125207990106,
23.5684701990171));
#57303=CARTESIAN_POINT('Ctrl Pts',(-8.43117946113315,-31.0315441194603,
23.3713907464486));
#57304=CARTESIAN_POINT('Ctrl Pts',(-5.82092773125088,-34.1367532614996,
23.1743112938802));
#57305=CARTESIAN_POINT('Ctrl Pts',(-6.98719013400071,-38.02205504092,22.9772318413117));
#57306=CARTESIAN_POINT('Ctrl Pts',(-10.8760470041931,-39.1764077393554,
22.7801523887433));
#57307=CARTESIAN_POINT('Ctrl Pts',(-13.9732439844587,-36.5566541680469,
22.5830729361748));
#57308=CARTESIAN_POINT('Ctrl Pts',(-13.4799282636722,-32.5301944936914,
22.3859934836064));
#57309=CARTESIAN_POINT('Ctrl Pts',(-9.84189586331774,-30.7356309915362,
22.188914031038));
#57310=CARTESIAN_POINT('Ctrl Pts',(-6.34673787835349,-32.7946619693375,
21.9918345784695));
#57311=CARTESIAN_POINT('Ctrl Pts',(-6.15293367338478,-36.8465970432031,
21.7947551259011));
#57312=CARTESIAN_POINT('Ctrl Pts',(-9.43561884691396,-39.2298125097838,
21.5976756733326));
#57313=CARTESIAN_POINT('Ctrl Pts',(-13.2283199422864,-37.7906612676727,
21.4005962207642));
#57314=CARTESIAN_POINT('Ctrl Pts',(-14.1036759686402,-33.8296652103491,
21.2035167681957));
#57315=CARTESIAN_POINT('Ctrl Pts',(-11.2706514465257,-30.9262689315915,
21.0064373156273));
#57316=CARTESIAN_POINT('Ctrl Pts',(-7.28937372476156,-31.7041927873809,
20.8093578630588));
#57317=CARTESIAN_POINT('Ctrl Pts',(-5.75761534513151,-35.4604481596895,
20.6122784104904));
#57318=CARTESIAN_POINT('Ctrl Pts',(-8.05958482152201,-38.800608970493,20.415198957922));
#57319=CARTESIAN_POINT('Ctrl Pts',(-12.1150547274729,-38.7062627789383,
20.2181195053535));
#57320=CARTESIAN_POINT('Ctrl Pts',(-14.2592072629438,-35.2626673047419,
20.0210400527851));
#57321=CARTESIAN_POINT('Ctrl Pts',(-12.5544295377709,-31.581707012512,19.8239606002167));
#57322=CARTESIAN_POINT('Ctrl Pts',(-8.54128381794652,-30.9897642925976,
19.6268811476482));
#57323=CARTESIAN_POINT('Ctrl Pts',(-5.8463390740638,-34.0217646445317,19.4298016950797));
#57324=CARTESIAN_POINT('Ctrl Pts',(-6.90494736897375,-37.9377658306266,
19.2327222425113));
#57325=CARTESIAN_POINT('Ctrl Pts',(-10.7604658120663,-39.198995561795,19.0356427899429));
#57326=CARTESIAN_POINT('Ctrl Pts',(-13.9287816550082,-36.6656915753799,
18.8385633373744));
#57327=CARTESIAN_POINT('Ctrl Pts',(-13.5467448681375,-32.6271781044991,
18.641483884806));
#57328=CARTESIAN_POINT('Ctrl Pts',(-9.95964954597322,-30.7328580819148,
18.4444044322375));
#57329=CARTESIAN_POINT('Ctrl Pts',(-6.40894116482391,-32.6947603663233,
18.2473249796691));
#57330=CARTESIAN_POINT('Ctrl Pts',(-6.10352783950584,-36.739602085502,18.0502455271006));
#57331=CARTESIAN_POINT('Ctrl Pts',(-9.31894647808413,-39.2128966624903,
17.8531660745322));
#57332=CARTESIAN_POINT('Ctrl Pts',(-13.1504205136935,-37.878146840399,17.6560866219638));
#57333=CARTESIAN_POINT('Ctrl Pts',(-14.1337370029317,-33.944414957856,17.4590071693953));
#57334=CARTESIAN_POINT('Ctrl Pts',(-11.3839329844517,-30.9607478208279,
17.2619277168269));
#57335=CARTESIAN_POINT('Ctrl Pts',(-7.37751712397162,-31.6352037815626,
17.0648025238468));
#57336=CARTESIAN_POINT('Ctrl Pts',(-6.29608191923271,-34.1016794171405,
16.9333704817227));
#57337=CARTESIAN_POINT('Ctrl Pts',(-6.39314366348305,-35.293536698974,16.8676315904548));
#57338=CARTESIAN_POINT('Ctrl Pts',(-10.876306543056,-38.2683376357742,30.4048515204486));
#57339=CARTESIAN_POINT('Ctrl Pts',(-11.9555436345827,-37.978972634294,30.3391583695924));
#57340=CARTESIAN_POINT('Ctrl Pts',(-13.7869017391321,-36.2523274719879,
30.2077720678801));
#57341=CARTESIAN_POINT('Ctrl Pts',(-13.1230361243285,-32.5127266497326,
30.0106926153117));
#57342=CARTESIAN_POINT('Ctrl Pts',(-9.63168279934295,-31.0277140064789,
29.8136131627432));
#57343=CARTESIAN_POINT('Ctrl Pts',(-6.47578718563735,-33.1290067666977,
29.6165337101748));
#57344=CARTESIAN_POINT('Ctrl Pts',(-6.50331433051971,-36.9227325675234,
29.4194542576064));
#57345=CARTESIAN_POINT('Ctrl Pts',(-9.69136025511198,-38.9781008429219,
29.2223748050379));
#57346=CARTESIAN_POINT('Ctrl Pts',(-13.1579847245288,-37.4389872549895,
29.0252953524695));
#57347=CARTESIAN_POINT('Ctrl Pts',(-13.7709902485295,-33.6956163105424,
28.8282158999011));
#57348=CARTESIAN_POINT('Ctrl Pts',(-10.9761708820405,-31.1310873307082,
28.6311364473326));
#57349=CARTESIAN_POINT('Ctrl Pts',(-7.29925427046318,-32.0627365315584,
28.4340569947642));
#57350=CARTESIAN_POINT('Ctrl Pts',(-6.06290721462558,-35.6487376552842,
28.2369775421957));
#57351=CARTESIAN_POINT('Ctrl Pts',(-8.38441455967752,-38.6484787776224,
28.0398980896273));
#57352=CARTESIAN_POINT('Ctrl Pts',(-12.1658772977107,-38.3511954248215,
27.8428186370589));
#57353=CARTESIAN_POINT('Ctrl Pts',(-13.9900981944685,-35.0255243857861,
27.6457391844904));
#57354=CARTESIAN_POINT('Ctrl Pts',(-12.2085743619008,-31.67678934832,27.448659731922));
#57355=CARTESIAN_POINT('Ctrl Pts',(-8.43122252006548,-31.3311486882979,
27.2515802793535));
#57356=CARTESIAN_POINT('Ctrl Pts',(-6.07153195208776,-34.3009497638899,
27.0545008267851));
#57357=CARTESIAN_POINT('Ctrl Pts',(-7.26189145632214,-37.9024633414879,
26.8574213742166));
#57358=CARTESIAN_POINT('Ctrl Pts',(-10.9266052171908,-38.881099717343,26.6603419216482));
#57359=CARTESIAN_POINT('Ctrl Pts',(-13.7539710465455,-36.3524916101345,
26.4632624690798));
#57360=CARTESIAN_POINT('Ctrl Pts',(-13.188975153351,-32.6016735869645,26.2661830165113));
#57361=CARTESIAN_POINT('Ctrl Pts',(-9.74218901680736,-31.0181580065441,
26.0691035639429));
#57362=CARTESIAN_POINT('Ctrl Pts',(-6.52837965989463,-33.0329249213308,
25.8720241113744));
#57363=CARTESIAN_POINT('Ctrl Pts',(-6.4517793402429,-36.8252841682075,25.674944658806));
#57364=CARTESIAN_POINT('Ctrl Pts',(-9.58160968267994,-38.9681836769399,
25.4778652062375));
#57365=CARTESIAN_POINT('Ctrl Pts',(-13.0895279947817,-37.5251433462124,
25.2807857536691));
#57366=CARTESIAN_POINT('Ctrl Pts',(-13.8055237492966,-33.8001995405442,
25.0837063011006));
#57367=CARTESIAN_POINT('Ctrl Pts',(-11.0825710252086,-31.1594828310307,
24.8866268485322));
#57368=CARTESIAN_POINT('Ctrl Pts',(-7.3813282611952,-31.989337203565,24.6895473959638));
#57369=CARTESIAN_POINT('Ctrl Pts',(-6.04650804135964,-35.5398457950117,
24.4924679433953));
#57370=CARTESIAN_POINT('Ctrl Pts',(-8.2843511531998,-38.6025104002618,24.2953884908269));
#57371=CARTESIAN_POINT('Ctrl Pts',(-12.0725795419546,-38.409684177713,24.0983090382584));
#57372=CARTESIAN_POINT('Ctrl Pts',(-13.9878740765231,-35.1356189487886,
23.90122958569));
#57373=CARTESIAN_POINT('Ctrl Pts',(-12.2994350930632,-31.7389985583748,
23.7041501331215));
#57374=CARTESIAN_POINT('Ctrl Pts',(-8.53305905381608,-31.2892566230088,
23.5070706805531));
#57375=CARTESIAN_POINT('Ctrl Pts',(-6.09231771499001,-34.1928127175841,
23.3099912279846));
#57376=CARTESIAN_POINT('Ctrl Pts',(-7.18284274969174,-37.8258020412897,
23.1129117754162));
#57377=CARTESIAN_POINT('Ctrl Pts',(-10.8191562956977,-38.9051907908123,
22.9158323228478));
#57378=CARTESIAN_POINT('Ctrl Pts',(-13.7152205402609,-36.4555646624855,
22.7187528702793));
#57379=CARTESIAN_POINT('Ctrl Pts',(-13.2539408640396,-32.6905842723531,
22.5216734177109));
#57380=CARTESIAN_POINT('Ctrl Pts',(-9.85216318494415,-31.0125601665875,
22.3245939651425));
#57381=CARTESIAN_POINT('Ctrl Pts',(-6.58398162146904,-32.9378771649101,
22.127514512574));
#57382=CARTESIAN_POINT('Ctrl Pts',(-6.40276310936531,-36.7266785758257,
21.9304350600056));
#57383=CARTESIAN_POINT('Ctrl Pts',(-9.47226989817816,-38.9551274422788,
21.7333556074371));
#57384=CARTESIAN_POINT('Ctrl Pts',(-13.0186720490941,-37.6094350367414,
21.5362761548687));
#57385=CARTESIAN_POINT('Ctrl Pts',(-13.8371822392237,-33.9056670402069,
21.3391967023002));
#57386=CARTESIAN_POINT('Ctrl Pts',(-11.1881350282313,-31.1908180318022,
21.1421172497318));
#57387=CARTESIAN_POINT('Ctrl Pts',(-7.4654024635467,-31.9182233205518,20.9450377971633));
#57388=CARTESIAN_POINT('Ctrl Pts',(-6.03311685083878,-35.4305465426475,
20.7479583445949));
#57389=CARTESIAN_POINT('Ctrl Pts',(-8.18559586174073,-38.553796486676,20.5508788920265));
#57390=CARTESIAN_POINT('Ctrl Pts',(-11.9777025518743,-38.4655771600677,
20.353799439458));
#57391=CARTESIAN_POINT('Ctrl Pts',(-13.9826132929195,-35.2456096251953,
20.1567199868896));
#57392=CARTESIAN_POINT('Ctrl Pts',(-12.3885442536368,-31.8036918021093,
19.9596405343211));
#57393=CARTESIAN_POINT('Ctrl Pts',(-8.63601320654501,-31.2501899884059,
19.7625610817527));
#57394=CARTESIAN_POINT('Ctrl Pts',(-6.11607883893393,-34.0852914897597,
19.5654816291843));
#57395=CARTESIAN_POINT('Ctrl Pts',(-7.10594085010763,-37.7469865930994,
19.3684021766158));
#57396=CARTESIAN_POINT('Ctrl Pts',(-10.7110809746912,-38.9263117544921,
19.1713227240473));
#57397=CARTESIAN_POINT('Ctrl Pts',(-13.6736456054499,-36.5575211536964,
18.9742432714789));
#57398=CARTESIAN_POINT('Ctrl Pts',(-13.3164183817332,-32.7812697435577,
18.7771638189105));
#57399=CARTESIAN_POINT('Ctrl Pts',(-9.9622699144086,-31.0099673304008,18.5800843663421));
#57400=CARTESIAN_POINT('Ctrl Pts',(-6.64214541117603,-32.8444631966324,
18.3830049137736));
#57401=CARTESIAN_POINT('Ctrl Pts',(-6.3565657025225,-36.6266318970639,18.1859254612052));
#57402=CARTESIAN_POINT('Ctrl Pts',(-9.36317426175285,-38.9393101142802,
17.9888460086367));
#57403=CARTESIAN_POINT('Ctrl Pts',(-12.9458314286048,-37.6912392747999,
17.7917665560683));
#57404=CARTESIAN_POINT('Ctrl Pts',(-13.865291102535,-34.0129649108121,17.5946871034998));
#57405=CARTESIAN_POINT('Ctrl Pts',(-11.2940600351478,-31.2230578534687,
17.3976076509314));
#57406=CARTESIAN_POINT('Ctrl Pts',(-7.54782180867489,-31.8537144777848,
17.2004824579512));
#57407=CARTESIAN_POINT('Ctrl Pts',(-6.53661527282589,-34.1600165773275,
17.0690504158272));
#57408=CARTESIAN_POINT('Ctrl Pts',(-6.62737380346809,-35.2744743533532,
17.0033115245594));
#57409=CARTESIAN_POINT('',(-12.5757531795041,-32.7919405097392,30.0016970964046));
#57410=CARTESIAN_POINT('Ctrl Pts',(-12.5735562464391,-32.7938238264104,
30.0016970964046));
#57411=CARTESIAN_POINT('Ctrl Pts',(-12.5615843318249,-32.7798583072438,
30.0011313976031));
#57412=CARTESIAN_POINT('Ctrl Pts',(-12.5494987379337,-32.7659902394485,
30.0005656988015));
#57413=CARTESIAN_POINT('Ctrl Pts',(-12.5373010662035,-32.7522214606544,
30.));
#57414=CARTESIAN_POINT('Ctrl Pts',(-11.0579044229731,-38.9456385074984,
30.));
#57415=CARTESIAN_POINT('Ctrl Pts',(-11.1744096706663,-38.9036233586964,
30.));
#57416=CARTESIAN_POINT('Ctrl Pts',(-11.2885140055709,-38.8559987888831,
30.));
#57417=CARTESIAN_POINT('Ctrl Pts',(-11.3999875271948,-38.8031290833885,
30.));
#57418=CARTESIAN_POINT('Ctrl Pts',(-11.5131043589436,-38.7494799881242,
30.));
#57419=CARTESIAN_POINT('Ctrl Pts',(-11.6235128455776,-38.690429357792,30.));
#57420=CARTESIAN_POINT('Ctrl Pts',(-11.7309450457163,-38.6263105171745,
30.));
#57421=CARTESIAN_POINT('Ctrl Pts',(-11.8388142181791,-38.5619308780369,
30.));
#57422=CARTESIAN_POINT('Ctrl Pts',(-11.9436834175853,-38.4924410128984,
30.));
#57423=CARTESIAN_POINT('Ctrl Pts',(-12.0452448209239,-38.4181410778747,
30.));
#57424=CARTESIAN_POINT('Ctrl Pts',(-12.1415282742907,-38.3477023669682,
30.));
#57425=CARTESIAN_POINT('Ctrl Pts',(-12.2348389156493,-38.2729397397906,
30.));
#57426=CARTESIAN_POINT('Ctrl Pts',(-12.3248772751976,-38.1940868171024,
30.));
#57427=CARTESIAN_POINT('Ctrl Pts',(-12.3423412091291,-38.1787924221463,
30.));
#57428=CARTESIAN_POINT('Ctrl Pts',(-12.3596819162977,-38.1633440964326,
30.));
#57429=CARTESIAN_POINT('Ctrl Pts',(-12.3768970324285,-38.1477434784525,
30.));
#57430=CARTESIAN_POINT('Ctrl Pts',(-12.3882097974424,-38.1374916669666,
30.));
#57431=CARTESIAN_POINT('Ctrl Pts',(-12.3994663625361,-38.1271758271379,
30.));
#57432=CARTESIAN_POINT('Ctrl Pts',(-12.4106599136893,-38.1168023488082,
30.));
#57433=CARTESIAN_POINT('Ctrl Pts',(-12.5011105162613,-38.0329784261902,
30.));
#57434=CARTESIAN_POINT('Ctrl Pts',(-12.587570228655,-37.9452850315018,30.));
#57435=CARTESIAN_POINT('Ctrl Pts',(-12.6697818789516,-37.854037402353,30.));
#57436=CARTESIAN_POINT('Ctrl Pts',(-12.7516039958967,-37.7632221206229,
30.));
#57437=CARTESIAN_POINT('Ctrl Pts',(-12.8292186797432,-37.6688854688381,
30.));
#57438=CARTESIAN_POINT('Ctrl Pts',(-12.902329952052,-37.5713094616899,30.));
#57439=CARTESIAN_POINT('Ctrl Pts',(-12.973771793756,-37.4759615155162,30.));
#57440=CARTESIAN_POINT('Ctrl Pts',(-13.0409138149038,-37.3775197612551,
30.));
#57441=CARTESIAN_POINT('Ctrl Pts',(-13.1034339775746,-37.2762304601522,
30.));
#57442=CARTESIAN_POINT('Ctrl Pts',(-13.1564891880338,-37.1902753864973,
30.));
#57443=CARTESIAN_POINT('Ctrl Pts',(-13.2062154030788,-37.1022692102076,
30.));
#57444=CARTESIAN_POINT('Ctrl Pts',(-13.2523866301025,-37.012357944282,30.));
#57445=CARTESIAN_POINT('Ctrl Pts',(-13.2633295087652,-36.9910483942254,
30.));
#57446=CARTESIAN_POINT('Ctrl Pts',(-13.2740725700391,-36.9696318241106,
30.));
#57447=CARTESIAN_POINT('Ctrl Pts',(-13.2846125648802,-36.948110170831,30.));
#57448=CARTESIAN_POINT('Ctrl Pts',(-13.2922655181554,-36.9324835780826,
30.));
#57449=CARTESIAN_POINT('Ctrl Pts',(-13.2998074679507,-36.9168095952847,
30.));
#57450=CARTESIAN_POINT('Ctrl Pts',(-13.3072357732831,-36.9010928608241,
30.));
#57451=CARTESIAN_POINT('Ctrl Pts',(-13.3571186448737,-36.795551177783,30.));
#57452=CARTESIAN_POINT('Ctrl Pts',(-13.4019075471307,-36.6880280906304,
30.));
#57453=CARTESIAN_POINT('Ctrl Pts',(-13.4413371254717,-36.5787736678,30.));
#57454=CARTESIAN_POINT('Ctrl Pts',(-13.4805534288888,-36.4701102030702,
30.));
#57455=CARTESIAN_POINT('Ctrl Pts',(-13.5144685808348,-36.3597334673255,
30.));
#57456=CARTESIAN_POINT('Ctrl Pts',(-13.5427714797555,-36.2478788313556,
30.));
#57457=CARTESIAN_POINT('Ctrl Pts',(-13.5490241675936,-36.2231678600901,
30.));
#57458=CARTESIAN_POINT('Ctrl Pts',(-13.5550027386183,-36.1983847374895,
30.));
#57459=CARTESIAN_POINT('Ctrl Pts',(-13.5607034802902,-36.1735319763925,
30.));
#57460=CARTESIAN_POINT('Ctrl Pts',(-13.5872167898843,-36.0579454462257,
30.));
#57461=CARTESIAN_POINT('Ctrl Pts',(-13.6077246013846,-35.9408518074948,
30.));
#57462=CARTESIAN_POINT('Ctrl Pts',(-13.622313567663,-35.8226895292052,30.));
#57463=CARTESIAN_POINT('Ctrl Pts',(-13.6304386582349,-35.7568809451723,
30.));
#57464=CARTESIAN_POINT('Ctrl Pts',(-13.6367269390635,-35.6907410456955,
30.));
#57465=CARTESIAN_POINT('Ctrl Pts',(-13.6411867179029,-35.6243477453809,
30.));
#57466=CARTESIAN_POINT('Ctrl Pts',(-13.6425502406279,-35.6040488074671,
30.));
#57467=CARTESIAN_POINT('Ctrl Pts',(-13.6437428108378,-35.5837261979104,
30.));
#57468=CARTESIAN_POINT('Ctrl Pts',(-13.6447645818877,-35.5633821868984,
30.));
#57469=CARTESIAN_POINT('Ctrl Pts',(-13.6454919371615,-35.5489001522975,
30.));
#57470=CARTESIAN_POINT('Ctrl Pts',(-13.6461326209842,-35.5344089094296,
30.));
#57471=CARTESIAN_POINT('Ctrl Pts',(-13.6466864886703,-35.5199186950792,
30.));
#57472=CARTESIAN_POINT('Ctrl Pts',(-13.6511186439618,-35.4039652249222,
30.));
#57473=CARTESIAN_POINT('Ctrl Pts',(-13.6500048268794,-35.2879090483184,
30.));
#57474=CARTESIAN_POINT('Ctrl Pts',(-13.6434927288465,-35.172153928784,30.));
#57475=CARTESIAN_POINT('Ctrl Pts',(-13.6369459111642,-35.055781653741,30.));
#57476=CARTESIAN_POINT('Ctrl Pts',(-13.6249427915427,-34.939712732213,30.));
#57477=CARTESIAN_POINT('Ctrl Pts',(-13.6075814117316,-34.8243668994998,
30.));
#57478=CARTESIAN_POINT('Ctrl Pts',(-13.5904442763799,-34.710510905969,30.));
#57479=CARTESIAN_POINT('Ctrl Pts',(-13.568085985003,-34.5973586326097,30.));
#57480=CARTESIAN_POINT('Ctrl Pts',(-13.5405558990396,-34.4853357966022,
30.));
#57481=CARTESIAN_POINT('Ctrl Pts',(-13.5211239058209,-34.4062649577923,
30.));
#57482=CARTESIAN_POINT('Ctrl Pts',(-13.4991142948317,-34.327757263627,30.));
#57483=CARTESIAN_POINT('Ctrl Pts',(-13.474532315096,-34.2499724344563,30.));
#57484=CARTESIAN_POINT('Ctrl Pts',(-13.4674334198858,-34.2275093799274,
30.));
#57485=CARTESIAN_POINT('Ctrl Pts',(-13.4601199377529,-34.2051066720009,
30.));
#57486=CARTESIAN_POINT('Ctrl Pts',(-13.4525918509037,-34.1827683167229,
30.));
#57487=CARTESIAN_POINT('Ctrl Pts',(-13.4468393693237,-34.1656987770326,
30.));
#57488=CARTESIAN_POINT('Ctrl Pts',(-13.4409618009596,-34.1486676726928,
30.));
#57489=CARTESIAN_POINT('Ctrl Pts',(-13.4349636292873,-34.1316889240451,
30.));
#57490=CARTESIAN_POINT('Ctrl Pts',(-13.3973629896804,-34.0252545230712,
30.));
#57491=CARTESIAN_POINT('Ctrl Pts',(-13.3549838287623,-33.920747099218,30.));
#57492=CARTESIAN_POINT('Ctrl Pts',(-13.307891120105,-33.8185692933513,30.));
#57493=CARTESIAN_POINT('Ctrl Pts',(-13.267579990653,-33.7311055887387,30.));
#57494=CARTESIAN_POINT('Ctrl Pts',(-13.2238142902954,-33.6453489675918,
30.));
#57495=CARTESIAN_POINT('Ctrl Pts',(-13.1766120348928,-33.5615721686833,
30.));
#57496=CARTESIAN_POINT('Ctrl Pts',(-13.1583494816227,-33.5291589240236,
30.));
#57497=CARTESIAN_POINT('Ctrl Pts',(-13.1395722952297,-33.4970422713474,
30.));
#57498=CARTESIAN_POINT('Ctrl Pts',(-13.1202807524539,-33.4652389414177,
30.));
#57499=CARTESIAN_POINT('Ctrl Pts',(-13.1062080395183,-33.4420391829693,
30.));
#57500=CARTESIAN_POINT('Ctrl Pts',(-13.0918589518343,-33.4190020869106,
30.));
#57501=CARTESIAN_POINT('Ctrl Pts',(-13.0772443148201,-33.3961510770974,
30.));
#57502=CARTESIAN_POINT('Ctrl Pts',(-13.0739471956041,-33.3909957999949,
30.));
#57503=CARTESIAN_POINT('Ctrl Pts',(-13.0706366360367,-33.3858500994359,
30.));
#57504=CARTESIAN_POINT('Ctrl Pts',(-13.0673128268107,-33.3807143197486,
30.));
#57505=CARTESIAN_POINT('Ctrl Pts',(-13.0087456693047,-33.2902193492488,
30.));
#57506=CARTESIAN_POINT('Ctrl Pts',(-12.946022899502,-33.2027323003118,30.));
#57507=CARTESIAN_POINT('Ctrl Pts',(-12.879180959548,-33.1186350334298,30.));
#57508=CARTESIAN_POINT('Ctrl Pts',(-12.8123390195941,-33.0345377665478,
30.));
#57509=CARTESIAN_POINT('Ctrl Pts',(-12.7413776235882,-32.9538296256876,
30.));
#57510=CARTESIAN_POINT('Ctrl Pts',(-12.6663019920974,-32.8769345953137,
30.));
#57511=CARTESIAN_POINT('Ctrl Pts',(-12.6374947385807,-32.8474292206645,
30.));
#57512=CARTESIAN_POINT('Ctrl Pts',(-12.6080814062809,-32.8184857731937,
30.));
#57513=CARTESIAN_POINT('Ctrl Pts',(-12.5780826598067,-32.7901129261999,
30.));
#57514=CARTESIAN_POINT('Origin',(130.,35.,17.));
#57515=CARTESIAN_POINT('Ctrl Pts',(133.378768828602,34.7273715616999,17.));
#57516=CARTESIAN_POINT('Ctrl Pts',(133.398288233977,34.8335416259198,17.));
#57517=CARTESIAN_POINT('Ctrl Pts',(133.412279007432,34.9404514354858,17.0000000000001));
#57518=CARTESIAN_POINT('Ctrl Pts',(133.420978703021,35.0477528815053,17.0000000000001));
#57519=CARTESIAN_POINT('Ctrl Pts',(133.42967839861,35.1550543275247,17.0000000000002));
#57520=CARTESIAN_POINT('Ctrl Pts',(133.433086897826,35.2627480950217,17.0000000000003));
#57521=CARTESIAN_POINT('Ctrl Pts',(133.431392514054,35.3705051659232,17.0000000000002));
#57522=CARTESIAN_POINT('Ctrl Pts',(133.430532515791,35.425198143565,17.0000000000001));
#57523=CARTESIAN_POINT('Ctrl Pts',(133.428357163319,35.479907669662,17.0000000000001));
#57524=CARTESIAN_POINT('Ctrl Pts',(133.424886375688,35.5345917347118,17.0000000000001));
#57525=CARTESIAN_POINT('Ctrl Pts',(133.423593503532,35.5549616082467,17.0000000000001));
#57526=CARTESIAN_POINT('Ctrl Pts',(133.422121399213,35.5753190427029,17.));
#57527=CARTESIAN_POINT('Ctrl Pts',(133.420471724452,35.5956591262037,17.));
#57528=CARTESIAN_POINT('Ctrl Pts',(133.411386020314,35.7076836204683,17.));
#57529=CARTESIAN_POINT('Ctrl Pts',(133.396916614694,35.8192070065116,17.0000000000002));
#57530=CARTESIAN_POINT('Ctrl Pts',(133.377281468097,35.9298641207523,17.0000000000002));
#57531=CARTESIAN_POINT('Ctrl Pts',(133.36026028628,36.025789804401,17.0000000000001));
#57532=CARTESIAN_POINT('Ctrl Pts',(133.339356307749,36.1210651259812,17.));
#57533=CARTESIAN_POINT('Ctrl Pts',(133.314680099781,36.2154569772683,17.0000000000001));
#57534=CARTESIAN_POINT('Ctrl Pts',(133.305738302252,36.2496612935773,17.0000000000002));
#57535=CARTESIAN_POINT('Ctrl Pts',(133.296300907899,36.2837496130644,17.0000000000001));
#57536=CARTESIAN_POINT('Ctrl Pts',(133.286372264486,36.3177108224521,17.0000000000001));
#57537=CARTESIAN_POINT('Ctrl Pts',(133.27907397728,36.3426748230392,17.0000000000001));
#57538=CARTESIAN_POINT('Ctrl Pts',(133.271508428315,36.3675755235939,17.));
#57539=CARTESIAN_POINT('Ctrl Pts',(133.263687370245,36.3923772787486,17.));
#57540=CARTESIAN_POINT('Ctrl Pts',(133.229058695359,36.5021900314774,17.));
#57541=CARTESIAN_POINT('Ctrl Pts',(133.189398803451,36.6101610148702,16.9999999999999));
#57542=CARTESIAN_POINT('Ctrl Pts',(133.144932484444,36.7159227801683,17.));
#57543=CARTESIAN_POINT('Ctrl Pts',(133.099884875903,36.8230671246546,17.));
#57544=CARTESIAN_POINT('Ctrl Pts',(133.049904265293,36.9279449826529,17.));
#57545=CARTESIAN_POINT('Ctrl Pts',(132.995171184149,37.0301762722481,16.9999999999999));
#57546=CARTESIAN_POINT('Ctrl Pts',(132.940661033746,37.1319911683814,16.9999999999999));
#57547=CARTESIAN_POINT('Ctrl Pts',(132.881436812319,37.2311818991061,17.0000000000001));
#57548=CARTESIAN_POINT('Ctrl Pts',(132.817627108291,37.327361736492,17.0000000000001));
#57549=CARTESIAN_POINT('Ctrl Pts',(132.780025706327,37.3840380176536,17.0000000000001));
#57550=CARTESIAN_POINT('Ctrl Pts',(132.74083110084,37.4396685072474,17.0000000000001));
#57551=CARTESIAN_POINT('Ctrl Pts',(132.70006195955,37.4941703136841,16.9999999999999));
#57552=CARTESIAN_POINT('Ctrl Pts',(132.678439734566,37.5230757623517,16.9999999999999));
#57553=CARTESIAN_POINT('Ctrl Pts',(132.656374531928,37.5516636796183,16.9999999999999));
#57554=CARTESIAN_POINT('Ctrl Pts',(132.633868515218,37.579921261406,17.));
#57555=CARTESIAN_POINT('Ctrl Pts',(132.623918667431,37.592413860219,17.));
#57556=CARTESIAN_POINT('Ctrl Pts',(132.613883456604,37.6048407975903,17.0000000000001));
#57557=CARTESIAN_POINT('Ctrl Pts',(132.60377100071,37.6171915760467,17.0000000000001));
#57558=CARTESIAN_POINT('Ctrl Pts',(132.528292267067,37.7093770082662,17.));
#57559=CARTESIAN_POINT('Ctrl Pts',(132.448399939567,37.7974650775518,17.0000000000002));
#57560=CARTESIAN_POINT('Ctrl Pts',(132.364284930497,37.8810681553255,17.));
#57561=CARTESIAN_POINT('Ctrl Pts',(132.340799781667,37.9044103714878,17.));
#57562=CARTESIAN_POINT('Ctrl Pts',(132.316985154723,37.9274028855291,17.));
#57563=CARTESIAN_POINT('Ctrl Pts',(132.292844514065,37.9500370350214,17.));
#57564=CARTESIAN_POINT('Ctrl Pts',(132.208770395894,38.0288645270553,17.0000000000001));
#57565=CARTESIAN_POINT('Ctrl Pts',(132.12074560811,38.1033478921207,17.0000000000001));
#57566=CARTESIAN_POINT('Ctrl Pts',(132.029196142605,38.1734758687271,17.0000000000001));
#57567=CARTESIAN_POINT('Ctrl Pts',(131.937646677099,38.2436038453334,17.0000000000001));
#57568=CARTESIAN_POINT('Ctrl Pts',(131.842571858722,38.3093767105707,17.0000000000001));
#57569=CARTESIAN_POINT('Ctrl Pts',(131.744357347521,38.3707491714389,17.));
#57570=CARTESIAN_POINT('Ctrl Pts',(131.688282851896,38.4057891033832,16.9999999999999));
#57571=CARTESIAN_POINT('Ctrl Pts',(131.631184222155,38.4393939844899,17.));
#57572=CARTESIAN_POINT('Ctrl Pts',(131.573128638195,38.4715498712856,17.));
#57573=CARTESIAN_POINT('Ctrl Pts',(131.556944790657,38.4805137974726,17.));
#57574=CARTESIAN_POINT('Ctrl Pts',(131.540686561425,38.4893650974868,16.9999999999999));
#57575=CARTESIAN_POINT('Ctrl Pts',(131.524355368347,38.4981034100422,17.));
#57576=CARTESIAN_POINT('Ctrl Pts',(131.511360721652,38.5050564405907,17.0000000000001));
#57577=CARTESIAN_POINT('Ctrl Pts',(131.498320953668,38.5119373168649,17.));
#57578=CARTESIAN_POINT('Ctrl Pts',(131.485245644539,38.5187414041372,17.));
#57579=CARTESIAN_POINT('Ctrl Pts',(131.379199746276,38.5739252272921,17.));
#57580=CARTESIAN_POINT('Ctrl Pts',(131.270663835054,38.6241445793112,17.));
#57581=CARTESIAN_POINT('Ctrl Pts',(131.160092156422,38.6693989331698,17.));
#57582=CARTESIAN_POINT('Ctrl Pts',(131.047638905155,38.7154233698825,16.9999999999999));
#57583=CARTESIAN_POINT('Ctrl Pts',(130.93307935156,38.7563127793653,17.));
#57584=CARTESIAN_POINT('Ctrl Pts',(130.81685155244,38.7920288702004,17.));
#57585=CARTESIAN_POINT('Ctrl Pts',(130.699197470088,38.8281832491378,17.));
#57586=CARTESIAN_POINT('Ctrl Pts',(130.579833172242,38.8590369618314,17.));
#57587=CARTESIAN_POINT('Ctrl Pts',(130.459183611273,38.884506012631,17.));
#57588=CARTESIAN_POINT('Ctrl Pts',(130.384593215661,38.9002520009274,17.));
#57589=CARTESIAN_POINT('Ctrl Pts',(130.309511030868,38.9139389657507,17.));
#57590=CARTESIAN_POINT('Ctrl Pts',(130.234033981252,38.9255377255911,17.));
#57591=CARTESIAN_POINT('Ctrl Pts',(130.197793530202,38.9311068925151,17.));
#57592=CARTESIAN_POINT('Ctrl Pts',(130.16146201578,38.9361945229447,17.));
#57593=CARTESIAN_POINT('Ctrl Pts',(130.125050048296,38.9407967639506,17.));
#57594=CARTESIAN_POINT('Ctrl Pts',(130.107526906085,38.9430115776289,17.));
#57595=CARTESIAN_POINT('Ctrl Pts',(130.089983170934,38.9451141902373,17.));
#57596=CARTESIAN_POINT('Ctrl Pts',(130.072426243663,38.9471034374065,17.));
#57597=CARTESIAN_POINT('Ctrl Pts',(129.946714063481,38.9613469661689,17.));
#57598=CARTESIAN_POINT('Ctrl Pts',(129.820703192049,38.969740803944,17.));
#57599=CARTESIAN_POINT('Ctrl Pts',(129.694857535268,38.9722500045349,17.));
#57600=CARTESIAN_POINT('Ctrl Pts',(129.568768076596,38.9747640662221,17.));
#57601=CARTESIAN_POINT('Ctrl Pts',(129.442843586438,38.971370981313,17.));
#57602=CARTESIAN_POINT('Ctrl Pts',(129.317528116281,38.9619883570952,17.));
#57603=CARTESIAN_POINT('Ctrl Pts',(129.194473565428,38.9527750125059,17.));
#57604=CARTESIAN_POINT('Ctrl Pts',(129.072005379203,38.9377864472662,17.));
#57605=CARTESIAN_POINT('Ctrl Pts',(128.950535432686,38.916896007705,17.));
#57606=CARTESIAN_POINT('Ctrl Pts',(128.859101902848,38.90117124052,17.));
#57607=CARTESIAN_POINT('Ctrl Pts',(128.768233713755,38.8821015413518,17.0000000000001));
#57608=CARTESIAN_POINT('Ctrl Pts',(128.678107721738,38.859613353343,17.));
#57609=CARTESIAN_POINT('Ctrl Pts',(128.630400716805,38.8477095276847,17.));
#57610=CARTESIAN_POINT('Ctrl Pts',(128.582901718775,38.8348475473756,16.9999999999999));
#57611=CARTESIAN_POINT('Ctrl Pts',(128.535626794907,38.8210452480852,17.));
#57612=CARTESIAN_POINT('Ctrl Pts',(126.824949217806,37.5702679880679,17.));
#57613=CARTESIAN_POINT('Ctrl Pts',(126.754722583789,37.4668131880797,17.0000000000002));
#57614=CARTESIAN_POINT('Ctrl Pts',(126.689770370388,37.3600639476932,17.0000000000001));
#57615=CARTESIAN_POINT('Ctrl Pts',(126.630097099889,37.2504517185812,17.));
#57616=CARTESIAN_POINT('Ctrl Pts',(126.569576179664,37.1392824644374,16.9999999999999));
#57617=CARTESIAN_POINT('Ctrl Pts',(126.514485103446,37.0251674270994,17.0000000000002));
#57618=CARTESIAN_POINT('Ctrl Pts',(126.464879687316,36.9085416396813,17.));
#57619=CARTESIAN_POINT('Ctrl Pts',(126.443235336355,36.8576542634462,16.9999999999998));
#57620=CARTESIAN_POINT('Ctrl Pts',(126.422636031133,36.8062887679583,17.));
#57621=CARTESIAN_POINT('Ctrl Pts',(126.403089494403,36.7544810720487,17.));
#57622=CARTESIAN_POINT('Ctrl Pts',(126.392820972199,36.7272645639194,17.0000000000001));
#57623=CARTESIAN_POINT('Ctrl Pts',(126.38284168639,36.6999218975391,16.9999999999999));
#57624=CARTESIAN_POINT('Ctrl Pts',(126.373162067941,36.6724850908568,16.9999999999999));
#57625=CARTESIAN_POINT('Ctrl Pts',(126.331490348817,36.5543669121558,16.9999999999999));
#57626=CARTESIAN_POINT('Ctrl Pts',(126.295333444097,36.4344165564152,16.9999999999998));
#57627=CARTESIAN_POINT('Ctrl Pts',(126.264731412048,36.3130621740795,17.));
#57628=CARTESIAN_POINT('Ctrl Pts',(126.239068026807,36.2112923223389,17.0000000000001));
#57629=CARTESIAN_POINT('Ctrl Pts',(126.217312167367,36.1085345475138,16.9999999999999));
#57630=CARTESIAN_POINT('Ctrl Pts',(126.199515719586,36.0050412373779,16.9999999999998));
#57631=CARTESIAN_POINT('Ctrl Pts',(126.191672794255,35.9594315565208,16.9999999999998));
#57632=CARTESIAN_POINT('Ctrl Pts',(126.184599194475,35.9136790581849,17.0000000000001));
#57633=CARTESIAN_POINT('Ctrl Pts',(126.178300953791,35.8678056462447,17.));
#57634=CARTESIAN_POINT('Ctrl Pts',(126.175607684965,35.8481891475192,17.));
#57635=CARTESIAN_POINT('Ctrl Pts',(126.173056211163,35.828550541702,16.9999999999998));
#57636=CARTESIAN_POINT('Ctrl Pts',(126.170647058657,35.8088915581212,16.9999999999999));
#57637=CARTESIAN_POINT('Ctrl Pts',(126.168408509338,35.7906247177321,16.9999999999999));
#57638=CARTESIAN_POINT('Ctrl Pts',(126.166293315633,35.7723438132087,17.0000000000001));
#57639=CARTESIAN_POINT('Ctrl Pts',(126.164302713477,35.7540600423693,17.0000000000001));
#57640=CARTESIAN_POINT('Ctrl Pts',(126.151059358918,35.6324192317109,17.));
#57641=CARTESIAN_POINT('Ctrl Pts',(126.143310499907,35.510523911799,16.9999999999999));
#57642=CARTESIAN_POINT('Ctrl Pts',(126.141090098496,35.3887717903632,17.));
#57643=CARTESIAN_POINT('Ctrl Pts',(126.138887312408,35.267985576692,17.));
#57644=CARTESIAN_POINT('Ctrl Pts',(126.142125699594,35.1473394639188,16.9999999999999));
#57645=CARTESIAN_POINT('Ctrl Pts',(126.150888803704,35.0272284639509,17.));
#57646=CARTESIAN_POINT('Ctrl Pts',(126.15944062651,34.9100133794443,17.0000000000001));
#57647=CARTESIAN_POINT('Ctrl Pts',(126.173254171156,34.7933072394163,16.9999999999999));
#57648=CARTESIAN_POINT('Ctrl Pts',(126.192452956354,34.6774945709228,17.));
#57649=CARTESIAN_POINT('Ctrl Pts',(126.204155767891,34.6068998005225,17.));
#57650=CARTESIAN_POINT('Ctrl Pts',(126.217860418479,34.5366373940648,17.));
#57651=CARTESIAN_POINT('Ctrl Pts',(126.233603126139,34.4667993207977,17.));
#57652=CARTESIAN_POINT('Ctrl Pts',(126.243156003279,34.4244206812378,17.));
#57653=CARTESIAN_POINT('Ctrl Pts',(126.253459458477,34.3821983693281,17.));
#57654=CARTESIAN_POINT('Ctrl Pts',(126.264522704234,34.3401537713521,16.9999999999999));
#57655=CARTESIAN_POINT('Ctrl Pts',(126.269462731949,34.3213797620011,16.9999999999999));
#57656=CARTESIAN_POINT('Ctrl Pts',(126.27455474766,34.3026397937225,16.9999999999999));
#57657=CARTESIAN_POINT('Ctrl Pts',(126.279793700241,34.2839559596265,16.9999999999999));
#57658=CARTESIAN_POINT('Ctrl Pts',(126.311063324684,34.1724381578618,16.9999999999998));
#57659=CARTESIAN_POINT('Ctrl Pts',(126.347606076099,34.0627526620742,16.9999999999999));
#57660=CARTESIAN_POINT('Ctrl Pts',(126.389497418337,33.9552547881673,16.9999999999998));
#57661=CARTESIAN_POINT('Ctrl Pts',(126.402467602738,33.9219718429867,16.9999999999998));
#57662=CARTESIAN_POINT('Ctrl Pts',(126.415950855001,33.8888987507312,16.9999999999999));
#57663=CARTESIAN_POINT('Ctrl Pts',(126.429950338727,33.8560464984648,16.9999999999999));
#57664=CARTESIAN_POINT('Ctrl Pts',(126.475866889916,33.7482952304651,16.9999999999998));
#57665=CARTESIAN_POINT('Ctrl Pts',(126.527333732362,33.6429171859707,17.));
#57666=CARTESIAN_POINT('Ctrl Pts',(126.584005799438,33.5401814510135,17.));
#57667=CARTESIAN_POINT('Ctrl Pts',(126.641108069226,33.4366658399347,17.));
#57668=CARTESIAN_POINT('Ctrl Pts',(126.703495652404,33.3358321983157,16.9999999999999));
#57669=CARTESIAN_POINT('Ctrl Pts',(126.770851333061,33.2379941517966,16.9999999999999));
#57670=CARTESIAN_POINT('Ctrl Pts',(126.804494181508,33.1891259562828,16.9999999999999));
#57671=CARTESIAN_POINT('Ctrl Pts',(126.839376958759,33.1410057578031,16.9999999999999));
#57672=CARTESIAN_POINT('Ctrl Pts',(126.875462529273,33.0936769067577,17.));
#57673=CARTESIAN_POINT('Ctrl Pts',(126.886664671689,33.0789844819944,17.));
#57674=CARTESIAN_POINT('Ctrl Pts',(126.897982734747,33.0643683404368,17.));
#57675=CARTESIAN_POINT('Ctrl Pts',(126.909415630747,33.0498298403455,16.9999999999999));
#57676=CARTESIAN_POINT('Ctrl Pts',(126.919261036269,33.0373100527876,16.9999999999999));
#57677=CARTESIAN_POINT('Ctrl Pts',(126.929188667834,33.0248516240596,17.0000000000002));
#57678=CARTESIAN_POINT('Ctrl Pts',(126.939192716546,33.0124613276602,17.0000000000002));
#57679=CARTESIAN_POINT('Ctrl Pts',(127.011948576822,32.922351143313,17.));
#57680=CARTESIAN_POINT('Ctrl Pts',(127.088821101316,32.8357421178869,17.0000000000001));
#57681=CARTESIAN_POINT('Ctrl Pts',(127.169466870983,32.7528788149574,17.0000000000001));
#57682=CARTESIAN_POINT('Ctrl Pts',(127.249991207905,32.6701402838339,17.0000000000001));
#57683=CARTESIAN_POINT('Ctrl Pts',(127.334278242301,32.5911357022543,17.0000000000001));
#57684=CARTESIAN_POINT('Ctrl Pts',(127.422017428112,32.5161493067951,17.));
#57685=CARTESIAN_POINT('Ctrl Pts',(127.509023135241,32.4417897797291,16.9999999999999));
#57686=CARTESIAN_POINT('Ctrl Pts',(127.599424292657,32.3713811155938,17.0000000000001));
#57687=CARTESIAN_POINT('Ctrl Pts',(127.692937081477,32.3052474021187,17.0000000000001));
#57688=CARTESIAN_POINT('Ctrl Pts',(127.745229281574,32.2682655366242,17.0000000000001));
#57689=CARTESIAN_POINT('Ctrl Pts',(127.79849477284,32.2326213384267,17.));
#57690=CARTESIAN_POINT('Ctrl Pts',(127.852685200275,32.1983787022165,17.));
#57691=CARTESIAN_POINT('Ctrl Pts',(127.881422505441,32.1802197554612,17.0000000000001));
#57692=CARTESIAN_POINT('Ctrl Pts',(127.91041993099,32.1624550478516,16.9999999999999));
#57693=CARTESIAN_POINT('Ctrl Pts',(127.939670295583,32.1450947484183,16.9999999999999));
#57694=CARTESIAN_POINT('Ctrl Pts',(127.95623701152,32.1352622846765,16.9999999999999));
#57695=CARTESIAN_POINT('Ctrl Pts',(127.972886663471,32.1255586278457,17.));
#57696=CARTESIAN_POINT('Ctrl Pts',(127.98959836262,32.1159965954256,17.));
#57697=CARTESIAN_POINT('Ctrl Pts',(128.086647842483,32.060467216604,17.));
#57698=CARTESIAN_POINT('Ctrl Pts',(128.1859309852,32.0096238875741,17.));
#57699=CARTESIAN_POINT('Ctrl Pts',(128.287161065264,31.9637255550784,17.));
#57700=CARTESIAN_POINT('Ctrl Pts',(128.385832953704,31.9189871221864,16.9999999999999));
#57701=CARTESIAN_POINT('Ctrl Pts',(128.486355341507,31.8789467189593,17.));
#57702=CARTESIAN_POINT('Ctrl Pts',(128.588474407863,31.8438911608433,17.));
#57703=CARTESIAN_POINT('Ctrl Pts',(128.688986058153,31.8093873984823,17.));
#57704=CARTESIAN_POINT('Ctrl Pts',(128.791045115042,31.77971256302,17.));
#57705=CARTESIAN_POINT('Ctrl Pts',(128.894411452207,31.7551894334429,17.));
#57706=CARTESIAN_POINT('Ctrl Pts',(128.959370158269,31.7397783159591,16.9999999999999));
#57707=CARTESIAN_POINT('Ctrl Pts',(129.024845149963,31.7264027373315,17.));
#57708=CARTESIAN_POINT('Ctrl Pts',(129.090775656524,31.7151536247108,17.));
#57709=CARTESIAN_POINT('Ctrl Pts',(129.131408312752,31.7082208503425,17.));
#57710=CARTESIAN_POINT('Ctrl Pts',(129.172213968367,31.7020959537143,17.));
#57711=CARTESIAN_POINT('Ctrl Pts',(129.213170778782,31.6967753652515,17.));
#57712=CARTESIAN_POINT('Ctrl Pts',(132.567055762672,37.2043908438416,29.9966205380558));
#57713=CARTESIAN_POINT('Ctrl Pts',(133.295540430453,36.3561521436381,29.9308807084033));
#57714=CARTESIAN_POINT('Ctrl Pts',(133.83237619187,33.895265814678,29.7994477278945));
#57715=CARTESIAN_POINT('Ctrl Pts',(131.173364181338,31.1840944667917,29.6023215965296));
#57716=CARTESIAN_POINT('Ctrl Pts',(127.452981029627,31.9293652704744,29.4052421439611));
#57717=CARTESIAN_POINT('Ctrl Pts',(126.035010474348,35.4458461447659,29.2081626913928));
#57718=CARTESIAN_POINT('Ctrl Pts',(128.199728311344,38.5611777251301,29.0110832388244));
#57719=CARTESIAN_POINT('Ctrl Pts',(131.991478805662,38.4575237094584,28.814003786256));
#57720=CARTESIAN_POINT('Ctrl Pts',(133.983498870357,35.2298082435239,28.6169243336875));
#57721=CARTESIAN_POINT('Ctrl Pts',(132.375780304869,31.7942237028353,28.4198448811191));
#57722=CARTESIAN_POINT('Ctrl Pts',(128.621113708042,31.2557076608804,28.2227654285506));
#57723=CARTESIAN_POINT('Ctrl Pts',(126.112518820413,34.1007607740198,28.0256859759822));
#57724=CARTESIAN_POINT('Ctrl Pts',(127.116930471706,37.7584542688539,27.8286065234137));
#57725=CARTESIAN_POINT('Ctrl Pts',(130.726696014798,38.9233967594309,27.6315270708453));
#57726=CARTESIAN_POINT('Ctrl Pts',(133.679765016802,36.5428773444799,27.4344476182769));
#57727=CARTESIAN_POINT('Ctrl Pts',(133.307530816144,32.7680990489065,27.2373681657084));
#57728=CARTESIAN_POINT('Ctrl Pts',(129.946370574694,31.0102302563085,27.04028871314));
#57729=CARTESIAN_POINT('Ctrl Pts',(126.633673911154,32.8578074562423,26.8432092605715));
#57730=CARTESIAN_POINT('Ctrl Pts',(126.363034667212,36.6412261742564,26.646129808003));
#57731=CARTESIAN_POINT('Ctrl Pts',(129.379022266619,38.941513226243,26.4490503554346));
#57732=CARTESIAN_POINT('Ctrl Pts',(132.956170568106,37.6799618681735,26.2519709028662));
#57733=CARTESIAN_POINT('Ctrl Pts',(133.861907804393,33.9966017081917,26.0548914502976));
#57734=CARTESIAN_POINT('Ctrl Pts',(131.277743819111,31.2199853542158,25.8578119977293));
#57735=CARTESIAN_POINT('Ctrl Pts',(127.538917441336,31.8592655873322,25.6607325451609));
#57736=CARTESIAN_POINT('Ctrl Pts',(126.024104543952,35.3367422307258,25.4636530925924));
#57737=CARTESIAN_POINT('Ctrl Pts',(128.102200410904,38.5099140622057,25.2665736400239));
#57738=CARTESIAN_POINT('Ctrl Pts',(131.895286234357,38.5112718631302,25.0694941874556));
#57739=CARTESIAN_POINT('Ctrl Pts',(133.975653351649,35.3395886244166,24.8724147348871));
#57740=CARTESIAN_POINT('Ctrl Pts',(132.4633304881,31.8610283670508,24.6753352823186));
#57741=CARTESIAN_POINT('Ctrl Pts',(128.724962750633,31.2190715400751,24.4782558297502));
#57742=CARTESIAN_POINT('Ctrl Pts',(126.138811553627,33.9938370967647,24.2811763771818));
#57743=CARTESIAN_POINT('Ctrl Pts',(127.041911510654,37.6778447481953,24.0840969246132));
#57744=CARTESIAN_POINT('Ctrl Pts',(130.618155712909,38.9419568136729,23.8870174720449));
#57745=CARTESIAN_POINT('Ctrl Pts',(133.635789382529,36.6438295447349,23.6899380194764));
#57746=CARTESIAN_POINT('Ctrl Pts',(133.36785891173,32.8602181520236,23.492858566908));
#57747=CARTESIAN_POINT('Ctrl Pts',(130.056485791714,31.0102695126623,23.2957791143395));
#57748=CARTESIAN_POINT('Ctrl Pts',(126.694067995515,32.765731979379,23.0986996617711));
#57749=CARTESIAN_POINT('Ctrl Pts',(126.319131183993,36.54024178803,22.9016202092026));
#57750=CARTESIAN_POINT('Ctrl Pts',(129.270495572856,38.922876915867,22.7045407566343));
#57751=CARTESIAN_POINT('Ctrl Pts',(132.881093303896,37.7605146948486,22.5074613040658));
#57752=CARTESIAN_POINT('Ctrl Pts',(133.888125248107,34.103550301869,22.3103818514974));
#57753=CARTESIAN_POINT('Ctrl Pts',(131.381563981988,31.2566831592799,22.1133023989289));
#57754=CARTESIAN_POINT('Ctrl Pts',(127.626520859714,31.7925498013699,21.9162229463605));
#57755=CARTESIAN_POINT('Ctrl Pts',(126.016326388125,35.2269020942195,21.719143493792));
#57756=CARTESIAN_POINT('Ctrl Pts',(128.006069588758,38.4562091259181,21.5220640412236));
#57757=CARTESIAN_POINT('Ctrl Pts',(131.797673559676,38.5622338184465,21.3249845886551));
#57758=CARTESIAN_POINT('Ctrl Pts',(133.964768748078,35.4491645373762,21.1279051360867));
#57759=CARTESIAN_POINT('Ctrl Pts',(132.549010076058,31.930197458527,20.9308256835183));
#57760=CARTESIAN_POINT('Ctrl Pts',(128.829780213618,31.1853275840279,20.7337462309498));
#57761=CARTESIAN_POINT('Ctrl Pts',(126.168046195167,33.8876735824175,20.5366667783814));
#57762=CARTESIAN_POINT('Ctrl Pts',(126.9691447818,37.5951987763752,20.3395873258129));
#57763=CARTESIAN_POINT('Ctrl Pts',(130.509144924881,38.9575132726843,20.1425078732445));
#57764=CARTESIAN_POINT('Ctrl Pts',(133.589044636381,36.7435305517908,19.9454284206759));
#57765=CARTESIAN_POINT('Ctrl Pts',(133.425622140562,32.9539664760638,19.7483489681076));
#57766=CARTESIAN_POINT('Ctrl Pts',(130.166557985232,31.0133476248247,19.5512695155392));
#57767=CARTESIAN_POINT('Ctrl Pts',(126.756979795506,32.6753576816052,19.3541900629707));
#57768=CARTESIAN_POINT('Ctrl Pts',(126.278031123947,36.4380851034208,19.1571106104022));
#57769=CARTESIAN_POINT('Ctrl Pts',(129.162524208194,38.9012515335436,18.9600311578338));
#57770=CARTESIAN_POINT('Ctrl Pts',(132.803822361966,37.8389681260754,18.7629517052654));
#57771=CARTESIAN_POINT('Ctrl Pts',(133.911380442483,34.2111754685922,18.5658722526969));
#57772=CARTESIAN_POINT('Ctrl Pts',(131.484334235672,31.296244554003,18.3687928001285));
#57773=CARTESIAN_POINT('Ctrl Pts',(127.715927186878,31.7282504513906,18.1717133475601));
#57774=CARTESIAN_POINT('Ctrl Pts',(126.011591887548,35.1169436079755,17.9746338949916));
#57775=CARTESIAN_POINT('Ctrl Pts',(127.911437177851,38.3997593110105,17.7775544424232));
#57776=CARTESIAN_POINT('Ctrl Pts',(131.698733478907,38.6107159277045,17.5804749898547));
#57777=CARTESIAN_POINT('Ctrl Pts',(133.950778465968,35.5579159759099,17.3833955372863));
#57778=CARTESIAN_POINT('Ctrl Pts',(132.632927527639,32.0027018980742,17.1863160847178));
#57779=CARTESIAN_POINT('Ctrl Pts',(128.935134083485,31.1524060608917,16.9892366321493));
#57780=CARTESIAN_POINT('Ctrl Pts',(126.201082349571,33.7865904288514,16.792157179581));
#57781=CARTESIAN_POINT('Ctrl Pts',(126.667056495351,36.2605541243663,16.6607708778687));
#57782=CARTESIAN_POINT('Ctrl Pts',(127.37006770175,37.1289835220537,16.5950777270125));
#57783=CARTESIAN_POINT('Ctrl Pts',(132.745392601518,37.3575328598391,30.1323365495442));
#57784=CARTESIAN_POINT('Ctrl Pts',(133.524486085317,36.4503658688749,30.0665967198915));
#57785=CARTESIAN_POINT('Ctrl Pts',(134.098616553793,33.8185184353491,29.9351637393829));
#57786=CARTESIAN_POINT('Ctrl Pts',(131.254879379394,30.9189983438223,29.738037608018));
#57787=CARTESIAN_POINT('Ctrl Pts',(127.276036173865,31.7160441191073,29.5409581554496));
#57788=CARTESIAN_POINT('Ctrl Pts',(125.759557284609,35.4768196799831,29.3438787028811));
#57789=CARTESIAN_POINT('Ctrl Pts',(128.074661000111,38.8085775624481,29.1467992503127));
#57790=CARTESIAN_POINT('Ctrl Pts',(132.129829534149,38.6977225619917,28.9497197977443));
#57791=CARTESIAN_POINT('Ctrl Pts',(134.260237929328,35.2457733332921,28.7526403451758));
#57792=CARTESIAN_POINT('Ctrl Pts',(132.540828978734,31.5715140838237,28.5555608926074));
#57793=CARTESIAN_POINT('Ctrl Pts',(128.525320610746,30.9955866034469,28.3584814400389));
#57794=CARTESIAN_POINT('Ctrl Pts',(125.842450240398,34.038289407694,28.1614019874705));
#57795=CARTESIAN_POINT('Ctrl Pts',(126.916639728775,37.9500878210208,27.964322534902));
#57796=CARTESIAN_POINT('Ctrl Pts',(130.777180570673,39.1959604433965,27.7672430823336));
#57797=CARTESIAN_POINT('Ctrl Pts',(133.935403273804,36.6500631221882,27.5701636297652));
#57798=CARTESIAN_POINT('Ctrl Pts',(133.537309459333,32.6130458685179,27.3730841771967));
#57799=CARTESIAN_POINT('Ctrl Pts',(129.942644865919,30.7330555512775,27.1760047246283));
#57800=CARTESIAN_POINT('Ctrl Pts',(126.399810680779,32.7089864403492,26.9789252720598));
#57801=CARTESIAN_POINT('Ctrl Pts',(126.110369762197,36.7552443783039,26.7818458194914));
#57802=CARTESIAN_POINT('Ctrl Pts',(129.335882102866,39.2153354856822,26.5847663669229));
#57803=CARTESIAN_POINT('Ctrl Pts',(133.161539739229,37.86614244701,26.3876869143545));
#57804=CARTESIAN_POINT('Ctrl Pts',(134.130199767414,33.9268942705633,26.190607461786));
#57805=CARTESIAN_POINT('Ctrl Pts',(131.366510411901,30.9573826197811,25.9935280092176));
#57806=CARTESIAN_POINT('Ctrl Pts',(127.367942704426,31.6410745160834,25.7964485566492));
#57807=CARTESIAN_POINT('Ctrl Pts',(125.747893704466,35.360136169341,25.5993691040807));
#57808=CARTESIAN_POINT('Ctrl Pts',(127.970357704405,38.753752543465,25.4022896515123));
#57809=CARTESIAN_POINT('Ctrl Pts',(132.0269543347,38.7552046726578,25.2052101989438));
#57810=CARTESIAN_POINT('Ctrl Pts',(134.251847371815,35.3631803058548,25.0081307463754));
#57811=CARTESIAN_POINT('Ctrl Pts',(132.63446139171,31.6429597584955,24.8110512938069));
#57812=CARTESIAN_POINT('Ctrl Pts',(128.636384186906,30.956405321735,24.6139718412385));
#57813=CARTESIAN_POINT('Ctrl Pts',(125.870569565381,33.923937597838,24.41689238867));
#57814=CARTESIAN_POINT('Ctrl Pts',(126.836409098946,37.8638782478409,24.2198129361016));
#57815=CARTESIAN_POINT('Ctrl Pts',(130.661099827081,39.2158098897313,24.0227334835332));
#57816=CARTESIAN_POINT('Ctrl Pts',(133.888372592688,36.7580286084536,23.8256540309647));
#57817=CARTESIAN_POINT('Ctrl Pts',(133.601828629387,32.7115646104299,23.6285745783963));
#57818=CARTESIAN_POINT('Ctrl Pts',(130.060409936129,30.7330975348234,23.4314951258278));
#57819=CARTESIAN_POINT('Ctrl Pts',(126.464400423935,32.610514355466,23.2344156732594));
#57820=CARTESIAN_POINT('Ctrl Pts',(126.063416244566,36.647244470064,23.0373362206909));
#57821=CARTESIAN_POINT('Ctrl Pts',(129.219815912774,39.1954044855965,22.8402567681225));
#57822=CARTESIAN_POINT('Ctrl Pts',(133.081246755844,37.9522913875984,22.6431773155541));
#57823=CARTESIAN_POINT('Ctrl Pts',(134.158238572435,34.0412727278192,22.4460978629857));
#57824=CARTESIAN_POINT('Ctrl Pts',(131.477543102034,30.9966298710407,22.2490184104172));
#57825=CARTESIAN_POINT('Ctrl Pts',(127.461632050868,31.5697238941575,22.0519389578488));
#57826=CARTESIAN_POINT('Ctrl Pts',(125.739575189624,35.2426652898614,21.8548595052803));
#57827=CARTESIAN_POINT('Ctrl Pts',(127.867548543914,38.6963166525534,21.6577800527119));
#57828=CARTESIAN_POINT('Ctrl Pts',(131.922560375371,38.8097070239969,21.4607006001434));
#57829=CARTESIAN_POINT('Ctrl Pts',(134.2402066001,35.4803686058201,21.263621147575));
#57830=CARTESIAN_POINT('Ctrl Pts',(132.726093256627,31.7169341203904,21.0665416950066));
#57831=CARTESIAN_POINT('Ctrl Pts',(128.748483460936,30.9203171273822,20.8694622424381));
#57832=CARTESIAN_POINT('Ctrl Pts',(125.901835177042,33.8103987604358,20.6723827898697));
#57833=CARTESIAN_POINT('Ctrl Pts',(126.758587166934,37.7754907484812,20.4753033373012));
#57834=CARTESIAN_POINT('Ctrl Pts',(130.54451591204,39.2324470770089,20.2782238847328));
#57835=CARTESIAN_POINT('Ctrl Pts',(133.838380425747,36.8646559794346,20.0811444321643));
#57836=CARTESIAN_POINT('Ctrl Pts',(133.663604747919,32.8118257574478,19.8840649795959));
#57837=CARTESIAN_POINT('Ctrl Pts',(130.178128993934,30.7363894876046,19.6869855270274));
#57838=CARTESIAN_POINT('Ctrl Pts',(126.531682791835,32.5138616328864,19.489906074459));
#57839=CARTESIAN_POINT('Ctrl Pts',(126.019460907712,36.537990822286,19.2928266218906));
#57840=CARTESIAN_POINT('Ctrl Pts',(129.104343631249,39.1722767586888,19.0957471693221));
#57841=CARTESIAN_POINT('Ctrl Pts',(132.998607696976,38.0361950848947,18.8986677167537));
#57842=CARTESIAN_POINT('Ctrl Pts',(134.183109336644,34.1563747605664,18.7015882641852));
#57843=CARTESIAN_POINT('Ctrl Pts',(131.587452944362,31.0389396494094,18.5045088116168));
#57844=CARTESIAN_POINT('Ctrl Pts',(127.55724955661,31.5009575812933,18.3074293590484));
#57845=CARTESIAN_POINT('Ctrl Pts',(125.734511776882,35.1250678387278,18.1103499064799));
#57846=CARTESIAN_POINT('Ctrl Pts',(127.766341891317,38.6359451925881,17.9132704539115));
#57847=CARTESIAN_POINT('Ctrl Pts',(131.816746793257,38.8615572510151,17.716191001343));
#57848=CARTESIAN_POINT('Ctrl Pts',(134.225244394153,35.5966751540052,17.5191115487746));
#57849=CARTESIAN_POINT('Ctrl Pts',(132.815840567169,31.794475541502,17.3220320962061));
#57850=CARTESIAN_POINT('Ctrl Pts',(128.86115640676,30.8851085014681,17.1249526436377));
#57851=CARTESIAN_POINT('Ctrl Pts',(125.937166397815,33.7022932233556,16.9278731910693));
#57852=CARTESIAN_POINT('Ctrl Pts',(126.435512398289,36.3481265257936,16.796486889357));
#57853=CARTESIAN_POINT('Ctrl Pts',(127.187362744862,37.2768868893281,16.7307937385008));
#57854=CARTESIAN_POINT('Ctrl Pts',(132.923729440365,37.5106748758366,30.2680525610325));
#57855=CARTESIAN_POINT('Ctrl Pts',(133.753431740182,36.5445795941117,30.2023127313799));
#57856=CARTESIAN_POINT('Ctrl Pts',(134.364856915716,33.7417710560202,30.0708797508712));
#57857=CARTESIAN_POINT('Ctrl Pts',(131.336394577451,30.653902220853,29.8737536195064));
#57858=CARTESIAN_POINT('Ctrl Pts',(127.099091318103,31.5027229677401,29.676674166938));
#57859=CARTESIAN_POINT('Ctrl Pts',(125.484104094871,35.5077932152003,29.4795947143695));
#57860=CARTESIAN_POINT('Ctrl Pts',(127.949593688879,39.0559773997662,29.2825152618011));
#57861=CARTESIAN_POINT('Ctrl Pts',(132.268180262635,38.937921414525,29.0854358092327));
#57862=CARTESIAN_POINT('Ctrl Pts',(134.536976988299,35.2617384230603,28.8883563566642));
#57863=CARTESIAN_POINT('Ctrl Pts',(132.705877652598,31.3488044648121,28.6912769040958));
#57864=CARTESIAN_POINT('Ctrl Pts',(128.42952751345,30.7354655460134,28.4941974515273));
#57865=CARTESIAN_POINT('Ctrl Pts',(125.572381660382,33.9758180413684,28.2971179989589));
#57866=CARTESIAN_POINT('Ctrl Pts',(126.716348985843,38.1417213731875,28.1000385463904));
#57867=CARTESIAN_POINT('Ctrl Pts',(130.827665126547,39.4685241273619,27.902959093822));
#57868=CARTESIAN_POINT('Ctrl Pts',(134.191041530805,36.7572488998967,27.7058796412536));
#57869=CARTESIAN_POINT('Ctrl Pts',(133.767088102523,32.4579926881293,27.5088001886851));
#57870=CARTESIAN_POINT('Ctrl Pts',(129.938919157145,30.4558808462466,27.3117207361167));
#57871=CARTESIAN_POINT('Ctrl Pts',(126.165947450404,32.5601654244561,27.1146412835482));
#57872=CARTESIAN_POINT('Ctrl Pts',(125.857704857182,36.8692625823514,26.9175618309798));
#57873=CARTESIAN_POINT('Ctrl Pts',(129.292741939113,39.4891577451213,26.7204823784113));
#57874=CARTESIAN_POINT('Ctrl Pts',(133.366908910353,38.0523230258466,26.5234029258429));
#57875=CARTESIAN_POINT('Ctrl Pts',(134.398491730435,33.8571868329348,26.3263234732744));
#57876=CARTESIAN_POINT('Ctrl Pts',(131.455277004692,30.6947798853466,26.129244020706));
#57877=CARTESIAN_POINT('Ctrl Pts',(127.196967967518,31.4228834448347,25.9321645681376));
#57878=CARTESIAN_POINT('Ctrl Pts',(125.471682864979,35.3835301079562,25.7350851155691));
#57879=CARTESIAN_POINT('Ctrl Pts',(127.838514997906,38.9975910247243,25.5380056630007));
#57880=CARTESIAN_POINT('Ctrl Pts',(132.158622435042,38.9991374821854,25.3409262104322));
#57881=CARTESIAN_POINT('Ctrl Pts',(134.528041391981,35.3867719872929,25.1438467578638));
#57882=CARTESIAN_POINT('Ctrl Pts',(132.80559229532,31.42489114994,24.9467673052954));
#57883=CARTESIAN_POINT('Ctrl Pts',(128.547805623179,30.693739103395,24.7496878527269));
#57884=CARTESIAN_POINT('Ctrl Pts',(125.602327577135,33.8540380989111,24.5526084001585));
#57885=CARTESIAN_POINT('Ctrl Pts',(126.630906687238,38.0499117474868,24.35552894759));
#57886=CARTESIAN_POINT('Ctrl Pts',(130.704043941251,39.4896629657897,24.1584494950216));
#57887=CARTESIAN_POINT('Ctrl Pts',(134.140955802847,36.8722276721723,23.9613700424531));
#57888=CARTESIAN_POINT('Ctrl Pts',(133.835798347043,32.5629110688361,23.7642905898847));
#57889=CARTESIAN_POINT('Ctrl Pts',(130.064334080544,30.4559255569845,23.5672111373162));
#57890=CARTESIAN_POINT('Ctrl Pts',(126.234732852354,32.455296731553,23.3701316847478));
#57891=CARTESIAN_POINT('Ctrl Pts',(125.807701305139,36.7542471520982,23.1730522321794));
#57892=CARTESIAN_POINT('Ctrl Pts',(129.169136252694,39.467932055326,22.9759727796109));
#57893=CARTESIAN_POINT('Ctrl Pts',(133.281400207792,38.1440680803481,22.7788933270425));
#57894=CARTESIAN_POINT('Ctrl Pts',(134.428351896762,33.9789951537694,22.581813874474));
#57895=CARTESIAN_POINT('Ctrl Pts',(131.573522222081,30.7365765828016,22.3847344219056));
#57896=CARTESIAN_POINT('Ctrl Pts',(127.296743242023,31.3468979869451,22.1876549693372));
#57897=CARTESIAN_POINT('Ctrl Pts',(125.462823991122,35.2584284855033,21.9905755167687));
#57898=CARTESIAN_POINT('Ctrl Pts',(127.729027499068,38.9364241791886,21.7934960642003));
#57899=CARTESIAN_POINT('Ctrl Pts',(132.047447191065,39.0571802295473,21.5964166116318));
#57900=CARTESIAN_POINT('Ctrl Pts',(134.515644452122,35.5115726742641,21.3993371590634));
#57901=CARTESIAN_POINT('Ctrl Pts',(132.903176437197,31.5036707822537,21.202257706495));
#57902=CARTESIAN_POINT('Ctrl Pts',(128.667186708253,30.6553066707365,21.0051782539265));
#57903=CARTESIAN_POINT('Ctrl Pts',(125.635624158919,33.7331239384541,20.8080988013581));
#57904=CARTESIAN_POINT('Ctrl Pts',(126.548029552068,37.9557827205871,20.6110193487896));
#57905=CARTESIAN_POINT('Ctrl Pts',(130.579886899199,39.5073808813335,20.4139398962212));
#57906=CARTESIAN_POINT('Ctrl Pts',(134.087716215113,36.9857814070785,20.2168604436527));
#57907=CARTESIAN_POINT('Ctrl Pts',(133.901587355275,32.6696850388319,20.0197809910843));
#57908=CARTESIAN_POINT('Ctrl Pts',(130.189700002638,30.4594313503844,19.8227015385158));
#57909=CARTESIAN_POINT('Ctrl Pts',(126.306385788164,32.3523655841678,19.6256220859474));
#57910=CARTESIAN_POINT('Ctrl Pts',(125.760890691477,36.6378965411511,19.428542633379));
#57911=CARTESIAN_POINT('Ctrl Pts',(129.046163054305,39.443301983834,19.2314631808105));
#57912=CARTESIAN_POINT('Ctrl Pts',(133.193393031986,38.2334220437139,19.0343837282421));
#57913=CARTESIAN_POINT('Ctrl Pts',(134.454838230805,34.1015740525406,18.8373042756736));
#57914=CARTESIAN_POINT('Ctrl Pts',(131.690571653052,30.7816347448159,18.6402248231052));
#57915=CARTESIAN_POINT('Ctrl Pts',(127.398571926341,31.273664711196,18.4431453705367));
#57916=CARTESIAN_POINT('Ctrl Pts',(125.457431666217,35.1331920694799,18.2460659179683));
#57917=CARTESIAN_POINT('Ctrl Pts',(127.621246604782,38.8721310741658,18.0489864653999));
#57918=CARTESIAN_POINT('Ctrl Pts',(131.934760107606,39.1123985743256,17.8519070128314));
#57919=CARTESIAN_POINT('Ctrl Pts',(134.499710322339,35.6354343321004,17.654827560263));
#57920=CARTESIAN_POINT('Ctrl Pts',(132.998753606699,31.5862491849297,17.4577481076945));
#57921=CARTESIAN_POINT('Ctrl Pts',(128.787178730035,30.6178109420444,17.2606686551261));
#57922=CARTESIAN_POINT('Ctrl Pts',(125.673250446058,33.6179960178598,17.0635892025576));
#57923=CARTESIAN_POINT('Ctrl Pts',(126.203968301227,36.4356989272208,16.9322029008454));
#57924=CARTESIAN_POINT('Ctrl Pts',(127.004657787973,37.4247902566023,16.8665097499892));
#57925=CARTESIAN_POINT('Ctrl Pts',(133.102066279211,37.6638168918341,30.4037685725209));
#57926=CARTESIAN_POINT('Ctrl Pts',(133.982377395047,36.6387933193483,30.3380287428683));
#57927=CARTESIAN_POINT('Ctrl Pts',(134.631097277639,33.6650236766912,30.2065957623595));
#57928=CARTESIAN_POINT('Ctrl Pts',(131.417909775507,30.3888060978836,30.0094696309947));
#57929=CARTESIAN_POINT('Ctrl Pts',(126.922146462341,31.289401816373,29.8123901784262));
#57930=CARTESIAN_POINT('Ctrl Pts',(125.208650905131,35.5387667504174,29.6153107258578));
#57931=CARTESIAN_POINT('Ctrl Pts',(127.824526377647,39.3033772370842,29.4182312732893));
#57932=CARTESIAN_POINT('Ctrl Pts',(132.406530991122,39.1781202670583,29.221151820721));
#57933=CARTESIAN_POINT('Ctrl Pts',(134.813716047271,35.2777035128283,29.0240723681525));
#57934=CARTESIAN_POINT('Ctrl Pts',(132.870926326462,31.1260948458003,28.8269929155841));
#57935=CARTESIAN_POINT('Ctrl Pts',(128.333734416155,30.4753444885799,28.6299134630156));
#57936=CARTESIAN_POINT('Ctrl Pts',(125.302313080367,33.9133466750426,28.4328340104471));
#57937=CARTESIAN_POINT('Ctrl Pts',(126.516058242912,38.3333549253541,28.2357545578788));
#57938=CARTESIAN_POINT('Ctrl Pts',(130.87814968242,39.7410878113275,28.0386751053102));
#57939=CARTESIAN_POINT('Ctrl Pts',(134.446679787807,36.8644346776051,27.8415956527419));
#57940=CARTESIAN_POINT('Ctrl Pts',(133.996866745713,32.3029395077406,27.6445162001734));
#57941=CARTESIAN_POINT('Ctrl Pts',(129.935193448372,30.1787061412156,27.447436747605));
#57942=CARTESIAN_POINT('Ctrl Pts',(125.932084220027,32.4113444085631,27.2503572950365));
#57943=CARTESIAN_POINT('Ctrl Pts',(125.605039952166,36.9832807863989,27.0532778424681));
#57944=CARTESIAN_POINT('Ctrl Pts',(129.249601775359,39.7629800045605,26.8561983898996));
#57945=CARTESIAN_POINT('Ctrl Pts',(133.572278081476,38.2385036046833,26.6591189373312));
#57946=CARTESIAN_POINT('Ctrl Pts',(134.666783693457,33.7874793953062,26.4620394847627));
#57947=CARTESIAN_POINT('Ctrl Pts',(131.544043597482,30.4321771509119,26.2649600321943));
#57948=CARTESIAN_POINT('Ctrl Pts',(127.025993230609,31.204692373586,26.0678805796259));
#57949=CARTESIAN_POINT('Ctrl Pts',(125.195472025492,35.4069240465715,25.8708011270574));
#57950=CARTESIAN_POINT('Ctrl Pts',(127.706672291407,39.2414295059836,25.673721674489));
#57951=CARTESIAN_POINT('Ctrl Pts',(132.290290535385,39.2430702917129,25.4766422219205));
#57952=CARTESIAN_POINT('Ctrl Pts',(134.804235412148,35.410363668731,25.2795627693521));
#57953=CARTESIAN_POINT('Ctrl Pts',(132.976723198929,31.2068225413846,25.0824833167836));
#57954=CARTESIAN_POINT('Ctrl Pts',(128.459227059453,30.4310728850549,24.8854038642152));
#57955=CARTESIAN_POINT('Ctrl Pts',(125.334085588889,33.7841385999844,24.6883244116468));
#57956=CARTESIAN_POINT('Ctrl Pts',(126.425404275529,38.2359452471325,24.4912449590783));
#57957=CARTESIAN_POINT('Ctrl Pts',(130.746988055422,39.7635160418482,24.2941655065099));
#57958=CARTESIAN_POINT('Ctrl Pts',(134.393539013006,36.9864267358912,24.0970860539414));
#57959=CARTESIAN_POINT('Ctrl Pts',(134.0697680647,32.4142575272423,23.900006601373));
#57960=CARTESIAN_POINT('Ctrl Pts',(130.068258224959,30.1787535791456,23.7029271488045));
#57961=CARTESIAN_POINT('Ctrl Pts',(126.005065280775,32.3000791076401,23.5058476962361));
#57962=CARTESIAN_POINT('Ctrl Pts',(125.551986365712,36.8612498341322,23.3087682436676));
#57963=CARTESIAN_POINT('Ctrl Pts',(129.118456592612,39.7404596250554,23.1116887910992));
#57964=CARTESIAN_POINT('Ctrl Pts',(133.481553659739,38.3358447730979,22.9146093385308));
#57965=CARTESIAN_POINT('Ctrl Pts',(134.698465221089,33.9167175797195,22.7175298859623));
#57966=CARTESIAN_POINT('Ctrl Pts',(131.669501342127,30.4765232945625,22.5204504333939));
#57967=CARTESIAN_POINT('Ctrl Pts',(127.131854433178,31.1240720797326,22.3233709808255));
#57968=CARTESIAN_POINT('Ctrl Pts',(125.186072792621,35.2741916811453,22.126291528257));
#57969=CARTESIAN_POINT('Ctrl Pts',(127.590506454223,39.1765317058238,21.9292120756886));
#57970=CARTESIAN_POINT('Ctrl Pts',(132.17233400676,39.3046534350976,21.7321326231201));
#57971=CARTESIAN_POINT('Ctrl Pts',(134.791082304144,35.5427767427079,21.5350531705517));
#57972=CARTESIAN_POINT('Ctrl Pts',(133.080259617766,31.2904074441171,21.3379737179832));
#57973=CARTESIAN_POINT('Ctrl Pts',(128.585889955571,30.3902962140908,21.1408942654148));
#57974=CARTESIAN_POINT('Ctrl Pts',(125.369413140795,33.6558491164725,20.9438148128464));
#57975=CARTESIAN_POINT('Ctrl Pts',(126.337471937201,38.136074692693,20.7467353602779));
#57976=CARTESIAN_POINT('Ctrl Pts',(130.615257886358,39.7823146856582,20.5496559077095));
#57977=CARTESIAN_POINT('Ctrl Pts',(134.33705200448,37.1069068347224,20.352576455141));
#57978=CARTESIAN_POINT('Ctrl Pts',(134.139569962632,32.5275443202159,20.1554970025726));
#57979=CARTESIAN_POINT('Ctrl Pts',(130.201271011341,30.1824732131642,19.9584175500041));
#57980=CARTESIAN_POINT('Ctrl Pts',(126.081088784494,32.1908695354491,19.7613380974357));
#57981=CARTESIAN_POINT('Ctrl Pts',(125.502320475242,36.7378022600163,19.5642586448672));
#57982=CARTESIAN_POINT('Ctrl Pts',(128.987982477359,39.7143272089792,19.3671791922988));
#57983=CARTESIAN_POINT('Ctrl Pts',(133.388178366997,38.4306490025331,19.1700997397304));
#57984=CARTESIAN_POINT('Ctrl Pts',(134.726567124965,34.0467733445149,18.9730202871619));
#57985=CARTESIAN_POINT('Ctrl Pts',(131.793690361742,30.5243298402222,18.7759408345935));
#57986=CARTESIAN_POINT('Ctrl Pts',(127.239894296073,31.0463718410988,18.5788613820251));
#57987=CARTESIAN_POINT('Ctrl Pts',(125.180351555551,35.1413163002321,18.3817819294566));
#57988=CARTESIAN_POINT('Ctrl Pts',(127.476151318247,39.1083169557435,18.1847024768882));
#57989=CARTESIAN_POINT('Ctrl Pts',(132.052773421955,39.3632398976362,17.9876230243197));
#57990=CARTESIAN_POINT('Ctrl Pts',(134.774176250524,35.6741935101957,17.7905435717513));
#57991=CARTESIAN_POINT('Ctrl Pts',(133.181666646227,31.3780228283574,17.5934641191828));
#57992=CARTESIAN_POINT('Ctrl Pts',(128.713201053309,30.3505133826207,17.3963846666144));
#57993=CARTESIAN_POINT('Ctrl Pts',(125.409334494302,33.533698812364,17.199305214046));
#57994=CARTESIAN_POINT('Ctrl Pts',(125.972424204166,36.5232713286481,17.0679189123336));
#57995=CARTESIAN_POINT('Ctrl Pts',(126.821952831084,37.5726936238766,17.0022257614775));
#57996=CARTESIAN_POINT('Ctrl Pts',(132.573234427015,37.2065515280923,30.));
#57997=CARTESIAN_POINT('Ctrl Pts',(132.649853019674,37.1336332793624,29.9999999999999));
#57998=CARTESIAN_POINT('Ctrl Pts',(132.722534994398,37.0570775958444,29.9999999999998));
#57999=CARTESIAN_POINT('Ctrl Pts',(132.791284483358,36.977300375456,30.));
#58000=CARTESIAN_POINT('Ctrl Pts',(132.861752925125,36.895528474395,30.0000000000001));
#58001=CARTESIAN_POINT('Ctrl Pts',(132.928090170014,36.8103715162712,30.));
#58002=CARTESIAN_POINT('Ctrl Pts',(132.990274451397,36.722229072783,30.));
#58003=CARTESIAN_POINT('Ctrl Pts',(133.053778947546,36.6322153050177,30.0000000000001));
#58004=CARTESIAN_POINT('Ctrl Pts',(133.112952713737,36.5390874001683,30.0000000000001));
#58005=CARTESIAN_POINT('Ctrl Pts',(133.167739109377,36.4432284799637,30.0000000000002));
#58006=CARTESIAN_POINT('Ctrl Pts',(133.220861751636,36.3502806036549,30.0000000000002));
#58007=CARTESIAN_POINT('Ctrl Pts',(133.269859583631,36.2547642631004,29.9999999999999));
#58008=CARTESIAN_POINT('Ctrl Pts',(133.314646019766,36.1569996980181,30.));
#58009=CARTESIAN_POINT('Ctrl Pts',(133.321659778676,36.1416893239718,30.));
#58010=CARTESIAN_POINT('Ctrl Pts',(133.328570937711,36.1263220445087,30.));
#58011=CARTESIAN_POINT('Ctrl Pts',(133.335376683319,36.110904481846,30.));
#58012=CARTESIAN_POINT('Ctrl Pts',(133.381298957067,36.0068733331781,29.9999999999998));
#58013=CARTESIAN_POINT('Ctrl Pts',(133.422281347888,35.9008837141508,29.9999999999999));
#58014=CARTESIAN_POINT('Ctrl Pts',(133.458300951026,35.7933676203473,29.9999999999999));
#58015=CARTESIAN_POINT('Ctrl Pts',(133.494921707518,35.6840571241977,30.));
#58016=CARTESIAN_POINT('Ctrl Pts',(133.526413089524,35.5731680825438,29.9999999999999));
#58017=CARTESIAN_POINT('Ctrl Pts',(133.552712099049,35.4611166522047,30.));
#58018=CARTESIAN_POINT('Ctrl Pts',(133.579063193468,35.3488433052603,30.0000000000001));
#58019=CARTESIAN_POINT('Ctrl Pts',(133.600201707779,35.2354021361399,30.0000000000001));
#58020=CARTESIAN_POINT('Ctrl Pts',(133.616019384666,35.1211857228107,30.0000000000001));
#58021=CARTESIAN_POINT('Ctrl Pts',(133.629397241759,35.0245867806253,30.));
#58022=CARTESIAN_POINT('Ctrl Pts',(133.638968470452,34.9274325880293,30.));
#58023=CARTESIAN_POINT('Ctrl Pts',(133.644639510987,34.8299528255702,30.));
#58024=CARTESIAN_POINT('Ctrl Pts',(133.645720632867,34.8113693745521,30.));
#58025=CARTESIAN_POINT('Ctrl Pts',(133.646659929478,34.7927740807523,29.9999999999998));
#58026=CARTESIAN_POINT('Ctrl Pts',(133.647456638038,34.7741685247524,29.9999999999998));
#58027=CARTESIAN_POINT('Ctrl Pts',(133.648145835737,34.7580736727038,29.9999999999998));
#58028=CARTESIAN_POINT('Ctrl Pts',(133.648728075031,34.7419763134874,29.9999999999998));
#58029=CARTESIAN_POINT('Ctrl Pts',(133.649202920447,34.725885226351,29.9999999999998));
#58030=CARTESIAN_POINT('Ctrl Pts',(133.652701331799,34.6073345568996,29.9999999999999));
#58031=CARTESIAN_POINT('Ctrl Pts',(133.650379787513,34.4889991098537,30.));
#58032=CARTESIAN_POINT('Ctrl Pts',(133.642173285556,34.3713070999481,30.));
#58033=CARTESIAN_POINT('Ctrl Pts',(133.63399714229,34.2540504735288,29.9999999999999));
#58034=CARTESIAN_POINT('Ctrl Pts',(133.619979819363,34.1374316460575,30.0000000000001));
#58035=CARTESIAN_POINT('Ctrl Pts',(133.600008773635,34.0218568079166,29.9999999999999));
#58036=CARTESIAN_POINT('Ctrl Pts',(133.596501616631,34.0015604694782,29.9999999999998));
#58037=CARTESIAN_POINT('Ctrl Pts',(133.592810721572,33.9812963033916,29.9999999999998));
#58038=CARTESIAN_POINT('Ctrl Pts',(133.58893531302,33.9610664860445,29.9999999999998));
#58039=CARTESIAN_POINT('Ctrl Pts',(133.567331333046,33.848292680912,29.9999999999999));
#58040=CARTESIAN_POINT('Ctrl Pts',(133.539997632525,33.736586010492,29.9999999999997));
#58041=CARTESIAN_POINT('Ctrl Pts',(133.50723292845,33.6262060673214,29.9999999999999));
#58042=CARTESIAN_POINT('Ctrl Pts',(133.486427399802,33.556115000282,29.9999999999999));
#58043=CARTESIAN_POINT('Ctrl Pts',(133.463430868005,33.4865589247505,30.));
#58044=CARTESIAN_POINT('Ctrl Pts',(133.438309219098,33.4176060315415,29.9999999999998));
#58045=CARTESIAN_POINT('Ctrl Pts',(133.432143579052,33.4006828303125,29.9999999999997));
#58046=CARTESIAN_POINT('Ctrl Pts',(133.425849892516,33.3837959724792,29.9999999999997));
#58047=CARTESIAN_POINT('Ctrl Pts',(133.419429062893,33.36694648716,29.9999999999998));
#58048=CARTESIAN_POINT('Ctrl Pts',(133.413620392469,33.3517034246926,29.9999999999998));
#58049=CARTESIAN_POINT('Ctrl Pts',(133.407709371309,33.3364955207696,30.));
#58050=CARTESIAN_POINT('Ctrl Pts',(133.401699885338,33.3213308991472,29.9999999999999));
#58051=CARTESIAN_POINT('Ctrl Pts',(133.358585042201,33.2125328612307,29.9999999999998));
#58052=CARTESIAN_POINT('Ctrl Pts',(133.310362255848,33.1058466822621,29.9999999999999));
#58053=CARTESIAN_POINT('Ctrl Pts',(133.257394148206,33.0015290590835,29.9999999999999));
#58054=CARTESIAN_POINT('Ctrl Pts',(133.20269552755,32.8938032906528,29.9999999999999));
#58055=CARTESIAN_POINT('Ctrl Pts',(133.14293630787,32.7886026856914,30.0000000000001));
#58056=CARTESIAN_POINT('Ctrl Pts',(133.078459117678,32.6862135768433,30.));
#58057=CARTESIAN_POINT('Ctrl Pts',(133.013981927485,32.5838244679953,29.9999999999999));
#58058=CARTESIAN_POINT('Ctrl Pts',(132.944786300179,32.4842461433536,29.9999999999999));
#58059=CARTESIAN_POINT('Ctrl Pts',(132.871164169375,32.387779114913,29.9999999999999));
#58060=CARTESIAN_POINT('Ctrl Pts',(132.817180895344,32.3170448672846,29.9999999999998));
#58061=CARTESIAN_POINT('Ctrl Pts',(132.760816619589,32.2479836595213,29.9999999999998));
#58062=CARTESIAN_POINT('Ctrl Pts',(132.702171320135,32.1807222077868,30.));
#58063=CARTESIAN_POINT('Ctrl Pts',(132.682391185113,32.1580359804248,30.0000000000001));
#58064=CARTESIAN_POINT('Ctrl Pts',(132.662351459987,32.1355545656877,30.));
#58065=CARTESIAN_POINT('Ctrl Pts',(132.64205568799,32.1132830596148,29.9999999999999));
#58066=CARTESIAN_POINT('Ctrl Pts',(132.629127996341,32.099096894973,29.9999999999999));
#58067=CARTESIAN_POINT('Ctrl Pts',(132.616095952342,32.0849954975785,30.));
#58068=CARTESIAN_POINT('Ctrl Pts',(132.602971467161,32.0709916880355,30.));
#58069=CARTESIAN_POINT('Ctrl Pts',(132.51706134301,31.9793256912457,30.));
#58070=CARTESIAN_POINT('Ctrl Pts',(132.42708576349,31.8917189352439,30.0000000000001));
#58071=CARTESIAN_POINT('Ctrl Pts',(132.333380954484,31.8084868081493,30.));
#58072=CARTESIAN_POINT('Ctrl Pts',(132.249610606485,31.7340788420559,30.));
#58073=CARTESIAN_POINT('Ctrl Pts',(132.162858888468,31.6631669226728,30.));
#58074=CARTESIAN_POINT('Ctrl Pts',(132.073335746272,31.595994443417,29.9999999999999));
#58075=CARTESIAN_POINT('Ctrl Pts',(132.035647395435,31.5677154989709,29.9999999999998));
#58076=CARTESIAN_POINT('Ctrl Pts',(131.997467538981,31.5400995537595,30.0000000000001));
#58077=CARTESIAN_POINT('Ctrl Pts',(131.958810535468,31.5131659774618,30.));
#58078=CARTESIAN_POINT('Ctrl Pts',(131.941207933923,31.5009016794395,30.));
#58079=CARTESIAN_POINT('Ctrl Pts',(131.923504430989,31.4887775667498,29.9999999999999));
#58080=CARTESIAN_POINT('Ctrl Pts',(131.905707752497,31.4767998318809,29.9999999999999));
#58081=CARTESIAN_POINT('Ctrl Pts',(131.800671830913,31.4061072910769,30.));
#58082=CARTESIAN_POINT('Ctrl Pts',(131.692537776855,31.3406064541469,29.9999999999999));
#58083=CARTESIAN_POINT('Ctrl Pts',(131.581620848268,31.2806265875096,30.));
#58084=CARTESIAN_POINT('Ctrl Pts',(131.47135331977,31.2209978929718,30.));
#58085=CARTESIAN_POINT('Ctrl Pts',(131.35833483295,31.1668249847331,29.9999999999999));
#58086=CARTESIAN_POINT('Ctrl Pts',(131.242839295058,31.1184677488179,29.9999999999999));
#58087=CARTESIAN_POINT('Ctrl Pts',(131.228328688645,31.1123922516138,29.9999999999999));
#58088=CARTESIAN_POINT('Ctrl Pts',(131.213778942246,31.1064086096793,30.));
#58089=CARTESIAN_POINT('Ctrl Pts',(131.199190565814,31.1005175866223,30.));
#58090=CARTESIAN_POINT('Ctrl Pts',(131.153580206964,31.0820993838236,30.0000000000001));
#58091=CARTESIAN_POINT('Ctrl Pts',(131.107592287516,31.0645864316864,29.9999999999999));
#58092=CARTESIAN_POINT('Ctrl Pts',(131.061251469589,31.0479717576683,30.));
#58093=CARTESIAN_POINT('Ctrl Pts',(128.941097384543,31.0506385600526,29.9977746450279));
#58094=CARTESIAN_POINT('Ctrl Pts',(127.636979564161,31.4002985726558,29.9320814941718));
#58095=CARTESIAN_POINT('Ctrl Pts',(125.424202813788,33.4879278405674,29.8006951924595));
#58096=CARTESIAN_POINT('Ctrl Pts',(126.226059929022,38.0051538371624,29.603615739891));
#58097=CARTESIAN_POINT('Ctrl Pts',(130.44507746161,39.800374185406,29.4065362873226));
#58098=CARTESIAN_POINT('Ctrl Pts',(134.258668943317,37.2607564345166,29.2094568347541));
#58099=CARTESIAN_POINT('Ctrl Pts',(134.225375111656,32.6766551184777,29.0123773821857));
#58100=CARTESIAN_POINT('Ctrl Pts',(130.372971419078,30.1928228717204,28.8152979296172));
#58101=CARTESIAN_POINT('Ctrl Pts',(126.183887676755,32.0527554421128,28.6182184770488));
#58102=CARTESIAN_POINT('Ctrl Pts',(125.443145000095,36.5762024021472,28.4211390244803));
#58103=CARTESIAN_POINT('Ctrl Pts',(128.820393548648,39.6751961014325,28.2240595719119));
#58104=CARTESIAN_POINT('Ctrl Pts',(133.26357927699,38.5493816503394,28.0269801193435));
#58105=CARTESIAN_POINT('Ctrl Pts',(134.757576919438,34.216068226713,27.829900666775));
#58106=CARTESIAN_POINT('Ctrl Pts',(131.952271869581,30.5911819197693,27.6328212142066));
#58107=CARTESIAN_POINT('Ctrl Pts',(127.382756390785,30.9504203203026,27.4357417616381));
#58108=CARTESIAN_POINT('Ctrl Pts',(125.178370646884,34.9691560811274,27.2386623090697));
#58109=CARTESIAN_POINT('Ctrl Pts',(127.331161511516,39.015763607638,27.0415828565013));
#58110=CARTESIAN_POINT('Ctrl Pts',(131.895708724517,39.4334351099692,26.8445034039328));
#58111=CARTESIAN_POINT('Ctrl Pts',(134.747155692316,35.8447314423668,26.6474239513644));
#58112=CARTESIAN_POINT('Ctrl Pts',(133.308726840317,31.4926670259735,26.4503444987959));
#58113=CARTESIAN_POINT('Ctrl Pts',(128.88029144574,30.3100841245265,26.2532650462275));
#58114=CARTESIAN_POINT('Ctrl Pts',(125.463706238897,33.3656508795297,26.056185593659));
#58115=CARTESIAN_POINT('Ctrl Pts',(126.146446541373,37.8981345429696,25.8591061410906));
#58116=CARTESIAN_POINT('Ctrl Pts',(130.311538460064,39.8116527210156,25.6620266885222));
#58117=CARTESIAN_POINT('Ctrl Pts',(134.19510153501,37.3770109853911,25.4649472359537));
#58118=CARTESIAN_POINT('Ctrl Pts',(134.287665263084,32.7943289680552,25.2678677833853));
#58119=CARTESIAN_POINT('Ctrl Pts',(130.505582318982,30.2048519697683,25.0707883308168));
#58120=CARTESIAN_POINT('Ctrl Pts',(126.266618361204,31.9486200414821,24.8737088782484));
#58121=CARTESIAN_POINT('Ctrl Pts',(125.401410016033,36.4498373257519,24.6766294256799));
#58122=CARTESIAN_POINT('Ctrl Pts',(128.691822571263,39.6408759870467,24.4795499731115));
#58123=CARTESIAN_POINT('Ctrl Pts',(133.164399547228,38.6380810350471,24.2824705205431));
#58124=CARTESIAN_POINT('Ctrl Pts',(134.777394577013,34.3476510384955,24.0853910679746));
#58125=CARTESIAN_POINT('Ctrl Pts',(132.073187850764,30.6467310848586,23.8883116154062));
#58126=CARTESIAN_POINT('Ctrl Pts',(127.495497558176,30.8797420431519,23.6912321628377));
#58127=CARTESIAN_POINT('Ctrl Pts',(125.181058116145,34.8361182374327,23.4941527102693));
#58128=CARTESIAN_POINT('Ctrl Pts',(127.221365603193,38.9405899305759,23.2970732577009));
#58129=CARTESIAN_POINT('Ctrl Pts',(131.772649544859,39.4840575044465,23.0999938051324));
#58130=CARTESIAN_POINT('Ctrl Pts',(134.722038226556,35.9754040696121,22.902914352564));
#58131=CARTESIAN_POINT('Ctrl Pts',(133.404249182998,31.5853044627455,22.7058348999955));
#58132=CARTESIAN_POINT('Ctrl Pts',(129.010132590199,30.2809724918095,22.5087554474271));
#58133=CARTESIAN_POINT('Ctrl Pts',(125.510532297232,33.2410975416826,22.3116759948586));
#58134=CARTESIAN_POINT('Ctrl Pts',(126.067942062277,37.7906949827236,22.1145965422902));
#58135=CARTESIAN_POINT('Ctrl Pts',(130.17864581635,39.8184171450895,21.9175170897218));
#58136=CARTESIAN_POINT('Ctrl Pts',(134.127912197006,37.4918665706579,21.7204376371533));
#58137=CARTESIAN_POINT('Ctrl Pts',(134.346896412782,32.9134838391122,21.5233581845849));
#58138=CARTESIAN_POINT('Ctrl Pts',(130.63770837377,30.2206291063118,21.3262787320164));
#58139=CARTESIAN_POINT('Ctrl Pts',(126.352240593858,31.8467620723114,21.129199279448));
#58140=CARTESIAN_POINT('Ctrl Pts',(125.363153938779,36.3223905339553,20.9321198268796));
#58141=CARTESIAN_POINT('Ctrl Pts',(128.564259164265,39.6030105735538,20.7350403743111));
#58142=CARTESIAN_POINT('Ctrl Pts',(133.062804393718,38.7240149543763,20.5379609217427));
#58143=CARTESIAN_POINT('Ctrl Pts',(134.793576466494,34.4797281235888,20.3408814691742));
#58144=CARTESIAN_POINT('Ctrl Pts',(132.192523632706,30.7055968965927,20.1438020166058));
#58145=CARTESIAN_POINT('Ctrl Pts',(127.610146760738,30.8122010707778,19.9467225640373));
#58146=CARTESIAN_POINT('Ctrl Pts',(125.187415297971,34.7032055790439,19.7496431114689));
#58147=CARTESIAN_POINT('Ctrl Pts',(127.113686096751,38.8624148252036,19.5525636589004));
#58148=CARTESIAN_POINT('Ctrl Pts',(131.64824009618,39.531265336693,19.355484206332));
#58149=CARTESIAN_POINT('Ctrl Pts',(134.693324896921,36.1053330286121,19.1584047537636));
#58150=CARTESIAN_POINT('Ctrl Pts',(133.497178144898,31.680544119862,18.9613253011951));
#58151=CARTESIAN_POINT('Ctrl Pts',(129.140729119686,30.2554514731342,18.7642458486267));
#58152=CARTESIAN_POINT('Ctrl Pts',(125.560774363793,33.117890665288,18.5671663960582));
#58153=CARTESIAN_POINT('Ctrl Pts',(125.992438636684,37.6811157912653,18.3700869434898));
#58154=CARTESIAN_POINT('Ctrl Pts',(130.045603791983,39.8215414336961,18.1730074909214));
#58155=CARTESIAN_POINT('Ctrl Pts',(134.057606652229,37.6047633296345,17.9759280383529));
#58156=CARTESIAN_POINT('Ctrl Pts',(134.40276000298,33.0343540557215,17.7788485857845));
#58157=CARTESIAN_POINT('Ctrl Pts',(130.76946668054,30.2397849523119,17.581769133216));
#58158=CARTESIAN_POINT('Ctrl Pts',(126.440396857374,31.7478458997171,17.3846896806476));
#58159=CARTESIAN_POINT('Ctrl Pts',(125.328932767176,36.1928190026923,17.1876102280791));
#58160=CARTESIAN_POINT('Ctrl Pts',(128.436719226379,39.5639595163822,16.9905307755107));
#58161=CARTESIAN_POINT('Ctrl Pts',(132.961965747045,38.80210666434,16.793404651506));
#58162=CARTESIAN_POINT('Ctrl Pts',(134.185068670941,36.0149711949963,16.6619716783574));
#58163=CARTESIAN_POINT('Ctrl Pts',(134.075375956471,34.6682761845988,16.5962318560649));
#58164=CARTESIAN_POINT('Ctrl Pts',(129.001973237821,31.2776856407296,30.1334903360346));
#58165=CARTESIAN_POINT('Ctrl Pts',(127.772828586768,31.6072438504722,30.0677971851784));
#58166=CARTESIAN_POINT('Ctrl Pts',(125.68726341452,33.5748562148862,29.9364108834662));
#58167=CARTESIAN_POINT('Ctrl Pts',(126.443022111084,37.8323888431025,29.7393314308977));
#58168=CARTESIAN_POINT('Ctrl Pts',(130.419490150884,39.5244027501432,29.5422519783293));
#58169=CARTESIAN_POINT('Ctrl Pts',(134.013839908078,37.1307865251062,29.3451725257608));
#58170=CARTESIAN_POINT('Ctrl Pts',(133.982460124397,32.8102232106304,29.1480930731924));
#58171=CARTESIAN_POINT('Ctrl Pts',(130.351529453544,30.4691854052259,28.9510136206239));
#58172=CARTESIAN_POINT('Ctrl Pts',(126.403274323357,32.2221912567589,28.7539341680555));
#58173=CARTESIAN_POINT('Ctrl Pts',(125.705116622731,36.4855872079176,28.5568547154871));
#58174=CARTESIAN_POINT('Ctrl Pts',(128.888208613234,39.406421100065,28.3597752629186));
#58175=CARTESIAN_POINT('Ctrl Pts',(133.075957516191,38.3453292347345,28.1626958103502));
#58176=CARTESIAN_POINT('Ctrl Pts',(134.484065880482,34.2611361252281,27.9656163577817));
#58177=CARTESIAN_POINT('Ctrl Pts',(131.840036604358,30.8446429639338,27.7685369052133));
#58178=CARTESIAN_POINT('Ctrl Pts',(127.533220593652,31.1832289042281,27.5714574526448));
#58179=CARTESIAN_POINT('Ctrl Pts',(125.455564032542,34.9709292846803,27.3743780000764));
#58180=CARTESIAN_POINT('Ctrl Pts',(127.484591881671,38.7848990950663,27.177298547508));
#58181=CARTESIAN_POINT('Ctrl Pts',(131.786725250034,39.1785588434143,26.9802190949395));
#58182=CARTESIAN_POINT('Ctrl Pts',(134.474243765198,35.7961681971786,26.7831396423711));
#58183=CARTESIAN_POINT('Ctrl Pts',(133.118509565632,31.6943020813675,26.5860601898026));
#58184=CARTESIAN_POINT('Ctrl Pts',(128.944663006135,30.5797053593359,26.3889807372342));
#58185=CARTESIAN_POINT('Ctrl Pts',(125.724495804809,33.4596089034412,26.1919012846657));
#58186=CARTESIAN_POINT('Ctrl Pts',(126.367985662651,37.7315220418359,25.9948218320973));
#58187=CARTESIAN_POINT('Ctrl Pts',(130.293628248766,39.5350328876198,25.7977423795289));
#58188=CARTESIAN_POINT('Ctrl Pts',(133.953926962576,37.240357652143,25.6006629269604));
#58189=CARTESIAN_POINT('Ctrl Pts',(134.041169241965,32.9211320415018,25.403583474392));
#58190=CARTESIAN_POINT('Ctrl Pts',(130.47651661018,30.4805229556309,25.2065040218235));
#58191=CARTESIAN_POINT('Ctrl Pts',(126.481248856545,32.1240425552611,25.0094245692551));
#58192=CARTESIAN_POINT('Ctrl Pts',(125.665780964847,36.3664868050984,24.8123451166866));
#58193=CARTESIAN_POINT('Ctrl Pts',(128.767029125719,39.3740740342083,24.6152656641182));
#58194=CARTESIAN_POINT('Ctrl Pts',(132.982479586188,38.428929330187,24.4181862115498));
#58195=CARTESIAN_POINT('Ctrl Pts',(134.502744229496,34.3851542980842,24.2211067589813));
#58196=CARTESIAN_POINT('Ctrl Pts',(131.95400117809,30.8969986315528,24.0240273064129));
#58197=CARTESIAN_POINT('Ctrl Pts',(127.639480320101,31.1166138906552,23.8269478538444));
#58198=CARTESIAN_POINT('Ctrl Pts',(125.45809700036,34.8455397290669,23.629868401276));
#58199=CARTESIAN_POINT('Ctrl Pts',(127.38110809262,38.7140471201781,23.4327889487075));
#58200=CARTESIAN_POINT('Ctrl Pts',(131.670740689378,39.2262709783325,23.2357094961391));
#58201=CARTESIAN_POINT('Ctrl Pts',(134.450570291679,35.9193285116128,23.0386300435706));
#58202=CARTESIAN_POINT('Ctrl Pts',(133.208540370156,31.7816138319748,22.8415505910022));
#58203=CARTESIAN_POINT('Ctrl Pts',(129.067039639369,30.5522673417899,22.6444711384338));
#58204=CARTESIAN_POINT('Ctrl Pts',(125.768629853308,33.3422160831047,22.4473916858653));
#58205=CARTESIAN_POINT('Ctrl Pts',(126.293994372097,37.6302591354298,22.2503122332969));
#58206=CARTESIAN_POINT('Ctrl Pts',(130.168375545651,39.54140842788,22.0532327807285));
#58207=CARTESIAN_POINT('Ctrl Pts',(133.890600310547,37.3486102394997,21.85615332816));
#58208=CARTESIAN_POINT('Ctrl Pts',(134.096995218492,33.0334367505684,21.6590738755916));
#58209=CARTESIAN_POINT('Ctrl Pts',(130.601046795236,30.4953930714198,21.4619944230231));
#58210=CARTESIAN_POINT('Ctrl Pts',(126.561948704086,32.028040356674,21.2649149704547));
#58211=CARTESIAN_POINT('Ctrl Pts',(125.629724212925,36.2463668742282,21.0678355178862));
#58212=CARTESIAN_POINT('Ctrl Pts',(128.646799283805,39.3383854869563,20.8707560653178));
#58213=CARTESIAN_POINT('Ctrl Pts',(132.886725094102,38.5099229456693,20.6736766127494));
#58214=CARTESIAN_POINT('Ctrl Pts',(134.51799582915,34.5096383286925,20.4765971601809));
#58215=CARTESIAN_POINT('Ctrl Pts',(132.066476397554,30.9524802732359,20.2795177076125));
#58216=CARTESIAN_POINT('Ctrl Pts',(127.747538389606,31.0529558195643,20.082438255044));
#58217=CARTESIAN_POINT('Ctrl Pts',(125.464088710552,34.7202681619105,19.8853588024756));
#58218=CARTESIAN_POINT('Ctrl Pts',(127.279619034421,38.6403662677949,19.6882793499071));
#58219=CARTESIAN_POINT('Ctrl Pts',(131.553483486084,39.2707648527254,19.4911998973387));
#58220=CARTESIAN_POINT('Ctrl Pts',(134.423507678942,36.0417879109675,19.2941204447703));
#58221=CARTESIAN_POINT('Ctrl Pts',(133.296126886236,31.8713782024045,19.0970409922018));
#58222=CARTESIAN_POINT('Ctrl Pts',(129.190128230872,30.5282135154378,18.8999615396334));
#58223=CARTESIAN_POINT('Ctrl Pts',(125.815983525196,33.2260923167344,18.7028820870649));
#58224=CARTESIAN_POINT('Ctrl Pts',(126.222831605778,37.5269796042843,18.5058026344965));
#58225=CARTESIAN_POINT('Ctrl Pts',(130.04298204971,39.5443531024862,18.3087231819281));
#58226=CARTESIAN_POINT('Ctrl Pts',(133.824336601125,37.4550166126422,18.1116437293596));
#58227=CARTESIAN_POINT('Ctrl Pts',(134.149647235057,33.1473581907137,17.9145642767912));
#58228=CARTESIAN_POINT('Ctrl Pts',(130.725230373951,30.5134476561202,17.7174848242227));
#58229=CARTESIAN_POINT('Ctrl Pts',(126.645036902149,31.9348108320508,17.5204053716543));
#58230=CARTESIAN_POINT('Ctrl Pts',(125.597470401674,36.1242443542447,17.3233259190859));
#58231=CARTESIAN_POINT('Ctrl Pts',(128.526591561774,39.3015794581679,17.1262464665174));
#58232=CARTESIAN_POINT('Ctrl Pts',(132.791683617603,38.5835251970098,16.9291203425127));
#58233=CARTESIAN_POINT('Ctrl Pts',(133.944470883522,35.9566209400755,16.7976873693641));
#58234=CARTESIAN_POINT('Ctrl Pts',(133.841084355752,34.6873468432416,16.7319475470716));
#58235=CARTESIAN_POINT('Ctrl Pts',(129.062849091099,31.5047327214066,30.2692060270413));
#58236=CARTESIAN_POINT('Ctrl Pts',(127.908677609375,31.8141891282886,30.2035128761852));
#58237=CARTESIAN_POINT('Ctrl Pts',(125.950324015252,33.661784589205,30.072126574473));
#58238=CARTESIAN_POINT('Ctrl Pts',(126.659984293147,37.6596238490425,29.8750471219045));
#58239=CARTESIAN_POINT('Ctrl Pts',(130.393902840157,39.2484313148805,29.6779676693361));
#58240=CARTESIAN_POINT('Ctrl Pts',(133.76901087284,37.0008166156958,29.4808882167676));
#58241=CARTESIAN_POINT('Ctrl Pts',(133.739545137138,32.9437913027832,29.2838087641992));
#58242=CARTESIAN_POINT('Ctrl Pts',(130.330087488009,30.7455479387316,29.0867293116307));
#58243=CARTESIAN_POINT('Ctrl Pts',(126.622660969959,32.3916270714049,28.8896498590623));
#58244=CARTESIAN_POINT('Ctrl Pts',(125.967088245366,36.3949720136881,28.6925704064939));
#58245=CARTESIAN_POINT('Ctrl Pts',(128.956023677822,39.1376460986974,28.4954909539254));
#58246=CARTESIAN_POINT('Ctrl Pts',(132.888335755391,38.1412768191297,28.298411501357));
#58247=CARTESIAN_POINT('Ctrl Pts',(134.210554841525,34.3062040237431,28.1013320487885));
#58248=CARTESIAN_POINT('Ctrl Pts',(131.727801339134,31.0981040080983,27.9042525962201));
#58249=CARTESIAN_POINT('Ctrl Pts',(127.683684796518,31.4160374881537,27.7071731436516));
#58250=CARTESIAN_POINT('Ctrl Pts',(125.732757418202,34.972702488233,27.5100936910832));
#58251=CARTESIAN_POINT('Ctrl Pts',(127.638022251826,38.5540345824945,27.3130142385148));
#58252=CARTESIAN_POINT('Ctrl Pts',(131.67774177555,38.9236825768594,27.1159347859463));
#58253=CARTESIAN_POINT('Ctrl Pts',(134.201331838081,35.7476049519903,26.9188553333779));
#58254=CARTESIAN_POINT('Ctrl Pts',(132.928292290948,31.8959371367615,26.7217758808094));
#58255=CARTESIAN_POINT('Ctrl Pts',(129.00903456653,30.8493265941452,26.524696428241));
#58256=CARTESIAN_POINT('Ctrl Pts',(125.985285370721,33.5535669273527,26.3276169756725));
#58257=CARTESIAN_POINT('Ctrl Pts',(126.589524783929,37.5649095407024,26.1305375231041));
#58258=CARTESIAN_POINT('Ctrl Pts',(130.27571803747,39.2584130542239,25.9334580705357));
#58259=CARTESIAN_POINT('Ctrl Pts',(133.712752390142,37.103704318895,25.7363786179672));
#58260=CARTESIAN_POINT('Ctrl Pts',(133.794673220847,33.0479351149484,25.5392991653988));
#58261=CARTESIAN_POINT('Ctrl Pts',(130.447450901378,30.7561939414936,25.3422197128302));
#58262=CARTESIAN_POINT('Ctrl Pts',(126.695879351888,32.2994650690403,25.1451402602619));
#58263=CARTESIAN_POINT('Ctrl Pts',(125.930151913661,36.2831362844449,24.9480608076934));
#58264=CARTESIAN_POINT('Ctrl Pts',(128.842235680176,39.1072720813698,24.750981355125));
#58265=CARTESIAN_POINT('Ctrl Pts',(132.800559625146,38.2197776253269,24.5539019025566));
#58266=CARTESIAN_POINT('Ctrl Pts',(134.228093881978,34.4226575576729,24.3568224499881));
#58267=CARTESIAN_POINT('Ctrl Pts',(131.834814505417,31.1472661782472,24.1597429974197));
#58268=CARTESIAN_POINT('Ctrl Pts',(127.783463082027,31.3534857381584,23.9626635448512));
#58269=CARTESIAN_POINT('Ctrl Pts',(125.735135884574,34.8549612207012,23.7655840922828));
#58270=CARTESIAN_POINT('Ctrl Pts',(127.540850582046,38.4875043097803,23.5685046397144));
#58271=CARTESIAN_POINT('Ctrl Pts',(131.568831833898,38.9684844522186,23.3714251871459));
#58272=CARTESIAN_POINT('Ctrl Pts',(134.179102356802,35.8632529536134,23.1743457345775));
#58273=CARTESIAN_POINT('Ctrl Pts',(133.012831557314,31.977923201204,22.977266282009));
#58274=CARTESIAN_POINT('Ctrl Pts',(129.123946688539,30.8235621917705,22.7801868294405));
#58275=CARTESIAN_POINT('Ctrl Pts',(126.026727409382,33.4433346245269,22.5831073768721));
#58276=CARTESIAN_POINT('Ctrl Pts',(126.520046681916,37.4698232881361,22.3860279243037));
#58277=CARTESIAN_POINT('Ctrl Pts',(130.158105274952,39.2643997106705,22.1889484717353));
#58278=CARTESIAN_POINT('Ctrl Pts',(133.653288424089,37.2053539083415,21.9918690191668));
#58279=CARTESIAN_POINT('Ctrl Pts',(133.847094024202,33.1533896620248,21.7947895665984));
#58280=CARTESIAN_POINT('Ctrl Pts',(130.564385216702,30.7701570365278,21.5977101140299));
#58281=CARTESIAN_POINT('Ctrl Pts',(126.771656814313,32.2093186410366,21.4006306614615));
#58282=CARTESIAN_POINT('Ctrl Pts',(125.896294487071,36.1703432145012,21.203551208893));
#58283=CARTESIAN_POINT('Ctrl Pts',(128.729339403346,39.0737604003589,21.0064717563246));
#58284=CARTESIAN_POINT('Ctrl Pts',(132.710645794485,38.2958309369622,20.8093923037562));
#58285=CARTESIAN_POINT('Ctrl Pts',(134.242415191807,34.5395485337962,20.6123128511877));
#58286=CARTESIAN_POINT('Ctrl Pts',(131.940429162402,31.1993636498791,20.4152333986193));
#58287=CARTESIAN_POINT('Ctrl Pts',(127.884930018473,31.2937105683511,20.2181539460508));
#58288=CARTESIAN_POINT('Ctrl Pts',(125.740762123133,34.7373307447771,20.0210744934824));
#58289=CARTESIAN_POINT('Ctrl Pts',(127.44555197209,38.4183177103862,19.8239950409139));
#58290=CARTESIAN_POINT('Ctrl Pts',(131.458726875989,39.0102643687579,19.6269155883455));
#58291=CARTESIAN_POINT('Ctrl Pts',(134.153690460965,35.978242793323,19.429836135777));
#58292=CARTESIAN_POINT('Ctrl Pts',(133.095075627576,32.0622122849472,19.2327566832086));
#58293=CARTESIAN_POINT('Ctrl Pts',(129.239527342058,30.8009755577414,19.0356772306402));
#58294=CARTESIAN_POINT('Ctrl Pts',(126.071192686599,33.3342939681808,18.8385977780717));
#58295=CARTESIAN_POINT('Ctrl Pts',(126.453224574871,37.3728434173031,18.6415183255033));
#58296=CARTESIAN_POINT('Ctrl Pts',(130.040360307437,39.2671647712763,18.4444388729348));
#58297=CARTESIAN_POINT('Ctrl Pts',(133.591066550021,37.3052698956499,18.2473594203664));
#58298=CARTESIAN_POINT('Ctrl Pts',(133.896534467132,33.260362325706,18.050279967798));
#58299=CARTESIAN_POINT('Ctrl Pts',(130.680994067359,30.7871103599285,17.8532005152295));
#58300=CARTESIAN_POINT('Ctrl Pts',(126.849676946924,32.1217757643844,17.6561210626611));
#58301=CARTESIAN_POINT('Ctrl Pts',(125.866008036171,36.055669705797,17.4590416100926));
#58302=CARTESIAN_POINT('Ctrl Pts',(128.61646389717,39.0391993999536,17.2619621575242));
#58303=CARTESIAN_POINT('Ctrl Pts',(132.621401488161,38.3649437296796,17.0648360335194));
#58304=CARTESIAN_POINT('Ctrl Pts',(133.703873096103,35.8982706851548,16.9334030603708));
#58305=CARTESIAN_POINT('Ctrl Pts',(133.606792755035,34.7064175018843,16.8676632380784));
#58306=CARTESIAN_POINT('Ctrl Pts',(129.123724944377,31.7317798020836,30.4049217180481));
#58307=CARTESIAN_POINT('Ctrl Pts',(128.044526631981,32.021134406105,30.3392285671919));
#58308=CARTESIAN_POINT('Ctrl Pts',(126.213384615984,33.7487129635239,30.2078422654796));
#58309=CARTESIAN_POINT('Ctrl Pts',(126.876946475209,37.4868588549827,30.0107628129112));
#58310=CARTESIAN_POINT('Ctrl Pts',(130.368315529432,38.9724598796177,29.8136833603428));
#58311=CARTESIAN_POINT('Ctrl Pts',(133.524181837602,36.8708467062855,29.6166039077743));
#58312=CARTESIAN_POINT('Ctrl Pts',(133.496630149878,33.077359394936,29.4195244552059));
#58313=CARTESIAN_POINT('Ctrl Pts',(130.308645522475,31.0219104722371,29.2224450026374));
#58314=CARTESIAN_POINT('Ctrl Pts',(126.842047616561,32.5610628860511,29.025365550069));
#58315=CARTESIAN_POINT('Ctrl Pts',(126.229059868002,36.3043568194586,28.8282860975006));
#58316=CARTESIAN_POINT('Ctrl Pts',(129.023838742409,38.8688710973299,28.6312066449321));
#58317=CARTESIAN_POINT('Ctrl Pts',(132.70071399459,37.9372244035248,28.4341271923637));
#58318=CARTESIAN_POINT('Ctrl Pts',(133.937043802569,34.3512719222581,28.2370477397952));
#58319=CARTESIAN_POINT('Ctrl Pts',(131.615566073911,31.351565052263,28.0399682872268));
#58320=CARTESIAN_POINT('Ctrl Pts',(127.834148999385,31.6488460720792,27.8428888346583));
#58321=CARTESIAN_POINT('Ctrl Pts',(126.009950803862,34.9744756917859,27.6458093820899));
#58322=CARTESIAN_POINT('Ctrl Pts',(127.791452621982,38.3231700699227,27.4487299295215));
#58323=CARTESIAN_POINT('Ctrl Pts',(131.568758301068,38.6688063103047,27.251650476953));
#58324=CARTESIAN_POINT('Ctrl Pts',(133.928419910963,35.6990417068019,27.0545710243846));
#58325=CARTESIAN_POINT('Ctrl Pts',(132.738075016263,32.0975721921556,26.8574915718161));
#58326=CARTESIAN_POINT('Ctrl Pts',(129.073406126925,31.1189478289545,26.6604121192477));
#58327=CARTESIAN_POINT('Ctrl Pts',(126.246074936632,33.6475249512642,26.4633326666792));
#58328=CARTESIAN_POINT('Ctrl Pts',(126.811063905207,37.3982970395687,26.2662532141108));
#58329=CARTESIAN_POINT('Ctrl Pts',(130.257807826173,38.9817932208281,26.0691737615424));
#58330=CARTESIAN_POINT('Ctrl Pts',(133.471577817707,36.9670509856468,25.8720943089739));
#58331=CARTESIAN_POINT('Ctrl Pts',(133.54817719973,33.174738188395,25.6750148564055));
#58332=CARTESIAN_POINT('Ctrl Pts',(130.418385192576,31.0318649273562,25.477935403837));
#58333=CARTESIAN_POINT('Ctrl Pts',(126.910509847231,32.4748875828193,25.2808559512686));
#58334=CARTESIAN_POINT('Ctrl Pts',(126.194522862476,36.1997857637913,25.0837764987001));
#58335=CARTESIAN_POINT('Ctrl Pts',(128.917442234633,38.8404701285314,24.8866970461317));
#58336=CARTESIAN_POINT('Ctrl Pts',(132.618639664104,38.0106259204668,24.6896175935632));
#58337=CARTESIAN_POINT('Ctrl Pts',(133.953443534461,34.4601608172618,24.4925381409948));
#58338=CARTESIAN_POINT('Ctrl Pts',(131.715627832744,31.3975337249415,24.2954586884264));
#58339=CARTESIAN_POINT('Ctrl Pts',(127.927445843952,31.5903575856617,24.0983792358579));
#58340=CARTESIAN_POINT('Ctrl Pts',(126.012174768787,34.8643827123355,23.9012997832895));
#58341=CARTESIAN_POINT('Ctrl Pts',(127.700593071473,38.2609614993825,23.704220330721));
#58342=CARTESIAN_POINT('Ctrl Pts',(131.466922978418,38.7106979261046,23.5071408781526));
#58343=CARTESIAN_POINT('Ctrl Pts',(133.907634421926,35.8071773956141,23.3100614255842));
#58344=CARTESIAN_POINT('Ctrl Pts',(132.817122744472,32.1742325704332,23.1129819730157));
#58345=CARTESIAN_POINT('Ctrl Pts',(129.180853737708,31.0948570417509,22.9159025204473));
#58346=CARTESIAN_POINT('Ctrl Pts',(126.284824965458,33.5444531659491,22.7188230678788));
#58347=CARTESIAN_POINT('Ctrl Pts',(126.746098991737,37.3093874408423,22.5217436153104));
#58348=CARTESIAN_POINT('Ctrl Pts',(130.147835004252,38.987390993461,22.324664162742));
#58349=CARTESIAN_POINT('Ctrl Pts',(133.415976537629,37.0620975771833,22.1275847101735));
#58350=CARTESIAN_POINT('Ctrl Pts',(133.59719282991,33.273342573481,21.9305052576051));
#58351=CARTESIAN_POINT('Ctrl Pts',(130.527723638169,31.0449210016357,21.7334258050366));
#58352=CARTESIAN_POINT('Ctrl Pts',(126.981364924541,32.3905969253993,21.5363463524682));
#58353=CARTESIAN_POINT('Ctrl Pts',(126.162864761217,36.0943195547742,21.3392668998997));
#58354=CARTESIAN_POINT('Ctrl Pts',(128.811879522886,38.8091353137614,21.1421874473313));
#58355=CARTESIAN_POINT('Ctrl Pts',(132.534566494868,38.0817389282551,20.9451079947628));
#58356=CARTESIAN_POINT('Ctrl Pts',(133.966834554464,34.5694587389,20.7480285421944));
#58357=CARTESIAN_POINT('Ctrl Pts',(131.81438192725,31.4462470265224,20.550949089626));
#58358=CARTESIAN_POINT('Ctrl Pts',(128.022321647341,31.5344653171377,20.3538696370575));
#58359=CARTESIAN_POINT('Ctrl Pts',(126.017435535714,34.7543933276437,20.1567901844891));
#58360=CARTESIAN_POINT('Ctrl Pts',(127.61148490976,38.1962691529774,19.9597107319206));
#58361=CARTESIAN_POINT('Ctrl Pts',(131.363970265893,38.7497638847903,19.7626312793522));
#58362=CARTESIAN_POINT('Ctrl Pts',(133.883873242987,35.9146976756785,19.5655518267837));
#58363=CARTESIAN_POINT('Ctrl Pts',(132.894024368916,32.2530463674897,19.3684723742153));
#58364=CARTESIAN_POINT('Ctrl Pts',(129.288926453244,31.073737600045,19.1713929216469));
#58365=CARTESIAN_POINT('Ctrl Pts',(126.326401848002,33.4424956196272,18.9743134690784));
#58366=CARTESIAN_POINT('Ctrl Pts',(126.683617543965,37.218707230322,18.77723401651));
#58367=CARTESIAN_POINT('Ctrl Pts',(130.037738565164,38.9899764400662,18.5801545639415));
#58368=CARTESIAN_POINT('Ctrl Pts',(133.357796498917,37.1555231786576,18.3830751113731));
#58369=CARTESIAN_POINT('Ctrl Pts',(133.643421699208,33.3733664606983,18.1859956588046));
#58370=CARTESIAN_POINT('Ctrl Pts',(130.636757760769,31.0607730637369,17.9889162062362));
#58371=CARTESIAN_POINT('Ctrl Pts',(127.054316991698,32.3087406967181,17.7918367536678));
#58372=CARTESIAN_POINT('Ctrl Pts',(126.134545670668,35.9870950573493,17.5947573010993));
#58373=CARTESIAN_POINT('Ctrl Pts',(128.706336232565,38.7768193417394,17.3976778485309));
#58374=CARTESIAN_POINT('Ctrl Pts',(132.451119358719,38.1463622623494,17.2005517245261));
#58375=CARTESIAN_POINT('Ctrl Pts',(133.463275308683,35.839920430234,17.0691187513775));
#58376=CARTESIAN_POINT('Ctrl Pts',(133.372501154318,34.7254881605269,17.0033789290851));
#58377=CARTESIAN_POINT('',(127.424194198253,37.2080440111198,30.0017033528262));
#58378=CARTESIAN_POINT('Ctrl Pts',(127.426413840714,37.2061412790735,30.0017033528262));
#58379=CARTESIAN_POINT('Ctrl Pts',(127.438461580037,37.220195635187,30.0011355685508));
#58380=CARTESIAN_POINT('Ctrl Pts',(127.450624448196,37.234151300005,30.0005677842754));
#58381=CARTESIAN_POINT('Ctrl Pts',(127.462900812983,37.2480064007332,30.));
#58382=CARTESIAN_POINT('Ctrl Pts',(128.942095577027,31.0543614925016,30.));
#58383=CARTESIAN_POINT('Ctrl Pts',(128.825609397642,31.0963697647221,30.));
#58384=CARTESIAN_POINT('Ctrl Pts',(128.7115241043,31.1439906471432,30.0000000000001));
#58385=CARTESIAN_POINT('Ctrl Pts',(128.600069328297,31.1968590882299,30.0000000000001));
#58386=CARTESIAN_POINT('Ctrl Pts',(128.486962920038,31.2505109791227,30.0000000000001));
#58387=CARTESIAN_POINT('Ctrl Pts',(128.376564964256,31.309567722175,30.0000000000001));
#58388=CARTESIAN_POINT('Ctrl Pts',(128.269143169485,31.3736951260073,30.0000000000001));
#58389=CARTESIAN_POINT('Ctrl Pts',(128.161272060922,31.4380907559205,30.0000000000001));
#58390=CARTESIAN_POINT('Ctrl Pts',(128.056401487506,31.5076002570416,30.));
#58391=CARTESIAN_POINT('Ctrl Pts',(127.954839131891,31.581922498923,30.));
#58392=CARTESIAN_POINT('Ctrl Pts',(127.858557800154,31.6523801442061,30.));
#58393=CARTESIAN_POINT('Ctrl Pts',(127.765249473048,31.7271638358833,30.));
#58394=CARTESIAN_POINT('Ctrl Pts',(127.675213472941,31.8060391429531,30.));
#58395=CARTESIAN_POINT('Ctrl Pts',(127.65810181963,31.8210296679401,30.));
#58396=CARTESIAN_POINT('Ctrl Pts',(127.641108479803,31.8361680316025,30.0000000000001));
#58397=CARTESIAN_POINT('Ctrl Pts',(127.624235676082,31.8514526866952,30.));
#58398=CARTESIAN_POINT('Ctrl Pts',(127.613109396249,31.8615317080905,29.9999999999999));
#58399=CARTESIAN_POINT('Ctrl Pts',(127.602036828276,31.8716732131105,30.));
#58400=CARTESIAN_POINT('Ctrl Pts',(127.591025310482,31.8818703533532,30.));
#58401=CARTESIAN_POINT('Ctrl Pts',(127.50054824138,31.9656560202932,30.));
#58402=CARTESIAN_POINT('Ctrl Pts',(127.414059076834,32.0533125866699,30.));
#58403=CARTESIAN_POINT('Ctrl Pts',(127.331814436228,32.1445238770439,30.0000000000001));
#58404=CARTESIAN_POINT('Ctrl Pts',(127.250266160805,32.2349628816326,30.0000000000002));
#58405=CARTESIAN_POINT('Ctrl Pts',(127.172890401673,32.3288974156517,29.9999999999999));
#58406=CARTESIAN_POINT('Ctrl Pts',(127.099979115674,32.4260477080103,30.));
#58407=CARTESIAN_POINT('Ctrl Pts',(127.027478544049,32.5226507459768,30.0000000000001));
#58408=CARTESIAN_POINT('Ctrl Pts',(126.959391861292,32.6224340934605,29.9999999999998));
#58409=CARTESIAN_POINT('Ctrl Pts',(126.896054072652,32.7251403611992,29.9999999999999));
#58410=CARTESIAN_POINT('Ctrl Pts',(126.84349765552,32.8103639467586,29.9999999999999));
#58411=CARTESIAN_POINT('Ctrl Pts',(126.794211742569,32.8976005531388,30.0000000000002));
#58412=CARTESIAN_POINT('Ctrl Pts',(126.748416226718,32.9867074968054,30.));
#58413=CARTESIAN_POINT('Ctrl Pts',(126.738576987573,33.0058522648458,29.9999999999999));
#58414=CARTESIAN_POINT('Ctrl Pts',(126.728898970669,33.0250833755648,29.9999999999999));
#58415=CARTESIAN_POINT('Ctrl Pts',(126.719384526347,33.0443994188612,30.));
#58416=CARTESIAN_POINT('Ctrl Pts',(126.712239720925,33.0589046664819,30.0000000000001));
#58417=CARTESIAN_POINT('Ctrl Pts',(126.705188026154,33.0734561576526,30.0000000000002));
#58418=CARTESIAN_POINT('Ctrl Pts',(126.69823518144,33.0880428789924,30.0000000000002));
#58419=CARTESIAN_POINT('Ctrl Pts',(126.647578219101,33.1943186587582,29.9999999999999));
#58420=CARTESIAN_POINT('Ctrl Pts',(126.602089235897,33.3026149502714,30.0000000000002));
#58421=CARTESIAN_POINT('Ctrl Pts',(126.562038428248,33.4126741616684,30.0000000000001));
#58422=CARTESIAN_POINT('Ctrl Pts',(126.522813048182,33.5204651064788,30.));
#58423=CARTESIAN_POINT('Ctrl Pts',(126.488803776214,33.6299476902416,30.0000000000001));
#58424=CARTESIAN_POINT('Ctrl Pts',(126.460313221096,33.7408906127765,30.0000000000002));
#58425=CARTESIAN_POINT('Ctrl Pts',(126.452962461272,33.7695146523725,30.0000000000002));
#58426=CARTESIAN_POINT('Ctrl Pts',(126.445979335698,33.798235932397,30.0000000000002));
#58427=CARTESIAN_POINT('Ctrl Pts',(126.43936961117,33.8270505216889,30.0000000000001));
#58428=CARTESIAN_POINT('Ctrl Pts',(126.412872443509,33.942562900497,30.));
#58429=CARTESIAN_POINT('Ctrl Pts',(126.392372079654,34.0595756139416,30.0000000000003));
#58430=CARTESIAN_POINT('Ctrl Pts',(126.377782167101,34.1776518198943,30.0000000000002));
#58431=CARTESIAN_POINT('Ctrl Pts',(126.369641800959,34.243531827449,30.0000000000002));
#58432=CARTESIAN_POINT('Ctrl Pts',(126.363342301581,34.3097427527037,30.0000000000003));
#58433=CARTESIAN_POINT('Ctrl Pts',(126.358875354926,34.3762065420342,30.0000000000001));
#58434=CARTESIAN_POINT('Ctrl Pts',(126.357511103473,34.3965052668978,30.0000000000001));
#58435=CARTESIAN_POINT('Ctrl Pts',(126.356317816527,34.4168275625855,30.));
#58436=CARTESIAN_POINT('Ctrl Pts',(126.355295341418,34.4371711620536,29.9999999999999));
#58437=CARTESIAN_POINT('Ctrl Pts',(126.354567496136,34.4516526812134,29.9999999999999));
#58438=CARTESIAN_POINT('Ctrl Pts',(126.353926326219,34.4661433569147,30.));
#58439=CARTESIAN_POINT('Ctrl Pts',(126.3533719768,34.4806329555477,30.));
#58440=CARTESIAN_POINT('Ctrl Pts',(126.348947719107,34.5962743110845,30.0000000000001));
#58441=CARTESIAN_POINT('Ctrl Pts',(126.350040381804,34.7120147207867,29.9999999999999));
#58442=CARTESIAN_POINT('Ctrl Pts',(126.356503489409,34.8274542927884,30.));
#58443=CARTESIAN_POINT('Ctrl Pts',(126.363113345688,34.9455149884253,30.0000000000001));
#58444=CARTESIAN_POINT('Ctrl Pts',(126.375340459208,35.0632620236151,30.0000000000001));
#58445=CARTESIAN_POINT('Ctrl Pts',(126.393082807289,35.1802576232764,30.0000000000001));
#58446=CARTESIAN_POINT('Ctrl Pts',(126.41082515537,35.2972532229377,30.0000000000001));
#58447=CARTESIAN_POINT('Ctrl Pts',(126.43408309937,35.4134983511588,30.0000000000001));
#58448=CARTESIAN_POINT('Ctrl Pts',(126.462804371977,35.5285305607672,30.0000000000002));
#58449=CARTESIAN_POINT('Ctrl Pts',(126.481403668795,35.6030230193498,30.0000000000002));
#58450=CARTESIAN_POINT('Ctrl Pts',(126.502295055159,35.6770062918083,30.0000000000003));
#58451=CARTESIAN_POINT('Ctrl Pts',(126.525474399776,35.7503463986096,30.0000000000001));
#58452=CARTESIAN_POINT('Ctrl Pts',(126.532574556592,35.7728114970735,30.));
#58453=CARTESIAN_POINT('Ctrl Pts',(126.539889441554,35.7952161935211,30.0000000000002));
#58454=CARTESIAN_POINT('Ctrl Pts',(126.547419073731,35.8175564842859,30.0000000000002));
#58455=CARTESIAN_POINT('Ctrl Pts',(126.553170507578,35.8346208908098,30.0000000000002));
#58456=CARTESIAN_POINT('Ctrl Pts',(126.559047009417,35.8516468460435,30.));
#58457=CARTESIAN_POINT('Ctrl Pts',(126.56504410264,35.8686204532914,30.));
#58458=CARTESIAN_POINT('Ctrl Pts',(126.60289081843,35.9757382294415,29.9999999999999));
#58459=CARTESIAN_POINT('Ctrl Pts',(126.645579997457,36.0809032528098,29.9999999999999));
#58460=CARTESIAN_POINT('Ctrl Pts',(126.693045639272,36.1837053875735,29.9999999999999));
#58461=CARTESIAN_POINT('Ctrl Pts',(126.733092203321,36.2704391199489,30.));
#58462=CARTESIAN_POINT('Ctrl Pts',(126.776539630878,36.3554907358829,30.0000000000001));
#58463=CARTESIAN_POINT('Ctrl Pts',(126.823370488022,36.4385941868589,30.));
#58464=CARTESIAN_POINT('Ctrl Pts',(126.844837183414,36.4766877981435,29.9999999999999));
#58465=CARTESIAN_POINT('Ctrl Pts',(126.867015069518,36.5143717765041,30.0000000000001));
#58466=CARTESIAN_POINT('Ctrl Pts',(126.889903763462,36.5516189055333,30.));
#58467=CARTESIAN_POINT('Ctrl Pts',(126.903889590876,36.574378260852,30.));
#58468=CARTESIAN_POINT('Ctrl Pts',(126.918143120974,36.5969778174688,30.));
#58469=CARTESIAN_POINT('Ctrl Pts',(126.932649224775,36.6193883664837,30.));
#58470=CARTESIAN_POINT('Ctrl Pts',(126.991211921456,36.7098621561641,30.0000000000001));
#58471=CARTESIAN_POINT('Ctrl Pts',(127.053930557615,36.7973297766238,30.0000000000001));
#58472=CARTESIAN_POINT('Ctrl Pts',(127.120768818292,36.8814100270898,30.0000000000001));
#58473=CARTESIAN_POINT('Ctrl Pts',(127.187607078969,36.9654902775559,30.0000000000001));
#58474=CARTESIAN_POINT('Ctrl Pts',(127.258565249867,37.0461838130672,30.));
#58475=CARTESIAN_POINT('Ctrl Pts',(127.333638243439,37.1230673427468,30.0000000000001));
#58476=CARTESIAN_POINT('Ctrl Pts',(127.362444717677,37.1525685430013,30.0000000000001));
#58477=CARTESIAN_POINT('Ctrl Pts',(127.391857367042,37.1815082646089,30.));
#58478=CARTESIAN_POINT('Ctrl Pts',(127.421855523101,37.2098778099405,30.));
#58479=CARTESIAN_POINT('Origin',(-10.,35.,17.));
#58480=CARTESIAN_POINT('Ctrl Pts',(-6.62123117139838,34.7273715616997,17.));
#58481=CARTESIAN_POINT('Ctrl Pts',(-6.60195934569834,34.8321949891012,17.));
#58482=CARTESIAN_POINT('Ctrl Pts',(-6.58807244351625,34.9377386945817,17.));
#58483=CARTESIAN_POINT('Ctrl Pts',(-6.5793423594526,35.0436676563277,17.));
#58484=CARTESIAN_POINT('Ctrl Pts',(-6.57037143927326,35.1525188716857,17.));
#58485=CARTESIAN_POINT('Ctrl Pts',(-6.5668456742337,35.261777509942,17.));
#58486=CARTESIAN_POINT('Ctrl Pts',(-6.56856898097211,35.3711000441821,17.));
#58487=CARTESIAN_POINT('Ctrl Pts',(-6.56942692580178,35.4255260502596,17.));
#58488=CARTESIAN_POINT('Ctrl Pts',(-6.57158666510304,35.4799681405241,17.));
#58489=CARTESIAN_POINT('Ctrl Pts',(-6.57502867344059,35.5343849332849,17.));
#58490=CARTESIAN_POINT('Ctrl Pts',(-6.57632046539286,35.5548076539941,17.));
#58491=CARTESIAN_POINT('Ctrl Pts',(-6.57779235581878,35.5752179805597,17.));
#58492=CARTESIAN_POINT('Ctrl Pts',(-6.57944266526219,35.5956107924917,17.));
#58493=CARTESIAN_POINT('Ctrl Pts',(-6.58842152809188,35.7065622639138,17.));
#58494=CARTESIAN_POINT('Ctrl Pts',(-6.60267946638345,35.8170216916155,17.));
#58495=CARTESIAN_POINT('Ctrl Pts',(-6.62200532182683,35.9266343683881,17.));
#58496=CARTESIAN_POINT('Ctrl Pts',(-6.641707143771,36.038379457599,17.));
#58497=CARTESIAN_POINT('Ctrl Pts',(-6.66667597712323,36.1492453277495,17.));
#58498=CARTESIAN_POINT('Ctrl Pts',(-6.69674117187053,36.2588637823476,17.));
#58499=CARTESIAN_POINT('Ctrl Pts',(-6.70213341047965,36.2785240196461,17.));
#58500=CARTESIAN_POINT('Ctrl Pts',(-6.70768971886736,36.2981441321776,17.));
#58501=CARTESIAN_POINT('Ctrl Pts',(-6.71340928846767,36.3177219893546,17.));
#58502=CARTESIAN_POINT('Ctrl Pts',(-6.72069554508889,36.3426625533225,17.));
#58503=CARTESIAN_POINT('Ctrl Pts',(-6.72824855494793,36.367539909623,17.));
#58504=CARTESIAN_POINT('Ctrl Pts',(-6.73605660535735,36.392318482591,17.));
#58505=CARTESIAN_POINT('Ctrl Pts',(-6.77081652375714,36.5026278593585,17.));
#58506=CARTESIAN_POINT('Ctrl Pts',(-6.81065343512221,36.6110784621336,17.));
#58507=CARTESIAN_POINT('Ctrl Pts',(-6.85534048320785,36.7172979594713,17.));
#58508=CARTESIAN_POINT('Ctrl Pts',(-6.90044237101414,36.8245035158237,17.));
#58509=CARTESIAN_POINT('Ctrl Pts',(-6.95048498501844,36.9294372298153,17.));
#58510=CARTESIAN_POINT('Ctrl Pts',(-7.0052885201046,37.0317182304336,17.));
#58511=CARTESIAN_POINT('Ctrl Pts',(-7.05981854622386,37.1334887754623,17.));
#58512=CARTESIAN_POINT('Ctrl Pts',(-7.11906233324677,37.2326339054117,17.));
#58513=CARTESIAN_POINT('Ctrl Pts',(-7.18289248555842,37.328767082928,17.));
#58514=CARTESIAN_POINT('Ctrl Pts',(-7.22018203267521,37.3849280432681,17.));
#58515=CARTESIAN_POINT('Ctrl Pts',(-7.25903777040094,37.4400607782531,17.));
#58516=CARTESIAN_POINT('Ctrl Pts',(-7.29944172118395,37.4940845629917,17.));
#58517=CARTESIAN_POINT('Ctrl Pts',(-7.3210590200253,37.522988872511,17.));
#58518=CARTESIAN_POINT('Ctrl Pts',(-7.34311959600719,37.5515756830289,17.));
#58519=CARTESIAN_POINT('Ctrl Pts',(-7.36562131389244,37.5798321948882,17.));
#58520=CARTESIAN_POINT('Ctrl Pts',(-7.37556893692007,37.5923239134976,17.));
#58521=CARTESIAN_POINT('Ctrl Pts',(-7.38560197216116,37.6047499703436,17.));
#58522=CARTESIAN_POINT('Ctrl Pts',(-7.39571231655314,37.6170998830206,17.));
#58523=CARTESIAN_POINT('Ctrl Pts',(-7.47117575693862,37.7092794233932,17.));
#58524=CARTESIAN_POINT('Ctrl Pts',(-7.55105630936717,37.7973622554539,17.));
#58525=CARTESIAN_POINT('Ctrl Pts',(-7.63516399751822,37.8809609308377,17.));
#58526=CARTESIAN_POINT('Ctrl Pts',(-7.65864155501132,37.904296404096,17.));
#58527=CARTESIAN_POINT('Ctrl Pts',(-7.68244878202814,37.9272824054679,17.));
#58528=CARTESIAN_POINT('Ctrl Pts',(-7.70658223699224,37.9499102825999,17.));
#58529=CARTESIAN_POINT('Ctrl Pts',(-7.78963819592032,38.0277847533917,17.));
#58530=CARTESIAN_POINT('Ctrl Pts',(-7.87655463462689,38.1014199334542,17.));
#58531=CARTESIAN_POINT('Ctrl Pts',(-7.96691983219225,38.1708050440767,17.));
#58532=CARTESIAN_POINT('Ctrl Pts',(-8.05961255392386,38.2419772976049,17.));
#58533=CARTESIAN_POINT('Ctrl Pts',(-8.15593450042321,38.3086781586375,17.));
#58534=CARTESIAN_POINT('Ctrl Pts',(-8.25548340140922,38.3708605803994,17.));
#58535=CARTESIAN_POINT('Ctrl Pts',(-8.31141688788464,38.4057989836583,17.));
#58536=CARTESIAN_POINT('Ctrl Pts',(-8.3683698237762,38.4393102584732,17.));
#58537=CARTESIAN_POINT('Ctrl Pts',(-8.4262754553306,38.4713805519023,17.));
#58538=CARTESIAN_POINT('Ctrl Pts',(-8.44233384032758,38.4802742830477,17.));
#58539=CARTESIAN_POINT('Ctrl Pts',(-8.45846551033602,38.4890571689273,17.));
#58540=CARTESIAN_POINT('Ctrl Pts',(-8.47466907811928,38.4977288564759,17.));
#58541=CARTESIAN_POINT('Ctrl Pts',(-8.48766521757792,38.504684019822,17.));
#58542=CARTESIAN_POINT('Ctrl Pts',(-8.50070673982194,38.5115671407453,17.));
#58543=CARTESIAN_POINT('Ctrl Pts',(-8.51378382562772,38.5183734543627,17.));
#58544=CARTESIAN_POINT('Ctrl Pts',(-8.61982299463778,38.5735643318048,17.));
#58545=CARTESIAN_POINT('Ctrl Pts',(-8.7283547505616,38.6237926959064,17.));
#58546=CARTESIAN_POINT('Ctrl Pts',(-8.83892423282891,38.6690579537086,17.));
#58547=CARTESIAN_POINT('Ctrl Pts',(-8.9513815803523,38.7150960713069,17.));
#58548=CARTESIAN_POINT('Ctrl Pts',(-9.06594749383451,38.7560005407811,17.));
#58549=CARTESIAN_POINT('Ctrl Pts',(-9.18218323047418,38.7917330299808,17.));
#58550=CARTESIAN_POINT('Ctrl Pts',(-9.29985553091803,38.827907138962,17.));
#58551=CARTESIAN_POINT('Ctrl Pts',(-9.41923996013768,38.8587810364494,17.));
#58552=CARTESIAN_POINT('Ctrl Pts',(-9.53991077851995,38.8842706896853,17.));
#58553=CARTESIAN_POINT('Ctrl Pts',(-9.61457604005369,38.900042453321,17.));
#58554=CARTESIAN_POINT('Ctrl Pts',(-9.68973433655139,38.9137519461733,17.));
#58555=CARTESIAN_POINT('Ctrl Pts',(-9.7652883226987,38.9253699046292,17.));
#58556=CARTESIAN_POINT('Ctrl Pts',(-9.80157135144814,38.9309491565279,17.));
#58557=CARTESIAN_POINT('Ctrl Pts',(-9.83794566222605,38.936045954135,17.));
#58558=CARTESIAN_POINT('Ctrl Pts',(-9.87440059370104,38.9406564316365,17.));
#58559=CARTESIAN_POINT('Ctrl Pts',(-9.89072243089403,38.9427206643786,17.));
#58560=CARTESIAN_POINT('Ctrl Pts',(-9.90706094261734,38.9446874628517,17.));
#58561=CARTESIAN_POINT('Ctrl Pts',(-9.92341361539116,38.9465562749007,17.));
#58562=CARTESIAN_POINT('Ctrl Pts',(-10.049134669734,38.9609238969046,17.));
#58563=CARTESIAN_POINT('Ctrl Pts',(-10.1751588854043,38.9694430949161,17.));
#58564=CARTESIAN_POINT('Ctrl Pts',(-10.3010213929365,38.9720792792337,17.));
#58565=CARTESIAN_POINT('Ctrl Pts',(-10.4271447298256,38.9747209266099,17.));
#58566=CARTESIAN_POINT('Ctrl Pts',(-10.5531065751926,38.9714554663851,17.));
#58567=CARTESIAN_POINT('Ctrl Pts',(-10.6784618767559,38.9622008961875,17.));
#58568=CARTESIAN_POINT('Ctrl Pts',(-10.8015648493969,38.9531126080367,17.));
#58569=CARTESIAN_POINT('Ctrl Pts',(-10.9240837583291,38.938248640579,17.));
#58570=CARTESIAN_POINT('Ctrl Pts',(-11.0456058184429,38.9174827178352,17.));
#58571=CARTESIAN_POINT('Ctrl Pts',(-11.1383506190094,38.9016343084053,17.));
#58572=CARTESIAN_POINT('Ctrl Pts',(-11.2305150666145,38.8823472846425,17.));
#58573=CARTESIAN_POINT('Ctrl Pts',(-11.3219144398766,38.8595450271519,17.));
#58574=CARTESIAN_POINT('Ctrl Pts',(-11.3696279828065,38.8476414828184,17.));
#58575=CARTESIAN_POINT('Ctrl Pts',(-11.4171329813549,38.8347796560283,17.));
#58576=CARTESIAN_POINT('Ctrl Pts',(-11.464413394279,38.8209773893083,17.));
#58577=CARTESIAN_POINT('Ctrl Pts',(-13.1750507821943,37.570267988068,17.));
#58578=CARTESIAN_POINT('Ctrl Pts',(-13.2457830638452,37.4660682901415,17.));
#58579=CARTESIAN_POINT('Ctrl Pts',(-13.3111684943071,37.3585303558788,17.));
#58580=CARTESIAN_POINT('Ctrl Pts',(-13.3712015697569,37.2480942554894,17.));
#58581=CARTESIAN_POINT('Ctrl Pts',(-13.4312346452066,37.1376581551,17.));
#58582=CARTESIAN_POINT('Ctrl Pts',(-13.4859153844916,37.0243229867705,17.));
#58583=CARTESIAN_POINT('Ctrl Pts',(-13.5351882493577,36.908514120475,17.));
#58584=CARTESIAN_POINT('Ctrl Pts',(-13.5568750177871,36.8575424533667,17.));
#58585=CARTESIAN_POINT('Ctrl Pts',(-13.5775135207773,36.8060914717338,17.));
#58586=CARTESIAN_POINT('Ctrl Pts',(-13.5970959340666,36.7541972265355,17.));
#58587=CARTESIAN_POINT('Ctrl Pts',(-13.6073225862103,36.727096154463,17.));
#58588=CARTESIAN_POINT('Ctrl Pts',(-13.6172624893017,36.6998701487207,17.));
#58589=CARTESIAN_POINT('Ctrl Pts',(-13.6269052970792,36.6725509192079,17.));
#58590=CARTESIAN_POINT('Ctrl Pts',(-13.6685921142032,36.5544471727738,17.));
#58591=CARTESIAN_POINT('Ctrl Pts',(-13.7047658650663,36.4345131254237,17.));
#58592=CARTESIAN_POINT('Ctrl Pts',(-13.7353857954243,36.3131762502625,17.));
#58593=CARTESIAN_POINT('Ctrl Pts',(-13.7610637989098,36.2114226320506,17.));
#58594=CARTESIAN_POINT('Ctrl Pts',(-13.7828351362415,36.1086819645596,17.));
#58595=CARTESIAN_POINT('Ctrl Pts',(-13.8006475130466,36.0052062251963,17.));
#58596=CARTESIAN_POINT('Ctrl Pts',(-13.8084978850862,35.9596018086737,17.));
#58597=CARTESIAN_POINT('Ctrl Pts',(-13.8155789355258,35.9138546491184,17.));
#58598=CARTESIAN_POINT('Ctrl Pts',(-13.821884594521,35.8679866185036,17.));
#58599=CARTESIAN_POINT('Ctrl Pts',(-13.8245836173036,35.8483536412497,17.));
#58600=CARTESIAN_POINT('Ctrl Pts',(-13.8271405674798,35.8286985223403,17.));
#58601=CARTESIAN_POINT('Ctrl Pts',(-13.8295549143713,35.8090229935632,17.));
#58602=CARTESIAN_POINT('Ctrl Pts',(-13.8317980116041,35.7907430503162,17.));
#58603=CARTESIAN_POINT('Ctrl Pts',(-13.8339175340875,35.7724490669597,17.));
#58604=CARTESIAN_POINT('Ctrl Pts',(-13.8359122468823,35.7541522042298,17.));
#58605=CARTESIAN_POINT('Ctrl Pts',(-13.8491708905682,35.6325349046639,17.));
#58606=CARTESIAN_POINT('Ctrl Pts',(-13.8569353644682,35.5106633232552,17.));
#58607=CARTESIAN_POINT('Ctrl Pts',(-13.8591710359411,35.3889344818084,17.));
#58608=CARTESIAN_POINT('Ctrl Pts',(-13.8613888966442,35.2681754091286,17.));
#58609=CARTESIAN_POINT('Ctrl Pts',(-13.8581656100447,35.1475559779588,17.));
#58610=CARTESIAN_POINT('Ctrl Pts',(-13.8494169850101,35.0274704860568,17.));
#58611=CARTESIAN_POINT('Ctrl Pts',(-13.8408792900479,34.9102802652854,17.));
#58612=CARTESIAN_POINT('Ctrl Pts',(-13.8270792795936,34.7935978726728,17.));
#58613=CARTESIAN_POINT('Ctrl Pts',(-13.8078928234413,34.6778071494505,17.));
#58614=CARTESIAN_POINT('Ctrl Pts',(-13.7961972995813,34.607224382343,17.));
#58615=CARTESIAN_POINT('Ctrl Pts',(-13.7824994107177,34.5369733219596,17.));
#58616=CARTESIAN_POINT('Ctrl Pts',(-13.7667627942638,34.4671457809156,17.));
#58617=CARTESIAN_POINT('Ctrl Pts',(-13.7572176645193,34.4247915085752,17.));
#58618=CARTESIAN_POINT('Ctrl Pts',(-13.7469223466112,34.3825931317931,17.));
#58619=CARTESIAN_POINT('Ctrl Pts',(-13.7358676068506,34.340571973438,17.));
#58620=CARTESIAN_POINT('Ctrl Pts',(-13.7309282145613,34.3217964083807,17.));
#58621=CARTESIAN_POINT('Ctrl Pts',(-13.7258367127005,34.3030548272173,17.));
#58622=CARTESIAN_POINT('Ctrl Pts',(-13.7205981502818,34.2843693290194,17.));
#58623=CARTESIAN_POINT('Ctrl Pts',(-13.689338264928,34.1728680267999,17.));
#58624=CARTESIAN_POINT('Ctrl Pts',(-13.6528033562578,34.0631963206846,17.));
#58625=CARTESIAN_POINT('Ctrl Pts',(-13.6109173793413,33.9557088671316,17.));
#58626=CARTESIAN_POINT('Ctrl Pts',(-13.5979450581991,33.9224194020434,17.));
#58627=CARTESIAN_POINT('Ctrl Pts',(-13.5844591309443,33.8893395894124,17.));
#58628=CARTESIAN_POINT('Ctrl Pts',(-13.5704564135702,33.8564804057572,17.));
#58629=CARTESIAN_POINT('Ctrl Pts',(-13.5243066910341,33.7481841252616,17.));
#58630=CARTESIAN_POINT('Ctrl Pts',(-13.4725467214683,33.6422818048275,17.));
#58631=CARTESIAN_POINT('Ctrl Pts',(-13.4155273320418,33.539047281335,17.));
#58632=CARTESIAN_POINT('Ctrl Pts',(-13.3586530947265,33.4360755580789,17.));
#58633=CARTESIAN_POINT('Ctrl Pts',(-13.2965453659658,33.3357575270244,17.));
#58634=CARTESIAN_POINT('Ctrl Pts',(-13.2295170803124,33.2384027306936,17.));
#58635=CARTESIAN_POINT('Ctrl Pts',(-13.1958682827822,33.1895297541822,17.));
#58636=CARTESIAN_POINT('Ctrl Pts',(-13.1609789634487,33.1414041960367,17.));
#58637=CARTESIAN_POINT('Ctrl Pts',(-13.1248863292235,33.0940694733039,17.));
#58638=CARTESIAN_POINT('Ctrl Pts',(-13.1136852563331,33.0793795042573,17.));
#58639=CARTESIAN_POINT('Ctrl Pts',(-13.1023682800586,33.06476572469,17.));
#58640=CARTESIAN_POINT('Ctrl Pts',(-13.090936489294,33.0502294936717,17.));
#58641=CARTESIAN_POINT('Ctrl Pts',(-13.0810912756462,33.0377106938654,17.));
#58642=CARTESIAN_POINT('Ctrl Pts',(-13.0711638284922,33.0252531825434,17.));
#58643=CARTESIAN_POINT('Ctrl Pts',(-13.0611599663059,33.0128637449684,17.));
#58644=CARTESIAN_POINT('Ctrl Pts',(-12.9882950661098,32.9226230843549,17.));
#58645=CARTESIAN_POINT('Ctrl Pts',(-12.9113010014507,32.8358909574534,17.));
#58646=CARTESIAN_POINT('Ctrl Pts',(-12.8305230803461,32.7529134373871,17.));
#58647=CARTESIAN_POINT('Ctrl Pts',(-12.7496940850864,32.6698834524061,17.));
#58648=CARTESIAN_POINT('Ctrl Pts',(-12.6650756390752,32.5906122997939,17.));
#58649=CARTESIAN_POINT('Ctrl Pts',(-12.5769819956178,32.5153878223483,17.));
#58650=CARTESIAN_POINT('Ctrl Pts',(-12.4904417698574,32.4414898314677,17.));
#58651=CARTESIAN_POINT('Ctrl Pts',(-12.4005470330641,32.371496714977,17.));
#58652=CARTESIAN_POINT('Ctrl Pts',(-12.3075770876119,32.3057274062505,17.));
#58653=CARTESIAN_POINT('Ctrl Pts',(-12.2551730571484,32.2686554595983,17.));
#58654=CARTESIAN_POINT('Ctrl Pts',(-12.2017917003474,32.2329263645682,17.));
#58655=CARTESIAN_POINT('Ctrl Pts',(-12.1474817625173,32.198604486143,17.));
#58656=CARTESIAN_POINT('Ctrl Pts',(-12.1187454577522,32.1804442009734,17.));
#58657=CARTESIAN_POINT('Ctrl Pts',(-12.0897491736939,32.1626779784828,17.));
#58658=CARTESIAN_POINT('Ctrl Pts',(-12.0605001014649,32.1453159941706,17.));
#58659=CARTESIAN_POINT('Ctrl Pts',(-12.0439204100942,32.1354744395659,17.));
#58660=CARTESIAN_POINT('Ctrl Pts',(-12.0272576783142,32.1257618412,17.));
#58661=CARTESIAN_POINT('Ctrl Pts',(-12.0105328383307,32.1161910461162,17.));
#58662=CARTESIAN_POINT('Ctrl Pts',(-11.9136863575601,32.0607706162074,17.));
#58663=CARTESIAN_POINT('Ctrl Pts',(-11.8146169520547,32.0100152898296,17.));
#58664=CARTESIAN_POINT('Ctrl Pts',(-11.7136099215379,31.9641826653935,17.));
#58665=CARTESIAN_POINT('Ctrl Pts',(-11.6141161250821,31.9190366811649,17.));
#58666=CARTESIAN_POINT('Ctrl Pts',(-11.512741606946,31.8786667193764,17.));
#58667=CARTESIAN_POINT('Ctrl Pts',(-11.4097470166284,31.8433673104104,17.));
#58668=CARTESIAN_POINT('Ctrl Pts',(-11.3098310001791,31.8091230232492,17.));
#58669=CARTESIAN_POINT('Ctrl Pts',(-11.2083897167571,31.7796505908842,17.));
#58670=CARTESIAN_POINT('Ctrl Pts',(-11.1056593067708,31.7552673702842,17.));
#58671=CARTESIAN_POINT('Ctrl Pts',(-11.0406608290356,31.7398398817588,17.));
#58672=CARTESIAN_POINT('Ctrl Pts',(-10.9751462807458,31.7264506838377,17.));
#58673=CARTESIAN_POINT('Ctrl Pts',(-10.9091766549683,31.7151909620675,17.));
#58674=CARTESIAN_POINT('Ctrl Pts',(-10.8685408754868,31.708255231184,17.));
#58675=CARTESIAN_POINT('Ctrl Pts',(-10.8277324413485,31.7021276870367,17.));
#58676=CARTESIAN_POINT('Ctrl Pts',(-10.7867731801703,31.6968047429727,17.));
#58677=CARTESIAN_POINT('Ctrl Pts',(-7.43281944318039,37.2044345752726,29.9966888174997));
#58678=CARTESIAN_POINT('Ctrl Pts',(-6.70433239249398,36.3561656695364,29.9309499309566));
#58679=CARTESIAN_POINT('Ctrl Pts',(-6.16680179062131,33.8959591706789,29.7995178935572));
#58680=CARTESIAN_POINT('Ctrl Pts',(-8.82688724400274,31.1837581319228,29.6023927053017));
#58681=CARTESIAN_POINT('Ctrl Pts',(-12.5469209189557,31.9295115870956,29.4053132527333));
#58682=CARTESIAN_POINT('Ctrl Pts',(-13.9650991559566,35.445741398928,29.2082338001648));
#58683=CARTESIAN_POINT('Ctrl Pts',(-11.8002654955171,38.5612862953215,29.0111543475964));
#58684=CARTESIAN_POINT('Ctrl Pts',(-8.00850991085725,38.4575298371214,28.8140748950279));
#58685=CARTESIAN_POINT('Ctrl Pts',(-6.01644546373737,35.2298316539741,28.6169954424595));
#58686=CARTESIAN_POINT('Ctrl Pts',(-7.62419319279026,31.7941726174109,28.419915989891));
#58687=CARTESIAN_POINT('Ctrl Pts',(-11.3789020069552,31.255667443897,28.2228365373226));
#58688=CARTESIAN_POINT('Ctrl Pts',(-13.8875300071254,34.1007462780832,28.0257570847542));
#58689=CARTESIAN_POINT('Ctrl Pts',(-12.8831049662547,37.7584902581075,27.8286776321857));
#58690=CARTESIAN_POINT('Ctrl Pts',(-9.27329511580484,38.9234444319071,27.6315981796173));
#58691=CARTESIAN_POINT('Ctrl Pts',(-6.32018930815337,36.5428969771351,27.4345187270488));
#58692=CARTESIAN_POINT('Ctrl Pts',(-6.69242821576807,32.7680711157438,27.2374392744804));
#58693=CARTESIAN_POINT('Ctrl Pts',(-10.0536300766488,31.0101809435409,27.0403598219119));
#58694=CARTESIAN_POINT('Ctrl Pts',(-13.3663678211108,32.8577808295107,26.8432803693435));
#58695=CARTESIAN_POINT('Ctrl Pts',(-13.6370104108175,36.6412465561122,26.6462009167751));
#58696=CARTESIAN_POINT('Ctrl Pts',(-10.6209854317379,38.9415620618598,26.4491214642066));
#58697=CARTESIAN_POINT('Ctrl Pts',(-7.04379278912358,37.6799950971764,26.2520420116382));
#58698=CARTESIAN_POINT('Ctrl Pts',(-6.13804432686434,33.9965892654983,26.0549625590698));
#58699=CARTESIAN_POINT('Ctrl Pts',(-8.72224034293969,31.2199385031057,25.8578831065013));
#58700=CARTESIAN_POINT('Ctrl Pts',(-12.4611130642332,31.8592266559683,25.6608036539329));
#58701=CARTESIAN_POINT('Ctrl Pts',(-13.9759447379094,35.3367464054446,25.4637242013644));
#58702=CARTESIAN_POINT('Ctrl Pts',(-11.8978231126421,38.5099575677875,25.266644748796));
#58703=CARTESIAN_POINT('Ctrl Pts',(-8.10469027325444,38.5113153861208,25.0695652962275));
#58704=CARTESIAN_POINT('Ctrl Pts',(-6.02429736947304,35.3395928335728,24.8724858436591));
#58705=CARTESIAN_POINT('Ctrl Pts',(-7.53663897851176,31.8609894590311,24.6754063910907));
#58706=CARTESIAN_POINT('Ctrl Pts',(-11.275053053664,31.2190246748164,24.4783269385222));
#58707=CARTESIAN_POINT('Ctrl Pts',(-13.8612363064412,33.9938246252232,24.2812474859537));
#58708=CARTESIAN_POINT('Ctrl Pts',(-12.9581251553404,37.6778779405159,24.0841680333854));
#58709=CARTESIAN_POINT('Ctrl Pts',(-9.38183662494831,38.9420056748818,23.8870885808168));
#58710=CARTESIAN_POINT('Ctrl Pts',(-6.36416555126165,36.6438499202713,23.6900091282485));
#58711=CARTESIAN_POINT('Ctrl Pts',(-6.63209934310249,32.8601916290756,23.49292967568));
#58712=CARTESIAN_POINT('Ctrl Pts',(-9.94351350813597,31.0102200592936,23.2958502231116));
#58713=CARTESIAN_POINT('Ctrl Pts',(-13.3059729820585,32.7657042852594,23.0987707705431));
#58714=CARTESIAN_POINT('Ctrl Pts',(-13.6809144409843,36.5402608795793,22.9016913179747));
#58715=CARTESIAN_POINT('Ctrl Pts',(-10.7295134694718,38.9229255405774,22.7046118654062));
#58716=CARTESIAN_POINT('Ctrl Pts',(-7.11887098447587,37.7605489118768,22.5075324128378));
#58717=CARTESIAN_POINT('Ctrl Pts',(-6.11182655793853,34.1035391902405,22.3104529602694));
#58718=CARTESIAN_POINT('Ctrl Pts',(-8.61841889329849,31.2566367602235,22.1133735077009));
#58719=CARTESIAN_POINT('Ctrl Pts',(-12.3735085599531,31.7925100445471,21.9162940551325));
#58720=CARTESIAN_POINT('Ctrl Pts',(-13.9837229901626,35.2269049066077,21.719214602564));
#58721=CARTESIAN_POINT('Ctrl Pts',(-11.9939551263463,38.4562519663969,21.5221351499956));
#58722=CARTESIAN_POINT('Ctrl Pts',(-8.20230415784552,38.5622779725406,21.3250556974271));
#58723=CARTESIAN_POINT('Ctrl Pts',(-6.0351821079984,35.4491701055871,21.1279762448587));
#58724=CARTESIAN_POINT('Ctrl Pts',(-7.45095832845666,31.930159406377,20.9308967922902));
#58725=CARTESIAN_POINT('Ctrl Pts',(-11.1702342916329,31.1852803033251,20.7338173397218));
#58726=CARTESIAN_POINT('Ctrl Pts',(-13.8320013021391,33.887659789551,20.5367378871533));
#58727=CARTESIAN_POINT('Ctrl Pts',(-13.0308927869956,37.5952309547061,20.3396584345849));
#58728=CARTESIAN_POINT('Ctrl Pts',(-9.49084876237968,38.9575623066672,20.1425789820165));
#58729=CARTESIAN_POINT('Ctrl Pts',(-6.41091088066521,36.7435522016327,19.945499529448));
#58730=CARTESIAN_POINT('Ctrl Pts',(-6.57433539009964,32.9539410414412,19.7484200768796));
#58731=CARTESIAN_POINT('Ctrl Pts',(-9.83343996764695,31.0132983502615,19.5513406243111));
#58732=CARTESIAN_POINT('Ctrl Pts',(-13.2430603653772,32.6753285998351,19.3542611717427));
#58733=CARTESIAN_POINT('Ctrl Pts',(-13.7220150885897,36.4381034351505,19.1571817191743));
#58734=CARTESIAN_POINT('Ctrl Pts',(-10.8374860072516,38.9012989358204,18.9601022666058));
#58735=CARTESIAN_POINT('Ctrl Pts',(-7.19614323312918,37.83900510415,18.7630228140374));
#58736=CARTESIAN_POINT('Ctrl Pts',(-6.08857033917078,34.2111623607691,18.5659433614689));
#58737=CARTESIAN_POINT('Ctrl Pts',(-8.51564891709047,31.296204798029,18.3688639089005));
#58738=CARTESIAN_POINT('Ctrl Pts',(-12.2840978586159,31.7281986361625,18.1717844563321));
#58739=CARTESIAN_POINT('Ctrl Pts',(-13.9884644187953,35.1169654331458,17.9747050037636));
#58740=CARTESIAN_POINT('Ctrl Pts',(-12.0885742745814,38.3997651167831,17.7776255511952));
#58741=CARTESIAN_POINT('Ctrl Pts',(-8.30127578536255,38.6108242790529,17.5805460986267));
#58742=CARTESIAN_POINT('Ctrl Pts',(-6.0491089823217,35.5578143756796,17.3834666460583));
#58743=CARTESIAN_POINT('Ctrl Pts',(-7.36717462669024,32.002845380223,17.1863871934898));
#58744=CARTESIAN_POINT('Ctrl Pts',(-11.0646050703342,31.1520769786589,16.9893077409214));
#58745=CARTESIAN_POINT('Ctrl Pts',(-13.7997717921734,33.78727260672,16.7922282883529));
#58746=CARTESIAN_POINT('Ctrl Pts',(-13.3330648228068,36.2606000081635,16.6608419866407));
#58747=CARTESIAN_POINT('Ctrl Pts',(-12.6300280270065,37.1290610164239,16.5951488357845));
#58748=CARTESIAN_POINT('Ctrl Pts',(-7.25452804718548,37.3575331630446,30.1323685894149));
#58749=CARTESIAN_POINT('Ctrl Pts',(-6.47544737039588,36.4503517484157,30.0666297028717));
#58750=CARTESIAN_POINT('Ctrl Pts',(-5.90058512032913,33.8192832313211,29.9351976654724));
#58751=CARTESIAN_POINT('Ctrl Pts',(-8.74541424033318,30.9187190841993,29.7380724772169));
#58752=CARTESIAN_POINT('Ctrl Pts',(-12.7238052775268,31.7162653220174,29.5409930246485));
#58753=CARTESIAN_POINT('Ctrl Pts',(-14.2404763832793,35.4766982617231,29.34391357208));
#58754=CARTESIAN_POINT('Ctrl Pts',(-11.9252944294986,38.8086186083696,29.1468341195116));
#58755=CARTESIAN_POINT('Ctrl Pts',(-7.87020037623567,38.6976562356004,28.9497546669431));
#58756=CARTESIAN_POINT('Ctrl Pts',(-5.73978650517466,35.2457935255776,28.7526752143747));
#58757=CARTESIAN_POINT('Ctrl Pts',(-7.45919275635956,31.5715270236516,28.5555957618062));
#58758=CARTESIAN_POINT('Ctrl Pts',(-11.4746671307238,30.995622517675,28.3585163092378));
#58759=CARTESIAN_POINT('Ctrl Pts',(-14.1575200357198,34.038292859679,28.1614368566694));
#58760=CARTESIAN_POINT('Ctrl Pts',(-13.0833373994071,37.9500681654932,27.9643574041009));
#58761=CARTESIAN_POINT('Ctrl Pts',(-9.2228252616548,39.1959287271839,27.7672779515325));
#58762=CARTESIAN_POINT('Ctrl Pts',(-6.06462544315624,36.6500515967036,27.570198498964));
#58763=CARTESIAN_POINT('Ctrl Pts',(-6.46271644532108,32.6130630406483,27.3731190463956));
#58764=CARTESIAN_POINT('Ctrl Pts',(-10.0573547002275,30.733086912327,27.1760395938271));
#58765=CARTESIAN_POINT('Ctrl Pts',(-13.6001629924959,32.7090031187187,26.9789601412587));
#58766=CARTESIAN_POINT('Ctrl Pts',(-13.8896017845213,36.7552315810001,26.7818806886903));
#58767=CARTESIAN_POINT('Ctrl Pts',(-10.6641130408276,39.2153046315217,26.5848012361218));
#58768=CARTESIAN_POINT('Ctrl Pts',(-6.83848338496921,37.8661214940384,26.3877217835534));
#58769=CARTESIAN_POINT('Ctrl Pts',(-5.86983044280201,33.9269021139128,26.190642330985));
#58770=CARTESIAN_POINT('Ctrl Pts',(-8.63349958319917,30.9574121921154,25.9935628784165));
#58771=CARTESIAN_POINT('Ctrl Pts',(-12.6320380436851,31.6410990830854,25.7964834258481));
#58772=CARTESIAN_POINT('Ctrl Pts',(-14.2520751938827,35.3601335359538,25.5994039732796));
#58773=CARTESIAN_POINT('Ctrl Pts',(-12.0296274499745,38.753725086586,25.4023245207112));
#58774=CARTESIAN_POINT('Ctrl Pts',(-7.97306049126402,38.7551772057762,25.2052450681427));
#58775=CARTESIAN_POINT('Ctrl Pts',(-5.74818372792402,35.3631776492987,25.0081656155743));
#58776=CARTESIAN_POINT('Ctrl Pts',(-7.36555787781011,31.6429843133059,24.8110861630058));
#58777=CARTESIAN_POINT('Ctrl Pts',(-11.363605839054,30.9564348982,24.6140067104374));
#58778=CARTESIAN_POINT('Ctrl Pts',(-14.1294002302886,33.9239454686098,24.416927257869));
#58779=CARTESIAN_POINT('Ctrl Pts',(-13.1635677612655,37.8638573002654,24.2198478053005));
#58780=CARTESIAN_POINT('Ctrl Pts',(-9.338905008472,39.21577905359,24.0227683527321));
#58781=CARTESIAN_POINT('Ctrl Pts',(-6.11165584844781,36.7580157495165,23.8256889001636));
#58782=CARTESIAN_POINT('Ctrl Pts',(-6.39819771585024,32.7115813489765,23.6286094475952));
#58783=CARTESIAN_POINT('Ctrl Pts',(-9.93959050573454,30.7331287446795,23.4315299950267));
#58784=CARTESIAN_POINT('Ctrl Pts',(-13.5355737152546,32.6105318331355,23.2344505424584));
#58785=CARTESIAN_POINT('Ctrl Pts',(-13.9365549616627,36.6472324214472,23.0373710898898));
#58786=CARTESIAN_POINT('Ctrl Pts',(-10.780178380642,39.1953737987086,22.8402916373215));
#58787=CARTESIAN_POINT('Ctrl Pts',(-6.91877578164541,37.952269793333,22.643212184753));
#58788=CARTESIAN_POINT('Ctrl Pts',(-5.84179184261089,34.0412797403541,22.4461327321845));
#58789=CARTESIAN_POINT('Ctrl Pts',(-8.52246770531536,30.9966591532869,22.2490532796161));
#58790=CARTESIAN_POINT('Ctrl Pts',(-12.5383493824794,31.569748984645,22.0519738270477));
#58791=CARTESIAN_POINT('Ctrl Pts',(-14.260393647895,35.2426635148013,21.8548943744792));
#58792=CARTESIAN_POINT('Ctrl Pts',(-12.1324358584799,38.6962896164025,21.6578149219108));
#58793=CARTESIAN_POINT('Ctrl Pts',(-8.07745368699706,38.8096791578444,21.4607354693423));
#58794=CARTESIAN_POINT('Ctrl Pts',(-5.75982441453476,35.480365093003,21.2636560167739));
#58795=CARTESIAN_POINT('Ctrl Pts',(-7.27392668303485,31.7169581325262,21.0665765642054));
#58796=CARTESIAN_POINT('Ctrl Pts',(-11.2515073851604,30.9203469708242,20.869497111637));
#58797=CARTESIAN_POINT('Ctrl Pts',(-14.0981348468943,33.8104074558905,20.6724176590685));
#58798=CARTESIAN_POINT('Ctrl Pts',(-13.2413891249602,37.775470458552,20.4753382065001));
#58799=CARTESIAN_POINT('Ctrl Pts',(-9.45548806884112,39.2324160977332,20.2782587539317));
#58800=CARTESIAN_POINT('Ctrl Pts',(-6.16164765383978,36.86464238175,20.0811793013632));
#58801=CARTESIAN_POINT('Ctrl Pts',(-6.33642204041841,32.8118416838248,19.8840998487948));
#58802=CARTESIAN_POINT('Ctrl Pts',(-9.82187232757338,30.736420823802,19.6870203962264));
#58803=CARTESIAN_POINT('Ctrl Pts',(-13.4682918000352,32.5138795314929,19.4899409436579));
#58804=CARTESIAN_POINT('Ctrl Pts',(-13.9805100605527,36.5379801143958,19.2928614910895));
#58805=CARTESIAN_POINT('Ctrl Pts',(-10.8956496408777,39.172245220301,19.095782038521));
#58806=CARTESIAN_POINT('Ctrl Pts',(-7.00141460922806,38.0361747897458,18.8987025859526));
#58807=CARTESIAN_POINT('Ctrl Pts',(-5.81692047305108,34.1563773696868,18.7016231333842));
#58808=CARTESIAN_POINT('Ctrl Pts',(-8.41256032598399,31.0389752022047,18.5045436808157));
#58809=CARTESIAN_POINT('Ctrl Pts',(-12.4427290833343,31.5009711312537,18.3074642282473));
#58810=CARTESIAN_POINT('Ctrl Pts',(-14.2654643700508,35.1250887146591,18.1103847756788));
#58811=CARTESIAN_POINT('Ctrl Pts',(-12.233626332593,38.6358797395415,17.9133053231104));
#58812=CARTESIAN_POINT('Ctrl Pts',(-8.18329892127581,38.8615970187009,17.7162258705419));
#58813=CARTESIAN_POINT('Ctrl Pts',(-5.77471851411159,35.5965547375453,17.5191464179735));
#58814=CARTESIAN_POINT('Ctrl Pts',(-7.18432418012883,31.7946921672543,17.322066965405));
#58815=CARTESIAN_POINT('Ctrl Pts',(-11.1385421853802,30.8848376661246,17.1249875128366));
#58816=CARTESIAN_POINT('Ctrl Pts',(-14.0636669885939,33.7030483555917,16.9279080602682));
#58817=CARTESIAN_POINT('Ctrl Pts',(-13.5645470917968,36.3481490255669,16.7965217585559));
#58818=CARTESIAN_POINT('Ctrl Pts',(-12.8126841970975,37.2769248897959,16.7308286076997));
#58819=CARTESIAN_POINT('Ctrl Pts',(-7.07623665119056,37.5106317508166,30.2680483613301));
#58820=CARTESIAN_POINT('Ctrl Pts',(-6.24656234829778,36.544537827295,30.2023094747869));
#58821=CARTESIAN_POINT('Ctrl Pts',(-5.63436845003696,33.7426072919634,30.0708774373876));
#58822=CARTESIAN_POINT('Ctrl Pts',(-8.66394123666363,30.6536800364758,29.8737522491321));
#58823=CARTESIAN_POINT('Ctrl Pts',(-12.9006896360979,31.5030190569393,29.6766727965637));
#58824=CARTESIAN_POINT('Ctrl Pts',(-14.515853610602,35.5076551245181,29.4795933439952));
#58825=CARTESIAN_POINT('Ctrl Pts',(-12.0503233634801,39.0559509214177,29.2825138914268));
#58826=CARTESIAN_POINT('Ctrl Pts',(-7.73189084161409,38.9377826340795,29.0854344388583));
#58827=CARTESIAN_POINT('Ctrl Pts',(-5.46312754661196,35.2617553971811,28.8883549862899));
#58828=CARTESIAN_POINT('Ctrl Pts',(-7.29419231992886,31.3488814298923,28.6912755337214));
#58829=CARTESIAN_POINT('Ctrl Pts',(-11.5704322544924,30.7355775914529,28.494196081153));
#58830=CARTESIAN_POINT('Ctrl Pts',(-14.4275100643141,33.9758394412748,28.2971166285846));
#58831=CARTESIAN_POINT('Ctrl Pts',(-13.2835698325594,38.1416460728787,28.1000371760161));
#58832=CARTESIAN_POINT('Ctrl Pts',(-9.17235540750479,39.4684130224607,27.9029577234477));
#58833=CARTESIAN_POINT('Ctrl Pts',(-5.80906157815909,36.7572062162722,27.7058782708792));
#58834=CARTESIAN_POINT('Ctrl Pts',(-6.23300467487411,32.4580549655527,27.5087988183108));
#58835=CARTESIAN_POINT('Ctrl Pts',(-10.0610793238064,30.4559928811131,27.3117193657423));
#58836=CARTESIAN_POINT('Ctrl Pts',(-13.8339581638812,32.5602254079266,27.1146399131739));
#58837=CARTESIAN_POINT('Ctrl Pts',(-14.1421931582251,36.8692166058882,26.9175604606055));
#58838=CARTESIAN_POINT('Ctrl Pts',(-10.7072406499173,39.4890472011835,26.7204810080371));
#58839=CARTESIAN_POINT('Ctrl Pts',(-6.63317398081481,38.0522478909004,26.5234015554685));
#58840=CARTESIAN_POINT('Ctrl Pts',(-5.60161655873972,33.8572149623272,26.3263221029002));
#58841=CARTESIAN_POINT('Ctrl Pts',(-8.54475882345865,30.6948858811251,26.1292426503317));
#58842=CARTESIAN_POINT('Ctrl Pts',(-12.8029630231369,31.4229715102027,25.9321631977633));
#58843=CARTESIAN_POINT('Ctrl Pts',(-14.5282056498561,35.383520666463,25.7350837451948));
#58844=CARTESIAN_POINT('Ctrl Pts',(-12.161431787307,38.9974926053846,25.5380042926264));
#58845=CARTESIAN_POINT('Ctrl Pts',(-7.8414307092736,38.9990390254316,25.3409248400579));
#58846=CARTESIAN_POINT('Ctrl Pts',(-5.47207008637501,35.3867624650245,25.1438453874895));
#58847=CARTESIAN_POINT('Ctrl Pts',(-7.19447677710844,31.4249791675809,24.946765934921));
#58848=CARTESIAN_POINT('Ctrl Pts',(-11.4521586244438,30.6938451215836,24.7496864823526));
#58849=CARTESIAN_POINT('Ctrl Pts',(-14.3975641541361,33.8540663119965,24.5526070297842));
#58850=CARTESIAN_POINT('Ctrl Pts',(-13.3690103671906,38.0498366600148,24.3555275772157));
#58851=CARTESIAN_POINT('Ctrl Pts',(-9.29597339199564,39.4895524322982,24.1584481246473));
#58852=CARTESIAN_POINT('Ctrl Pts',(-5.859146145634,36.8721815787616,23.9613686720789));
#58853=CARTESIAN_POINT('Ctrl Pts',(-6.16429608859798,32.5629710688776,23.7642892195104));
#58854=CARTESIAN_POINT('Ctrl Pts',(-9.93566750333314,30.4560374300653,23.5672097669419));
#58855=CARTESIAN_POINT('Ctrl Pts',(-13.7651744484508,32.4553593810116,23.3701303143735));
#58856=CARTESIAN_POINT('Ctrl Pts',(-14.1921954823411,36.7542039633153,23.1730508618051));
#58857=CARTESIAN_POINT('Ctrl Pts',(-10.8308432918122,39.4678220568397,22.9759714092366));
#58858=CARTESIAN_POINT('Ctrl Pts',(-6.71868057881495,38.1439906747893,22.7788919566682));
#58859=CARTESIAN_POINT('Ctrl Pts',(-5.57175712728321,33.9790202904677,22.5818125040997));
#58860=CARTESIAN_POINT('Ctrl Pts',(-8.42651651733225,30.7366815463504,22.3847330515313));
#58861=CARTESIAN_POINT('Ctrl Pts',(-12.7031902050059,31.3469879247428,22.1876535989628));
#58862=CARTESIAN_POINT('Ctrl Pts',(-14.5370643056275,35.2584221229949,21.9905741463944));
#58863=CARTESIAN_POINT('Ctrl Pts',(-12.2709165906135,38.9363272664081,21.793494693826));
#58864=CARTESIAN_POINT('Ctrl Pts',(-7.95260321614858,39.0570803431483,21.5964152412575));
#58865=CARTESIAN_POINT('Ctrl Pts',(-5.48446672107112,35.5115600804189,21.3993357886891));
#58866=CARTESIAN_POINT('Ctrl Pts',(-7.09689503761302,31.5037568586754,21.2022563361206));
#58867=CARTESIAN_POINT('Ctrl Pts',(-11.3327804786878,30.6554136383235,21.0051768835522));
#58868=CARTESIAN_POINT('Ctrl Pts',(-14.3642683916493,33.7331551222299,20.8080974309837));
#58869=CARTESIAN_POINT('Ctrl Pts',(-13.4518854629247,37.9557099623979,20.6110179784153));
#58870=CARTESIAN_POINT('Ctrl Pts',(-9.42012737530255,39.5072698887991,20.4139385258469));
#58871=CARTESIAN_POINT('Ctrl Pts',(-5.91238442701437,36.9857325618673,20.2168590732784));
#58872=CARTESIAN_POINT('Ctrl Pts',(-6.09850869073715,32.6697423262084,20.01977962071));
#58873=CARTESIAN_POINT('Ctrl Pts',(-9.8103046874998,30.4595432973425,19.8227001681415));
#58874=CARTESIAN_POINT('Ctrl Pts',(-13.6935232346933,32.3524304631507,19.6256207155731));
#58875=CARTESIAN_POINT('Ctrl Pts',(-14.2390050325155,36.637856793641,19.4285412630047));
#58876=CARTESIAN_POINT('Ctrl Pts',(-10.9538132745039,39.4431915047816,19.2314618104362));
#58877=CARTESIAN_POINT('Ctrl Pts',(-6.80668598532695,38.2333444753415,19.0343823578678));
#58878=CARTESIAN_POINT('Ctrl Pts',(-5.54527060693137,34.1015923786047,18.8373029052994));
#58879=CARTESIAN_POINT('Ctrl Pts',(-8.3094717348775,30.7817456063805,18.6402234527309));
#58880=CARTESIAN_POINT('Ctrl Pts',(-12.6013603080527,31.2737436263448,18.4431440001625));
#58881=CARTESIAN_POINT('Ctrl Pts',(-14.5424643213063,35.1332119961725,18.246064547594));
#58882=CARTESIAN_POINT('Ctrl Pts',(-12.3786783906047,38.8719943622999,18.0489850950256));
#58883=CARTESIAN_POINT('Ctrl Pts',(-8.06532205718906,39.112369758349,17.8519056424571));
#58884=CARTESIAN_POINT('Ctrl Pts',(-5.50032804590148,35.635295099411,17.6548261898887));
#58885=CARTESIAN_POINT('Ctrl Pts',(-7.00147373356744,31.5865389542858,17.4577467373202));
#58886=CARTESIAN_POINT('Ctrl Pts',(-11.212479300426,30.6175983535903,17.2606672847518));
#58887=CARTESIAN_POINT('Ctrl Pts',(-14.3275621850144,33.6188241044634,17.0635878321833));
#58888=CARTESIAN_POINT('Ctrl Pts',(-13.7960293607869,36.4356980429703,16.932201530471));
#58889=CARTESIAN_POINT('Ctrl Pts',(-12.9953403671885,37.424788763168,16.8665083796149));
#58890=CARTESIAN_POINT('Ctrl Pts',(-6.89794525519566,37.6637303385885,30.4037281332453));
#58891=CARTESIAN_POINT('Ctrl Pts',(-6.01767732619968,36.6387239061743,30.3379892467021));
#58892=CARTESIAN_POINT('Ctrl Pts',(-5.36815177974479,33.6659313526057,30.2065572093028));
#58893=CARTESIAN_POINT('Ctrl Pts',(-8.58246823299407,30.3886409887524,30.0094320210473));
#58894=CARTESIAN_POINT('Ctrl Pts',(-13.077573994669,31.2897727918613,29.8123525684789));
#58895=CARTESIAN_POINT('Ctrl Pts',(-14.7912308379247,35.5386119873131,29.6152731159104));
#58896=CARTESIAN_POINT('Ctrl Pts',(-12.1753522974616,39.303283234466,29.418193663342));
#58897=CARTESIAN_POINT('Ctrl Pts',(-7.59358130699251,39.1779090325584,29.2211142107735));
#58898=CARTESIAN_POINT('Ctrl Pts',(-5.18646858804926,35.2777172687847,29.0240347582051));
#58899=CARTESIAN_POINT('Ctrl Pts',(-7.12919188349817,31.1262358361329,28.8269553056366));
#58900=CARTESIAN_POINT('Ctrl Pts',(-11.6661973782611,30.4755326652309,28.6298758530682));
#58901=CARTESIAN_POINT('Ctrl Pts',(-14.6975000929084,33.9133860228706,28.4327964004997));
#58902=CARTESIAN_POINT('Ctrl Pts',(-13.4838022657118,38.3332239802643,28.2357169479313));
#58903=CARTESIAN_POINT('Ctrl Pts',(-9.12188555335475,39.7408973177375,28.0386374953629));
#58904=CARTESIAN_POINT('Ctrl Pts',(-5.55349771316196,36.8643608358407,27.8415580427944));
#58905=CARTESIAN_POINT('Ctrl Pts',(-6.00329290442712,32.3030468904572,27.644478590226));
#58906=CARTESIAN_POINT('Ctrl Pts',(-10.0648039473853,30.178898849899,27.4473991376575));
#58907=CARTESIAN_POINT('Ctrl Pts',(-14.0677533352663,32.4114476971345,27.2503196850891));
#58908=CARTESIAN_POINT('Ctrl Pts',(-14.3947845319289,36.9832016307762,27.0532402325207));
#58909=CARTESIAN_POINT('Ctrl Pts',(-10.7503682590069,39.7627897708452,26.8561607799522));
#58910=CARTESIAN_POINT('Ctrl Pts',(-6.42786457666041,38.2383742877625,26.6590813273838));
#58911=CARTESIAN_POINT('Ctrl Pts',(-5.3334026746774,33.7875278107416,26.4620018748153));
#58912=CARTESIAN_POINT('Ctrl Pts',(-8.45601806371814,30.4323595701348,26.2649224222469));
#58913=CARTESIAN_POINT('Ctrl Pts',(-12.9738880025887,31.2048439373198,26.0678429696785));
#58914=CARTESIAN_POINT('Ctrl Pts',(-14.8043361058294,35.4069077969722,25.87076351711));
#58915=CARTESIAN_POINT('Ctrl Pts',(-12.2932361246394,39.241260124183,25.6736840645416));
#58916=CARTESIAN_POINT('Ctrl Pts',(-7.70980092728317,39.2429008450869,25.4766046119731));
#58917=CARTESIAN_POINT('Ctrl Pts',(-5.19595644482599,35.4103472807504,25.2795251594047));
#58918=CARTESIAN_POINT('Ctrl Pts',(-7.02339567640677,31.2069740218558,25.0824457068363));
#58919=CARTESIAN_POINT('Ctrl Pts',(-11.5407114098338,30.431255344967,24.8853662542678));
#58920=CARTESIAN_POINT('Ctrl Pts',(-14.6657280779835,33.7841871553832,24.6882868016994));
#58921=CARTESIAN_POINT('Ctrl Pts',(-13.5744529731157,38.2358160197642,24.4912073491309));
#58922=CARTESIAN_POINT('Ctrl Pts',(-9.25304177551932,39.7633258110065,24.2941278965625));
#58923=CARTESIAN_POINT('Ctrl Pts',(-5.60663644282017,36.9863474080067,24.097048443994));
#58924=CARTESIAN_POINT('Ctrl Pts',(-5.93039446134574,32.4143607887785,23.8999689914256));
#58925=CARTESIAN_POINT('Ctrl Pts',(-9.93174450093171,30.1789461154511,23.7028895388571));
#58926=CARTESIAN_POINT('Ctrl Pts',(-13.994775181647,32.3001869288876,23.5058100862887));
#58927=CARTESIAN_POINT('Ctrl Pts',(-14.4478360030196,36.8611755051832,23.3087306337203));
#58928=CARTESIAN_POINT('Ctrl Pts',(-10.8815082029825,39.7402703149709,23.1116511811518));
#58929=CARTESIAN_POINT('Ctrl Pts',(-6.51858537598449,38.3357115562455,22.9145717285834));
#58930=CARTESIAN_POINT('Ctrl Pts',(-5.30172241195556,33.9167608405812,22.7174922760149));
#58931=CARTESIAN_POINT('Ctrl Pts',(-8.33056532934912,30.4767039394141,22.5204128234465));
#58932=CARTESIAN_POINT('Ctrl Pts',(-12.8680310275323,31.1242268648406,22.323333370878));
#58933=CARTESIAN_POINT('Ctrl Pts',(-14.8137349633598,35.2741807311886,22.1262539183096));
#58934=CARTESIAN_POINT('Ctrl Pts',(-12.409397322747,39.1763649164138,21.9291744657412));
#58935=CARTESIAN_POINT('Ctrl Pts',(-7.82775274530012,39.3044815284521,21.7320950131727));
#58936=CARTESIAN_POINT('Ctrl Pts',(-5.20910902760746,35.5427550678348,21.5350155606043));
#58937=CARTESIAN_POINT('Ctrl Pts',(-6.91986339219122,31.2905555848246,21.3379361080358));
#58938=CARTESIAN_POINT('Ctrl Pts',(-11.4140535722153,30.3904803058226,21.1408566554674));
#58939=CARTESIAN_POINT('Ctrl Pts',(-14.6304019364044,33.6559027885695,20.9437772028989));
#58940=CARTESIAN_POINT('Ctrl Pts',(-13.6623818008893,38.1359494662436,20.7466977503305));
#58941=CARTESIAN_POINT('Ctrl Pts',(-9.384766681764,39.7821236798649,20.549618297762));
#58942=CARTESIAN_POINT('Ctrl Pts',(-5.66312120018892,37.1068227419848,20.3525388451936));
#58943=CARTESIAN_POINT('Ctrl Pts',(-5.86059534105592,32.5276429685921,20.1554593926252));
#58944=CARTESIAN_POINT('Ctrl Pts',(-9.79873704742623,30.182665770883,19.9583799400567));
#58945=CARTESIAN_POINT('Ctrl Pts',(-13.9187546693514,32.1909813948084,19.7613004874883));
#58946=CARTESIAN_POINT('Ctrl Pts',(-14.4975000044784,36.7377334728862,19.5642210349199));
#58947=CARTESIAN_POINT('Ctrl Pts',(-11.0119769081301,39.714137789262,19.3671415823514));
#58948=CARTESIAN_POINT('Ctrl Pts',(-6.61195736142583,38.4305141609372,19.170062129783));
#58949=CARTESIAN_POINT('Ctrl Pts',(-5.27362074081168,34.0468073875224,18.9729826772145));
#58950=CARTESIAN_POINT('Ctrl Pts',(-8.20638314377102,30.5245160105561,18.7759032246461));
#58951=CARTESIAN_POINT('Ctrl Pts',(-12.7599915327711,31.046516121436,18.5788237720777));
#58952=CARTESIAN_POINT('Ctrl Pts',(-14.8194642725618,35.1413352776858,18.3817443195092));
#58953=CARTESIAN_POINT('Ctrl Pts',(-12.5237304486164,39.1081089850583,18.1846648669408));
#58954=CARTESIAN_POINT('Ctrl Pts',(-7.9473451931023,39.3631424979969,17.9875854143723));
#58955=CARTESIAN_POINT('Ctrl Pts',(-5.22593757769137,35.6740354612769,17.7905059618039));
#58956=CARTESIAN_POINT('Ctrl Pts',(-6.81862328700602,31.3783857413171,17.5934265092354));
#58957=CARTESIAN_POINT('Ctrl Pts',(-11.2864164154719,30.350359041056,17.396347056667));
#58958=CARTESIAN_POINT('Ctrl Pts',(-14.5914573814348,33.5345998533351,17.1992676040985));
#58959=CARTESIAN_POINT('Ctrl Pts',(-14.027511629777,36.5232470603737,17.0678813023862));
#58960=CARTESIAN_POINT('Ctrl Pts',(-13.1779965372794,37.5726526365399,17.0021881515301));
#58961=CARTESIAN_POINT('Ctrl Pts',(-7.42676557298524,37.2065515280923,30.));
#58962=CARTESIAN_POINT('Ctrl Pts',(-7.34847363574758,37.1320407500307,30.));
#58963=CARTESIAN_POINT('Ctrl Pts',(-7.27428885024511,37.0537355480842,30.));
#58964=CARTESIAN_POINT('Ctrl Pts',(-7.20420769434694,36.9720784599283,30.));
#58965=CARTESIAN_POINT('Ctrl Pts',(-7.13363378334808,36.889847223898,30.));
#58966=CARTESIAN_POINT('Ctrl Pts',(-7.06722107630683,36.8042162244444,30.));
#58967=CARTESIAN_POINT('Ctrl Pts',(-7.00499287349493,36.7155880934709,30.));
#58968=CARTESIAN_POINT('Ctrl Pts',(-6.94120645481753,36.6247406832387,30.));
#58969=CARTESIAN_POINT('Ctrl Pts',(-6.88181624422247,36.5307436329052,30.));
#58970=CARTESIAN_POINT('Ctrl Pts',(-6.8268818722938,36.4339872175739,30.));
#58971=CARTESIAN_POINT('Ctrl Pts',(-6.77575400980664,36.3439352423875,30.));
#58972=CARTESIAN_POINT('Ctrl Pts',(-6.72848597396037,36.2514921521688,30.));
#58973=CARTESIAN_POINT('Ctrl Pts',(-6.68515714892584,36.1569468353438,30.));
#58974=CARTESIAN_POINT('Ctrl Pts',(-6.67815238204425,36.1416621396804,30.));
#58975=CARTESIAN_POINT('Ctrl Pts',(-6.67124986444939,36.1263207030674,30.));
#58976=CARTESIAN_POINT('Ctrl Pts',(-6.664452461429,36.1109292548971,30.));
#58977=CARTESIAN_POINT('Ctrl Pts',(-6.61833776570796,36.0065111489012,30.));
#58978=CARTESIAN_POINT('Ctrl Pts',(-6.57720059468109,35.9001204628048,30.));
#58979=CARTESIAN_POINT('Ctrl Pts',(-6.54106484244435,35.7921934874974,30.));
#58980=CARTESIAN_POINT('Ctrl Pts',(-6.50446358285172,35.6828761771951,30.));
#58981=CARTESIAN_POINT('Ctrl Pts',(-6.47299300143779,35.571982021054,30.));
#58982=CARTESIAN_POINT('Ctrl Pts',(-6.44671693976219,35.4599265310262,30.));
#58983=CARTESIAN_POINT('Ctrl Pts',(-6.42039387087784,35.3476705765652,30.));
#58984=CARTESIAN_POINT('Ctrl Pts',(-6.39928354477019,35.2342483047979,30.));
#58985=CARTESIAN_POINT('Ctrl Pts',(-6.38349503862451,35.1200514719229,30.));
#58986=CARTESIAN_POINT('Ctrl Pts',(-6.37020038024279,35.0238924137234,30.));
#58987=CARTESIAN_POINT('Ctrl Pts',(-6.36067977039915,34.9271834452265,30.));
#58988=CARTESIAN_POINT('Ctrl Pts',(-6.35502598487487,34.8301507851366,30.));
#58989=CARTESIAN_POINT('Ctrl Pts',(-6.35382226773603,34.8094920821356,30.));
#58990=CARTESIAN_POINT('Ctrl Pts',(-6.35279385607806,34.7888170008357,30.));
#58991=CARTESIAN_POINT('Ctrl Pts',(-6.35194202070525,34.7681330554352,30.));
#58992=CARTESIAN_POINT('Ctrl Pts',(-6.35128574764422,34.7521976803671,30.));
#58993=CARTESIAN_POINT('Ctrl Pts',(-6.35073447381912,34.7362615104886,30.));
#58994=CARTESIAN_POINT('Ctrl Pts',(-6.35028852693944,34.7203312537507,30.));
#58995=CARTESIAN_POINT('Ctrl Pts',(-6.34696763355239,34.6017012404777,30.));
#58996=CARTESIAN_POINT('Ctrl Pts',(-6.34947949264528,34.4832921867427,30.));
#58997=CARTESIAN_POINT('Ctrl Pts',(-6.3578907267476,34.3655323240003,30.));
#58998=CARTESIAN_POINT('Ctrl Pts',(-6.36625571653258,34.2484198959146,30.));
#58999=CARTESIAN_POINT('Ctrl Pts',(-6.38045508742067,34.1319486514061,30.));
#59000=CARTESIAN_POINT('Ctrl Pts',(-6.40060258265579,34.0165227778237,30.));
#59001=CARTESIAN_POINT('Ctrl Pts',(-6.40380809020162,33.998158286137,30.));
#59002=CARTESIAN_POINT('Ctrl Pts',(-6.40716427052324,33.9798202372895,30.));
#59003=CARTESIAN_POINT('Ctrl Pts',(-6.4106717030966,33.9615102423084,30.));
#59004=CARTESIAN_POINT('Ctrl Pts',(-6.43232586871275,33.8484681080808,30.));
#59005=CARTESIAN_POINT('Ctrl Pts',(-6.45974073675761,33.7364949627291,30.));
#59006=CARTESIAN_POINT('Ctrl Pts',(-6.49261497570932,33.6258527948074,30.));
#59007=CARTESIAN_POINT('Ctrl Pts',(-6.5133569109009,33.5560433406674,30.));
#59008=CARTESIAN_POINT('Ctrl Pts',(-6.53627330083344,33.4867637689423,30.));
#59009=CARTESIAN_POINT('Ctrl Pts',(-6.56129893452937,33.4180815844293,30.));
#59010=CARTESIAN_POINT('Ctrl Pts',(-6.56744615902576,33.4012106906796,30.));
#59011=CARTESIAN_POINT('Ctrl Pts',(-6.57372068647934,33.384375851465,30.));
#59012=CARTESIAN_POINT('Ctrl Pts',(-6.5801216201336,33.3675780879759,30.));
#59013=CARTESIAN_POINT('Ctrl Pts',(-6.58592025317676,33.3523609225308,30.));
#59014=CARTESIAN_POINT('Ctrl Pts',(-6.59182097681593,33.3371786053701,30.));
#59015=CARTESIAN_POINT('Ctrl Pts',(-6.59781984998277,33.3220394150435,30.));
#59016=CARTESIAN_POINT('Ctrl Pts',(-6.64115049854471,33.2126870554737,30.));
#59017=CARTESIAN_POINT('Ctrl Pts',(-6.68964292214754,33.1054651171024,30.));
#59018=CARTESIAN_POINT('Ctrl Pts',(-6.74292857838681,33.0006347052758,30.));
#59019=CARTESIAN_POINT('Ctrl Pts',(-6.7971983889184,32.8938681382613,30.));
#59020=CARTESIAN_POINT('Ctrl Pts',(-6.85644039141944,32.7895815913385,30.));
#59021=CARTESIAN_POINT('Ctrl Pts',(-6.92032038581974,32.6880544158277,30.));
#59022=CARTESIAN_POINT('Ctrl Pts',(-6.9852980783428,32.5847826222873,30.));
#59023=CARTESIAN_POINT('Ctrl Pts',(-7.05507485691378,32.484365082995,30.));
#59024=CARTESIAN_POINT('Ctrl Pts',(-7.12935095295689,32.3871103075363,30.));
#59025=CARTESIAN_POINT('Ctrl Pts',(-7.18304703332837,32.3168023549413,30.));
#59026=CARTESIAN_POINT('Ctrl Pts',(-7.23909566705282,32.2481475927666,30.));
#59027=CARTESIAN_POINT('Ctrl Pts',(-7.29739847574476,32.1812706915235,30.));
#59028=CARTESIAN_POINT('Ctrl Pts',(-7.31474064201097,32.1613781620425,30.));
#59029=CARTESIAN_POINT('Ctrl Pts',(-7.33228232709857,32.1416429873077,30.));
#59030=CARTESIAN_POINT('Ctrl Pts',(-7.35002113254827,32.1220685998336,30.));
#59031=CARTESIAN_POINT('Ctrl Pts',(-7.36801595625955,32.1022117017549,30.));
#59032=CARTESIAN_POINT('Ctrl Pts',(-7.38621564046034,32.0825183614633,30.));
#59033=CARTESIAN_POINT('Ctrl Pts',(-7.40459523086067,32.0630154735846,30.));
#59034=CARTESIAN_POINT('Ctrl Pts',(-7.49052313537484,31.971835950489,30.));
#59035=CARTESIAN_POINT('Ctrl Pts',(-7.58048269396152,31.884701382044,30.));
#59036=CARTESIAN_POINT('Ctrl Pts',(-7.6741413572269,31.8019256291752,30.));
#59037=CARTESIAN_POINT('Ctrl Pts',(-7.7679471631547,31.7190198312658,30.));
#59038=CARTESIAN_POINT('Ctrl Pts',(-7.86546422372204,31.6404857796622,30.));
#59039=CARTESIAN_POINT('Ctrl Pts',(-7.96640243919652,31.5666660266351,30.));
#59040=CARTESIAN_POINT('Ctrl Pts',(-7.99169676439379,31.5481673754526,30.));
#59041=CARTESIAN_POINT('Ctrl Pts',(-8.01720611984243,31.5299649311879,30.));
#59042=CARTESIAN_POINT('Ctrl Pts',(-8.04292631309347,31.512064441274,30.));
#59043=CARTESIAN_POINT('Ctrl Pts',(-8.06988678062553,31.4933007573303,30.));
#59044=CARTESIAN_POINT('Ctrl Pts',(-8.0970847011253,31.4748651824742,30.));
#59045=CARTESIAN_POINT('Ctrl Pts',(-8.12448495777706,31.4567841571235,30.));
#59046=CARTESIAN_POINT('Ctrl Pts',(-8.23136544948198,31.3862552965884,30.));
#59047=CARTESIAN_POINT('Ctrl Pts',(-8.34138288217212,31.3210724845241,30.));
#59048=CARTESIAN_POINT('Ctrl Pts',(-8.45421443341316,31.2615806352042,30.));
#59049=CARTESIAN_POINT('Ctrl Pts',(-8.56704598465418,31.2020887858843,30.));
#59050=CARTESIAN_POINT('Ctrl Pts',(-8.68269223981398,31.1482870733463,30.0000000000001));
#59051=CARTESIAN_POINT('Ctrl Pts',(-8.80086775832496,31.1005606444914,30.0000000000001));
#59052=CARTESIAN_POINT('Ctrl Pts',(-8.84648330399997,31.0821383255308,30.0000000000001));
#59053=CARTESIAN_POINT('Ctrl Pts',(-8.89247604481757,31.064621682834,30.));
#59054=CARTESIAN_POINT('Ctrl Pts',(-8.93882133655981,31.0480037218324,30.));
#59055=CARTESIAN_POINT('Ctrl Pts',(-11.0588859455903,31.0507007332205,29.9978118085731));
#59056=CARTESIAN_POINT('Ctrl Pts',(-12.3629832357829,31.4003552412704,29.932118657717));
#59057=CARTESIAN_POINT('Ctrl Pts',(-14.5759074258155,33.4867445316354,29.8007323560046));
#59058=CARTESIAN_POINT('Ctrl Pts',(-13.7737234475427,38.005501208821,29.6036529034362));
#59059=CARTESIAN_POINT('Ctrl Pts',(-9.55494358652074,39.7999145328719,29.4065734508678));
#59060=CARTESIAN_POINT('Ctrl Pts',(-5.74151403809183,37.2608171620003,29.2094939982993));
#59061=CARTESIAN_POINT('Ctrl Pts',(-5.77477638536515,32.6766638459004,29.0124145457309));
#59062=CARTESIAN_POINT('Ctrl Pts',(-9.62705490761888,30.1930581540609,28.8153350931624));
#59063=CARTESIAN_POINT('Ctrl Pts',(-13.8159539064568,32.0528472439456,28.618255640594));
#59064=CARTESIAN_POINT('Ctrl Pts',(-14.5566797841821,36.5761533733236,28.4211761880255));
#59065=CARTESIAN_POINT('Ctrl Pts',(-11.1795570301019,39.6750043826236,28.2240967354571));
#59066=CARTESIAN_POINT('Ctrl Pts',(-6.73655125706319,38.5492452105912,28.0270172828887));
#59067=CARTESIAN_POINT('Ctrl Pts',(-5.24261006855395,34.2160972081087,27.8299378303202));
#59068=CARTESIAN_POINT('Ctrl Pts',(-8.04780575158656,30.5913570973815,27.6328583777518));
#59069=CARTESIAN_POINT('Ctrl Pts',(-12.6171399548574,30.9505797199039,27.4357789251833));
#59070=CARTESIAN_POINT('Ctrl Pts',(-14.8214390660459,34.9691575849492,27.2386994726149));
#59071=CARTESIAN_POINT('Ctrl Pts',(-12.6687329951577,39.0156048483263,27.0416200200464));
#59072=CARTESIAN_POINT('Ctrl Pts',(-8.10436619426024,39.4332600799899,26.844540567478));
#59073=CARTESIAN_POINT('Ctrl Pts',(-5.25303178258637,35.8446980379474,26.6474611149096));
#59074=CARTESIAN_POINT('Ctrl Pts',(-6.69140385677929,31.4928055757625,26.4503816623411));
#59075=CARTESIAN_POINT('Ctrl Pts',(-11.1196643226323,30.3102693513275,26.2533022097727));
#59076=CARTESIAN_POINT('Ctrl Pts',(-14.5361145946286,33.3657154368998,26.0562227572043));
#59077=CARTESIAN_POINT('Ctrl Pts',(-13.8534012531181,37.8980200725724,25.8591433046358));
#59078=CARTESIAN_POINT('Ctrl Pts',(-9.68847384569797,39.8114626767306,25.6620638520674));
#59079=CARTESIAN_POINT('Ctrl Pts',(-5.80506415833992,37.3769170998905,25.4649843994989));
#59080=CARTESIAN_POINT('Ctrl Pts',(-5.71250408699149,32.7944160857802,25.2679049469305));
#59081=CARTESIAN_POINT('Ctrl Pts',(-9.49443764986189,30.2050413634305,25.070825494362));
#59082=CARTESIAN_POINT('Ctrl Pts',(-13.7332341815699,31.9487405618712,24.8737460417936));
#59083=CARTESIAN_POINT('Ctrl Pts',(-14.5984083535233,36.449780061507,24.6766665892252));
#59084=CARTESIAN_POINT('Ctrl Pts',(-11.3081257596992,39.6406926864939,24.4795871366567));
#59085=CARTESIAN_POINT('Ctrl Pts',(-6.83572543698307,38.6379373418252,24.2825076840883));
#59086=CARTESIAN_POINT('Ctrl Pts',(-5.22279411564314,34.347676804315,24.0854282315198));
#59087=CARTESIAN_POINT('Ctrl Pts',(-7.9268940338903,30.6469030258237,23.8883487789514));
#59088=CARTESIAN_POINT('Ctrl Pts',(-12.5044035215461,30.8799047808937,23.6912693263829));
#59089=CARTESIAN_POINT('Ctrl Pts',(-14.8187515502098,34.836124710266,23.4941898738145));
#59090=CARTESIAN_POINT('Ctrl Pts',(-12.7785246491449,38.9404342891812,23.297110421246));
#59091=CARTESIAN_POINT('Ctrl Pts',(-8.22742046944141,39.4838803977224,23.1000309686776));
#59092=CARTESIAN_POINT('Ctrl Pts',(-5.27814827968767,35.9753655441003,22.9029515161092));
#59093=CARTESIAN_POINT('Ctrl Pts',(-6.5958852745562,31.5854393328981,22.7058720635407));
#59094=CARTESIAN_POINT('Ctrl Pts',(-10.9898283130341,30.2811588791444,22.5087926109723));
#59095=CARTESIAN_POINT('Ctrl Pts',(-14.4892903823489,33.241167013002,22.3117131584039));
#59096=CARTESIAN_POINT('Ctrl Pts',(-13.9319026333332,37.7905847587297,22.1146337058354));
#59097=CARTESIAN_POINT('Ctrl Pts',(-9.82136123958291,39.8182268321212,21.917554253267));
#59098=CARTESIAN_POINT('Ctrl Pts',(-5.8722508431256,37.4917681495545,21.7204748006985));
#59099=CARTESIAN_POINT('Ctrl Pts',(-5.65327527635101,32.9135662500072,21.5233953481301));
#59100=CARTESIAN_POINT('Ctrl Pts',(-9.36231681406144,30.2208178773872,21.3263158955616));
#59101=CARTESIAN_POINT('Ctrl Pts',(-13.6476153301248,31.8468866149734,21.1292364429932));
#59102=CARTESIAN_POINT('Ctrl Pts',(-14.6366629208727,36.322338304894,20.9321569904247));
#59103=CARTESIAN_POINT('Ctrl Pts',(-11.435684126237,39.6028287659043,20.7350775378563));
#59104=CARTESIAN_POINT('Ctrl Pts',(-6.93731658184864,38.7238678721151,20.5379980852879));
#59105=CARTESIAN_POINT('Ctrl Pts',(-5.20661285740024,34.4797486630162,20.3409186327194));
#59106=CARTESIAN_POINT('Ctrl Pts',(-7.8075629807243,30.7057665311668,20.143839180151));
#59107=CARTESIAN_POINT('Ctrl Pts',(-12.3897588173874,30.8123664406772,19.9467597275825));
#59108=CARTESIAN_POINT('Ctrl Pts',(-14.8123946775176,34.7032173689442,19.7496802750141));
#59109=CARTESIAN_POINT('Ctrl Pts',(-12.886199790056,38.8622621440323,19.5526008224457));
#59110=CARTESIAN_POINT('Ctrl Pts',(-8.35182522203339,39.5310866051571,19.3555213698772));
#59111=CARTESIAN_POINT('Ctrl Pts',(-5.30686005482489,36.1052889229368,19.1584419173088));
#59112=CARTESIAN_POINT('Ctrl Pts',(-6.50296079309576,31.6806760610448,18.9613624647403));
#59113=CARTESIAN_POINT('Ctrl Pts',(-10.859235384841,30.2556373346469,18.7642830121719));
#59114=CARTESIAN_POINT('Ctrl Pts',(-14.4390532842977,33.1179677999974,18.5672035596034));
#59115=CARTESIAN_POINT('Ctrl Pts',(-14.007397374698,37.6810048575257,18.370124107035));
#59116=CARTESIAN_POINT('Ctrl Pts',(-9.95440886694127,39.8213599285263,18.1730446544665));
#59117=CARTESIAN_POINT('Ctrl Pts',(-5.94253301752884,37.6046449412306,17.9759652018981));
#59118=CARTESIAN_POINT('Ctrl Pts',(-5.59745277486287,33.0344578654708,17.7788857493297));
#59119=CARTESIAN_POINT('Ctrl Pts',(-9.23049066470893,30.2399305822798,17.5818062967612));
#59120=CARTESIAN_POINT('Ctrl Pts',(-13.5595988951335,31.7480386482111,17.3847268441928));
#59121=CARTESIAN_POINT('Ctrl Pts',(-14.670627205324,36.1926844691458,17.1876473916243));
#59122=CARTESIAN_POINT('Ctrl Pts',(-11.5636807183284,39.5638721263731,16.9905679390559));
#59123=CARTESIAN_POINT('Ctrl Pts',(-7.03690372967489,38.8018166892409,16.7934427493524));
#59124=CARTESIAN_POINT('Ctrl Pts',(-5.81501543623371,36.0149950038524,16.6620107105051));
#59125=CARTESIAN_POINT('Ctrl Pts',(-5.92468352323803,34.6683388238581,16.5962718225139));
#59126=CARTESIAN_POINT('Ctrl Pts',(-10.9980261816851,31.2776878057835,30.1334916301794));
#59127=CARTESIAN_POINT('Ctrl Pts',(-12.227170117816,31.6072458238412,30.0677984793232));
#59128=CARTESIAN_POINT('Ctrl Pts',(-14.312905875226,33.5737193100963,29.9364121776109));
#59129=CARTESIAN_POINT('Ctrl Pts',(-13.5568276439693,37.8327591918477,29.7393327250425));
#59130=CARTESIAN_POINT('Ctrl Pts',(-9.58052332753221,39.5240381115701,29.5422532724741));
#59131=CARTESIAN_POINT('Ctrl Pts',(-5.98627170185645,37.1308760675081,29.3451738199056));
#59132=CARTESIAN_POINT('Ctrl Pts',(-6.01762228647917,32.8101982368328,29.1480943673372));
#59133=CARTESIAN_POINT('Ctrl Pts',(-9.6484900304161,30.4693384721336,28.9510149147687));
#59134=CARTESIAN_POINT('Ctrl Pts',(-13.5966308955247,32.2222356673857,28.7539354622003));
#59135=CARTESIAN_POINT('Ctrl Pts',(-14.2947833476373,36.4855635203007,28.5568560096318));
#59136=CARTESIAN_POINT('Ctrl Pts',(-11.111761662089,39.4063072069101,28.3597765570634));
#59137=CARTESIAN_POINT('Ctrl Pts',(-6.92411888022353,38.3452513560518,28.162697104495));
#59138=CARTESIAN_POINT('Ctrl Pts',(-5.51604237657456,34.2611522388586,27.9656176519265));
#59139=CARTESIAN_POINT('Ctrl Pts',(-8.16000865837793,30.8447450730304,27.7685381993581));
#59140=CARTESIAN_POINT('Ctrl Pts',(-12.4667191088512,31.1833212755231,27.5714587467896));
#59141=CARTESIAN_POINT('Ctrl Pts',(-14.5443255162198,34.9709302613231,27.3743792942212));
#59142=CARTESIAN_POINT('Ctrl Pts',(-12.5153468248265,38.7848068440426,27.1772998416527));
#59143=CARTESIAN_POINT('Ctrl Pts',(-8.21331827389517,39.1784572252324,26.9802203890843));
#59144=CARTESIAN_POINT('Ctrl Pts',(-5.5258650996976,35.7961487835401,26.7831409365158));
#59145=CARTESIAN_POINT('Ctrl Pts',(-6.88156633931391,31.6943825496736,26.5860614839474));
#59146=CARTESIAN_POINT('Ctrl Pts',(-11.0553113046209,30.5798129232734,26.388982031379));
#59147=CARTESIAN_POINT('Ctrl Pts',(-14.2754001480669,33.4596463962052,26.1919025788106));
#59148=CARTESIAN_POINT('Ctrl Pts',(-13.6319259455329,37.7314555637656,25.9948231262421));
#59149=CARTESIAN_POINT('Ctrl Pts',(-9.70637889796551,39.5349225226521,25.7977436736737));
#59150=CARTESIAN_POINT('Ctrl Pts',(-6.0461692612876,37.2403031292128,25.6006642211052));
#59151=CARTESIAN_POINT('Ctrl Pts',(-5.9589291057552,32.9211826340111,25.4035847685368));
#59152=CARTESIAN_POINT('Ctrl Pts',(-9.52349498639276,30.4806329432155,25.2065053159683));
#59153=CARTESIAN_POINT('Ctrl Pts',(-13.5186655098071,32.1241125457867,25.0094258633998));
#59154=CARTESIAN_POINT('Ctrl Pts',(-14.3341135558625,36.3664535496901,24.8123464108315));
#59155=CARTESIAN_POINT('Ctrl Pts',(-11.2329408682335,39.373967585048,24.615266958263));
#59156=CARTESIAN_POINT('Ctrl Pts',(-7.01759299659966,38.4288458824024,24.4181875056946));
#59157=CARTESIAN_POINT('Ctrl Pts',(-5.49736535106264,34.3851692612172,24.2211080531261));
#59158=CARTESIAN_POINT('Ctrl Pts',(-8.04604637524828,30.8970984838035,24.0240286005577));
#59159=CARTESIAN_POINT('Ctrl Pts',(-12.3604622333652,31.1167083982678,23.8269491479892));
#59160=CARTESIAN_POINT('Ctrl Pts',(-14.5417924661031,34.8455434880719,23.6298696954208));
#59161=CARTESIAN_POINT('Ctrl Pts',(-12.6188281729981,38.7139567336685,23.4327902428523));
#59162=CARTESIAN_POINT('Ctrl Pts',(-8.32929997042302,39.2261681261397,23.2357107902839));
#59163=CARTESIAN_POINT('Ctrl Pts',(-5.54953801915008,35.9193061384744,23.0386313377155));
#59164=CARTESIAN_POINT('Ctrl Pts',(-6.7915377141413,31.7816921558822,22.841551885147));
#59165=CARTESIAN_POINT('Ctrl Pts',(-10.9329376557458,30.5523755835666,22.6444724325786));
#59166=CARTESIAN_POINT('Ctrl Pts',(-14.2312671703968,33.3422564275734,22.4473929800101));
#59167=CARTESIAN_POINT('Ctrl Pts',(-13.7059154371107,37.6301951244339,22.2503135274417));
#59168=CARTESIAN_POINT('Ctrl Pts',(-9.83162855196778,39.5412979063323,22.0532340748733));
#59169=CARTESIAN_POINT('Ctrl Pts',(-6.10949437269923,37.3485530828893,21.8561546223048));
#59170=CARTESIAN_POINT('Ctrl Pts',(-5.9031044874614,33.0334846094467,21.6590751697364));
#59171=CARTESIAN_POINT('Ctrl Pts',(-9.3989678323361,30.4955026976495,21.4619957171679));
#59172=CARTESIAN_POINT('Ctrl Pts',(-13.4379676256357,32.0281126827842,21.2649162645995));
#59173=CARTESIAN_POINT('Ctrl Pts',(-14.3701694313254,36.2463365434447,21.067836812031));
#59174=CARTESIAN_POINT('Ctrl Pts',(-11.3531677822158,39.3382799038139,20.8707573594626));
#59175=CARTESIAN_POINT('Ctrl Pts',(-7.11334516218977,38.5098375315904,20.6736779068942));
#59176=CARTESIAN_POINT('Ctrl Pts',(-5.48211411513276,34.509650253147,20.4765984543257));
#59177=CARTESIAN_POINT('Ctrl Pts',(-7.93357390751589,30.9525787928234,20.2795190017573));
#59178=CARTESIAN_POINT('Ctrl Pts',(-12.2524067654289,31.0530518429187,20.0824395491888));
#59179=CARTESIAN_POINT('Ctrl Pts',(-14.5358009564349,34.7202750331171,19.8853600966204));
#59180=CARTESIAN_POINT('Ctrl Pts',(-12.7203146552709,38.6402775542801,19.6882806440519));
#59181=CARTESIAN_POINT('Ctrl Pts',(-8.44655452529733,39.2706611436872,19.4912011914835));
#59182=CARTESIAN_POINT('Ctrl Pts',(-5.57659957703449,36.0417621350167,19.2941217389151));
#59183=CARTESIAN_POINT('Ctrl Pts',(-6.70395409306934,31.8714551266196,19.0970422863466));
#59184=CARTESIAN_POINT('Ctrl Pts',(-10.8098505923823,30.5283208969295,18.8999628337782));
#59185=CARTESIAN_POINT('Ctrl Pts',(-14.1839174635131,33.2261381235637,18.7028833812097));
#59186=CARTESIAN_POINT('Ctrl Pts',(-13.7770710972414,37.5269133584954,18.5058039286413));
#59187=CARTESIAN_POINT('Ctrl Pts',(-9.95702922998006,39.5442509271512,18.3087244760728));
#59188=CARTESIAN_POINT('Ctrl Pts',(-6.17573705960266,37.4549422496039,18.1116450235044));
#59189=CARTESIAN_POINT('Ctrl Pts',(-5.85049039975504,33.1474279457251,17.914565570936));
#59190=CARTESIAN_POINT('Ctrl Pts',(-9.27471842754193,30.5135168945186,17.7174861183675));
#59191=CARTESIAN_POINT('Ctrl Pts',(-13.3550099596984,31.9349460303737,17.5204066657991));
#59192=CARTESIAN_POINT('Ctrl Pts',(-14.4021816090919,36.1241345979269,17.3233272132306));
#59193=CARTESIAN_POINT('Ctrl Pts',(-11.4738077346166,39.3015623079627,17.1262477606622));
#59194=CARTESIAN_POINT('Ctrl Pts',(-7.20720851102714,38.583306218796,16.9291225709587));
#59195=CARTESIAN_POINT('Ctrl Pts',(-6.05554858671976,35.9566578840173,16.7976905321114));
#59196=CARTESIAN_POINT('Ctrl Pts',(-6.15891346995523,34.6874011421,16.7319516441202));
#59197=CARTESIAN_POINT('Ctrl Pts',(-10.9371664177797,31.5046748783465,30.2691714517856));
#59198=CARTESIAN_POINT('Ctrl Pts',(-12.0913569998491,31.8141364064121,30.2034783009294));
#59199=CARTESIAN_POINT('Ctrl Pts',(-14.0499043246364,33.6606940885572,30.0720919992171));
#59200=CARTESIAN_POINT('Ctrl Pts',(-13.3399318403958,37.6600171748744,29.8750125466487));
#59201=CARTESIAN_POINT('Ctrl Pts',(-9.60610306854369,39.2481616902682,29.6779330940803));
#59202=CARTESIAN_POINT('Ctrl Pts',(-6.23102936562104,37.0009349730159,29.4808536415118));
#59203=CARTESIAN_POINT('Ctrl Pts',(-6.2604681875932,32.943732627765,29.2837741889434));
#59204=CARTESIAN_POINT('Ctrl Pts',(-9.6699251532133,30.7456187902063,29.0866947363749));
#59205=CARTESIAN_POINT('Ctrl Pts',(-13.3773078845926,32.3916240908258,28.8896152838065));
#59206=CARTESIAN_POINT('Ctrl Pts',(-14.0328869110925,36.3949736672779,28.6925358312381));
#59207=CARTESIAN_POINT('Ctrl Pts',(-11.0439662940763,39.1376100311967,28.4954563786696));
#59208=CARTESIAN_POINT('Ctrl Pts',(-7.11168650338384,38.1412575015122,28.2983769261012));
#59209=CARTESIAN_POINT('Ctrl Pts',(-5.78947468459519,34.3062072696085,28.1012974735327));
#59210=CARTESIAN_POINT('Ctrl Pts',(-8.27221156516931,31.0981330486793,27.9042180209643));
#59211=CARTESIAN_POINT('Ctrl Pts',(-12.316298262845,31.4160628311424,27.7071385683959));
#59212=CARTESIAN_POINT('Ctrl Pts',(-14.2672119663938,34.9727029376968,27.5100591158274));
#59213=CARTESIAN_POINT('Ctrl Pts',(-12.3619606544954,38.5540088397591,27.312979663259));
#59214=CARTESIAN_POINT('Ctrl Pts',(-8.32227035353011,38.9236543704749,27.1159002106905));
#59215=CARTESIAN_POINT('Ctrl Pts',(-5.7986984168088,35.7475995291328,26.9188207581221));
#59216=CARTESIAN_POINT('Ctrl Pts',(-7.07172882184853,31.8959595235848,26.7217413055536));
#59217=CARTESIAN_POINT('Ctrl Pts',(-10.9909582866094,30.8493564952194,26.5246618529852));
#59218=CARTESIAN_POINT('Ctrl Pts',(-14.0146857015052,33.5535773555107,26.3275824004167));
#59219=CARTESIAN_POINT('Ctrl Pts',(-13.4104506379478,37.5648910549589,26.1305029478483));
#59220=CARTESIAN_POINT('Ctrl Pts',(-9.72428395023304,39.2583823685737,25.9334234952798));
#59221=CARTESIAN_POINT('Ctrl Pts',(-6.28727436423529,37.1036891585352,25.7363440427114));
#59222=CARTESIAN_POINT('Ctrl Pts',(-6.20535412451891,33.0479491822421,25.539264590143));
#59223=CARTESIAN_POINT('Ctrl Pts',(-9.55255232292363,30.7562245230005,25.3421851375745));
#59224=CARTESIAN_POINT('Ctrl Pts',(-13.3040968380443,32.2994845297022,25.1451056850062));
#59225=CARTESIAN_POINT('Ctrl Pts',(-14.0698187582016,36.2831270378733,24.9480262324377));
#59226=CARTESIAN_POINT('Ctrl Pts',(-11.1577559767678,39.1072424836022,24.7509467798692));
#59227=CARTESIAN_POINT('Ctrl Pts',(-7.19946055621625,38.2197544229795,24.5538673273008));
#59228=CARTESIAN_POINT('Ctrl Pts',(-5.77193658648213,34.4226617181194,24.3567878747323));
#59229=CARTESIAN_POINT('Ctrl Pts',(-8.16519871660625,31.1472939417833,24.1597084221639));
#59230=CARTESIAN_POINT('Ctrl Pts',(-12.2165209451842,31.3535120156418,23.9626289695954));
#59231=CARTESIAN_POINT('Ctrl Pts',(-14.2648333819964,34.8549622658775,23.765549517027));
#59232=CARTESIAN_POINT('Ctrl Pts',(-12.4591316968514,38.4874791781558,23.5684700644586));
#59233=CARTESIAN_POINT('Ctrl Pts',(-8.43117947140467,38.968455854557,23.3713906118901));
#59234=CARTESIAN_POINT('Ctrl Pts',(-5.82092775861246,35.8632467328487,23.1743111593217));
#59235=CARTESIAN_POINT('Ctrl Pts',(-6.98719015372643,31.9779449788662,22.9772317067532));
#59236=CARTESIAN_POINT('Ctrl Pts',(-10.8760469984575,30.8235922879887,22.7801522541848));
#59237=CARTESIAN_POINT('Ctrl Pts',(-13.9732439584446,33.4433458421448,22.5830728016163));
#59238=CARTESIAN_POINT('Ctrl Pts',(-13.4799282408882,37.4698054901383,22.3859933490479));
#59239=CARTESIAN_POINT('Ctrl Pts',(-9.84189586435265,39.2643689805436,22.1889138964794));
#59240=CARTESIAN_POINT('Ctrl Pts',(-6.34673790227287,37.205338016224,21.991834443911));
#59241=CARTESIAN_POINT('Ctrl Pts',(-6.15293369857177,33.1534029688861,21.7947549913426));
#59242=CARTESIAN_POINT('Ctrl Pts',(-9.43561885061076,30.7701875179118,21.5976755387741));
#59243=CARTESIAN_POINT('Ctrl Pts',(-13.2283199211465,32.2093387505949,21.4005960862057));
#59244=CARTESIAN_POINT('Ctrl Pts',(-14.1036759417782,36.1703347819953,21.2035166336372));
#59245=CARTESIAN_POINT('Ctrl Pts',(-11.2706514381948,39.0737310417233,21.0064371810688));
#59246=CARTESIAN_POINT('Ctrl Pts',(-7.2893737425309,38.2958071910657,20.8093577285003));
#59247=CARTESIAN_POINT('Ctrl Pts',(-5.75761537286527,34.5395518432776,20.6122782759319));
#59248=CARTESIAN_POINT('Ctrl Pts',(-8.05958483430744,31.19939105448,20.4151988233635));
#59249=CARTESIAN_POINT('Ctrl Pts',(-12.1150547134704,31.2937372451604,20.218119370795));
#59250=CARTESIAN_POINT('Ctrl Pts',(-14.2592072353523,34.7373326972899,20.0210399182266));
#59251=CARTESIAN_POINT('Ctrl Pts',(-12.5544295204857,38.4182929645279,19.8239604656581));
#59252=CARTESIAN_POINT('Ctrl Pts',(-8.54128382856128,39.0102356822172,19.6268810130897));
#59253=CARTESIAN_POINT('Ctrl Pts',(-5.84633909924408,35.9782353470966,19.4298015605213));
#59254=CARTESIAN_POINT('Ctrl Pts',(-6.90494739304291,32.0622341921945,19.2327221079528));
#59255=CARTESIAN_POINT('Ctrl Pts',(-10.7604657999234,30.8010044592122,19.0356426553844));
#59256=CARTESIAN_POINT('Ctrl Pts',(-13.9287816427284,33.3343084471301,18.8385632028159));
#59257=CARTESIAN_POINT('Ctrl Pts',(-13.5467448197848,37.3728218594653,18.6414837502475));
#59258=CARTESIAN_POINT('Ctrl Pts',(-9.95964959301886,39.2671419257761,18.444404297679));
#59259=CARTESIAN_POINT('Ctrl Pts',(-6.40894110167649,37.3052395579773,18.2473248451106));
#59260=CARTESIAN_POINT('Ctrl Pts',(-6.10352802464721,33.2603980259793,18.0502453925421));
#59261=CARTESIAN_POINT('Ctrl Pts',(-9.31894619037493,30.7871032067572,17.8531659399737));
#59262=CARTESIAN_POINT('Ctrl Pts',(-13.1504210242633,32.1218534125364,17.6560864874053));
#59263=CARTESIAN_POINT('Ctrl Pts',(-14.1337360128598,36.0555847267079,17.4590070348368));
#59264=CARTESIAN_POINT('Ctrl Pts',(-11.3839347509046,39.0392524895524,17.2619275822684));
#59265=CARTESIAN_POINT('Ctrl Pts',(-7.3775132923794,38.3647957483509,17.064802392565));
#59266=CARTESIAN_POINT('Ctrl Pts',(-6.2960817372058,35.8983207641823,16.9333703537176));
#59267=CARTESIAN_POINT('Ctrl Pts',(-6.39314341667241,34.7064634603417,16.8676314657265));
#59268=CARTESIAN_POINT('Ctrl Pts',(-10.8763066538745,31.7316619509095,30.4048512733919));
#59269=CARTESIAN_POINT('Ctrl Pts',(-11.9555438818821,32.021026988983,30.3391581225357));
#59270=CARTESIAN_POINT('Ctrl Pts',(-13.7869027740469,33.7476688670181,30.2077718208234));
#59271=CARTESIAN_POINT('Ctrl Pts',(-13.1230360368224,37.487275157901,30.010692368255));
#59272=CARTESIAN_POINT('Ctrl Pts',(-9.63168280955517,38.9722852689663,29.8136129156865));
#59273=CARTESIAN_POINT('Ctrl Pts',(-6.47578702938564,36.8709938785236,29.6165334631181));
#59274=CARTESIAN_POINT('Ctrl Pts',(-6.50331408870724,33.0772670186974,29.4194540105497));
#59275=CARTESIAN_POINT('Ctrl Pts',(-9.6913602760105,31.0218991082791,29.2223745579812));
#59276=CARTESIAN_POINT('Ctrl Pts',(-13.1579848736605,32.5610125142658,29.0252951054128));
#59277=CARTESIAN_POINT('Ctrl Pts',(-13.7709904745478,36.3043838142549,28.8282156528444));
#59278=CARTESIAN_POINT('Ctrl Pts',(-10.9761709260635,38.8689128554832,28.6311362002759));
#59279=CARTESIAN_POINT('Ctrl Pts',(-7.29925412654417,37.9372636469728,28.4340567477075));
#59280=CARTESIAN_POINT('Ctrl Pts',(-6.0629069926158,34.3512623003585,28.236977295139));
#59281=CARTESIAN_POINT('Ctrl Pts',(-8.38441447196068,31.3515210243283,28.0398978425706));
#59282=CARTESIAN_POINT('Ctrl Pts',(-12.1658774168387,31.6488043867616,27.8428183900021));
#59283=CARTESIAN_POINT('Ctrl Pts',(-13.9900984165678,34.9744756140705,27.6457389374337));
#59284=CARTESIAN_POINT('Ctrl Pts',(-12.2085744841641,38.3232108354754,27.4486594848652));
#59285=CARTESIAN_POINT('Ctrl Pts',(-8.43122243316505,38.6688515157174,27.2515800322968));
#59286=CARTESIAN_POINT('Ctrl Pts',(-6.07153173392002,35.6990502747255,27.0545005797284));
#59287=CARTESIAN_POINT('Ctrl Pts',(-7.26189130438314,32.097536497496,26.8574211271599));
#59288=CARTESIAN_POINT('Ctrl Pts',(-10.9266052685981,31.1189000671652,26.6603416745915));
#59289=CARTESIAN_POINT('Ctrl Pts',(-13.7539712549434,33.6475083148162,26.463262222023));
#59290=CARTESIAN_POINT('Ctrl Pts',(-13.1889753303626,37.398326546152,26.2661827694546));
#59291=CARTESIAN_POINT('Ctrl Pts',(-9.74218900250058,38.9818422144952,26.0691033168861));
#59292=CARTESIAN_POINT('Ctrl Pts',(-6.52837946718296,36.9670751878574,25.8720238643177));
#59293=CARTESIAN_POINT('Ctrl Pts',(-6.45177914328262,33.1747157304732,25.6749444117493));
#59294=CARTESIAN_POINT('Ctrl Pts',(-9.58160965945451,31.0318161027855,25.4778649591808));
#59295=CARTESIAN_POINT('Ctrl Pts',(-13.0895281662815,32.4748565136177,25.2807855066124));
#59296=CARTESIAN_POINT('Ctrl Pts',(-13.8055239605408,36.1998005260564,25.0837060540439));
#59297=CARTESIAN_POINT('Ctrl Pts',(-11.0825710853022,38.8405173821563,24.8866266014755));
#59298=CARTESIAN_POINT('Ctrl Pts',(-7.38132811583285,38.0106629635567,24.6895471489071));
#59299=CARTESIAN_POINT('Ctrl Pts',(-6.04650782190161,34.4601541750215,24.4924676963386));
#59300=CARTESIAN_POINT('Ctrl Pts',(-8.28435105796425,31.3974893997631,24.2953882437702));
#59301=CARTESIAN_POINT('Ctrl Pts',(-12.0725796570033,31.5903156330156,24.0983087912017));
#59302=CARTESIAN_POINT('Ctrl Pts',(-13.9878742978896,34.8643810436833,23.9012293386333));
#59303=CARTESIAN_POINT('Ctrl Pts',(-12.2994352207047,38.2610016226431,23.7041498860648));
#59304=CARTESIAN_POINT('Ctrl Pts',(-8.53305897238628,38.7107435829743,23.5070704334964));
#59305=CARTESIAN_POINT('Ctrl Pts',(-6.09231749807485,35.8071873272227,23.309990980928));
#59306=CARTESIAN_POINT('Ctrl Pts',(-7.18284259331154,32.1741978018502,23.1129115283595));
#59307=CARTESIAN_POINT('Ctrl Pts',(-10.819156341169,31.0948089924109,22.9158320757911));
#59308=CARTESIAN_POINT('Ctrl Pts',(-13.7152207464925,33.5444352567162,22.7187526232226));
#59309=CARTESIAN_POINT('Ctrl Pts',(-13.2539410446657,37.3094158558426,22.5216731706542));
#59310=CARTESIAN_POINT('Ctrl Pts',(-9.85216317673751,38.9874400547548,22.3245937180858));
#59311=CARTESIAN_POINT('Ctrl Pts',(-6.5839814318465,37.0621229495586,22.1275142655173));
#59312=CARTESIAN_POINT('Ctrl Pts',(-6.40276290968217,33.2733213283256,21.9304348129489));
#59313=CARTESIAN_POINT('Ctrl Pts',(-9.47226986888541,31.0448723381741,21.7333553603804));
#59314=CARTESIAN_POINT('Ctrl Pts',(-13.0186722166574,32.3905648184057,21.536275907812));
#59315=CARTESIAN_POINT('Ctrl Pts',(-13.8371824522311,36.094333020546,21.3391964552435));
#59316=CARTESIAN_POINT('Ctrl Pts',(-11.1881350941738,38.8091821796328,21.1421170026751));
#59317=CARTESIAN_POINT('Ctrl Pts',(-7.46540232287201,38.081776850541,20.9450375501066));
#59318=CARTESIAN_POINT('Ctrl Pts',(-6.0331166305978,34.5694534334084,20.7479580975382));
#59319=CARTESIAN_POINT('Ctrl Pts',(-8.185595761099,31.4462033161365,20.5508786449698));
#59320=CARTESIAN_POINT('Ctrl Pts',(-11.9777026615119,31.534422647402,20.3537991924013));
#59321=CARTESIAN_POINT('Ctrl Pts',(-13.9826135142697,34.7543903614628,20.1567197398329));
#59322=CARTESIAN_POINT('Ctrl Pts',(-12.3885443857005,38.1963083747756,19.9596402872644));
#59323=CARTESIAN_POINT('Ctrl Pts',(-8.63601313182522,38.7498102207472,19.762560834696));
#59324=CARTESIAN_POINT('Ctrl Pts',(-6.11607862145368,35.9147085591765,19.5654813821276));
#59325=CARTESIAN_POINT('Ctrl Pts',(-7.1059406930165,32.2530132577694,19.3684019295591));
#59326=CARTESIAN_POINT('Ctrl Pts',(-10.7110810074646,31.0736880214948,19.1713224769907));
#59327=CARTESIAN_POINT('Ctrl Pts',(-13.6736458219438,33.4424787706964,18.9742430244222));
#59328=CARTESIAN_POINT('Ctrl Pts',(-13.3164185423282,37.218730360435,18.7771635718538));
#59329=CARTESIAN_POINT('Ctrl Pts',(-9.96226995605767,38.990032924401,18.5800841192853));
#59330=CARTESIAN_POINT('Ctrl Pts',(-6.64214514375032,37.1555368663507,18.3830046667169));
#59331=CARTESIAN_POINT('Ctrl Pts',(-6.35656564953937,33.3733681062335,18.1859252141485));
#59332=CARTESIAN_POINT('Ctrl Pts',(-9.36317395320792,31.0606895189958,17.98884576158));
#59333=CARTESIAN_POINT('Ctrl Pts',(-12.9458320888283,32.308760794699,17.7917663090116));
#59334=CARTESIAN_POINT('Ctrl Pts',(-13.8652904166277,35.987034855489,17.5946868564431));
#59335=CARTESIAN_POINT('Ctrl Pts',(-11.2940617671928,38.776942671142,17.3976074038747));
#59336=CARTESIAN_POINT('Ctrl Pts',(-7.54781807373163,38.146285277906,17.2004822141713));
#59337=CARTESIAN_POINT('Ctrl Pts',(-6.53661488769183,35.8399836443472,17.0690501753239));
#59338=CARTESIAN_POINT('Ctrl Pts',(-6.62737336338959,34.7255257785834,17.0033112873327));
#59339=CARTESIAN_POINT('',(-12.5757516043532,37.208058672647,30.0016980799398));
#59340=CARTESIAN_POINT('Ctrl Pts',(-12.5735559834512,37.206176480371,30.0016980799398));
#59341=CARTESIAN_POINT('Ctrl Pts',(-12.5615840841705,37.2201419782817,30.0011320532932));
#59342=CARTESIAN_POINT('Ctrl Pts',(-12.5494985059473,37.2340100250842,30.0005660266466));
#59343=CARTESIAN_POINT('Ctrl Pts',(-12.5373008502128,37.2477787831567,30.));
#59344=CARTESIAN_POINT('Ctrl Pts',(-11.0579044229731,31.0543614925016,30.));
#59345=CARTESIAN_POINT('Ctrl Pts',(-11.1744097379893,31.0963766655822,30.));
#59346=CARTESIAN_POINT('Ctrl Pts',(-11.2885141402515,31.1440012484697,30.));
#59347=CARTESIAN_POINT('Ctrl Pts',(-11.3999877282899,31.1968709585829,30.));
#59348=CARTESIAN_POINT('Ctrl Pts',(-11.5131045963172,31.2505200437767,30.));
#59349=CARTESIAN_POINT('Ctrl Pts',(-11.6235131197498,31.3095706523587,30.));
#59350=CARTESIAN_POINT('Ctrl Pts',(-11.7309453563639,31.3736894626584,30.));
#59351=CARTESIAN_POINT('Ctrl Pts',(-11.8388145215838,31.4380690451737,30.));
#59352=CARTESIAN_POINT('Ctrl Pts',(-11.94368371586,31.507558840894,30.));
#59353=CARTESIAN_POINT('Ctrl Pts',(-12.045245115667,31.5818586971976,30.));
#59354=CARTESIAN_POINT('Ctrl Pts',(-12.141528578336,31.6522973427294,30.));
#59355=CARTESIAN_POINT('Ctrl Pts',(-12.2348392296536,31.7270598973032,30.));
#59356=CARTESIAN_POINT('Ctrl Pts',(-12.3248775992634,31.8059127430533,30.));
#59357=CARTESIAN_POINT('Ctrl Pts',(-12.3423428346842,31.8212082611818,30.));
#59358=CARTESIAN_POINT('Ctrl Pts',(-12.3596848250068,31.8366577328144,30.));
#59359=CARTESIAN_POINT('Ctrl Pts',(-12.3769012054219,31.8522595191162,30.));
#59360=CARTESIAN_POINT('Ctrl Pts',(-12.3882150003473,31.8625122787807,30.));
#59361=CARTESIAN_POINT('Ctrl Pts',(-12.399472582474,31.8728290762095,30.));
#59362=CARTESIAN_POINT('Ctrl Pts',(-12.4106671396558,31.8832035231787,30.));
#59363=CARTESIAN_POINT('Ctrl Pts',(-12.5011175434017,31.9670275549618,30.));
#59364=CARTESIAN_POINT('Ctrl Pts',(-12.587577051358,32.0547210466236,30.));
#59365=CARTESIAN_POINT('Ctrl Pts',(-12.6697884900426,32.1459687647768,30.));
#59366=CARTESIAN_POINT('Ctrl Pts',(-12.7516103599846,32.2367840946956,30.));
#59367=CARTESIAN_POINT('Ctrl Pts',(-12.8292247934612,32.3311207836379,30.));
#59368=CARTESIAN_POINT('Ctrl Pts',(-12.9023358107026,32.428696821173,30.));
#59369=CARTESIAN_POINT('Ctrl Pts',(-12.9737773812525,32.5240447677968,30.));
#59370=CARTESIAN_POINT('Ctrl Pts',(-13.0409191293949,32.6224865141385,30.));
#59371=CARTESIAN_POINT('Ctrl Pts',(-13.1034390161676,32.7237758029549,30.));
#59372=CARTESIAN_POINT('Ctrl Pts',(-13.1564936425993,32.8097302993092,30.));
#59373=CARTESIAN_POINT('Ctrl Pts',(-13.2062193154101,32.8977358680952,30.));
#59374=CARTESIAN_POINT('Ctrl Pts',(-13.2523900459045,32.9876465015809,30.));
#59375=CARTESIAN_POINT('Ctrl Pts',(-13.2633342592225,33.0089587299534,30.));
#59376=CARTESIAN_POINT('Ctrl Pts',(-13.2740786046814,33.0303780053924,30.));
#59377=CARTESIAN_POINT('Ctrl Pts',(-13.284619831996,33.0519023903029,30.));
#59378=CARTESIAN_POINT('Ctrl Pts',(-13.2922709150539,33.0675253203285,30.));
#59379=CARTESIAN_POINT('Ctrl Pts',(-13.2998110412698,33.0831956068833,30.));
#59380=CARTESIAN_POINT('Ctrl Pts',(-13.3072375789992,33.0989086300593,30.));
#59381=CARTESIAN_POINT('Ctrl Pts',(-13.3571203304174,33.2044502508889,30.));
#59382=CARTESIAN_POINT('Ctrl Pts',(-13.4019091124834,33.3119732815046,30.));
#59383=CARTESIAN_POINT('Ctrl Pts',(-13.4413385699665,33.4212276569007,30.));
#59384=CARTESIAN_POINT('Ctrl Pts',(-13.480554760447,33.5298910945909,30.));
#59385=CARTESIAN_POINT('Ctrl Pts',(-13.5144697968334,33.6402678129294,30.));
#59386=CARTESIAN_POINT('Ctrl Pts',(-13.5427725767595,33.752122444386,30.));
#59387=CARTESIAN_POINT('Ctrl Pts',(-13.5490249649288,33.7768323342352,30.));
#59388=CARTESIAN_POINT('Ctrl Pts',(-13.5550032600854,33.8016143697398,30.));
#59389=CARTESIAN_POINT('Ctrl Pts',(-13.5607037501708,33.8264660384264,30.));
#59390=CARTESIAN_POINT('Ctrl Pts',(-13.5872170560123,33.9420525726855,30.));
#59391=CARTESIAN_POINT('Ctrl Pts',(-13.6077248602857,34.0591462330772,30.));
#59392=CARTESIAN_POINT('Ctrl Pts',(-13.6223138164184,34.1773085476865,30.));
#59393=CARTESIAN_POINT('Ctrl Pts',(-13.6304389010778,34.2431171498245,30.));
#59394=CARTESIAN_POINT('Ctrl Pts',(-13.6367271752067,34.3092570719329,30.));
#59395=CARTESIAN_POINT('Ctrl Pts',(-13.6411869466529,34.3756503989149,30.));
#59396=CARTESIAN_POINT('Ctrl Pts',(-13.6425504665288,34.3959493362173,30.));
#59397=CARTESIAN_POINT('Ctrl Pts',(-13.6437430339725,34.4162719455193,30.));
#59398=CARTESIAN_POINT('Ctrl Pts',(-13.6447648023415,34.4366159566223,30.));
#59399=CARTESIAN_POINT('Ctrl Pts',(-13.6454921557764,34.4510979926728,30.));
#59400=CARTESIAN_POINT('Ctrl Pts',(-13.6461328377877,34.4655892371793,30.));
#59401=CARTESIAN_POINT('Ctrl Pts',(-13.6466867036911,34.4800794533411,30.));
#59402=CARTESIAN_POINT('Ctrl Pts',(-13.6511188462219,34.5960329773438,30.));
#59403=CARTESIAN_POINT('Ctrl Pts',(-13.6500050144421,34.7120892190283,30.));
#59404=CARTESIAN_POINT('Ctrl Pts',(-13.6434929003203,34.8278444120361,30.));
#59405=CARTESIAN_POINT('Ctrl Pts',(-13.6369460662828,34.9442167641516,30.));
#59406=CARTESIAN_POINT('Ctrl Pts',(-13.6249429285982,35.0602857712229,30.));
#59407=CARTESIAN_POINT('Ctrl Pts',(-13.6075815295661,35.1756316950981,30.));
#59408=CARTESIAN_POINT('Ctrl Pts',(-13.5904443779721,35.2894877604727,30.));
#59409=CARTESIAN_POINT('Ctrl Pts',(-13.5680860708864,35.4026401113781,30.));
#59410=CARTESIAN_POINT('Ctrl Pts',(-13.5405559702548,35.514663028091,30.));
#59411=CARTESIAN_POINT('Ctrl Pts',(-13.5211239632378,35.5937339378838,30.));
#59412=CARTESIAN_POINT('Ctrl Pts',(-13.4991143380556,35.6722417044066,30.));
#59413=CARTESIAN_POINT('Ctrl Pts',(-13.4745323439232,35.7500266063154,30.));
#59414=CARTESIAN_POINT('Ctrl Pts',(-13.4674334526882,35.7724896561152,30.));
#59415=CARTESIAN_POINT('Ctrl Pts',(-13.4601199750053,35.7948923594824,30.));
#59416=CARTESIAN_POINT('Ctrl Pts',(-13.4525918930855,35.8172307103604,30.));
#59417=CARTESIAN_POINT('Ctrl Pts',(-13.4468394074071,35.8343002700268,30.));
#59418=CARTESIAN_POINT('Ctrl Pts',(-13.4409618348628,35.8513313943885,30.));
#59419=CARTESIAN_POINT('Ctrl Pts',(-13.4349636589554,35.8683101630108,30.));
#59420=CARTESIAN_POINT('Ctrl Pts',(-13.3973630090629,35.9747446431643,30.));
#59421=CARTESIAN_POINT('Ctrl Pts',(-13.3549838397234,36.0792521464373,30.));
#59422=CARTESIAN_POINT('Ctrl Pts',(-13.3078911250007,36.1814300295353,30.));
#59423=CARTESIAN_POINT('Ctrl Pts',(-13.2675799744265,36.2688938348217,30.));
#59424=CARTESIAN_POINT('Ctrl Pts',(-13.2238142519443,36.3546505536924,30.));
#59425=CARTESIAN_POINT('Ctrl Pts',(-13.1766119737641,36.4384274454971,30.));
#59426=CARTESIAN_POINT('Ctrl Pts',(-13.1551452588006,36.4765276119769,30.));
#59427=CARTESIAN_POINT('Ctrl Pts',(-13.132967502798,36.514218007177,30.));
#59428=CARTESIAN_POINT('Ctrl Pts',(-13.110079097282,36.5514713768243,30.));
#59429=CARTESIAN_POINT('Ctrl Pts',(-13.0960864911787,36.5742458652932,30.));
#59430=CARTESIAN_POINT('Ctrl Pts',(-13.0818259721494,36.5968603357343,30.));
#59431=CARTESIAN_POINT('Ctrl Pts',(-13.0673126858154,36.6192855347161,30.));
#59432=CARTESIAN_POINT('Ctrl Pts',(-13.0087455119247,36.7097805816736,30.));
#59433=CARTESIAN_POINT('Ctrl Pts',(-12.9460227269703,36.7972676999888,30.));
#59434=CARTESIAN_POINT('Ctrl Pts',(-12.8791807735713,36.8813650266868,30.));
#59435=CARTESIAN_POINT('Ctrl Pts',(-12.8123388201723,36.9654623533848,30.));
#59436=CARTESIAN_POINT('Ctrl Pts',(-12.7413774124275,37.0461705445025,30.));
#59437=CARTESIAN_POINT('Ctrl Pts',(-12.6663017713996,37.1230656129614,30.));
#59438=CARTESIAN_POINT('Ctrl Pts',(-12.6374945150854,37.1525710013412,30.));
#59439=CARTESIAN_POINT('Ctrl Pts',(-12.6080811803488,37.1815144607823,30.));
#59440=CARTESIAN_POINT('Ctrl Pts',(-12.5780824317837,37.2098873180834,30.));
#59441=CARTESIAN_POINT('Origin',(130.,-35.,16.));
#59442=CARTESIAN_POINT('Origin',(-10.,-35.,16.));
#59443=CARTESIAN_POINT('Origin',(-10.,35.,16.));
#59444=CARTESIAN_POINT('Origin',(130.,35.,16.));
#59445=CARTESIAN_POINT('Origin',(140.,-60.,20.));
#59446=CARTESIAN_POINT('',(135.5,-60.,30.));
#59447=CARTESIAN_POINT('Origin',(140.,-60.,30.));
#59448=CARTESIAN_POINT('',(135.5,-60.,10.));
#59449=CARTESIAN_POINT('',(135.5,-60.,20.));
#59450=CARTESIAN_POINT('Origin',(140.,-60.,10.));
#59451=CARTESIAN_POINT('Origin',(-20.,-60.,20.));
#59452=CARTESIAN_POINT('',(-24.5,-60.,30.));
#59453=CARTESIAN_POINT('Origin',(-20.,-60.,30.));
#59454=CARTESIAN_POINT('',(-24.5,-60.,10.));
#59455=CARTESIAN_POINT('',(-24.5,-60.,20.));
#59456=CARTESIAN_POINT('Origin',(-20.,-60.,10.));
#59457=CARTESIAN_POINT('Origin',(-20.,60.,20.));
#59458=CARTESIAN_POINT('',(-24.5,60.,30.));
#59459=CARTESIAN_POINT('Origin',(-20.,60.,30.));
#59460=CARTESIAN_POINT('',(-24.5,60.,10.));
#59461=CARTESIAN_POINT('',(-24.5,60.,20.));
#59462=CARTESIAN_POINT('Origin',(-20.,60.,10.));
#59463=CARTESIAN_POINT('Origin',(140.,60.,20.));
#59464=CARTESIAN_POINT('',(135.5,60.,30.));
#59465=CARTESIAN_POINT('Origin',(140.,60.,30.));
#59466=CARTESIAN_POINT('',(135.5,60.,10.));
#59467=CARTESIAN_POINT('',(135.5,60.,20.));
#59468=CARTESIAN_POINT('Origin',(140.,60.,10.));
#59469=CARTESIAN_POINT('Origin',(160.,75.,10.));
#59470=CARTESIAN_POINT('',(165.,75.,10.));
#59471=CARTESIAN_POINT('',(-45.,75.,10.));
#59472=CARTESIAN_POINT('',(110.,75.,10.));
#59473=CARTESIAN_POINT('',(-45.,75.,30.));
#59474=CARTESIAN_POINT('',(-45.,75.,10.));
#59475=CARTESIAN_POINT('',(165.,75.,30.));
#59476=CARTESIAN_POINT('',(110.,75.,30.));
#59477=CARTESIAN_POINT('',(165.,75.,10.));
#59478=CARTESIAN_POINT('Origin',(165.,-70.,10.));
#59479=CARTESIAN_POINT('',(165.,-75.,10.));
#59480=CARTESIAN_POINT('',(165.,-35.,10.));
#59481=CARTESIAN_POINT('',(165.,-75.,30.));
#59482=CARTESIAN_POINT('',(165.,-35.,30.));
#59483=CARTESIAN_POINT('',(165.,-75.,10.));
#59484=CARTESIAN_POINT('Origin',(-40.,-75.,10.));
#59485=CARTESIAN_POINT('',(-45.,-75.,10.));
#59486=CARTESIAN_POINT('',(10.,-75.,10.));
#59487=CARTESIAN_POINT('',(-45.,-75.,30.));
#59488=CARTESIAN_POINT('',(10.,-75.,30.));
#59489=CARTESIAN_POINT('',(-45.,-75.,10.));
#59490=CARTESIAN_POINT('Origin',(-45.,70.,10.));
#59491=CARTESIAN_POINT('',(-45.,35.,10.));
#59492=CARTESIAN_POINT('',(-45.,35.,30.));
#59493=CARTESIAN_POINT('Origin',(60.,0.,30.));
#59494=CARTESIAN_POINT('Origin',(60.,0.,10.));
#289351=UNCERTAINTY_MEASURE_WITH_UNIT(LENGTH_MEASURE(0.01),#289388,
'DISTANCE_ACCURACY_VALUE',
'Maximum model space distance between geometric entities at asserted c
onnectivities');
#289368=UNCERTAINTY_MEASURE_WITH_UNIT(LENGTH_MEASURE(0.01),#289388,
'DISTANCE_ACCURACY_VALUE',
'Maximum model space distance between geometric entities at asserted c
onnectivities');
#289370=(
GEOMETRIC_REPRESENTATION_CONTEXT(3)
GLOBAL_UNCERTAINTY_ASSIGNED_CONTEXT((#289351))
GLOBAL_UNIT_ASSIGNED_CONTEXT((#289388,#289390,#289391))
REPRESENTATION_CONTEXT('','3D')
);
#289387=(
GEOMETRIC_REPRESENTATION_CONTEXT(3)
GLOBAL_UNCERTAINTY_ASSIGNED_CONTEXT((#289368))
GLOBAL_UNIT_ASSIGNED_CONTEXT((#289388,#289390,#289391))
REPRESENTATION_CONTEXT('','3D')
);
#289388=(
LENGTH_UNIT()
NAMED_UNIT(*)
SI_UNIT(.MILLI.,.METRE.)
);
#289390=(
NAMED_UNIT(*)
PLANE_ANGLE_UNIT()
SI_UNIT($,.RADIAN.)
);
#289391=(
NAMED_UNIT(*)
SI_UNIT($,.STERADIAN.)
SOLID_ANGLE_UNIT()
);
#289393=SHAPE_DEFINITION_REPRESENTATION(#289411,#289454);
#289411=PRODUCT_DEFINITION_SHAPE('',$,#289473);
#289454=SHAPE_REPRESENTATION('',(#17047),#289370);
#289471=PRODUCT_DEFINITION_CONTEXT('part definition',#289527,'design');
#289473=PRODUCT_DEFINITION('Base plate','Base plate',#289491,#289471);
#289491=PRODUCT_DEFINITION_FORMATION('',$,#289530);
#289527=APPLICATION_CONTEXT(
'Core Data for Automotive Mechanical Design Process');
#289528=PRODUCT_CONTEXT('part definition',#289527,'mechanical');
#289530=PRODUCT('Base plate','Base plate','Base plate',(#289528));
#289548=PRESENTATION_STYLE_ASSIGNMENT((#289555));
#289555=SURFACE_STYLE_USAGE(.BOTH.,#289562);
#289562=SURFACE_SIDE_STYLE('',(#289569));
#289569=SURFACE_STYLE_FILL_AREA(#289576);
#289576=FILL_AREA_STYLE('Opaque(104,114,127)',(#289583));
#289583=FILL_AREA_STYLE_COLOUR('Opaque(104,114,127)',#289590);
#289590=COLOUR_RGB('Opaque(104,114,127)',0.407843137254902,0.447058823529412,
0.498039215686275);
ENDSEC;
END-ISO-10303-21;
